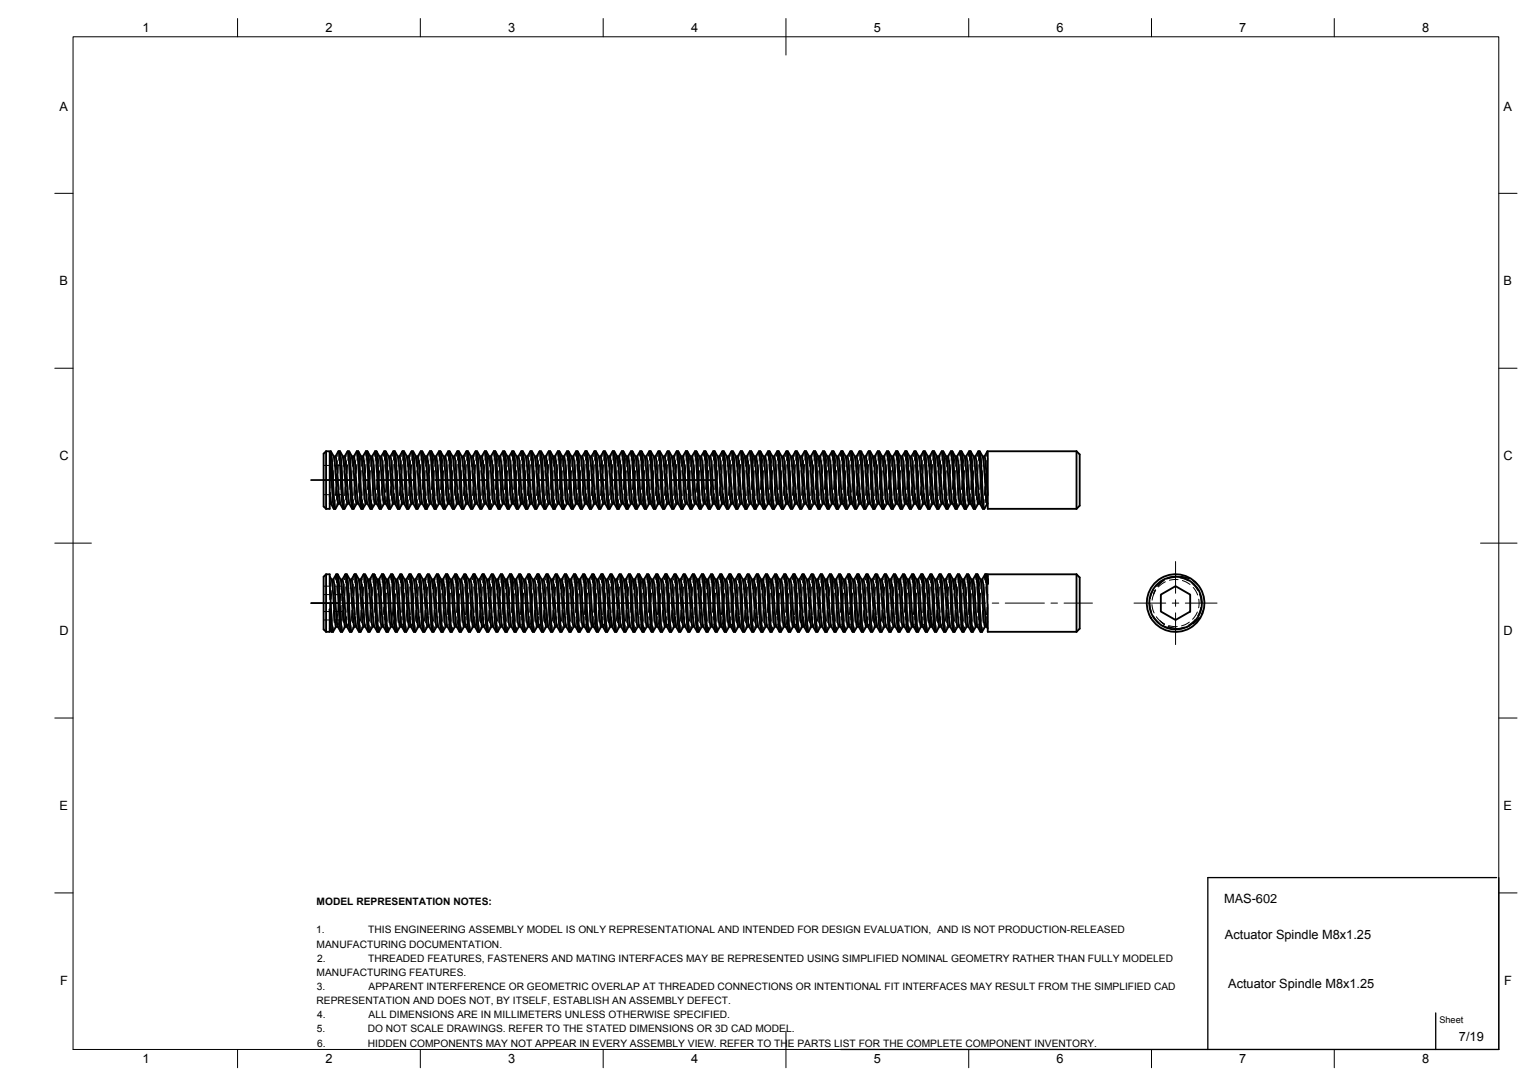
ISO-10303-21;
HEADER;
/* Generated by software containing ST-Developer
 * from STEP Tools, Inc. (www.steptools.com) 
 */

FILE_DESCRIPTION(
/* description */ (''),
/* implementation_level */ '2;1');

FILE_NAME(
/* name */ 'Actuator Spindle M8x1.25.step',
/* time_stamp */ '2026-10-15T14:42:47-07:00',
/* author */ (''),
/* organization */ (''),
/* preprocessor_version */ 'ST-DEVELOPER v20.2',
/* originating_system */ 'Autodesk Translation Framework v15.15.0.0',
/* authorisation */ '');

FILE_SCHEMA (('AUTOMOTIVE_DESIGN { 1 0 10303 214 3 1 1 }'));
ENDSEC;

DATA;
#10=MECHANICAL_DESIGN_GEOMETRIC_PRESENTATION_REPRESENTATION('',(#238),#85789);
#163=CONICAL_SURFACE('',#10500,0.375,0.785398163397451);
#164=CONICAL_SURFACE('',#10501,0.38,0.785398163397437);
#202=SHAPE_REPRESENTATION_RELATIONSHIP('SRR','None',#85867,#220);
#220=ADVANCED_BREP_SHAPE_REPRESENTATION('',(#256),#85775);
#238=STYLED_ITEM('',(#85966),#256);
#256=MANIFOLD_SOLID_BREP('Body1',#9885);
#381=B_SPLINE_SURFACE_WITH_KNOTS('',3,3,((#71919,#71920,#71921,#71922,#71923,
#71924,#71925,#71926,#71927,#71928,#71929,#71930,#71931,#71932,#71933,#71934,
#71935,#71936,#71937,#71938,#71939,#71940,#71941,#71942,#71943,#71944,#71945,
#71946,#71947,#71948,#71949,#71950,#71951,#71952,#71953,#71954,#71955,#71956,
#71957,#71958,#71959,#71960,#71961,#71962,#71963,#71964,#71965,#71966,#71967,
#71968,#71969,#71970,#71971,#71972,#71973,#71974,#71975,#71976,#71977,#71978,
#71979,#71980,#71981,#71982,#71983,#71984,#71985,#71986,#71987,#71988,#71989,
#71990,#71991,#71992,#71993,#71994,#71995,#71996,#71997,#71998,#71999,#72000,
#72001,#72002,#72003,#72004,#72005,#72006,#72007,#72008,#72009,#72010,#72011,
#72012,#72013,#72014,#72015,#72016,#72017,#72018,#72019,#72020,#72021,#72022,
#72023,#72024,#72025,#72026,#72027,#72028,#72029,#72030,#72031,#72032,#72033,
#72034,#72035,#72036,#72037,#72038,#72039,#72040,#72041,#72042,#72043,#72044,
#72045,#72046,#72047,#72048,#72049,#72050,#72051,#72052,#72053,#72054,#72055,
#72056,#72057,#72058,#72059,#72060,#72061,#72062,#72063,#72064,#72065,#72066,
#72067,#72068,#72069,#72070,#72071,#72072,#72073,#72074,#72075,#72076,#72077,
#72078,#72079,#72080,#72081,#72082,#72083,#72084,#72085,#72086,#72087,#72088,
#72089,#72090,#72091,#72092,#72093,#72094,#72095,#72096,#72097,#72098,#72099,
#72100,#72101,#72102,#72103,#72104,#72105,#72106,#72107,#72108,#72109,#72110,
#72111,#72112,#72113,#72114,#72115,#72116,#72117,#72118,#72119,#72120,#72121,
#72122,#72123,#72124,#72125,#72126,#72127,#72128,#72129,#72130,#72131,#72132,
#72133,#72134,#72135,#72136,#72137,#72138,#72139,#72140,#72141,#72142,#72143,
#72144,#72145,#72146,#72147,#72148,#72149,#72150,#72151,#72152,#72153,#72154,
#72155,#72156,#72157,#72158,#72159,#72160,#72161,#72162,#72163,#72164,#72165,
#72166,#72167,#72168,#72169,#72170,#72171,#72172,#72173,#72174,#72175,#72176,
#72177,#72178,#72179,#72180,#72181,#72182,#72183,#72184,#72185,#72186,#72187,
#72188,#72189,#72190,#72191,#72192,#72193,#72194,#72195,#72196,#72197,#72198,
#72199,#72200,#72201,#72202,#72203,#72204,#72205,#72206,#72207,#72208,#72209,
#72210,#72211,#72212,#72213,#72214,#72215,#72216,#72217,#72218,#72219,#72220,
#72221,#72222,#72223,#72224,#72225,#72226,#72227,#72228,#72229,#72230,#72231,
#72232,#72233,#72234,#72235,#72236,#72237,#72238,#72239,#72240,#72241,#72242,
#72243,#72244,#72245,#72246,#72247,#72248,#72249,#72250,#72251,#72252,#72253,
#72254,#72255,#72256,#72257,#72258,#72259,#72260,#72261,#72262,#72263,#72264,
#72265,#72266,#72267,#72268,#72269,#72270,#72271,#72272,#72273,#72274,#72275,
#72276,#72277,#72278,#72279,#72280,#72281,#72282,#72283,#72284,#72285,#72286,
#72287,#72288,#72289,#72290,#72291,#72292,#72293,#72294,#72295,#72296,#72297,
#72298,#72299,#72300,#72301,#72302,#72303,#72304,#72305,#72306,#72307,#72308,
#72309,#72310,#72311,#72312,#72313,#72314,#72315,#72316,#72317,#72318,#72319,
#72320,#72321,#72322,#72323,#72324,#72325,#72326,#72327,#72328,#72329,#72330,
#72331,#72332,#72333,#72334,#72335,#72336,#72337,#72338,#72339,#72340,#72341,
#72342,#72343,#72344,#72345,#72346,#72347,#72348,#72349,#72350,#72351,#72352,
#72353,#72354,#72355,#72356,#72357,#72358,#72359,#72360,#72361,#72362,#72363,
#72364,#72365,#72366,#72367,#72368,#72369,#72370,#72371,#72372,#72373,#72374,
#72375,#72376),(#72377,#72378,#72379,#72380,#72381,#72382,#72383,#72384,
#72385,#72386,#72387,#72388,#72389,#72390,#72391,#72392,#72393,#72394,#72395,
#72396,#72397,#72398,#72399,#72400,#72401,#72402,#72403,#72404,#72405,#72406,
#72407,#72408,#72409,#72410,#72411,#72412,#72413,#72414,#72415,#72416,#72417,
#72418,#72419,#72420,#72421,#72422,#72423,#72424,#72425,#72426,#72427,#72428,
#72429,#72430,#72431,#72432,#72433,#72434,#72435,#72436,#72437,#72438,#72439,
#72440,#72441,#72442,#72443,#72444,#72445,#72446,#72447,#72448,#72449,#72450,
#72451,#72452,#72453,#72454,#72455,#72456,#72457,#72458,#72459,#72460,#72461,
#72462,#72463,#72464,#72465,#72466,#72467,#72468,#72469,#72470,#72471,#72472,
#72473,#72474,#72475,#72476,#72477,#72478,#72479,#72480,#72481,#72482,#72483,
#72484,#72485,#72486,#72487,#72488,#72489,#72490,#72491,#72492,#72493,#72494,
#72495,#72496,#72497,#72498,#72499,#72500,#72501,#72502,#72503,#72504,#72505,
#72506,#72507,#72508,#72509,#72510,#72511,#72512,#72513,#72514,#72515,#72516,
#72517,#72518,#72519,#72520,#72521,#72522,#72523,#72524,#72525,#72526,#72527,
#72528,#72529,#72530,#72531,#72532,#72533,#72534,#72535,#72536,#72537,#72538,
#72539,#72540,#72541,#72542,#72543,#72544,#72545,#72546,#72547,#72548,#72549,
#72550,#72551,#72552,#72553,#72554,#72555,#72556,#72557,#72558,#72559,#72560,
#72561,#72562,#72563,#72564,#72565,#72566,#72567,#72568,#72569,#72570,#72571,
#72572,#72573,#72574,#72575,#72576,#72577,#72578,#72579,#72580,#72581,#72582,
#72583,#72584,#72585,#72586,#72587,#72588,#72589,#72590,#72591,#72592,#72593,
#72594,#72595,#72596,#72597,#72598,#72599,#72600,#72601,#72602,#72603,#72604,
#72605,#72606,#72607,#72608,#72609,#72610,#72611,#72612,#72613,#72614,#72615,
#72616,#72617,#72618,#72619,#72620,#72621,#72622,#72623,#72624,#72625,#72626,
#72627,#72628,#72629,#72630,#72631,#72632,#72633,#72634,#72635,#72636,#72637,
#72638,#72639,#72640,#72641,#72642,#72643,#72644,#72645,#72646,#72647,#72648,
#72649,#72650,#72651,#72652,#72653,#72654,#72655,#72656,#72657,#72658,#72659,
#72660,#72661,#72662,#72663,#72664,#72665,#72666,#72667,#72668,#72669,#72670,
#72671,#72672,#72673,#72674,#72675,#72676,#72677,#72678,#72679,#72680,#72681,
#72682,#72683,#72684,#72685,#72686,#72687,#72688,#72689,#72690,#72691,#72692,
#72693,#72694,#72695,#72696,#72697,#72698,#72699,#72700,#72701,#72702,#72703,
#72704,#72705,#72706,#72707,#72708,#72709,#72710,#72711,#72712,#72713,#72714,
#72715,#72716,#72717,#72718,#72719,#72720,#72721,#72722,#72723,#72724,#72725,
#72726,#72727,#72728,#72729,#72730,#72731,#72732,#72733,#72734,#72735,#72736,
#72737,#72738,#72739,#72740,#72741,#72742,#72743,#72744,#72745,#72746,#72747,
#72748,#72749,#72750,#72751,#72752,#72753,#72754,#72755,#72756,#72757,#72758,
#72759,#72760,#72761,#72762,#72763,#72764,#72765,#72766,#72767,#72768,#72769,
#72770,#72771,#72772,#72773,#72774,#72775,#72776,#72777,#72778,#72779,#72780,
#72781,#72782,#72783,#72784,#72785,#72786,#72787,#72788,#72789,#72790,#72791,
#72792,#72793,#72794,#72795,#72796,#72797,#72798,#72799,#72800,#72801,#72802,
#72803,#72804,#72805,#72806,#72807,#72808,#72809,#72810,#72811,#72812,#72813,
#72814,#72815,#72816,#72817,#72818,#72819,#72820,#72821,#72822,#72823,#72824,
#72825,#72826,#72827,#72828,#72829,#72830,#72831,#72832,#72833,#72834),
(#72835,#72836,#72837,#72838,#72839,#72840,#72841,#72842,#72843,#72844,
#72845,#72846,#72847,#72848,#72849,#72850,#72851,#72852,#72853,#72854,#72855,
#72856,#72857,#72858,#72859,#72860,#72861,#72862,#72863,#72864,#72865,#72866,
#72867,#72868,#72869,#72870,#72871,#72872,#72873,#72874,#72875,#72876,#72877,
#72878,#72879,#72880,#72881,#72882,#72883,#72884,#72885,#72886,#72887,#72888,
#72889,#72890,#72891,#72892,#72893,#72894,#72895,#72896,#72897,#72898,#72899,
#72900,#72901,#72902,#72903,#72904,#72905,#72906,#72907,#72908,#72909,#72910,
#72911,#72912,#72913,#72914,#72915,#72916,#72917,#72918,#72919,#72920,#72921,
#72922,#72923,#72924,#72925,#72926,#72927,#72928,#72929,#72930,#72931,#72932,
#72933,#72934,#72935,#72936,#72937,#72938,#72939,#72940,#72941,#72942,#72943,
#72944,#72945,#72946,#72947,#72948,#72949,#72950,#72951,#72952,#72953,#72954,
#72955,#72956,#72957,#72958,#72959,#72960,#72961,#72962,#72963,#72964,#72965,
#72966,#72967,#72968,#72969,#72970,#72971,#72972,#72973,#72974,#72975,#72976,
#72977,#72978,#72979,#72980,#72981,#72982,#72983,#72984,#72985,#72986,#72987,
#72988,#72989,#72990,#72991,#72992,#72993,#72994,#72995,#72996,#72997,#72998,
#72999,#73000,#73001,#73002,#73003,#73004,#73005,#73006,#73007,#73008,#73009,
#73010,#73011,#73012,#73013,#73014,#73015,#73016,#73017,#73018,#73019,#73020,
#73021,#73022,#73023,#73024,#73025,#73026,#73027,#73028,#73029,#73030,#73031,
#73032,#73033,#73034,#73035,#73036,#73037,#73038,#73039,#73040,#73041,#73042,
#73043,#73044,#73045,#73046,#73047,#73048,#73049,#73050,#73051,#73052,#73053,
#73054,#73055,#73056,#73057,#73058,#73059,#73060,#73061,#73062,#73063,#73064,
#73065,#73066,#73067,#73068,#73069,#73070,#73071,#73072,#73073,#73074,#73075,
#73076,#73077,#73078,#73079,#73080,#73081,#73082,#73083,#73084,#73085,#73086,
#73087,#73088,#73089,#73090,#73091,#73092,#73093,#73094,#73095,#73096,#73097,
#73098,#73099,#73100,#73101,#73102,#73103,#73104,#73105,#73106,#73107,#73108,
#73109,#73110,#73111,#73112,#73113,#73114,#73115,#73116,#73117,#73118,#73119,
#73120,#73121,#73122,#73123,#73124,#73125,#73126,#73127,#73128,#73129,#73130,
#73131,#73132,#73133,#73134,#73135,#73136,#73137,#73138,#73139,#73140,#73141,
#73142,#73143,#73144,#73145,#73146,#73147,#73148,#73149,#73150,#73151,#73152,
#73153,#73154,#73155,#73156,#73157,#73158,#73159,#73160,#73161,#73162,#73163,
#73164,#73165,#73166,#73167,#73168,#73169,#73170,#73171,#73172,#73173,#73174,
#73175,#73176,#73177,#73178,#73179,#73180,#73181,#73182,#73183,#73184,#73185,
#73186,#73187,#73188,#73189,#73190,#73191,#73192,#73193,#73194,#73195,#73196,
#73197,#73198,#73199,#73200,#73201,#73202,#73203,#73204,#73205,#73206,#73207,
#73208,#73209,#73210,#73211,#73212,#73213,#73214,#73215,#73216,#73217,#73218,
#73219,#73220,#73221,#73222,#73223,#73224,#73225,#73226,#73227,#73228,#73229,
#73230,#73231,#73232,#73233,#73234,#73235,#73236,#73237,#73238,#73239,#73240,
#73241,#73242,#73243,#73244,#73245,#73246,#73247,#73248,#73249,#73250,#73251,
#73252,#73253,#73254,#73255,#73256,#73257,#73258,#73259,#73260,#73261,#73262,
#73263,#73264,#73265,#73266,#73267,#73268,#73269,#73270,#73271,#73272,#73273,
#73274,#73275,#73276,#73277,#73278,#73279,#73280,#73281,#73282,#73283,#73284,
#73285,#73286,#73287,#73288,#73289,#73290,#73291,#73292),(#73293,#73294,
#73295,#73296,#73297,#73298,#73299,#73300,#73301,#73302,#73303,#73304,#73305,
#73306,#73307,#73308,#73309,#73310,#73311,#73312,#73313,#73314,#73315,#73316,
#73317,#73318,#73319,#73320,#73321,#73322,#73323,#73324,#73325,#73326,#73327,
#73328,#73329,#73330,#73331,#73332,#73333,#73334,#73335,#73336,#73337,#73338,
#73339,#73340,#73341,#73342,#73343,#73344,#73345,#73346,#73347,#73348,#73349,
#73350,#73351,#73352,#73353,#73354,#73355,#73356,#73357,#73358,#73359,#73360,
#73361,#73362,#73363,#73364,#73365,#73366,#73367,#73368,#73369,#73370,#73371,
#73372,#73373,#73374,#73375,#73376,#73377,#73378,#73379,#73380,#73381,#73382,
#73383,#73384,#73385,#73386,#73387,#73388,#73389,#73390,#73391,#73392,#73393,
#73394,#73395,#73396,#73397,#73398,#73399,#73400,#73401,#73402,#73403,#73404,
#73405,#73406,#73407,#73408,#73409,#73410,#73411,#73412,#73413,#73414,#73415,
#73416,#73417,#73418,#73419,#73420,#73421,#73422,#73423,#73424,#73425,#73426,
#73427,#73428,#73429,#73430,#73431,#73432,#73433,#73434,#73435,#73436,#73437,
#73438,#73439,#73440,#73441,#73442,#73443,#73444,#73445,#73446,#73447,#73448,
#73449,#73450,#73451,#73452,#73453,#73454,#73455,#73456,#73457,#73458,#73459,
#73460,#73461,#73462,#73463,#73464,#73465,#73466,#73467,#73468,#73469,#73470,
#73471,#73472,#73473,#73474,#73475,#73476,#73477,#73478,#73479,#73480,#73481,
#73482,#73483,#73484,#73485,#73486,#73487,#73488,#73489,#73490,#73491,#73492,
#73493,#73494,#73495,#73496,#73497,#73498,#73499,#73500,#73501,#73502,#73503,
#73504,#73505,#73506,#73507,#73508,#73509,#73510,#73511,#73512,#73513,#73514,
#73515,#73516,#73517,#73518,#73519,#73520,#73521,#73522,#73523,#73524,#73525,
#73526,#73527,#73528,#73529,#73530,#73531,#73532,#73533,#73534,#73535,#73536,
#73537,#73538,#73539,#73540,#73541,#73542,#73543,#73544,#73545,#73546,#73547,
#73548,#73549,#73550,#73551,#73552,#73553,#73554,#73555,#73556,#73557,#73558,
#73559,#73560,#73561,#73562,#73563,#73564,#73565,#73566,#73567,#73568,#73569,
#73570,#73571,#73572,#73573,#73574,#73575,#73576,#73577,#73578,#73579,#73580,
#73581,#73582,#73583,#73584,#73585,#73586,#73587,#73588,#73589,#73590,#73591,
#73592,#73593,#73594,#73595,#73596,#73597,#73598,#73599,#73600,#73601,#73602,
#73603,#73604,#73605,#73606,#73607,#73608,#73609,#73610,#73611,#73612,#73613,
#73614,#73615,#73616,#73617,#73618,#73619,#73620,#73621,#73622,#73623,#73624,
#73625,#73626,#73627,#73628,#73629,#73630,#73631,#73632,#73633,#73634,#73635,
#73636,#73637,#73638,#73639,#73640,#73641,#73642,#73643,#73644,#73645,#73646,
#73647,#73648,#73649,#73650,#73651,#73652,#73653,#73654,#73655,#73656,#73657,
#73658,#73659,#73660,#73661,#73662,#73663,#73664,#73665,#73666,#73667,#73668,
#73669,#73670,#73671,#73672,#73673,#73674,#73675,#73676,#73677,#73678,#73679,
#73680,#73681,#73682,#73683,#73684,#73685,#73686,#73687,#73688,#73689,#73690,
#73691,#73692,#73693,#73694,#73695,#73696,#73697,#73698,#73699,#73700,#73701,
#73702,#73703,#73704,#73705,#73706,#73707,#73708,#73709,#73710,#73711,#73712,
#73713,#73714,#73715,#73716,#73717,#73718,#73719,#73720,#73721,#73722,#73723,
#73724,#73725,#73726,#73727,#73728,#73729,#73730,#73731,#73732,#73733,#73734,
#73735,#73736,#73737,#73738,#73739,#73740,#73741,#73742,#73743,#73744,#73745,
#73746,#73747,#73748,#73749,#73750)),.UNSPECIFIED.,.F.,.F.,.F.,(4,4),(4,
1,1,1,1,1,1,1,1,1,1,1,1,1,1,1,1,1,1,1,1,1,1,1,1,1,1,1,1,1,1,1,1,1,1,1,1,
1,1,1,1,1,1,1,1,1,1,1,1,1,1,1,1,1,1,1,1,1,1,1,1,1,1,1,1,1,1,1,1,1,1,1,1,
1,1,1,1,1,1,1,1,1,1,1,1,1,1,1,1,1,1,1,1,1,1,1,1,1,1,1,1,1,1,1,1,1,1,1,1,
1,1,1,1,1,1,1,1,1,1,1,1,1,1,1,1,1,1,1,1,1,1,1,1,1,1,1,1,1,1,1,1,1,1,1,1,
1,1,1,1,1,1,1,1,1,1,1,1,1,1,1,1,1,1,1,1,1,1,1,1,1,1,1,1,1,1,1,1,1,1,1,1,
1,1,1,1,1,1,1,1,1,1,1,1,1,1,1,1,1,1,1,1,1,1,1,1,1,1,1,1,1,1,1,1,1,1,1,1,
1,1,1,1,1,1,1,1,1,1,1,1,1,1,1,1,1,1,1,1,1,1,1,1,1,1,1,1,1,1,1,1,1,1,1,1,
1,1,1,1,1,1,1,1,1,1,1,1,1,1,1,1,1,1,1,1,1,1,1,1,1,1,1,1,1,1,1,1,1,1,1,1,
1,1,1,1,1,1,1,1,1,1,1,1,1,1,1,1,1,1,1,1,1,1,1,1,1,1,1,1,1,1,1,1,1,1,1,1,
1,1,1,1,1,1,1,1,1,1,1,1,1,1,1,1,1,1,1,1,1,1,1,1,1,1,1,1,1,1,1,1,1,1,1,1,
1,1,1,1,1,1,1,1,1,1,1,1,1,1,1,1,1,1,1,1,1,1,1,1,1,1,1,1,1,1,1,1,1,1,1,1,
1,1,1,1,1,1,1,1,1,1,1,1,1,1,1,1,1,1,1,1,1,1,1,1,1,1,1,1,1,1,1,1,1,1,1,1,
1,1,1,1,1,1,1,1,1,1,1,1,1,1,1,1,1,1,1,1,1,1,4),(-0.000668976878624835,0.0823370872655779),
(12.7582013990964,13.7569938028644,14.7557862066324,15.7545786104004,16.7533710141684,
17.7521634179365,18.7509558217045,19.7497482254725,20.7485406292405,21.7473330330085,
22.7461254367765,23.7449178405445,24.7437102443125,25.7425026480806,26.7412950518486,
27.7400874556166,28.7388798593846,29.7376722631526,30.7364646669206,31.7352570706886,
32.7340494744567,33.7328418782247,34.7316342819927,35.7304266857607,36.7292190895287,
37.7280114932967,38.7268038970647,39.7255963008328,40.7243887046008,41.7231811083688,
42.7219735121368,43.7207659159048,44.7195583196728,45.7183507234408,46.7171431272089,
47.7159355309769,48.7147279347449,49.7135203385129,50.7123127422809,51.7111051460489,
52.7098975498169,53.708689953585,54.707482357353,55.706274761121,56.705067164889,
57.703859568657,58.702651972425,59.701444376193,60.700236779961,61.6990291837291,
62.6978215874971,63.6966139912651,64.6954063950331,65.6941987988011,66.6929912025691,
67.6917836063371,68.6905760101052,69.6893684138732,70.6881608176412,71.6869532214092,
72.6857456251772,73.6845380289452,74.6833304327132,75.6821228364813,76.6809152402493,
77.6797076440173,78.6785000477853,79.6772924515533,80.6760848553213,81.6748772590893,
82.6736696628573,83.6724620666254,84.6712544703934,85.6700468741614,86.6688392779294,
87.6676316816974,88.6664240854654,89.6652164892334,90.6640088930015,91.6628012967695,
92.6615937005375,93.6603861043055,94.6591785080735,95.6579709118415,96.6567633156095,
97.6555557193776,98.6543481231456,99.6531405269136,100.651932930682,101.65072533445,
102.649517738218,103.648310141986,104.647102545754,105.645894949522,106.64468735329,
107.643479757058,108.642272160826,109.641064564594,110.639856968362,111.63864937213,
112.637441775898,113.636234179666,114.635026583434,115.633818987202,116.63261139097,
117.631403794738,118.630196198506,119.628988602274,120.627781006042,121.62657340981,
122.625365813578,123.624158217346,124.622950621114,125.621743024882,126.62053542865,
127.619327832418,128.618120236186,129.616912639954,130.615705043722,131.61449744749,
132.613289851258,133.612082255026,134.610874658794,135.609667062562,136.60845946633,
137.607251870098,138.606044273866,139.604836677634,140.603629081402,141.60242148517,
142.601213888938,143.600006292706,144.598798696474,145.597591100242,146.59638350401,
147.595175907778,148.593968311546,149.592760715314,150.591553119082,151.59034552285,
152.589137926618,153.587930330386,154.586722734154,155.585515137922,156.58430754169,
157.583099945458,158.581892349226,159.580684752994,160.579477156762,161.57826956053,
162.577061964298,163.575854368066,164.574646771834,165.573439175602,166.572231579371,
167.571023983139,168.569816386907,169.568608790675,170.567401194443,171.566193598211,
172.564986001979,173.563778405747,174.562570809515,175.561363213283,176.560155617051,
177.558948020819,178.557740424587,179.556532828355,180.555325232123,181.554117635891,
182.552910039659,183.551702443427,184.550494847195,185.549287250963,186.548079654731,
187.546872058499,188.545664462267,189.544456866035,190.543249269803,191.542041673571,
192.540834077339,193.539626481107,194.538418884875,195.537211288643,196.536003692411,
197.534796096179,198.533588499947,199.532380903715,200.531173307483,201.529965711251,
202.528758115019,203.527550518787,204.526342922555,205.525135326323,206.523927730091,
207.522720133859,208.521512537627,209.520304941395,210.519097345163,211.517889748931,
212.516682152699,213.515474556467,214.514266960235,215.513059364003,216.511851767771,
217.510644171539,218.509436575307,219.508228979075,220.507021382843,221.505813786611,
222.504606190379,223.503398594147,224.502190997915,225.500983401683,226.499775805451,
227.498568209219,228.497360612987,229.496153016755,230.494945420523,231.493737824291,
232.492530228059,233.491322631827,234.490115035595,235.488907439363,236.487699843131,
237.486492246899,238.485284650667,239.484077054436,240.482869458204,241.481661861972,
242.48045426574,243.479246669508,244.478039073276,245.476831477044,246.475623880812,
247.47441628458,248.473208688348,249.472001092116,250.470793495884,251.469585899652,
252.46837830342,253.467170707188,254.465963110956,255.464755514724,256.463547918492,
257.46234032226,258.461132726028,259.459925129796,260.458717533564,261.457509937332,
262.4563023411,263.455094744868,264.453887148636,265.452679552404,266.451471956172,
267.45026435994,268.449056763708,269.447849167476,270.446641571244,271.445433975012,
272.44422637878,273.443018782548,274.441811186316,275.440603590084,276.439395993852,
277.43818839762,278.436980801388,279.435773205156,280.434565608924,281.433358012692,
282.43215041646,283.430942820228,284.429735223996,285.428527627764,286.427320031532,
287.4261124353,288.424904839068,289.423697242836,290.422489646604,291.421282050372,
292.42007445414,293.418866857908,294.417659261676,295.416451665444,296.415244069212,
297.41403647298,298.412828876748,299.411621280516,300.410413684284,301.409206088052,
302.40799849182,303.406790895588,304.405583299356,305.404375703124,306.403168106892,
307.40196051066,308.400752914428,309.399545318196,310.398337721964,311.397130125733,
312.395922529501,313.394714933269,314.393507337037,315.392299740805,316.391092144573,
317.389884548341,318.388676952109,319.387469355877,320.386261759645,321.385054163413,
322.383846567181,323.382638970949,324.381431374717,325.380223778485,326.379016182253,
327.377808586021,328.376600989789,329.375393393557,330.374185797325,331.372978201093,
332.371770604861,333.370563008629,334.369355412397,335.368147816165,336.366940219933,
337.365732623701,338.364525027469,339.363317431237,340.362109835005,341.360902238773,
342.359694642541,343.358487046309,344.357279450077,345.356071853845,346.354864257613,
347.353656661381,348.352449065149,349.351241468917,350.350033872685,351.348826276453,
352.347618680221,353.346411083989,354.345203487757,355.343995891525,356.342788295293,
357.341580699061,358.340373102829,359.339165506597,360.337957910365,361.336750314133,
362.335542717901,363.334335121669,364.333127525437,365.331919929205,366.330712332973,
367.329504736741,368.328297140509,369.327089544277,370.325881948045,371.324674351813,
372.323466755581,373.322259159349,374.321051563117,375.319843966885,376.318636370653,
377.317428774421,378.316221178189,379.315013581957,380.313805985725,381.312598389493,
382.311390793261,383.31018319703,384.308975600798,385.307768004566,386.306560408334,
387.305352812102,388.30414521587,389.302937619638,390.301730023406,391.300522427174,
392.299314830942,393.29810723471,394.296899638478,395.295692042246,396.294484446014,
397.293276849782,398.29206925355,399.290861657318,400.289654061086,401.288446464854,
402.287238868622,403.28603127239,404.284823676158,405.283616079926,406.282408483694,
407.281200887462,408.27999329123,409.278785694998,410.277578098766,411.276370502534,
412.275162906302,413.27395531007,414.272747713838,415.271540117606,416.270332521374,
417.269124925142,418.26791732891,419.266709732678,420.265502136446,421.264294540214,
422.263086943982,423.26187934775,424.260671751518,425.259464155286,426.258256559054,
427.257048962822,428.25584136659,429.254633770358,430.253426174126,431.252218577894,
432.251010981662,433.24980338543,434.248595789198,435.247388192966,436.246180596734,
437.244973000502,438.24376540427,439.242557808038,440.241350211806,441.240142615574,
442.238935019342,443.23772742311,444.236519826878,445.235312230646,446.234104634414,
447.232897038182,448.23168944195,449.230481845718,450.229274249486,451.228066653254,
452.226859057022,453.22565146079,454.224443864559,455.223236268327,456.222028672094,
457.220821075863,458.219613479631,459.218405883399,460.217198287167,461.215990690935,
462.214783094703,463.213575498471,464.212367902239,465.211160306007,466.209952709775,
467.209414090422),.UNSPECIFIED.);
#382=B_SPLINE_SURFACE_WITH_KNOTS('',3,3,((#73883,#73884,#73885,#73886,#73887,
#73888,#73889,#73890,#73891,#73892,#73893,#73894,#73895,#73896,#73897,#73898,
#73899,#73900,#73901,#73902,#73903,#73904,#73905,#73906,#73907,#73908,#73909,
#73910,#73911,#73912,#73913,#73914,#73915,#73916,#73917,#73918,#73919,#73920,
#73921,#73922,#73923,#73924,#73925,#73926,#73927,#73928,#73929,#73930,#73931,
#73932,#73933,#73934,#73935,#73936,#73937,#73938,#73939,#73940,#73941,#73942,
#73943,#73944,#73945,#73946,#73947,#73948,#73949,#73950,#73951,#73952,#73953,
#73954,#73955,#73956,#73957,#73958,#73959,#73960,#73961,#73962,#73963,#73964,
#73965,#73966,#73967,#73968,#73969,#73970,#73971,#73972,#73973,#73974,#73975,
#73976,#73977,#73978,#73979,#73980,#73981,#73982,#73983,#73984,#73985,#73986,
#73987,#73988,#73989,#73990,#73991,#73992,#73993,#73994,#73995,#73996,#73997,
#73998,#73999,#74000,#74001,#74002,#74003,#74004,#74005,#74006,#74007,#74008,
#74009,#74010,#74011,#74012,#74013,#74014,#74015,#74016,#74017,#74018,#74019,
#74020,#74021,#74022,#74023,#74024,#74025,#74026,#74027,#74028,#74029,#74030,
#74031,#74032,#74033,#74034,#74035,#74036,#74037,#74038,#74039,#74040,#74041,
#74042,#74043,#74044,#74045,#74046,#74047,#74048,#74049,#74050,#74051,#74052,
#74053,#74054,#74055,#74056,#74057,#74058,#74059,#74060,#74061,#74062,#74063,
#74064,#74065,#74066,#74067,#74068,#74069,#74070,#74071,#74072,#74073,#74074,
#74075,#74076,#74077,#74078,#74079,#74080,#74081,#74082,#74083,#74084,#74085,
#74086,#74087,#74088,#74089,#74090,#74091,#74092,#74093,#74094,#74095,#74096,
#74097,#74098,#74099,#74100,#74101,#74102,#74103,#74104,#74105,#74106,#74107,
#74108,#74109,#74110,#74111,#74112,#74113,#74114,#74115,#74116,#74117,#74118,
#74119,#74120,#74121,#74122,#74123,#74124,#74125,#74126,#74127,#74128,#74129,
#74130,#74131,#74132,#74133,#74134,#74135,#74136,#74137,#74138,#74139,#74140,
#74141,#74142,#74143,#74144,#74145,#74146,#74147,#74148,#74149,#74150,#74151,
#74152,#74153,#74154,#74155,#74156,#74157,#74158,#74159,#74160,#74161,#74162,
#74163,#74164,#74165,#74166,#74167,#74168,#74169,#74170,#74171,#74172,#74173,
#74174,#74175,#74176,#74177,#74178,#74179,#74180,#74181,#74182,#74183,#74184,
#74185,#74186,#74187,#74188,#74189,#74190,#74191,#74192,#74193,#74194,#74195,
#74196,#74197,#74198,#74199,#74200,#74201,#74202,#74203,#74204,#74205,#74206,
#74207,#74208,#74209,#74210,#74211,#74212,#74213,#74214,#74215,#74216,#74217,
#74218,#74219,#74220,#74221,#74222,#74223,#74224,#74225,#74226,#74227,#74228,
#74229,#74230,#74231,#74232,#74233,#74234,#74235,#74236,#74237,#74238,#74239,
#74240,#74241,#74242,#74243,#74244,#74245,#74246,#74247,#74248,#74249,#74250,
#74251,#74252,#74253,#74254,#74255,#74256,#74257,#74258,#74259,#74260,#74261,
#74262,#74263,#74264,#74265,#74266,#74267,#74268,#74269,#74270,#74271,#74272,
#74273,#74274,#74275,#74276,#74277,#74278,#74279,#74280,#74281,#74282,#74283,
#74284,#74285,#74286,#74287,#74288,#74289,#74290,#74291,#74292,#74293,#74294,
#74295,#74296,#74297,#74298,#74299,#74300,#74301,#74302,#74303,#74304,#74305,
#74306,#74307,#74308,#74309,#74310,#74311,#74312,#74313,#74314,#74315,#74316,
#74317,#74318,#74319,#74320,#74321,#74322,#74323,#74324,#74325,#74326,#74327,
#74328,#74329,#74330,#74331,#74332,#74333,#74334,#74335,#74336,#74337,#74338,
#74339,#74340),(#74341,#74342,#74343,#74344,#74345,#74346,#74347,#74348,
#74349,#74350,#74351,#74352,#74353,#74354,#74355,#74356,#74357,#74358,#74359,
#74360,#74361,#74362,#74363,#74364,#74365,#74366,#74367,#74368,#74369,#74370,
#74371,#74372,#74373,#74374,#74375,#74376,#74377,#74378,#74379,#74380,#74381,
#74382,#74383,#74384,#74385,#74386,#74387,#74388,#74389,#74390,#74391,#74392,
#74393,#74394,#74395,#74396,#74397,#74398,#74399,#74400,#74401,#74402,#74403,
#74404,#74405,#74406,#74407,#74408,#74409,#74410,#74411,#74412,#74413,#74414,
#74415,#74416,#74417,#74418,#74419,#74420,#74421,#74422,#74423,#74424,#74425,
#74426,#74427,#74428,#74429,#74430,#74431,#74432,#74433,#74434,#74435,#74436,
#74437,#74438,#74439,#74440,#74441,#74442,#74443,#74444,#74445,#74446,#74447,
#74448,#74449,#74450,#74451,#74452,#74453,#74454,#74455,#74456,#74457,#74458,
#74459,#74460,#74461,#74462,#74463,#74464,#74465,#74466,#74467,#74468,#74469,
#74470,#74471,#74472,#74473,#74474,#74475,#74476,#74477,#74478,#74479,#74480,
#74481,#74482,#74483,#74484,#74485,#74486,#74487,#74488,#74489,#74490,#74491,
#74492,#74493,#74494,#74495,#74496,#74497,#74498,#74499,#74500,#74501,#74502,
#74503,#74504,#74505,#74506,#74507,#74508,#74509,#74510,#74511,#74512,#74513,
#74514,#74515,#74516,#74517,#74518,#74519,#74520,#74521,#74522,#74523,#74524,
#74525,#74526,#74527,#74528,#74529,#74530,#74531,#74532,#74533,#74534,#74535,
#74536,#74537,#74538,#74539,#74540,#74541,#74542,#74543,#74544,#74545,#74546,
#74547,#74548,#74549,#74550,#74551,#74552,#74553,#74554,#74555,#74556,#74557,
#74558,#74559,#74560,#74561,#74562,#74563,#74564,#74565,#74566,#74567,#74568,
#74569,#74570,#74571,#74572,#74573,#74574,#74575,#74576,#74577,#74578,#74579,
#74580,#74581,#74582,#74583,#74584,#74585,#74586,#74587,#74588,#74589,#74590,
#74591,#74592,#74593,#74594,#74595,#74596,#74597,#74598,#74599,#74600,#74601,
#74602,#74603,#74604,#74605,#74606,#74607,#74608,#74609,#74610,#74611,#74612,
#74613,#74614,#74615,#74616,#74617,#74618,#74619,#74620,#74621,#74622,#74623,
#74624,#74625,#74626,#74627,#74628,#74629,#74630,#74631,#74632,#74633,#74634,
#74635,#74636,#74637,#74638,#74639,#74640,#74641,#74642,#74643,#74644,#74645,
#74646,#74647,#74648,#74649,#74650,#74651,#74652,#74653,#74654,#74655,#74656,
#74657,#74658,#74659,#74660,#74661,#74662,#74663,#74664,#74665,#74666,#74667,
#74668,#74669,#74670,#74671,#74672,#74673,#74674,#74675,#74676,#74677,#74678,
#74679,#74680,#74681,#74682,#74683,#74684,#74685,#74686,#74687,#74688,#74689,
#74690,#74691,#74692,#74693,#74694,#74695,#74696,#74697,#74698,#74699,#74700,
#74701,#74702,#74703,#74704,#74705,#74706,#74707,#74708,#74709,#74710,#74711,
#74712,#74713,#74714,#74715,#74716,#74717,#74718,#74719,#74720,#74721,#74722,
#74723,#74724,#74725,#74726,#74727,#74728,#74729,#74730,#74731,#74732,#74733,
#74734,#74735,#74736,#74737,#74738,#74739,#74740,#74741,#74742,#74743,#74744,
#74745,#74746,#74747,#74748,#74749,#74750,#74751,#74752,#74753,#74754,#74755,
#74756,#74757,#74758,#74759,#74760,#74761,#74762,#74763,#74764,#74765,#74766,
#74767,#74768,#74769,#74770,#74771,#74772,#74773,#74774,#74775,#74776,#74777,
#74778,#74779,#74780,#74781,#74782,#74783,#74784,#74785,#74786,#74787,#74788,
#74789,#74790,#74791,#74792,#74793,#74794,#74795,#74796,#74797,#74798),
(#74799,#74800,#74801,#74802,#74803,#74804,#74805,#74806,#74807,#74808,
#74809,#74810,#74811,#74812,#74813,#74814,#74815,#74816,#74817,#74818,#74819,
#74820,#74821,#74822,#74823,#74824,#74825,#74826,#74827,#74828,#74829,#74830,
#74831,#74832,#74833,#74834,#74835,#74836,#74837,#74838,#74839,#74840,#74841,
#74842,#74843,#74844,#74845,#74846,#74847,#74848,#74849,#74850,#74851,#74852,
#74853,#74854,#74855,#74856,#74857,#74858,#74859,#74860,#74861,#74862,#74863,
#74864,#74865,#74866,#74867,#74868,#74869,#74870,#74871,#74872,#74873,#74874,
#74875,#74876,#74877,#74878,#74879,#74880,#74881,#74882,#74883,#74884,#74885,
#74886,#74887,#74888,#74889,#74890,#74891,#74892,#74893,#74894,#74895,#74896,
#74897,#74898,#74899,#74900,#74901,#74902,#74903,#74904,#74905,#74906,#74907,
#74908,#74909,#74910,#74911,#74912,#74913,#74914,#74915,#74916,#74917,#74918,
#74919,#74920,#74921,#74922,#74923,#74924,#74925,#74926,#74927,#74928,#74929,
#74930,#74931,#74932,#74933,#74934,#74935,#74936,#74937,#74938,#74939,#74940,
#74941,#74942,#74943,#74944,#74945,#74946,#74947,#74948,#74949,#74950,#74951,
#74952,#74953,#74954,#74955,#74956,#74957,#74958,#74959,#74960,#74961,#74962,
#74963,#74964,#74965,#74966,#74967,#74968,#74969,#74970,#74971,#74972,#74973,
#74974,#74975,#74976,#74977,#74978,#74979,#74980,#74981,#74982,#74983,#74984,
#74985,#74986,#74987,#74988,#74989,#74990,#74991,#74992,#74993,#74994,#74995,
#74996,#74997,#74998,#74999,#75000,#75001,#75002,#75003,#75004,#75005,#75006,
#75007,#75008,#75009,#75010,#75011,#75012,#75013,#75014,#75015,#75016,#75017,
#75018,#75019,#75020,#75021,#75022,#75023,#75024,#75025,#75026,#75027,#75028,
#75029,#75030,#75031,#75032,#75033,#75034,#75035,#75036,#75037,#75038,#75039,
#75040,#75041,#75042,#75043,#75044,#75045,#75046,#75047,#75048,#75049,#75050,
#75051,#75052,#75053,#75054,#75055,#75056,#75057,#75058,#75059,#75060,#75061,
#75062,#75063,#75064,#75065,#75066,#75067,#75068,#75069,#75070,#75071,#75072,
#75073,#75074,#75075,#75076,#75077,#75078,#75079,#75080,#75081,#75082,#75083,
#75084,#75085,#75086,#75087,#75088,#75089,#75090,#75091,#75092,#75093,#75094,
#75095,#75096,#75097,#75098,#75099,#75100,#75101,#75102,#75103,#75104,#75105,
#75106,#75107,#75108,#75109,#75110,#75111,#75112,#75113,#75114,#75115,#75116,
#75117,#75118,#75119,#75120,#75121,#75122,#75123,#75124,#75125,#75126,#75127,
#75128,#75129,#75130,#75131,#75132,#75133,#75134,#75135,#75136,#75137,#75138,
#75139,#75140,#75141,#75142,#75143,#75144,#75145,#75146,#75147,#75148,#75149,
#75150,#75151,#75152,#75153,#75154,#75155,#75156,#75157,#75158,#75159,#75160,
#75161,#75162,#75163,#75164,#75165,#75166,#75167,#75168,#75169,#75170,#75171,
#75172,#75173,#75174,#75175,#75176,#75177,#75178,#75179,#75180,#75181,#75182,
#75183,#75184,#75185,#75186,#75187,#75188,#75189,#75190,#75191,#75192,#75193,
#75194,#75195,#75196,#75197,#75198,#75199,#75200,#75201,#75202,#75203,#75204,
#75205,#75206,#75207,#75208,#75209,#75210,#75211,#75212,#75213,#75214,#75215,
#75216,#75217,#75218,#75219,#75220,#75221,#75222,#75223,#75224,#75225,#75226,
#75227,#75228,#75229,#75230,#75231,#75232,#75233,#75234,#75235,#75236,#75237,
#75238,#75239,#75240,#75241,#75242,#75243,#75244,#75245,#75246,#75247,#75248,
#75249,#75250,#75251,#75252,#75253,#75254,#75255,#75256),(#75257,#75258,
#75259,#75260,#75261,#75262,#75263,#75264,#75265,#75266,#75267,#75268,#75269,
#75270,#75271,#75272,#75273,#75274,#75275,#75276,#75277,#75278,#75279,#75280,
#75281,#75282,#75283,#75284,#75285,#75286,#75287,#75288,#75289,#75290,#75291,
#75292,#75293,#75294,#75295,#75296,#75297,#75298,#75299,#75300,#75301,#75302,
#75303,#75304,#75305,#75306,#75307,#75308,#75309,#75310,#75311,#75312,#75313,
#75314,#75315,#75316,#75317,#75318,#75319,#75320,#75321,#75322,#75323,#75324,
#75325,#75326,#75327,#75328,#75329,#75330,#75331,#75332,#75333,#75334,#75335,
#75336,#75337,#75338,#75339,#75340,#75341,#75342,#75343,#75344,#75345,#75346,
#75347,#75348,#75349,#75350,#75351,#75352,#75353,#75354,#75355,#75356,#75357,
#75358,#75359,#75360,#75361,#75362,#75363,#75364,#75365,#75366,#75367,#75368,
#75369,#75370,#75371,#75372,#75373,#75374,#75375,#75376,#75377,#75378,#75379,
#75380,#75381,#75382,#75383,#75384,#75385,#75386,#75387,#75388,#75389,#75390,
#75391,#75392,#75393,#75394,#75395,#75396,#75397,#75398,#75399,#75400,#75401,
#75402,#75403,#75404,#75405,#75406,#75407,#75408,#75409,#75410,#75411,#75412,
#75413,#75414,#75415,#75416,#75417,#75418,#75419,#75420,#75421,#75422,#75423,
#75424,#75425,#75426,#75427,#75428,#75429,#75430,#75431,#75432,#75433,#75434,
#75435,#75436,#75437,#75438,#75439,#75440,#75441,#75442,#75443,#75444,#75445,
#75446,#75447,#75448,#75449,#75450,#75451,#75452,#75453,#75454,#75455,#75456,
#75457,#75458,#75459,#75460,#75461,#75462,#75463,#75464,#75465,#75466,#75467,
#75468,#75469,#75470,#75471,#75472,#75473,#75474,#75475,#75476,#75477,#75478,
#75479,#75480,#75481,#75482,#75483,#75484,#75485,#75486,#75487,#75488,#75489,
#75490,#75491,#75492,#75493,#75494,#75495,#75496,#75497,#75498,#75499,#75500,
#75501,#75502,#75503,#75504,#75505,#75506,#75507,#75508,#75509,#75510,#75511,
#75512,#75513,#75514,#75515,#75516,#75517,#75518,#75519,#75520,#75521,#75522,
#75523,#75524,#75525,#75526,#75527,#75528,#75529,#75530,#75531,#75532,#75533,
#75534,#75535,#75536,#75537,#75538,#75539,#75540,#75541,#75542,#75543,#75544,
#75545,#75546,#75547,#75548,#75549,#75550,#75551,#75552,#75553,#75554,#75555,
#75556,#75557,#75558,#75559,#75560,#75561,#75562,#75563,#75564,#75565,#75566,
#75567,#75568,#75569,#75570,#75571,#75572,#75573,#75574,#75575,#75576,#75577,
#75578,#75579,#75580,#75581,#75582,#75583,#75584,#75585,#75586,#75587,#75588,
#75589,#75590,#75591,#75592,#75593,#75594,#75595,#75596,#75597,#75598,#75599,
#75600,#75601,#75602,#75603,#75604,#75605,#75606,#75607,#75608,#75609,#75610,
#75611,#75612,#75613,#75614,#75615,#75616,#75617,#75618,#75619,#75620,#75621,
#75622,#75623,#75624,#75625,#75626,#75627,#75628,#75629,#75630,#75631,#75632,
#75633,#75634,#75635,#75636,#75637,#75638,#75639,#75640,#75641,#75642,#75643,
#75644,#75645,#75646,#75647,#75648,#75649,#75650,#75651,#75652,#75653,#75654,
#75655,#75656,#75657,#75658,#75659,#75660,#75661,#75662,#75663,#75664,#75665,
#75666,#75667,#75668,#75669,#75670,#75671,#75672,#75673,#75674,#75675,#75676,
#75677,#75678,#75679,#75680,#75681,#75682,#75683,#75684,#75685,#75686,#75687,
#75688,#75689,#75690,#75691,#75692,#75693,#75694,#75695,#75696,#75697,#75698,
#75699,#75700,#75701,#75702,#75703,#75704,#75705,#75706,#75707,#75708,#75709,
#75710,#75711,#75712,#75713,#75714)),.UNSPECIFIED.,.F.,.F.,.F.,(4,4),(4,
1,1,1,1,1,1,1,1,1,1,1,1,1,1,1,1,1,1,1,1,1,1,1,1,1,1,1,1,1,1,1,1,1,1,1,1,
1,1,1,1,1,1,1,1,1,1,1,1,1,1,1,1,1,1,1,1,1,1,1,1,1,1,1,1,1,1,1,1,1,1,1,1,
1,1,1,1,1,1,1,1,1,1,1,1,1,1,1,1,1,1,1,1,1,1,1,1,1,1,1,1,1,1,1,1,1,1,1,1,
1,1,1,1,1,1,1,1,1,1,1,1,1,1,1,1,1,1,1,1,1,1,1,1,1,1,1,1,1,1,1,1,1,1,1,1,
1,1,1,1,1,1,1,1,1,1,1,1,1,1,1,1,1,1,1,1,1,1,1,1,1,1,1,1,1,1,1,1,1,1,1,1,
1,1,1,1,1,1,1,1,1,1,1,1,1,1,1,1,1,1,1,1,1,1,1,1,1,1,1,1,1,1,1,1,1,1,1,1,
1,1,1,1,1,1,1,1,1,1,1,1,1,1,1,1,1,1,1,1,1,1,1,1,1,1,1,1,1,1,1,1,1,1,1,1,
1,1,1,1,1,1,1,1,1,1,1,1,1,1,1,1,1,1,1,1,1,1,1,1,1,1,1,1,1,1,1,1,1,1,1,1,
1,1,1,1,1,1,1,1,1,1,1,1,1,1,1,1,1,1,1,1,1,1,1,1,1,1,1,1,1,1,1,1,1,1,1,1,
1,1,1,1,1,1,1,1,1,1,1,1,1,1,1,1,1,1,1,1,1,1,1,1,1,1,1,1,1,1,1,1,1,1,1,1,
1,1,1,1,1,1,1,1,1,1,1,1,1,1,1,1,1,1,1,1,1,1,1,1,1,1,1,1,1,1,1,1,1,1,1,1,
1,1,1,1,1,1,1,1,1,1,1,1,1,1,1,1,1,1,1,1,1,1,1,1,1,1,1,1,1,1,1,1,1,1,1,1,
1,1,1,1,1,1,1,1,1,1,1,1,1,1,1,1,1,1,1,1,1,1,4),(-0.000353810282139617,0.0826815503419868),
(16.0580139323897,17.0574752807613,18.0562676845293,19.0550600882973,20.0538524920653,
21.0526448958333,22.0514372996014,23.0502297033694,24.0490221071374,25.0478145109054,
26.0466069146734,27.0453993184414,28.0441917222094,29.0429841259775,30.0417765297455,
31.0405689335135,32.0393613372815,33.0381537410495,34.0369461448175,35.0357385485855,
36.0345309523535,37.0333233561216,38.0321157598896,39.0309081636576,40.0297005674256,
41.0284929711936,42.0272853749616,43.0260777787296,44.0248701824977,45.0236625862657,
46.0224549900337,47.0212473938017,48.0200397975697,49.0188322013377,50.0176246051057,
51.0164170088737,52.0152094126418,53.0140018164098,54.0127942201778,55.0115866239458,
56.0103790277138,57.0091714314818,58.0079638352498,59.0067562390179,60.0055486427859,
61.0043410465539,62.0031334503219,63.0019258540899,64.0007182578579,64.9995106616259,
65.9983030653939,66.997095469162,67.99588787293,68.994680276698,69.993472680466,
70.992265084234,71.991057488002,72.98984989177,73.9886422955381,74.9874346993061,
75.9862271030741,76.9850195068421,77.9838119106101,78.9826043143781,79.9813967181461,
80.9801891219142,81.9789815256821,82.9777739294502,83.9765663332182,84.9753587369862,
85.9741511407542,86.9729435445222,87.9717359482902,88.9705283520582,89.9693207558263,
90.9681131595943,91.9669055633623,92.9656979671303,93.9644903708983,94.9632827746663,
95.9620751784343,96.9608675822024,97.9596599859704,98.9584523897384,99.9572447935064,
100.956037197274,101.954829601042,102.95362200481,103.952414408578,104.951206812346,
105.949999216114,106.948791619882,107.947584023651,108.946376427419,109.945168831187,
110.943961234955,111.942753638723,112.941546042491,113.940338446259,114.939130850027,
115.937923253795,116.936715657563,117.935508061331,118.934300465099,119.933092868867,
120.931885272635,121.930677676403,122.929470080171,123.928262483939,124.927054887707,
125.925847291475,126.924639695243,127.923432099011,128.922224502779,129.921016906547,
130.919809310315,131.918601714083,132.917394117851,133.916186521619,134.914978925387,
135.913771329155,136.912563732923,137.911356136691,138.910148540459,139.908940944227,
140.907733347995,141.906525751763,142.905318155531,143.904110559299,144.902902963067,
145.901695366835,146.900487770603,147.899280174371,148.898072578139,149.896864981907,
150.895657385675,151.894449789443,152.893242193211,153.892034596979,154.890827000747,
155.889619404515,156.888411808283,157.887204212051,158.885996615819,159.884789019587,
160.883581423355,161.882373827123,162.881166230891,163.879958634659,164.878751038427,
165.877543442195,166.876335845963,167.875128249731,168.873920653499,169.872713057267,
170.871505461035,171.870297864803,172.869090268571,173.867882672339,174.866675076107,
175.865467479875,176.864259883643,177.863052287411,178.861844691179,179.860637094947,
180.859429498715,181.858221902483,182.857014306252,183.85580671002,184.854599113788,
185.853391517556,186.852183921324,187.850976325092,188.84976872886,189.848561132628,
190.847353536396,191.846145940164,192.844938343932,193.8437307477,194.842523151468,
195.841315555236,196.840107959004,197.838900362772,198.83769276654,199.836485170308,
200.835277574076,201.834069977844,202.832862381612,203.83165478538,204.830447189148,
205.829239592916,206.828031996684,207.826824400452,208.82561680422,209.824409207988,
210.823201611756,211.821994015524,212.820786419292,213.81957882306,214.818371226828,
215.817163630596,216.815956034364,217.814748438132,218.8135408419,219.812333245668,
220.811125649436,221.809918053204,222.808710456972,223.80750286074,224.806295264508,
225.805087668276,226.803880072044,227.802672475812,228.80146487958,229.800257283348,
230.799049687116,231.797842090884,232.796634494652,233.79542689842,234.794219302188,
235.793011705956,236.791804109724,237.790596513492,238.78938891726,239.788181321028,
240.786973724796,241.785766128564,242.784558532332,243.7833509361,244.782143339868,
245.780935743636,246.779728147404,247.778520551172,248.77731295494,249.776105358708,
250.774897762476,251.773690166244,252.772482570012,253.77127497378,254.770067377548,
255.768859781316,256.767652185084,257.766444588852,258.76523699262,259.764029396389,
260.762821800157,261.761614203925,262.760406607693,263.759199011461,264.757991415229,
265.756783818997,266.755576222765,267.754368626533,268.753161030301,269.751953434069,
270.750745837837,271.749538241605,272.748330645373,273.747123049141,274.745915452909,
275.744707856677,276.743500260445,277.742292664213,278.741085067981,279.739877471749,
280.738669875517,281.737462279285,282.736254683053,283.735047086821,284.733839490589,
285.732631894357,286.731424298125,287.730216701893,288.729009105661,289.727801509429,
290.726593913197,291.725386316965,292.724178720733,293.722971124501,294.721763528269,
295.720555932037,296.719348335805,297.718140739573,298.716933143341,299.715725547109,
300.714517950877,301.713310354645,302.712102758413,303.710895162181,304.709687565949,
305.708479969717,306.707272373485,307.706064777253,308.704857181021,309.703649584789,
310.702441988557,311.701234392325,312.700026796093,313.698819199861,314.697611603629,
315.696404007397,316.695196411165,317.693988814933,318.692781218701,319.691573622469,
320.690366026237,321.689158430005,322.687950833773,323.686743237541,324.685535641309,
325.684328045077,326.683120448845,327.681912852613,328.680705256381,329.679497660149,
330.678290063917,331.677082467685,332.675874871453,333.674667275221,334.67345967899,
335.672252082757,336.671044486525,337.669836890294,338.668629294062,339.66742169783,
340.666214101598,341.665006505366,342.663798909134,343.662591312902,344.66138371667,
345.660176120438,346.658968524206,347.657760927974,348.656553331742,349.65534573551,
350.654138139278,351.652930543046,352.651722946814,353.650515350582,354.64930775435,
355.648100158118,356.646892561886,357.645684965654,358.644477369422,359.64326977319,
360.642062176958,361.640854580726,362.639646984494,363.638439388262,364.63723179203,
365.636024195798,366.634816599566,367.633609003334,368.632401407102,369.63119381087,
370.629986214638,371.628778618406,372.627571022174,373.626363425942,374.62515582971,
375.623948233478,376.622740637246,377.621533041014,378.620325444782,379.61911784855,
380.617910252318,381.616702656086,382.615495059854,383.614287463622,384.61307986739,
385.611872271158,386.610664674926,387.609457078694,388.608249482462,389.60704188623,
390.605834289998,391.604626693766,392.603419097534,393.602211501302,394.60100390507,
395.599796308838,396.598588712606,397.597381116374,398.596173520142,399.59496592391,
400.593758327678,401.592550731446,402.591343135214,403.590135538982,404.58892794275,
405.587720346518,406.586512750286,407.585305154054,408.584097557822,409.58288996159,
410.581682365359,411.580474769127,412.579267172895,413.578059576663,414.576851980431,
415.575644384199,416.574436787967,417.573229191735,418.572021595503,419.570813999271,
420.569606403039,421.568398806807,422.567191210575,423.565983614343,424.564776018111,
425.563568421879,426.562360825647,427.561153229415,428.559945633183,429.558738036951,
430.557530440719,431.556322844487,432.555115248255,433.553907652023,434.552700055791,
435.551492459559,436.550284863327,437.549077267095,438.547869670863,439.546662074631,
440.545454478399,441.544246882167,442.543039285935,443.541831689703,444.540624093471,
445.539416497239,446.538208901007,447.537001304775,448.535793708543,449.534586112311,
450.533378516079,451.532170919847,452.530963323615,453.529755727383,454.528548131151,
455.527340534919,456.526132938687,457.524925342455,458.523717746223,459.522510149991,
460.521302553759,461.520094957527,462.518887361295,463.517679765063,464.516472168831,
465.515264572599,466.514056976367,467.512849380135,468.511641783903,469.510434187671,
470.509226591439),.UNSPECIFIED.);
#437=FACE_BOUND('',#3219,.T.);
#438=FACE_BOUND('',#3220,.T.);
#439=FACE_BOUND('',#3237,.T.);
#661=B_SPLINE_CURVE_WITH_KNOTS('',3,(#23900,#23901,#23902,#23903,#23904,
#23905),.UNSPECIFIED.,.F.,.F.,(4,1,1,4),(-454.450543714446,-453.451751310678,
-452.45295890691,-452.038622507886),.UNSPECIFIED.);
#662=B_SPLINE_CURVE_WITH_KNOTS('',3,(#23907,#23908,#23909,#23910,#23911,
#23912,#23913,#23914,#23915,#23916),.UNSPECIFIED.,.F.,.F.,(4,1,1,1,1,1,
1,4),(-452.038622507886,-451.454166503142,-450.455374099374,-449.456581695606,
-448.457789291838,-447.45899688807,-446.460204484302,-445.755437200706),
 .UNSPECIFIED.);
#663=B_SPLINE_CURVE_WITH_KNOTS('',3,(#23918,#23919,#23920,#23921,#23922,
#23923,#23924,#23925,#23926,#23927,#23928,#23929,#23930,#23931,#23932,#23933,
#23934,#23935,#23936,#23937,#23938,#23939,#23940,#23941,#23942,#23943,#23944,
#23945,#23946,#23947,#23948,#23949,#23950,#23951,#23952,#23953,#23954,#23955,
#23956,#23957,#23958,#23959,#23960,#23961,#23962,#23963,#23964,#23965,#23966,
#23967,#23968,#23969,#23970,#23971,#23972,#23973,#23974,#23975,#23976,#23977,
#23978,#23979,#23980,#23981,#23982,#23983,#23984,#23985,#23986,#23987,#23988,
#23989,#23990,#23991,#23992,#23993,#23994,#23995,#23996,#23997,#23998,#23999,
#24000,#24001,#24002,#24003,#24004,#24005,#24006,#24007,#24008,#24009,#24010,
#24011,#24012,#24013,#24014,#24015,#24016,#24017,#24018,#24019,#24020,#24021,
#24022,#24023,#24024,#24025,#24026,#24027,#24028,#24029,#24030,#24031,#24032,
#24033,#24034,#24035,#24036,#24037,#24038,#24039,#24040,#24041,#24042,#24043,
#24044,#24045,#24046,#24047,#24048,#24049,#24050),.UNSPECIFIED.,.F.,.F.,
(4,3,3,3,3,3,3,3,3,3,3,3,3,3,3,3,3,3,3,3,3,3,3,3,3,3,3,3,3,3,3,3,3,3,3,
3,3,3,3,3,3,3,3,3,4),(-445.755437031918,-445.563647569504,-445.461412080534,
-445.303982702834,-445.146842808848,-444.989871571425,-444.832819606925,
-444.675719587285,-444.51827995468,-444.462619676766,-444.305197863777,
-444.148065737253,-443.991102442813,-443.834058588833,-443.676966786957,
-443.519535409268,-443.463827272998,-443.306400089056,-443.149262491187,
-442.992293644092,-442.835244182094,-442.678146733064,-442.520709734799,
-442.46503486923,-442.307608665139,-442.150472048908,-441.993504181851,
-441.836455685854,-441.679359195915,-441.521923131783,-441.466242465462,
-441.308817158692,-441.151681465853,-440.994714545015,-440.837667018058,
-440.680571511596,-440.523136437804,-440.467450061694,-440.31012564541,
-440.153090641361,-439.996223862719,-439.839276201223,-439.682279418494,
-439.524944479556,-439.472251893657),.UNSPECIFIED.);
#664=B_SPLINE_CURVE_WITH_KNOTS('',3,(#24052,#24053,#24054,#24055,#24056,
#24057,#24058,#24059,#24060,#24061,#24062,#24063,#24064,#24065,#24066,#24067,
#24068,#24069,#24070,#24071,#24072,#24073,#24074,#24075,#24076,#24077,#24078,
#24079,#24080,#24081,#24082,#24083,#24084,#24085,#24086,#24087,#24088,#24089,
#24090,#24091,#24092,#24093,#24094,#24095,#24096,#24097,#24098,#24099,#24100,
#24101,#24102,#24103,#24104,#24105,#24106,#24107,#24108,#24109,#24110,#24111,
#24112,#24113,#24114,#24115,#24116,#24117,#24118,#24119,#24120,#24121,#24122,
#24123,#24124,#24125,#24126,#24127,#24128,#24129,#24130,#24131,#24132,#24133,
#24134,#24135,#24136,#24137,#24138,#24139,#24140,#24141,#24142,#24143,#24144,
#24145,#24146,#24147,#24148,#24149,#24150,#24151,#24152,#24153,#24154,#24155,
#24156,#24157,#24158,#24159,#24160,#24161,#24162,#24163,#24164,#24165,#24166,
#24167,#24168,#24169,#24170,#24171,#24172,#24173,#24174,#24175,#24176,#24177,
#24178,#24179,#24180,#24181,#24182,#24183,#24184,#24185,#24186,#24187),
 .UNSPECIFIED.,.F.,.F.,(4,3,3,3,3,3,3,3,3,3,3,3,3,3,3,3,3,3,3,3,3,3,3,3,
3,3,3,3,3,3,3,3,3,3,3,3,3,3,3,3,3,3,3,3,3,4),(-439.472251893527,-439.468657657926,
-439.311231772696,-439.15409548774,-438.997127963201,-438.840079822431,
-438.682983695525,-438.525548000696,-438.469865254158,-438.312439469266,
-438.155303287897,-437.998335869829,-437.841287838569,-437.684191823072,
-437.526756240826,-437.47107285039,-437.313646957827,-437.156510666562,
-436.999543136757,-436.842494992339,-436.685398862719,-436.527963166623,
-436.472280446622,-436.314854587534,-436.157718330119,-436.000750834421,
-435.84370272409,-435.686606628587,-435.529170966138,-435.473488042854,
-435.316062193978,-435.158925947163,-435.001958462417,-434.844910363434,
-434.687814279521,-434.530378628852,-434.474695639086,-434.317269775444,
-434.160133513544,-434.003166013446,-433.846117898893,-433.689021799266,
-433.531586132904,-433.475903235318,-433.282382207345,-433.189066586492),
 .UNSPECIFIED.);
#665=B_SPLINE_CURVE_WITH_KNOTS('',3,(#24189,#24190,#24191,#24192,#24193,
#24194,#24195,#24196,#24197,#24198,#24199,#24200,#24201,#24202,#24203,#24204,
#24205,#24206,#24207,#24208,#24209,#24210,#24211,#24212,#24213,#24214,#24215,
#24216,#24217,#24218,#24219,#24220,#24221,#24222,#24223,#24224,#24225,#24226,
#24227,#24228,#24229,#24230,#24231,#24232,#24233,#24234,#24235,#24236,#24237,
#24238,#24239,#24240,#24241,#24242,#24243,#24244,#24245,#24246,#24247,#24248,
#24249,#24250,#24251,#24252,#24253,#24254,#24255,#24256,#24257,#24258,#24259,
#24260,#24261,#24262,#24263,#24264,#24265,#24266,#24267,#24268,#24269,#24270,
#24271,#24272,#24273,#24274,#24275,#24276,#24277,#24278,#24279,#24280,#24281,
#24282,#24283,#24284,#24285,#24286,#24287,#24288,#24289,#24290,#24291,#24292,
#24293,#24294,#24295,#24296,#24297,#24298,#24299,#24300,#24301,#24302,#24303,
#24304,#24305,#24306,#24307,#24308,#24309,#24310,#24311,#24312,#24313,#24314,
#24315,#24316,#24317,#24318,#24319,#24320,#24321),.UNSPECIFIED.,.F.,.F.,
(4,3,3,3,3,3,3,3,3,3,3,3,3,3,3,3,3,3,3,3,3,3,3,3,3,3,3,3,3,3,3,3,3,3,3,
3,3,3,3,3,3,3,3,3,4),(-433.189066586347,-433.033254193185,-432.877394202068,
-432.721515030693,-432.565286838749,-432.47711083155,-432.319684974318,
-432.162548718947,-432.005581225473,-431.848533117611,-431.69143702472,
-431.534001365061,-431.478318427782,-431.320892568569,-431.163756311173,
-431.006788815636,-430.849740705678,-430.69264461067,-430.535208948895,
-430.479526024014,-430.322100165682,-430.16496390918,-430.007996414548,
-429.850948305499,-429.693852211404,-429.536416550533,-429.480733620246,
-429.323307761953,-429.166171505494,-429.00920401091,-428.852155901915,
-428.695059807878,-428.537624147069,-428.481941216478,-428.324515357926,
-428.167379101201,-428.010411606347,-427.853363497076,-427.696267402761,
-427.538831741673,-427.48314881271,-427.322417720406,-427.162039311243,
-427.001921757567,-426.905881279168),.UNSPECIFIED.);
#666=B_SPLINE_CURVE_WITH_KNOTS('',3,(#24323,#24324,#24325,#24326,#24327,
#24328,#24329,#24330,#24331,#24332,#24333,#24334,#24335,#24336,#24337,#24338,
#24339,#24340,#24341,#24342,#24343,#24344,#24345,#24346,#24347,#24348,#24349,
#24350,#24351,#24352,#24353,#24354,#24355,#24356,#24357,#24358,#24359,#24360,
#24361,#24362,#24363,#24364,#24365,#24366,#24367,#24368,#24369,#24370,#24371,
#24372,#24373,#24374,#24375,#24376,#24377,#24378,#24379,#24380,#24381,#24382,
#24383,#24384,#24385,#24386,#24387,#24388,#24389,#24390,#24391,#24392,#24393,
#24394,#24395,#24396,#24397,#24398,#24399,#24400,#24401,#24402,#24403,#24404,
#24405,#24406,#24407,#24408,#24409,#24410,#24411,#24412,#24413,#24414,#24415,
#24416,#24417,#24418,#24419,#24420,#24421,#24422,#24423,#24424,#24425,#24426,
#24427,#24428,#24429,#24430,#24431,#24432,#24433,#24434,#24435,#24436,#24437,
#24438,#24439,#24440,#24441,#24442,#24443,#24444,#24445,#24446,#24447,#24448,
#24449,#24450,#24451,#24452,#24453,#24454,#24455),.UNSPECIFIED.,.F.,.F.,
(4,3,3,3,3,3,3,3,3,3,3,3,3,3,3,3,3,3,3,3,3,3,3,3,3,3,3,3,3,3,3,3,3,3,3,
3,3,3,3,3,3,3,3,3,4),(-426.905881278986,-426.734684431719,-426.562354361466,
-426.484356408942,-426.326930550519,-426.169794293926,-426.012826799205,
-425.85577869007,-425.698682595891,-425.54124693494,-425.485564005174,-425.328138146718,
-425.171001890091,-425.014034395336,-424.856986286166,-424.699890191952,
-424.542454530965,-424.486771601406,-424.32934574297,-424.172209486364,
-424.015241991629,-423.85819388248,-423.701097788287,-423.543662127321,
-423.487979197638,-423.330553339199,-423.173417082591,-423.016449587854,
-422.859401478702,-422.702305384507,-422.544869723539,-422.48918679387,
-422.331760935427,-422.174624678815,-422.017657184074,-421.860609074918,
-421.703512980719,-421.546077319746,-421.490394390102,-421.335204760125,
-421.180302064992,-421.025459880721,-420.870661563784,-420.715596582732,
-420.622695971988),.UNSPECIFIED.);
#667=B_SPLINE_CURVE_WITH_KNOTS('',3,(#24457,#24458,#24459,#24460,#24461,
#24462,#24463,#24464,#24465,#24466,#24467),.UNSPECIFIED.,.F.,.F.,(4,1,1,
1,1,1,1,1,4),(-420.622695971988,-420.491601986334,-419.492809582566,-418.494017178798,
-417.49522477503,-416.496432371262,-415.497639967494,-414.498847563725,
-414.339510664809),.UNSPECIFIED.);
#668=B_SPLINE_CURVE_WITH_KNOTS('',3,(#24469,#24470,#24471,#24472,#24473,
#24474,#24475,#24476,#24477,#24478,#24479,#24480,#24481,#24482,#24483,#24484,
#24485,#24486,#24487,#24488,#24489,#24490,#24491,#24492,#24493,#24494,#24495,
#24496,#24497,#24498,#24499,#24500,#24501,#24502,#24503,#24504,#24505,#24506,
#24507,#24508,#24509,#24510,#24511,#24512,#24513,#24514,#24515,#24516,#24517,
#24518,#24519,#24520,#24521,#24522,#24523,#24524,#24525,#24526,#24527,#24528,
#24529,#24530,#24531,#24532,#24533,#24534,#24535,#24536,#24537,#24538,#24539,
#24540,#24541,#24542,#24543,#24544,#24545,#24546,#24547,#24548,#24549,#24550,
#24551,#24552,#24553,#24554,#24555,#24556,#24557,#24558,#24559,#24560,#24561,
#24562,#24563,#24564,#24565,#24566,#24567,#24568,#24569,#24570,#24571,#24572,
#24573,#24574,#24575,#24576,#24577,#24578,#24579,#24580,#24581,#24582,#24583,
#24584,#24585,#24586,#24587,#24588,#24589,#24590,#24591,#24592,#24593,#24594,
#24595,#24596,#24597,#24598,#24599,#24600,#24601),.UNSPECIFIED.,.F.,.F.,
(4,3,3,3,3,3,3,3,3,3,3,3,3,3,3,3,3,3,3,3,3,3,3,3,3,3,3,3,3,3,3,3,3,3,3,
3,3,3,3,3,3,3,3,3,4),(-414.339510664809,-414.18459996589,-414.02990276154,
-413.875168508411,-413.720414365598,-413.565333554294,-413.500055159957,
-413.342629301517,-413.185493044907,-413.028525550168,-412.871477441014,
-412.714381346817,-412.556945685847,-412.501262756189,-412.343836897749,
-412.186700641139,-412.0297331464,-411.872685037246,-411.715588943049,-411.558153282079,
-411.502470352421,-411.34504449398,-411.18790823737,-411.030940742631,-410.873892633478,
-410.71679653928,-410.55936087831,-410.503677948653,-410.346252090213,-410.189115833602,
-410.032148338863,-409.87510022971,-409.718004135513,-409.560568474542,
-409.504885544885,-409.347459686444,-409.190323429834,-409.033355935095,
-408.876307825941,-408.719211731744,-408.561776070773,-408.506093141117,
-408.336537608055,-408.167873380534,-408.056325619396),.UNSPECIFIED.);
#669=B_SPLINE_CURVE_WITH_KNOTS('',3,(#24603,#24604,#24605,#24606,#24607,
#24608,#24609,#24610,#24611,#24612),.UNSPECIFIED.,.F.,.F.,(4,1,1,1,1,1,
1,4),(-408.056325357629,-407.507300737349,-406.508508333581,-405.509715929813,
-404.510923526045,-403.512131122277,-402.513338718509,-401.773140050449),
 .UNSPECIFIED.);
#670=B_SPLINE_CURVE_WITH_KNOTS('',3,(#24614,#24615,#24616,#24617,#24618,
#24619,#24620,#24621,#24622,#24623,#24624,#24625,#24626,#24627,#24628,#24629,
#24630,#24631,#24632,#24633,#24634,#24635,#24636,#24637,#24638,#24639,#24640,
#24641,#24642,#24643,#24644,#24645,#24646,#24647,#24648,#24649,#24650,#24651,
#24652,#24653,#24654,#24655,#24656,#24657,#24658,#24659,#24660,#24661,#24662,
#24663,#24664,#24665,#24666,#24667,#24668,#24669,#24670,#24671,#24672,#24673,
#24674,#24675,#24676,#24677,#24678,#24679,#24680,#24681,#24682,#24683,#24684,
#24685,#24686,#24687,#24688,#24689,#24690,#24691,#24692,#24693,#24694,#24695,
#24696,#24697,#24698,#24699,#24700,#24701,#24702,#24703,#24704,#24705,#24706,
#24707,#24708,#24709,#24710,#24711,#24712,#24713,#24714,#24715,#24716,#24717,
#24718,#24719,#24720,#24721,#24722,#24723,#24724,#24725,#24726,#24727,#24728,
#24729,#24730,#24731,#24732,#24733,#24734,#24735,#24736,#24737,#24738,#24739,
#24740,#24741,#24742,#24743,#24744,#24745,#24746,#24747,#24748,#24749),
 .UNSPECIFIED.,.F.,.F.,(4,3,3,3,3,3,3,3,3,3,3,3,3,3,3,3,3,3,3,3,3,3,3,3,
3,3,3,3,3,3,3,3,3,3,3,3,3,3,3,3,3,3,3,3,3,4),(-401.773139972096,-401.571895517567,
-401.514546314741,-401.3571204563,-401.19998419969,-401.04301670495,-400.885968595796,
-400.728872501598,-400.571436840628,-400.515753910973,-400.358328052533,
-400.201191795923,-400.044224301183,-399.88717619203,-399.730080097833,
-399.572644436863,-399.516961507205,-399.359535648765,-399.202399392154,
-399.045431897415,-398.888383788262,-398.731287694065,-398.573852033095,
-398.518169103437,-398.360743244997,-398.203606988386,-398.046639493647,
-397.889591384493,-397.732495290296,-397.575059629326,-397.519376699669,
-397.361950841229,-397.204814584618,-397.047847089879,-396.890798980726,
-396.733702886529,-396.576267225559,-396.520584295901,-396.36315843746,
-396.20602218085,-396.049054686111,-395.892006576957,-395.73491048276,-395.577474821789,
-395.521791892133,-395.48995474327),.UNSPECIFIED.);
#671=B_SPLINE_CURVE_WITH_KNOTS('',3,(#24751,#24752,#24753,#24754,#24755,
#24756,#24757,#24758,#24759,#24760,#24761,#24762,#24763,#24764,#24765,#24766,
#24767,#24768,#24769,#24770,#24771,#24772,#24773,#24774,#24775,#24776,#24777,
#24778,#24779,#24780,#24781,#24782,#24783,#24784,#24785,#24786,#24787,#24788,
#24789,#24790,#24791,#24792,#24793,#24794,#24795,#24796,#24797,#24798,#24799,
#24800,#24801,#24802,#24803,#24804,#24805,#24806,#24807,#24808,#24809,#24810,
#24811,#24812,#24813,#24814,#24815,#24816,#24817,#24818,#24819,#24820,#24821,
#24822,#24823,#24824,#24825,#24826,#24827,#24828,#24829,#24830,#24831,#24832,
#24833,#24834,#24835,#24836,#24837,#24838,#24839,#24840,#24841,#24842,#24843,
#24844,#24845,#24846,#24847,#24848,#24849,#24850,#24851,#24852,#24853,#24854,
#24855,#24856,#24857,#24858,#24859,#24860,#24861,#24862,#24863,#24864,#24865,
#24866,#24867,#24868,#24869,#24870,#24871,#24872,#24873,#24874,#24875,#24876,
#24877,#24878,#24879,#24880,#24881,#24882,#24883),.UNSPECIFIED.,.F.,.F.,
(4,3,3,3,3,3,3,3,3,3,3,3,3,3,3,3,3,3,3,3,3,3,3,3,3,3,3,3,3,3,3,3,3,3,3,
3,3,3,3,3,3,3,3,3,4),(-395.489954743044,-395.333356255252,-395.177042096409,
-395.013531444398,-394.857291860972,-394.700987210959,-394.544356112011,
-394.522999488365,-394.365573629925,-394.208437373314,-394.051469878575,
-393.894421769422,-393.737325675225,-393.579890014255,-393.524207084597,
-393.366781226157,-393.209644969546,-393.052677474807,-392.895629365654,
-392.738533271457,-392.581097610486,-392.525414680829,-392.367988822388,
-392.210852565778,-392.053885071039,-391.896836961886,-391.739740867688,
-391.582305206718,-391.526622277061,-391.369196418621,-391.21206016201,
-391.055092667271,-390.898044558118,-390.740948463921,-390.583512802951,
-390.527829873293,-390.370404014853,-390.213267758243,-390.056300263504,
-389.89925215435,-389.742156060153,-389.584720399183,-389.529037469525,
-389.343111524021,-389.206769436297),.UNSPECIFIED.);
#672=B_SPLINE_CURVE_WITH_KNOTS('',3,(#24885,#24886,#24887,#24888,#24889,
#24890,#24891,#24892,#24893,#24894,#24895,#24896,#24897,#24898,#24899,#24900,
#24901,#24902,#24903,#24904,#24905,#24906,#24907,#24908,#24909,#24910,#24911,
#24912,#24913,#24914,#24915,#24916,#24917,#24918,#24919,#24920,#24921,#24922,
#24923,#24924,#24925,#24926,#24927,#24928,#24929,#24930,#24931,#24932,#24933,
#24934,#24935,#24936,#24937,#24938,#24939,#24940,#24941,#24942,#24943,#24944,
#24945,#24946,#24947,#24948,#24949,#24950,#24951,#24952,#24953,#24954,#24955,
#24956,#24957,#24958,#24959,#24960,#24961,#24962,#24963,#24964,#24965,#24966,
#24967,#24968,#24969,#24970,#24971,#24972,#24973,#24974,#24975,#24976,#24977,
#24978,#24979,#24980,#24981,#24982,#24983,#24984,#24985,#24986,#24987,#24988,
#24989,#24990,#24991,#24992,#24993,#24994,#24995,#24996,#24997,#24998,#24999,
#25000,#25001,#25002,#25003,#25004,#25005,#25006,#25007,#25008,#25009,#25010,
#25011,#25012,#25013,#25014,#25015,#25016,#25017),.UNSPECIFIED.,.F.,.F.,
(4,3,3,3,3,3,3,3,3,3,3,3,3,3,3,3,3,3,3,3,3,3,3,3,3,3,3,3,3,3,3,3,3,3,3,
3,3,3,3,3,3,3,3,3,4),(-389.20676943609,-389.050212150193,-388.893556938872,
-388.736841628448,-388.57977489144,-388.530245065757,-388.372819207317,
-388.215682950706,-388.058715455967,-387.901667346814,-387.744571252616,
-387.587135591646,-387.531452661989,-387.374026803549,-387.216890546938,
-387.059923052199,-386.902874943046,-386.745778848848,-386.588343187878,
-386.532660258221,-386.375234399781,-386.21809814317,-386.061130648431,
-385.904082539278,-385.746986445081,-385.589550784111,-385.533867854453,
-385.376441996013,-385.219305739402,-385.062338244663,-384.90529013551,
-384.748194041312,-384.590758380342,-384.535075450685,-384.377649592244,
-384.220513335634,-384.063545840895,-383.906497731741,-383.749401637544,
-383.591965976573,-383.536283046917,-383.377122321744,-383.218286232242,
-383.059621574311,-382.923584128911),.UNSPECIFIED.);
#673=B_SPLINE_CURVE_WITH_KNOTS('',3,(#25019,#25020,#25021,#25022,#25023,
#25024,#25025,#25026,#25027,#25028),.UNSPECIFIED.,.F.,.F.,(4,1,1,1,1,1,
1,4),(-382.923576795181,-382.537490643149,-381.538698239381,-380.539905835613,
-379.541113431845,-378.542321028077,-377.543528624309,-376.64040770302),
 .UNSPECIFIED.);
#674=B_SPLINE_CURVE_WITH_KNOTS('',3,(#25030,#25031,#25032,#25033,#25034,
#25035,#25036,#25037,#25038,#25039,#25040,#25041,#25042,#25043,#25044,#25045,
#25046,#25047,#25048,#25049,#25050,#25051,#25052,#25053,#25054,#25055,#25056,
#25057,#25058,#25059,#25060,#25061,#25062,#25063,#25064,#25065,#25066,#25067,
#25068,#25069,#25070,#25071,#25072,#25073,#25074,#25075,#25076,#25077,#25078,
#25079,#25080,#25081,#25082,#25083,#25084,#25085,#25086,#25087,#25088,#25089,
#25090,#25091,#25092,#25093,#25094,#25095,#25096,#25097,#25098,#25099,#25100,
#25101,#25102,#25103,#25104,#25105,#25106,#25107,#25108,#25109,#25110,#25111,
#25112,#25113,#25114,#25115,#25116,#25117,#25118,#25119,#25120,#25121,#25122,
#25123,#25124,#25125,#25126,#25127,#25128,#25129,#25130,#25131,#25132,#25133,
#25134,#25135,#25136,#25137,#25138,#25139,#25140,#25141,#25142,#25143,#25144,
#25145,#25146,#25147,#25148,#25149,#25150,#25151,#25152,#25153,#25154,#25155,
#25156,#25157,#25158,#25159,#25160,#25161,#25162),.UNSPECIFIED.,.F.,.F.,
(4,3,3,3,3,3,3,3,3,3,3,3,3,3,3,3,3,3,3,3,3,3,3,3,3,3,3,3,3,3,3,3,3,3,3,
3,3,3,3,3,3,3,3,3,4),(-376.640398821731,-376.544736220541,-376.3873103621,
-376.23017410549,-376.073206610751,-375.916158501597,-375.7590624074,-375.60162674643,
-375.545943816773,-375.388517958333,-375.231381701722,-375.074414206983,
-374.91736609783,-374.760270003632,-374.602834342662,-374.547151413005,
-374.389725554565,-374.232589297955,-374.075621803215,-373.918573694062,
-373.761477599865,-373.604041938895,-373.548359009237,-373.390933150797,
-373.233796894186,-373.076829399447,-372.919781290294,-372.762685196096,
-372.605249535126,-372.549566605469,-372.392140747029,-372.235004490418,
-372.078036995679,-371.920988886525,-371.763892792328,-371.606457131358,
-371.550774201701,-371.393348343261,-371.23621208665,-371.079244591911,
-370.922196482758,-370.76510038856,-370.60766472759,-370.551981797933,-370.357213514552),
 .UNSPECIFIED.);
#675=B_SPLINE_CURVE_WITH_KNOTS('',3,(#25164,#25165,#25166,#25167,#25168,
#25169,#25170,#25171,#25172,#25173),.UNSPECIFIED.,.F.,.F.,(4,1,1,1,1,1,
1,4),(-370.357209727041,-369.553189394165,-368.554396990397,-367.555604586629,
-366.556812182861,-365.558019779093,-364.559227375325,-364.074029310628),
 .UNSPECIFIED.);
#676=B_SPLINE_CURVE_WITH_KNOTS('',3,(#25175,#25176,#25177,#25178,#25179,
#25180,#25181,#25182,#25183,#25184,#25185,#25186,#25187,#25188,#25189,#25190,
#25191,#25192,#25193,#25194,#25195,#25196,#25197,#25198,#25199,#25200,#25201,
#25202,#25203,#25204,#25205,#25206,#25207,#25208,#25209,#25210,#25211,#25212,
#25213,#25214,#25215,#25216,#25217,#25218,#25219,#25220,#25221,#25222,#25223,
#25224,#25225,#25226,#25227,#25228,#25229,#25230,#25231,#25232,#25233,#25234,
#25235,#25236,#25237,#25238,#25239,#25240,#25241,#25242,#25243,#25244,#25245,
#25246,#25247,#25248,#25249,#25250,#25251,#25252,#25253,#25254,#25255,#25256,
#25257,#25258,#25259,#25260,#25261,#25262,#25263,#25264,#25265,#25266,#25267,
#25268,#25269,#25270,#25271,#25272,#25273,#25274,#25275,#25276,#25277,#25278,
#25279,#25280,#25281,#25282,#25283,#25284,#25285,#25286,#25287,#25288,#25289,
#25290,#25291,#25292,#25293,#25294,#25295,#25296,#25297,#25298,#25299,#25300,
#25301,#25302,#25303,#25304,#25305,#25306,#25307),.UNSPECIFIED.,.F.,.F.,
(4,3,3,3,3,3,3,3,3,3,3,3,3,3,3,3,3,3,3,3,3,3,3,3,3,3,3,3,3,3,3,3,3,3,3,
3,3,3,3,3,3,3,3,3,4),(-364.074028207372,-363.910363618122,-363.746409744268,
-363.581908190044,-363.560434971557,-363.403009113117,-363.245872856506,
-363.088905361767,-362.931857252614,-362.774761158417,-362.617325497447,
-362.561642567789,-362.404216709349,-362.247080452738,-362.090112957999,
-361.933064848846,-361.775968754648,-361.618533093678,-361.562850164021,
-361.40542430558,-361.24828804897,-361.091320554231,-360.934272445078,-360.77717635088,
-360.61974068991,-360.564057760253,-360.406631901813,-360.249495645202,
-360.092528150463,-359.93548004131,-359.778383947113,-359.620948286143,
-359.565265356485,-359.407839498044,-359.250703241434,-359.093735746695,
-358.936687637542,-358.779591543344,-358.622155882374,-358.566472952717,
-358.411148615583,-358.256067606148,-358.101147748962,-357.945995324577,
-357.790842900193),.UNSPECIFIED.);
#677=B_SPLINE_CURVE_WITH_KNOTS('',3,(#25309,#25310,#25311,#25312,#25313,
#25314,#25315,#25316,#25317,#25318,#25319),.UNSPECIFIED.,.F.,.F.,(4,1,1,
1,1,1,1,1,4),(-357.790842900193,-357.567680548949,-356.568888145181,-355.570095741413,
-354.571303337645,-353.572510933877,-352.573718530109,-351.574926126341,
-351.507657593013),.UNSPECIFIED.);
#678=B_SPLINE_CURVE_WITH_KNOTS('',3,(#25321,#25322,#25323,#25324,#25325,
#25326,#25327,#25328,#25329,#25330,#25331,#25332,#25333,#25334,#25335,#25336,
#25337,#25338,#25339,#25340,#25341,#25342,#25343,#25344,#25345,#25346,#25347,
#25348,#25349,#25350,#25351,#25352,#25353,#25354,#25355,#25356,#25357,#25358,
#25359,#25360,#25361,#25362,#25363,#25364,#25365,#25366,#25367,#25368,#25369,
#25370,#25371,#25372,#25373,#25374,#25375,#25376,#25377,#25378,#25379,#25380,
#25381,#25382,#25383,#25384,#25385,#25386,#25387,#25388,#25389,#25390,#25391,
#25392,#25393,#25394,#25395,#25396,#25397,#25398,#25399,#25400,#25401,#25402,
#25403,#25404,#25405,#25406,#25407,#25408,#25409,#25410,#25411,#25412,#25413,
#25414,#25415,#25416,#25417,#25418,#25419,#25420,#25421,#25422,#25423,#25424,
#25425,#25426,#25427,#25428,#25429,#25430,#25431,#25432,#25433,#25434,#25435,
#25436,#25437,#25438,#25439,#25440,#25441,#25442,#25443,#25444,#25445,#25446,
#25447,#25448,#25449,#25450),.UNSPECIFIED.,.F.,.F.,(4,3,3,3,3,3,3,3,3,3,
3,3,3,3,3,3,3,3,3,3,3,3,3,3,3,3,3,3,3,3,3,3,3,3,3,3,3,3,3,3,3,3,3,4),(-351.507657593013,
-351.351786036364,-351.19618592939,-351.040599679445,-350.885048669655,
-350.72913646519,-350.576133722573,-350.418707864133,-350.261571607522,
-350.104604112783,-349.94755600363,-349.790459909432,-349.633024248462,
-349.577341318805,-349.419915460365,-349.262779203754,-349.105811709015,
-348.948763599862,-348.791667505664,-348.634231844694,-348.578548915037,
-348.421123056597,-348.263986799986,-348.107019305247,-347.949971196094,
-347.792875101896,-347.635439440926,-347.579756511269,-347.422330652829,
-347.265194396218,-347.108226901479,-346.951178792326,-346.794082698128,
-346.636647037158,-346.580964107501,-346.423538249061,-346.266401992451,
-346.109434497712,-345.952386388559,-345.795290294362,-345.637854633392,
-345.582171703733,-345.402219924872,-345.224472530763),.UNSPECIFIED.);
#679=B_SPLINE_CURVE_WITH_KNOTS('',3,(#25452,#25453,#25454,#25455,#25456,
#25457,#25458,#25459,#25460,#25461),.UNSPECIFIED.,.F.,.F.,(4,1,1,1,1,1,
1,4),(-345.224472285833,-344.583379299965,-343.584586896197,-342.585794492429,
-341.587002088661,-340.588209684893,-339.589417281125,-338.941286978654),
 .UNSPECIFIED.);
#680=B_SPLINE_CURVE_WITH_KNOTS('',3,(#25463,#25464,#25465,#25466,#25467,
#25468,#25469,#25470,#25471,#25472,#25473,#25474,#25475,#25476,#25477,#25478,
#25479,#25480,#25481,#25482,#25483,#25484,#25485,#25486,#25487,#25488,#25489,
#25490,#25491,#25492,#25493,#25494,#25495,#25496,#25497,#25498,#25499,#25500,
#25501,#25502,#25503,#25504,#25505,#25506,#25507,#25508,#25509,#25510,#25511,
#25512,#25513,#25514,#25515,#25516,#25517,#25518,#25519,#25520,#25521,#25522,
#25523,#25524,#25525,#25526,#25527,#25528,#25529,#25530,#25531,#25532,#25533,
#25534,#25535,#25536,#25537,#25538,#25539,#25540,#25541,#25542,#25543,#25544,
#25545,#25546,#25547,#25548,#25549,#25550,#25551,#25552,#25553,#25554,#25555,
#25556,#25557,#25558,#25559,#25560,#25561,#25562,#25563,#25564,#25565,#25566,
#25567,#25568,#25569,#25570,#25571,#25572,#25573,#25574,#25575,#25576,#25577,
#25578,#25579,#25580,#25581,#25582,#25583,#25584,#25585,#25586,#25587,#25588,
#25589,#25590,#25591,#25592),.UNSPECIFIED.,.F.,.F.,(4,3,3,3,3,3,3,3,3,3,
3,3,3,3,3,3,3,3,3,3,3,3,3,3,3,3,3,3,3,3,3,3,3,3,3,3,3,3,3,3,3,3,3,4),(-338.941286736142,
-338.760252301847,-338.590624877357,-338.433199018916,-338.276062762304,
-338.119095267564,-337.962047158409,-337.804951064211,-337.64751540324,
-337.591832473588,-337.434406615148,-337.277270358537,-337.120302863798,
-336.963254754645,-336.806158660448,-336.648722999478,-336.59304006982,
-336.43561421138,-336.27847795477,-336.121510460031,-335.964462350878,-335.807366256681,
-335.649930595711,-335.594247666052,-335.436821807611,-335.279685551001,
-335.122718056262,-334.965669947108,-334.808573852911,-334.651138191941,
-334.595455262284,-334.438029403844,-334.280893147233,-334.123925652494,
-333.966877543341,-333.809781449143,-333.652345788173,-333.596662858516,
-333.440630649672,-333.284885507811,-333.128189548727,-332.972529747918,
-332.815315709696,-332.658101671474),.UNSPECIFIED.);
#681=B_SPLINE_CURVE_WITH_KNOTS('',3,(#25594,#25595,#25596,#25597,#25598,
#25599,#25600,#25601,#25602,#25603,#25604,#25605),.UNSPECIFIED.,.F.,.F.,
(4,2,1,1,1,1,1,1,4),(-332.658101671474,-332.597870454748,-331.59907805098,
-330.600285647212,-329.601493243444,-328.602700839676,-327.603908435908,
-326.60511603214,-326.374916364295),.UNSPECIFIED.);
#682=B_SPLINE_CURVE_WITH_KNOTS('',3,(#25607,#25608,#25609,#25610,#25611,
#25612,#25613,#25614,#25615,#25616,#25617,#25618,#25619,#25620,#25621,#25622,
#25623,#25624,#25625,#25626,#25627,#25628,#25629,#25630,#25631,#25632,#25633,
#25634,#25635,#25636,#25637,#25638,#25639,#25640,#25641,#25642,#25643,#25644,
#25645,#25646,#25647,#25648,#25649,#25650,#25651,#25652,#25653,#25654,#25655,
#25656,#25657,#25658,#25659,#25660,#25661,#25662,#25663,#25664,#25665,#25666,
#25667,#25668,#25669,#25670,#25671,#25672,#25673,#25674,#25675,#25676,#25677,
#25678,#25679,#25680,#25681,#25682,#25683,#25684,#25685,#25686,#25687,#25688,
#25689,#25690,#25691,#25692,#25693,#25694,#25695,#25696,#25697,#25698,#25699,
#25700,#25701,#25702,#25703,#25704,#25705,#25706,#25707,#25708,#25709,#25710,
#25711,#25712,#25713,#25714,#25715,#25716,#25717,#25718,#25719,#25720,#25721,
#25722,#25723,#25724,#25725,#25726,#25727,#25728,#25729,#25730,#25731,#25732,
#25733,#25734,#25735,#25736,#25737,#25738,#25739),.UNSPECIFIED.,.F.,.F.,
(4,3,3,3,3,3,3,3,3,3,3,3,3,3,3,3,3,3,3,3,3,3,3,3,3,3,3,3,3,3,3,3,3,3,3,
3,3,3,3,3,3,3,3,3,4),(-326.374916364295,-326.21983494529,-326.064772095614,
-325.909746049644,-325.754364066725,-325.606323628372,-325.448897769932,
-325.291761513322,-325.134794018582,-324.977745909429,-324.820649815232,
-324.663214154262,-324.607531224604,-324.450105366164,-324.292969109553,
-324.136001614814,-323.978953505661,-323.821857411464,-323.664421750494,
-323.608738820836,-323.451312962395,-323.294176705785,-323.137209211046,
-322.980161101892,-322.823065007695,-322.665629346725,-322.609946417068,
-322.452520558628,-322.295384302017,-322.138416807278,-321.981368698125,
-321.824272603927,-321.666836942957,-321.6111540133,-321.45372815486,-321.296591898249,
-321.13962440351,-320.982576294357,-320.825480200159,-320.668044539189,
-320.612361609532,-320.448407729625,-320.284879993641,-320.121782250729,
-320.091731057115),.UNSPECIFIED.);
#683=B_SPLINE_CURVE_WITH_KNOTS('',3,(#25741,#25742,#25743,#25744,#25745,
#25746,#25747,#25748,#25749,#25750),.UNSPECIFIED.,.F.,.F.,(4,1,1,1,1,1,
1,4),(-320.091729415284,-319.613569205764,-318.614776801996,-317.615984398228,
-316.61719199446,-315.618399590692,-314.619607186924,-313.808550197804),
 .UNSPECIFIED.);
#684=B_SPLINE_CURVE_WITH_KNOTS('',3,(#25752,#25753,#25754,#25755,#25756,
#25757,#25758,#25759,#25760,#25761,#25762,#25763,#25764,#25765,#25766,#25767,
#25768,#25769,#25770,#25771,#25772,#25773,#25774,#25775,#25776,#25777,#25778,
#25779,#25780,#25781,#25782,#25783,#25784,#25785,#25786,#25787,#25788,#25789,
#25790,#25791,#25792,#25793,#25794,#25795,#25796,#25797,#25798,#25799,#25800,
#25801,#25802,#25803,#25804,#25805,#25806,#25807,#25808,#25809,#25810,#25811,
#25812,#25813,#25814,#25815,#25816,#25817,#25818,#25819,#25820,#25821,#25822,
#25823,#25824,#25825,#25826,#25827,#25828,#25829,#25830,#25831,#25832,#25833,
#25834,#25835,#25836,#25837,#25838,#25839,#25840,#25841,#25842,#25843,#25844,
#25845,#25846,#25847,#25848,#25849,#25850,#25851,#25852,#25853,#25854,#25855,
#25856,#25857,#25858,#25859,#25860,#25861,#25862,#25863,#25864,#25865,#25866,
#25867,#25868,#25869,#25870,#25871,#25872,#25873,#25874,#25875,#25876,#25877,
#25878,#25879,#25880,#25881,#25882,#25883,#25884),.UNSPECIFIED.,.F.,.F.,
(4,3,3,3,3,3,3,3,3,3,3,3,3,3,3,3,3,3,3,3,3,3,3,3,3,3,3,3,3,3,3,3,3,3,3,
3,3,3,3,3,3,3,3,3,4),(-313.808545749936,-313.620814783156,-313.463388924717,
-313.306252668109,-313.149285173372,-312.992237064221,-312.835140970025,
-312.677705309057,-312.622022379388,-312.464596520947,-312.307460264337,
-312.150492769598,-311.993444660444,-311.836348566246,-311.678912905276,
-311.62322997562,-311.465804117179,-311.308667860569,-311.151700365829,
-310.994652256676,-310.837556162478,-310.680120501508,-310.624437571852,
-310.467011713412,-310.309875456802,-310.152907962063,-309.995859852909,
-309.838763758712,-309.681328097742,-309.625645168084,-309.468219309644,
-309.311083053033,-309.154115558294,-308.997067449141,-308.839971354943,
-308.682535693973,-308.626852764316,-308.469426905875,-308.312290649265,
-308.155323154526,-307.998275045372,-307.841178951175,-307.683743290205,
-307.628060360548,-307.525360442756),.UNSPECIFIED.);
#685=B_SPLINE_CURVE_WITH_KNOTS('',3,(#25886,#25887,#25888,#25889,#25890,
#25891,#25892,#25893,#25894,#25895,#25896,#25897,#25898,#25899,#25900,#25901,
#25902,#25903,#25904,#25905,#25906,#25907,#25908,#25909,#25910,#25911,#25912,
#25913,#25914,#25915,#25916,#25917,#25918,#25919,#25920,#25921,#25922,#25923,
#25924,#25925,#25926,#25927,#25928,#25929,#25930,#25931,#25932,#25933,#25934,
#25935,#25936,#25937,#25938,#25939,#25940,#25941,#25942,#25943,#25944,#25945,
#25946,#25947,#25948,#25949,#25950,#25951,#25952,#25953,#25954,#25955,#25956,
#25957,#25958,#25959,#25960,#25961,#25962,#25963,#25964,#25965,#25966,#25967,
#25968,#25969,#25970,#25971,#25972,#25973,#25974,#25975,#25976,#25977,#25978,
#25979,#25980,#25981,#25982,#25983,#25984,#25985,#25986,#25987,#25988,#25989,
#25990,#25991,#25992,#25993,#25994,#25995,#25996,#25997,#25998,#25999,#26000,
#26001,#26002,#26003,#26004,#26005,#26006,#26007,#26008,#26009,#26010,#26011,
#26012,#26013,#26014,#26015,#26016,#26017,#26018),.UNSPECIFIED.,.F.,.F.,
(4,3,3,3,3,3,3,3,3,3,3,3,3,3,3,3,3,3,3,3,3,3,3,3,3,3,3,3,3,3,3,3,3,3,3,
3,3,3,3,3,3,3,3,3,4),(-307.52536044253,-307.37001604778,-307.214924493805,
-307.05983056049,-306.904753186811,-306.749329999325,-306.62926795678,-306.47184209834,
-306.314705841729,-306.15773834699,-306.000690237837,-305.84359414364,-305.686158482669,
-305.630475553012,-305.473049694572,-305.315913437961,-305.158945943222,
-305.001897834069,-304.844801739871,-304.687366078901,-304.631683149244,
-304.474257290804,-304.317121034193,-304.160153539454,-304.003105430301,
-303.846009336103,-303.688573675134,-303.632890745476,-303.475464887036,
-303.318328630425,-303.161361135686,-303.004313026533,-302.847216932335,
-302.689781271365,-302.634098341708,-302.476672483268,-302.319536226657,
-302.162568731918,-302.005520622765,-301.848424528568,-301.690988867598,
-301.63530593794,-301.459521411222,-301.285103403596,-301.242175365152),
 .UNSPECIFIED.);
#686=B_SPLINE_CURVE_WITH_KNOTS('',3,(#26020,#26021,#26022,#26023,#26024,
#26025,#26026,#26027,#26028,#26029),.UNSPECIFIED.,.F.,.F.,(4,1,1,1,1,1,
1,4),(-301.242175135576,-300.636513534172,-299.637721130404,-298.638928726636,
-297.640136322868,-296.6413439191,-295.642551515332,-294.958989828397),
 .UNSPECIFIED.);
#687=B_SPLINE_CURVE_WITH_KNOTS('',3,(#26031,#26032,#26033,#26034,#26035,
#26036,#26037,#26038,#26039,#26040,#26041,#26042,#26043,#26044,#26045,#26046,
#26047,#26048,#26049,#26050,#26051,#26052,#26053,#26054,#26055,#26056,#26057,
#26058,#26059,#26060,#26061,#26062,#26063,#26064,#26065,#26066,#26067,#26068,
#26069,#26070,#26071,#26072,#26073,#26074,#26075,#26076,#26077,#26078,#26079,
#26080,#26081,#26082,#26083,#26084,#26085,#26086,#26087,#26088,#26089,#26090,
#26091,#26092,#26093,#26094,#26095,#26096,#26097,#26098,#26099,#26100,#26101,
#26102,#26103,#26104,#26105,#26106,#26107,#26108,#26109,#26110,#26111,#26112,
#26113,#26114,#26115,#26116,#26117,#26118,#26119,#26120,#26121,#26122,#26123,
#26124,#26125,#26126,#26127,#26128,#26129,#26130,#26131,#26132,#26133,#26134,
#26135,#26136,#26137,#26138,#26139,#26140,#26141,#26142,#26143,#26144,#26145,
#26146,#26147,#26148,#26149,#26150,#26151,#26152,#26153,#26154,#26155,#26156,
#26157,#26158,#26159,#26160,#26161,#26162,#26163),.UNSPECIFIED.,.F.,.F.,
(4,3,3,3,3,3,3,3,3,3,3,3,3,3,3,3,3,3,3,3,3,3,3,3,3,3,3,3,3,3,3,3,3,3,3,
3,3,3,3,3,3,3,3,3,4),(-294.958989620074,-294.771703088725,-294.643759111564,
-294.486333253124,-294.329196996514,-294.172229501775,-294.015181392622,
-293.858085298424,-293.700649637455,-293.644966707796,-293.487540849356,
-293.330404592745,-293.173437098006,-293.016388988853,-292.859292894655,
-292.701857233685,-292.646174304028,-292.488748445588,-292.331612188977,
-292.174644694238,-292.017596585085,-291.860500490887,-291.703064829917,
-291.64738190026,-291.48995604182,-291.332819785209,-291.17585229047,-291.018804181317,
-290.861708087119,-290.704272426149,-290.648589496492,-290.491163638052,
-290.334027381441,-290.177059886702,-290.020011777549,-289.862915683352,
-289.705480022382,-289.649797092724,-289.493023928706,-289.336539147324,
-289.180219794627,-289.023819424796,-288.867364041646,-288.710580833308,
-288.675804521405),.UNSPECIFIED.);
#688=B_SPLINE_CURVE_WITH_KNOTS('',3,(#26165,#26166,#26167,#26168,#26169,
#26170,#26171,#26172,#26173,#26174,#26175,#26176,#26177,#26178,#26179,#26180,
#26181,#26182,#26183,#26184,#26185,#26186,#26187,#26188,#26189,#26190,#26191,
#26192,#26193,#26194,#26195,#26196,#26197,#26198,#26199,#26200,#26201,#26202,
#26203,#26204,#26205,#26206,#26207,#26208,#26209,#26210,#26211,#26212,#26213,
#26214,#26215,#26216,#26217,#26218,#26219,#26220,#26221,#26222,#26223,#26224,
#26225,#26226,#26227,#26228,#26229,#26230,#26231,#26232,#26233,#26234,#26235,
#26236,#26237,#26238,#26239,#26240,#26241,#26242,#26243,#26244,#26245,#26246,
#26247,#26248,#26249,#26250,#26251,#26252,#26253,#26254,#26255,#26256,#26257,
#26258,#26259,#26260,#26261,#26262,#26263,#26264,#26265,#26266,#26267,#26268,
#26269,#26270,#26271,#26272,#26273,#26274,#26275,#26276,#26277,#26278,#26279,
#26280,#26281,#26282,#26283,#26284,#26285,#26286,#26287,#26288,#26289,#26290,
#26291,#26292,#26293,#26294,#26295,#26296,#26297,#26298,#26299,#26300),
 .UNSPECIFIED.,.F.,.F.,(4,3,3,3,3,3,3,3,3,3,3,3,3,3,3,3,3,3,3,3,3,3,3,3,
3,3,3,3,3,3,3,3,3,3,3,3,3,3,3,3,3,3,3,3,3,4),(-288.675804521217,-288.651004688956,
-288.493578830515,-288.336442573905,-288.179475079166,-288.022426970012,
-287.865330875815,-287.707895214845,-287.652212285188,-287.494786426748,
-287.337650170137,-287.180682675398,-287.023634566245,-286.866538472047,
-286.709102811077,-286.65341988142,-286.49599402298,-286.338857766369,-286.18189027163,
-286.024842162477,-285.867746068279,-285.710310407309,-285.654627477652,
-285.497201619212,-285.340065362601,-285.183097867862,-285.026049758709,
-284.868953664511,-284.711518003541,-284.655835073884,-284.498409215444,
-284.341272958833,-284.184305464094,-284.027257354941,-283.870161260743,
-283.712725599773,-283.657042670116,-283.499616811676,-283.342480555065,
-283.185513060326,-283.028464951173,-282.871368856975,-282.713933196005,
-282.658250266348,-282.459103445106,-282.392619214225),.UNSPECIFIED.);
#689=B_SPLINE_CURVE_WITH_KNOTS('',3,(#26302,#26303,#26304,#26305,#26306,
#26307,#26308,#26309,#26310,#26311,#26312,#26313,#26314,#26315,#26316,#26317,
#26318,#26319,#26320,#26321,#26322,#26323,#26324,#26325,#26326,#26327,#26328,
#26329,#26330,#26331,#26332,#26333,#26334,#26335,#26336,#26337,#26338,#26339,
#26340,#26341,#26342,#26343,#26344,#26345,#26346,#26347,#26348,#26349,#26350,
#26351,#26352,#26353,#26354,#26355,#26356,#26357,#26358,#26359,#26360,#26361,
#26362,#26363,#26364,#26365,#26366,#26367,#26368,#26369,#26370,#26371,#26372,
#26373,#26374,#26375,#26376,#26377,#26378,#26379,#26380,#26381,#26382,#26383,
#26384,#26385,#26386,#26387,#26388,#26389,#26390,#26391,#26392,#26393,#26394,
#26395,#26396,#26397,#26398,#26399,#26400,#26401,#26402,#26403,#26404,#26405,
#26406,#26407,#26408,#26409,#26410,#26411,#26412,#26413,#26414,#26415,#26416,
#26417,#26418,#26419,#26420,#26421,#26422,#26423,#26424,#26425,#26426,#26427,
#26428,#26429,#26430,#26431,#26432,#26433,#26434),.UNSPECIFIED.,.F.,.F.,
(4,3,3,3,3,3,3,3,3,3,3,3,3,3,3,3,3,3,3,3,3,3,3,3,3,3,3,3,3,3,3,3,3,3,3,
3,3,3,3,3,3,3,3,3,4),(-282.392619214038,-282.237144823419,-282.08164941839,
-281.926157026577,-281.770314486552,-281.65945786258,-281.50203200414,-281.344895747529,
-281.18792825279,-281.030880143637,-280.873784049439,-280.716348388469,
-280.660665458812,-280.503239600372,-280.346103343761,-280.189135849022,
-280.032087739869,-279.874991645671,-279.717555984701,-279.661873055044,
-279.504447196604,-279.347310939993,-279.190343445254,-279.033295336101,
-278.876199241903,-278.718763580933,-278.663080651276,-278.505654792836,
-278.348518536225,-278.191551041486,-278.034502932333,-277.877406838136,
-277.719971177166,-277.664288247508,-277.506862389068,-277.349726132458,
-277.192758637719,-277.035710528565,-276.878614434368,-276.721178773398,
-276.66549584374,-276.50366837988,-276.342216082717,-276.181083091226,-276.109433906858),
 .UNSPECIFIED.);
#690=B_SPLINE_CURVE_WITH_KNOTS('',3,(#26436,#26437,#26438,#26439,#26440,
#26441,#26442,#26443,#26444,#26445),.UNSPECIFIED.,.F.,.F.,(4,1,1,1,1,1,
1,4),(-276.109429479534,-275.666703439972,-274.667911036204,-273.669118632436,
-272.670326228668,-271.6715338249,-270.672741421132,-269.8262558826),
 .UNSPECIFIED.);
#691=B_SPLINE_CURVE_WITH_KNOTS('',3,(#26447,#26448,#26449,#26450,#26451,
#26452,#26453,#26454,#26455,#26456,#26457,#26458,#26459,#26460,#26461,#26462,
#26463,#26464,#26465,#26466,#26467,#26468,#26469,#26470,#26471,#26472,#26473,
#26474,#26475,#26476,#26477,#26478,#26479,#26480,#26481,#26482,#26483,#26484,
#26485,#26486,#26487,#26488,#26489,#26490,#26491,#26492,#26493,#26494,#26495,
#26496,#26497,#26498,#26499,#26500,#26501,#26502,#26503,#26504,#26505,#26506,
#26507,#26508,#26509,#26510,#26511,#26512,#26513,#26514,#26515,#26516,#26517,
#26518,#26519,#26520,#26521,#26522,#26523,#26524,#26525,#26526,#26527,#26528,
#26529,#26530,#26531,#26532,#26533,#26534,#26535,#26536,#26537,#26538,#26539,
#26540,#26541,#26542,#26543,#26544,#26545,#26546,#26547,#26548,#26549,#26550,
#26551,#26552,#26553,#26554,#26555,#26556,#26557,#26558,#26559,#26560,#26561,
#26562,#26563,#26564,#26565,#26566,#26567,#26568,#26569,#26570,#26571,#26572,
#26573,#26574,#26575,#26576,#26577,#26578,#26579),.UNSPECIFIED.,.F.,.F.,
(4,3,3,3,3,3,3,3,3,3,3,3,3,3,3,3,3,3,3,3,3,3,3,3,3,3,3,3,3,3,3,3,3,3,3,
3,3,3,3,3,3,3,3,3,4),(-269.826248599679,-269.673949017364,-269.516523158924,
-269.359386902313,-269.202419407574,-269.04537129842,-268.888275204223,
-268.730839543253,-268.675156613596,-268.517730755156,-268.360594498545,
-268.203627003806,-268.046578894653,-267.889482800455,-267.732047139485,
-267.676364209828,-267.518938351388,-267.361802094777,-267.204834600038,
-267.047786490885,-266.890690396687,-266.733254735717,-266.67757180606,
-266.52014594762,-266.363009691009,-266.20604219627,-266.048994087117,-265.891897992919,
-265.734462331949,-265.678779402292,-265.521353543852,-265.364217287242,
-265.207249792503,-265.050201683349,-264.893105589152,-264.735669928182,
-264.679986998524,-264.522561140083,-264.365424883473,-264.208457388733,
-264.051409279579,-263.894313185381,-263.736877524411,-263.681194594755,
-263.543063292499),.UNSPECIFIED.);
#692=B_SPLINE_CURVE_WITH_KNOTS('',3,(#26581,#26582,#26583,#26584,#26585,
#26586,#26587,#26588,#26589,#26590),.UNSPECIFIED.,.F.,.F.,(4,1,1,1,1,1,
1,4),(-263.543055204836,-262.682402190987,-261.683609787219,-260.684817383451,
-259.686024979683,-258.687232575916,-257.688440172147,-257.259883482651),
 .UNSPECIFIED.);
#693=B_SPLINE_CURVE_WITH_KNOTS('',3,(#26592,#26593,#26594,#26595,#26596,
#26597,#26598,#26599,#26600,#26601,#26602,#26603,#26604,#26605,#26606,#26607,
#26608,#26609,#26610,#26611,#26612,#26613,#26614,#26615,#26616,#26617,#26618,
#26619,#26620,#26621,#26622,#26623,#26624,#26625,#26626,#26627,#26628,#26629,
#26630,#26631,#26632,#26633,#26634,#26635,#26636,#26637,#26638,#26639,#26640,
#26641,#26642,#26643,#26644,#26645,#26646,#26647,#26648,#26649,#26650,#26651,
#26652,#26653,#26654,#26655,#26656,#26657,#26658,#26659,#26660,#26661,#26662,
#26663,#26664,#26665,#26666,#26667,#26668,#26669,#26670,#26671,#26672,#26673,
#26674,#26675,#26676,#26677,#26678,#26679,#26680,#26681,#26682,#26683,#26684,
#26685,#26686,#26687,#26688,#26689,#26690,#26691,#26692,#26693,#26694,#26695,
#26696,#26697,#26698,#26699,#26700,#26701,#26702,#26703,#26704,#26705,#26706,
#26707,#26708,#26709,#26710,#26711,#26712,#26713,#26714,#26715,#26716,#26717,
#26718,#26719,#26720,#26721,#26722,#26723,#26724),.UNSPECIFIED.,.F.,.F.,
(4,3,3,3,3,3,3,3,3,3,3,3,3,3,3,3,3,3,3,3,3,3,3,3,3,3,3,3,3,3,3,3,3,3,3,
3,3,3,3,3,3,3,3,3,4),(-257.259877985319,-257.09937952014,-256.93874742661,
-256.777648047078,-256.689647768379,-256.532221909939,-256.375085653328,
-256.218118158589,-256.061070049436,-255.903973955238,-255.746538294268,
-255.690855364611,-255.533429506171,-255.37629324956,-255.219325754821,
-255.062277645668,-254.905181551471,-254.7477458905,-254.692062960843,-254.534637102403,
-254.377500845792,-254.220533351053,-254.0634852419,-253.906389147702,-253.748953486732,
-253.693270557075,-253.535844698635,-253.378708442024,-253.221740947285,
-253.064692838132,-252.907596743934,-252.750161082964,-252.694478153307,
-252.537052294866,-252.379916038256,-252.222948543517,-252.065900434364,
-251.908804340166,-251.751368679196,-251.695685749539,-251.539571791047,
-251.383743775657,-251.228086863493,-251.072362179131,-250.97669267814),
 .UNSPECIFIED.);
#694=B_SPLINE_CURVE_WITH_KNOTS('',3,(#26726,#26727,#26728,#26729,#26730,
#26731,#26732,#26733,#26734,#26735,#26736,#26737,#26738,#26739,#26740,#26741,
#26742,#26743,#26744,#26745,#26746,#26747,#26748,#26749,#26750,#26751,#26752,
#26753,#26754,#26755,#26756,#26757,#26758,#26759,#26760,#26761,#26762,#26763,
#26764,#26765,#26766,#26767,#26768,#26769,#26770,#26771,#26772,#26773,#26774,
#26775,#26776,#26777,#26778,#26779,#26780,#26781,#26782,#26783,#26784,#26785,
#26786,#26787,#26788,#26789,#26790,#26791,#26792,#26793,#26794,#26795,#26796,
#26797,#26798,#26799,#26800,#26801,#26802,#26803,#26804,#26805,#26806,#26807,
#26808,#26809,#26810,#26811,#26812,#26813,#26814,#26815,#26816,#26817,#26818,
#26819,#26820,#26821,#26822,#26823,#26824,#26825,#26826,#26827,#26828,#26829,
#26830,#26831,#26832,#26833,#26834,#26835,#26836,#26837,#26838,#26839,#26840,
#26841,#26842,#26843,#26844,#26845,#26846,#26847,#26848,#26849,#26850,#26851,
#26852,#26853,#26854,#26855,#26856,#26857,#26858,#26859,#26860,#26861),
 .UNSPECIFIED.,.F.,.F.,(4,3,3,3,3,3,3,3,3,3,3,3,3,3,3,3,3,3,3,3,3,3,3,3,
3,3,3,3,3,3,3,3,3,3,3,3,3,3,3,3,3,3,3,3,3,4),(-250.976692678011,-250.781410048543,
-250.696893345771,-250.539467487331,-250.382331230722,-250.225363735984,
-250.068315626831,-249.911219532634,-249.753783871665,-249.698100942003,
-249.540675083563,-249.383538826952,-249.226571332213,-249.06952322306,
-248.912427128862,-248.754991467892,-248.699308538235,-248.541882679794,
-248.384746423184,-248.227778928445,-248.070730819291,-247.913634725094,
-247.756199064124,-247.700516134467,-247.543090276027,-247.385954019416,
-247.228986524677,-247.071938415524,-246.914842321327,-246.757406660357,
-246.701723730699,-246.544297872259,-246.387161615648,-246.230194120909,
-246.073146011756,-245.916049917558,-245.758614256588,-245.702931326931,
-245.545505468491,-245.388369211881,-245.231401717141,-245.074353607988,
-244.917257513791,-244.759821852821,-244.704138923163,-244.69350737096),
 .UNSPECIFIED.);
#695=B_SPLINE_CURVE_WITH_KNOTS('',3,(#26863,#26864,#26865,#26866,#26867,
#26868,#26869,#26870,#26871,#26872,#26873,#26874,#26875,#26876,#26877,#26878,
#26879,#26880,#26881,#26882,#26883,#26884,#26885,#26886,#26887,#26888,#26889,
#26890,#26891,#26892,#26893,#26894,#26895,#26896,#26897,#26898,#26899,#26900,
#26901,#26902,#26903,#26904,#26905,#26906,#26907,#26908,#26909,#26910,#26911,
#26912,#26913,#26914,#26915,#26916,#26917,#26918,#26919,#26920,#26921,#26922,
#26923,#26924,#26925,#26926,#26927,#26928,#26929,#26930,#26931,#26932,#26933,
#26934,#26935,#26936,#26937,#26938,#26939,#26940,#26941,#26942,#26943,#26944,
#26945,#26946,#26947,#26948,#26949,#26950,#26951,#26952,#26953,#26954,#26955,
#26956,#26957,#26958,#26959,#26960,#26961,#26962,#26963,#26964,#26965,#26966,
#26967,#26968,#26969,#26970,#26971,#26972,#26973,#26974,#26975,#26976,#26977,
#26978,#26979,#26980,#26981,#26982,#26983,#26984,#26985,#26986,#26987,#26988,
#26989,#26990,#26991,#26992,#26993,#26994,#26995),.UNSPECIFIED.,.F.,.F.,
(4,3,3,3,3,3,3,3,3,3,3,3,3,3,3,3,3,3,3,3,3,3,3,3,3,3,3,3,3,3,3,3,3,3,3,
3,3,3,3,3,3,3,3,3,4),(-244.693507370801,-244.536376405573,-244.379534057459,
-244.222858503389,-244.066101113119,-243.909292124089,-243.752147502817,
-243.705346519395,-243.547920660955,-243.390784404344,-243.233816909605,
-243.076768800452,-242.919672706254,-242.762237045284,-242.706554115627,
-242.549128257187,-242.391992000576,-242.235024505837,-242.077976396684,
-241.920880302486,-241.763444641516,-241.707761711859,-241.550335853419,
-241.393199596808,-241.236232102069,-241.079183992916,-240.922087898719,
-240.764652237749,-240.708969308091,-240.551543449651,-240.39440719304,
-240.237439698301,-240.080391589148,-239.92329549495,-239.76585983398,-239.710176904323,
-239.552751045882,-239.395614789272,-239.238647294533,-239.081599185379,
-238.924503091182,-238.767067430211,-238.711384500555,-238.521147976858,
-238.410322247389),.UNSPECIFIED.);
#696=B_SPLINE_CURVE_WITH_KNOTS('',3,(#26997,#26998,#26999,#27000,#27001,
#27002,#27003,#27004,#27005,#27006),.UNSPECIFIED.,.F.,.F.,(4,1,1,1,1,1,
1,4),(-238.410322063781,-237.712592096787,-236.713799693019,-235.715007289251,
-234.716214885483,-233.717422481715,-232.718630077947,-232.127136756601),
 .UNSPECIFIED.);
#697=B_SPLINE_CURVE_WITH_KNOTS('',3,(#27008,#27009,#27010,#27011,#27012,
#27013,#27014,#27015,#27016,#27017,#27018,#27019,#27020,#27021,#27022,#27023,
#27024,#27025,#27026,#27027,#27028,#27029,#27030,#27031,#27032,#27033,#27034,
#27035,#27036,#27037,#27038,#27039,#27040,#27041,#27042,#27043,#27044,#27045,
#27046,#27047,#27048,#27049,#27050,#27051,#27052,#27053,#27054,#27055,#27056,
#27057,#27058,#27059,#27060,#27061,#27062,#27063,#27064,#27065,#27066,#27067,
#27068,#27069,#27070,#27071,#27072,#27073,#27074,#27075,#27076,#27077,#27078,
#27079,#27080,#27081,#27082,#27083,#27084,#27085,#27086,#27087,#27088,#27089,
#27090,#27091,#27092,#27093,#27094,#27095,#27096,#27097,#27098,#27099,#27100,
#27101,#27102,#27103,#27104,#27105,#27106,#27107,#27108,#27109,#27110,#27111,
#27112,#27113,#27114,#27115,#27116,#27117,#27118,#27119,#27120,#27121,#27122,
#27123,#27124,#27125,#27126,#27127,#27128,#27129,#27130,#27131,#27132,#27133,
#27134,#27135,#27136,#27137,#27138,#27139,#27140),.UNSPECIFIED.,.F.,.F.,
(4,3,3,3,3,3,3,3,3,3,3,3,3,3,3,3,3,3,3,3,3,3,3,3,3,3,3,3,3,3,3,3,3,3,3,
3,3,3,3,3,3,3,3,3,4),(-232.127136544053,-231.954428880424,-231.780471113885,
-231.719837674179,-231.562411815739,-231.405275559128,-231.248308064389,
-231.091259955236,-230.934163861038,-230.776728200068,-230.721045270411,
-230.563619411971,-230.40648315536,-230.249515660621,-230.092467551468,
-229.93537145727,-229.7779357963,-229.722252866643,-229.564827008203,-229.407690751592,
-229.250723256853,-229.0936751477,-228.936579053502,-228.779143392532,-228.723460462875,
-228.566034604435,-228.408898347824,-228.251930853085,-228.094882743932,
-227.937786649734,-227.780350988764,-227.724668059107,-227.567242200666,
-227.410105944056,-227.253138449317,-227.096090340163,-226.938994245966,
-226.781558584996,-226.725875655339,-226.570583424025,-226.415577817779,
-226.260626803486,-226.105720181143,-225.950529992756,-225.843951449422),
 .UNSPECIFIED.);
#698=B_SPLINE_CURVE_WITH_KNOTS('',3,(#27142,#27143,#27144,#27145,#27146,
#27147,#27148,#27149,#27150,#27151,#27152),.UNSPECIFIED.,.F.,.F.,(4,1,1,
1,1,1,1,1,4),(-225.843951449422,-225.727083251571,-224.728290847803,-223.729498444035,
-222.730706040267,-221.731913636499,-220.733121232731,-219.734328828963,
-219.560766142242),.UNSPECIFIED.);
#699=B_SPLINE_CURVE_WITH_KNOTS('',3,(#27154,#27155,#27156,#27157,#27158,
#27159,#27160,#27161,#27162,#27163,#27164,#27165,#27166,#27167,#27168,#27169,
#27170,#27171,#27172,#27173,#27174,#27175,#27176,#27177,#27178,#27179,#27180,
#27181,#27182,#27183,#27184,#27185,#27186,#27187,#27188,#27189,#27190,#27191,
#27192,#27193,#27194,#27195,#27196,#27197,#27198,#27199,#27200,#27201,#27202,
#27203,#27204,#27205,#27206,#27207,#27208,#27209,#27210,#27211,#27212,#27213,
#27214,#27215,#27216,#27217,#27218,#27219,#27220,#27221,#27222,#27223,#27224,
#27225,#27226,#27227,#27228,#27229,#27230,#27231,#27232,#27233,#27234,#27235,
#27236,#27237,#27238,#27239,#27240,#27241,#27242,#27243,#27244,#27245,#27246,
#27247,#27248,#27249,#27250,#27251,#27252,#27253,#27254,#27255,#27256,#27257,
#27258,#27259,#27260,#27261,#27262,#27263,#27264,#27265,#27266,#27267,#27268,
#27269,#27270,#27271,#27272,#27273,#27274,#27275,#27276,#27277,#27278,#27279,
#27280,#27281,#27282,#27283,#27284,#27285,#27286),.UNSPECIFIED.,.F.,.F.,
(4,3,3,3,3,3,3,3,3,3,3,3,3,3,3,3,3,3,3,3,3,3,3,3,3,3,3,3,3,3,3,3,3,3,3,
3,3,3,3,3,3,3,3,3,4),(-219.560766142242,-219.405885364159,-219.251206515928,
-219.096480412599,-218.941724077899,-218.786644708032,-218.735536425195,
-218.578110566755,-218.420974310144,-218.264006815405,-218.106958706252,
-217.949862612054,-217.792426951084,-217.736744021427,-217.579318162987,
-217.422181906376,-217.265214411637,-217.108166302484,-216.951070208286,
-216.793634547316,-216.737951617659,-216.580525759219,-216.423389502608,
-216.266422007869,-216.109373898716,-215.952277804518,-215.794842143548,
-215.739159213891,-215.581733355451,-215.42459709884,-215.267629604101,
-215.110581494948,-214.95348540075,-214.79604973978,-214.740366810123,-214.582940951683,
-214.425804695073,-214.268837200334,-214.111789091181,-213.954692996983,
-213.797257336014,-213.741574406355,-213.573311654301,-213.405853618667,
-213.277581026691),.UNSPECIFIED.);
#700=B_SPLINE_CURVE_WITH_KNOTS('',3,(#27288,#27289,#27290,#27291,#27292,
#27293,#27294,#27295,#27296,#27297),.UNSPECIFIED.,.F.,.F.,(4,1,1,1,1,1,
1,4),(-213.277580835062,-212.742782002587,-211.743989598819,-210.745197195051,
-209.746404791283,-208.747612387515,-207.748819983747,-206.994395527883),
 .UNSPECIFIED.);
#701=B_SPLINE_CURVE_WITH_KNOTS('',3,(#27299,#27300,#27301,#27302,#27303,
#27304,#27305,#27306,#27307,#27308,#27309,#27310,#27311,#27312,#27313,#27314,
#27315,#27316,#27317,#27318,#27319,#27320,#27321,#27322,#27323,#27324,#27325,
#27326,#27327,#27328,#27329,#27330,#27331,#27332,#27333,#27334,#27335,#27336,
#27337,#27338,#27339,#27340,#27341,#27342,#27343,#27344,#27345,#27346,#27347,
#27348,#27349,#27350,#27351,#27352,#27353,#27354,#27355,#27356,#27357,#27358,
#27359,#27360,#27361,#27362,#27363,#27364,#27365,#27366,#27367,#27368,#27369,
#27370,#27371,#27372,#27373,#27374,#27375,#27376,#27377,#27378,#27379,#27380,
#27381,#27382,#27383,#27384,#27385,#27386,#27387,#27388,#27389,#27390,#27391,
#27392,#27393,#27394,#27395,#27396,#27397,#27398,#27399,#27400,#27401,#27402,
#27403,#27404,#27405,#27406,#27407,#27408,#27409,#27410,#27411,#27412,#27413,
#27414,#27415,#27416,#27417,#27418,#27419,#27420,#27421,#27422,#27423,#27424,
#27425,#27426,#27427,#27428,#27429,#27430,#27431,#27432,#27433,#27434),
 .UNSPECIFIED.,.F.,.F.,(4,3,3,3,3,3,3,3,3,3,3,3,3,3,3,3,3,3,3,3,3,3,3,3,
3,3,3,3,3,3,3,3,3,3,3,3,3,3,3,3,3,3,3,3,3,4),(-206.994395456771,-206.788485113507,
-206.750027579979,-206.592601721539,-206.435465464928,-206.278497970189,
-206.121449861036,-205.964353766838,-205.806918105868,-205.751235176211,
-205.593809317771,-205.43667306116,-205.279705566421,-205.122657457268,
-204.96556136307,-204.8081257021,-204.752442772443,-204.595016914003,-204.437880657392,
-204.280913162653,-204.1238650535,-203.966768959303,-203.809333298333,-203.753650368675,
-203.596224510235,-203.439088253624,-203.282120758885,-203.125072649732,
-202.967976555534,-202.810540894564,-202.754857964907,-202.597432106467,
-202.440295849856,-202.283328355117,-202.126280245964,-201.969184151766,
-201.811748490796,-201.756065561139,-201.598639702699,-201.441503446089,
-201.28453595135,-201.127487842197,-200.970391748,-200.81295608703,-200.757273157371,
-200.711210220703),.UNSPECIFIED.);
#702=B_SPLINE_CURVE_WITH_KNOTS('',3,(#27436,#27437,#27438,#27439,#27440,
#27441,#27442,#27443,#27444,#27445,#27446,#27447,#27448,#27449,#27450,#27451,
#27452,#27453,#27454,#27455,#27456,#27457,#27458,#27459,#27460,#27461,#27462,
#27463,#27464,#27465,#27466,#27467,#27468,#27469,#27470,#27471,#27472,#27473,
#27474,#27475,#27476,#27477,#27478,#27479,#27480,#27481,#27482,#27483,#27484,
#27485,#27486,#27487,#27488,#27489,#27490,#27491,#27492,#27493,#27494,#27495,
#27496,#27497,#27498,#27499,#27500,#27501,#27502,#27503,#27504,#27505,#27506,
#27507,#27508,#27509,#27510,#27511,#27512,#27513,#27514,#27515,#27516,#27517,
#27518,#27519,#27520,#27521,#27522,#27523,#27524,#27525,#27526,#27527,#27528,
#27529,#27530,#27531,#27532,#27533,#27534,#27535,#27536,#27537,#27538,#27539,
#27540,#27541,#27542,#27543,#27544,#27545,#27546,#27547,#27548,#27549,#27550,
#27551,#27552,#27553,#27554,#27555,#27556,#27557,#27558,#27559,#27560,#27561,
#27562,#27563,#27564,#27565),.UNSPECIFIED.,.F.,.F.,(4,3,3,3,3,3,3,3,3,3,
3,3,3,3,3,3,3,3,3,3,3,3,3,3,3,3,3,3,3,3,3,3,3,3,3,3,3,3,3,3,3,3,3,4),(-200.71121022055,
-200.554927857576,-200.39892543186,-200.238814262296,-200.08287729828,-199.920679025941,
-199.758480753603,-199.601054895162,-199.443918638552,-199.286951143813,
-199.129903034659,-198.972806940462,-198.815371279492,-198.759688349835,
-198.602262491394,-198.445126234784,-198.288158740045,-198.131110630891,
-197.974014536694,-197.816578875724,-197.760895946067,-197.603470087627,
-197.446333831017,-197.289366336277,-197.132318227124,-196.975222132927,
-196.817786471957,-196.762103542299,-196.604677683859,-196.447541427248,
-196.290573932509,-196.133525823356,-195.976429729158,-195.818994068188,
-195.763311138531,-195.605885280091,-195.44874902348,-195.291781528741,
-195.134733419588,-194.97763732539,-194.82020166442,-194.764518734763,-194.581155261081,
-194.428024913746),.UNSPECIFIED.);
#703=B_SPLINE_CURVE_WITH_KNOTS('',3,(#27567,#27568,#27569,#27570,#27571,
#27572,#27573,#27574,#27575,#27576,#27577,#27578,#27579,#27580,#27581,#27582,
#27583,#27584,#27585,#27586,#27587,#27588,#27589,#27590,#27591,#27592,#27593,
#27594,#27595,#27596,#27597,#27598,#27599,#27600,#27601,#27602,#27603,#27604,
#27605,#27606,#27607,#27608,#27609,#27610,#27611,#27612,#27613,#27614,#27615,
#27616,#27617,#27618,#27619,#27620,#27621,#27622,#27623,#27624,#27625,#27626,
#27627,#27628,#27629,#27630,#27631,#27632,#27633,#27634,#27635,#27636,#27637,
#27638,#27639,#27640,#27641,#27642,#27643,#27644,#27645,#27646,#27647,#27648,
#27649,#27650,#27651,#27652,#27653,#27654,#27655,#27656,#27657,#27658,#27659,
#27660,#27661,#27662,#27663,#27664,#27665,#27666,#27667,#27668,#27669,#27670,
#27671,#27672,#27673,#27674,#27675,#27676,#27677,#27678,#27679,#27680,#27681,
#27682,#27683,#27684,#27685,#27686,#27687,#27688,#27689,#27690,#27691,#27692,
#27693,#27694,#27695,#27696,#27697,#27698,#27699),.UNSPECIFIED.,.F.,.F.,
(4,3,3,3,3,3,3,3,3,3,3,3,3,3,3,3,3,3,3,3,3,3,3,3,3,3,3,3,3,3,3,3,3,3,3,
3,3,3,3,3,3,3,3,3,4),(-194.428024913524,-194.271102313192,-194.114059104038,
-193.956937816817,-193.799462526794,-193.765726330995,-193.608300472555,
-193.451164215944,-193.294196721205,-193.137148612052,-192.980052517854,
-192.822616856884,-192.766933927227,-192.609508068787,-192.452371812176,
-192.295404317437,-192.138356208284,-191.981260114086,-191.823824453116,
-191.768141523459,-191.610715665019,-191.453579408408,-191.296611913669,
-191.139563804516,-190.982467710318,-190.825032049348,-190.769349119691,
-190.611923261251,-190.45478700464,-190.297819509901,-190.140771400748,
-189.98367530655,-189.82623964558,-189.770556715923,-189.613130857483,-189.455994600873,
-189.299027106134,-189.14197899698,-188.984882902783,-188.827447241813,
-188.771764312155,-188.613149272119,-188.454850209973,-188.296688673262,
-188.144839606344),.UNSPECIFIED.);
#704=B_SPLINE_CURVE_WITH_KNOTS('',3,(#27701,#27702,#27703,#27704,#27705,
#27706,#27707,#27708,#27709,#27710),.UNSPECIFIED.,.F.,.F.,(4,1,1,1,1,1,
1,4),(-188.144832027655,-187.772971908386,-186.774179504619,-185.775387100851,
-184.776594697082,-183.777802293314,-182.779009889546,-181.861662808607),
 .UNSPECIFIED.);
#705=B_SPLINE_CURVE_WITH_KNOTS('',3,(#27712,#27713,#27714,#27715,#27716,
#27717,#27718,#27719,#27720,#27721,#27722,#27723,#27724,#27725,#27726,#27727,
#27728,#27729,#27730,#27731,#27732,#27733,#27734,#27735,#27736,#27737,#27738,
#27739,#27740,#27741,#27742,#27743,#27744,#27745,#27746,#27747,#27748,#27749,
#27750,#27751,#27752,#27753,#27754,#27755,#27756,#27757,#27758,#27759,#27760,
#27761,#27762,#27763,#27764,#27765,#27766,#27767,#27768,#27769,#27770,#27771,
#27772,#27773,#27774,#27775,#27776,#27777,#27778,#27779,#27780,#27781,#27782,
#27783,#27784,#27785,#27786,#27787,#27788,#27789,#27790,#27791,#27792,#27793,
#27794,#27795,#27796,#27797,#27798,#27799,#27800,#27801,#27802,#27803,#27804,
#27805,#27806,#27807,#27808,#27809,#27810,#27811,#27812,#27813,#27814,#27815,
#27816,#27817,#27818,#27819,#27820,#27821,#27822,#27823,#27824,#27825,#27826,
#27827,#27828,#27829,#27830,#27831,#27832,#27833,#27834,#27835,#27836,#27837,
#27838,#27839,#27840,#27841,#27842,#27843,#27844),.UNSPECIFIED.,.F.,.F.,
(4,3,3,3,3,3,3,3,3,3,3,3,3,3,3,3,3,3,3,3,3,3,3,3,3,3,3,3,3,3,3,3,3,3,3,
3,3,3,3,3,3,3,3,3,4),(-181.861654299165,-181.780217485778,-181.622791627338,
-181.465655370728,-181.308687875988,-181.151639766835,-180.994543672638,
-180.837108011668,-180.78142508201,-180.62399922357,-180.466862966959,-180.30989547222,
-180.152847363067,-179.995751268869,-179.838315607899,-179.782632678242,
-179.625206819802,-179.468070563191,-179.311103068452,-179.154054959299,
-178.996958865101,-178.839523204131,-178.783840274474,-178.626414416034,
-178.469278159423,-178.312310664684,-178.155262555531,-177.998166461333,
-177.840730800363,-177.785047870706,-177.627622012266,-177.470485755655,
-177.313518260916,-177.156470151763,-176.999374057565,-176.841938396595,
-176.786255466938,-176.628829608497,-176.471693351887,-176.314725857148,
-176.157677747994,-176.000581653797,-175.843145992827,-175.78746306317,
-175.578468991985),.UNSPECIFIED.);
#706=B_SPLINE_CURVE_WITH_KNOTS('',3,(#27846,#27847,#27848,#27849,#27850,
#27851,#27852,#27853,#27854,#27855),.UNSPECIFIED.,.F.,.F.,(4,1,1,1,1,1,
1,4),(-175.578466593548,-174.788670659402,-173.789878255634,-172.791085851866,
-171.792293448098,-170.79350104433,-169.794708640562,-169.295283684806),
 .UNSPECIFIED.);
#707=B_SPLINE_CURVE_WITH_KNOTS('',3,(#27857,#27858,#27859,#27860,#27861,
#27862,#27863,#27864,#27865,#27866),.UNSPECIFIED.,.F.,.F.,(4,1,1,1,1,1,
1,4),(-169.295283684806,-168.795916236794,-167.797123833026,-166.798331429258,
-165.79953902549,-164.800746621722,-163.801954217954,-163.012100781783),
 .UNSPECIFIED.);
#708=B_SPLINE_CURVE_WITH_KNOTS('',3,(#27868,#27869,#27870,#27871,#27872,
#27873,#27874,#27875,#27876,#27877,#27878,#27879,#27880,#27881,#27882,#27883,
#27884,#27885,#27886,#27887,#27888,#27889,#27890,#27891,#27892,#27893,#27894,
#27895,#27896,#27897,#27898,#27899,#27900,#27901,#27902,#27903,#27904,#27905,
#27906,#27907,#27908,#27909,#27910,#27911,#27912,#27913,#27914,#27915,#27916,
#27917,#27918,#27919,#27920,#27921,#27922,#27923,#27924,#27925,#27926,#27927,
#27928,#27929,#27930,#27931,#27932,#27933,#27934,#27935,#27936,#27937,#27938,
#27939,#27940,#27941,#27942,#27943,#27944,#27945,#27946,#27947,#27948,#27949,
#27950,#27951,#27952,#27953,#27954,#27955,#27956,#27957,#27958,#27959,#27960,
#27961,#27962,#27963,#27964,#27965,#27966,#27967,#27968,#27969,#27970,#27971,
#27972,#27973,#27974,#27975,#27976,#27977,#27978,#27979,#27980,#27981,#27982,
#27983,#27984,#27985,#27986,#27987,#27988,#27989,#27990,#27991,#27992,#27993,
#27994,#27995,#27996,#27997,#27998,#27999,#28000),.UNSPECIFIED.,.F.,.F.,
(4,3,3,3,3,3,3,3,3,3,3,3,3,3,3,3,3,3,3,3,3,3,3,3,3,3,3,3,3,3,3,3,3,3,3,
3,3,3,3,3,3,3,3,3,4),(-163.012098377626,-162.803161814186,-162.645735955746,
-162.488599699136,-162.331632204397,-162.174584095244,-162.017488001047,
-161.860052340077,-161.804369410418,-161.646943551978,-161.489807295367,
-161.332839800628,-161.175791691475,-161.018695597277,-160.861259936307,
-160.80557700665,-160.64815114821,-160.491014891599,-160.33404739686,-160.176999287707,
-160.019903193509,-159.862467532539,-159.806784602882,-159.649358744442,
-159.492222487831,-159.335254993092,-159.178206883939,-159.021110789741,
-158.863675128771,-158.807992199114,-158.650566340674,-158.493430084063,
-158.336462589324,-158.179414480171,-158.022318385973,-157.864882725003,
-157.809199795346,-157.651773936906,-157.494637680296,-157.337670185556,
-157.180622076403,-157.023525982206,-156.866090321236,-156.810407391578,
-156.728913070446),.UNSPECIFIED.);
#709=B_SPLINE_CURVE_WITH_KNOTS('',3,(#28002,#28003,#28004,#28005,#28006,
#28007,#28008,#28009,#28010,#28011),.UNSPECIFIED.,.F.,.F.,(4,1,1,1,1,1,
1,4),(-156.728904558766,-155.81161498781,-154.812822584042,-153.814030180274,
-152.815237776506,-151.816445372738,-150.81765296897,-150.445735341375),
 .UNSPECIFIED.);
#710=B_SPLINE_CURVE_WITH_KNOTS('',3,(#28013,#28014,#28015,#28016,#28017,
#28018,#28019,#28020,#28021,#28022,#28023,#28024,#28025,#28026,#28027,#28028,
#28029,#28030,#28031,#28032,#28033,#28034,#28035,#28036,#28037,#28038,#28039,
#28040,#28041,#28042,#28043,#28044,#28045,#28046,#28047,#28048,#28049,#28050,
#28051,#28052,#28053,#28054,#28055,#28056,#28057,#28058,#28059,#28060,#28061,
#28062,#28063,#28064,#28065,#28066,#28067,#28068,#28069,#28070,#28071,#28072,
#28073,#28074,#28075,#28076,#28077,#28078,#28079,#28080,#28081,#28082,#28083,
#28084,#28085,#28086,#28087,#28088,#28089,#28090,#28091,#28092,#28093,#28094,
#28095,#28096,#28097,#28098,#28099,#28100,#28101,#28102,#28103,#28104,#28105,
#28106,#28107,#28108,#28109,#28110,#28111,#28112,#28113,#28114,#28115,#28116,
#28117,#28118,#28119,#28120,#28121,#28122,#28123,#28124,#28125,#28126,#28127,
#28128,#28129,#28130,#28131,#28132,#28133,#28134,#28135,#28136,#28137,#28138,
#28139,#28140,#28141,#28142,#28143,#28144,#28145),.UNSPECIFIED.,.F.,.F.,
(4,3,3,3,3,3,3,3,3,3,3,3,3,3,3,3,3,3,3,3,3,3,3,3,3,3,3,3,3,3,3,3,3,3,3,
3,3,3,3,3,3,3,3,3,4),(-150.445727763267,-150.287559345543,-150.12936657424,
-149.970749373709,-149.818860565202,-149.661434706762,-149.504298450152,
-149.347330955412,-149.190282846259,-149.033186752062,-148.875751091092,
-148.820068161434,-148.662642302994,-148.505506046383,-148.348538551644,
-148.191490442491,-148.034394348293,-147.876958687323,-147.821275757666,
-147.663849899226,-147.506713642615,-147.349746147876,-147.192698038723,
-147.035601944525,-146.878166283555,-146.822483353898,-146.665057495458,
-146.507921238847,-146.350953744108,-146.193905634955,-146.036809540757,
-145.879373879787,-145.82369095013,-145.66626509169,-145.50912883508,-145.35216134034,
-145.195113231187,-145.03801713699,-144.88058147602,-144.824898546362,-144.659309523793,
-144.502171753509,-144.345219652649,-144.188289944736,-144.162542456087),
 .UNSPECIFIED.);
#711=B_SPLINE_CURVE_WITH_KNOTS('',3,(#28147,#28148,#28149,#28150,#28151,
#28152,#28153,#28154,#28155,#28156,#28157,#28158,#28159,#28160,#28161,#28162,
#28163,#28164,#28165,#28166,#28167,#28168,#28169,#28170,#28171,#28172,#28173,
#28174,#28175,#28176,#28177,#28178,#28179,#28180,#28181,#28182,#28183,#28184,
#28185,#28186,#28187,#28188,#28189,#28190,#28191,#28192,#28193,#28194,#28195,
#28196,#28197,#28198,#28199,#28200,#28201,#28202,#28203,#28204,#28205,#28206,
#28207,#28208,#28209,#28210,#28211,#28212,#28213,#28214,#28215,#28216,#28217,
#28218,#28219,#28220,#28221,#28222,#28223,#28224,#28225,#28226,#28227,#28228,
#28229,#28230,#28231,#28232,#28233,#28234,#28235,#28236,#28237,#28238,#28239,
#28240,#28241,#28242,#28243,#28244,#28245,#28246,#28247,#28248,#28249,#28250,
#28251,#28252,#28253,#28254,#28255,#28256,#28257,#28258,#28259,#28260,#28261,
#28262,#28263,#28264,#28265,#28266,#28267,#28268,#28269,#28270,#28271,#28272,
#28273,#28274,#28275,#28276),.UNSPECIFIED.,.F.,.F.,(4,3,3,3,3,3,3,3,3,3,
3,3,3,3,3,3,3,3,3,3,3,3,3,3,3,3,3,3,3,3,3,3,3,3,3,3,3,3,3,3,3,3,3,4),(-144.162542455865,
-143.979169095402,-143.826106142594,-143.668680284153,-143.511544027543,
-143.354576532803,-143.197528423649,-143.040432329451,-142.882996668481,
-142.827313738826,-142.669887880386,-142.512751623775,-142.355784129036,
-142.198736019883,-142.041639925685,-141.884204264715,-141.828521335058,
-141.671095476618,-141.513959220008,-141.356991725268,-141.199943616115,
-141.042847521918,-140.885411860948,-140.82972893129,-140.67230307285,-140.515166816239,
-140.3581993215,-140.201151212347,-140.044055118149,-139.886619457179,-139.830936527522,
-139.673510669082,-139.516374412471,-139.359406917732,-139.202358808579,
-139.045262714381,-138.887827053411,-138.832144123754,-138.675840847802,
-138.519825091293,-138.359708105736,-138.203776393364,-138.041566771214,
-137.879357149064),.UNSPECIFIED.);
#712=B_SPLINE_CURVE_WITH_KNOTS('',3,(#28278,#28279,#28280,#28281,#28282,
#28283,#28284,#28285,#28286,#28287,#28288,#28289,#28290,#28291,#28292,#28293,
#28294,#28295,#28296,#28297,#28298,#28299,#28300,#28301,#28302,#28303,#28304,
#28305,#28306,#28307,#28308,#28309,#28310,#28311,#28312,#28313,#28314,#28315,
#28316,#28317,#28318,#28319,#28320,#28321,#28322,#28323,#28324,#28325,#28326,
#28327,#28328,#28329,#28330,#28331,#28332,#28333,#28334,#28335,#28336,#28337,
#28338,#28339,#28340,#28341,#28342,#28343,#28344,#28345,#28346,#28347,#28348,
#28349,#28350,#28351,#28352,#28353,#28354,#28355,#28356,#28357,#28358,#28359,
#28360,#28361,#28362,#28363,#28364,#28365,#28366,#28367,#28368,#28369,#28370,
#28371,#28372,#28373,#28374,#28375,#28376,#28377,#28378,#28379,#28380,#28381,
#28382,#28383,#28384,#28385,#28386,#28387,#28388,#28389,#28390,#28391,#28392,
#28393,#28394,#28395,#28396,#28397,#28398,#28399,#28400,#28401,#28402,#28403,
#28404,#28405,#28406,#28407,#28408,#28409,#28410,#28411,#28412,#28413),
 .UNSPECIFIED.,.F.,.F.,(4,3,3,3,3,3,3,3,3,3,3,3,3,3,3,3,3,3,3,3,3,3,3,3,
3,3,3,3,3,3,3,3,3,3,3,3,3,3,3,3,3,3,3,3,3,4),(-137.879357148908,-137.833351719986,
-137.675925861546,-137.518789604935,-137.361822110196,-137.204774001043,
-137.047677906846,-136.890242245876,-136.834559316218,-136.677133457778,
-136.519997201167,-136.363029706428,-136.205981597275,-136.048885503077,
-135.891449842107,-135.83576691245,-135.67834105401,-135.521204797399,-135.36423730266,
-135.207189193507,-135.050093099309,-134.892657438339,-134.836974508682,
-134.679548650242,-134.522412393631,-134.365444898892,-134.208396789739,
-134.051300695541,-133.893865034571,-133.838182104914,-133.680756246474,
-133.523619989863,-133.366652495124,-133.209604385971,-133.052508291773,
-132.895072630803,-132.839389701146,-132.681963842706,-132.524827586096,
-132.367860091357,-132.210811982203,-132.053715888006,-131.896280227036,
-131.840597297378,-131.634707085204,-131.596171913192),.UNSPECIFIED.);
#713=B_SPLINE_CURVE_WITH_KNOTS('',3,(#28415,#28416,#28417,#28418,#28419,
#28420,#28421,#28422,#28423,#28424),.UNSPECIFIED.,.F.,.F.,(4,1,1,1,1,1,
1,4),(-131.596171841728,-130.84180489361,-129.843012489842,-128.844220086074,
-127.845427682306,-126.846635278538,-125.84784287477,-125.312986534549),
 .UNSPECIFIED.);
#714=B_SPLINE_CURVE_WITH_KNOTS('',3,(#28426,#28427,#28428,#28429,#28430,
#28431,#28432,#28433,#28434,#28435,#28436,#28437,#28438,#28439,#28440,#28441,
#28442,#28443,#28444,#28445,#28446,#28447,#28448,#28449,#28450,#28451,#28452,
#28453,#28454,#28455,#28456,#28457,#28458,#28459,#28460,#28461,#28462,#28463,
#28464,#28465,#28466,#28467,#28468,#28469,#28470,#28471,#28472,#28473,#28474,
#28475,#28476,#28477,#28478,#28479,#28480,#28481,#28482,#28483,#28484,#28485,
#28486,#28487,#28488,#28489,#28490,#28491,#28492,#28493,#28494,#28495,#28496,
#28497,#28498,#28499,#28500,#28501,#28502,#28503,#28504,#28505,#28506,#28507,
#28508,#28509,#28510,#28511,#28512,#28513,#28514,#28515,#28516,#28517,#28518,
#28519,#28520,#28521,#28522,#28523,#28524,#28525,#28526,#28527,#28528,#28529,
#28530,#28531,#28532,#28533,#28534,#28535,#28536,#28537,#28538,#28539,#28540,
#28541,#28542,#28543,#28544,#28545,#28546,#28547,#28548,#28549,#28550,#28551,
#28552,#28553,#28554,#28555,#28556,#28557,#28558),.UNSPECIFIED.,.F.,.F.,
(4,3,3,3,3,3,3,3,3,3,3,3,3,3,3,3,3,3,3,3,3,3,3,3,3,3,3,3,3,3,3,3,3,3,3,
3,3,3,3,3,3,3,3,3,4),(-125.312986342626,-125.145692167388,-124.977524770016,
-124.849050471002,-124.691624612562,-124.534488355952,-124.377520861213,
-124.220472752059,-124.063376657862,-123.905940996892,-123.850258067234,
-123.692832208794,-123.535695952183,-123.378728457444,-123.221680348291,
-123.064584254093,-122.907148593123,-122.851465663466,-122.694039805026,
-122.536903548415,-122.379936053676,-122.222887944523,-122.065791850325,
-121.908356189355,-121.852673259698,-121.695247401258,-121.538111144647,
-121.381143649908,-121.224095540755,-121.066999446557,-120.909563785587,
-120.85388085593,-120.69645499749,-120.539318740879,-120.38235124614,-120.225303136987,
-120.06820704279,-119.91077138182,-119.855088452162,-119.70000916941,-119.545219027811,
-119.390509726915,-119.235844442665,-119.080963609224,-119.029801227369),
 .UNSPECIFIED.);
#715=B_SPLINE_CURVE_WITH_KNOTS('',3,(#28560,#28561,#28562,#28563,#28564,
#28565,#28566,#28567,#28568,#28569,#28570),.UNSPECIFIED.,.F.,.F.,(4,1,1,
1,1,1,1,1,4),(-119.029801227369,-118.856296048394,-117.857503644626,-116.858711240858,
-115.85991883709,-114.861126433322,-113.862334029554,-112.863541625786,
-112.746615920189),.UNSPECIFIED.);
#716=B_SPLINE_CURVE_WITH_KNOTS('',3,(#28572,#28573,#28574,#28575,#28576,
#28577,#28578,#28579,#28580,#28581,#28582,#28583,#28584,#28585,#28586,#28587,
#28588,#28589,#28590,#28591,#28592,#28593,#28594,#28595,#28596,#28597,#28598,
#28599,#28600,#28601,#28602,#28603,#28604,#28605,#28606,#28607,#28608,#28609,
#28610,#28611,#28612,#28613,#28614,#28615,#28616,#28617,#28618,#28619,#28620,
#28621,#28622,#28623,#28624,#28625,#28626,#28627,#28628,#28629,#28630,#28631,
#28632,#28633,#28634,#28635,#28636,#28637,#28638,#28639,#28640,#28641,#28642,
#28643,#28644,#28645,#28646,#28647,#28648,#28649,#28650,#28651,#28652,#28653,
#28654,#28655,#28656,#28657,#28658,#28659,#28660,#28661,#28662,#28663,#28664,
#28665,#28666,#28667,#28668,#28669,#28670,#28671,#28672,#28673,#28674,#28675,
#28676,#28677,#28678,#28679,#28680,#28681,#28682,#28683,#28684,#28685,#28686,
#28687,#28688,#28689,#28690,#28691,#28692,#28693,#28694,#28695,#28696,#28697,
#28698,#28699,#28700,#28701,#28702,#28703,#28704),.UNSPECIFIED.,.F.,.F.,
(4,3,3,3,3,3,3,3,3,3,3,3,3,3,3,3,3,3,3,3,3,3,3,3,3,3,3,3,3,3,3,3,3,3,3,
3,3,3,3,3,3,3,3,3,4),(-112.746615920189,-112.591427658643,-112.436483398331,
-112.281528987221,-112.126582709523,-111.971296091352,-111.864749222017,
-111.707323363577,-111.550187106966,-111.393219612227,-111.236171503074,
-111.079075408876,-110.921639747906,-110.865956818249,-110.708530959809,
-110.551394703198,-110.394427208459,-110.237379099306,-110.080283005108,
-109.922847344138,-109.867164414481,-109.709738556041,-109.55260229943,
-109.395634804691,-109.238586695538,-109.08149060134,-108.92405494037,-108.868372010713,
-108.710946152273,-108.553809895662,-108.396842400923,-108.23979429177,
-108.082698197572,-107.925262536602,-107.869579606945,-107.712153748504,
-107.555017491894,-107.398049997155,-107.241001888001,-107.083905793803,
-106.926470132833,-106.870787203177,-106.696751389778,-106.523937038518,
-106.463430825477),.UNSPECIFIED.);
#717=B_SPLINE_CURVE_WITH_KNOTS('',3,(#28706,#28707,#28708,#28709,#28710,
#28711,#28712,#28713,#28714,#28715),.UNSPECIFIED.,.F.,.F.,(4,1,1,1,1,1,
1,4),(-106.46343061301,-105.871994799409,-104.873202395641,-103.874409991873,
-102.875617588105,-101.876825184337,-100.878032780569,-100.18024530583),
 .UNSPECIFIED.);
#718=B_SPLINE_CURVE_WITH_KNOTS('',3,(#28717,#28718,#28719,#28720,#28721,
#28722,#28723,#28724,#28725,#28726,#28727,#28728,#28729,#28730,#28731,#28732,
#28733,#28734,#28735,#28736,#28737,#28738,#28739,#28740,#28741,#28742,#28743,
#28744,#28745,#28746,#28747,#28748,#28749,#28750,#28751,#28752,#28753,#28754,
#28755,#28756,#28757,#28758,#28759,#28760,#28761,#28762,#28763,#28764,#28765,
#28766,#28767,#28768,#28769,#28770,#28771,#28772,#28773,#28774,#28775,#28776,
#28777,#28778,#28779,#28780,#28781,#28782,#28783,#28784,#28785,#28786,#28787,
#28788,#28789,#28790,#28791,#28792,#28793,#28794,#28795,#28796,#28797,#28798,
#28799,#28800,#28801,#28802,#28803,#28804,#28805,#28806,#28807,#28808,#28809,
#28810,#28811,#28812,#28813,#28814,#28815,#28816,#28817,#28818,#28819,#28820,
#28821,#28822,#28823,#28824,#28825,#28826,#28827,#28828,#28829,#28830,#28831,
#28832,#28833,#28834,#28835,#28836,#28837,#28838,#28839,#28840,#28841,#28842,
#28843,#28844,#28845,#28846,#28847,#28848,#28849),.UNSPECIFIED.,.F.,.F.,
(4,3,3,3,3,3,3,3,3,3,3,3,3,3,3,3,3,3,3,3,3,3,3,3,3,3,3,3,3,3,3,3,3,3,3,
3,3,3,3,3,3,3,3,3,4),(-100.180245122334,-99.9899960061537,-99.8792403768013,
-99.7218145183607,-99.5646782617502,-99.4077107670109,-99.2506626578573,
-99.0935665636596,-98.9361309026894,-98.8804479730333,-98.7230221145929,
-98.5658858579827,-98.4089183632435,-98.2518702540902,-98.0947741598927,
-97.9373384989227,-97.8816555692653,-97.7242297108249,-97.5670934542147,
-97.4101259594756,-97.2530778503222,-97.0959817561248,-96.9385460951547,
-96.8828631654973,-96.7254373070569,-96.5683010504466,-96.4113335557074,
-96.254285446554,-96.0971893523565,-95.9397536913864,-95.8840707617293,
-95.7266449032889,-95.5695086466786,-95.4125411519395,-95.2554930427861,
-95.0983969485886,-94.9409612876185,-94.8852783579613,-94.728144675395,
-94.571300053841,-94.4146226728758,-94.2578641017484,-94.1010543235121,
-93.9439094261303,-93.8970599988234),.UNSPECIFIED.);
#719=B_SPLINE_CURVE_WITH_KNOTS('',3,(#28851,#28852,#28853,#28854,#28855,
#28856,#28857,#28858,#28859,#28860,#28861,#28862,#28863,#28864,#28865,#28866,
#28867,#28868,#28869,#28870,#28871,#28872,#28873,#28874,#28875,#28876,#28877,
#28878,#28879,#28880,#28881,#28882,#28883,#28884,#28885,#28886,#28887,#28888,
#28889,#28890,#28891,#28892,#28893,#28894,#28895,#28896,#28897,#28898,#28899,
#28900,#28901,#28902,#28903,#28904,#28905,#28906,#28907,#28908,#28909,#28910,
#28911,#28912,#28913,#28914,#28915,#28916,#28917,#28918,#28919,#28920,#28921,
#28922,#28923,#28924,#28925,#28926,#28927,#28928,#28929,#28930,#28931,#28932,
#28933,#28934,#28935,#28936,#28937,#28938,#28939,#28940,#28941,#28942,#28943,
#28944,#28945,#28946,#28947,#28948,#28949,#28950,#28951,#28952,#28953,#28954,
#28955,#28956,#28957,#28958,#28959,#28960,#28961,#28962,#28963,#28964,#28965,
#28966,#28967,#28968,#28969,#28970,#28971,#28972,#28973,#28974,#28975,#28976,
#28977,#28978,#28979,#28980,#28981,#28982,#28983,#28984,#28985,#28986),
 .UNSPECIFIED.,.F.,.F.,(4,3,3,3,3,3,3,3,3,3,3,3,3,3,3,3,3,3,3,3,3,3,3,3,
3,3,3,3,3,3,3,3,3,3,3,3,3,3,3,3,3,3,3,3,3,4),(-93.8970599986506,-93.8864859541932,
-93.7290600957528,-93.5719238391426,-93.4149563444034,-93.25790823525,-93.1008121410525,
-92.9433764800825,-92.8876935504252,-92.7302676919848,-92.5731314353745,
-92.4161639406354,-92.259115831482,-92.1020197372846,-91.9445840763145,
-91.8889011466572,-91.7314752882168,-91.5743390316065,-91.4173715368674,
-91.260323427714,-91.1032273335165,-90.9457916725464,-90.8901087428892,
-90.7326828844488,-90.5755466278386,-90.4185791330994,-90.261531023946,
-90.1044349297486,-89.9469992687786,-89.8913163391212,-89.7338904806808,
-89.5767542240706,-89.4197867293314,-89.262738620178,-89.1056425259805,
-88.9482068650105,-88.8925239353532,-88.7350980769127,-88.5779618203025,
-88.4209943255633,-88.2639462164099,-88.1068501222124,-87.9494144612423,
-87.8937315315851,-87.6984636965869,-87.6138746916003),.UNSPECIFIED.);
#720=B_SPLINE_CURVE_WITH_KNOTS('',3,(#28988,#28989,#28990,#28991,#28992,
#28993,#28994,#28995,#28996,#28997,#28998,#28999,#29000,#29001,#29002,#29003,
#29004,#29005,#29006,#29007,#29008,#29009,#29010,#29011,#29012,#29013,#29014,
#29015,#29016,#29017,#29018,#29019,#29020,#29021,#29022,#29023,#29024,#29025,
#29026,#29027,#29028,#29029,#29030,#29031,#29032,#29033,#29034,#29035,#29036,
#29037,#29038,#29039,#29040,#29041,#29042,#29043,#29044,#29045,#29046,#29047,
#29048,#29049,#29050,#29051,#29052,#29053,#29054,#29055,#29056,#29057,#29058,
#29059,#29060,#29061,#29062,#29063,#29064,#29065,#29066,#29067,#29068,#29069,
#29070,#29071,#29072,#29073,#29074,#29075,#29076,#29077,#29078,#29079,#29080,
#29081,#29082,#29083,#29084,#29085,#29086,#29087,#29088,#29089,#29090,#29091,
#29092,#29093,#29094,#29095,#29096,#29097,#29098,#29099,#29100,#29101,#29102,
#29103,#29104,#29105,#29106,#29107,#29108,#29109,#29110,#29111,#29112,#29113,
#29114,#29115,#29116,#29117,#29118,#29119,#29120),.UNSPECIFIED.,.F.,.F.,
(4,3,3,3,3,3,3,3,3,3,3,3,3,3,3,3,3,3,3,3,3,3,3,3,3,3,3,3,3,3,3,3,3,3,3,
3,3,3,3,3,3,3,3,3,4),(-87.613874691471,-87.4581822547,-87.3024512341524,
-87.1467085139083,-86.9906166055535,-86.8949391278171,-86.7375132693767,
-86.5803770127665,-86.4234095180274,-86.2663614088741,-86.1092653146766,
-85.9518296537067,-85.8961467240491,-85.7387208656087,-85.5815846089985,
-85.4246171142593,-85.2675690051059,-85.1104729109085,-84.9530372499385,
-84.8973543202811,-84.7399284618406,-84.5827922052304,-84.4258247104913,
-84.2687766013378,-84.1116805071403,-83.9542448461704,-83.8985619165131,
-83.7411360580727,-83.5839998014625,-83.4270323067233,-83.2699841975699,
-83.1128881033725,-82.9554524424025,-82.8997695127451,-82.7423436543047,
-82.5852073976945,-82.4282399029553,-82.2711917938019,-82.1140956996044,
-81.9566600386343,-81.9009771089771,-81.7398987646841,-81.5791799583681,
-81.4187407475093,-81.3306893842914),.UNSPECIFIED.);
#721=B_SPLINE_CURVE_WITH_KNOTS('',3,(#29122,#29123,#29124,#29125,#29126,
#29127,#29128,#29129,#29130,#29131),.UNSPECIFIED.,.F.,.F.,(4,1,1,1,1,1,
1,4),(-81.3306838834889,-80.9021847052091,-79.9033923014411,-78.9045998976731,
-77.905807493905,-76.907015090137,-75.908222686369,-75.0475121675532),
 .UNSPECIFIED.);
#722=B_SPLINE_CURVE_WITH_KNOTS('',3,(#29133,#29134,#29135,#29136,#29137,
#29138,#29139,#29140,#29141,#29142,#29143,#29144,#29145,#29146,#29147,#29148,
#29149,#29150,#29151,#29152,#29153,#29154,#29155,#29156,#29157,#29158,#29159,
#29160,#29161,#29162,#29163,#29164,#29165,#29166,#29167,#29168,#29169,#29170,
#29171,#29172,#29173,#29174,#29175,#29176,#29177,#29178,#29179,#29180,#29181,
#29182,#29183,#29184,#29185,#29186,#29187,#29188,#29189,#29190,#29191,#29192,
#29193,#29194,#29195,#29196,#29197,#29198,#29199,#29200,#29201,#29202,#29203,
#29204,#29205,#29206,#29207,#29208,#29209,#29210,#29211,#29212,#29213,#29214,
#29215,#29216,#29217,#29218,#29219,#29220,#29221,#29222,#29223,#29224,#29225,
#29226,#29227,#29228,#29229,#29230,#29231,#29232,#29233,#29234,#29235,#29236,
#29237,#29238,#29239,#29240,#29241,#29242,#29243,#29244,#29245,#29246,#29247,
#29248,#29249,#29250,#29251,#29252,#29253,#29254,#29255,#29256,#29257,#29258,
#29259,#29260,#29261,#29262,#29263,#29264,#29265),.UNSPECIFIED.,.F.,.F.,
(4,3,3,3,3,3,3,3,3,3,3,3,3,3,3,3,3,3,3,3,3,3,3,3,3,3,3,3,3,3,3,3,3,3,3,
3,3,3,3,3,3,3,3,3,4),(-75.0475040771118,-74.909430282601,-74.7520044241609,
-74.5948681675511,-74.4379006728122,-74.2808525636592,-74.1237564694621,
-73.9663208084924,-73.910637878833,-73.7532120203925,-73.5960757637822,
-73.439108269043,-73.2820601598895,-73.124964065692,-72.9675284047219,-72.911845475065,
-72.7544196166245,-72.5972833600143,-72.4403158652751,-72.2832677561216,
-72.1261716619241,-71.968736000954,-71.913053071297,-71.7556272128566,-71.5984909562464,
-71.4415234615072,-71.2844753523538,-71.1273792581563,-70.9699435971863,
-70.9142606675289,-70.7568348090885,-70.5996985524782,-70.4427310577391,
-70.2856829485857,-70.1285868543882,-69.9711511934181,-69.9154682637609,
-69.7580424053205,-69.6009061487103,-69.4439386539711,-69.2868905448178,
-69.1297944506203,-68.9723587896503,-68.9166758599929,-68.7643187699322),
 .UNSPECIFIED.);
#723=B_SPLINE_CURVE_WITH_KNOTS('',3,(#29267,#29268,#29269,#29270,#29271,
#29272,#29273,#29274,#29275,#29276),.UNSPECIFIED.,.F.,.F.,(4,1,1,1,1,1,
1,4),(-68.7643114907279,-67.9178834562249,-66.9190910524569,-65.9202986486889,
-64.9215062449209,-63.9227138411528,-62.9239214373848,-62.4811378862089),
 .UNSPECIFIED.);
#724=B_SPLINE_CURVE_WITH_KNOTS('',3,(#29278,#29279,#29280,#29281,#29282,
#29283,#29284,#29285,#29286,#29287,#29288,#29289,#29290,#29291,#29292,#29293,
#29294,#29295,#29296,#29297,#29298,#29299,#29300,#29301,#29302,#29303,#29304,
#29305,#29306,#29307,#29308,#29309,#29310,#29311,#29312,#29313,#29314,#29315,
#29316,#29317,#29318,#29319,#29320,#29321,#29322,#29323,#29324,#29325,#29326,
#29327,#29328,#29329,#29330,#29331,#29332,#29333,#29334,#29335,#29336,#29337,
#29338,#29339,#29340,#29341,#29342,#29343,#29344,#29345,#29346,#29347,#29348,
#29349,#29350,#29351,#29352,#29353,#29354,#29355,#29356,#29357,#29358,#29359,
#29360,#29361,#29362,#29363,#29364,#29365,#29366,#29367,#29368,#29369,#29370,
#29371,#29372,#29373,#29374,#29375,#29376,#29377,#29378,#29379,#29380,#29381,
#29382,#29383,#29384,#29385,#29386,#29387,#29388,#29389,#29390,#29391,#29392,
#29393,#29394,#29395,#29396,#29397,#29398,#29399,#29400,#29401,#29402,#29403,
#29404,#29405,#29406,#29407,#29408,#29409,#29410),.UNSPECIFIED.,.F.,.F.,
(4,3,3,3,3,3,3,3,3,3,3,3,3,3,3,3,3,3,3,3,3,3,3,3,3,3,3,3,3,3,3,3,3,3,3,
3,3,3,3,3,3,3,3,3,4),(-62.4811334627526,-62.3199251441198,-62.1585495109481,
-61.9966903768796,-61.9251290336168,-61.7677031751763,-61.6105669185661,
-61.4535994238269,-61.2965513146734,-61.1394552204759,-60.9820195595058,
-60.9263366298488,-60.7689107714084,-60.6117745147981,-60.454807020059,
-60.2977589109056,-60.1406628167082,-59.9832271557382,-59.9275442260808,
-59.7701183676404,-59.6129821110303,-59.456014616291,-59.2989665071376,
-59.1418704129402,-58.9844347519701,-58.9287518223128,-58.7713259638724,
-58.6141897072622,-58.457222212523,-58.3001741033696,-58.1430780091721,
-57.9856423482021,-57.9299594185448,-57.7725335601044,-57.6153973034943,
-57.4584298087551,-57.3013816996017,-57.1442856054042,-56.9868499444341,
-56.9311670147768,-56.7753043145904,-56.6197160121704,-56.4642955554139,
-56.3087841197039,-56.1979481555731),.UNSPECIFIED.);
#725=B_SPLINE_CURVE_WITH_KNOTS('',3,(#29412,#29413,#29414,#29415,#29416,
#29417,#29418,#29419,#29420,#29421,#29422,#29423,#29424,#29425,#29426,#29427,
#29428,#29429,#29430,#29431,#29432,#29433,#29434,#29435,#29436,#29437,#29438,
#29439,#29440,#29441,#29442,#29443,#29444,#29445,#29446,#29447,#29448,#29449,
#29450,#29451,#29452,#29453,#29454,#29455,#29456,#29457,#29458,#29459,#29460,
#29461,#29462,#29463,#29464,#29465,#29466,#29467,#29468,#29469,#29470,#29471,
#29472,#29473,#29474,#29475,#29476,#29477,#29478,#29479,#29480,#29481,#29482,
#29483,#29484,#29485,#29486,#29487,#29488,#29489,#29490,#29491,#29492,#29493,
#29494,#29495,#29496,#29497,#29498,#29499,#29500,#29501,#29502,#29503,#29504,
#29505,#29506,#29507,#29508,#29509,#29510,#29511,#29512,#29513,#29514,#29515,
#29516,#29517,#29518,#29519,#29520,#29521,#29522,#29523,#29524,#29525,#29526,
#29527,#29528,#29529,#29530,#29531,#29532,#29533,#29534,#29535,#29536,#29537,
#29538,#29539,#29540,#29541,#29542,#29543,#29544,#29545,#29546,#29547),
 .UNSPECIFIED.,.F.,.F.,(4,3,3,3,3,3,3,3,3,3,3,3,3,3,3,3,3,3,3,3,3,3,3,3,
3,3,3,3,3,3,3,3,3,3,3,3,3,3,3,3,3,3,3,3,3,4),(-56.1979481553862,-55.9987847029591,
-55.9323746110087,-55.7749487525684,-55.6178124959584,-55.4608450012194,
-55.3037968920661,-55.1467007978688,-54.9892651368989,-54.9335822072407,
-54.7761563488003,-54.61902009219,-54.4620525974508,-54.3050044882974,-54.1479083941,
-53.9904727331299,-53.9347898034727,-53.7773639450323,-53.620227688422,
-53.4632601936828,-53.3062120845294,-53.1491159903319,-52.9916803293619,
-52.9359973997047,-52.7785715412643,-52.6214352846541,-52.4644677899149,
-52.3074196807615,-52.1503235865641,-51.9928879255941,-51.9372049959367,
-51.7797791374963,-51.622642880886,-51.4656753861469,-51.3086272769935,
-51.151531182796,-50.9940955218259,-50.9384125921687,-50.7809867337283,
-50.6238504771181,-50.466882982379,-50.3098348732256,-50.1527387790282,
-49.9953031180581,-49.9396201884007,-49.9147628483934),.UNSPECIFIED.);
#726=B_SPLINE_CURVE_WITH_KNOTS('',3,(#29549,#29550,#29551,#29552,#29553,
#29554,#29555,#29556,#29557,#29558,#29559,#29560,#29561,#29562,#29563,#29564,
#29565,#29566,#29567,#29568,#29569,#29570,#29571,#29572,#29573,#29574,#29575,
#29576,#29577,#29578,#29579,#29580,#29581,#29582,#29583,#29584,#29585,#29586,
#29587,#29588,#29589,#29590,#29591,#29592,#29593,#29594,#29595,#29596,#29597,
#29598,#29599,#29600,#29601,#29602,#29603,#29604,#29605,#29606,#29607,#29608,
#29609,#29610,#29611,#29612,#29613,#29614,#29615,#29616,#29617,#29618,#29619,
#29620,#29621,#29622,#29623,#29624,#29625,#29626,#29627,#29628,#29629,#29630,
#29631,#29632,#29633,#29634,#29635,#29636,#29637,#29638,#29639,#29640,#29641,
#29642,#29643,#29644,#29645,#29646,#29647,#29648,#29649,#29650,#29651,#29652,
#29653,#29654,#29655,#29656,#29657,#29658,#29659,#29660,#29661,#29662,#29663,
#29664,#29665,#29666,#29667,#29668,#29669,#29670,#29671,#29672,#29673,#29674,
#29675,#29676,#29677,#29678,#29679,#29680,#29681),.UNSPECIFIED.,.F.,.F.,
(4,3,3,3,3,3,3,3,3,3,3,3,3,3,3,3,3,3,3,3,3,3,3,3,3,3,3,3,3,3,3,3,3,3,3,
3,3,3,3,3,3,3,3,3,4),(-49.9147628482126,-49.7579972342683,-49.601517677362,
-49.4452012318009,-49.2888004018216,-49.1323425683609,-48.9755541490261,
-48.9408277846327,-48.7834019261923,-48.6262656695821,-48.4692981748429,
-48.3122500656895,-48.1551539714921,-47.9977183105221,-47.9420353808647,
-47.7846095224242,-47.627473265814,-47.4705057710747,-47.3134576619212,
-47.1563615677237,-46.9989259067536,-46.9432429770966,-46.7858171186562,
-46.6286808620461,-46.4717133673068,-46.3146652581534,-46.157569163956,
-46.000133502986,-45.9444505733286,-45.7870247148882,-45.629888458278,-45.4729209635388,
-45.3158728543854,-45.1587767601879,-45.0013410992178,-44.9456581695606,
-44.7882323111202,-44.6310960545101,-44.474128559771,-44.3170804506176,
-44.1599843564201,-44.0025486954501,-43.9468657657926,-43.7595906204688,
-43.6315777496244),.UNSPECIFIED.);
#727=B_SPLINE_CURVE_WITH_KNOTS('',3,(#29683,#29684,#29685,#29686,#29687,
#29688,#29689,#29690,#29691,#29692),.UNSPECIFIED.,.F.,.F.,(4,1,1,1,1,1,
1,4),(-43.6315775412138,-42.9480733620246,-41.9492809582566,-40.9504885544885,
-39.9516961507205,-38.9529037469525,-37.9541113431845,-37.3483922340342),
 .UNSPECIFIED.);
#728=B_SPLINE_CURVE_WITH_KNOTS('',3,(#29694,#29695,#29696,#29697,#29698,
#29699,#29700,#29701,#29702,#29703,#29704,#29705,#29706,#29707,#29708,#29709,
#29710,#29711,#29712,#29713,#29714,#29715,#29716,#29717,#29718,#29719,#29720,
#29721,#29722,#29723,#29724,#29725,#29726,#29727,#29728,#29729,#29730,#29731,
#29732,#29733,#29734,#29735,#29736,#29737,#29738,#29739,#29740,#29741,#29742,
#29743,#29744,#29745,#29746,#29747,#29748,#29749,#29750,#29751,#29752,#29753,
#29754,#29755,#29756,#29757,#29758,#29759,#29760,#29761,#29762,#29763,#29764,
#29765,#29766,#29767,#29768,#29769,#29770,#29771,#29772,#29773,#29774,#29775,
#29776,#29777,#29778,#29779,#29780,#29781,#29782,#29783,#29784,#29785,#29786,
#29787,#29788,#29789,#29790,#29791,#29792,#29793,#29794,#29795,#29796,#29797,
#29798,#29799,#29800,#29801,#29802,#29803,#29804,#29805,#29806,#29807,#29808,
#29809,#29810,#29811,#29812,#29813,#29814,#29815,#29816,#29817,#29818,#29819,
#29820,#29821,#29822,#29823,#29824,#29825,#29826),.UNSPECIFIED.,.F.,.F.,
(4,3,3,3,3,3,3,3,3,3,3,3,3,3,3,3,3,3,3,3,3,3,3,3,3,3,3,3,3,3,3,3,3,3,3,
3,3,3,3,3,3,3,3,3,4),(-37.3483920044007,-37.1740560776412,-36.9983336164258,
-36.9553189394165,-36.7978930809762,-36.6407568243661,-36.483789329627,
-36.3267412204737,-36.1696451262764,-36.0122094653064,-35.9565265356485,
-35.7991006772078,-35.6419644205973,-35.4849969258578,-35.3279488167041,
-35.1708527225064,-35.013417061536,-34.9577341318805,-34.8003082734402,
-34.6431720168302,-34.4862045220911,-34.3291564129379,-34.1720603187406,
-34.0146246577706,-33.9589417281124,-33.8015158696727,-33.6443796130633,
-33.4874121183249,-33.3303640091722,-33.1732679149755,-33.0158322540062,
-32.9601493243444,-32.8027234659016,-32.6455872092891,-32.4886197145476,
-32.3315716053919,-32.1744755111921,-32.0170398502199,-31.9613569205764,
-31.8059289511626,-31.6507874821997,-31.495695171176,-31.3406480503224,
-31.1853007557434,-31.0652069270835),.UNSPECIFIED.);
#729=B_SPLINE_CURVE_WITH_KNOTS('',3,(#29828,#29829,#29830,#29831,#29832,
#29833,#29834,#29835,#29836,#29837,#29838,#29839,#29840,#29841,#29842,#29843,
#29844,#29845,#29846,#29847,#29848,#29849,#29850,#29851,#29852,#29853,#29854,
#29855,#29856,#29857,#29858,#29859,#29860,#29861,#29862,#29863,#29864,#29865,
#29866,#29867,#29868,#29869,#29870,#29871,#29872,#29873,#29874,#29875,#29876,
#29877,#29878,#29879,#29880,#29881,#29882,#29883,#29884,#29885,#29886,#29887,
#29888,#29889,#29890,#29891,#29892,#29893,#29894,#29895,#29896,#29897,#29898,
#29899,#29900,#29901,#29902,#29903,#29904,#29905,#29906,#29907,#29908,#29909,
#29910,#29911,#29912,#29913,#29914,#29915,#29916,#29917,#29918,#29919,#29920,
#29921,#29922,#29923,#29924,#29925,#29926,#29927,#29928,#29929,#29930,#29931,
#29932,#29933,#29934,#29935,#29936,#29937,#29938,#29939,#29940,#29941,#29942,
#29943,#29944,#29945,#29946,#29947,#29948,#29949,#29950,#29951,#29952,#29953,
#29954,#29955,#29956,#29957,#29958,#29959,#29960),.UNSPECIFIED.,.F.,.F.,
(4,3,3,3,3,3,3,3,3,3,3,3,3,3,3,3,3,3,3,3,3,3,3,3,3,3,3,3,3,3,3,3,3,3,3,
3,3,3,3,3,3,3,3,3,4),(-31.0652069268547,-30.9625645168084,-30.8051386583722,
-30.6480024017662,-30.4910349070314,-30.3339867978823,-30.1768907036891,
-30.0194550427234,-29.9637721130404,-29.8063462545833,-29.6492099979563,
-29.4922425032005,-29.3351943940307,-29.1780982998169,-29.020662638831,
-28.9649797092724,-28.8075538508509,-28.6504175942594,-28.4934500995388,
-28.3364019904035,-28.1793058962238,-28.0218702352708,-27.9661873055044,
-27.8087614470865,-27.6516251904992,-27.4946576957833,-27.3376095866533,
-27.1805134924793,-27.0230778315326,-26.9673949017364,-26.8099690431787,
-26.652832786451,-26.4958652915946,-26.3388171823254,-26.181721088013,-26.0242854269309,
-25.9686024979683,-25.8111766396887,-25.6540403832383,-25.4970728886576,
-25.3400247796587,-25.1829286856137,-25.0254930247908,-24.9698100942003,
-24.7820216196751),.UNSPECIFIED.);
#730=B_SPLINE_CURVE_WITH_KNOTS('',3,(#29962,#29963,#29964,#29965,#29966,
#29967,#29968,#29969,#29970,#29971),.UNSPECIFIED.,.F.,.F.,(4,1,1,1,1,1,
1,4),(-24.7820171771123,-23.9710176904323,-22.9722252866643,-21.9734328828963,
-20.9746404791283,-19.9758480753603,-18.9770556715922,-18.4988379499898),
 .UNSPECIFIED.);
#731=B_SPLINE_CURVE_WITH_KNOTS('',3,(#29973,#29974,#29975,#29976,#29977,
#29978,#29979,#29980,#29981,#29982,#29983,#29984,#29985,#29986,#29987,#29988,
#29989,#29990,#29991,#29992,#29993,#29994,#29995,#29996,#29997,#29998,#29999,
#30000,#30001,#30002,#30003,#30004,#30005,#30006,#30007,#30008,#30009,#30010,
#30011,#30012,#30013,#30014,#30015,#30016,#30017,#30018,#30019,#30020,#30021,
#30022,#30023,#30024,#30025,#30026,#30027,#30028,#30029,#30030,#30031,#30032,
#30033,#30034,#30035,#30036,#30037,#30038,#30039,#30040,#30041,#30042,#30043,
#30044,#30045,#30046,#30047,#30048,#30049,#30050,#30051,#30052,#30053,#30054,
#30055,#30056,#30057,#30058,#30059,#30060,#30061,#30062,#30063,#30064,#30065,
#30066,#30067,#30068,#30069,#30070,#30071,#30072,#30073,#30074,#30075,#30076,
#30077,#30078,#30079,#30080,#30081,#30082,#30083,#30084,#30085,#30086,#30087,
#30088,#30089,#30090,#30091,#30092,#30093,#30094,#30095,#30096,#30097,#30098,
#30099,#30100,#30101,#30102,#30103,#30104,#30105),.UNSPECIFIED.,.F.,.F.,
(4,3,3,3,3,3,3,3,3,3,3,3,3,3,3,3,3,3,3,3,3,3,3,3,3,3,3,3,3,3,3,3,3,3,3,
3,3,3,3,3,3,3,3,3,4),(-18.4988363124955,-18.3356133666513,-18.1721238367137,
-18.0080989678902,-17.9782632678242,-17.8208373743237,-17.6637010824669,
-17.5067335524134,-17.3496854082564,-17.1925892791905,-17.035153584078,
-16.9794708640562,-16.8220450841236,-16.6649089058851,-16.5079414891278,
-16.3508934564909,-16.1937974380605,-16.0363618506131,-15.9806784602882,
-15.8232525681947,-15.6661162789071,-15.5091487525538,-15.3521006136902,
-15.1950044908435,-15.0375688032116,-14.9818860565202,-14.8244599770603,
-14.6673234979013,-14.5103557798413,-14.3533074488336,-14.196211133349,
-14.0387752552734,-13.9830936527522,-13.8256683799556,-13.668532708559,
-13.5115657966989,-13.3545182603062,-13.1974227337522,-13.0399876243365,
-12.9843012489842,-12.8289087549843,-12.6737644033177,-12.5187820442914,
-12.3636506841468,-12.2156510053159),.UNSPECIFIED.);
#732=B_SPLINE_CURVE_WITH_KNOTS('',3,(#30107,#30108,#30109,#30110,#30111,
#30112,#30113,#30114,#30115,#30116,#30117),.UNSPECIFIED.,.F.,.F.,(4,1,1,
1,1,1,1,1,4),(-12.2156510053159,-11.9855088452162,-10.9867164414481,-9.98792403768013,
-8.98913163391212,-7.99033923014411,-6.99154682637609,-5.99275442260808,
-5.93246569813632),.UNSPECIFIED.);
#733=B_SPLINE_CURVE_WITH_KNOTS('',3,(#30119,#30120,#30121,#30122,#30123,
#30124,#30125,#30126,#30127,#30128,#30129,#30130,#30131,#30132,#30133,#30134,
#30135,#30136,#30137,#30138,#30139,#30140,#30141,#30142,#30143,#30144,#30145,
#30146,#30147,#30148,#30149,#30150,#30151,#30152,#30153,#30154,#30155,#30156,
#30157,#30158,#30159,#30160,#30161,#30162,#30163,#30164,#30165,#30166,#30167,
#30168,#30169,#30170,#30171,#30172,#30173,#30174,#30175,#30176,#30177,#30178,
#30179,#30180,#30181,#30182,#30183,#30184,#30185,#30186,#30187,#30188,#30189,
#30190,#30191,#30192,#30193,#30194,#30195,#30196,#30197),.UNSPECIFIED.,
 .F.,.F.,(4,3,3,3,3,3,3,3,3,3,3,3,3,3,3,3,3,3,3,3,3,3,3,3,3,3,4),(-5.93246569813632,
-5.77641800085584,-5.62064407302824,-5.4639735594812,-5.30825355217736,
-5.15110778550871,-4.99396201884007,-4.8367491311759,-4.67982626504034,
-4.52307188923757,-4.36623406611058,-4.20934690291075,-4.05211503034409,
-3.99516961507205,-3.83744358884951,-3.68000888850026,-3.52274564504591,
-3.36540915336445,-3.20802859481956,-3.05031852022946,-2.99637721130404,
-2.8403043537898,-2.68451357335128,-2.52868632450517,-2.3729713138078,-2.21690906463917,
-2.06120457796682),.UNSPECIFIED.);
#734=B_SPLINE_CURVE_WITH_KNOTS('',3,(#30199,#30200,#30201,#30202),
 .UNSPECIFIED.,.F.,.F.,(4,4),(-0.00791600890681302,0.),.UNSPECIFIED.);
#735=B_SPLINE_CURVE_WITH_KNOTS('',3,(#30206,#30207,#30208,#30209,#30210,
#30211),.UNSPECIFIED.,.F.,.F.,(4,1,1,4),(0.,0.998792403768015,1.99758480753603,
2.94976186885485),.UNSPECIFIED.);
#736=B_SPLINE_CURVE_WITH_KNOTS('',3,(#30213,#30214,#30215,#30216,#30217,
#30218,#30219,#30220,#30221,#30222,#30223),.UNSPECIFIED.,.F.,.F.,(4,1,1,
1,1,1,1,1,4),(2.94976186885485,2.99637721130404,3.99516961507206,4.99396201884008,
5.9927544226081,6.99154682637612,7.99033923014414,8.98913163391216,9.23294717603444),
 .UNSPECIFIED.);
#737=B_SPLINE_CURVE_WITH_KNOTS('',3,(#30225,#30226,#30227,#30228,#30229,
#30230,#30231,#30232,#30233,#30234),.UNSPECIFIED.,.F.,.F.,(4,1,1,1,1,1,
1,4),(9.23294717603444,9.98792403768017,10.9867164414482,11.9855088452162,
12.9843012489842,13.9830936527522,14.9818860565202,15.516132483214),
 .UNSPECIFIED.);
#738=B_SPLINE_CURVE_WITH_KNOTS('',3,(#30236,#30237,#30238,#30239,#30240,
#30241,#30242,#30243,#30244,#30245,#30246,#30247,#30248,#30249,#30250,#30251,
#30252,#30253,#30254,#30255,#30256,#30257,#30258,#30259,#30260,#30261,#30262,
#30263,#30264,#30265,#30266,#30267,#30268,#30269,#30270,#30271,#30272,#30273,
#30274,#30275,#30276,#30277,#30278,#30279,#30280,#30281,#30282,#30283,#30284,
#30285,#30286,#30287,#30288,#30289,#30290,#30291,#30292,#30293,#30294,#30295,
#30296,#30297,#30298,#30299,#30300,#30301,#30302,#30303,#30304,#30305,#30306,
#30307,#30308,#30309,#30310,#30311,#30312,#30313,#30314,#30315,#30316,#30317,
#30318,#30319,#30320,#30321,#30322,#30323,#30324,#30325,#30326,#30327,#30328,
#30329,#30330,#30331,#30332,#30333,#30334,#30335,#30336,#30337,#30338,#30339,
#30340,#30341,#30342,#30343,#30344,#30345,#30346,#30347,#30348,#30349,#30350,
#30351,#30352,#30353,#30354,#30355,#30356,#30357,#30358,#30359,#30360,#30361,
#30362,#30363,#30364,#30365,#30366,#30367,#30368),.UNSPECIFIED.,.F.,.F.,
(4,3,3,3,3,3,3,3,3,3,3,3,3,3,3,3,3,3,3,3,3,3,3,3,3,3,3,3,3,3,3,3,3,3,3,
3,3,3,3,3,3,3,3,3,4),(15.5161326720168,15.6833768003707,15.8514912044741,
15.9806784602882,16.1381042453226,16.295240426837,16.4522078450532,16.6092558764632,
16.7663518921126,16.9237874745117,16.9794708640563,17.1368967565385,17.2940330477215,
17.4510005774442,17.6080487217782,17.7651448513149,17.9225805473274,17.9782632678243,
18.1356891269169,18.2928253843364,18.4497928800386,18.6068409903732,18.7639370858797,
18.9213727483317,18.9770556715923,19.1344815204902,19.2916177673265,19.4485852520946,
19.6056333511011,19.7627294350371,19.9201650857285,19.9758480753603,20.1332739389886,
20.2904102008745,20.4473777009587,20.6044258154971,20.7615219151095,20.9189575814576,
20.9746404791283,21.1297203095798,21.2845109513251,21.4392204316573,21.5938858731285,
21.7487661283071,21.7993177903936),.UNSPECIFIED.);
#739=B_SPLINE_CURVE_WITH_KNOTS('',3,(#30370,#30371,#30372,#30373,#30374,
#30375,#30376,#30377,#30378,#30379,#30380),.UNSPECIFIED.,.F.,.F.,(4,1,1,
1,1,1,1,1,4),(21.7993177903936,21.9734328828963,22.9722252866643,23.9710176904323,
24.9698100942003,25.9686024979684,26.9673949017364,27.9661873055044,28.0825030975732),
 .UNSPECIFIED.);
#740=B_SPLINE_CURVE_WITH_KNOTS('',3,(#30382,#30383,#30384,#30385,#30386,
#30387,#30388,#30389,#30390,#30391,#30392,#30393,#30394,#30395,#30396,#30397,
#30398,#30399,#30400,#30401,#30402,#30403,#30404,#30405,#30406,#30407,#30408,
#30409,#30410,#30411,#30412,#30413,#30414,#30415,#30416,#30417,#30418,#30419,
#30420,#30421,#30422,#30423,#30424,#30425,#30426,#30427,#30428,#30429,#30430,
#30431,#30432,#30433,#30434,#30435,#30436,#30437,#30438,#30439,#30440,#30441,
#30442,#30443,#30444,#30445,#30446,#30447,#30448,#30449,#30450,#30451,#30452,
#30453,#30454,#30455,#30456,#30457,#30458,#30459,#30460,#30461,#30462,#30463,
#30464,#30465,#30466,#30467,#30468,#30469,#30470,#30471,#30472,#30473,#30474,
#30475,#30476,#30477,#30478,#30479,#30480,#30481,#30482,#30483,#30484,#30485,
#30486,#30487,#30488,#30489,#30490,#30491,#30492,#30493,#30494,#30495,#30496,
#30497,#30498,#30499,#30500,#30501,#30502,#30503,#30504,#30505,#30506,#30507,
#30508,#30509,#30510,#30511,#30512,#30513,#30514),.UNSPECIFIED.,.F.,.F.,
(4,3,3,3,3,3,3,3,3,3,3,3,3,3,3,3,3,3,3,3,3,3,3,3,3,3,3,3,3,3,3,3,3,3,3,
3,3,3,3,3,3,3,3,3,4),(28.0825030975732,28.2376974030802,28.3926473134147,
28.5476070278282,28.7025582372351,28.8578500130469,28.9649797092724,29.1224055677287,
29.2795418243551,29.4365093191107,29.5935574282807,29.7506535224949,29.9080891834816,
29.9637721130404,30.1211979714765,30.2783342280825,30.4353017228172,30.5923498319662,
30.7494459261594,30.9068815871251,30.9625645168084,31.119990375247,31.2771266318553,
31.4340941265926,31.5911422357439,31.7482383299393,31.9056739909073,31.9613569205764,
32.118782779019,32.2759190356316,32.4328865303731,32.5899346395289,32.7470307337286,
32.904466394701,32.9601493243444,33.1175751827841,33.2747114393934,33.4316789341318,
33.5887270432845,33.7458231374812,33.9032587984505,33.9589417281124,34.1330497198208,
34.3059304641482,34.3656881914393),.UNSPECIFIED.);
#741=B_SPLINE_CURVE_WITH_KNOTS('',3,(#30516,#30517,#30518,#30519,#30520,
#30521,#30522,#30523,#30524,#30525),.UNSPECIFIED.,.F.,.F.,(4,1,1,1,1,1,
1,4),(34.3656884047528,34.9577341318804,35.9565265356485,36.9553189394165,
37.9541113431845,38.9529037469526,39.9516961507206,40.6488737119324),
 .UNSPECIFIED.);
#742=B_SPLINE_CURVE_WITH_KNOTS('',3,(#30527,#30528,#30529,#30530,#30531,
#30532,#30533,#30534,#30535,#30536,#30537,#30538,#30539,#30540,#30541,#30542,
#30543,#30544,#30545,#30546,#30547,#30548,#30549,#30550,#30551,#30552,#30553,
#30554,#30555,#30556,#30557,#30558,#30559,#30560,#30561,#30562,#30563,#30564,
#30565,#30566,#30567,#30568,#30569,#30570,#30571,#30572,#30573,#30574,#30575,
#30576,#30577,#30578,#30579,#30580,#30581,#30582,#30583,#30584,#30585,#30586,
#30587,#30588,#30589,#30590,#30591,#30592,#30593,#30594,#30595,#30596,#30597,
#30598,#30599,#30600,#30601,#30602,#30603,#30604,#30605,#30606,#30607,#30608,
#30609,#30610,#30611,#30612,#30613,#30614,#30615,#30616,#30617,#30618,#30619,
#30620,#30621,#30622,#30623,#30624,#30625,#30626,#30627,#30628,#30629,#30630,
#30631,#30632,#30633,#30634,#30635,#30636,#30637,#30638,#30639,#30640,#30641,
#30642,#30643,#30644,#30645,#30646,#30647,#30648,#30649,#30650,#30651,#30652,
#30653,#30654,#30655,#30656,#30657,#30658,#30659),.UNSPECIFIED.,.F.,.F.,
(4,3,3,3,3,3,3,3,3,3,3,3,3,3,3,3,3,3,3,3,3,3,3,3,3,3,3,3,3,3,3,3,3,3,3,
3,3,3,3,3,3,3,3,3,4),(40.6488738966027,40.8389897275225,40.9504885544886,
41.107914412929,41.2650506695392,41.4220181642784,41.5790662734318,41.7361623676293,
41.8935980285994,41.9492809582566,42.106706816697,42.2638430733072,42.4208105680465,
42.5778586771999,42.7349547713973,42.8923904323674,42.9480733620246,43.105499220465,
43.2626354770752,43.4196029718143,43.5766510809677,43.7337471751652,43.8911828361352,
43.9468657657926,44.1042916242331,44.2614278808433,44.4183953755826,44.575443484736,
44.7325395789335,44.8899752399036,44.9456581695607,45.1030840280011,45.2602202846113,
45.4171877793505,45.5742358885039,45.7313319827014,45.8887676436714,45.9444505733287,
46.1015680379833,46.2583964719956,46.4150577485581,46.5718002293858,46.7285940925013,
46.8857227911254,46.93205901893),.UNSPECIFIED.);
#743=B_SPLINE_CURVE_WITH_KNOTS('',3,(#30661,#30662,#30663,#30664,#30665,
#30666,#30667,#30668,#30669,#30670,#30671,#30672,#30673,#30674,#30675,#30676,
#30677,#30678,#30679,#30680,#30681,#30682,#30683,#30684,#30685,#30686,#30687,
#30688,#30689,#30690,#30691,#30692,#30693,#30694,#30695,#30696,#30697,#30698,
#30699,#30700,#30701,#30702,#30703,#30704,#30705,#30706,#30707,#30708,#30709,
#30710,#30711,#30712,#30713,#30714,#30715,#30716,#30717,#30718,#30719,#30720,
#30721,#30722,#30723,#30724,#30725,#30726,#30727,#30728,#30729,#30730,#30731,
#30732,#30733,#30734,#30735,#30736,#30737,#30738,#30739,#30740,#30741,#30742,
#30743,#30744,#30745,#30746,#30747,#30748,#30749,#30750,#30751,#30752,#30753,
#30754,#30755,#30756,#30757,#30758,#30759,#30760,#30761,#30762,#30763,#30764,
#30765,#30766,#30767,#30768,#30769,#30770,#30771,#30772,#30773,#30774,#30775,
#30776,#30777,#30778,#30779,#30780,#30781,#30782,#30783,#30784,#30785,#30786,
#30787,#30788,#30789,#30790,#30791,#30792,#30793,#30794,#30795,#30796),
 .UNSPECIFIED.,.F.,.F.,(4,3,3,3,3,3,3,3,3,3,3,3,3,3,3,3,3,3,3,3,3,3,3,3,
3,3,3,3,3,3,3,3,3,3,3,3,3,3,3,3,3,3,3,3,3,4),(46.932059019112,46.9432429770967,
47.1006688355372,47.2578050921474,47.4147725868865,47.57182069604,47.7289167902374,
47.8863524512075,47.9420353808647,48.0994612393051,48.2565974959154,48.4135649906546,
48.570613099808,48.7277091940054,48.8851448549755,48.9408277846327,49.0982536430731,
49.2553898996833,49.4123573944225,49.5694055035759,49.7265015977733,49.8839372587433,
49.9396201884007,50.0970460468411,50.2541823034514,50.4111497981906,50.568197907344,
50.7252940015415,50.8827296625115,50.9384125921687,51.0958384506091,51.2529747072194,
51.4099422019585,51.5669903111119,51.7240864053094,51.8815220662794,51.9372049959367,
52.0946308543771,52.2517671109873,52.4087346057264,52.5657827148798,52.7228788090773,
52.8803144700473,52.9359973997047,53.1314224868731,53.2152443261636),
 .UNSPECIFIED.);
#744=B_SPLINE_CURVE_WITH_KNOTS('',3,(#30798,#30799,#30800,#30801,#30802,
#30803,#30804,#30805,#30806,#30807,#30808,#30809,#30810,#30811,#30812,#30813,
#30814,#30815,#30816,#30817,#30818,#30819,#30820,#30821,#30822,#30823,#30824,
#30825,#30826,#30827,#30828,#30829,#30830,#30831,#30832,#30833,#30834,#30835,
#30836,#30837,#30838,#30839,#30840,#30841,#30842,#30843,#30844,#30845,#30846,
#30847,#30848,#30849,#30850,#30851,#30852,#30853,#30854,#30855,#30856,#30857,
#30858,#30859,#30860,#30861,#30862,#30863,#30864,#30865,#30866,#30867,#30868,
#30869,#30870,#30871,#30872,#30873,#30874,#30875,#30876,#30877,#30878,#30879,
#30880,#30881,#30882,#30883,#30884,#30885,#30886,#30887,#30888,#30889,#30890,
#30891,#30892,#30893,#30894,#30895,#30896,#30897,#30898,#30899,#30900,#30901,
#30902,#30903,#30904,#30905,#30906,#30907,#30908,#30909,#30910,#30911,#30912,
#30913,#30914,#30915,#30916,#30917,#30918,#30919,#30920,#30921,#30922,#30923,
#30924,#30925,#30926,#30927,#30928,#30929,#30930),.UNSPECIFIED.,.F.,.F.,
(4,3,3,3,3,3,3,3,3,3,3,3,3,3,3,3,3,3,3,3,3,3,3,3,3,3,3,3,3,3,3,3,3,3,3,
3,3,3,3,3,3,3,3,3,4),(53.2152443262915,53.370926689653,53.5266468618019,
53.6823780883531,53.8384585272822,53.9347898034727,54.0922156619131,54.2493519185232,
54.4063194132625,54.5633675224159,54.7204636166133,54.8778992775833,54.9335822072407,
55.0910080656812,55.2481443222914,55.4051118170306,55.562159926184,55.7192560203815,
55.8766916813516,55.9323746110088,56.0898004694492,56.2469367260595,56.4039042207987,
56.5609523299522,56.7180484241497,56.8754840851197,56.9311670147768,57.0885928732172,
57.2457291298273,57.4026966245663,57.5597447337196,57.7168408279169,57.8742764888869,
57.9299594185448,58.0873852769852,58.2445215335953,58.4014890283344,58.5585371374879,
58.7156332316853,58.8730688926553,58.9287518223128,59.0898611342064,59.250610284966,
59.4110781810322,59.4984296334711),.UNSPECIFIED.);
#745=B_SPLINE_CURVE_WITH_KNOTS('',3,(#30932,#30933,#30934,#30935,#30936,
#30937,#30938,#30939,#30940,#30941),.UNSPECIFIED.,.F.,.F.,(4,1,1,1,1,1,
1,4),(59.4984349204034,59.9275442260809,60.9263366298489,61.9251290336169,
62.9239214373849,63.9227138411529,64.9215062449209,65.7816068796228),
 .UNSPECIFIED.);
#746=B_SPLINE_CURVE_WITH_KNOTS('',3,(#30943,#30944,#30945,#30946,#30947,
#30948,#30949,#30950,#30951,#30952,#30953,#30954,#30955,#30956,#30957,#30958,
#30959,#30960,#30961,#30962,#30963,#30964,#30965,#30966,#30967,#30968,#30969,
#30970,#30971,#30972,#30973,#30974,#30975,#30976,#30977,#30978,#30979,#30980,
#30981,#30982,#30983,#30984,#30985,#30986,#30987,#30988,#30989,#30990,#30991,
#30992,#30993,#30994,#30995,#30996,#30997,#30998,#30999,#31000,#31001,#31002,
#31003,#31004,#31005,#31006,#31007,#31008,#31009,#31010,#31011,#31012,#31013,
#31014,#31015,#31016,#31017,#31018,#31019,#31020,#31021,#31022,#31023,#31024,
#31025,#31026,#31027,#31028,#31029,#31030,#31031,#31032,#31033,#31034,#31035,
#31036,#31037,#31038,#31039,#31040,#31041,#31042,#31043,#31044,#31045,#31046,
#31047,#31048,#31049,#31050,#31051,#31052,#31053,#31054,#31055,#31056,#31057,
#31058,#31059,#31060,#31061,#31062,#31063,#31064,#31065,#31066,#31067,#31068,
#31069,#31070,#31071,#31072,#31073,#31074,#31075),.UNSPECIFIED.,.F.,.F.,
(4,3,3,3,3,3,3,3,3,3,3,3,3,3,3,3,3,3,3,3,3,3,3,3,3,3,3,3,3,3,3,3,3,3,3,
3,3,3,3,3,3,3,3,3,4),(65.7816149406508,65.9202986486889,66.0777245071298,
66.2348607637404,66.39182825848,66.5488763676339,66.7059724618319,66.8634081228024,
66.9190910524569,67.0765169108973,67.2336531675074,67.3906206622465,67.5476687713999,
67.7047648655973,67.8622005265673,67.9178834562249,68.0753093146652,68.2324455712754,
68.3894130660145,68.5464611751678,68.7035572693652,68.8609929303351,68.9166758599929,
69.0741017184334,69.2312379750437,69.3882054697829,69.5452535789364,69.702349673134,
69.8597853341041,69.915468263761,70.0728941222014,70.2300303788117,70.3869978735509,
70.5440459827043,70.7011420769017,70.8585777378718,70.914260667529,71.0716865259694,
71.2288227825796,71.3857902773188,71.5428383864722,71.6999344806696,71.8573701416396,
71.913053071297,72.0648002478303),.UNSPECIFIED.);
#747=B_SPLINE_CURVE_WITH_KNOTS('',3,(#31077,#31078,#31079,#31080,#31081,
#31082,#31083,#31084,#31085,#31086),.UNSPECIFIED.,.F.,.F.,(4,1,1,1,1,1,
1,4),(72.0648075666675,72.911845475065,73.910637878833,74.909430282601,
75.908222686369,76.9070150901371,77.9058074939051,78.3479810907392),
 .UNSPECIFIED.);
#748=B_SPLINE_CURVE_WITH_KNOTS('',3,(#31088,#31089,#31090,#31091,#31092,
#31093,#31094,#31095,#31096,#31097,#31098,#31099,#31100,#31101,#31102,#31103,
#31104,#31105,#31106,#31107,#31108,#31109,#31110,#31111,#31112,#31113,#31114,
#31115,#31116,#31117,#31118,#31119,#31120,#31121,#31122,#31123,#31124,#31125,
#31126,#31127,#31128,#31129,#31130,#31131,#31132,#31133,#31134,#31135,#31136,
#31137,#31138,#31139,#31140,#31141,#31142,#31143,#31144,#31145,#31146,#31147,
#31148,#31149,#31150,#31151,#31152,#31153,#31154,#31155,#31156,#31157,#31158,
#31159,#31160,#31161,#31162,#31163,#31164,#31165,#31166,#31167,#31168,#31169,
#31170,#31171,#31172,#31173,#31174,#31175,#31176,#31177,#31178,#31179,#31180,
#31181,#31182,#31183,#31184,#31185,#31186,#31187,#31188,#31189,#31190,#31191,
#31192,#31193,#31194,#31195,#31196,#31197,#31198,#31199,#31200,#31201,#31202,
#31203,#31204,#31205,#31206,#31207,#31208,#31209,#31210,#31211,#31212,#31213,
#31214,#31215,#31216,#31217,#31218,#31219,#31220),.UNSPECIFIED.,.F.,.F.,
(4,3,3,3,3,3,3,3,3,3,3,3,3,3,3,3,3,3,3,3,3,3,3,3,3,3,3,3,3,3,3,3,3,3,3,
3,3,3,3,3,3,3,3,3,4),(78.3479855550099,78.5091623284623,78.6705049083517,
78.8323302432885,78.9045998976731,79.0620257561135,79.2191620127237,79.3761295074628,
79.5331776166161,79.6902737108135,79.8477093717835,79.9033923014411,80.0608181598815,
80.2179544164917,80.3749219112309,80.5319700203843,80.6890661145817,80.8465017755518,
80.9021847052091,81.0596105636496,81.2167468202599,81.3737143149991,81.5307624241525,
81.6878585183501,81.8452941793201,81.9009771089771,82.0584029674175,82.2155392240278,
82.3725067187669,82.5295548279203,82.6866509221178,82.8440865830878,82.8997695127452,
83.0571953711857,83.214331627796,83.371299122535,83.5283472316885,83.685443325886,
83.8428789868561,83.8985619165132,84.0544346455478,84.2100324943769,84.3654623696513,
84.5209822278603,84.6311708621895),.UNSPECIFIED.);
#749=B_SPLINE_CURVE_WITH_KNOTS('',3,(#31222,#31223,#31224,#31225,#31226,
#31227,#31228,#31229,#31230,#31231,#31232,#31233,#31234,#31235,#31236,#31237,
#31238,#31239,#31240,#31241,#31242,#31243,#31244,#31245,#31246,#31247,#31248,
#31249,#31250,#31251,#31252,#31253,#31254,#31255,#31256,#31257,#31258,#31259,
#31260,#31261,#31262,#31263,#31264,#31265,#31266,#31267,#31268,#31269,#31270,
#31271,#31272,#31273,#31274,#31275,#31276,#31277,#31278,#31279,#31280,#31281,
#31282,#31283,#31284,#31285,#31286,#31287,#31288,#31289,#31290,#31291,#31292,
#31293,#31294,#31295,#31296,#31297,#31298,#31299,#31300,#31301,#31302,#31303,
#31304,#31305,#31306,#31307,#31308,#31309,#31310,#31311,#31312,#31313,#31314,
#31315,#31316,#31317,#31318,#31319,#31320,#31321,#31322,#31323,#31324,#31325,
#31326,#31327,#31328,#31329,#31330,#31331,#31332,#31333,#31334,#31335,#31336,
#31337,#31338,#31339,#31340,#31341,#31342,#31343,#31344,#31345,#31346,#31347,
#31348,#31349,#31350,#31351,#31352,#31353,#31354,#31355,#31356,#31357),
 .UNSPECIFIED.,.F.,.F.,(4,3,3,3,3,3,3,3,3,3,3,3,3,3,3,3,3,3,3,3,3,3,3,3,
3,3,3,3,3,3,3,3,3,3,3,3,3,3,3,3,3,3,3,3,3,4),(84.6311708623796,84.8301583421363,
84.8973543202812,85.0547801787217,85.211916435332,85.3688839300712,85.5259320392247,
85.6830281334222,85.8404637943923,85.8961467240492,86.0535725824896,86.2107088390998,
86.367676333839,86.5247244429924,86.6818205371899,86.8392561981599,86.8949391278172,
87.0523649862576,87.2095012428678,87.366468737607,87.5235168467604,87.6806129409579,
87.8380486019279,87.8937315315852,88.0511573900256,88.2082936466359,88.365261141375,
88.5223092505284,88.6794053447259,88.8368410056959,88.8925239353532,89.0499497937936,
89.2070860504038,89.364053545143,89.5211016542964,89.6781977484939,89.8356334094639,
89.8913163391212,90.0487421975616,90.2058784541718,90.362845948911,90.5198940580644,
90.6769901522618,90.8344258132319,90.8901087428892,90.9143561693691),
 .UNSPECIFIED.);
#750=B_SPLINE_CURVE_WITH_KNOTS('',3,(#31359,#31360,#31361,#31362,#31363,
#31364,#31365,#31366,#31367,#31368,#31369,#31370,#31371,#31372,#31373,#31374,
#31375,#31376,#31377,#31378,#31379,#31380,#31381,#31382,#31383,#31384,#31385,
#31386,#31387,#31388,#31389,#31390,#31391,#31392,#31393,#31394,#31395,#31396,
#31397,#31398,#31399,#31400,#31401,#31402,#31403,#31404,#31405,#31406,#31407,
#31408,#31409,#31410,#31411,#31412,#31413,#31414,#31415,#31416,#31417,#31418,
#31419,#31420,#31421,#31422,#31423,#31424,#31425,#31426,#31427,#31428,#31429,
#31430,#31431,#31432,#31433,#31434,#31435,#31436,#31437,#31438,#31439,#31440,
#31441,#31442,#31443,#31444,#31445,#31446,#31447,#31448,#31449,#31450,#31451,
#31452,#31453,#31454,#31455,#31456,#31457,#31458,#31459,#31460,#31461,#31462,
#31463,#31464,#31465,#31466,#31467,#31468,#31469,#31470,#31471,#31472,#31473,
#31474,#31475,#31476,#31477,#31478,#31479,#31480,#31481,#31482,#31483,#31484,
#31485,#31486,#31487,#31488,#31489,#31490,#31491),.UNSPECIFIED.,.F.,.F.,
(4,3,3,3,3,3,3,3,3,3,3,3,3,3,3,3,3,3,3,3,3,3,3,3,3,3,3,3,3,3,3,3,3,3,3,
3,3,3,3,3,3,3,3,3,4),(90.9143561695458,91.071136765442,91.2276311674691,
91.3839622773045,91.540377642471,91.696849766663,91.8536526876333,91.8889011466572,
92.0463270050976,92.2034632617077,92.3604307564468,92.5174788656002,92.6745749597977,
92.8320106207677,92.8876935504252,93.0451194088657,93.202255665476,93.3592231602152,
93.5162712693686,93.6733673635661,93.8308030245362,93.8864859541933,94.0439118126337,
94.2010480692439,94.358015563983,94.5150636731364,94.6721597673337,94.8295954283037,
94.8852783579613,95.0427042164017,95.1998404730119,95.3568079677511,95.5138560769045,
95.6709521711019,95.8283878320719,95.8840707617293,96.0414966201698,96.19863287678,
96.3556003715192,96.5126484806726,96.6697445748702,96.8271802358402,96.8828631654974,
97.0702592987996,97.1975412690878),.UNSPECIFIED.);
#751=B_SPLINE_CURVE_WITH_KNOTS('',3,(#31493,#31494,#31495,#31496,#31497,
#31498,#31499,#31500,#31501,#31502),.UNSPECIFIED.,.F.,.F.,(4,1,1,1,1,1,
1,4),(97.1975414765487,97.8816555692654,98.8804479730334,99.8792403768014,
100.878032780569,101.876825184337,102.875617588105,103.480726783728),
 .UNSPECIFIED.);
#752=B_SPLINE_CURVE_WITH_KNOTS('',3,(#31504,#31505,#31506,#31507,#31508,
#31509,#31510,#31511,#31512,#31513,#31514,#31515,#31516,#31517,#31518,#31519,
#31520,#31521,#31522,#31523,#31524,#31525,#31526,#31527,#31528,#31529,#31530,
#31531,#31532,#31533,#31534,#31535,#31536,#31537,#31538,#31539,#31540,#31541,
#31542,#31543,#31544,#31545,#31546,#31547,#31548,#31549,#31550,#31551,#31552,
#31553,#31554,#31555,#31556,#31557,#31558,#31559,#31560,#31561,#31562,#31563,
#31564,#31565,#31566,#31567,#31568,#31569,#31570,#31571,#31572,#31573,#31574,
#31575,#31576,#31577,#31578,#31579,#31580,#31581,#31582,#31583,#31584,#31585,
#31586,#31587,#31588,#31589,#31590,#31591,#31592,#31593,#31594,#31595,#31596,
#31597,#31598,#31599,#31600,#31601,#31602,#31603,#31604,#31605,#31606,#31607,
#31608,#31609,#31610,#31611,#31612,#31613,#31614,#31615,#31616,#31617,#31618,
#31619,#31620,#31621,#31622,#31623,#31624,#31625,#31626,#31627,#31628,#31629,
#31630,#31631,#31632,#31633,#31634,#31635,#31636),.UNSPECIFIED.,.F.,.F.,
(4,3,3,3,3,3,3,3,3,3,3,3,3,3,3,3,3,3,3,3,3,3,3,3,3,3,3,3,3,3,3,3,3,3,3,
3,3,3,3,3,3,3,3,3,4),(103.480727012744,103.654990565238,103.830634353272,
103.874409991873,104.031835850313,104.188972106924,104.345939601663,104.502987710817,
104.660083805014,104.817519465984,104.873202395641,105.030628254081,105.187764510692,
105.344732005431,105.501780114584,105.658876208782,105.816311869752,105.871994799409,
106.029420657849,106.186556914459,106.343524409198,106.500572518352,106.657668612549,
106.815104273519,106.870787203177,107.028213061618,107.185349318228,107.342316812968,
107.499364922122,107.65646101632,107.81389667729,107.869579606946,108.027005465387,
108.184141721997,108.341109216736,108.49815732589,108.655253420087,108.812689081058,
108.868372010714,109.023793477623,109.178928442311,109.334014026415,109.48905446015,
109.644394363258,109.763912090679),.UNSPECIFIED.);
#753=B_SPLINE_CURVE_WITH_KNOTS('',3,(#31638,#31639,#31640,#31641,#31642,
#31643,#31644,#31645,#31646,#31647,#31648,#31649,#31650,#31651,#31652,#31653,
#31654,#31655,#31656,#31657,#31658,#31659,#31660,#31661,#31662,#31663,#31664,
#31665,#31666,#31667,#31668,#31669,#31670,#31671,#31672,#31673,#31674,#31675,
#31676,#31677,#31678,#31679,#31680,#31681,#31682,#31683,#31684,#31685,#31686,
#31687,#31688,#31689,#31690,#31691,#31692,#31693,#31694,#31695,#31696,#31697,
#31698,#31699,#31700,#31701,#31702,#31703,#31704,#31705,#31706,#31707,#31708,
#31709,#31710,#31711,#31712,#31713,#31714,#31715,#31716,#31717,#31718,#31719,
#31720,#31721,#31722,#31723,#31724,#31725,#31726,#31727,#31728,#31729,#31730,
#31731,#31732,#31733,#31734,#31735,#31736,#31737,#31738,#31739,#31740,#31741,
#31742,#31743,#31744,#31745,#31746,#31747,#31748,#31749,#31750,#31751,#31752,
#31753,#31754,#31755,#31756,#31757,#31758,#31759,#31760,#31761,#31762,#31763,
#31764,#31765,#31766,#31767,#31768,#31769,#31770),.UNSPECIFIED.,.F.,.F.,
(4,3,3,3,3,3,3,3,3,3,3,3,3,3,3,3,3,3,3,3,3,3,3,3,3,3,3,3,3,3,3,3,3,3,3,
3,3,3,3,3,3,3,3,3,4),(109.763912090908,109.867164414482,110.02459027292,
110.181726529529,110.338694024266,110.495742133417,110.652838227612,110.81027388858,
110.86595681825,111.023382676691,111.180518933301,111.337486428041,111.494534537194,
111.651630631392,111.809066292363,111.864749222018,112.022175080459,112.179311337069,
112.336278831809,112.493326940962,112.65042303516,112.80785869613,112.863541625786,
113.020967484226,113.178103740836,113.335071235575,113.492119344728,113.649215438926,
113.806651099895,113.862334029554,114.019759887994,114.176896144605,114.333863639344,
114.490911748497,114.648007842695,114.805443503665,114.861126433322,115.018552291763,
115.175688548373,115.332656043113,115.489704152267,115.646800246464,115.804235907435,
115.85991883709,116.047097398087),.UNSPECIFIED.);
#754=B_SPLINE_CURVE_WITH_KNOTS('',3,(#31772,#31773,#31774,#31775,#31776,
#31777,#31778,#31779,#31780,#31781),.UNSPECIFIED.,.F.,.F.,(4,1,1,1,1,1,
1,4),(116.047101897182,116.858711240858,117.857503644626,118.856296048394,
119.855088452162,120.85388085593,121.852673259698,122.330281021608),
 .UNSPECIFIED.);
#755=B_SPLINE_CURVE_WITH_KNOTS('',3,(#31783,#31784,#31785,#31786,#31787,
#31788,#31789,#31790,#31791,#31792,#31793,#31794,#31795,#31796,#31797,#31798,
#31799,#31800,#31801,#31802,#31803,#31804,#31805,#31806,#31807,#31808,#31809,
#31810,#31811,#31812,#31813,#31814,#31815,#31816,#31817,#31818,#31819,#31820,
#31821,#31822,#31823,#31824,#31825,#31826,#31827,#31828,#31829,#31830,#31831,
#31832,#31833,#31834,#31835,#31836,#31837,#31838,#31839,#31840,#31841,#31842,
#31843,#31844,#31845,#31846,#31847,#31848,#31849,#31850,#31851,#31852,#31853,
#31854,#31855,#31856,#31857,#31858,#31859,#31860,#31861,#31862,#31863,#31864,
#31865,#31866,#31867,#31868,#31869,#31870,#31871,#31872,#31873,#31874,#31875,
#31876,#31877,#31878,#31879,#31880,#31881,#31882,#31883,#31884,#31885,#31886,
#31887,#31888,#31889,#31890,#31891,#31892,#31893,#31894,#31895,#31896,#31897,
#31898,#31899,#31900,#31901,#31902,#31903,#31904,#31905,#31906,#31907,#31908,
#31909,#31910,#31911,#31912,#31913,#31914,#31915),.UNSPECIFIED.,.F.,.F.,
(4,3,3,3,3,3,3,3,3,3,3,3,3,3,3,3,3,3,3,3,3,3,3,3,3,3,3,3,3,3,3,3,3,3,3,
3,3,3,3,3,3,3,3,3,4),(122.330282705267,122.493467815871,122.656917583374,
122.820901647644,122.851465663466,123.008891521906,123.166027778516,123.322995273255,
123.480043382409,123.637139476606,123.794575137576,123.850258067234,124.007683925674,
124.164820182285,124.321787677024,124.478835786177,124.635931880375,124.793367541345,
124.849050471002,125.006476329442,125.163612586053,125.320580080792,125.477628189945,
125.634724284143,125.792159945113,125.84784287477,126.00526873321,126.162404989821,
126.31937248456,126.476420593713,126.633516687911,126.790952348881,126.846635278538,
127.004061136978,127.161197393589,127.318164888328,127.475212997481,127.632309091679,
127.789744752649,127.845427682306,128.000825675512,128.155975118574,128.310962499579,
128.466097903113,128.613468012447),.UNSPECIFIED.);
#756=B_SPLINE_CURVE_WITH_KNOTS('',3,(#31917,#31918,#31919,#31920,#31921,
#31922,#31923,#31924,#31925,#31926,#31927),.UNSPECIFIED.,.F.,.F.,(4,1,1,
1,1,1,1,1,4),(128.613468012447,128.844220086074,129.843012489842,130.84180489361,
131.840597297378,132.839389701146,133.838182104914,134.836974508682,134.896653319626),
 .UNSPECIFIED.);
#757=B_SPLINE_CURVE_WITH_KNOTS('',3,(#31929,#31930,#31931,#31932,#31933,
#31934,#31935,#31936,#31937,#31938,#31939,#31940,#31941,#31942,#31943,#31944,
#31945,#31946,#31947,#31948,#31949,#31950,#31951,#31952,#31953,#31954,#31955,
#31956,#31957,#31958,#31959,#31960,#31961,#31962,#31963,#31964,#31965,#31966,
#31967,#31968,#31969,#31970,#31971,#31972,#31973,#31974,#31975,#31976,#31977,
#31978,#31979,#31980,#31981,#31982,#31983,#31984,#31985,#31986,#31987,#31988,
#31989,#31990,#31991,#31992,#31993,#31994,#31995,#31996,#31997,#31998,#31999,
#32000,#32001,#32002,#32003,#32004,#32005,#32006,#32007,#32008,#32009,#32010,
#32011,#32012,#32013,#32014,#32015,#32016,#32017,#32018,#32019,#32020,#32021,
#32022,#32023,#32024,#32025,#32026,#32027,#32028,#32029,#32030,#32031,#32032,
#32033,#32034,#32035,#32036,#32037,#32038,#32039,#32040,#32041,#32042,#32043,
#32044,#32045,#32046,#32047,#32048,#32049,#32050,#32051,#32052,#32053,#32054,
#32055,#32056,#32057,#32058),.UNSPECIFIED.,.F.,.F.,(4,3,3,3,3,3,3,3,3,3,
3,3,3,3,3,3,3,3,3,3,3,3,3,3,3,3,3,3,3,3,3,3,3,3,3,3,3,3,3,3,3,3,3,4),(134.896653319626,
135.05266364742,135.208399238582,135.365241157049,135.520921408202,135.678344160326,
135.83576691245,135.99319277089,136.150329027501,136.30729652224,136.464344631393,
136.621440725591,136.778876386561,136.834559316218,136.991985174658,137.149121431269,
137.306088926008,137.463137035161,137.620233129359,137.777668790329,137.833351719986,
137.990777578426,138.147913835037,138.304881329776,138.461929438929,138.619025533127,
138.776461194097,138.832144123754,138.989569982194,139.146706238805,139.303673733544,
139.460721842697,139.617817936895,139.775253597865,139.830936527522,139.988362385962,
140.145498642573,140.302466137312,140.459514246465,140.616610340663,140.774046001633,
140.82972893129,141.010850350131,141.179838384518),.UNSPECIFIED.);
#758=B_SPLINE_CURVE_WITH_KNOTS('',3,(#32060,#32061,#32062,#32063,#32064,
#32065,#32066,#32067,#32068,#32069),.UNSPECIFIED.,.F.,.F.,(4,1,1,1,1,1,
1,4),(141.179838626806,141.828521335058,142.827313738826,143.826106142594,
144.824898546362,145.82369095013,146.822483353898,147.463023933985),
 .UNSPECIFIED.);
#759=B_SPLINE_CURVE_WITH_KNOTS('',3,(#32071,#32072,#32073,#32074,#32075,
#32076,#32077,#32078,#32079,#32080,#32081,#32082,#32083,#32084,#32085,#32086,
#32087,#32088,#32089,#32090,#32091,#32092,#32093,#32094,#32095,#32096,#32097,
#32098,#32099,#32100,#32101,#32102,#32103,#32104,#32105,#32106,#32107,#32108,
#32109,#32110,#32111,#32112,#32113,#32114,#32115,#32116,#32117,#32118,#32119,
#32120,#32121,#32122,#32123,#32124,#32125,#32126,#32127,#32128,#32129,#32130,
#32131,#32132,#32133,#32134,#32135,#32136,#32137,#32138,#32139,#32140,#32141,
#32142,#32143,#32144,#32145,#32146,#32147,#32148,#32149,#32150,#32151,#32152,
#32153,#32154,#32155,#32156,#32157,#32158,#32159,#32160,#32161,#32162,#32163,
#32164,#32165,#32166,#32167,#32168,#32169,#32170,#32171,#32172,#32173,#32174,
#32175,#32176,#32177,#32178,#32179,#32180,#32181,#32182,#32183,#32184,#32185,
#32186,#32187,#32188,#32189,#32190,#32191,#32192,#32193,#32194,#32195,#32196,
#32197,#32198,#32199,#32200),.UNSPECIFIED.,.F.,.F.,(4,3,3,3,3,3,3,3,3,3,
3,3,3,3,3,3,3,3,3,3,3,3,3,3,3,3,3,3,3,3,3,3,3,3,3,3,3,3,3,3,3,3,3,4),(147.463024178982,
147.642892926041,147.821275757666,147.978701616106,148.135837872716,148.292805367455,
148.449853476608,148.606949570805,148.764385231775,148.820068161434,148.977494019874,
149.134630276485,149.291597771224,149.448645880377,149.605741974574,149.763177635544,
149.818860565202,149.976286423642,150.133422680253,150.290390174992,150.447438284145,
150.604534378343,150.761970039313,150.81765296897,150.97507882741,151.132215084021,
151.28918257876,151.446230687913,151.603326782111,151.760762443081,151.816445372738,
151.973871231178,152.131007487789,152.287974982528,152.445023091681,152.602119185878,
152.759554846848,152.815237776506,152.971139595369,153.126754540017,153.282331372718,
153.437859901489,153.593727172196,153.746209241165),.UNSPECIFIED.);
#760=B_SPLINE_CURVE_WITH_KNOTS('',3,(#32202,#32203,#32204,#32205,#32206,
#32207,#32208,#32209,#32210,#32211,#32212),.UNSPECIFIED.,.F.,.F.,(4,1,1,
1,1,1,1,1,4),(153.746209241165,153.814030180274,154.812822584042,155.81161498781,
156.810407391578,157.809199795346,158.807992199114,159.806784602882,160.029394548344),
 .UNSPECIFIED.);
#761=B_SPLINE_CURVE_WITH_KNOTS('',3,(#32214,#32215,#32216,#32217,#32218,
#32219,#32220,#32221,#32222,#32223,#32224,#32225,#32226,#32227,#32228,#32229,
#32230,#32231,#32232,#32233,#32234,#32235,#32236,#32237,#32238,#32239,#32240,
#32241,#32242,#32243,#32244,#32245,#32246,#32247,#32248,#32249,#32250,#32251,
#32252,#32253,#32254,#32255,#32256,#32257,#32258,#32259,#32260,#32261,#32262,
#32263,#32264,#32265,#32266,#32267,#32268,#32269,#32270,#32271,#32272,#32273,
#32274,#32275,#32276,#32277,#32278,#32279,#32280,#32281,#32282,#32283,#32284,
#32285,#32286,#32287,#32288,#32289,#32290,#32291,#32292,#32293,#32294,#32295,
#32296,#32297,#32298,#32299,#32300,#32301,#32302,#32303,#32304,#32305,#32306,
#32307,#32308,#32309,#32310,#32311,#32312,#32313,#32314,#32315,#32316,#32317,
#32318,#32319,#32320,#32321,#32322,#32323,#32324,#32325,#32326,#32327,#32328,
#32329,#32330,#32331,#32332,#32333,#32334,#32335,#32336,#32337,#32338,#32339,
#32340,#32341,#32342,#32343,#32344,#32345,#32346),.UNSPECIFIED.,.F.,.F.,
(4,3,3,3,3,3,3,3,3,3,3,3,3,3,3,3,3,3,3,3,3,3,3,3,3,3,3,3,3,3,3,3,3,3,3,
3,3,3,3,3,3,3,3,3,4),(160.029394548344,160.184418985519,160.339708490802,
160.494663051404,160.650120029027,160.80557700665,160.96300286509,161.1201391217,
161.27710661644,161.434154725593,161.59125081979,161.74868648076,161.804369410418,
161.961795268858,162.118931525469,162.275899020208,162.432947129361,162.590043223559,
162.747478884529,162.803161814186,162.960587672626,163.117723929237,163.274691423976,
163.431739533129,163.588835627327,163.746271288297,163.801954217954,163.959380076394,
164.116516333005,164.273483827744,164.430531936897,164.587628031094,164.745063692064,
164.800746621722,164.958172480162,165.115308736773,165.272276231512,165.429324340665,
165.586420434863,165.743856095833,165.79953902549,165.96400090799,166.12802293368,
166.291588382925,166.312579855524),.UNSPECIFIED.);
#762=B_SPLINE_CURVE_WITH_KNOTS('',3,(#32348,#32349,#32350,#32351,#32352,
#32353,#32354,#32355,#32356,#32357),.UNSPECIFIED.,.F.,.F.,(4,1,1,1,1,1,
1,4),(166.31258091617,166.798331429258,167.797123833026,168.795916236794,
169.794708640562,170.79350104433,171.792293448098,172.595761427539),
 .UNSPECIFIED.);
#763=B_SPLINE_CURVE_WITH_KNOTS('',3,(#32359,#32360,#32361,#32362,#32363,
#32364,#32365,#32366,#32367,#32368,#32369,#32370,#32371,#32372,#32373,#32374,
#32375,#32376,#32377,#32378,#32379,#32380,#32381,#32382,#32383,#32384,#32385,
#32386,#32387,#32388,#32389,#32390,#32391,#32392,#32393,#32394,#32395,#32396,
#32397,#32398,#32399,#32400,#32401,#32402,#32403,#32404,#32405,#32406,#32407,
#32408,#32409,#32410,#32411,#32412,#32413,#32414,#32415,#32416,#32417,#32418,
#32419,#32420,#32421,#32422,#32423,#32424,#32425,#32426,#32427,#32428,#32429,
#32430,#32431,#32432,#32433,#32434,#32435,#32436,#32437,#32438,#32439,#32440,
#32441,#32442,#32443,#32444,#32445,#32446,#32447,#32448,#32449,#32450,#32451,
#32452,#32453,#32454,#32455,#32456,#32457,#32458,#32459,#32460,#32461,#32462,
#32463,#32464,#32465,#32466,#32467,#32468,#32469,#32470,#32471,#32472,#32473,
#32474,#32475,#32476,#32477,#32478,#32479,#32480,#32481,#32482,#32483,#32484,
#32485,#32486,#32487,#32488,#32489,#32490,#32491),.UNSPECIFIED.,.F.,.F.,
(4,3,3,3,3,3,3,3,3,3,3,3,3,3,3,3,3,3,3,3,3,3,3,3,3,3,3,3,3,3,3,3,3,3,3,
3,3,3,3,3,3,3,3,3,4),(172.595765162704,172.791085851866,172.948511710308,
173.105647966921,173.262615461662,173.419663570818,173.576759665017,173.734195325989,
173.789878255634,173.947304114074,174.104440370684,174.261407865423,174.418455974576,
174.575552068773,174.732987729743,174.788670659402,174.946096517842,175.103232774452,
175.260200269191,175.417248378344,175.574344472541,175.731780133511,175.78746306317,
175.944888921611,176.102025178221,176.25899267296,176.416040782114,176.573136876312,
176.730572537282,176.786255466938,176.943681325378,177.100817581989,177.257785076728,
177.414833185881,177.571929280079,177.729364941049,177.785047870706,177.942473729146,
178.099609985756,178.256577480495,178.413625589649,178.570721683846,178.728157344816,
178.783840274474,178.878950469883),.UNSPECIFIED.);
#764=B_SPLINE_CURVE_WITH_KNOTS('',3,(#32493,#32494,#32495,#32496,#32497,
#32498,#32499,#32500,#32501,#32502),.UNSPECIFIED.,.F.,.F.,(4,1,1,1,1,1,
1,4),(178.878959343412,179.782632678242,180.781425082011,181.780217485779,
182.779009889547,183.777802293315,184.776594697083,185.162128430314),
 .UNSPECIFIED.);
#765=B_SPLINE_CURVE_WITH_KNOTS('',3,(#32504,#32505,#32506,#32507,#32508,
#32509,#32510,#32511,#32512,#32513,#32514,#32515,#32516,#32517,#32518,#32519,
#32520,#32521,#32522,#32523,#32524,#32525,#32526,#32527,#32528,#32529,#32530,
#32531,#32532,#32533,#32534,#32535,#32536,#32537,#32538,#32539,#32540,#32541,
#32542,#32543,#32544,#32545,#32546,#32547,#32548,#32549,#32550,#32551,#32552,
#32553,#32554,#32555,#32556,#32557,#32558,#32559,#32560,#32561,#32562,#32563,
#32564,#32565,#32566,#32567,#32568,#32569,#32570,#32571,#32572,#32573,#32574,
#32575,#32576,#32577,#32578,#32579,#32580,#32581,#32582,#32583,#32584,#32585,
#32586,#32587,#32588,#32589,#32590,#32591,#32592,#32593,#32594,#32595,#32596,
#32597,#32598,#32599,#32600,#32601,#32602,#32603,#32604,#32605,#32606,#32607,
#32608,#32609,#32610,#32611,#32612,#32613,#32614,#32615,#32616,#32617,#32618,
#32619,#32620,#32621,#32622,#32623,#32624,#32625,#32626,#32627,#32628,#32629,
#32630,#32631,#32632,#32633,#32634,#32635,#32636),.UNSPECIFIED.,.F.,.F.,
(4,3,3,3,3,3,3,3,3,3,3,3,3,3,3,3,3,3,3,3,3,3,3,3,3,3,3,3,3,3,3,3,3,3,3,
3,3,3,3,3,3,3,3,3,4),(185.162135777063,185.320796314776,185.479504458316,
185.638644472916,185.775387100851,185.932812959291,186.089949215902,186.246916710641,
186.403964819794,186.561060913992,186.718496574962,186.774179504619,186.931605363059,
187.08874161967,187.245709114409,187.402757223562,187.559853317759,187.717288978729,
187.772971908387,187.930397766827,188.087534023438,188.244501518177,188.401549627331,
188.558645721528,188.716081382498,188.771764312155,188.929190170595,189.086326427206,
189.243293921945,189.400342031098,189.557438125296,189.714873786266,189.770556715923,
189.927982574364,190.085118830974,190.242086325713,190.399134434867,190.556230529064,
190.713666190034,190.769349119691,190.926450963375,191.083227689836,191.239819279954,
191.396408525495,191.445321084242),.UNSPECIFIED.);
#766=B_SPLINE_CURVE_WITH_KNOTS('',3,(#32638,#32639,#32640,#32641,#32642,
#32643,#32644,#32645,#32646,#32647,#32648,#32649,#32650,#32651,#32652,#32653,
#32654,#32655,#32656,#32657,#32658,#32659,#32660,#32661,#32662,#32663,#32664,
#32665,#32666,#32667,#32668,#32669,#32670,#32671,#32672,#32673,#32674,#32675,
#32676,#32677,#32678,#32679,#32680,#32681,#32682,#32683,#32684,#32685,#32686,
#32687,#32688,#32689,#32690,#32691,#32692,#32693,#32694,#32695,#32696,#32697,
#32698,#32699,#32700,#32701,#32702,#32703,#32704,#32705,#32706,#32707,#32708,
#32709,#32710,#32711,#32712,#32713,#32714,#32715,#32716,#32717,#32718,#32719,
#32720,#32721,#32722,#32723,#32724,#32725,#32726,#32727,#32728,#32729,#32730,
#32731,#32732,#32733,#32734,#32735,#32736,#32737,#32738,#32739,#32740,#32741,
#32742,#32743,#32744,#32745,#32746,#32747,#32748,#32749,#32750,#32751,#32752,
#32753,#32754,#32755,#32756,#32757,#32758,#32759,#32760,#32761,#32762,#32763,
#32764,#32765,#32766,#32767,#32768,#32769,#32770),.UNSPECIFIED.,.F.,.F.,
(4,3,3,3,3,3,3,3,3,3,3,3,3,3,3,3,3,3,3,3,3,3,3,3,3,3,3,3,3,3,3,3,3,3,3,
3,3,3,3,3,3,3,3,3,4),(191.44532108445,191.631142952482,191.768141523459,
191.925567381899,192.082703638508,192.239671133246,192.396719242399,192.553815336595,
192.711250997564,192.766933927227,192.924359785667,193.081496042278,193.238463537017,
193.39551164617,193.552607740368,193.710043401338,193.765726330995,193.923152189436,
194.080288446046,194.237255940785,194.394304049939,194.551400144136,194.708835805107,
194.764518734763,194.921944593203,195.079080849813,195.236048344553,195.393096453706,
195.550192547903,195.707628208873,195.763311138531,195.920736996971,196.077873253582,
196.234840748321,196.391888857474,196.548984951672,196.706420612642,196.762103542299,
196.918699351543,197.075007110055,197.238381930338,197.39460584084,197.550891671694,
197.70749924213,197.728506391186),.UNSPECIFIED.);
#767=B_SPLINE_CURVE_WITH_KNOTS('',3,(#32772,#32773,#32774,#32775,#32776,
#32777,#32778,#32779,#32780,#32781,#32782,#32783,#32784,#32785,#32786,#32787,
#32788,#32789,#32790,#32791,#32792,#32793,#32794,#32795,#32796,#32797,#32798,
#32799,#32800,#32801,#32802,#32803,#32804,#32805,#32806,#32807,#32808,#32809,
#32810,#32811,#32812,#32813,#32814,#32815,#32816,#32817,#32818,#32819,#32820,
#32821,#32822,#32823,#32824,#32825,#32826,#32827,#32828,#32829,#32830,#32831,
#32832,#32833,#32834,#32835,#32836,#32837,#32838,#32839,#32840,#32841,#32842,
#32843,#32844,#32845,#32846,#32847,#32848,#32849,#32850,#32851,#32852,#32853,
#32854,#32855,#32856,#32857,#32858,#32859,#32860,#32861,#32862,#32863,#32864,
#32865,#32866,#32867,#32868,#32869,#32870,#32871,#32872,#32873,#32874,#32875,
#32876,#32877,#32878,#32879,#32880,#32881,#32882,#32883,#32884,#32885,#32886,
#32887,#32888,#32889,#32890,#32891,#32892,#32893,#32894,#32895,#32896,#32897,
#32898,#32899,#32900,#32901,#32902,#32903,#32904,#32905,#32906,#32907),
 .UNSPECIFIED.,.F.,.F.,(4,3,3,3,3,3,3,3,3,3,3,3,3,3,3,3,3,3,3,3,3,3,3,3,
3,3,3,3,3,3,3,3,3,3,3,3,3,3,3,3,3,3,3,3,3,4),(197.728506391422,197.760895946067,
197.918321804507,198.075458061117,198.232425555857,198.38947366501,198.546569759207,
198.704005420177,198.759688349835,198.917114208275,199.074250464886,199.231217959625,
199.388266068778,199.545362162976,199.702797823946,199.758480753603,199.915906612043,
200.073042868654,200.230010363393,200.387058472546,200.544154566744,200.701590227714,
200.757273157371,200.914699015811,201.071835272422,201.228802767161,201.385850876314,
201.542946970511,201.700382631481,201.756065561139,201.913491419579,202.07062767619,
202.227595170929,202.384643280082,202.54173937428,202.69917503525,202.754857964907,
202.912283823348,203.069420079958,203.226387574697,203.383435683851,203.540531778049,
203.697967439019,203.753650368675,203.955064998701,204.011691621862),
 .UNSPECIFIED.);
#768=B_SPLINE_CURVE_WITH_KNOTS('',3,(#32909,#32910,#32911,#32912,#32913,
#32914,#32915,#32916,#32917,#32918),.UNSPECIFIED.,.F.,.F.,(4,1,1,1,1,1,
1,4),(204.011691698601,204.752442772443,205.751235176211,206.750027579979,
207.748819983747,208.747612387515,209.746404791283,210.294877005781),
 .UNSPECIFIED.);
#769=B_SPLINE_CURVE_WITH_KNOTS('',3,(#32920,#32921,#32922,#32923,#32924,
#32925,#32926,#32927,#32928,#32929,#32930,#32931,#32932,#32933,#32934,#32935,
#32936,#32937,#32938,#32939,#32940,#32941,#32942,#32943,#32944,#32945,#32946,
#32947,#32948,#32949,#32950,#32951,#32952,#32953,#32954,#32955,#32956,#32957,
#32958,#32959,#32960,#32961,#32962,#32963,#32964,#32965,#32966,#32967,#32968,
#32969,#32970,#32971,#32972,#32973,#32974,#32975,#32976,#32977,#32978,#32979,
#32980,#32981,#32982,#32983,#32984,#32985,#32986,#32987,#32988,#32989,#32990,
#32991,#32992,#32993,#32994,#32995,#32996,#32997,#32998,#32999,#33000,#33001,
#33002,#33003,#33004,#33005,#33006,#33007,#33008,#33009,#33010,#33011,#33012,
#33013,#33014,#33015,#33016,#33017,#33018,#33019,#33020,#33021,#33022,#33023,
#33024,#33025,#33026,#33027,#33028,#33029,#33030,#33031,#33032,#33033,#33034,
#33035,#33036,#33037,#33038,#33039,#33040,#33041,#33042,#33043,#33044,#33045,
#33046,#33047,#33048,#33049,#33050,#33051,#33052),.UNSPECIFIED.,.F.,.F.,
(4,3,3,3,3,3,3,3,3,3,3,3,3,3,3,3,3,3,3,3,3,3,3,3,3,3,3,3,3,3,3,3,3,3,3,
3,3,3,3,3,3,3,3,3,4),(210.294877264932,210.46333437215,210.632735937725,
210.745197195051,210.902623053491,211.059759310102,211.216726804841,211.373774913994,
211.530871008192,211.688306669162,211.743989598819,211.901415457259,212.05855171387,
212.215519208609,212.372567317762,212.52966341196,212.68709907293,212.742782002587,
212.900207861027,213.057344117638,213.214311612377,213.37135972153,213.528455815728,
213.685891476698,213.741574406355,213.899000264795,214.056136521406,214.213104016145,
214.370152125298,214.527248219496,214.684683880466,214.740366810123,214.897792668563,
215.054928925173,215.211896419913,215.368944529066,215.526040623263,215.683476284233,
215.739159213891,215.894242030097,216.04903664284,216.203757367494,216.358434417139,
216.513343457364,216.578062312961),.UNSPECIFIED.);
#770=B_SPLINE_CURVE_WITH_KNOTS('',3,(#33054,#33055,#33056,#33057,#33058,
#33059,#33060,#33061,#33062,#33063,#33064),.UNSPECIFIED.,.F.,.F.,(4,1,1,
1,1,1,1,1,4),(216.578062312961,216.737951617659,217.736744021427,218.735536425195,
219.734328828963,220.733121232731,221.731913636499,222.730706040267,222.86124762014),
 .UNSPECIFIED.);
#771=B_SPLINE_CURVE_WITH_KNOTS('',3,(#33066,#33067,#33068,#33069,#33070,
#33071,#33072,#33073,#33074,#33075,#33076,#33077,#33078,#33079,#33080,#33081,
#33082,#33083,#33084,#33085,#33086,#33087,#33088,#33089,#33090,#33091,#33092,
#33093,#33094,#33095,#33096,#33097,#33098,#33099,#33100,#33101,#33102,#33103,
#33104,#33105,#33106,#33107,#33108,#33109,#33110,#33111,#33112,#33113,#33114,
#33115,#33116,#33117,#33118,#33119,#33120,#33121,#33122,#33123,#33124,#33125,
#33126,#33127,#33128,#33129,#33130,#33131,#33132,#33133,#33134,#33135,#33136,
#33137,#33138,#33139,#33140,#33141,#33142,#33143,#33144,#33145,#33146,#33147,
#33148,#33149,#33150,#33151,#33152,#33153,#33154,#33155,#33156,#33157,#33158,
#33159,#33160,#33161,#33162,#33163,#33164,#33165,#33166,#33167,#33168,#33169,
#33170,#33171,#33172,#33173,#33174,#33175,#33176,#33177,#33178,#33179,#33180,
#33181,#33182,#33183,#33184,#33185,#33186,#33187,#33188,#33189,#33190,#33191,
#33192,#33193,#33194,#33195,#33196,#33197,#33198),.UNSPECIFIED.,.F.,.F.,
(4,3,3,3,3,3,3,3,3,3,3,3,3,3,3,3,3,3,3,3,3,3,3,3,3,3,3,3,3,3,3,3,3,3,3,
3,3,3,3,3,3,3,3,3,4),(222.86124762014,223.016316100705,223.171149712576,
223.326001519616,223.480853724508,223.636041436024,223.729498444035,223.886924302475,
224.044060559086,224.201028053825,224.358076162978,224.515172257176,224.672607918146,
224.728290847803,224.885716706243,225.042852962854,225.199820457593,225.356868566746,
225.513964660944,225.671400321914,225.727083251571,225.884509110011,226.041645366622,
226.198612861361,226.355660970514,226.512757064712,226.670192725682,226.725875655339,
226.883301513779,227.04043777039,227.197405265129,227.354453374282,227.51154946848,
227.66898512945,227.724668059107,227.882093917547,228.039230174158,228.196197668897,
228.35324577805,228.510341872248,228.667777533218,228.723460462875,228.895945905797,
229.067330276234,229.144432927137),.UNSPECIFIED.);
#772=B_SPLINE_CURVE_WITH_KNOTS('',3,(#33200,#33201,#33202,#33203,#33204,
#33205,#33206,#33207,#33208,#33209,#33210,#33211,#33212,#33213,#33214,#33215,
#33216,#33217,#33218,#33219,#33220,#33221,#33222,#33223,#33224,#33225,#33226,
#33227,#33228,#33229,#33230,#33231,#33232,#33233,#33234,#33235,#33236,#33237,
#33238,#33239,#33240,#33241,#33242,#33243,#33244,#33245,#33246,#33247,#33248,
#33249,#33250,#33251,#33252,#33253,#33254,#33255,#33256,#33257,#33258,#33259,
#33260,#33261,#33262,#33263,#33264,#33265,#33266,#33267,#33268,#33269,#33270,
#33271,#33272,#33273,#33274,#33275,#33276,#33277,#33278,#33279,#33280,#33281,
#33282,#33283,#33284,#33285,#33286,#33287,#33288,#33289,#33290,#33291,#33292,
#33293,#33294,#33295,#33296,#33297,#33298,#33299,#33300,#33301,#33302,#33303,
#33304,#33305,#33306,#33307,#33308,#33309,#33310,#33311,#33312,#33313,#33314,
#33315,#33316,#33317,#33318,#33319,#33320,#33321,#33322,#33323,#33324,#33325,
#33326,#33327,#33328,#33329,#33330,#33331,#33332),.UNSPECIFIED.,.F.,.F.,
(4,3,3,3,3,3,3,3,3,3,3,3,3,3,3,3,3,3,3,3,3,3,3,3,3,3,3,3,3,3,3,3,3,3,3,
3,3,3,3,3,3,3,3,3,4),(229.14443292732,229.304574268111,229.464832452386,
229.625550244693,229.722252866643,229.879678725084,230.036814981694,230.193782476433,
230.350830585587,230.507926679784,230.665362340755,230.721045270411,230.878471128851,
231.035607385462,231.192574880201,231.349622989354,231.506719083552,231.664154744522,
231.719837674179,231.877263532619,232.03439978923,232.191367283969,232.348415393122,
232.50551148732,232.66294714829,232.718630077947,232.876055936387,233.033192192998,
233.190159687737,233.34720779689,233.504303891088,233.661739552058,233.717422481715,
233.874848340155,234.031984596766,234.188952091505,234.346000200658,234.503096294856,
234.660531955826,234.716214885483,234.872477893564,235.028448536676,235.184246088232,
235.34009904764,235.427618234499),.UNSPECIFIED.);
#773=B_SPLINE_CURVE_WITH_KNOTS('',3,(#33334,#33335,#33336,#33337,#33338,
#33339,#33340,#33341,#33342,#33343,#33344,#33345,#33346,#33347,#33348,#33349,
#33350,#33351,#33352,#33353,#33354,#33355,#33356,#33357,#33358,#33359,#33360,
#33361,#33362,#33363,#33364,#33365,#33366,#33367,#33368,#33369,#33370,#33371,
#33372,#33373,#33374,#33375,#33376,#33377,#33378,#33379,#33380,#33381,#33382,
#33383,#33384,#33385,#33386,#33387,#33388,#33389,#33390,#33391,#33392,#33393,
#33394,#33395,#33396,#33397,#33398,#33399,#33400,#33401,#33402,#33403,#33404,
#33405,#33406,#33407,#33408,#33409,#33410,#33411,#33412,#33413,#33414,#33415,
#33416,#33417,#33418,#33419,#33420,#33421,#33422,#33423,#33424,#33425,#33426,
#33427,#33428,#33429,#33430,#33431,#33432,#33433,#33434,#33435,#33436,#33437,
#33438,#33439,#33440,#33441,#33442,#33443,#33444,#33445,#33446,#33447,#33448,
#33449,#33450,#33451,#33452,#33453,#33454,#33455,#33456,#33457,#33458,#33459,
#33460,#33461,#33462,#33463,#33464,#33465,#33466,#33467,#33468,#33469),
 .UNSPECIFIED.,.F.,.F.,(4,3,3,3,3,3,3,3,3,3,3,3,3,3,3,3,3,3,3,3,3,3,3,3,
3,3,3,3,3,3,3,3,3,3,3,3,3,3,3,3,3,3,3,3,3,4),(235.427618234645,235.621005037013,
235.715007289251,235.872433147691,236.029569404302,236.186536899041,236.343585008195,
236.500681102392,236.658116763362,236.713799693019,236.871225551459,237.02836180807,
237.185329302809,237.342377411962,237.49947350616,237.65690916713,237.712592096787,
237.870017955227,238.027154211838,238.184121706577,238.34116981573,238.498265909927,
238.655701570897,238.711384500555,238.868810358995,239.025946615606,239.182914110345,
239.339962219498,239.497058313696,239.654493974666,239.710176904323,239.867602762763,
240.024739019374,240.181706514113,240.338754623266,240.495850717464,240.653286378434,
240.708969308091,240.866395166531,241.023531423141,241.18049891788,241.337547027033,
241.49464312123,241.6520787822,241.707761711859,241.710803541679),
 .UNSPECIFIED.);
#774=B_SPLINE_CURVE_WITH_KNOTS('',3,(#33471,#33472,#33473,#33474,#33475,
#33476,#33477,#33478,#33479,#33480,#33481,#33482,#33483,#33484,#33485,#33486,
#33487,#33488,#33489,#33490,#33491,#33492,#33493,#33494,#33495,#33496,#33497,
#33498,#33499,#33500,#33501,#33502,#33503,#33504,#33505,#33506,#33507,#33508,
#33509,#33510,#33511,#33512,#33513,#33514,#33515,#33516,#33517,#33518,#33519,
#33520,#33521,#33522,#33523,#33524,#33525,#33526,#33527,#33528,#33529,#33530,
#33531,#33532,#33533,#33534,#33535,#33536,#33537,#33538,#33539,#33540,#33541,
#33542,#33543,#33544,#33545,#33546,#33547,#33548,#33549,#33550,#33551,#33552,
#33553,#33554,#33555,#33556,#33557,#33558,#33559,#33560,#33561,#33562,#33563,
#33564,#33565,#33566,#33567,#33568,#33569,#33570,#33571,#33572,#33573,#33574,
#33575,#33576,#33577,#33578,#33579,#33580,#33581,#33582,#33583,#33584,#33585,
#33586,#33587,#33588,#33589,#33590,#33591,#33592,#33593,#33594,#33595,#33596,
#33597,#33598,#33599,#33600,#33601,#33602,#33603),.UNSPECIFIED.,.F.,.F.,
(4,3,3,3,3,3,3,3,3,3,3,3,3,3,3,3,3,3,3,3,3,3,3,3,3,3,3,3,3,3,3,3,3,3,3,
3,3,3,3,3,3,3,3,3,4),(241.710803541844,241.868143106838,242.02519326494,
242.1820751511,242.339037937249,242.496049703508,242.653399897405,242.706554115627,
242.863979974067,243.021116230678,243.178083725417,243.33513183457,243.492227928768,
243.649663589738,243.705346519395,243.862772377836,244.019908634446,244.176876129185,
244.333924238339,244.491020332536,244.648455993506,244.704138923163,244.861564781603,
245.018701038214,245.175668532953,245.332716642106,245.489812736304,245.647248397274,
245.702931326931,245.860357185371,246.017493441982,246.174460936721,246.331509045874,
246.488605140071,246.646040801041,246.701723730699,246.859149589139,247.01628584575,
247.173253340489,247.330301449642,247.48739754384,247.64483320481,247.700516134467,
247.89246141975,247.993988848699),.UNSPECIFIED.);
#775=B_SPLINE_CURVE_WITH_KNOTS('',3,(#33605,#33606,#33607,#33608,#33609,
#33610,#33611,#33612,#33613,#33614,#33615,#33616,#33617,#33618,#33619,#33620,
#33621,#33622,#33623,#33624,#33625,#33626,#33627,#33628,#33629,#33630,#33631,
#33632,#33633,#33634,#33635,#33636,#33637,#33638,#33639,#33640,#33641,#33642,
#33643,#33644,#33645,#33646,#33647,#33648,#33649,#33650,#33651,#33652,#33653,
#33654,#33655,#33656,#33657,#33658,#33659,#33660,#33661,#33662,#33663,#33664,
#33665,#33666,#33667,#33668,#33669,#33670,#33671,#33672,#33673,#33674,#33675,
#33676,#33677,#33678,#33679,#33680,#33681,#33682,#33683,#33684,#33685,#33686,
#33687,#33688,#33689,#33690,#33691,#33692,#33693,#33694,#33695,#33696,#33697,
#33698,#33699,#33700,#33701,#33702,#33703,#33704,#33705,#33706,#33707,#33708,
#33709,#33710,#33711,#33712,#33713,#33714,#33715,#33716,#33717,#33718,#33719,
#33720,#33721,#33722,#33723,#33724,#33725,#33726,#33727,#33728,#33729,#33730,
#33731,#33732,#33733,#33734,#33735,#33736,#33737),.UNSPECIFIED.,.F.,.F.,
(4,3,3,3,3,3,3,3,3,3,3,3,3,3,3,3,3,3,3,3,3,3,3,3,3,3,3,3,3,3,3,3,3,3,3,
3,3,3,3,3,3,3,3,3,4),(247.993988848858,248.149923326116,248.305914227325,
248.461931588476,248.618298001352,248.699308538235,248.856734396675,249.013870653285,
249.170838148025,249.327886257178,249.484982351375,249.642418012345,249.698100942003,
249.855526800444,250.012663057055,250.169630551794,250.326678660948,250.483774755146,
250.641210416116,250.696893345772,250.854319204212,251.011455460823,251.168422955562,
251.325471064715,251.482567158913,251.640002819883,251.69568574954,251.85311160798,
252.01024786459,252.167215359329,252.324263468482,252.48135956268,252.63879522365,
252.694478153308,252.851904011749,253.009040268359,253.166007763098,253.323055872252,
253.480151966449,253.637587627419,253.693270557076,253.853683463077,254.013749755245,
254.173572614727,254.277174156038),.UNSPECIFIED.);
#776=B_SPLINE_CURVE_WITH_KNOTS('',3,(#33739,#33740,#33741,#33742,#33743,
#33744,#33745,#33746,#33747,#33748,#33749,#33750,#33751,#33752,#33753,#33754,
#33755,#33756,#33757,#33758,#33759,#33760,#33761,#33762,#33763,#33764,#33765,
#33766,#33767,#33768,#33769,#33770,#33771,#33772,#33773,#33774,#33775,#33776,
#33777,#33778,#33779,#33780,#33781,#33782,#33783,#33784,#33785,#33786,#33787,
#33788,#33789,#33790,#33791,#33792,#33793,#33794,#33795,#33796,#33797,#33798,
#33799,#33800,#33801,#33802,#33803,#33804,#33805,#33806,#33807,#33808,#33809,
#33810,#33811,#33812,#33813,#33814,#33815,#33816,#33817,#33818,#33819,#33820,
#33821,#33822,#33823,#33824,#33825,#33826,#33827,#33828,#33829,#33830,#33831,
#33832,#33833,#33834,#33835,#33836,#33837,#33838,#33839,#33840,#33841,#33842,
#33843,#33844,#33845,#33846,#33847,#33848,#33849,#33850,#33851,#33852,#33853,
#33854,#33855,#33856,#33857,#33858,#33859,#33860,#33861,#33862,#33863,#33864,
#33865,#33866,#33867,#33868,#33869,#33870,#33871),.UNSPECIFIED.,.F.,.F.,
(4,3,3,3,3,3,3,3,3,3,3,3,3,3,3,3,3,3,3,3,3,3,3,3,3,3,3,3,3,3,3,3,3,3,3,
3,3,3,3,3,3,3,3,3,4),(254.27717415623,254.449061850417,254.622135068757,
254.692062960844,254.849488819284,255.006625075894,255.163592570633,255.320640679786,
255.477736773983,255.635172434953,255.690855364612,255.848281223052,256.005417479663,
256.162384974402,256.319433083555,256.476529177753,256.633964838723,256.68964776838,
256.84707362682,257.004209883431,257.16117737817,257.318225487324,257.475321581521,
257.632757242491,257.688440172148,257.845866030588,258.003002287199,258.159969781938,
258.317017891091,258.474113985288,258.631549646258,258.687232575916,258.844658434356,
259.001794690967,259.158762185706,259.315810294859,259.472906389057,259.630342050027,
259.686024979684,259.841258359922,259.996204973962,260.151093896897,260.305938742112,
260.461058165079,260.560359463218),.UNSPECIFIED.);
#777=B_SPLINE_CURVE_WITH_KNOTS('',3,(#33873,#33874,#33875,#33876,#33877,
#33878,#33879,#33880,#33881,#33882,#33883),.UNSPECIFIED.,.F.,.F.,(4,1,1,
1,1,1,1,1,4),(260.560359463218,260.684817383452,261.68360978722,262.682402190988,
263.681194594756,264.679986998524,265.678779402292,266.67757180606,266.843544770397),
 .UNSPECIFIED.);
#778=B_SPLINE_CURVE_WITH_KNOTS('',3,(#33885,#33886,#33887,#33888,#33889,
#33890,#33891,#33892,#33893,#33894,#33895,#33896,#33897,#33898,#33899,#33900,
#33901,#33902,#33903,#33904,#33905,#33906,#33907,#33908,#33909,#33910,#33911,
#33912,#33913,#33914,#33915,#33916,#33917,#33918,#33919,#33920,#33921,#33922,
#33923,#33924,#33925,#33926,#33927,#33928,#33929,#33930,#33931,#33932,#33933,
#33934,#33935,#33936,#33937,#33938,#33939,#33940,#33941,#33942,#33943,#33944,
#33945,#33946,#33947,#33948,#33949,#33950,#33951,#33952,#33953,#33954,#33955,
#33956,#33957,#33958,#33959,#33960,#33961,#33962,#33963,#33964,#33965,#33966,
#33967,#33968,#33969,#33970,#33971,#33972,#33973,#33974,#33975,#33976,#33977,
#33978,#33979,#33980,#33981,#33982,#33983,#33984,#33985,#33986,#33987,#33988,
#33989,#33990,#33991,#33992,#33993,#33994,#33995,#33996,#33997,#33998,#33999,
#34000,#34001,#34002,#34003,#34004,#34005,#34006,#34007,#34008,#34009,#34010,
#34011,#34012,#34013,#34014,#34015,#34016,#34017),.UNSPECIFIED.,.F.,.F.,
(4,3,3,3,3,3,3,3,3,3,3,3,3,3,3,3,3,3,3,3,3,3,3,3,3,3,3,3,3,3,3,3,3,3,3,
3,3,3,3,3,3,3,3,3,4),(266.843544770397,266.998437545715,267.153122139019,
267.3078484695,267.4625994556,267.617675353046,267.676364209828,267.833790068268,
267.990926324879,268.147893819617,268.304941928771,268.462038022968,268.619473683938,
268.675156613596,268.832582472036,268.989718728646,269.146686223386,269.303734332539,
269.460830426736,269.618266087706,269.673949017364,269.831374875804,269.988511132415,
270.145478627154,270.302526736308,270.459622830505,270.617058491475,270.672741421132,
270.830167279572,270.987303536183,271.144271030922,271.301319140075,271.458415234273,
271.615850895243,271.6715338249,271.82895968334,271.986095939951,272.14306343469,
272.300111543843,272.457207638041,272.614643299011,272.670326228668,272.839266884683,
273.007357802531,273.126729847806),.UNSPECIFIED.);
#779=B_SPLINE_CURVE_WITH_KNOTS('',3,(#34019,#34020,#34021,#34022,#34023,
#34024,#34025,#34026,#34027,#34028),.UNSPECIFIED.,.F.,.F.,(4,1,1,1,1,1,
1,4),(273.126730077577,273.669118632436,274.667911036204,275.666703439972,
276.66549584374,277.664288247508,278.663080651276,279.409915384756),
 .UNSPECIFIED.);
#780=B_SPLINE_CURVE_WITH_KNOTS('',3,(#34030,#34031,#34032,#34033,#34034,
#34035,#34036,#34037,#34038,#34039,#34040,#34041,#34042,#34043,#34044,#34045,
#34046,#34047,#34048,#34049,#34050,#34051,#34052,#34053,#34054,#34055,#34056,
#34057,#34058,#34059,#34060,#34061,#34062,#34063,#34064,#34065,#34066,#34067,
#34068,#34069,#34070,#34071,#34072,#34073,#34074,#34075,#34076,#34077,#34078,
#34079,#34080,#34081,#34082,#34083,#34084,#34085,#34086,#34087,#34088,#34089,
#34090,#34091,#34092,#34093,#34094,#34095,#34096,#34097,#34098,#34099,#34100,
#34101,#34102,#34103,#34104,#34105,#34106,#34107,#34108,#34109,#34110,#34111,
#34112,#34113,#34114,#34115,#34116,#34117,#34118,#34119,#34120,#34121,#34122,
#34123,#34124,#34125,#34126,#34127,#34128,#34129,#34130,#34131,#34132,#34133,
#34134,#34135,#34136,#34137,#34138,#34139,#34140,#34141,#34142,#34143,#34144,
#34145,#34146,#34147,#34148,#34149,#34150,#34151,#34152,#34153,#34154,#34155,
#34156,#34157,#34158,#34159,#34160,#34161,#34162,#34163,#34164,#34165),
 .UNSPECIFIED.,.F.,.F.,(4,3,3,3,3,3,3,3,3,3,3,3,3,3,3,3,3,3,3,3,3,3,3,3,
3,3,3,3,3,3,3,3,3,3,3,3,3,3,3,3,3,3,3,3,3,4),(279.409915502333,279.613260937759,
279.661873055044,279.819298913484,279.976435170093,280.133402664831,280.290450773984,
280.447546868181,280.60498252915,280.660665458812,280.818091317252,280.975227573863,
281.132195068602,281.289243177756,281.446339271953,281.603774932923,281.65945786258,
281.816883721021,281.974019977631,282.13098747237,282.288035581524,282.445131675721,
282.602567336692,282.658250266348,282.815676124788,282.972812381398,283.129779876137,
283.286827985291,283.443924079488,283.601359740458,283.657042670116,283.814468528556,
283.971604785167,284.128572279906,284.285620389059,284.442716483257,284.600152144227,
284.655835073884,284.813260932324,284.970397188935,285.127364683674,285.284412792827,
285.441508887025,285.598944547995,285.654627477652,285.693100691936),
 .UNSPECIFIED.);
#781=B_SPLINE_CURVE_WITH_KNOTS('',3,(#34167,#34168,#34169,#34170,#34171,
#34172,#34173,#34174,#34175,#34176),.UNSPECIFIED.,.F.,.F.,(4,1,1,1,1,1,
1,4),(285.69310580607,286.65341988142,287.652212285188,288.651004688956,
289.649797092724,290.648589496492,291.64738190026,291.976278941454),
 .UNSPECIFIED.);
#782=B_SPLINE_CURVE_WITH_KNOTS('',3,(#34178,#34179,#34180,#34181,#34182,
#34183,#34184,#34185,#34186,#34187,#34188,#34189,#34190,#34191,#34192,#34193,
#34194,#34195,#34196,#34197,#34198,#34199,#34200,#34201,#34202,#34203,#34204,
#34205,#34206,#34207,#34208,#34209,#34210,#34211,#34212,#34213,#34214,#34215,
#34216,#34217,#34218,#34219,#34220,#34221,#34222,#34223,#34224,#34225,#34226,
#34227,#34228,#34229,#34230,#34231,#34232,#34233,#34234,#34235,#34236,#34237,
#34238,#34239,#34240,#34241,#34242,#34243,#34244,#34245,#34246,#34247,#34248,
#34249,#34250,#34251,#34252,#34253,#34254,#34255,#34256,#34257,#34258,#34259,
#34260,#34261,#34262,#34263,#34264,#34265,#34266,#34267,#34268,#34269,#34270,
#34271,#34272,#34273,#34274,#34275,#34276,#34277,#34278,#34279,#34280,#34281,
#34282,#34283,#34284,#34285,#34286,#34287,#34288,#34289,#34290,#34291,#34292,
#34293,#34294,#34295,#34296,#34297,#34298,#34299,#34300,#34301,#34302,#34303,
#34304,#34305,#34306,#34307,#34308,#34309,#34310),.UNSPECIFIED.,.F.,.F.,
(4,3,3,3,3,3,3,3,3,3,3,3,3,3,3,3,3,3,3,3,3,3,3,3,3,3,3,3,3,3,3,3,3,3,3,
3,3,3,3,3,3,3,3,3,4),(291.976285999115,292.133008839732,292.289839990702,
292.446739507181,292.603991533183,292.646174304028,292.803600162468,292.960736419079,
293.117703913818,293.274752022971,293.431848117168,293.589283778138,293.644966707796,
293.802392566236,293.959528822847,294.116496317586,294.273544426739,294.430640520936,
294.588076181906,294.643759111564,294.801184970004,294.958321226615,295.115288721354,
295.272336830507,295.429432924705,295.586868585675,295.642551515332,295.799977373772,
295.957113630383,296.114081125122,296.271129234275,296.428225328473,296.585660989443,
296.6413439191,296.79876977754,296.95590603415,297.112873528889,297.269921638043,
297.42701773224,297.58445339321,297.640136322868,297.799036718426,297.957616676704,
298.116041131907,298.259471306295),.UNSPECIFIED.);
#783=B_SPLINE_CURVE_WITH_KNOTS('',3,(#34312,#34313,#34314,#34315,#34316,
#34317,#34318,#34319,#34320,#34321),.UNSPECIFIED.,.F.,.F.,(4,1,1,1,1,1,
1,4),(298.259478779105,298.638928726636,299.637721130404,300.636513534172,
301.63530593794,302.634098341708,303.632890745476,304.542647862618),
 .UNSPECIFIED.);
#784=B_SPLINE_CURVE_WITH_KNOTS('',3,(#34323,#34324,#34325,#34326,#34327,
#34328,#34329,#34330,#34331,#34332,#34333,#34334,#34335,#34336,#34337,#34338,
#34339,#34340,#34341,#34342,#34343,#34344,#34345,#34346,#34347,#34348,#34349,
#34350,#34351,#34352,#34353,#34354,#34355,#34356,#34357,#34358,#34359,#34360,
#34361,#34362,#34363,#34364,#34365,#34366,#34367,#34368,#34369,#34370,#34371,
#34372,#34373,#34374,#34375,#34376,#34377,#34378,#34379,#34380,#34381,#34382,
#34383,#34384,#34385,#34386,#34387,#34388,#34389,#34390,#34391,#34392,#34393,
#34394,#34395,#34396,#34397,#34398,#34399,#34400,#34401,#34402,#34403,#34404,
#34405,#34406,#34407,#34408,#34409,#34410,#34411,#34412,#34413,#34414,#34415,
#34416,#34417,#34418,#34419,#34420,#34421,#34422,#34423,#34424,#34425,#34426,
#34427,#34428,#34429,#34430,#34431,#34432,#34433,#34434,#34435,#34436,#34437,
#34438,#34439,#34440,#34441,#34442,#34443,#34444,#34445,#34446,#34447,#34448,
#34449,#34450,#34451,#34452,#34453,#34454,#34455),.UNSPECIFIED.,.F.,.F.,
(4,3,3,3,3,3,3,3,3,3,3,3,3,3,3,3,3,3,3,3,3,3,3,3,3,3,3,3,3,3,3,3,3,3,3,
3,3,3,3,3,3,3,3,3,4),(304.542656613474,304.631683149244,304.789109007684,
304.946245264295,305.103212759034,305.260260868187,305.417356962385,305.574792623355,
305.630475553012,305.787901411452,305.945037668063,306.102005162802,306.259053271955,
306.416149366152,306.573585027122,306.62926795678,306.78669381522,306.943830071831,
307.10079756657,307.257845675723,307.414941769921,307.572377430891,307.628060360548,
307.785486218988,307.942622475599,308.099589970338,308.256638079491,308.413734173689,
308.571169834659,308.626852764316,308.784278622756,308.941414879367,309.098382374106,
309.255430483259,309.412526577457,309.569962238427,309.625645168084,309.783071026524,
309.940207283134,310.097174777873,310.254222887027,310.411318981224,310.568754642194,
310.624437571852,310.825841920654),.UNSPECIFIED.);
#785=B_SPLINE_CURVE_WITH_KNOTS('',3,(#34457,#34458,#34459,#34460,#34461,
#34462,#34463,#34464,#34465,#34466,#34467,#34468,#34469,#34470,#34471,#34472,
#34473,#34474,#34475,#34476,#34477,#34478,#34479,#34480,#34481,#34482,#34483,
#34484,#34485,#34486,#34487,#34488,#34489,#34490,#34491,#34492,#34493,#34494,
#34495,#34496,#34497,#34498,#34499,#34500,#34501,#34502,#34503,#34504,#34505,
#34506,#34507,#34508,#34509,#34510,#34511,#34512,#34513,#34514,#34515,#34516,
#34517,#34518,#34519,#34520,#34521,#34522,#34523,#34524,#34525,#34526,#34527,
#34528,#34529,#34530,#34531,#34532,#34533,#34534,#34535,#34536,#34537,#34538,
#34539,#34540,#34541,#34542,#34543,#34544,#34545,#34546,#34547,#34548,#34549,
#34550,#34551,#34552,#34553,#34554,#34555,#34556,#34557,#34558,#34559,#34560,
#34561,#34562,#34563,#34564,#34565,#34566,#34567,#34568,#34569,#34570,#34571,
#34572,#34573,#34574,#34575,#34576,#34577,#34578,#34579,#34580,#34581,#34582,
#34583,#34584,#34585,#34586,#34587,#34588,#34589),.UNSPECIFIED.,.F.,.F.,
(4,3,3,3,3,3,3,3,3,3,3,3,3,3,3,3,3,3,3,3,3,3,3,3,3,3,3,3,3,3,3,3,3,3,3,
3,3,3,3,3,3,3,3,3,4),(310.825841920814,310.98075688353,311.141375156553,
311.296181572029,311.451044128878,311.606222849238,311.62322997562,311.78065583406,
311.937792090671,312.09475958541,312.251807694563,312.408903788761,312.566339449731,
312.622022379388,312.779448237828,312.936584494439,313.093551989178,313.250600098331,
313.407696192529,313.565131853499,313.620814783156,313.778240641596,313.935376898207,
314.092344392946,314.249392502099,314.406488596297,314.563924257267,314.619607186924,
314.777033045364,314.934169301975,315.091136796714,315.248184905867,315.405281000065,
315.562716661035,315.618399590692,315.775825449132,315.932961705742,316.089929200481,
316.246977309634,316.404073403831,316.561509064801,316.61719199446,316.78318166121,
316.948512755425,317.109027227671),.UNSPECIFIED.);
#786=B_SPLINE_CURVE_WITH_KNOTS('',3,(#34591,#34592,#34593,#34594,#34595,
#34596,#34597,#34598,#34599,#34600,#34601,#34602,#34603,#34604,#34605,#34606,
#34607,#34608,#34609,#34610,#34611,#34612,#34613,#34614,#34615,#34616,#34617,
#34618,#34619,#34620,#34621,#34622,#34623,#34624,#34625,#34626,#34627,#34628,
#34629,#34630,#34631,#34632,#34633,#34634,#34635,#34636,#34637,#34638,#34639,
#34640,#34641,#34642,#34643,#34644,#34645,#34646,#34647,#34648,#34649,#34650,
#34651,#34652,#34653,#34654,#34655,#34656,#34657,#34658,#34659,#34660,#34661,
#34662,#34663,#34664,#34665,#34666,#34667,#34668,#34669,#34670,#34671,#34672,
#34673,#34674,#34675,#34676,#34677,#34678,#34679,#34680,#34681,#34682,#34683,
#34684,#34685,#34686,#34687,#34688,#34689,#34690,#34691,#34692,#34693,#34694,
#34695,#34696,#34697,#34698,#34699,#34700,#34701,#34702,#34703,#34704,#34705,
#34706,#34707,#34708,#34709,#34710,#34711,#34712,#34713,#34714,#34715,#34716,
#34717,#34718,#34719,#34720),.UNSPECIFIED.,.F.,.F.,(4,3,3,3,3,3,3,3,3,3,
3,3,3,3,3,3,3,3,3,3,3,3,3,3,3,3,3,3,3,3,3,3,3,3,3,3,3,3,3,3,3,3,3,4),(317.109027227834,
317.273126322695,317.444555360461,317.615984398228,317.773410256669,317.93054651328,
318.087514008019,318.244562117173,318.401658211371,318.559093872342,318.614776801996,
318.772202660437,318.929338917047,319.086306411786,319.243354520939,319.400450615137,
319.557886276107,319.613569205764,319.770995064204,319.928131320814,320.085098815553,
320.242146924706,320.399243018903,320.556678679873,320.612361609532,320.769787467973,
320.926923724584,321.083891219324,321.240939328478,321.398035422676,321.555471083646,
321.611154013301,321.768579871741,321.925716128351,322.08268362309,322.239731732243,
322.39682782644,322.554263487409,322.609946417068,322.76521431044,322.921963866583,
323.076831294499,323.234521914756,323.392212535013),.UNSPECIFIED.);
#787=B_SPLINE_CURVE_WITH_KNOTS('',3,(#34722,#34723,#34724,#34725,#34726,
#34727,#34728,#34729,#34730,#34731,#34732),.UNSPECIFIED.,.F.,.F.,(4,1,1,
1,1,1,1,1,4),(323.392212535013,323.608738820837,324.607531224605,325.606323628372,
326.605116032141,327.603908435909,328.602700839677,329.601493243445,329.675397842193),
 .UNSPECIFIED.);
#788=B_SPLINE_CURVE_WITH_KNOTS('',3,(#34734,#34735,#34736,#34737,#34738,
#34739,#34740,#34741,#34742,#34743,#34744,#34745,#34746,#34747,#34748,#34749,
#34750,#34751,#34752,#34753,#34754,#34755,#34756,#34757,#34758,#34759,#34760,
#34761,#34762,#34763,#34764,#34765,#34766,#34767,#34768,#34769,#34770,#34771,
#34772,#34773,#34774,#34775,#34776,#34777,#34778,#34779,#34780,#34781,#34782,
#34783,#34784,#34785,#34786,#34787,#34788,#34789,#34790,#34791,#34792,#34793,
#34794,#34795,#34796,#34797,#34798,#34799,#34800,#34801,#34802,#34803,#34804,
#34805,#34806,#34807,#34808,#34809,#34810,#34811,#34812,#34813,#34814,#34815,
#34816,#34817,#34818,#34819,#34820,#34821,#34822,#34823,#34824,#34825,#34826,
#34827,#34828,#34829,#34830,#34831,#34832,#34833,#34834,#34835,#34836,#34837,
#34838,#34839,#34840,#34841,#34842,#34843,#34844,#34845,#34846,#34847,#34848,
#34849,#34850,#34851,#34852,#34853,#34854,#34855,#34856,#34857,#34858,#34859,
#34860,#34861,#34862,#34863),.UNSPECIFIED.,.F.,.F.,(4,3,3,3,3,3,3,3,3,3,
3,3,3,3,3,3,3,3,3,3,3,3,3,3,3,3,3,3,3,3,3,3,3,3,3,3,3,3,3,3,3,3,3,4),(329.675397842193,
329.831155571038,329.986644937876,330.142123120359,330.297569297493,330.453373608074,
330.600285647213,330.757711505653,330.914847762264,331.071815257003,331.228863366156,
331.385959460353,331.543395121324,331.599078050981,331.756503909421,331.913640166032,
332.070607660771,332.227655769924,332.384751864121,332.542187525091,332.597870454749,
332.755296313189,332.9124325698,333.069400064539,333.226448173692,333.38354426789,
333.54097992886,333.596662858517,333.754088716957,333.911224973568,334.068192468307,
334.22524057746,334.382336671657,334.539772332627,334.595455262285,334.752881120726,
334.910017377336,335.066984872075,335.224032981229,335.381129075426,335.538564736397,
335.594247666053,335.776415407595,335.958583149137),.UNSPECIFIED.);
#789=B_SPLINE_CURVE_WITH_KNOTS('',3,(#34865,#34866,#34867,#34868,#34869,
#34870,#34871,#34872,#34873,#34874,#34875,#34876,#34877,#34878,#34879,#34880,
#34881,#34882,#34883,#34884,#34885,#34886,#34887,#34888,#34889,#34890,#34891,
#34892,#34893,#34894,#34895,#34896,#34897,#34898,#34899,#34900,#34901,#34902,
#34903,#34904,#34905,#34906,#34907,#34908,#34909,#34910,#34911,#34912,#34913,
#34914,#34915,#34916,#34917,#34918,#34919,#34920,#34921,#34922,#34923,#34924,
#34925,#34926,#34927,#34928,#34929,#34930,#34931,#34932,#34933,#34934,#34935,
#34936,#34937,#34938,#34939,#34940,#34941,#34942,#34943,#34944,#34945,#34946,
#34947,#34948,#34949,#34950,#34951,#34952,#34953,#34954,#34955,#34956,#34957,
#34958,#34959,#34960,#34961,#34962,#34963,#34964,#34965,#34966,#34967,#34968,
#34969,#34970,#34971,#34972,#34973,#34974,#34975,#34976,#34977,#34978,#34979,
#34980,#34981,#34982,#34983,#34984,#34985,#34986,#34987,#34988,#34989,#34990,
#34991,#34992,#34993,#34994,#34995,#34996,#34997),.UNSPECIFIED.,.F.,.F.,
(4,3,3,3,3,3,3,3,3,3,3,3,3,3,3,3,3,3,3,3,3,3,3,3,3,3,3,3,3,3,3,3,3,3,3,
3,3,3,3,3,3,3,3,3,4),(335.958583149372,336.117197379484,336.275121374349,
336.434080722085,336.593040069821,336.750465928261,336.907602184871,337.06456967961,
337.221617788763,337.37871388296,337.53614954393,337.591832473589,337.749258332029,
337.90639458864,338.063362083379,338.220410192532,338.377506286729,338.534941947699,
338.590624877357,338.748050735798,338.905186992408,339.062154487147,339.219202596301,
339.376298690498,339.533734351468,339.589417281125,339.746843139565,339.903979396176,
340.060946890915,340.217995000068,340.375091094266,340.532526755236,340.588209684893,
340.745635543333,340.902771799944,341.059739294683,341.216787403836,341.373883498034,
341.531319159004,341.587002088661,341.750693680634,341.908058796137,342.065232937769,
342.222371717184,342.241768456552),.UNSPECIFIED.);
#790=B_SPLINE_CURVE_WITH_KNOTS('',3,(#34999,#35000,#35001,#35002,#35003,
#35004,#35005,#35006,#35007,#35008,#35009,#35010,#35011,#35012,#35013,#35014,
#35015,#35016,#35017,#35018,#35019,#35020,#35021,#35022,#35023,#35024,#35025,
#35026,#35027,#35028,#35029,#35030,#35031,#35032,#35033,#35034,#35035,#35036,
#35037,#35038,#35039,#35040,#35041,#35042,#35043,#35044,#35045,#35046,#35047,
#35048,#35049,#35050,#35051,#35052,#35053,#35054,#35055,#35056,#35057,#35058,
#35059,#35060,#35061,#35062,#35063,#35064,#35065,#35066,#35067,#35068,#35069,
#35070,#35071,#35072,#35073,#35074,#35075,#35076,#35077,#35078,#35079,#35080,
#35081,#35082,#35083,#35084,#35085,#35086,#35087,#35088,#35089,#35090,#35091,
#35092,#35093,#35094,#35095,#35096,#35097,#35098,#35099,#35100,#35101,#35102,
#35103,#35104,#35105,#35106,#35107,#35108,#35109,#35110,#35111,#35112,#35113,
#35114,#35115,#35116,#35117,#35118,#35119,#35120,#35121,#35122,#35123,#35124,
#35125,#35126,#35127,#35128),.UNSPECIFIED.,.F.,.F.,(4,3,3,3,3,3,3,3,3,3,
3,3,3,3,3,3,3,3,3,3,3,3,3,3,3,3,3,3,3,3,3,3,3,3,3,3,3,3,3,3,3,3,3,4),(342.241768456779,
342.423867884614,342.585794492429,342.743220350869,342.900356607479,343.057324102218,
343.214372211372,343.371468305569,343.528903966539,343.584586896197,343.742012754637,
343.899149011248,344.056116505987,344.21316461514,344.370260709338,344.527696370308,
344.583379299965,344.740805158405,344.897941415016,345.054908909755,345.211957018908,
345.369053113106,345.526488774076,345.582171703733,345.739597562173,345.896733818784,
346.053701313523,346.210749422676,346.367845516874,346.525281177844,346.580964107501,
346.738389965942,346.895526222552,347.052493717291,347.209541826445,347.366637920642,
347.524073581612,347.579756511269,347.735910813974,347.891777852744,348.050071830491,
348.205854264497,348.365404014114,348.524953763731),.UNSPECIFIED.);
#791=B_SPLINE_CURVE_WITH_KNOTS('',3,(#35130,#35131,#35132,#35133,#35134,
#35135,#35136,#35137,#35138,#35139,#35140,#35141),.UNSPECIFIED.,.F.,.F.,
(4,2,1,1,1,1,1,1,4),(348.524953763731,348.578548915037,349.577341318805,
350.576133722573,351.574926126341,352.573718530109,353.572510933877,354.571303337645,
354.808138699911),.UNSPECIFIED.);
#792=B_SPLINE_CURVE_WITH_KNOTS('',3,(#35143,#35144,#35145,#35146,#35147,
#35148,#35149,#35150,#35151,#35152,#35153,#35154,#35155,#35156,#35157,#35158,
#35159,#35160,#35161,#35162,#35163,#35164,#35165,#35166,#35167,#35168,#35169,
#35170,#35171,#35172,#35173,#35174,#35175,#35176,#35177,#35178,#35179,#35180,
#35181,#35182,#35183,#35184,#35185,#35186,#35187,#35188,#35189,#35190,#35191,
#35192,#35193,#35194,#35195,#35196,#35197,#35198,#35199,#35200,#35201,#35202,
#35203,#35204,#35205,#35206,#35207,#35208,#35209,#35210,#35211,#35212,#35213,
#35214,#35215,#35216,#35217,#35218,#35219,#35220,#35221,#35222,#35223,#35224,
#35225,#35226,#35227,#35228,#35229,#35230,#35231,#35232,#35233,#35234,#35235,
#35236,#35237,#35238,#35239,#35240,#35241,#35242,#35243,#35244,#35245,#35246,
#35247,#35248,#35249,#35250,#35251,#35252,#35253,#35254,#35255,#35256,#35257,
#35258,#35259,#35260,#35261,#35262,#35263,#35264,#35265,#35266,#35267,#35268,
#35269,#35270,#35271,#35272,#35273,#35274,#35275),.UNSPECIFIED.,.F.,.F.,
(4,3,3,3,3,3,3,3,3,3,3,3,3,3,3,3,3,3,3,3,3,3,3,3,3,3,3,3,3,3,3,3,3,3,3,
3,3,3,3,3,3,3,3,3,4),(354.808139070911,354.963278088943,355.118405533254,
355.273502210574,355.428953389041,355.570095741413,355.727521599853,355.884657856464,
356.041625351203,356.198673460356,356.355769554553,356.513205215523,356.568888145181,
356.726314003621,356.883450260232,357.040417754971,357.197465864124,357.354561958322,
357.511997619292,357.567680548949,357.725106407389,357.882242664,358.039210158739,
358.196258267892,358.35335436209,358.51079002306,358.566472952717,358.723898811157,
358.881035067768,359.038002562507,359.19505067166,359.352146765858,359.509582426828,
359.565265356485,359.722691214925,359.879827471535,360.036794966274,360.193843075428,
360.350939169625,360.508374830595,360.564057760253,360.727583305717,360.890693796198,
361.053396591264,361.091324378091),.UNSPECIFIED.);
#793=B_SPLINE_CURVE_WITH_KNOTS('',3,(#35277,#35278,#35279,#35280,#35281,
#35282,#35283,#35284,#35285,#35286),.UNSPECIFIED.,.F.,.F.,(4,1,1,1,1,1,
1,4),(361.091326518203,361.562850164021,362.561642567789,363.560434971557,
364.559227375325,365.558019779093,366.556812182861,367.37450968527),
 .UNSPECIFIED.);
#794=B_SPLINE_CURVE_WITH_KNOTS('',3,(#35288,#35289,#35290,#35291,#35292,
#35293,#35294,#35295,#35296,#35297,#35298),.UNSPECIFIED.,.F.,.F.,(4,1,1,
1,1,1,1,1,4),(367.37450968527,367.555604586629,368.554396990397,369.553189394165,
370.551981797933,371.550774201701,372.549566605469,373.548359009237,373.65769499245),
 .UNSPECIFIED.);
#795=B_SPLINE_CURVE_WITH_KNOTS('',3,(#35300,#35301,#35302,#35303,#35304,
#35305,#35306,#35307,#35308,#35309,#35310,#35311,#35312,#35313,#35314,#35315,
#35316,#35317,#35318,#35319,#35320,#35321,#35322,#35323,#35324,#35325,#35326,
#35327,#35328,#35329,#35330,#35331,#35332,#35333,#35334,#35335,#35336,#35337,
#35338,#35339,#35340,#35341,#35342,#35343,#35344,#35345,#35346,#35347,#35348,
#35349,#35350,#35351,#35352,#35353,#35354,#35355,#35356,#35357,#35358,#35359,
#35360,#35361,#35362,#35363,#35364,#35365,#35366,#35367,#35368,#35369,#35370,
#35371,#35372,#35373,#35374,#35375,#35376,#35377,#35378,#35379,#35380,#35381,
#35382,#35383,#35384,#35385,#35386,#35387,#35388,#35389,#35390,#35391,#35392,
#35393,#35394,#35395,#35396,#35397,#35398,#35399,#35400,#35401,#35402,#35403,
#35404,#35405,#35406,#35407,#35408,#35409,#35410,#35411,#35412,#35413,#35414,
#35415,#35416,#35417,#35418,#35419,#35420,#35421,#35422,#35423,#35424,#35425,
#35426,#35427,#35428,#35429,#35430,#35431,#35432),.UNSPECIFIED.,.F.,.F.,
(4,3,3,3,3,3,3,3,3,3,3,3,3,3,3,3,3,3,3,3,3,3,3,3,3,3,3,3,3,3,3,3,3,3,3,
3,3,3,3,3,3,3,3,3,4),(373.65769499245,373.812962610095,373.967981418969,
374.123006149566,374.278018188158,374.43337343482,374.547151413005,374.704577271445,
374.861713528056,375.018681022795,375.175729131948,375.332825226146,375.490260887116,
375.545943816773,375.703369675213,375.860505931824,376.017473426563,376.174521535716,
376.331617629914,376.489053290884,376.544736220541,376.702162078981,376.859298335592,
377.016265830331,377.173313939484,377.330410033682,377.487845694652,377.543528624309,
377.700954482749,377.85809073936,378.015058234099,378.172106343252,378.32920243745,
378.48663809842,378.542321028077,378.699746886517,378.856883143128,379.013850637867,
379.17089874702,379.327994841218,379.485430502188,379.541113431845,379.716064966872,
379.889720377981,379.94088007731),.UNSPECIFIED.);
#796=B_SPLINE_CURVE_WITH_KNOTS('',3,(#35434,#35435,#35436,#35437,#35438,
#35439,#35440,#35441,#35442,#35443),.UNSPECIFIED.,.F.,.F.,(4,1,1,1,1,1,
1,4),(379.940880299629,380.539905835613,381.538698239381,382.537490643149,
383.536283046917,384.535075450685,385.533867854453,386.224065606809),
 .UNSPECIFIED.);
#797=B_SPLINE_CURVE_WITH_KNOTS('',3,(#35445,#35446,#35447,#35448,#35449,
#35450,#35451,#35452,#35453,#35454,#35455,#35456,#35457,#35458,#35459,#35460,
#35461,#35462,#35463,#35464,#35465,#35466,#35467,#35468,#35469,#35470,#35471,
#35472,#35473,#35474,#35475,#35476,#35477,#35478,#35479,#35480,#35481,#35482,
#35483,#35484,#35485,#35486,#35487,#35488,#35489,#35490,#35491,#35492,#35493,
#35494,#35495,#35496,#35497,#35498,#35499,#35500,#35501,#35502,#35503,#35504,
#35505,#35506,#35507,#35508,#35509,#35510,#35511,#35512,#35513,#35514,#35515,
#35516,#35517,#35518,#35519,#35520,#35521,#35522,#35523,#35524,#35525,#35526,
#35527,#35528,#35529,#35530,#35531,#35532,#35533,#35534,#35535,#35536,#35537,
#35538,#35539,#35540,#35541,#35542,#35543,#35544,#35545,#35546,#35547,#35548,
#35549,#35550,#35551,#35552,#35553,#35554,#35555,#35556,#35557,#35558,#35559,
#35560,#35561,#35562,#35563,#35564,#35565,#35566,#35567,#35568,#35569,#35570,
#35571,#35572,#35573,#35574,#35575,#35576,#35577),.UNSPECIFIED.,.F.,.F.,
(4,3,3,3,3,3,3,3,3,3,3,3,3,3,3,3,3,3,3,3,3,3,3,3,3,3,3,3,3,3,3,3,3,3,3,
3,3,3,3,3,3,3,3,3,4),(386.224065804283,386.412697267132,386.532660258221,
386.690086116662,386.847222373273,387.004189868013,387.161237977167,387.318334071365,
387.475769732336,387.531452661989,387.688878520429,387.84601477704,388.002982271779,
388.160030380932,388.317126475129,388.4745621361,388.530245065757,388.687670924197,
388.844807180807,389.001774675546,389.1588227847,389.315918878897,389.473354539867,
389.529037469525,389.686463327965,389.843599584576,390.000567079315,390.157615188469,
390.314711282666,390.472146943636,390.527829873293,390.685255731733,390.842391988344,
390.999359483083,391.156407592236,391.313503686434,391.470939347404,391.526622277061,
391.683559019512,391.840207071128,391.996688881692,392.15325191782,392.30986826289,
392.466816005711,392.507250913988),.UNSPECIFIED.);
#798=B_SPLINE_CURVE_WITH_KNOTS('',3,(#35579,#35580,#35581,#35582,#35583,
#35584,#35585,#35586,#35587,#35588,#35589,#35590),.UNSPECIFIED.,.F.,.F.,
(4,2,1,1,1,1,1,1,4),(392.507250913988,392.525414680829,393.524207084597,
394.522999488365,395.521791892133,396.520584295901,397.51937669967,398.518169103438,
398.790432579651),.UNSPECIFIED.);
#799=B_SPLINE_CURVE_WITH_KNOTS('',3,(#35592,#35593,#35594,#35595,#35596,
#35597,#35598,#35599,#35600,#35601,#35602,#35603,#35604,#35605,#35606,#35607,
#35608,#35609,#35610,#35611,#35612,#35613,#35614,#35615,#35616,#35617,#35618,
#35619,#35620,#35621,#35622,#35623,#35624,#35625,#35626,#35627,#35628,#35629,
#35630,#35631,#35632,#35633,#35634,#35635,#35636,#35637,#35638,#35639,#35640,
#35641,#35642,#35643,#35644,#35645,#35646,#35647,#35648,#35649,#35650,#35651,
#35652,#35653,#35654,#35655,#35656,#35657,#35658,#35659,#35660,#35661,#35662,
#35663,#35664,#35665,#35666,#35667,#35668,#35669,#35670,#35671,#35672,#35673,
#35674,#35675,#35676,#35677,#35678,#35679,#35680,#35681,#35682,#35683,#35684,
#35685,#35686,#35687,#35688,#35689,#35690,#35691,#35692,#35693,#35694,#35695,
#35696,#35697,#35698,#35699,#35700,#35701,#35702,#35703,#35704,#35705,#35706,
#35707,#35708,#35709,#35710,#35711,#35712,#35713,#35714,#35715,#35716,#35717,
#35718,#35719,#35720,#35721,#35722,#35723,#35724),.UNSPECIFIED.,.F.,.F.,
(4,3,3,3,3,3,3,3,3,3,3,3,3,3,3,3,3,3,3,3,3,3,3,3,3,3,3,3,3,3,3,3,3,3,3,
3,3,3,3,3,3,3,3,3,4),(398.790436221168,398.946007945138,399.101608749528,
399.257213317091,399.413167483264,399.516961507206,399.674387365646,399.831523622256,
399.988491116995,400.145539226149,400.302635320346,400.460070981316,400.515753910974,
400.673179769414,400.830316026025,400.987283520764,401.144331629917,401.301427724115,
401.458863385085,401.514546314742,401.671972173182,401.829108429793,401.986075924532,
402.143124033685,402.300220127883,402.457655788853,402.51333871851,402.67076457695,
402.827900833561,402.9848683283,403.141916437453,403.299012531651,403.456448192621,
403.512131122278,403.669556980718,403.826693237329,403.983660732068,404.140708841221,
404.297804935419,404.455240596389,404.510923526046,404.672394501581,404.833497892842,
404.994300774243,405.073621528348),.UNSPECIFIED.);
#800=B_SPLINE_CURVE_WITH_KNOTS('',3,(#35726,#35727,#35728,#35729,#35730,
#35731,#35732,#35733,#35734,#35735),.UNSPECIFIED.,.F.,.F.,(4,1,1,1,1,1,
1,4),(405.073626388949,405.509715929814,406.508508333582,407.50730073735,
408.506093141118,409.504885544886,410.503677948654,411.356799146851),
 .UNSPECIFIED.);
#801=B_SPLINE_CURVE_WITH_KNOTS('',3,(#35737,#35738,#35739,#35740,#35741,
#35742,#35743,#35744,#35745,#35746,#35747,#35748,#35749,#35750,#35751,#35752,
#35753,#35754,#35755,#35756,#35757,#35758,#35759,#35760,#35761,#35762,#35763,
#35764,#35765,#35766,#35767,#35768,#35769,#35770,#35771,#35772,#35773,#35774,
#35775,#35776,#35777,#35778,#35779,#35780,#35781,#35782,#35783,#35784,#35785,
#35786,#35787,#35788,#35789,#35790,#35791,#35792,#35793,#35794,#35795,#35796,
#35797,#35798,#35799,#35800,#35801,#35802,#35803,#35804,#35805,#35806,#35807,
#35808,#35809,#35810,#35811,#35812,#35813,#35814,#35815,#35816,#35817,#35818,
#35819,#35820,#35821,#35822,#35823,#35824,#35825,#35826,#35827,#35828,#35829,
#35830,#35831,#35832,#35833,#35834,#35835,#35836,#35837,#35838,#35839,#35840,
#35841,#35842,#35843,#35844,#35845,#35846,#35847,#35848,#35849,#35850,#35851,
#35852,#35853,#35854,#35855,#35856,#35857,#35858,#35859,#35860,#35861,#35862,
#35863,#35864,#35865,#35866,#35867,#35868,#35869),.UNSPECIFIED.,.F.,.F.,
(4,3,3,3,3,3,3,3,3,3,3,3,3,3,3,3,3,3,3,3,3,3,3,3,3,3,3,3,3,3,3,3,3,3,3,
3,3,3,3,3,3,3,3,3,4),(411.356806835527,411.502470352422,411.659896210861,
411.81703246747,411.973999962208,412.13104807136,412.288144165556,412.445579826525,
412.50126275619,412.658688614631,412.815824871241,412.97279236598,413.129840475134,
413.286936569332,413.444372230302,413.500055159958,413.657481018399,413.814617275009,
413.971584769748,414.128632878902,414.285728973099,414.443164634069,414.498847563726,
414.656273422166,414.813409678776,414.970377173515,415.127425282669,415.284521376866,
415.441957037836,415.497639967494,415.655065825935,415.812202082545,415.969169577284,
416.126217686438,416.283313780635,416.440749441605,416.496432371262,416.653858229702,
416.810994486313,416.967961981052,417.125010090205,417.282106184402,417.439541845373,
417.49522477503,417.639992142707),.UNSPECIFIED.);
#802=B_SPLINE_CURVE_WITH_KNOTS('',3,(#35871,#35872,#35873,#35874,#35875,
#35876,#35877,#35878,#35879,#35880),.UNSPECIFIED.,.F.,.F.,(4,1,1,1,1,1,
1,4),(417.63999988239,418.494017178798,419.492809582566,420.491601986334,
421.490394390102,422.48918679387,423.487979197638,423.923172532797),
 .UNSPECIFIED.);
#803=B_SPLINE_CURVE_WITH_KNOTS('',3,(#35882,#35883,#35884,#35885,#35886,
#35887,#35888,#35889,#35890,#35891,#35892,#35893,#35894,#35895,#35896,#35897,
#35898,#35899,#35900,#35901,#35902,#35903,#35904,#35905,#35906,#35907,#35908,
#35909,#35910,#35911,#35912,#35913,#35914,#35915,#35916,#35917,#35918,#35919,
#35920,#35921,#35922,#35923,#35924,#35925,#35926,#35927,#35928,#35929,#35930,
#35931,#35932,#35933,#35934,#35935,#35936,#35937,#35938,#35939,#35940,#35941,
#35942,#35943,#35944,#35945,#35946,#35947,#35948,#35949,#35950,#35951,#35952,
#35953,#35954,#35955,#35956,#35957,#35958,#35959,#35960,#35961,#35962,#35963,
#35964,#35965,#35966,#35967,#35968,#35969,#35970,#35971,#35972,#35973,#35974,
#35975,#35976,#35977,#35978,#35979,#35980,#35981,#35982,#35983,#35984,#35985,
#35986,#35987,#35988,#35989,#35990,#35991,#35992,#35993,#35994,#35995,#35996,
#35997,#35998,#35999,#36000,#36001,#36002,#36003,#36004,#36005,#36006,#36007,
#36008,#36009,#36010,#36011,#36012,#36013,#36014),.UNSPECIFIED.,.F.,.F.,
(4,3,3,3,3,3,3,3,3,3,3,3,3,3,3,3,3,3,3,3,3,3,3,3,3,3,3,3,3,3,3,3,3,3,3,
3,3,3,3,3,3,3,3,3,4),(423.923177449886,424.08400036725,424.244972248657,
424.406418676567,424.486771601406,424.644197459863,424.80133371649,424.958301211245,
425.115349320415,425.272445414628,425.429881075614,425.485564005174,425.642989863596,
425.800126120187,425.957093614907,426.114141724043,426.271237818222,426.428673479175,
426.484356408942,426.64178226736,426.798918523948,426.955886018664,427.112934127794,
427.270030221968,427.427465882915,427.48314881271,427.640574671267,427.797710927994,
427.95467842285,428.111726532119,428.268822626431,428.426258287513,428.481941216478,
428.639367074758,428.796503331209,428.95347082579,429.110518934789,429.267615028834,
429.425050689657,429.480733620246,429.636725845168,429.792437589937,429.947979823974,
430.103600649651,430.206362757066),.UNSPECIFIED.);
#804=B_SPLINE_CURVE_WITH_KNOTS('',3,(#36016,#36017,#36018,#36019,#36020,
#36021,#36022,#36023,#36024,#36025,#36026),.UNSPECIFIED.,.F.,.F.,(4,1,1,
1,1,1,1,1,4),(430.206366472598,430.479526024014,431.478318427782,432.47711083155,
433.475903235318,434.474695639086,435.473488042854,436.472280446622,436.489548064245),
 .UNSPECIFIED.);
#805=B_SPLINE_CURVE_WITH_KNOTS('',3,(#36028,#36029,#36030,#36031,#36032,
#36033,#36034,#36035,#36036,#36037,#36038,#36039,#36040,#36041,#36042,#36043,
#36044,#36045,#36046,#36047,#36048,#36049,#36050,#36051,#36052,#36053,#36054,
#36055,#36056,#36057,#36058,#36059,#36060,#36061,#36062,#36063,#36064,#36065,
#36066,#36067,#36068,#36069,#36070,#36071,#36072,#36073,#36074,#36075,#36076,
#36077,#36078,#36079,#36080,#36081,#36082,#36083,#36084,#36085,#36086,#36087,
#36088,#36089,#36090,#36091,#36092,#36093,#36094,#36095,#36096,#36097,#36098,
#36099,#36100,#36101,#36102,#36103,#36104,#36105,#36106,#36107,#36108,#36109,
#36110,#36111,#36112,#36113,#36114,#36115,#36116,#36117,#36118,#36119,#36120,
#36121,#36122,#36123,#36124,#36125,#36126,#36127,#36128,#36129,#36130,#36131,
#36132,#36133,#36134,#36135,#36136,#36137,#36138,#36139,#36140,#36141,#36142,
#36143,#36144,#36145,#36146,#36147,#36148,#36149,#36150,#36151,#36152,#36153,
#36154,#36155,#36156,#36157,#36158,#36159,#36160),.UNSPECIFIED.,.F.,.F.,
(4,3,3,3,3,3,3,3,3,3,3,3,3,3,3,3,3,3,3,3,3,3,3,3,3,3,3,3,3,3,3,3,3,3,3,
3,3,3,3,3,3,3,3,3,4),(436.489548064245,436.646504491129,436.803173327651,
436.959676946089,437.11626346617,437.272904027796,437.429877834427,437.47107285039,
437.628498630474,437.785634808864,437.942602225772,438.099650258557,438.256746277134,
438.414181864723,438.469865254158,438.627291146232,438.784427435501,438.941394961838,
439.098443100689,439.255539223524,439.412974911147,439.468657657926,439.626083736926,
439.783220215622,439.940187933218,440.097236263765,440.254332578791,440.411768456417,
440.467450061694,440.624875335439,440.782011007782,440.938977920586,441.096025457905,
441.253120985378,441.410556095686,441.466242465462,441.623668724918,441.780805375985,
441.93777325746,442.094821737711,442.251918194449,442.409354199941,442.46503486923,
442.653850055278,442.772733175584),.UNSPECIFIED.);
#806=B_SPLINE_CURVE_WITH_KNOTS('',3,(#36162,#36163,#36164,#36165,#36166,
#36167,#36168,#36169,#36170,#36171),.UNSPECIFIED.,.F.,.F.,(4,1,1,1,1,1,
1,4),(442.772733371425,443.463827272998,444.462619676766,445.461412080534,
446.460204484302,447.45899688807,448.457789291838,449.055918678604),
 .UNSPECIFIED.);
#807=B_SPLINE_CURVE_WITH_KNOTS('',3,(#36173,#36174,#36175,#36176,#36177,
#36178,#36179,#36180,#36181,#36182,#36183,#36184,#36185,#36186,#36187,#36188,
#36189,#36190,#36191,#36192,#36193,#36194,#36195,#36196,#36197,#36198,#36199,
#36200,#36201,#36202,#36203,#36204,#36205,#36206,#36207,#36208,#36209,#36210,
#36211,#36212,#36213,#36214,#36215,#36216,#36217,#36218,#36219,#36220,#36221,
#36222,#36223,#36224,#36225,#36226,#36227,#36228,#36229,#36230,#36231,#36232,
#36233,#36234,#36235,#36236,#36237,#36238,#36239,#36240,#36241,#36242),
 .UNSPECIFIED.,.F.,.F.,(4,3,3,3,3,3,3,3,3,3,3,3,3,3,3,3,3,3,3,3,3,3,3,4),
(449.055918897709,449.229610385918,449.404629850206,449.456581695606,449.613794725139,
449.770717733325,449.92747225092,450.084310213884,450.241197515991,450.398429524026,
450.455374099374,450.613100063877,450.770534703474,450.927797887324,451.085134321733,
451.242514824289,451.400224845591,451.454166503142,451.6102390889,451.766029595577,
451.921856980043,452.07757171625,452.233633694466,452.389339133442),
 .UNSPECIFIED.);
#808=B_SPLINE_CURVE_WITH_KNOTS('',3,(#36243,#36244,#36245,#36246),
 .UNSPECIFIED.,.F.,.F.,(4,4),(-0.00791586410721434,0.),.UNSPECIFIED.);
#809=B_SPLINE_CURVE_WITH_KNOTS('',3,(#36252,#36253,#36254,#36255,#36256,
#36257,#36258,#36259,#36260,#36261,#36262,#36263,#36264,#36265,#36266,#36267,
#36268,#36269,#36270,#36271,#36272,#36273,#36274,#36275,#36276,#36277,#36278,
#36279,#36280,#36281,#36282,#36283,#36284,#36285,#36286,#36287,#36288,#36289,
#36290,#36291,#36292,#36293,#36294,#36295,#36296,#36297,#36298,#36299,#36300,
#36301,#36302,#36303,#36304,#36305,#36306,#36307,#36308,#36309,#36310,#36311,
#36312,#36313,#36314,#36315,#36316,#36317,#36318,#36319,#36320,#36321,#36322,
#36323,#36324,#36325,#36326,#36327,#36328,#36329,#36330,#36331,#36332,#36333,
#36334,#36335,#36336,#36337,#36338,#36339,#36340,#36341,#36342,#36343,#36344,
#36345,#36346,#36347,#36348,#36349,#36350,#36351,#36352,#36353,#36354,#36355,
#36356,#36357,#36358,#36359,#36360,#36361,#36362,#36363,#36364,#36365,#36366,
#36367,#36368,#36369,#36370,#36371,#36372,#36373,#36374,#36375,#36376,#36377,
#36378,#36379,#36380,#36381,#36382,#36383,#36384,#36385,#36386,#36387,#36388,
#36389,#36390,#36391,#36392,#36393,#36394,#36395,#36396,#36397,#36398,#36399,
#36400,#36401,#36402,#36403,#36404,#36405,#36406,#36407,#36408,#36409,#36410,
#36411,#36412,#36413,#36414,#36415,#36416,#36417,#36418,#36419,#36420,#36421,
#36422,#36423,#36424,#36425,#36426,#36427,#36428,#36429,#36430,#36431,#36432,
#36433,#36434,#36435,#36436,#36437,#36438,#36439,#36440,#36441,#36442,#36443,
#36444,#36445,#36446,#36447,#36448,#36449,#36450,#36451,#36452,#36453,#36454,
#36455,#36456,#36457,#36458,#36459,#36460,#36461,#36462,#36463,#36464,#36465,
#36466,#36467,#36468,#36469,#36470,#36471,#36472,#36473,#36474,#36475,#36476,
#36477,#36478,#36479,#36480,#36481,#36482,#36483,#36484,#36485,#36486,#36487,
#36488,#36489,#36490,#36491,#36492,#36493,#36494,#36495,#36496,#36497,#36498,
#36499,#36500,#36501,#36502,#36503,#36504,#36505,#36506,#36507,#36508,#36509,
#36510,#36511,#36512,#36513,#36514,#36515,#36516,#36517,#36518,#36519,#36520,
#36521,#36522,#36523,#36524,#36525,#36526,#36527,#36528,#36529,#36530,#36531,
#36532,#36533,#36534,#36535,#36536,#36537,#36538,#36539,#36540,#36541,#36542,
#36543,#36544,#36545,#36546,#36547,#36548,#36549,#36550,#36551,#36552,#36553,
#36554,#36555,#36556,#36557,#36558,#36559,#36560,#36561,#36562,#36563,#36564,
#36565,#36566,#36567,#36568,#36569,#36570,#36571,#36572,#36573,#36574,#36575,
#36576,#36577,#36578,#36579,#36580,#36581,#36582,#36583,#36584,#36585,#36586,
#36587,#36588,#36589,#36590,#36591,#36592,#36593,#36594,#36595,#36596,#36597,
#36598,#36599,#36600,#36601,#36602,#36603,#36604,#36605,#36606,#36607,#36608,
#36609,#36610,#36611,#36612,#36613,#36614,#36615,#36616,#36617,#36618,#36619,
#36620,#36621,#36622,#36623,#36624,#36625,#36626,#36627,#36628,#36629,#36630,
#36631,#36632,#36633,#36634,#36635,#36636,#36637,#36638,#36639,#36640,#36641,
#36642,#36643,#36644,#36645,#36646,#36647,#36648,#36649,#36650,#36651,#36652,
#36653,#36654,#36655,#36656,#36657,#36658,#36659,#36660,#36661,#36662,#36663,
#36664,#36665,#36666,#36667,#36668,#36669,#36670,#36671,#36672,#36673,#36674,
#36675,#36676,#36677,#36678,#36679,#36680,#36681,#36682,#36683,#36684,#36685,
#36686,#36687,#36688,#36689,#36690,#36691,#36692,#36693,#36694,#36695,#36696,
#36697,#36698,#36699,#36700,#36701,#36702,#36703,#36704,#36705,#36706,#36707,
#36708,#36709,#36710,#36711,#36712,#36713,#36714,#36715,#36716,#36717,#36718,
#36719,#36720,#36721,#36722,#36723,#36724,#36725,#36726,#36727,#36728,#36729,
#36730,#36731,#36732,#36733,#36734,#36735,#36736,#36737,#36738,#36739,#36740,
#36741,#36742,#36743,#36744,#36745,#36746,#36747,#36748,#36749,#36750,#36751,
#36752,#36753,#36754,#36755,#36756,#36757),.UNSPECIFIED.,.F.,.F.,(4,2,2,
2,2,2,2,2,2,2,2,2,2,2,2,2,2,2,2,2,2,2,2,2,2,2,2,2,2,2,2,2,2,2,2,2,2,2,2,
2,2,2,2,2,2,2,2,2,2,2,2,2,2,2,2,2,2,2,2,2,2,2,2,2,2,2,2,2,2,2,2,2,2,2,2,
2,2,2,2,2,2,2,2,2,2,2,2,2,2,2,2,2,2,2,2,2,2,2,2,2,2,2,2,2,2,2,2,2,2,2,2,
2,2,2,2,2,2,2,2,2,2,2,2,2,2,2,2,2,2,2,2,2,2,2,2,2,2,2,2,2,2,2,2,2,2,2,2,
2,2,2,2,2,2,2,2,2,2,2,2,2,2,2,2,2,2,2,2,2,2,2,2,2,2,2,2,2,2,2,2,2,2,2,2,
2,2,2,2,2,2,2,2,2,2,2,2,2,2,2,2,2,2,2,2,2,2,2,2,2,2,2,2,2,2,2,2,2,2,2,2,
2,2,2,2,2,2,2,2,2,2,2,2,2,2,2,2,2,2,2,2,2,2,2,2,2,2,2,2,2,2,2,2,2,4),(-4.17452195813823,
-4.17439487871219,-4.17304371703842,-4.16751898071022,-4.07124317834127,
-4.02097805912889,-4.01701665778691,-4.01534436649435,-4.01413689822972,
-4.01303804791001,-4.01157109034297,-4.00799980412009,-3.97328510288968,
-3.96118187303754,-3.9582040937554,-3.89038190714491,-3.87738595554472,
-3.85814999858147,-3.85480064281765,-3.85370197759768,-3.85308691584411,
-3.85245796441397,-3.85164581171374,-3.85007115774084,-3.84152283536915,
-3.77306526540815,-3.69755844438976,-3.69408939869832,-3.69250543612561,
-3.69131332219653,-3.69019345986971,-3.68864403344617,-3.68552149338136,
-3.65627889517135,-3.56912341648603,-3.55046426996838,-3.5348819440858,
-3.53192697001401,-3.5308802384808,-3.5302665262556,-3.5296160239285,-3.52876217519765,
-3.52699267942285,-3.51447063710142,-3.4256357067731,-3.37485758225468,
-3.37133073336013,-3.36973597872587,-3.3685421000649,-3.3674252013535,-3.36588714975239,
-3.36198324460933,-3.29990085229795,-3.21557943783811,-3.20968778140487,
-3.20834675534203,-3.20771412400482,-3.2070622900077,-3.20632719290959,
-3.20508990975243,-3.20076038784155,-3.11858442813876,-3.05192537786328,
-3.04847706608442,-3.04689684025256,-3.04570516431406,-3.04458397065106,
-3.04302993385378,-3.03903110229173,-2.9736797987165,-2.92623538023344,
-2.89150516915689,-2.88837953755055,-2.88611908469317,-2.8851899209631,
-2.88457346685516,-2.88390536838238,-2.88295809372591,-2.88070618432958,
-2.846599585726,-2.82902895629226,-2.77999802358922,-2.72939691692005,-2.72587105570796,
-2.72427652294097,-2.72308271924257,-2.72196582464215,-2.72042767521092,
-2.71652297644831,-2.6541488213404,-2.64041511211457,-2.59287158752175,
-2.57370876219136,-2.56462291761118,-2.56310018676764,-2.5622999809912,
-2.56170844946875,-2.56096241590814,-2.55968830753537,-2.55525276888979,
-2.45753641714127,-2.41157754200579,-2.40425448525077,-2.40213215900515,
-2.40082880405687,-2.39964586996712,-2.39812641827048,-2.39499263315095,
-2.37482154214041,-2.36901236391043,-2.29320657331557,-2.26810504573274,
-2.24489949690437,-2.24115118541617,-2.24000487821059,-2.23928736561258,
-2.2386225564605,-2.23775013322241,-2.23627684319443,-2.22724976920248,
-2.12312025780303,-2.08757228391103,-2.08143573950935,-2.07937077994688,
-2.07820909670758,-2.07714875883562,-2.0757300491835,-2.07308560424089,
-2.05858157330693,-2.02958123014083,-1.97997480343435,-1.92993335560801,
-1.9194627325079,-1.91774992846371,-1.91691055448302,-1.91625274508118,
-1.91551208466408,-1.91425954678137,-1.90944716770033,-1.87364533974832,
-1.77763326522993,-1.76032089329098,-1.75736695874268,-1.75586440948753,
-1.75468473501134,-1.75337481351886,-1.75121865243197,-1.74354918289198,
-1.71778119473499,-1.67436127825297,-1.59993326204173,-1.59587681081144,
-1.59464687167504,-1.59398463612504,-1.5933295392782,-1.59252085711016,
-1.59095721723457,-1.58088363471824,-1.55707818709128,-1.46645659202487,
-1.43821329232126,-1.43477389122103,-1.43321229954982,-1.43201914392537,
-1.43074664416405,-1.42876366757775,-1.42266901134504,-1.38863668929722,
-1.29214239504961,-1.28788675215526,-1.28676987080638,-1.27406106364352,
-1.27228294938027,-1.27142652550335,-1.27077572626754,-1.27007213124424,
-1.26894548662688,-1.26539033076042,-1.21319444198684,-1.14094231228655,
-1.13310940677126,-1.11547537849553,-1.11249762009222,-1.11098684629006,
-1.10980260227608,-1.10848954203071,-1.10633262823352,-1.09870476246025,
-1.07304168430524,-1.02985381806037,-0.962252279246089,-0.9516570962742,
-0.949972117162118,-0.949136321961259,-0.948489038628986,-0.947784741284802,
-0.946630355721876,-0.942753838349444,-0.918104484049999,-0.871376559550471,
-0.822886524110304,-0.814246672214374,-0.812483583562317,-0.806669877582027,
-0.791872501432713,-0.789320986427135,-0.787787048264001,-0.786605308780887,
-0.785335469360111,-0.783336799056528,-0.777037574735127,-0.740984582715386,
-0.687841760955233,-0.669496699765245,-0.629806478653441,-0.627297823410744,
-0.62630856066437,-0.625633113403179,-0.624970056093921,-0.624298559150293,
-0.622583053997668,-0.607486838643412,-0.579308217741458,-0.56048587428884,
-0.490617654251995,-0.469131099911989,-0.465927403096475,-0.464405844367376,
-0.463213996302834,-0.461913463564495,-0.459823609433707,-0.452868693162849,
-0.410757858894963,-0.363208647058619,-0.337648196126533,-0.306577047628254,
-0.304350317573486,-0.303399891016416,-0.302721331596898,-0.302028285969172,
-0.301001549021682,-0.298306739488092,-0.240705848798112,-0.177330690865758,
-0.151226259779667,-0.147821601327506,-0.146251722472837,-0.145042059850584,
-0.143741943667973,-0.141694963979227,-0.135236843584198,-0.0982832532670226,
-0.00581586883394552),.UNSPECIFIED.);
#810=B_SPLINE_CURVE_WITH_KNOTS('',3,(#36761,#36762,#36763,#36764,#36765,
#36766,#36767,#36768,#36769,#36770,#36771,#36772,#36773,#36774,#36775,#36776,
#36777,#36778,#36779,#36780,#36781,#36782,#36783,#36784,#36785,#36786,#36787,
#36788,#36789,#36790,#36791,#36792,#36793,#36794,#36795,#36796,#36797,#36798,
#36799,#36800,#36801,#36802,#36803,#36804,#36805,#36806,#36807,#36808,#36809,
#36810,#36811,#36812,#36813,#36814,#36815,#36816,#36817,#36818,#36819,#36820,
#36821,#36822,#36823,#36824,#36825,#36826,#36827,#36828,#36829,#36830,#36831,
#36832,#36833,#36834,#36835,#36836,#36837,#36838,#36839,#36840,#36841,#36842,
#36843,#36844,#36845,#36846,#36847,#36848,#36849,#36850,#36851,#36852,#36853,
#36854,#36855,#36856,#36857,#36858,#36859,#36860),.UNSPECIFIED.,.F.,.F.,
(4,3,3,3,3,3,3,3,3,3,3,3,3,3,3,3,3,3,3,3,3,3,3,3,3,3,3,3,3,3,3,3,3,4),(461.814120077872,
461.996678916982,462.180661142849,462.214783094703,462.380022213048,462.544944361337,
462.712102145621,462.876947800157,463.045261649314,463.213575498471,463.379353738302,
463.544813520999,463.711702116309,463.877070819623,464.044719360931,464.212367902239,
464.378036200707,464.543393437582,464.710335154688,464.8756207972,465.043390551604,
465.211160306007,465.37487731671,465.538278868406,465.706197328749,465.869554386492,
466.039753548133,466.209952709775,466.379993374218,466.54965327262,466.719100095224,
466.888395573125,467.05782179669,467.208745113543),.UNSPECIFIED.);
#811=B_SPLINE_CURVE_WITH_KNOTS('',3,(#36862,#36863,#36864,#36865,#36866,
#36867,#36868,#36869,#36870,#36871,#36872,#36873,#36874,#36875,#36876,#36877,
#36878,#36879,#36880,#36881,#36882,#36883,#36884,#36885,#36886,#36887,#36888,
#36889,#36890,#36891,#36892,#36893,#36894,#36895,#36896,#36897,#36898,#36899,
#36900,#36901,#36902,#36903,#36904,#36905,#36906,#36907,#36908,#36909,#36910,
#36911,#36912,#36913,#36914,#36915,#36916,#36917,#36918,#36919,#36920,#36921,
#36922,#36923,#36924,#36925,#36926,#36927,#36928,#36929,#36930,#36931,#36932,
#36933,#36934,#36935,#36936,#36937,#36938,#36939,#36940,#36941,#36942,#36943,
#36944,#36945,#36946,#36947,#36948,#36949,#36950,#36951,#36952,#36953,#36954,
#36955,#36956,#36957,#36958,#36959,#36960,#36961,#36962,#36963,#36964,#36965,
#36966,#36967,#36968,#36969,#36970,#36971,#36972,#36973,#36974,#36975,#36976,
#36977,#36978,#36979,#36980,#36981,#36982,#36983,#36984,#36985,#36986,#36987,
#36988,#36989,#36990,#36991,#36992,#36993,#36994,#36995,#36996,#36997,#36998,
#36999,#37000,#37001,#37002,#37003,#37004,#37005,#37006,#37007,#37008,#37009,
#37010,#37011,#37012,#37013,#37014,#37015,#37016,#37017,#37018,#37019,#37020,
#37021,#37022,#37023,#37024,#37025,#37026,#37027,#37028,#37029,#37030,#37031,
#37032,#37033,#37034,#37035,#37036,#37037,#37038,#37039,#37040,#37041,#37042,
#37043,#37044,#37045,#37046,#37047,#37048,#37049,#37050,#37051,#37052,#37053,
#37054,#37055,#37056,#37057,#37058,#37059,#37060,#37061,#37062,#37063,#37064,
#37065,#37066,#37067,#37068,#37069,#37070,#37071,#37072,#37073,#37074,#37075,
#37076,#37077,#37078,#37079,#37080,#37081,#37082,#37083,#37084,#37085,#37086,
#37087,#37088,#37089,#37090,#37091,#37092,#37093,#37094,#37095,#37096,#37097,
#37098,#37099,#37100,#37101,#37102,#37103,#37104,#37105,#37106,#37107,#37108,
#37109,#37110,#37111,#37112,#37113,#37114,#37115,#37116,#37117,#37118,#37119,
#37120,#37121,#37122,#37123,#37124,#37125,#37126,#37127,#37128,#37129,#37130,
#37131,#37132,#37133,#37134,#37135,#37136,#37137,#37138,#37139,#37140,#37141,
#37142,#37143,#37144,#37145,#37146,#37147,#37148,#37149,#37150,#37151,#37152,
#37153,#37154,#37155,#37156,#37157,#37158,#37159,#37160,#37161,#37162,#37163,
#37164,#37165,#37166,#37167,#37168,#37169,#37170,#37171,#37172,#37173,#37174,
#37175,#37176,#37177,#37178,#37179,#37180,#37181,#37182,#37183,#37184,#37185,
#37186,#37187,#37188,#37189,#37190,#37191,#37192,#37193,#37194,#37195,#37196,
#37197,#37198,#37199,#37200,#37201,#37202,#37203,#37204,#37205,#37206,#37207,
#37208,#37209,#37210,#37211,#37212,#37213,#37214,#37215,#37216,#37217,#37218,
#37219,#37220,#37221,#37222,#37223,#37224,#37225,#37226,#37227,#37228,#37229,
#37230,#37231,#37232,#37233,#37234,#37235,#37236,#37237,#37238,#37239,#37240,
#37241,#37242,#37243,#37244,#37245,#37246,#37247,#37248,#37249,#37250,#37251,
#37252,#37253,#37254,#37255,#37256,#37257,#37258,#37259,#37260,#37261,#37262,
#37263,#37264,#37265,#37266,#37267,#37268,#37269,#37270,#37271,#37272,#37273,
#37274,#37275,#37276,#37277,#37278,#37279,#37280,#37281,#37282,#37283,#37284,
#37285,#37286,#37287,#37288,#37289,#37290,#37291,#37292,#37293,#37294,#37295,
#37296,#37297,#37298,#37299,#37300,#37301,#37302,#37303,#37304,#37305,#37306,
#37307,#37308,#37309,#37310,#37311,#37312,#37313,#37314,#37315,#37316,#37317,
#37318,#37319,#37320,#37321,#37322,#37323,#37324,#37325,#37326,#37327,#37328,
#37329,#37330,#37331,#37332,#37333,#37334,#37335,#37336,#37337,#37338,#37339,
#37340,#37341,#37342,#37343,#37344,#37345,#37346,#37347,#37348,#37349,#37350,
#37351,#37352,#37353,#37354,#37355,#37356,#37357,#37358,#37359,#37360,#37361,
#37362,#37363,#37364,#37365,#37366,#37367,#37368,#37369,#37370,#37371,#37372,
#37373,#37374,#37375,#37376,#37377,#37378,#37379,#37380,#37381,#37382,#37383,
#37384,#37385,#37386,#37387,#37388,#37389,#37390,#37391,#37392,#37393,#37394,
#37395,#37396,#37397,#37398,#37399,#37400,#37401,#37402,#37403,#37404,#37405,
#37406,#37407),.UNSPECIFIED.,.F.,.F.,(4,2,2,2,2,2,2,2,2,2,2,2,2,2,2,2,2,
2,2,2,2,2,2,2,2,2,2,2,2,2,2,2,2,2,2,2,2,2,2,2,2,2,2,2,2,2,2,2,2,2,2,2,2,
2,2,2,2,2,2,2,2,2,2,2,2,2,2,2,2,2,2,2,2,2,2,2,2,2,2,2,2,2,2,2,2,2,2,2,2,
2,2,2,2,2,2,2,2,2,2,2,2,2,2,2,2,2,2,2,2,2,2,2,2,2,2,2,2,2,2,2,2,2,2,2,2,
2,2,2,2,2,2,2,2,2,2,2,2,2,2,2,2,2,2,2,2,2,2,2,2,2,2,2,2,2,2,2,2,2,2,2,2,
2,2,2,2,2,2,2,2,2,2,2,2,2,2,2,2,2,2,2,2,2,2,2,2,2,2,2,2,2,2,2,2,2,2,2,2,
2,2,2,2,2,2,2,2,2,2,2,2,2,2,2,2,2,2,2,2,2,2,2,2,2,2,2,2,2,2,2,2,2,2,2,2,
2,2,2,2,2,2,2,2,2,2,2,2,2,2,2,2,2,2,2,2,2,2,2,2,2,2,2,2,2,2,2,2,2,2,2,2,
2,2,2,4),(-4.0609209577756,-4.03439321587138,-4.03202807571868,-4.03052003469874,
-4.02935948148285,-4.02822854629725,-4.02710794456281,-4.02556121498386,
-4.0216162442498,-4.01215908496159,-4.00388370548196,-4.00093305540347,
-3.99428904551967,-3.91873599607122,-3.87220276864995,-3.86938848356587,
-3.86835932384938,-3.86766582874838,-3.86699358753679,-3.86618053102651,
-3.8642152986347,-3.84635442487326,-3.83486398267195,-3.74760157037942,
-3.7234393793014,-3.71524001563234,-3.70974579616973,-3.70784583793269,
-3.70674393341832,-3.70556180449928,-3.70404874302576,-3.70094705356752,
-3.68147362314665,-3.61903469940853,-3.61262187825567,-3.60527147043571,
-3.58079108255082,-3.56407050344909,-3.54798380771523,-3.54624993420277,
-3.54540667860522,-3.54481003896041,-3.54417970546147,-3.54310804563247,
-3.54022069661968,-3.53952156374914,-3.48257860387633,-3.43265590626405,
-3.40325216161727,-3.39353828947865,-3.38936163390965,-3.38711944361243,
-3.38519418901268,-3.38394694089309,-3.38275686070036,-3.38120416118785,
-3.37780404584238,-3.3506621669407,-3.34773906234186,-3.26554351356637,
-3.25161369395554,-3.23434213896093,-3.22499747588465,-3.2234650725166,
-3.22266352656457,-3.22207235386216,-3.22142335000057,-3.22026045340737,
-3.21674254182672,-3.15757669428901,-3.10841311809563,-3.07103655670531,
-3.06675776042096,-3.06447505468622,-3.06300280933877,-3.06162833065377,
-3.06047769156413,-3.05910398508388,-3.0567299255297,-3.04765934519056,
-3.04405390035487,-3.04140484031206,-3.03667589549175,-2.94284246935056,
-2.90670832928653,-2.90187060822497,-2.90061455799448,-2.89987241325827,
-2.89921440724647,-2.89837570211009,-2.89672209553241,-2.8869985567319,
-2.78348914037489,-2.74800551641451,-2.74385673988027,-2.74162474667482,
-2.73970543804909,-2.73845927642587,-2.73726706900813,-2.73570746443624,
-2.73227548412224,-2.70421493127265,-2.68405882127573,-2.61733468972596,
-2.58372331487403,-2.58065226290383,-2.5784234476627,-2.57748879271198,
-2.57681643961353,-2.57619983968093,-2.57536179578987,-2.57371799905378,
-2.56069484014506,-2.47137188838082,-2.42649443838459,-2.42173191388313,
-2.41814775891608,-2.41654305129541,-2.4153481323626,-2.41423488022111,
-2.41270905730336,-2.40887383573535,-2.35682755459862,-2.32103693855499,
-2.2852853276149,-2.26020966070372,-2.25628431377604,-2.25511895574868,
-2.25439757655385,-2.25373506052437,-2.25287353623011,-2.25106556977928,
-2.23790071218223,-2.2373472829386,-2.23493750603952,-2.23404679642131,
-2.14624863249812,-2.09906537571398,-2.09550871743851,-2.09390897257151,
-2.09271478742372,-2.09160008133662,-2.09006892886611,-2.0862028946839,
-2.03072694426372,-1.95510369053103,-1.9537167130423,-1.9350259399944,-1.93301371475446,
-1.93220672578147,-1.93153694824017,-1.93084478355361,-1.9298122889228,
-1.92695601908714,-1.90795003050569,-1.87171203057028,-1.79704687752457,
-1.79559057131351,-1.77578747397896,-1.77267171358367,-1.77115635367021,
-1.76997450057847,-1.76867019849177,-1.76654151457586,-1.75915004078413,
-1.71243495772883,-1.61562634520975,-1.6111292899295,-1.60984875534357,
-1.60910147516649,-1.60851036405338,-1.60771254222833,-1.6062002744661,
-1.59733729142129,-1.57840112291465,-1.53177633150656,-1.48324703370828,
-1.45365517357835,-1.45052395126507,-1.44897260408948,-1.44785247230227,
-1.44666111040255,-1.44507991820199,-1.44162400375511,-1.37189982512988,
-1.29991349191457,-1.2892206701147,-1.28749709406024,-1.28665570221722,
-1.28601254744694,-1.28529232581667,-1.28453511863891,-1.28341150400969,
-1.2813973641174,-1.2653768742639,-1.24558351684465,-1.16119822249368,-1.15358879321061,
-1.13056623712461,-1.12763702464534,-1.12613690667462,-1.12503003572176,
-1.12383008227053,-1.12219758857568,-1.11846145279996,-1.11344638931789,
-1.08779003937515,-1.0445925519493,-0.977297545623666,-0.966541711980067,
-0.964815020125381,-0.963973006930939,-0.963330382181621,-0.962610803367827,
-0.961854416453928,-0.960732749519643,-0.958723488056508,-0.942771741214701,
-0.923152353188501,-0.83686818747535,-0.808177203438175,-0.804770117859193,
-0.803332640447792,-0.802131979067573,-0.800898253959374,-0.79909223911427,
-0.794294574676434,-0.734845483977622,-0.647556156406522,-0.643014023176239,
-0.641743547849181,-0.640991097522692,-0.640348640109639,-0.63954966544356,
-0.638681977310649,-0.637294631095284,-0.634595557617483,-0.607894259800219,
-0.558522785536575,-0.524607542742761,-0.522661135807599,-0.507119234441697,
-0.504636140169383,-0.484956702527465,-0.481845869628993,-0.480331171432535,
-0.479149046927936,-0.477843643597691,-0.475711351835398,-0.468289728454649,
-0.421261761948019,-0.3788988760285,-0.334917217031607,-0.321347113347151,
-0.319499460976579,-0.318643031633751,-0.317996770370094,-0.317291566010471,
-0.316556003234873,-0.315484609900675,-0.31360124079712,-0.30950414220205,
-0.223780335750519,-0.163513190743061,-0.159616851340557,-0.158080336353971,
-0.156964049035915,-0.155770351035245,-0.154175025343039,-0.150643605247865,
-0.0987622606105739,-0.057506443010482,-0.000958348145723925),
 .UNSPECIFIED.);
#812=B_SPLINE_CURVE_WITH_KNOTS('',3,(#37409,#37410,#37411,#37412,#37413,
#37414,#37415,#37416,#37417,#37418,#37419,#37420,#37421,#37422,#37423,#37424,
#37425,#37426,#37427,#37428,#37429,#37430,#37431,#37432,#37433,#37434,#37435,
#37436,#37437,#37438,#37439,#37440,#37441,#37442,#37443,#37444,#37445,#37446,
#37447,#37448,#37449,#37450,#37451,#37452,#37453,#37454,#37455,#37456,#37457,
#37458,#37459,#37460,#37461,#37462,#37463,#37464,#37465,#37466,#37467,#37468,
#37469,#37470,#37471,#37472,#37473,#37474,#37475,#37476,#37477,#37478,#37479,
#37480,#37481,#37482,#37483,#37484,#37485,#37486,#37487,#37488,#37489,#37490,
#37491,#37492,#37493,#37494,#37495,#37496,#37497,#37498,#37499,#37500,#37501,
#37502,#37503,#37504,#37505,#37506,#37507,#37508,#37509,#37510,#37511,#37512,
#37513,#37514,#37515,#37516,#37517,#37518,#37519,#37520,#37521,#37522,#37523,
#37524,#37525,#37526),.UNSPECIFIED.,.F.,.F.,(4,3,3,3,3,3,3,3,3,3,3,3,3,
3,3,3,3,3,3,3,3,3,3,3,3,3,3,3,3,3,3,3,3,3,3,3,3,3,3,4),(442.964564156351,
443.171659902652,443.23772742311,443.403190236612,443.568336524023,443.735382349737,
443.900448657001,444.068484241939,444.236519826878,444.401982638167,444.56712892337,
444.734174750189,444.899241055297,445.067276642971,445.235312230646,445.400775043039,
445.565921329316,445.73296715559,445.898033461685,446.06606904805,446.234104634414,
446.399567452715,446.564713744946,446.731759568255,446.896825880289,447.064861459235,
447.232897038182,447.398359840069,447.563506115897,447.73055194741,447.895618243399,
448.063653842675,448.23168944195,448.397152256145,448.562298544091,448.729344369498,
448.894410676911,449.062446261315,449.230481845718,449.24774946334),
 .UNSPECIFIED.);
#813=B_SPLINE_CURVE_WITH_KNOTS('',3,(#37528,#37529,#37530,#37531,#37532,
#37533,#37534,#37535,#37536,#37537,#37538,#37539,#37540,#37541,#37542,#37543,
#37544,#37545,#37546,#37547,#37548,#37549,#37550,#37551,#37552,#37553,#37554,
#37555,#37556,#37557,#37558,#37559,#37560,#37561,#37562,#37563,#37564,#37565,
#37566,#37567,#37568,#37569,#37570,#37571,#37572,#37573,#37574,#37575,#37576,
#37577,#37578,#37579,#37580,#37581,#37582,#37583,#37584,#37585,#37586,#37587,
#37588,#37589,#37590,#37591,#37592,#37593,#37594,#37595,#37596,#37597,#37598,
#37599,#37600,#37601,#37602,#37603,#37604,#37605,#37606,#37607,#37608,#37609,
#37610,#37611,#37612,#37613,#37614,#37615,#37616,#37617,#37618,#37619,#37620,
#37621,#37622,#37623,#37624,#37625,#37626,#37627,#37628,#37629,#37630,#37631,
#37632,#37633,#37634,#37635,#37636,#37637,#37638,#37639,#37640,#37641,#37642,
#37643,#37644,#37645,#37646,#37647,#37648,#37649,#37650,#37651,#37652,#37653,
#37654,#37655,#37656,#37657,#37658,#37659,#37660,#37661,#37662,#37663,#37664,
#37665,#37666,#37667,#37668,#37669,#37670,#37671,#37672,#37673,#37674,#37675,
#37676,#37677,#37678,#37679,#37680,#37681,#37682,#37683,#37684,#37685,#37686,
#37687,#37688,#37689,#37690,#37691,#37692,#37693,#37694,#37695,#37696,#37697,
#37698,#37699,#37700,#37701,#37702,#37703,#37704,#37705,#37706,#37707,#37708,
#37709,#37710,#37711,#37712,#37713,#37714,#37715,#37716,#37717,#37718,#37719,
#37720,#37721,#37722,#37723,#37724,#37725,#37726,#37727,#37728,#37729,#37730,
#37731,#37732,#37733,#37734,#37735,#37736,#37737,#37738,#37739,#37740,#37741,
#37742,#37743,#37744,#37745,#37746,#37747,#37748,#37749,#37750,#37751,#37752,
#37753,#37754,#37755,#37756,#37757,#37758,#37759,#37760,#37761,#37762,#37763,
#37764,#37765,#37766,#37767,#37768,#37769,#37770,#37771,#37772,#37773,#37774,
#37775,#37776,#37777,#37778,#37779,#37780,#37781,#37782,#37783,#37784,#37785,
#37786,#37787,#37788,#37789,#37790,#37791,#37792,#37793,#37794,#37795,#37796,
#37797,#37798,#37799,#37800,#37801,#37802,#37803,#37804,#37805,#37806,#37807,
#37808,#37809,#37810,#37811,#37812,#37813,#37814,#37815,#37816,#37817,#37818,
#37819,#37820,#37821,#37822,#37823,#37824,#37825,#37826,#37827,#37828,#37829,
#37830,#37831,#37832,#37833,#37834,#37835,#37836,#37837,#37838,#37839,#37840,
#37841,#37842,#37843,#37844,#37845,#37846,#37847,#37848,#37849,#37850,#37851,
#37852,#37853,#37854,#37855,#37856,#37857,#37858,#37859,#37860,#37861,#37862,
#37863,#37864,#37865,#37866,#37867,#37868,#37869,#37870,#37871,#37872,#37873,
#37874,#37875,#37876,#37877,#37878,#37879,#37880,#37881,#37882,#37883,#37884,
#37885,#37886,#37887,#37888,#37889,#37890,#37891,#37892,#37893,#37894,#37895,
#37896,#37897,#37898,#37899,#37900,#37901,#37902,#37903,#37904,#37905,#37906,
#37907,#37908,#37909,#37910,#37911,#37912,#37913,#37914,#37915,#37916,#37917,
#37918,#37919,#37920,#37921,#37922,#37923,#37924,#37925,#37926,#37927,#37928,
#37929,#37930,#37931,#37932,#37933,#37934,#37935,#37936,#37937,#37938,#37939,
#37940,#37941,#37942,#37943,#37944,#37945,#37946,#37947,#37948,#37949,#37950,
#37951,#37952,#37953,#37954,#37955,#37956,#37957,#37958,#37959,#37960,#37961,
#37962,#37963,#37964,#37965,#37966,#37967,#37968,#37969,#37970,#37971,#37972,
#37973,#37974,#37975,#37976,#37977,#37978,#37979,#37980,#37981,#37982,#37983,
#37984,#37985,#37986,#37987,#37988,#37989,#37990,#37991,#37992,#37993,#37994,
#37995,#37996,#37997,#37998,#37999,#38000,#38001,#38002,#38003,#38004,#38005,
#38006,#38007,#38008,#38009,#38010,#38011,#38012,#38013,#38014,#38015,#38016,
#38017,#38018,#38019,#38020,#38021,#38022,#38023,#38024,#38025,#38026,#38027,
#38028,#38029,#38030,#38031,#38032,#38033,#38034,#38035,#38036,#38037,#38038,
#38039,#38040,#38041,#38042,#38043,#38044,#38045,#38046,#38047,#38048,#38049,
#38050,#38051,#38052,#38053,#38054,#38055,#38056,#38057),.UNSPECIFIED.,
 .F.,.F.,(4,2,2,2,2,2,2,2,2,2,2,2,2,2,2,2,2,2,2,2,2,2,2,2,2,2,2,2,2,2,2,
2,2,2,2,2,2,2,2,2,2,2,2,2,2,2,2,2,2,2,2,2,2,2,2,2,2,2,2,2,2,2,2,2,2,2,2,
2,2,2,2,2,2,2,2,2,2,2,2,2,2,2,2,2,2,2,2,2,2,2,2,2,2,2,2,2,2,2,2,2,2,2,2,
2,2,2,2,2,2,2,2,2,2,2,2,2,2,2,2,2,2,2,2,2,2,2,2,2,2,2,2,2,2,2,2,2,2,2,2,
2,2,2,2,2,2,2,2,2,2,2,2,2,2,2,2,2,2,2,2,2,2,2,2,2,2,2,2,2,2,2,2,2,2,2,2,
2,2,2,2,2,2,2,2,2,2,2,2,2,2,2,2,2,2,2,2,2,2,2,2,2,2,2,2,2,2,2,2,2,2,2,2,
2,2,2,2,2,2,2,2,2,2,2,2,2,2,2,2,2,2,2,2,2,2,2,2,2,2,2,2,2,2,2,2,2,2,2,2,
2,2,2,2,2,2,2,2,2,2,2,2,2,2,2,2,2,4),(-4.06054070524022,-3.99326051522267,
-3.99084428973821,-3.98931615075845,-3.98815039828341,-3.9869598316091,
-3.98583955478882,-3.98428658768096,-3.98028941894997,-3.91492271730446,
-3.89784305425163,-3.88168222377462,-3.8380713848695,-3.82863919750129,
-3.82709453356329,-3.8262900523961,-3.82563527152188,-3.82497056070661,
-3.82372888627286,-3.81957427593269,-3.74572513344288,-3.71937329977857,
-3.6862450786394,-3.67528013525912,-3.66839009918962,-3.66684849532081,
-3.66567798593909,-3.66448493392157,-3.66336908462542,-3.66183291190795,
-3.65793606789556,-3.59717372685146,-3.54276346777064,-3.51528145248087,
-3.50611532054715,-3.50458209341171,-3.50378001734271,-3.50318868262822,
-3.50253991045274,-3.50137728144466,-3.49785946278574,-3.43882426589436,
-3.40366292571612,-3.36436568411959,-3.34715033410808,-3.34439294550577,
-3.34321876996622,-3.34202373463892,-3.34091099648772,-3.33938684556923,
-3.33556085018345,-3.28432065404834,-3.21647747064557,-3.19358693672542,
-3.18369494262758,-3.18211699045145,-3.18130551124483,-3.18071312094093,
-3.18006904065185,-3.17912903492342,-3.17641828224889,-3.12853473407145,
-3.07577633330864,-3.03068256462879,-3.02590696022578,-3.02234437803812,
-3.02074693341714,-3.01954774819364,-3.01844087030313,-3.01693965210507,
-3.01400506094663,-2.99081508337822,-2.9763909121661,-2.89394559692313,
-2.86478218931693,-2.86051073143986,-2.85929602441597,-2.8585635696021,
-2.85790416305989,-2.85705019405579,-2.85526214381779,-2.84314230454785,
-2.84059228620198,-2.83282051251006,-2.817411616467,-2.74375975325612,-2.70705827826076,
-2.70282637917681,-2.69959266466719,-2.69806013403569,-2.69687168889515,
-2.69574679483467,-2.69417681033429,-2.69007707858343,-2.62117099375599,
-2.57691919067398,-2.55016405954213,-2.53865515159709,-2.5370404052921,
-2.53622126402496,-2.53556546133188,-2.53481137501156,-2.53353312678784,
-2.52891455966321,-2.44162726308138,-2.38043945137047,-2.37701431828801,
-2.37543923089102,-2.37424914701846,-2.37312777059087,-2.37157080257494,
-2.36754980656784,-2.31785008679071,-2.2927495632976,-2.24442945571271,
-2.21920637061212,-2.21526738715837,-2.2141005949072,-2.2133789238333,-2.21271663834819,
-2.21185601493605,-2.21005196114373,-2.19698443919665,-2.19383724275246,
-2.09593000097063,-2.06151341737643,-2.05537760401702,-2.05339089919288,
-2.05211847979351,-2.05092715038737,-2.04937046576136,-2.04675857594624,
-2.03104681987095,-2.00018903714906,-1.89649175050529,-1.89259974624666,
-1.89138933387924,-1.89073085713579,-1.89007530094762,-1.88925972897669,
-1.88766232294627,-1.87666583152726,-1.84848841454193,-1.80430877568617,
-1.76243080427412,-1.73519416476745,-1.73178888311709,-1.7302343950116,
-1.72904317930188,-1.72776935545361,-1.72577729684793,-1.71960036080034,
-1.68480867900998,-1.58511244918773,-1.58466726188599,-1.58400038227583,
-1.57099684002269,-1.56935353426866,-1.56851554481753,-1.56789888880882,
-1.56722640704725,-1.56629139935074,-1.56406090175465,-1.56098713675671,
-1.52732831510471,-1.44443562120157,-1.41263262841465,-1.40909090643026,
-1.40765350960922,-1.40645291839276,-1.40521926831581,-1.40341336871755,
-1.39861604174526,-1.33917040317465,-1.25186972236286,-1.24734225255723,
-1.24607338656308,-1.24532133852643,-1.24467130491806,-1.24386825644434,
-1.2423103831265,-1.24032727550266,-1.22474461305183,-1.20607691229983,
-1.14438025761629,-1.09048239542283,-1.08662903660657,-1.08509983565135,
-1.08398546816295,-1.08279062542378,-1.08118823267201,-1.07761840113263,
-1.02466724597505,-0.941159406369667,-0.938807059458008,-0.936068876591834,
-0.925373720310044,-0.923649920493063,-0.92280843870987,-0.922150272100306,
-0.921425238248575,-0.920293060536237,-0.918900933774189,-0.916189100617598,
-0.889269126479808,-0.842096112473254,-0.768651788895451,-0.764147673727876,
-0.762513352248259,-0.761370684610278,-0.760306743782586,-0.758851318376796,
-0.756031252266613,-0.737463917338268,-0.721333257226002,-0.676176616696737,
-0.627001089408738,-0.622974664504605,-0.603192450440141,-0.601354113354206,
-0.6004672624776,-0.599837660986247,-0.599240023440999,-0.598598800769223,
-0.597195423405945,-0.590329047383933,-0.576735512846013,-0.537794237235253,
-0.466422934081607,-0.444043731308734,-0.441138033208306,-0.439643913526779,
-0.438538502051963,-0.437337258003372,-0.435697867853547,-0.431923422307785,
-0.372418154913922,-0.345927432654378,-0.316207596183532,-0.303440638885575,
-0.301491700462127,-0.29572331895682,-0.292460426386885,-0.280178858544415,
-0.27856171791013,-0.277730409380508,-0.277115405793912,-0.276493627558292,
-0.275834062359139,-0.274954698785619,-0.270835113653864,-0.244989287461306,
-0.225911490542072,-0.159529503985296,-0.146375748866441,-0.140912668496702,
-0.121244625231708,-0.118134463827853,-0.116619957686544,-0.11543792180178,
-0.114132553933041,-0.112000179080363,-0.104576891054096,-0.0575288054657179,
-0.000958222783552507),.UNSPECIFIED.);
#814=B_SPLINE_CURVE_WITH_KNOTS('',3,(#38059,#38060,#38061,#38062,#38063,
#38064,#38065,#38066,#38067,#38068,#38069),.UNSPECIFIED.,.F.,.F.,(4,1,1,
1,1,1,1,1,4),(424.115008234622,424.260671751518,425.259464155286,426.258256559054,
427.257048962822,428.25584136659,429.254633770358,430.253426174126,430.398193541802),
 .UNSPECIFIED.);
#815=B_SPLINE_CURVE_WITH_KNOTS('',3,(#38071,#38072,#38073,#38074,#38075,
#38076,#38077,#38078,#38079,#38080,#38081,#38082,#38083,#38084,#38085,#38086,
#38087,#38088,#38089,#38090,#38091,#38092,#38093,#38094,#38095,#38096,#38097,
#38098,#38099,#38100,#38101,#38102,#38103,#38104,#38105,#38106,#38107,#38108,
#38109,#38110,#38111,#38112,#38113,#38114,#38115,#38116,#38117,#38118,#38119,
#38120,#38121,#38122,#38123,#38124,#38125,#38126,#38127,#38128,#38129,#38130,
#38131,#38132,#38133,#38134,#38135,#38136,#38137,#38138,#38139,#38140,#38141,
#38142,#38143,#38144,#38145,#38146,#38147,#38148,#38149,#38150,#38151,#38152,
#38153,#38154,#38155,#38156,#38157,#38158,#38159,#38160,#38161,#38162,#38163,
#38164,#38165,#38166,#38167,#38168,#38169,#38170,#38171,#38172,#38173,#38174,
#38175,#38176,#38177,#38178,#38179,#38180,#38181,#38182,#38183,#38184,#38185,
#38186,#38187,#38188,#38189,#38190,#38191,#38192,#38193,#38194,#38195,#38196,
#38197,#38198,#38199,#38200,#38201,#38202,#38203,#38204,#38205,#38206,#38207,
#38208,#38209,#38210,#38211,#38212,#38213,#38214,#38215,#38216,#38217,#38218,
#38219,#38220,#38221,#38222,#38223,#38224,#38225,#38226,#38227,#38228,#38229,
#38230,#38231,#38232,#38233,#38234,#38235,#38236,#38237,#38238,#38239,#38240,
#38241,#38242,#38243,#38244,#38245,#38246,#38247,#38248,#38249,#38250,#38251,
#38252,#38253,#38254,#38255,#38256,#38257,#38258,#38259,#38260,#38261,#38262,
#38263,#38264,#38265,#38266,#38267,#38268,#38269,#38270,#38271,#38272,#38273,
#38274,#38275,#38276,#38277,#38278,#38279,#38280,#38281,#38282,#38283,#38284,
#38285,#38286,#38287,#38288,#38289,#38290,#38291,#38292,#38293,#38294,#38295,
#38296,#38297,#38298,#38299,#38300,#38301,#38302,#38303,#38304,#38305,#38306,
#38307,#38308,#38309,#38310,#38311,#38312,#38313,#38314,#38315,#38316,#38317,
#38318,#38319,#38320,#38321,#38322,#38323,#38324,#38325,#38326,#38327,#38328,
#38329,#38330,#38331,#38332,#38333,#38334,#38335,#38336,#38337,#38338,#38339,
#38340,#38341,#38342,#38343,#38344,#38345,#38346,#38347,#38348,#38349,#38350,
#38351,#38352,#38353,#38354,#38355,#38356,#38357,#38358,#38359,#38360,#38361,
#38362,#38363,#38364,#38365,#38366,#38367,#38368,#38369,#38370,#38371,#38372,
#38373,#38374,#38375,#38376,#38377,#38378,#38379,#38380,#38381,#38382,#38383,
#38384,#38385,#38386,#38387,#38388,#38389,#38390,#38391,#38392,#38393,#38394,
#38395,#38396,#38397,#38398,#38399,#38400,#38401,#38402,#38403,#38404,#38405,
#38406,#38407,#38408,#38409,#38410,#38411,#38412,#38413,#38414,#38415,#38416,
#38417,#38418,#38419,#38420,#38421,#38422,#38423,#38424,#38425,#38426,#38427,
#38428,#38429,#38430,#38431,#38432,#38433,#38434,#38435,#38436,#38437,#38438,
#38439,#38440,#38441,#38442,#38443,#38444,#38445,#38446,#38447,#38448,#38449,
#38450,#38451,#38452,#38453,#38454,#38455,#38456,#38457,#38458,#38459,#38460,
#38461,#38462,#38463,#38464,#38465,#38466,#38467,#38468,#38469,#38470,#38471,
#38472,#38473,#38474,#38475,#38476,#38477,#38478,#38479,#38480,#38481,#38482,
#38483,#38484,#38485,#38486,#38487,#38488,#38489,#38490,#38491,#38492,#38493,
#38494,#38495,#38496,#38497,#38498,#38499,#38500,#38501,#38502,#38503,#38504,
#38505,#38506,#38507,#38508,#38509,#38510,#38511,#38512,#38513,#38514,#38515,
#38516,#38517,#38518,#38519,#38520,#38521,#38522,#38523,#38524,#38525,#38526,
#38527,#38528,#38529,#38530,#38531,#38532,#38533,#38534,#38535,#38536,#38537,
#38538,#38539,#38540,#38541,#38542,#38543,#38544,#38545,#38546,#38547,#38548,
#38549,#38550,#38551,#38552,#38553,#38554,#38555,#38556,#38557,#38558,#38559,
#38560,#38561,#38562,#38563,#38564,#38565,#38566,#38567,#38568,#38569,#38570,
#38571,#38572,#38573,#38574,#38575,#38576,#38577,#38578,#38579,#38580,#38581,
#38582,#38583,#38584,#38585,#38586,#38587,#38588,#38589,#38590,#38591,#38592,
#38593,#38594,#38595,#38596,#38597,#38598,#38599,#38600,#38601,#38602,#38603,
#38604),.UNSPECIFIED.,.F.,.F.,(4,2,2,2,2,2,2,2,2,2,2,2,2,2,2,2,2,2,2,2,
2,2,2,2,2,2,2,2,2,2,2,2,2,2,2,2,2,2,2,2,2,2,2,2,2,2,2,2,2,2,2,2,2,2,2,2,
2,2,2,2,2,2,2,2,2,2,2,2,2,2,2,2,2,2,2,2,2,2,2,2,2,2,2,2,2,2,2,2,2,2,2,2,
2,2,2,2,2,2,2,2,2,2,2,2,2,2,2,2,2,2,2,2,2,2,2,2,2,2,2,2,2,2,2,2,2,2,2,2,
2,2,2,2,2,2,2,2,2,2,2,2,2,2,2,2,2,2,2,2,2,2,2,2,2,2,2,2,2,2,2,2,2,2,2,2,
2,2,2,2,2,2,2,2,2,2,2,2,2,2,2,2,2,2,2,2,2,2,2,2,2,2,2,2,2,2,2,2,2,2,2,2,
2,2,2,2,2,2,2,2,2,2,2,2,2,2,2,2,2,2,2,2,2,2,2,2,2,2,2,2,2,2,2,2,2,2,2,2,
2,2,2,2,2,2,2,2,2,2,2,2,2,2,2,2,2,2,2,2,2,2,2,2,2,2,2,2,2,2,4),(-4.06128115076983,
-4.00337659414285,-3.95352302031363,-3.94957161734353,-3.94790154736699,
-3.94669494696125,-3.9455963828194,-3.94412906224133,-3.94055326902321,
-3.90559299010059,-3.8368217081903,-3.81768545738403,-3.79159930410022,
-3.78755815697234,-3.78668393196703,-3.78602630358188,-3.78540356010347,
-3.78478696598889,-3.78394907758219,-3.78230602442402,-3.76930673038337,
-3.76863966891963,-3.76819168911594,-3.75999889310883,-3.74441486304274,
-3.70533616580739,-3.66160033400585,-3.63578804248566,-3.6307197329802,
-3.62695177247449,-3.62531371958506,-3.62411288752704,-3.6230074560461,
-3.62151270429965,-3.6186039949592,-3.59613200008761,-3.52500687123347,
-3.48608234689981,-3.47507879755007,-3.46882499231493,-3.4662541052831,
-3.4643704359761,-3.46348018927821,-3.46281245739004,-3.46218948636098,
-3.46132714418981,-3.45912151703814,-3.42855538280345,-3.35907064735365,
-3.30773731462055,-3.30420911024686,-3.30261452431006,-3.30142109014958,
-3.30030483839994,-3.2987680409429,-3.29486923924047,-3.23392552169708,
-3.14880966393129,-3.14473376851407,-3.14196324095807,-3.14094514444701,
-3.14033173564655,-3.13966607051309,-3.13878578942747,-3.13680953610409,
-3.11941123736714,-3.03329993736812,-2.98501206607016,-2.98144836068129,
-2.97984716754302,-2.97865259497721,-2.97753802799056,-2.97600784860362,
-2.9721483542671,-2.91753651599664,-2.86807179042429,-2.8220572752161,-2.82017292792062,
-2.81867839614772,-2.81788893339083,-2.81729702038061,-2.81664971294239,
-2.81549516423628,-2.81204450935921,-2.75356883955704,-2.70437714124751,
-2.66271084634879,-2.65893443580827,-2.65729481503383,-2.65609364060156,
-2.65498845929144,-2.65349490229749,-2.6505910268777,-2.62825383294246,
-2.61606463596482,-2.53348155342824,-2.49863139135094,-2.49639056203132,
-2.49545374118098,-2.49478087569752,-2.49416453650912,-2.49332793739305,
-2.4916902107832,-2.47884728178292,-2.47806462670788,-2.47769236150409,
-2.47504493173271,-2.39790274120544,-2.36139330307826,-2.33875490108667,
-2.33580258184672,-2.33431993345178,-2.33325240956193,-2.33212112374322,
-2.33052823529818,-2.32628713884829,-2.25466613807874,-2.2093451006254,
-2.18508298235749,-2.17492628945015,-2.17335939963952,-2.1725500318806,
-2.17189469691472,-2.17123236148917,-2.17000344137782,-2.16596020381263,
-2.09676533278558,-2.05116792033457,-2.03140263621282,-2.01598204196407,
-2.01338474614578,-2.01183193430983,-2.0106407342294,-2.00936568881703,
-2.00736914768313,-2.00115816462975,-1.96606095971846,-1.86481930244715,
-1.85250218388215,-1.85088350930598,-1.85005173062519,-1.84943653542393,
-1.84876241531573,-1.84781942465291,-1.84554278641683,-1.80695006036606,
-1.71343611487381,-1.6934499114707,-1.69032494587288,-1.68880742949498,
-1.687624944379,-1.68632101109549,-1.68419533076884,-1.67683751282148,-1.63049373803252,
-1.57868466808116,-1.53109496508983,-1.52838549505615,-1.52744538764341,
-1.52680107799704,-1.52620834710958,-1.52539620912519,-1.52381631789719,
-1.51332027859801,-1.48741257196877,-1.37919231130839,-1.37721715169979,
-1.36919970601454,-1.36693359164968,-1.36558531054388,-1.36441002992956,
-1.36299285283188,-1.36032092503336,-1.35697180176389,-1.33244220570106,
-1.30905353004349,-1.23891413147441,-1.20758216523041,-1.20536578365824,
-1.20450157852215,-1.20387808014675,-1.20321059344723,-1.20230376136192,
-1.20032258346949,-1.17594256282558,-1.15235604387838,-1.07786204735764,
-1.04849551262255,-1.04537029860268,-1.04382044329179,-1.04270069403241,
-1.04150909383619,-1.03995816966256,-1.0366441828275,-1.03227559272862,
-0.993545917142618,-0.936759736440181,-0.900595964710359,-0.897359591211616,
-0.884318026493944,-0.882514669170517,-0.88165400466934,-0.880991517306588,
-0.880269449090748,-0.879101641326377,-0.875479742595385,-0.855345527380135,
-0.833722679499318,-0.77513345553407,-0.759604049652812,-0.749048769023668,
-0.743696504220069,-0.742457047935872,-0.741444596131449,-0.725098798543921,
-0.722452903789449,-0.720885835671027,-0.719692308580539,-0.718423090326915,
-0.716492130495393,-0.710770547526889,-0.702131962488849,-0.676242052192464,
-0.629271359365302,-0.573991840740875,-0.561699969203501,-0.5600825111822,
-0.559251144753252,-0.55863614999014,-0.557962140697752,-0.557019112314918,
-0.555965932379833,-0.547989704585828,-0.519751055138522,-0.465130511749062,
-0.404051412908648,-0.400151822098393,-0.398614797756203,-0.39749841033699,
-0.396304858474342,-0.395133871924719,-0.393591707124422,-0.386700638707445,
-0.375734121714229,-0.342562064166752,-0.315967694274086,-0.242234264453372,
-0.238109900227528,-0.236871385224489,-0.236207106160641,-0.235551937691001,
-0.234745804418132,-0.233194404707153,-0.223614723738133,-0.18027538427235,
-0.164193136826247,-0.147201617351755,-0.134960680961682,-0.0813583254433141,
-0.0775075171895236,-0.0759787046126711,-0.0748644000197485,-0.0736694170058863,
-0.0724958425958789,-0.0709465811315708,-0.0684807738006665,-0.000956977264331218),
 .UNSPECIFIED.);
#816=B_SPLINE_CURVE_WITH_KNOTS('',3,(#38606,#38607,#38608,#38609,#38610,
#38611,#38612,#38613,#38614,#38615,#38616,#38617,#38618,#38619,#38620,#38621,
#38622,#38623,#38624,#38625,#38626,#38627,#38628,#38629,#38630,#38631,#38632,
#38633,#38634,#38635,#38636,#38637,#38638,#38639,#38640,#38641,#38642,#38643,
#38644,#38645,#38646,#38647,#38648,#38649,#38650,#38651,#38652,#38653,#38654,
#38655,#38656,#38657,#38658,#38659,#38660,#38661,#38662,#38663,#38664,#38665,
#38666,#38667,#38668,#38669,#38670,#38671,#38672,#38673,#38674,#38675,#38676,
#38677,#38678,#38679,#38680,#38681,#38682,#38683,#38684,#38685,#38686,#38687,
#38688,#38689,#38690,#38691,#38692,#38693,#38694,#38695,#38696,#38697,#38698,
#38699,#38700,#38701,#38702,#38703,#38704,#38705,#38706,#38707,#38708,#38709,
#38710,#38711,#38712,#38713,#38714,#38715,#38716,#38717,#38718,#38719,#38720,
#38721,#38722,#38723,#38724,#38725,#38726,#38727,#38728,#38729,#38730,#38731,
#38732,#38733,#38734,#38735,#38736,#38737,#38738,#38739,#38740,#38741,#38742,
#38743,#38744,#38745,#38746,#38747,#38748,#38749,#38750,#38751,#38752,#38753,
#38754,#38755,#38756,#38757,#38758,#38759,#38760,#38761,#38762,#38763,#38764,
#38765,#38766,#38767,#38768,#38769,#38770,#38771,#38772,#38773,#38774,#38775,
#38776,#38777,#38778,#38779,#38780,#38781,#38782,#38783,#38784,#38785,#38786,
#38787,#38788,#38789,#38790,#38791,#38792,#38793,#38794,#38795,#38796,#38797,
#38798,#38799,#38800,#38801,#38802,#38803,#38804,#38805,#38806,#38807,#38808,
#38809,#38810,#38811,#38812,#38813,#38814,#38815,#38816,#38817,#38818,#38819,
#38820,#38821,#38822,#38823,#38824,#38825,#38826,#38827,#38828,#38829,#38830,
#38831,#38832,#38833,#38834,#38835,#38836,#38837,#38838,#38839,#38840,#38841,
#38842,#38843,#38844,#38845,#38846,#38847,#38848,#38849,#38850,#38851,#38852,
#38853,#38854,#38855,#38856,#38857,#38858,#38859,#38860,#38861,#38862,#38863,
#38864,#38865,#38866,#38867,#38868,#38869,#38870,#38871,#38872,#38873,#38874,
#38875,#38876,#38877,#38878,#38879,#38880,#38881,#38882,#38883,#38884,#38885,
#38886,#38887,#38888,#38889,#38890,#38891,#38892,#38893,#38894,#38895,#38896,
#38897,#38898,#38899,#38900,#38901,#38902,#38903,#38904,#38905,#38906,#38907,
#38908,#38909,#38910,#38911,#38912,#38913,#38914,#38915,#38916,#38917,#38918,
#38919,#38920,#38921,#38922,#38923,#38924,#38925,#38926,#38927,#38928,#38929,
#38930,#38931,#38932,#38933,#38934,#38935,#38936,#38937,#38938,#38939,#38940,
#38941,#38942,#38943,#38944,#38945,#38946,#38947,#38948,#38949,#38950,#38951,
#38952,#38953,#38954,#38955,#38956,#38957,#38958,#38959,#38960,#38961,#38962,
#38963,#38964,#38965,#38966,#38967,#38968,#38969,#38970,#38971,#38972,#38973,
#38974,#38975,#38976,#38977,#38978,#38979,#38980,#38981,#38982,#38983,#38984,
#38985,#38986,#38987,#38988,#38989,#38990,#38991,#38992,#38993,#38994,#38995,
#38996,#38997,#38998,#38999,#39000,#39001,#39002,#39003,#39004,#39005,#39006,
#39007,#39008,#39009,#39010,#39011,#39012,#39013,#39014,#39015,#39016,#39017,
#39018,#39019,#39020,#39021,#39022,#39023,#39024,#39025,#39026,#39027,#39028,
#39029,#39030,#39031,#39032,#39033,#39034,#39035,#39036,#39037,#39038,#39039,
#39040,#39041,#39042,#39043,#39044,#39045,#39046,#39047,#39048,#39049,#39050,
#39051,#39052,#39053,#39054,#39055,#39056,#39057,#39058,#39059,#39060,#39061,
#39062,#39063,#39064,#39065,#39066,#39067,#39068,#39069,#39070,#39071,#39072,
#39073,#39074,#39075,#39076,#39077,#39078,#39079,#39080,#39081,#39082,#39083,
#39084,#39085,#39086,#39087,#39088,#39089,#39090,#39091,#39092,#39093,#39094,
#39095,#39096,#39097,#39098,#39099,#39100,#39101,#39102,#39103,#39104,#39105,
#39106,#39107,#39108,#39109,#39110,#39111,#39112,#39113,#39114,#39115,#39116,
#39117,#39118,#39119,#39120,#39121,#39122,#39123,#39124,#39125,#39126,#39127,
#39128,#39129,#39130,#39131,#39132,#39133,#39134,#39135,#39136,#39137,#39138,
#39139,#39140,#39141,#39142,#39143,#39144,#39145,#39146,#39147,#39148,#39149,
#39150,#39151,#39152,#39153,#39154,#39155,#39156,#39157,#39158,#39159),
 .UNSPECIFIED.,.F.,.F.,(4,2,2,2,2,2,2,2,2,2,2,2,2,2,2,2,2,2,2,2,2,2,2,2,
2,2,2,2,2,2,2,2,2,2,2,2,2,2,2,2,2,2,2,2,2,2,2,2,2,2,2,2,2,2,2,2,2,2,2,2,
2,2,2,2,2,2,2,2,2,2,2,2,2,2,2,2,2,2,2,2,2,2,2,2,2,2,2,2,2,2,2,2,2,2,2,2,
2,2,2,2,2,2,2,2,2,2,2,2,2,2,2,2,2,2,2,2,2,2,2,2,2,2,2,2,2,2,2,2,2,2,2,2,
2,2,2,2,2,2,2,2,2,2,2,2,2,2,2,2,2,2,2,2,2,2,2,2,2,2,2,2,2,2,2,2,2,2,2,2,
2,2,2,2,2,2,2,2,2,2,2,2,2,2,2,2,2,2,2,2,2,2,2,2,2,2,2,2,2,2,2,2,2,2,2,2,
2,2,2,2,2,2,2,2,2,2,2,2,2,2,2,2,2,2,2,2,2,2,2,2,2,2,2,2,2,2,2,2,2,2,2,2,
2,2,2,2,2,2,2,2,2,2,2,2,2,2,2,2,2,2,2,2,2,2,2,2,2,2,2,2,2,2,2,2,2,2,2,2,
4),(-4.05985743828913,-3.98106395518661,-3.97680103017906,-3.97486204276291,
-3.97332002043937,-3.97251595153039,-3.9718610068192,-3.97119569804348,
-3.96995167127704,-3.9657787694658,-3.88585078515522,-3.86156563159282,
-3.82145877603785,-3.81454745049971,-3.81300456299151,-3.81183342341244,
-3.81063987760159,-3.80952398859958,-3.80798842330925,-3.80409660868656,
-3.74463547220707,-3.71789674876764,-3.69343816938377,-3.6637093792152,
-3.65616423834442,-3.65171328125454,-3.65048402520685,-3.64974826673558,
-3.64908951364081,-3.64824133078364,-3.64648296426891,-3.63504026937692,
-3.63169376695359,-3.57314380418947,-3.53617855770479,-3.50740527140734,
-3.49303723778487,-3.49049128560377,-3.48931798295473,-3.48812328122201,
-3.48700928408048,-3.48548096369386,-3.48163176439891,-3.42811659408292,
-3.37055317819946,-3.34110133333759,-3.32983839807071,-3.32822471360337,
-3.32740572167076,-3.32681231171474,-3.32617151466645,-3.32504913309249,
-3.3218238451119,-3.2668501478598,-3.22121042548354,-3.19142570765562,-3.17175828935828,
-3.16840941546383,-3.16681013853851,-3.16561041803425,-3.16450363120402,
-3.16300342809437,-3.16007345325645,-3.13702141581217,-3.12169001243361,
-3.12059699685356,-3.05160505551728,-3.01851110288221,-3.00906417778853,
-3.00622573654037,-3.00518367675347,-3.00448942659501,-3.00382110778999,
-3.00301977642636,-3.00104176527535,-2.9835754275094,-2.98258362100267,
-2.96169349755182,-2.90110354445804,-2.8543562195395,-2.84698763269912,
-2.84486545126362,-2.84355282047403,-2.84237259512579,-2.84087192920865,
-2.83792982668611,-2.82086845005743,-2.72774275613119,-2.69977444870512,
-2.68481544954595,-2.68306703983701,-2.68222073105265,-2.68162336705582,
-2.68099335091522,-2.68010482418368,-2.67825944683945,-2.65817256352403,
-2.57653368260059,-2.53141716864186,-2.52663953363931,-2.52304606603765,
-2.52143941812909,-2.52024394585335,-2.51913081867179,-2.51760616259377,
-2.51377904289108,-2.46261765454206,-2.41120234152801,-2.38668470816203,
-2.36471386623158,-2.36108729843683,-2.35995542605194,-2.35924140515383,
-2.35857605299654,-2.35769737667367,-2.35572968591057,-2.3386122673445,
-2.30475007271722,-2.27176024030886,-2.20383193979933,-2.20038124661493,
-2.19880105498407,-2.19760987191412,-2.19648948516118,-2.19493711269822,
-2.1918017124163,-2.16204976718353,-2.15533292734962,-2.15275649463431,
-2.07765511115172,-2.05105530133829,-2.03933454567053,-2.03771254873463,
-2.03689177143429,-2.03624166189933,-2.0355873184034,-2.03439792951514,
-2.0306758647374,-2.00696098453929,-1.98169586986702,-1.90736841965064,
-1.90030844786412,-1.88066125606198,-1.87755227542641,-1.87603809151406,
-1.87485619231357,-1.8735508584449,-1.87141827480954,-1.86399168064906,
-1.81690468959429,-1.73053643092043,-1.7296787087585,-1.7169314927229,-1.71529718085327,
-1.71446144291625,-1.71384530708451,-1.71317221686676,-1.71223429750922,
-1.70998713566387,-1.70688451499964,-1.67263436164602,-1.59667365656093,
-1.58012220228514,-1.57730250298544,-1.5579116062293,-1.55481437597069,
-1.55330244804808,-1.55212073037944,-1.55081398492712,-1.54867544280821,
-1.54119225270003,-1.49349391160159,-1.41226623373603,-1.41137044057747,
-1.40810797810299,-1.40771070033884,-1.40654210682658,-1.39418190137152,
-1.39256172677024,-1.39172959774865,-1.39111434957101,-1.39044038598459,
-1.38949799400813,-1.38722461899358,-1.3508423790782,-1.25468698857249,
-1.23510004256043,-1.23199369686486,-1.23047997103966,-1.22929805428327,
-1.22801882442329,-1.22601249914877,-1.22361457160696,-1.21903537545228,
-1.17708311059049,-1.11623759507788,-1.07280239378291,-1.07007881361724,
-1.06913670367478,-1.06849186704026,-1.06789932858539,-1.06708846882598,
-1.06551450329995,-1.05517373512465,-1.02999223416893,-0.942734046483729,
-0.912974669409553,-0.909838954291059,-0.908286468547347,-0.907166022319952,
-0.905974796722467,-0.904426378215918,-0.901116681102006,-0.896759600139733,
-0.886479685882287,-0.877946982304953,-0.8477495815758,-0.805027311266354,
-0.764761127191685,-0.764375447447097,-0.761909822788837,-0.748807362816994,
-0.747001668251853,-0.746140539198567,-0.745477990564899,-0.744756162913993,
-0.743589392958526,-0.739652996946715,-0.714468018027886,-0.634921719703111,
-0.617202650393045,-0.590239216616583,-0.587181911668168,-0.585649195014072,
-0.584533991959473,-0.583339878398973,-0.582167749984219,-0.579618215288261,
-0.565297903938635,-0.53661582355207,-0.504538023011802,-0.429480439559194,
-0.425194615601626,-0.423937544995388,-0.423269560418945,-0.422620992515017,
-0.421823837010682,-0.420314780187632,-0.411522214186124,-0.392719808588656,
-0.355169878331043,-0.317400746147991,-0.306945402869458,-0.306369479989895,
-0.299572074835488,-0.290155004601213,-0.267426832381596,-0.264508421846414,
-0.263011075402667,-0.261904898166456,-0.26070439083222,-0.259520738794475,
-0.257943610873731,-0.250507995535723,-0.218273638583761,-0.196668849510435,
-0.116468794268212,-0.103532088314514,-0.101890955606238,-0.101053461440696,
-0.100436872281089,-0.0997641562184845,-0.0988282840761091,-0.0965932001016937,
-0.0935115890801095,-0.0596963921842725,-0.000958062901417849),
 .UNSPECIFIED.);
#817=B_SPLINE_CURVE_WITH_KNOTS('',3,(#39161,#39162,#39163,#39164,#39165,
#39166,#39167,#39168,#39169,#39170,#39171,#39172,#39173,#39174,#39175,#39176,
#39177,#39178,#39179,#39180,#39181,#39182,#39183,#39184,#39185,#39186,#39187,
#39188,#39189,#39190,#39191,#39192,#39193,#39194,#39195,#39196,#39197,#39198,
#39199,#39200,#39201,#39202,#39203,#39204,#39205,#39206,#39207,#39208,#39209,
#39210,#39211,#39212,#39213,#39214,#39215,#39216,#39217,#39218,#39219,#39220,
#39221,#39222,#39223,#39224,#39225,#39226,#39227,#39228,#39229,#39230,#39231,
#39232,#39233,#39234,#39235,#39236,#39237,#39238,#39239,#39240,#39241,#39242,
#39243,#39244,#39245,#39246,#39247,#39248,#39249,#39250,#39251,#39252,#39253,
#39254,#39255,#39256,#39257,#39258,#39259,#39260,#39261,#39262,#39263,#39264,
#39265,#39266,#39267,#39268,#39269,#39270,#39271,#39272,#39273,#39274,#39275,
#39276,#39277,#39278,#39279,#39280,#39281,#39282,#39283,#39284,#39285,#39286,
#39287,#39288,#39289,#39290,#39291,#39292,#39293,#39294,#39295,#39296,#39297,
#39298,#39299,#39300,#39301,#39302,#39303,#39304,#39305,#39306,#39307,#39308,
#39309,#39310,#39311,#39312,#39313,#39314,#39315,#39316,#39317,#39318,#39319,
#39320,#39321,#39322,#39323,#39324,#39325,#39326,#39327,#39328,#39329,#39330,
#39331,#39332,#39333,#39334,#39335,#39336,#39337,#39338,#39339,#39340,#39341,
#39342,#39343,#39344,#39345,#39346,#39347,#39348,#39349,#39350,#39351,#39352,
#39353,#39354,#39355,#39356,#39357,#39358,#39359,#39360,#39361,#39362,#39363,
#39364,#39365,#39366,#39367,#39368,#39369,#39370,#39371,#39372,#39373,#39374,
#39375,#39376,#39377,#39378,#39379,#39380,#39381,#39382,#39383,#39384,#39385,
#39386,#39387,#39388,#39389,#39390,#39391,#39392,#39393,#39394,#39395,#39396,
#39397,#39398,#39399,#39400,#39401,#39402,#39403,#39404,#39405,#39406,#39407,
#39408,#39409,#39410,#39411,#39412,#39413,#39414,#39415,#39416,#39417,#39418,
#39419,#39420,#39421,#39422,#39423,#39424,#39425,#39426,#39427,#39428,#39429,
#39430,#39431,#39432,#39433,#39434,#39435,#39436,#39437,#39438,#39439,#39440,
#39441,#39442,#39443,#39444,#39445,#39446,#39447,#39448,#39449,#39450,#39451,
#39452,#39453,#39454,#39455,#39456,#39457,#39458,#39459,#39460,#39461,#39462,
#39463,#39464,#39465,#39466,#39467,#39468,#39469,#39470,#39471,#39472,#39473,
#39474,#39475,#39476,#39477,#39478,#39479,#39480,#39481,#39482,#39483,#39484,
#39485,#39486,#39487,#39488,#39489,#39490,#39491,#39492,#39493,#39494,#39495,
#39496,#39497,#39498,#39499,#39500,#39501,#39502,#39503,#39504,#39505,#39506,
#39507,#39508,#39509,#39510,#39511,#39512,#39513,#39514,#39515,#39516,#39517,
#39518,#39519,#39520,#39521,#39522,#39523,#39524,#39525,#39526,#39527,#39528,
#39529,#39530,#39531,#39532,#39533,#39534,#39535,#39536,#39537,#39538,#39539,
#39540,#39541,#39542,#39543,#39544,#39545,#39546,#39547,#39548,#39549,#39550,
#39551,#39552,#39553,#39554,#39555,#39556,#39557,#39558,#39559,#39560,#39561,
#39562,#39563,#39564,#39565,#39566,#39567,#39568,#39569,#39570,#39571,#39572,
#39573,#39574,#39575,#39576,#39577,#39578,#39579,#39580,#39581,#39582,#39583,
#39584,#39585,#39586,#39587,#39588,#39589,#39590,#39591,#39592,#39593,#39594,
#39595,#39596,#39597,#39598,#39599,#39600,#39601,#39602,#39603,#39604,#39605,
#39606,#39607,#39608,#39609,#39610,#39611,#39612,#39613,#39614,#39615,#39616,
#39617,#39618,#39619,#39620,#39621,#39622,#39623,#39624,#39625,#39626,#39627,
#39628,#39629,#39630,#39631,#39632,#39633,#39634,#39635,#39636,#39637,#39638,
#39639,#39640,#39641,#39642,#39643,#39644,#39645,#39646,#39647,#39648,#39649,
#39650,#39651,#39652,#39653,#39654,#39655,#39656,#39657,#39658,#39659,#39660,
#39661,#39662,#39663,#39664,#39665,#39666,#39667,#39668,#39669,#39670,#39671,
#39672,#39673,#39674,#39675,#39676,#39677,#39678,#39679,#39680,#39681,#39682,
#39683,#39684,#39685,#39686,#39687,#39688,#39689,#39690),.UNSPECIFIED.,
 .F.,.F.,(4,2,2,2,2,2,2,2,2,2,2,2,2,2,2,2,2,2,2,2,2,2,2,2,2,2,2,2,2,2,2,
2,2,2,2,2,2,2,2,2,2,2,2,2,2,2,2,2,2,2,2,2,2,2,2,2,2,2,2,2,2,2,2,2,2,2,2,
2,2,2,2,2,2,2,2,2,2,2,2,2,2,2,2,2,2,2,2,2,2,2,2,2,2,2,2,2,2,2,2,2,2,2,2,
2,2,2,2,2,2,2,2,2,2,2,2,2,2,2,2,2,2,2,2,2,2,2,2,2,2,2,2,2,2,2,2,2,2,2,2,
2,2,2,2,2,2,2,2,2,2,2,2,2,2,2,2,2,2,2,2,2,2,2,2,2,2,2,2,2,2,2,2,2,2,2,2,
2,2,2,2,2,2,2,2,2,2,2,2,2,2,2,2,2,2,2,2,2,2,2,2,2,2,2,2,2,2,2,2,2,2,2,2,
2,2,2,2,2,2,2,2,2,2,2,2,2,2,2,2,2,2,2,2,2,2,2,2,2,2,2,2,2,2,2,2,2,2,2,2,
2,2,2,2,2,2,2,2,2,2,2,2,2,2,2,2,2,4),(-4.06149043156728,-4.00581837979675,
-4.00334052717035,-4.00178628162882,-4.00061102447297,-3.99941522130083,
-3.99830270846965,-3.99678032563153,-3.9929663227205,-3.94283496208982,
-3.93559399747636,-3.87968837448941,-3.84519178415838,-3.84047227863743,
-3.83922752365697,-3.83848824736919,-3.83783011075537,-3.83698779698057,
-3.83531667968692,-3.82524707161149,-3.74956953807414,-3.72705312271508,
-3.70183475903954,-3.68877618215616,-3.68357298393008,-3.67975352803847,
-3.67846556257491,-3.67736342681777,-3.67618331263081,-3.6746837860935,
-3.67174704957063,-3.65478633014764,-3.6497991264112,-3.64080269878064,
-3.62963927160084,-3.62119804548356,-3.56915981071388,-3.56226667259324,
-3.55375611423414,-3.52996644183405,-3.51854339461683,-3.51693125579535,
-3.51611256109848,-3.51545668146772,-3.51479972799191,-3.5135971869704,
-3.50976983199108,-3.4438120568791,-3.40895540672335,-3.37551292595806,
-3.36485612104462,-3.36038094796908,-3.35701000241388,-3.35544335312315,
-3.35424924112962,-3.35313409756134,-3.3516015533835,-3.34854486019619,
-3.3216003522927,-3.30781712735768,-3.23425926036023,-3.20760663529798,
-3.19595596739138,-3.1943362950531,-3.19351602136316,-3.1928599871863,-3.19210638615152,
-3.19083068630761,-3.18623814228809,-3.09927251374508,-3.06419745889802,
-3.0398873146221,-3.03495246253299,-3.03313056723441,-3.03203058020372,
-3.03084154274146,-3.02930145570258,-3.02674681264277,-3.01209429340659,
-2.92550237231264,-2.87597029708654,-2.87234064557186,-2.87120838025185,
-2.87049425032792,-2.86982889785374,-2.86895036320901,-2.86698358020463,
-2.84988436079185,-2.84610545088336,-2.8339040425937,-2.76707668920941,
-2.74317764024306,-2.71744032039752,-2.7139981239142,-2.71126457943566,
-2.70983467542399,-2.70877036626216,-2.70762957077994,-2.70600174033468,
-2.70153932156986,-2.62636815547472,-2.57848969904921,-2.55497182236745,
-2.54996177484238,-2.54869112691636,-2.54794601922052,-2.54728880331071,
-2.54645577824458,-2.54514290787178,-2.53874260340388,-2.53753068473454,
-2.43187177127406,-2.39608482198018,-2.38979856009269,-2.38779313408404,
-2.38651625470472,-2.38532603246938,-2.3837783271904,-2.38119788586569,
-2.36608168458047,-2.32868683484901,-2.30734968855432,-2.26884607016408,
-2.23915095658938,-2.2278257226389,-2.22621691611165,-2.22539893422557,
-2.22474313903802,-2.22398803317378,-2.22270568490794,-2.21804897784234,
-2.1224969681484,-2.07489168827986,-2.06741711229514,-2.06527989616845,
-2.06397371394796,-2.06279234437239,-2.06128063840442,-2.05818307814034,
-2.03876978304821,-2.03128645458859,-2.00806069687948,-1.91679494318129,
-1.90531267034533,-1.90355244270604,-1.90270386033932,-1.90204502495239,
-1.90130941352252,-1.9000809464414,-1.89553587648808,-1.86332732056405,
-1.77640356362562,-1.74694669602831,-1.74381948038043,-1.74226926418756,
-1.74114954963591,-1.73995826071737,-1.7383765341345,-1.73491693651275,
-1.66348636388095,-1.59378958334992,-1.5825878482876,-1.58084044382942,
-1.57999439925936,-1.57933586474762,-1.57859881715422,-1.57736392762368,
-1.57275065278929,-1.5396694464484,-1.45177421040225,-1.42415310459325,
-1.42073536778248,-1.41917852633211,-1.41798689147565,-1.41671396585027,
-1.41472609853827,-1.40858381501322,-1.37410887584643,-1.2758921062224,
-1.27551632601284,-1.27306129249557,-1.25994681084638,-1.25814062957277,
-1.25727939546349,-1.25661682381564,-1.25590959008994,-1.25478076286552,
-1.25344606864184,-1.2508869384759,-1.22653272970793,-1.16286503555609,
-1.10223416078169,-1.09833655796127,-1.09679991229468,-1.09568365846267,
-1.0944901167414,-1.09289520753166,-1.08936555611704,-1.03779243771172,
-0.954186998239568,-0.952818853464944,-0.950404095374525,-0.937242366165131,
-0.935434237443029,-0.934572568802144,-0.93390988750529,-0.933202848443735,
-0.93207816308745,-0.930746999402649,-0.928197281272552,-0.843264101451716,
-0.779452437028871,-0.775546063270499,-0.774007904665031,-0.772891230327678,
-0.771697874907397,-0.770104309525041,-0.766582089573682,-0.71652326986269,
-0.632559474657294,-0.614681095467125,-0.612889293889667,-0.612013881822162,
-0.611387364557665,-0.610758022268843,-0.60990144278341,-0.608095843627627,
-0.605707421512541,-0.600049862069215,-0.581766784428509,-0.54946158457254,
-0.477931658881291,-0.455610072691515,-0.452706520684026,-0.451212959758374,
-0.450107693983158,-0.44890634864501,-0.447266354709601,-0.443488469021795,
-0.400776041374453,-0.360042451484228,-0.317073704317198,-0.310223492392585,
-0.308061028469674,-0.304857846820642,-0.291805659796358,-0.290001525663102,
-0.289140664167135,-0.288478104317273,-0.287864276067738,-0.286820424401417,
-0.283894010626118,-0.279512944889678,-0.266531095712988,-0.245716058379996,
-0.149910075152829,-0.132532027916332,-0.129573024619506,-0.128068681687065,
-0.126887980762742,-0.125577311835715,-0.123420817605302,-0.115759217333069,
-0.0900082820838625,-0.000958367751892826),.UNSPECIFIED.);
#818=B_SPLINE_CURVE_WITH_KNOTS('',3,(#39692,#39693,#39694,#39695,#39696,
#39697,#39698,#39699,#39700,#39701,#39702,#39703,#39704,#39705,#39706,#39707,
#39708,#39709,#39710,#39711,#39712,#39713,#39714,#39715,#39716,#39717,#39718,
#39719,#39720,#39721,#39722,#39723,#39724,#39725,#39726,#39727,#39728,#39729,
#39730,#39731,#39732,#39733,#39734,#39735,#39736,#39737,#39738,#39739,#39740,
#39741,#39742,#39743,#39744,#39745,#39746,#39747,#39748,#39749,#39750,#39751,
#39752,#39753,#39754,#39755,#39756,#39757,#39758,#39759,#39760,#39761,#39762,
#39763,#39764,#39765,#39766,#39767,#39768,#39769,#39770,#39771,#39772,#39773,
#39774,#39775,#39776,#39777,#39778,#39779,#39780,#39781,#39782,#39783,#39784,
#39785,#39786,#39787,#39788,#39789,#39790,#39791,#39792,#39793,#39794,#39795,
#39796,#39797,#39798,#39799,#39800,#39801,#39802,#39803,#39804,#39805,#39806,
#39807,#39808,#39809,#39810,#39811,#39812,#39813,#39814,#39815,#39816,#39817,
#39818,#39819,#39820,#39821,#39822,#39823,#39824,#39825,#39826,#39827,#39828,
#39829,#39830,#39831,#39832,#39833,#39834,#39835,#39836,#39837,#39838,#39839,
#39840,#39841,#39842,#39843,#39844,#39845,#39846,#39847,#39848,#39849,#39850,
#39851,#39852,#39853,#39854,#39855,#39856,#39857,#39858,#39859,#39860,#39861,
#39862,#39863,#39864,#39865,#39866,#39867,#39868,#39869,#39870,#39871,#39872,
#39873,#39874,#39875,#39876,#39877,#39878,#39879,#39880,#39881,#39882,#39883,
#39884,#39885,#39886,#39887,#39888,#39889,#39890,#39891,#39892,#39893,#39894,
#39895,#39896,#39897,#39898,#39899,#39900,#39901,#39902,#39903,#39904,#39905,
#39906,#39907,#39908,#39909,#39910,#39911,#39912,#39913,#39914,#39915,#39916,
#39917,#39918,#39919,#39920,#39921,#39922,#39923,#39924,#39925,#39926,#39927,
#39928,#39929,#39930,#39931,#39932,#39933,#39934,#39935,#39936,#39937,#39938,
#39939,#39940,#39941,#39942,#39943,#39944,#39945,#39946,#39947,#39948,#39949,
#39950,#39951,#39952,#39953,#39954,#39955,#39956,#39957,#39958,#39959,#39960,
#39961,#39962,#39963,#39964,#39965,#39966,#39967,#39968,#39969,#39970,#39971,
#39972,#39973,#39974,#39975,#39976,#39977,#39978,#39979,#39980,#39981,#39982,
#39983,#39984,#39985,#39986,#39987,#39988,#39989,#39990,#39991,#39992,#39993,
#39994,#39995,#39996,#39997,#39998,#39999,#40000,#40001,#40002,#40003,#40004,
#40005,#40006,#40007,#40008,#40009,#40010,#40011,#40012,#40013,#40014,#40015,
#40016,#40017,#40018,#40019,#40020,#40021,#40022,#40023,#40024,#40025,#40026,
#40027,#40028,#40029,#40030,#40031,#40032,#40033,#40034,#40035,#40036,#40037,
#40038,#40039,#40040,#40041,#40042,#40043,#40044,#40045,#40046,#40047,#40048,
#40049,#40050,#40051,#40052,#40053,#40054,#40055,#40056,#40057,#40058,#40059,
#40060,#40061,#40062,#40063,#40064,#40065,#40066,#40067,#40068,#40069,#40070,
#40071,#40072,#40073,#40074,#40075,#40076,#40077,#40078,#40079,#40080,#40081,
#40082,#40083,#40084,#40085,#40086,#40087,#40088,#40089,#40090,#40091,#40092,
#40093,#40094,#40095,#40096,#40097,#40098,#40099,#40100,#40101,#40102,#40103,
#40104,#40105,#40106,#40107,#40108,#40109,#40110,#40111,#40112,#40113,#40114,
#40115,#40116,#40117,#40118,#40119,#40120,#40121,#40122,#40123,#40124,#40125,
#40126,#40127,#40128,#40129,#40130,#40131,#40132,#40133,#40134,#40135,#40136,
#40137,#40138,#40139,#40140,#40141,#40142,#40143,#40144,#40145,#40146,#40147,
#40148,#40149,#40150,#40151,#40152,#40153,#40154,#40155,#40156,#40157,#40158,
#40159,#40160,#40161,#40162,#40163,#40164,#40165,#40166,#40167,#40168,#40169,
#40170,#40171,#40172,#40173,#40174,#40175,#40176,#40177,#40178,#40179,#40180,
#40181,#40182,#40183,#40184,#40185,#40186,#40187,#40188,#40189,#40190,#40191,
#40192,#40193,#40194,#40195,#40196,#40197,#40198,#40199,#40200,#40201,#40202,
#40203,#40204,#40205,#40206,#40207,#40208,#40209,#40210,#40211,#40212,#40213,
#40214,#40215,#40216,#40217,#40218,#40219,#40220,#40221,#40222,#40223,#40224,
#40225,#40226,#40227,#40228,#40229),.UNSPECIFIED.,.F.,.F.,(4,2,2,2,2,2,
2,2,2,2,2,2,2,2,2,2,2,2,2,2,2,2,2,2,2,2,2,2,2,2,2,2,2,2,2,2,2,2,2,2,2,2,
2,2,2,2,2,2,2,2,2,2,2,2,2,2,2,2,2,2,2,2,2,2,2,2,2,2,2,2,2,2,2,2,2,2,2,2,
2,2,2,2,2,2,2,2,2,2,2,2,2,2,2,2,2,2,2,2,2,2,2,2,2,2,2,2,2,2,2,2,2,2,2,2,
2,2,2,2,2,2,2,2,2,2,2,2,2,2,2,2,2,2,2,2,2,2,2,2,2,2,2,2,2,2,2,2,2,2,2,2,
2,2,2,2,2,2,2,2,2,2,2,2,2,2,2,2,2,2,2,2,2,2,2,2,2,2,2,2,2,2,2,2,2,2,2,2,
2,2,2,2,2,2,2,2,2,2,2,2,2,2,2,2,2,2,2,2,2,2,2,2,2,2,2,2,2,2,2,2,2,2,2,2,
2,2,2,2,2,2,2,2,2,2,2,2,2,2,2,2,2,2,2,2,2,2,2,2,2,2,2,2,2,2,2,2,2,2,2,2,
2,2,2,2,2,2,2,2,2,2,4),(-4.05959170843589,-4.02798711726565,-4.02657574666584,
-4.02569821081773,-4.02503952340485,-4.02441785342737,-4.02380279807382,
-4.02297028217099,-4.02134745348974,-4.0088930553482,-4.00781230425048,
-4.00480247029707,-4.00114129986191,-3.99233246825957,-3.98763530297311,
-3.9434148687593,-3.86927957203281,-3.86581573957689,-3.86423358099403,
-3.86304258753128,-3.86192360430866,-3.86037511972845,-3.85725362582928,
-3.82797508100751,-3.74835191021271,-3.72072764495734,-3.71415512390831,
-3.70470467091717,-3.70317176642285,-3.70251732366205,-3.70189290390233,
-3.70127357243822,-3.70042444524356,-3.69829465712175,-3.67238030116506,
-3.62040322323536,-3.61386687090801,-3.60607360222308,-3.57809194091337,
-3.55232520402001,-3.54464998508198,-3.54249273969563,-3.54118226876108,
-3.54000216914384,-3.53849917290203,-3.53554465022416,-3.5182343440434,
-3.51716278962261,-3.44842864192744,-3.41466763944054,-3.39216925670531,
-3.38562606821739,-3.38296857253047,-3.38099666855917,-3.38011091194923,
-3.37948878097006,-3.37887302211558,-3.37803784867234,-3.37640480201369,
-3.36367387713198,-3.36281187431033,-3.36071597296969,-3.35921473934554,
-3.27710713547334,-3.2295566911765,-3.22208803118854,-3.21995181281495,
-3.21864608964093,-3.21746503683688,-3.21595359983778,-3.21285611134719,
-3.1934310514034,-3.19164298126378,-3.11651102403723,-3.06491849121795,
-3.06124173862927,-3.05950275761514,-3.05848997089653,-3.0575870177305,
-3.05692949007532,-3.05631226864745,-3.05547136787374,-3.05338928383838,
-3.02995432911439,-2.93804353213902,-2.90513156133943,-2.89916269867738,
-2.89719680546365,-2.89592905286439,-2.8947359090102,-2.89316789906629,
-2.89051719910072,-2.87405772839289,-2.86864187383323,-2.79501023455936,
-2.73883219948443,-2.73701457363469,-2.73556391599424,-2.73478390243403,
-2.73413569056969,-2.73346759948526,-2.73220895436189,-2.7279057944492,
-2.64578563096422,-2.57912436625523,-2.57567932553791,-2.57410069523568,
-2.57291026331147,-2.571790270368,-2.5702379465274,-2.56710109160943,-2.53724638501829,
-2.45240391603141,-2.41867513926482,-2.41559887887888,-2.41336722508491,
-2.41243227407602,-2.41176003166997,-2.41114373973155,-2.41030645342166,
-2.40866515011107,-2.39570330269601,-2.39501330388163,-2.39461986295685,
-2.35709791092524,-2.32507368568797,-2.28800103281986,-2.26219999296711,
-2.25450712227595,-2.25234806647501,-2.25103716404954,-2.24985710736786,
-2.2483547576235,-2.24540337338364,-2.22815376632442,-2.22710952100059,
-2.13180547075541,-2.09629386730067,-2.09150163144771,-2.09025047514336,
-2.08950988168835,-2.08885218442694,-2.08801259258559,-2.08629709132287,
-2.07575758475101,-2.03111979608886,-1.96202548950655,-1.93401694556256,
-1.93058726062162,-1.92902832378566,-1.92783647108931,-1.9265646579175,
-1.92458130412699,-1.91847439723487,-1.84860619257299,-1.773215877696,-1.76890874629722,
-1.76764943626648,-1.76698109419472,-1.76633270332482,-1.76553651031646,
-1.76403148021447,-1.75532006576985,-1.736692212934,-1.69376311188224,-1.61347885469631,
-1.60864071011227,-1.60676991358382,-1.6056473715245,-1.60445772764382,
-1.60288605630931,-1.59947947694814,-1.54223161526436,-1.45742577332668,
-1.44700629233833,-1.44529663457791,-1.44445813270749,-1.44380046163443,
-1.4430590051924,-1.44180432220659,-1.43697426621603,-1.40093573483828,
-1.30514423660583,-1.28793023346886,-1.28498034768431,-1.28347816113017,
-1.28232213462967,-1.28104467696072,-1.27971133456328,-1.2777586111607,
-1.27431441707586,-1.24854296775392,-1.22462062232874,-1.12803431070674,
-1.12351111501504,-1.12222777887664,-1.12147989787315,-1.12088889653328,
-1.12009196880907,-1.11858380023822,-1.10980843781875,-1.09104153112899,
-1.04549286747864,-0.967707292849795,-0.9630985500505,-0.961448635164033,
-0.960301833748963,-0.95914578438976,-0.957684738309002,-0.956095222590293,
-0.953533309485896,-0.948519761545539,-0.922869431236602,-0.879683448242287,
-0.805052043420515,-0.800803387252043,-0.799550588532969,-0.798883484985961,
-0.798234893918666,-0.797436457537563,-0.795921249659214,-0.786993428910357,
-0.767954563458636,-0.714399064015869,-0.64441466213088,-0.640272145304883,
-0.638694996162758,-0.637568032008948,-0.636403942213641,-0.634889982478615,
-0.633227355967408,-0.630490671408316,-0.625005403129887,-0.610980677314018,
-0.579014859223885,-0.482701703188247,-0.478134850864779,-0.476861754824126,
-0.476108695900897,-0.475452491655252,-0.474631177215927,-0.473006793268334,
-0.46121491224806,-0.434680390385411,-0.389734046836864,-0.363625549918173,
-0.321079887567511,-0.3173748532572,-0.315871108856177,-0.314763235660489,
-0.313587787999309,-0.312006293674183,-0.310250194492015,-0.307288458700993,
-0.301182403455599,-0.284969422389137,-0.267066104057562,-0.217777237427747,
-0.158675528990929,-0.155256064423844,-0.154106105485343,-0.153459647922484,
-0.15286742197733,-0.152059677053076,-0.150500785779767,-0.140551006233259,
-0.117516965148734,-0.0706498920877946,-0.000957648626825045),
 .UNSPECIFIED.);
#819=B_SPLINE_CURVE_WITH_KNOTS('',3,(#40231,#40232,#40233,#40234,#40235,
#40236,#40237,#40238,#40239,#40240,#40241,#40242,#40243,#40244,#40245,#40246,
#40247,#40248,#40249,#40250,#40251,#40252,#40253,#40254,#40255,#40256,#40257,
#40258,#40259,#40260,#40261,#40262,#40263,#40264,#40265,#40266,#40267,#40268,
#40269,#40270,#40271,#40272,#40273,#40274,#40275,#40276,#40277,#40278,#40279,
#40280,#40281,#40282,#40283,#40284,#40285,#40286,#40287,#40288,#40289,#40290,
#40291,#40292,#40293,#40294,#40295,#40296,#40297,#40298,#40299,#40300,#40301,
#40302,#40303,#40304,#40305,#40306,#40307,#40308,#40309,#40310,#40311,#40312,
#40313,#40314,#40315,#40316,#40317,#40318,#40319,#40320,#40321,#40322,#40323,
#40324,#40325,#40326,#40327,#40328,#40329,#40330,#40331,#40332,#40333,#40334,
#40335,#40336,#40337,#40338,#40339,#40340,#40341,#40342,#40343,#40344,#40345,
#40346,#40347,#40348,#40349,#40350,#40351,#40352,#40353,#40354,#40355,#40356,
#40357,#40358,#40359,#40360,#40361,#40362,#40363,#40364,#40365,#40366,#40367,
#40368,#40369,#40370,#40371,#40372,#40373,#40374,#40375,#40376,#40377,#40378,
#40379,#40380,#40381,#40382,#40383,#40384,#40385,#40386,#40387,#40388,#40389,
#40390,#40391,#40392,#40393,#40394,#40395,#40396,#40397,#40398,#40399,#40400,
#40401,#40402,#40403,#40404,#40405,#40406,#40407,#40408,#40409,#40410,#40411,
#40412,#40413,#40414,#40415,#40416,#40417,#40418,#40419,#40420,#40421,#40422,
#40423,#40424,#40425,#40426,#40427,#40428,#40429,#40430,#40431,#40432,#40433,
#40434,#40435,#40436,#40437,#40438,#40439,#40440,#40441,#40442,#40443,#40444,
#40445,#40446,#40447,#40448,#40449,#40450,#40451,#40452,#40453,#40454,#40455,
#40456,#40457,#40458,#40459,#40460,#40461,#40462,#40463,#40464,#40465,#40466,
#40467,#40468,#40469,#40470,#40471,#40472,#40473,#40474,#40475,#40476,#40477,
#40478,#40479,#40480,#40481,#40482,#40483,#40484,#40485,#40486,#40487,#40488,
#40489,#40490,#40491,#40492,#40493,#40494,#40495,#40496,#40497,#40498,#40499,
#40500,#40501,#40502,#40503,#40504,#40505,#40506,#40507,#40508,#40509,#40510,
#40511,#40512,#40513,#40514,#40515,#40516,#40517,#40518,#40519,#40520,#40521,
#40522,#40523,#40524,#40525,#40526,#40527,#40528,#40529,#40530,#40531,#40532,
#40533,#40534,#40535,#40536,#40537,#40538,#40539,#40540,#40541,#40542,#40543,
#40544,#40545,#40546,#40547,#40548,#40549,#40550,#40551,#40552,#40553,#40554,
#40555,#40556,#40557,#40558,#40559,#40560,#40561,#40562,#40563,#40564,#40565,
#40566,#40567,#40568,#40569,#40570,#40571,#40572,#40573,#40574,#40575,#40576,
#40577,#40578,#40579,#40580,#40581,#40582,#40583,#40584,#40585,#40586,#40587,
#40588,#40589,#40590,#40591,#40592,#40593,#40594,#40595,#40596,#40597,#40598,
#40599,#40600,#40601,#40602,#40603,#40604,#40605,#40606,#40607,#40608,#40609,
#40610,#40611,#40612,#40613,#40614,#40615,#40616,#40617,#40618,#40619,#40620,
#40621,#40622,#40623,#40624,#40625,#40626,#40627,#40628,#40629,#40630,#40631,
#40632,#40633,#40634,#40635,#40636,#40637,#40638,#40639,#40640,#40641,#40642,
#40643,#40644,#40645,#40646,#40647,#40648,#40649,#40650,#40651,#40652,#40653,
#40654,#40655,#40656,#40657,#40658,#40659,#40660,#40661,#40662,#40663,#40664,
#40665,#40666,#40667,#40668,#40669,#40670,#40671,#40672,#40673,#40674,#40675,
#40676,#40677,#40678,#40679,#40680,#40681,#40682,#40683,#40684,#40685,#40686,
#40687,#40688,#40689,#40690,#40691,#40692,#40693,#40694,#40695,#40696,#40697,
#40698,#40699,#40700,#40701,#40702,#40703,#40704,#40705,#40706,#40707,#40708,
#40709,#40710,#40711,#40712,#40713,#40714,#40715,#40716,#40717,#40718,#40719,
#40720,#40721,#40722,#40723,#40724,#40725,#40726,#40727,#40728,#40729,#40730,
#40731,#40732,#40733,#40734,#40735,#40736,#40737,#40738,#40739,#40740,#40741,
#40742,#40743,#40744,#40745,#40746,#40747,#40748,#40749,#40750,#40751,#40752,
#40753,#40754,#40755,#40756,#40757,#40758,#40759,#40760,#40761,#40762,#40763,
#40764,#40765,#40766,#40767,#40768),.UNSPECIFIED.,.F.,.F.,(4,2,2,2,2,2,
2,2,2,2,2,2,2,2,2,2,2,2,2,2,2,2,2,2,2,2,2,2,2,2,2,2,2,2,2,2,2,2,2,2,2,2,
2,2,2,2,2,2,2,2,2,2,2,2,2,2,2,2,2,2,2,2,2,2,2,2,2,2,2,2,2,2,2,2,2,2,2,2,
2,2,2,2,2,2,2,2,2,2,2,2,2,2,2,2,2,2,2,2,2,2,2,2,2,2,2,2,2,2,2,2,2,2,2,2,
2,2,2,2,2,2,2,2,2,2,2,2,2,2,2,2,2,2,2,2,2,2,2,2,2,2,2,2,2,2,2,2,2,2,2,2,
2,2,2,2,2,2,2,2,2,2,2,2,2,2,2,2,2,2,2,2,2,2,2,2,2,2,2,2,2,2,2,2,2,2,2,2,
2,2,2,2,2,2,2,2,2,2,2,2,2,2,2,2,2,2,2,2,2,2,2,2,2,2,2,2,2,2,2,2,2,2,2,2,
2,2,2,2,2,2,2,2,2,2,2,2,2,2,2,2,2,2,2,2,2,2,2,2,2,2,2,2,2,2,2,2,2,2,2,2,
2,2,2,2,2,2,2,2,2,2,4),(-4.06107074159402,-4.05792311628498,-4.05505650757302,
-4.05370667619582,-4.05259411403693,-4.05153489084243,-4.05017190820217,
-4.04784210490371,-4.0400948612384,-3.93199530309746,-3.89746054387593,
-3.89273812527517,-3.89149306368082,-3.89075369604527,-3.89009553725701,
-3.88925327460879,-3.88758250956353,-3.87752097976065,-3.8329010998466,
-3.74206956993004,-3.73625782372181,-3.73340214139118,-3.73169003707714,
-3.7301406158905,-3.72897086964434,-3.72785500279065,-3.72631964798947,
-3.72242931441017,-3.66334154064967,-3.63357801875161,-3.6095968340008,
-3.57480694936298,-3.57167926388291,-3.56941789073379,-3.5684776896975,
-3.56780428551313,-3.56718881993942,-3.56635535935952,-3.56472954220267,
-3.55220740780105,-3.45124318580869,-3.42216011295069,-3.41476286397144,
-3.41134991418941,-3.40940977234448,-3.40769653027833,-3.40649592577635,
-3.40530301910232,-3.40384782014859,-3.40034032993913,-3.36812601629823,
-3.30885430922902,-3.29670936875526,-3.28408722341385,-3.25190585175597,
-3.24736375079728,-3.24613568924646,-3.2454002408586,-3.24474149748169,
-3.24389296294816,-3.2421325801564,-3.23064271199369,-3.22889460598271,
-3.13766056856445,-3.11518768505876,-3.0978575536199,-3.09144417073204,
-3.08837338372757,-3.08657262658688,-3.08496109143267,-3.08422957136854,
-3.08307422431332,-3.08157287593419,-3.07862660602756,-3.06147774582934,
-2.96760109378171,-2.9263314851616,-2.92405188672545,-2.92310866049859,
-2.92243472855039,-2.92181996208877,-2.92098912924519,-2.91937337264755,
-2.90711995962076,-2.90383673018631,-2.90348884890933,-2.90216993680237,
-2.82659539722198,-2.77308276103603,-2.76783062472699,-2.76517994034335,
-2.76355330198508,-2.76206548727548,-2.76090529718656,-2.75976937624903,
-2.75815870001489,-2.75380551969949,-2.68523113948357,-2.63071785528902,
-2.61158196328927,-2.6025657961901,-2.60104678115628,-2.60024761945674,
-2.59959910054777,-2.59893265756538,-2.59768278639568,-2.59345855794327,
-2.51561258175736,-2.44455929077339,-2.44110104609599,-2.43951967186602,
-2.43832853823853,-2.4372088878825,-2.43535300003718,-2.430606158018,-2.35644157996629,
-2.32154146527208,-2.29147218849282,-2.28006957227897,-2.27845833559954,
-2.27763991479335,-2.27698416316504,-2.27622954893315,-2.27494905409372,
-2.27030910629864,-2.17460824598838,-2.12176670714617,-2.11838631518486,
-2.11681970664643,-2.11563093859031,-2.11450702992522,-2.11262875425422,
-2.10774354659412,-2.03074199268243,-1.96056778899028,-1.95664786367709,
-1.95543405589394,-1.95477490662266,-1.95411945766315,-1.95330516073203,
-1.95171383258012,-1.94088853168741,-1.91348114940625,-1.83555327327358,
-1.81902461912921,-1.81385186794283,-1.79837384614871,-1.79577411452154,
-1.794220875633,-1.79302995314925,-1.79175579531467,-1.78976187043001,-1.78356863919322,
-1.74862592498321,-1.6481671615945,-1.63500535769052,-1.63319747792301,
-1.6323359560139,-1.63167340033351,-1.63095187098498,-1.62978622831091,
-1.62585952717989,-1.60077650712587,-1.55311615216838,-1.47805206329176,
-1.47362265767696,-1.47200005079682,-1.47086079708855,-1.46979624400581,
-1.46833410814099,-1.46548062513414,-1.44596870537084,-1.42667819134169,
-1.3293843991285,-1.32837123575537,-1.32705135095524,-1.31236557973351,
-1.31066505810144,-1.30981248943284,-1.30919204807235,-1.30853602327453,
-1.30764469821822,-1.30664796874454,-1.30494874151072,-1.25941885562339,
-1.17012498809876,-1.15299958690595,-1.15005397843829,-1.14855252708944,
-1.14737217627416,-1.14605991459967,-1.14389624544586,-1.13616262978701,
-1.11110702888269,-1.06866311766076,-1.00288118907866,-1.00077557592566,
-0.989457363641942,-0.98770449530953,-0.986857327793933,-0.986213632432669,
-0.985540233875388,-0.984414129577513,-0.983082568101587,-0.980531701875951,
-0.895536280521014,-0.831804152416426,-0.827898274939483,-0.826360288186352,
-0.825243730393034,-0.824050491819685,-0.822457069219483,-0.81893511095283,
-0.768863694892824,-0.757168978242177,-0.670295445749342,-0.665869313808614,
-0.664596510676812,-0.663850925036437,-0.663206762745967,-0.662398481959153,
-0.661517129204842,-0.660097023996654,-0.657309889348625,-0.650329849046117,
-0.635813018063733,-0.61119151185388,-0.536618651195705,-0.508303071883821,
-0.504862921997067,-0.503301738897064,-0.502109205807514,-0.50083767116124,
-0.498856820316133,-0.492773497165741,-0.3994197498584,-0.385142560644,
-0.360855134446266,-0.34424935647815,-0.342491366236673,-0.341624353986918,
-0.34100008658254,-0.340346422548127,-0.33945549313304,-0.338471074793271,
-0.336801977663959,-0.333325827066347,-0.323885484307112,-0.300378522497625,
-0.214977475826035,-0.185568068886635,-0.182441649627592,-0.180891475629612,
-0.179771626636407,-0.178580041525473,-0.17699766082912,-0.173535592333841,
-0.101309985512579,-0.0368048490202745,-0.0326796191665078,-0.0212083070452828,
-0.0194483451149031,-0.0185997227515182,-0.0179648019798001,-0.0173504645605992,
-0.0166340895606322,-0.0156094238509372,-0.0138416644030553,-0.0009566108525659),
 .UNSPECIFIED.);
#820=B_SPLINE_CURVE_WITH_KNOTS('',3,(#40770,#40771,#40772,#40773,#40774,
#40775,#40776,#40777,#40778,#40779,#40780,#40781,#40782,#40783,#40784,#40785,
#40786,#40787,#40788,#40789,#40790,#40791,#40792,#40793,#40794,#40795,#40796,
#40797,#40798,#40799,#40800,#40801,#40802,#40803,#40804,#40805,#40806,#40807,
#40808,#40809,#40810,#40811,#40812,#40813,#40814,#40815,#40816,#40817,#40818,
#40819,#40820,#40821,#40822,#40823,#40824,#40825,#40826,#40827,#40828,#40829,
#40830,#40831,#40832,#40833,#40834,#40835,#40836,#40837,#40838,#40839,#40840,
#40841,#40842,#40843,#40844,#40845,#40846,#40847,#40848,#40849,#40850,#40851,
#40852,#40853,#40854,#40855,#40856,#40857,#40858,#40859,#40860,#40861,#40862,
#40863,#40864,#40865,#40866,#40867,#40868,#40869,#40870,#40871,#40872,#40873,
#40874,#40875,#40876,#40877,#40878,#40879,#40880,#40881,#40882,#40883,#40884,
#40885,#40886,#40887,#40888,#40889,#40890,#40891,#40892,#40893,#40894,#40895,
#40896,#40897,#40898,#40899,#40900,#40901,#40902,#40903,#40904,#40905,#40906,
#40907,#40908,#40909,#40910,#40911,#40912,#40913,#40914,#40915,#40916,#40917,
#40918,#40919,#40920,#40921,#40922,#40923,#40924,#40925,#40926,#40927,#40928,
#40929,#40930,#40931,#40932,#40933,#40934,#40935,#40936,#40937,#40938,#40939,
#40940,#40941,#40942,#40943,#40944,#40945,#40946,#40947,#40948,#40949,#40950,
#40951,#40952,#40953,#40954,#40955,#40956,#40957,#40958,#40959,#40960,#40961,
#40962,#40963,#40964,#40965,#40966,#40967,#40968,#40969,#40970,#40971,#40972,
#40973,#40974,#40975,#40976,#40977,#40978,#40979,#40980,#40981,#40982,#40983,
#40984,#40985,#40986,#40987,#40988,#40989,#40990,#40991,#40992,#40993,#40994,
#40995,#40996,#40997,#40998,#40999,#41000,#41001,#41002,#41003,#41004,#41005,
#41006,#41007,#41008,#41009,#41010,#41011,#41012,#41013,#41014,#41015,#41016,
#41017,#41018,#41019,#41020,#41021,#41022,#41023,#41024,#41025,#41026,#41027,
#41028,#41029,#41030,#41031,#41032,#41033,#41034,#41035,#41036,#41037,#41038,
#41039,#41040,#41041,#41042,#41043,#41044,#41045,#41046,#41047,#41048,#41049,
#41050,#41051,#41052,#41053,#41054,#41055,#41056,#41057,#41058,#41059,#41060,
#41061,#41062,#41063,#41064,#41065,#41066,#41067,#41068,#41069,#41070,#41071,
#41072,#41073,#41074,#41075,#41076,#41077,#41078,#41079,#41080,#41081,#41082,
#41083,#41084,#41085,#41086,#41087,#41088,#41089,#41090,#41091,#41092,#41093,
#41094,#41095,#41096,#41097,#41098,#41099,#41100,#41101,#41102,#41103,#41104,
#41105,#41106,#41107,#41108,#41109,#41110,#41111,#41112,#41113,#41114,#41115,
#41116,#41117,#41118,#41119,#41120,#41121,#41122,#41123,#41124,#41125,#41126,
#41127,#41128,#41129,#41130,#41131,#41132,#41133,#41134,#41135,#41136,#41137,
#41138,#41139,#41140,#41141,#41142,#41143,#41144,#41145,#41146,#41147,#41148,
#41149,#41150,#41151,#41152,#41153,#41154,#41155,#41156,#41157,#41158,#41159,
#41160,#41161,#41162,#41163,#41164,#41165,#41166,#41167,#41168,#41169,#41170,
#41171,#41172,#41173,#41174,#41175,#41176,#41177,#41178,#41179,#41180,#41181,
#41182,#41183,#41184,#41185,#41186,#41187,#41188,#41189,#41190,#41191,#41192,
#41193,#41194,#41195,#41196,#41197,#41198,#41199,#41200,#41201,#41202,#41203,
#41204,#41205,#41206,#41207,#41208,#41209,#41210,#41211,#41212,#41213,#41214,
#41215,#41216,#41217,#41218,#41219,#41220,#41221,#41222,#41223,#41224,#41225,
#41226,#41227,#41228,#41229,#41230,#41231,#41232,#41233,#41234,#41235,#41236,
#41237,#41238,#41239,#41240,#41241,#41242,#41243,#41244,#41245,#41246,#41247,
#41248,#41249,#41250,#41251,#41252,#41253,#41254,#41255,#41256,#41257,#41258,
#41259,#41260,#41261,#41262,#41263,#41264,#41265,#41266,#41267,#41268,#41269,
#41270,#41271,#41272,#41273,#41274,#41275,#41276,#41277,#41278,#41279,#41280,
#41281,#41282,#41283,#41284,#41285,#41286,#41287,#41288,#41289,#41290,#41291,
#41292,#41293,#41294,#41295,#41296,#41297,#41298,#41299,#41300,#41301,#41302,
#41303,#41304,#41305,#41306,#41307,#41308,#41309,#41310,#41311,#41312,#41313),
 .UNSPECIFIED.,.F.,.F.,(4,2,2,2,2,2,2,2,2,2,2,2,2,2,2,2,2,2,2,2,2,2,2,2,
2,2,2,2,2,2,2,2,2,2,2,2,2,2,2,2,2,2,2,2,2,2,2,2,2,2,2,2,2,2,2,2,2,2,2,2,
2,2,2,2,2,2,2,2,2,2,2,2,2,2,2,2,2,2,2,2,2,2,2,2,2,2,2,2,2,2,2,2,2,2,2,2,
2,2,2,2,2,2,2,2,2,2,2,2,2,2,2,2,2,2,2,2,2,2,2,2,2,2,2,2,2,2,2,2,2,2,2,2,
2,2,2,2,2,2,2,2,2,2,2,2,2,2,2,2,2,2,2,2,2,2,2,2,2,2,2,2,2,2,2,2,2,2,2,2,
2,2,2,2,2,2,2,2,2,2,2,2,2,2,2,2,2,2,2,2,2,2,2,2,2,2,2,2,2,2,2,2,2,2,2,2,
2,2,2,2,2,2,2,2,2,2,2,2,2,2,2,2,2,2,2,2,2,2,2,2,2,2,2,2,2,2,2,2,2,2,2,2,
2,2,2,2,2,2,2,2,2,2,2,2,2,2,2,2,2,2,2,2,2,2,2,2,2,2,2,2,2,2,2,4),(-4.05989992915858,
-3.97542443936791,-3.93765455717652,-3.92075434847969,-3.91800229329291,
-3.91656200837748,-3.91550079003599,-3.9143529952597,-3.91269759599141,
-3.90804737278844,-3.90631984662432,-3.80199691578861,-3.77276469656581,
-3.7624611628741,-3.75875738490944,-3.75700914207113,-3.75599266351523,
-3.75508712065577,-3.75442878185482,-3.75381229442994,-3.75297385899741,
-3.7509052150137,-3.72808158417878,-3.70106738734646,-3.67010396306551,
-3.59933306399446,-3.59587696631157,-3.59429641058669,-3.59310582598412,
-3.59198664222436,-3.59043695264855,-3.58731013996494,-3.55781949030078,
-3.50926534502195,-3.46260451063372,-3.44410441135709,-3.43797090977061,
-3.43543693431227,-3.43411204714131,-3.4329901408467,-3.43228475338396,
-3.43163940778628,-3.43078546161704,-3.42894856062762,-3.4156186331254,
-3.41336492226598,-3.37186293663109,-3.32767837629357,-3.27709402895805,
-3.27357159087048,-3.27197866744232,-3.27078609390776,-3.26967036873029,
-3.26813385911199,-3.26423347986733,-3.20212173215203,-3.1178012262114,
-3.11400200536771,-3.11222071053332,-3.11119076549668,-3.11027612591858,
-3.10961580166741,-3.10900141840892,-3.10817148144552,-3.10655857385836,
-3.09435390097841,-3.02852226239184,-2.98547801671621,-2.9598898293343,
-2.95489291930771,-2.95116798346484,-2.94953809268848,-2.94833916501601,
-2.94723261366667,-2.94573197376895,-2.94279891321758,-2.91963642512135,
-2.90924047069381,-2.82808197429416,-2.80811523523283,-2.79203145273174,
-2.79001350443487,-2.78888858665651,-2.78813101468013,-2.7874106617429,
-2.78676854826433,-2.78592895750131,-2.78421292656896,-2.77365769947996,
-2.70263332844547,-2.66325605466512,-2.63750362485612,-2.62983551501849,
-2.62767905344853,-2.6263688005181,-2.62518873038106,-2.62368554267905,
-2.6207299201731,-2.60339672062262,-2.59988350424946,-2.50659162148337,
-2.47160765921039,-2.46847128889202,-2.46620507044399,-2.46526420928015,
-2.46459082196739,-2.46397572556954,-2.46314326925843,-2.46152089551297,
-2.44908318904217,-2.44798724320224,-2.44719932912115,-2.35930037503475,
-2.31433114387829,-2.30956342873598,-2.30597627554167,-2.30437120860514,
-2.30317641546634,-2.30206356321773,-2.30053872793626,-2.29670827133356,
-2.24497720441269,-2.18356750964765,-2.15778809962833,-2.14500176960697,
-2.14334811708189,-2.14252109110296,-2.14192678431162,-2.14128980403439,
-2.14018583739283,-2.13709092590166,-2.08189503917666,-2.03127542672754,
-2.01340219610737,-2.00541130457527,-1.98633703691398,-1.98325594197837,
-1.98174770766263,-1.98056696349491,-1.97925933553833,-1.97711489369088,
-1.96956686947523,-1.94404662555513,-1.90115540616016,-1.82611898482838,
-1.82183424126883,-1.82057758765004,-1.81990984550191,-1.81926152612959,
-1.81846469480406,-1.81695630714273,-1.80816910186986,-1.78937795610727,
-1.74357943140737,-1.66624566491097,-1.6615519351191,-1.65988960276889,
-1.65873956150045,-1.65767825263551,-1.65624084775174,-1.65350433614937,
-1.63699137157467,-1.60130056304688,-1.50365757092414,-1.49921723976541,
-1.49794307209154,-1.49719730067033,-1.4966061252213,-1.49580660541988,
-1.49428589520743,-1.48523174864873,-1.46608681513765,-1.41865485452393,
-1.34325277039749,-1.33879352171768,-1.33716642457734,-1.33602601164056,
-1.3348673659768,-1.33339313369555,-1.33178343321872,-1.32917319361608,
-1.32402987412637,-1.27256836805075,-1.18764356064116,-1.17730115115038,
-1.17559538295946,-1.17475765623421,-1.17410006170739,-1.17335811896915,
-1.17210128045753,-1.16724715466541,-1.14410806064156,-1.09852152421232,
-1.06305474521822,-1.01959415314777,-1.01587383840937,-1.01436765133685,
-1.01325933700123,-1.01208498608285,-1.01050489176729,-1.0087524102339,
-1.00579911276715,-0.999716081230722,-0.909180692343531,-0.86463435908407,
-0.854630615426017,-0.852962805667472,-0.852121178630782,-0.851463096720103,
-0.850723363950881,-0.849476650676588,-0.844736036962455,-0.809959015231754,
-0.716801035759007,-0.713222103223423,-0.695616152401385,-0.692645460919935,
-0.691138689759898,-0.689957793804983,-0.688674980095775,-0.686599911262268,
-0.684141212044954,-0.679401829828679,-0.667887674497593,-0.645236433402913,
-0.542631233300566,-0.531856118149043,-0.530128443210877,-0.529286221068031,
-0.528628009626192,-0.527888490519846,-0.526642964388592,-0.521916366951134,
-0.487334555192299,-0.477630447403251,-0.469693261699333,-0.462940795973436,
-0.404264453894064,-0.398833268763276,-0.393157078777552,-0.373071154468099,
-0.369941760184237,-0.368423412135481,-0.367240874792499,-0.366139496366874,
-0.364248863128718,-0.358827964164018,-0.350763826460689,-0.327132169738837,
-0.305848227375618,-0.222471394104182,-0.209343778077339,-0.20753681575816,
-0.206675320794779,-0.206012599221801,-0.205290695751057,-0.204124040741387,
-0.200190203975901,-0.175036332214692,-0.0902231898238672,-0.0835047851764577,
-0.0757971263120287,-0.0702444836189663,-0.0502993545465698,-0.047176311950564,
-0.0456591956395599,-0.0444767807691945,-0.0433753113320354,-0.042096307549911,
-0.0402758606323557,-0.0371576634159707,-0.000956516702297368),
 .UNSPECIFIED.);
#821=B_SPLINE_CURVE_WITH_KNOTS('',3,(#41315,#41316,#41317,#41318,#41319,
#41320,#41321,#41322,#41323,#41324,#41325,#41326,#41327,#41328,#41329,#41330,
#41331,#41332,#41333,#41334,#41335,#41336,#41337,#41338,#41339,#41340,#41341,
#41342,#41343,#41344,#41345,#41346,#41347,#41348,#41349,#41350,#41351,#41352,
#41353,#41354,#41355,#41356,#41357,#41358,#41359,#41360,#41361,#41362,#41363,
#41364,#41365,#41366,#41367,#41368,#41369,#41370,#41371,#41372,#41373,#41374,
#41375,#41376,#41377,#41378,#41379,#41380,#41381,#41382,#41383,#41384,#41385,
#41386,#41387,#41388,#41389,#41390,#41391,#41392,#41393,#41394,#41395,#41396,
#41397,#41398,#41399,#41400,#41401,#41402,#41403,#41404,#41405,#41406,#41407,
#41408,#41409,#41410,#41411,#41412,#41413,#41414,#41415,#41416,#41417,#41418,
#41419,#41420,#41421,#41422,#41423,#41424,#41425,#41426,#41427,#41428,#41429,
#41430,#41431,#41432,#41433,#41434,#41435,#41436,#41437,#41438,#41439,#41440,
#41441,#41442,#41443,#41444,#41445,#41446,#41447,#41448,#41449,#41450,#41451,
#41452,#41453,#41454,#41455,#41456,#41457,#41458,#41459,#41460,#41461,#41462,
#41463,#41464,#41465,#41466,#41467,#41468,#41469,#41470,#41471,#41472,#41473,
#41474,#41475,#41476,#41477,#41478,#41479,#41480,#41481,#41482,#41483,#41484,
#41485,#41486,#41487,#41488,#41489,#41490,#41491,#41492,#41493,#41494,#41495,
#41496,#41497,#41498,#41499,#41500,#41501,#41502,#41503,#41504,#41505,#41506,
#41507,#41508,#41509,#41510,#41511,#41512,#41513,#41514,#41515,#41516,#41517,
#41518,#41519,#41520,#41521,#41522,#41523,#41524,#41525,#41526,#41527,#41528,
#41529,#41530,#41531,#41532,#41533,#41534,#41535,#41536,#41537,#41538,#41539,
#41540,#41541,#41542,#41543,#41544,#41545,#41546,#41547,#41548,#41549,#41550,
#41551,#41552,#41553,#41554,#41555,#41556,#41557,#41558,#41559,#41560,#41561,
#41562,#41563,#41564,#41565,#41566,#41567,#41568,#41569,#41570,#41571,#41572,
#41573,#41574,#41575,#41576,#41577,#41578,#41579,#41580,#41581,#41582,#41583,
#41584,#41585,#41586,#41587,#41588,#41589,#41590,#41591,#41592,#41593,#41594,
#41595,#41596,#41597,#41598,#41599,#41600,#41601,#41602,#41603,#41604,#41605,
#41606,#41607,#41608,#41609,#41610,#41611,#41612,#41613,#41614,#41615,#41616,
#41617,#41618,#41619,#41620,#41621,#41622,#41623,#41624,#41625,#41626,#41627,
#41628,#41629,#41630,#41631,#41632,#41633,#41634,#41635,#41636,#41637,#41638,
#41639,#41640,#41641,#41642,#41643,#41644,#41645,#41646,#41647,#41648,#41649,
#41650,#41651,#41652,#41653,#41654,#41655,#41656,#41657,#41658,#41659,#41660,
#41661,#41662,#41663,#41664,#41665,#41666,#41667,#41668,#41669,#41670,#41671,
#41672,#41673,#41674,#41675,#41676,#41677,#41678,#41679,#41680,#41681,#41682,
#41683,#41684,#41685,#41686,#41687,#41688,#41689,#41690,#41691,#41692,#41693,
#41694,#41695,#41696,#41697,#41698,#41699,#41700,#41701,#41702,#41703,#41704,
#41705,#41706,#41707,#41708,#41709,#41710,#41711,#41712,#41713,#41714,#41715,
#41716,#41717,#41718,#41719,#41720,#41721,#41722,#41723,#41724,#41725,#41726,
#41727,#41728,#41729,#41730,#41731,#41732,#41733,#41734,#41735,#41736,#41737,
#41738,#41739,#41740,#41741,#41742,#41743,#41744,#41745,#41746,#41747,#41748,
#41749,#41750,#41751,#41752,#41753,#41754,#41755,#41756,#41757,#41758,#41759,
#41760,#41761,#41762,#41763,#41764,#41765,#41766,#41767,#41768,#41769,#41770,
#41771,#41772,#41773,#41774,#41775,#41776,#41777,#41778,#41779,#41780,#41781,
#41782,#41783,#41784,#41785,#41786,#41787,#41788,#41789,#41790,#41791,#41792,
#41793,#41794,#41795,#41796,#41797,#41798,#41799,#41800,#41801,#41802,#41803,
#41804,#41805,#41806,#41807,#41808,#41809,#41810,#41811,#41812,#41813,#41814,
#41815,#41816,#41817,#41818,#41819,#41820,#41821,#41822,#41823,#41824,#41825,
#41826,#41827,#41828,#41829,#41830,#41831,#41832,#41833,#41834,#41835,#41836,
#41837,#41838,#41839,#41840,#41841,#41842,#41843,#41844,#41845,#41846,#41847,
#41848,#41849,#41850,#41851,#41852,#41853,#41854,#41855,#41856,#41857,#41858,
#41859,#41860,#41861,#41862),.UNSPECIFIED.,.F.,.F.,(4,2,2,2,2,2,2,2,2,2,
2,2,2,2,2,2,2,2,2,2,2,2,2,2,2,2,2,2,2,2,2,2,2,2,2,2,2,2,2,2,2,2,2,2,2,2,
2,2,2,2,2,2,2,2,2,2,2,2,2,2,2,2,2,2,2,2,2,2,2,2,2,2,2,2,2,2,2,2,2,2,2,2,
2,2,2,2,2,2,2,2,2,2,2,2,2,2,2,2,2,2,2,2,2,2,2,2,2,2,2,2,2,2,2,2,2,2,2,2,
2,2,2,2,2,2,2,2,2,2,2,2,2,2,2,2,2,2,2,2,2,2,2,2,2,2,2,2,2,2,2,2,2,2,2,2,
2,2,2,2,2,2,2,2,2,2,2,2,2,2,2,2,2,2,2,2,2,2,2,2,2,2,2,2,2,2,2,2,2,2,2,2,
2,2,2,2,2,2,2,2,2,2,2,2,2,2,2,2,2,2,2,2,2,2,2,2,2,2,2,2,2,2,2,2,2,2,2,2,
2,2,2,2,2,2,2,2,2,2,2,2,2,2,2,2,2,2,2,2,2,2,2,2,2,2,2,2,2,2,2,2,2,2,2,2,
2,2,2,2,2,2,2,2,2,2,2,4),(-4.06041562041457,-3.97343373173595,-3.95442637936347,
-3.94552365114943,-3.9440094887776,-3.943211233984,-3.94262004933636,-3.9418730039183,
-3.94059365560091,-3.93610794809912,-3.83922561225848,-3.82378937695582,
-3.79883945183429,-3.7904400024817,-3.78484711605959,-3.78293070092868,
-3.78182868750865,-3.78064830464436,-3.77914651357275,-3.77619929512866,
-3.75904312305322,-3.75541945648697,-3.7453832706041,-3.69732964688064,
-3.65701679974696,-3.62669353702674,-3.62230232341125,-3.6210886746521,
-3.62035636985202,-3.61969677087007,-3.61885619033214,-3.61709054005959,
-3.60548840513624,-3.51441887903404,-3.48000390925606,-3.46927265032198,
-3.46477437144957,-3.46240747593738,-3.46046666904196,-3.45918231783831,
-3.45800178343789,-3.45649788911251,-3.45354051305316,-3.43618873919216,
-3.43267368496004,-3.34938925944133,-3.30125482638702,-3.29899089305309,
-3.29805022928541,-3.29737671144118,-3.29676129938635,-3.29592813578425,
-3.29430355912873,-3.28181680640983,-3.28075703227766,-3.28037076031094,
-3.18055889701578,-3.1513675222654,-3.144181290362,-3.14084068950504,-3.13817341164928,
-3.13675796465361,-3.13559024372659,-3.13424376827514,-3.13198473102816,
-3.12403044560653,-3.12208368966232,-3.11903957250021,-3.11780884970613,
-3.11727654513758,-3.01779313833982,-2.9816575315634,-2.97682098244964,
-2.97556562844794,-2.97482397204346,-2.97416624943387,-2.97332785229426,
-2.97161898594325,-2.96121786679749,-2.87640807894311,-2.82493709196789,
-2.81979239873427,-2.81718149568649,-2.81557142903982,-2.81409538474537,
-2.81293664330545,-2.8117957851141,-2.81016745872443,-2.80570115155815,
-2.73039280987081,-2.68284351026427,-2.66372927624845,-2.65459362421853,
-2.65306911543051,-2.65226871850029,-2.65167737901053,-2.65093204250992,
-2.64966014263574,-2.64524146220511,-2.54740940156743,-2.49724161640787,
-2.49328380176823,-2.49161267734301,-2.49040592455061,-2.48930763870141,
-2.48784130693746,-2.48427092634136,-2.44953359574334,-2.38894156324582,
-2.33479000225473,-2.33116065888664,-2.3300285409666,-2.32931451650866,
-2.32864927141295,-2.32777089134027,-2.32580450750855,-2.30871097218493,
-2.30795433433687,-2.21148500795778,-2.17740349962264,-2.17130406700221,
-2.16932155794159,-2.16804987991084,-2.16685786560042,-2.16529830206433,
-2.16186555155248,-2.13376380973773,-2.04300015957484,-2.03018259416502,
-2.02902064859929,-2.02623546315635,-2.02351236954705,-2.02312326527646,
-2.0220348670207,-2.00958164150667,-2.00795839386974,-2.00712560524734,
-2.00651031913182,-2.00583678158825,-2.00489581178174,-2.00262981289646,
-1.94255157521496,-1.8753141094043,-1.86999915480501,-1.85061091931076,
-1.84751433983441,-1.84600275672387,-1.84482132092562,-1.84351489979493,
-1.84137691708646,-1.83389596665621,-1.78621390301534,-1.69046509587776,
-1.68598186903667,-1.6847028005894,-1.68395582202063,-1.68336463433024,
-1.68256630618228,-1.68105177716823,-1.67214069206191,-1.65312563544515,
-1.60618808240319,-1.55857587910291,-1.54870089229428,-1.54513009798313,
-1.5277634439923,-1.5248048741991,-1.52330055441126,-1.52211977532819,-1.52080892043176,
-1.51865189280043,-1.51098608940735,-1.4852261079304,-1.44182071639483,
-1.37969492070576,-1.36443061245622,-1.36252200274486,-1.36165416321048,
-1.36099052740503,-1.36027170789321,-1.3591416760238,-1.35551061089498,
-1.33334748547279,-1.29921277754502,-1.21616519692179,-1.20973743340778,
-1.20347601002975,-1.20139492324095,-1.20023046698983,-1.19917136678551,
-1.19775983746112,-1.19519860151676,-1.18207388930441,-1.15628747752221,
-1.0798590212369,-1.06037940120976,-1.05897140949891,-1.04182132728312,
-1.03985296054016,-1.03897411040627,-1.0383086791725,-1.03759462594159,
-1.03648553617086,-1.0330470238798,-1.01276700576541,-0.978282491595887,
-0.926031259196154,-0.907175992822879,-0.901971993996287,-0.882629988255019,
-0.879535055799057,-0.878023586020754,-0.876841923804009,-0.875534930454254,
-0.873395281027855,-0.866062899257342,-0.845347959064553,-0.822499607975562,
-0.767714687448652,-0.720346744892809,-0.717637366356654,-0.716697317367491,
-0.716053055579729,-0.7154603749953,-0.714648315348204,-0.713100295116653,
-0.703295363356361,-0.681328181737579,-0.631702109315803,-0.562038965925123,
-0.557622006226427,-0.556001113337803,-0.554862175966818,-0.553797212589503,
-0.552333416039696,-0.550767739263672,-0.543513221464304,-0.510480090555925,
-0.457090986234711,-0.413789226998515,-0.396595588845203,-0.394625226119335,
-0.393746006282068,-0.393080507627494,-0.392366596534047,-0.391634700669151,
-0.390572149836311,-0.38230141922074,-0.36477321204531,-0.339801867883332,
-0.316013676478843,-0.267491300050972,-0.237991136785178,-0.2348621134535,
-0.233311232442798,-0.232191145826705,-0.230999561446941,-0.229417613474607,
-0.227688461671877,-0.224791860166281,-0.206410607915776,-0.167801940267825,
-0.153709455984689,-0.139205909096901,-0.0764075034383618,-0.0727010087366635,
-0.0715135301317433,-0.0708595309664283,-0.0702092879277642,-0.0693876372283512,
-0.0685038164500342,-0.0670778526692987,-0.0642749993481048,-0.00095719944665948),
 .UNSPECIFIED.);
#822=B_SPLINE_CURVE_WITH_KNOTS('',3,(#41864,#41865,#41866,#41867,#41868,
#41869,#41870,#41871,#41872,#41873,#41874,#41875,#41876,#41877,#41878,#41879,
#41880,#41881,#41882,#41883,#41884,#41885,#41886,#41887,#41888,#41889,#41890,
#41891,#41892,#41893,#41894,#41895,#41896,#41897,#41898,#41899,#41900,#41901,
#41902,#41903,#41904,#41905,#41906,#41907,#41908,#41909,#41910,#41911,#41912,
#41913,#41914,#41915,#41916,#41917,#41918,#41919,#41920,#41921,#41922,#41923,
#41924,#41925,#41926,#41927,#41928,#41929,#41930,#41931,#41932,#41933,#41934,
#41935,#41936,#41937,#41938,#41939,#41940,#41941,#41942,#41943,#41944,#41945,
#41946,#41947,#41948,#41949,#41950,#41951,#41952,#41953,#41954,#41955,#41956,
#41957,#41958,#41959,#41960,#41961,#41962,#41963,#41964,#41965,#41966,#41967,
#41968,#41969,#41970,#41971,#41972,#41973,#41974,#41975,#41976,#41977,#41978,
#41979,#41980,#41981,#41982,#41983,#41984,#41985,#41986,#41987,#41988,#41989,
#41990,#41991,#41992,#41993,#41994,#41995,#41996,#41997,#41998,#41999,#42000,
#42001,#42002,#42003,#42004,#42005,#42006,#42007,#42008,#42009,#42010,#42011,
#42012,#42013,#42014,#42015,#42016,#42017,#42018,#42019,#42020,#42021,#42022,
#42023,#42024,#42025,#42026,#42027,#42028,#42029,#42030,#42031,#42032,#42033,
#42034,#42035,#42036,#42037,#42038,#42039,#42040,#42041,#42042,#42043,#42044,
#42045,#42046,#42047,#42048,#42049,#42050,#42051,#42052,#42053,#42054,#42055,
#42056,#42057,#42058,#42059,#42060,#42061,#42062,#42063,#42064,#42065,#42066,
#42067,#42068,#42069,#42070,#42071,#42072,#42073,#42074,#42075,#42076,#42077,
#42078,#42079,#42080,#42081,#42082,#42083,#42084,#42085,#42086,#42087,#42088,
#42089,#42090,#42091,#42092,#42093,#42094,#42095,#42096,#42097,#42098,#42099,
#42100,#42101,#42102,#42103,#42104,#42105,#42106,#42107,#42108,#42109,#42110,
#42111,#42112,#42113,#42114,#42115,#42116,#42117,#42118,#42119,#42120,#42121,
#42122,#42123,#42124,#42125,#42126,#42127,#42128,#42129,#42130,#42131,#42132,
#42133,#42134,#42135,#42136,#42137,#42138,#42139,#42140,#42141,#42142,#42143,
#42144,#42145,#42146,#42147,#42148,#42149,#42150,#42151,#42152,#42153,#42154,
#42155,#42156,#42157,#42158,#42159,#42160,#42161,#42162,#42163,#42164,#42165,
#42166,#42167,#42168,#42169,#42170,#42171,#42172,#42173,#42174,#42175,#42176,
#42177,#42178,#42179,#42180,#42181,#42182,#42183,#42184,#42185,#42186,#42187,
#42188,#42189,#42190,#42191,#42192,#42193,#42194,#42195,#42196,#42197,#42198,
#42199,#42200,#42201,#42202,#42203,#42204,#42205,#42206,#42207,#42208,#42209,
#42210,#42211,#42212,#42213,#42214,#42215,#42216,#42217,#42218,#42219,#42220,
#42221,#42222,#42223,#42224,#42225,#42226,#42227,#42228,#42229,#42230,#42231,
#42232,#42233,#42234,#42235,#42236,#42237,#42238,#42239,#42240,#42241,#42242,
#42243,#42244,#42245,#42246,#42247,#42248,#42249,#42250,#42251,#42252,#42253,
#42254,#42255,#42256,#42257,#42258,#42259,#42260,#42261,#42262,#42263,#42264,
#42265,#42266,#42267,#42268,#42269,#42270,#42271,#42272,#42273,#42274,#42275,
#42276,#42277,#42278,#42279,#42280,#42281,#42282,#42283,#42284,#42285,#42286,
#42287,#42288,#42289,#42290,#42291,#42292,#42293,#42294,#42295,#42296,#42297,
#42298,#42299,#42300,#42301,#42302,#42303,#42304,#42305,#42306,#42307,#42308,
#42309,#42310,#42311,#42312,#42313,#42314,#42315,#42316,#42317,#42318,#42319,
#42320,#42321,#42322,#42323,#42324,#42325,#42326,#42327,#42328,#42329,#42330,
#42331,#42332,#42333,#42334,#42335,#42336,#42337,#42338,#42339,#42340,#42341,
#42342,#42343,#42344,#42345,#42346,#42347,#42348,#42349,#42350,#42351,#42352,
#42353,#42354,#42355,#42356,#42357,#42358,#42359,#42360,#42361,#42362,#42363,
#42364,#42365,#42366,#42367,#42368,#42369,#42370,#42371,#42372,#42373,#42374,
#42375,#42376,#42377,#42378,#42379,#42380,#42381,#42382,#42383,#42384,#42385,
#42386,#42387,#42388,#42389,#42390,#42391,#42392,#42393,#42394,#42395,#42396,
#42397,#42398,#42399,#42400,#42401,#42402,#42403,#42404,#42405,#42406,#42407,
#42408,#42409,#42410,#42411,#42412,#42413),.UNSPECIFIED.,.F.,.F.,(4,2,2,
2,2,2,2,2,2,2,2,2,2,2,2,2,2,2,2,2,2,2,2,2,2,2,2,2,2,2,2,2,2,2,2,2,2,2,2,
2,2,2,2,2,2,2,2,2,2,2,2,2,2,2,2,2,2,2,2,2,2,2,2,2,2,2,2,2,2,2,2,2,2,2,2,
2,2,2,2,2,2,2,2,2,2,2,2,2,2,2,2,2,2,2,2,2,2,2,2,2,2,2,2,2,2,2,2,2,2,2,2,
2,2,2,2,2,2,2,2,2,2,2,2,2,2,2,2,2,2,2,2,2,2,2,2,2,2,2,2,2,2,2,2,2,2,2,2,
2,2,2,2,2,2,2,2,2,2,2,2,2,2,2,2,2,2,2,2,2,2,2,2,2,2,2,2,2,2,2,2,2,2,2,2,
2,2,2,2,2,2,2,2,2,2,2,2,2,2,2,2,2,2,2,2,2,2,2,2,2,2,2,2,2,2,2,2,2,2,2,2,
2,2,2,2,2,2,2,2,2,2,2,2,2,2,2,2,2,2,2,2,2,2,2,2,2,2,2,2,2,2,2,2,2,2,2,2,
2,2,2,2,2,2,2,2,2,2,2,2,2,2,2,2,2,2,2,4),(-4.06118295712417,-3.98211311604588,
-3.97644294279158,-3.97363861190561,-3.97194779832783,-3.97039356686888,
-3.96920630782604,-3.96807792437117,-3.96617799409728,-3.96115936628375,
-3.88063000612101,-3.86738208081769,-3.85530621393031,-3.82455397146885,
-3.81447091198009,-3.81022650951905,-3.80933937825198,-3.80867698975359,
-3.80800771516406,-3.80738693666036,-3.80653300532399,-3.8048270122616,
-3.78996955365318,-3.74420383960097,-3.71058124848428,-3.66945208894434,
-3.65783372939953,-3.65062812128208,-3.6485023565452,-3.64719852771346,
-3.646016239894,-3.64449911967408,-3.64137547730347,-3.62141062734092,-3.61584327457818,
-3.60996843848164,-3.56324438329713,-3.51729269495054,-3.48952380635042,
-3.48716796591025,-3.4864248372299,-3.48570321263414,-3.48504058017505,
-3.48417897362813,-3.48237097094483,-3.46921022854859,-3.46865148064511,
-3.42969023402925,-3.37730868182414,-3.35520199811677,-3.33028716769455,
-3.32687968901845,-3.32528588792883,-3.32409247509484,-3.32297583243125,
-3.32143785155262,-3.31753263986351,-3.25456046812247,-3.2030118460561,
-3.16975020542093,-3.16513981973647,-3.16390663852299,-3.16316425798306,
-3.1625065981479,-3.16166922071452,-3.15996563090189,-3.14967028922102,
-3.11975194399027,-3.05528580736834,-3.01238489575362,-3.00774493928961,
-3.00426724670723,-3.00266367227569,-3.00146864842984,-3.00035461527145,
-2.99882665741777,-2.99498052075771,-2.94185030915788,-2.86921429642131,
-2.84602740326167,-2.84230128704041,-2.84115732267686,-2.84043530822821,
-2.8397727183528,-2.83891171403643,-2.83710691366071,-2.82404061289285,
-2.82341841818583,-2.81554325220902,-2.73458895160555,-2.68987839994468,
-2.68270085362783,-2.68057876481697,-2.67927572959313,-2.67809320051751,
-2.67657442987716,-2.67344262427273,-2.65330016605262,-2.6474347849823,
-2.55816159860061,-2.52436800867107,-2.52128767476886,-2.5190533820556,
-2.51811762759138,-2.51744491812701,-2.51682827845283,-2.51599063521607,
-2.51434897543042,-2.50139846809973,-2.50069396172303,-2.50030745961547,
-2.49611419600537,-2.39974424935917,-2.36568378350806,-2.35958598376295,
-2.35760331310739,-2.35633135360042,-2.3551389493318,-2.35357869400014,
-2.35014368186173,-2.32199384286331,-2.29888025520422,-2.23652893784328,
-2.20171556484457,-2.19697265285033,-2.19572567293247,-2.19498584889564,
-2.19432772821767,-2.19348611110426,-2.19176136089304,-2.18104455412962,
-2.12971248022178,-2.08066028111303,-2.04350005525189,-2.03706571655508,
-2.03504246157936,-2.03376147465491,-2.03257245622639,-2.03103342476346,
-2.02771181533641,-1.98265141333053,-1.93173207378056,-1.89325120690849,
-1.89075578823583,-1.87546977624396,-1.8735604454921,-1.87269247641007,
-1.87202882472033,-1.87131007337671,-1.87015720271819,-1.86634745038487,
-1.80231610756,-1.73520862996575,-1.73050394039338,-1.71588025371117,-1.71332703843383,
-1.71178728240709,-1.71059818782047,-1.70931759750449,-1.70729598052919,
-1.7008751298571,-1.66383362274122,-1.61480484408027,-1.55509371647749,
-1.55154713338003,-1.55038059160043,-1.5497308394822,-1.54913936049699,
-1.54833819448639,-1.54681032248342,-1.53760121559862,-1.51867611163583,
-1.43242489056261,-1.41531919246473,-1.39376633022646,-1.39057272416088,
-1.38904182794259,-1.38785779492124,-1.3865610690264,-1.38446694909769,
-1.37754816629822,-1.33545229980823,-1.2486627014256,-1.24747675315554,
-1.23014820467172,-1.22817389191375,-1.227293935712,-1.22662829719309,-1.22591465705775,
-1.22480752906661,-1.22139152473007,-1.20131909365852,-1.18020668891759,
-1.11699025287132,-1.07200283660609,-1.06825850763392,-1.0667479787668,
-1.06563840473277,-1.06444029415,-1.06281875574569,-1.0592447868625,-1.05444598372259,
-1.00897857547919,-0.942659332969499,-0.930458760582793,-0.92756937748556,
-0.925593923114355,-0.924126266116316,-0.923102869098739,-0.922744752673963,
-0.918996009614837,-0.907196344752186,-0.905421716912551,-0.904570190128336,
-0.903910878779164,-0.903176643667838,-0.901979284361568,-0.897736699952111,
-0.890656098386216,-0.864007414556588,-0.814926569374454,-0.749708244432522,
-0.745711008230603,-0.744157569267698,-0.74303679961236,-0.741845567971649,
-0.740265923008089,-0.736931913235841,-0.710715145917066,-0.687631517090654,
-0.632997939871476,-0.585963303592128,-0.583250732446281,-0.582310204413956,
-0.581665798425558,-0.581073132881324,-0.580441933148174,-0.579647286269328,
-0.576769176761861,-0.551118626112138,-0.507552637445211,-0.42819069875983,
-0.423358545685806,-0.421488347259271,-0.420365659671687,-0.419175484552386,
-0.417602475056706,-0.415885694530514,-0.405890347343375,-0.388003491259941,
-0.349198859767511,-0.317635880389431,-0.274134685423581,-0.261926768880253,
-0.260312994489756,-0.259482565055744,-0.258867793410923,-0.258193538498627,
-0.257522546673939,-0.256612516479973,-0.251983468614956,-0.216101133322779,
-0.192485391147722,-0.163640355683076,-0.104291462426126,-0.100399528533765,
-0.0988637483901995,-0.0977476442925963,-0.0965538130989758,-0.0949577418306583,
-0.0932090108039047,-0.0902650433328994,-0.0842084620057397,-0.0681728321545726,
-0.000957725592193056),.UNSPECIFIED.);
#823=B_SPLINE_CURVE_WITH_KNOTS('',3,(#42415,#42416,#42417,#42418,#42419,
#42420,#42421,#42422,#42423,#42424,#42425),.UNSPECIFIED.,.F.,.F.,(4,1,1,
1,1,1,1,1,4),(317.30085801257,317.389884548341,318.388676952109,319.387469355877,
320.386261759645,321.385054163413,322.383846567181,323.382638970949,323.584043319749),
 .UNSPECIFIED.);
#824=B_SPLINE_CURVE_WITH_KNOTS('',3,(#42427,#42428,#42429,#42430,#42431,
#42432,#42433,#42434,#42435,#42436,#42437,#42438,#42439,#42440,#42441,#42442,
#42443,#42444,#42445,#42446,#42447,#42448,#42449,#42450,#42451,#42452,#42453,
#42454,#42455,#42456,#42457,#42458,#42459,#42460,#42461,#42462,#42463,#42464,
#42465,#42466,#42467,#42468,#42469,#42470,#42471,#42472,#42473,#42474,#42475,
#42476,#42477,#42478,#42479,#42480,#42481,#42482,#42483,#42484,#42485,#42486,
#42487,#42488,#42489,#42490,#42491,#42492,#42493,#42494,#42495,#42496,#42497,
#42498,#42499,#42500,#42501,#42502,#42503,#42504,#42505,#42506,#42507,#42508,
#42509,#42510,#42511,#42512,#42513,#42514,#42515,#42516,#42517,#42518,#42519,
#42520,#42521,#42522,#42523,#42524,#42525,#42526,#42527,#42528,#42529,#42530,
#42531,#42532,#42533,#42534,#42535,#42536,#42537,#42538,#42539,#42540,#42541,
#42542,#42543,#42544,#42545,#42546,#42547,#42548,#42549,#42550,#42551,#42552,
#42553,#42554,#42555,#42556,#42557,#42558,#42559,#42560,#42561,#42562,#42563,
#42564,#42565,#42566,#42567,#42568,#42569,#42570,#42571,#42572,#42573,#42574,
#42575,#42576,#42577,#42578,#42579,#42580,#42581,#42582,#42583,#42584,#42585,
#42586,#42587,#42588,#42589,#42590,#42591,#42592,#42593,#42594,#42595,#42596,
#42597,#42598,#42599,#42600,#42601,#42602,#42603,#42604,#42605,#42606,#42607,
#42608,#42609,#42610,#42611,#42612,#42613,#42614,#42615,#42616,#42617,#42618,
#42619,#42620,#42621,#42622,#42623,#42624,#42625,#42626,#42627,#42628,#42629,
#42630,#42631,#42632,#42633,#42634,#42635,#42636,#42637,#42638,#42639,#42640,
#42641,#42642,#42643,#42644,#42645,#42646,#42647,#42648,#42649,#42650,#42651,
#42652,#42653,#42654,#42655,#42656,#42657,#42658,#42659,#42660,#42661,#42662,
#42663,#42664,#42665,#42666,#42667,#42668,#42669,#42670,#42671,#42672,#42673,
#42674,#42675,#42676,#42677,#42678,#42679,#42680,#42681,#42682,#42683,#42684,
#42685,#42686,#42687,#42688,#42689,#42690,#42691,#42692,#42693,#42694,#42695,
#42696,#42697,#42698,#42699,#42700,#42701,#42702,#42703,#42704,#42705,#42706,
#42707,#42708,#42709,#42710,#42711,#42712,#42713,#42714,#42715,#42716,#42717,
#42718,#42719,#42720,#42721,#42722,#42723,#42724,#42725,#42726,#42727,#42728,
#42729,#42730,#42731,#42732,#42733,#42734,#42735,#42736,#42737,#42738,#42739,
#42740,#42741,#42742,#42743,#42744,#42745,#42746,#42747,#42748,#42749,#42750,
#42751,#42752,#42753,#42754,#42755,#42756,#42757,#42758,#42759,#42760,#42761,
#42762,#42763,#42764,#42765,#42766,#42767,#42768,#42769,#42770,#42771,#42772,
#42773,#42774,#42775,#42776,#42777,#42778,#42779,#42780,#42781,#42782,#42783,
#42784,#42785,#42786,#42787,#42788,#42789,#42790,#42791,#42792,#42793,#42794,
#42795,#42796,#42797,#42798,#42799,#42800,#42801,#42802,#42803,#42804,#42805,
#42806,#42807,#42808,#42809,#42810,#42811,#42812,#42813,#42814,#42815,#42816,
#42817,#42818,#42819,#42820,#42821,#42822,#42823,#42824,#42825,#42826,#42827,
#42828,#42829,#42830,#42831,#42832,#42833,#42834,#42835,#42836,#42837,#42838,
#42839,#42840,#42841,#42842,#42843,#42844,#42845,#42846,#42847,#42848,#42849,
#42850,#42851,#42852,#42853,#42854,#42855,#42856,#42857,#42858,#42859,#42860,
#42861,#42862,#42863,#42864,#42865,#42866,#42867,#42868,#42869,#42870,#42871,
#42872,#42873,#42874,#42875,#42876,#42877,#42878,#42879,#42880,#42881,#42882,
#42883,#42884,#42885,#42886,#42887,#42888,#42889,#42890,#42891,#42892,#42893,
#42894,#42895,#42896,#42897,#42898,#42899,#42900,#42901,#42902,#42903,#42904,
#42905,#42906,#42907,#42908,#42909,#42910,#42911,#42912,#42913,#42914,#42915,
#42916,#42917,#42918,#42919,#42920,#42921,#42922,#42923,#42924,#42925,#42926,
#42927,#42928,#42929,#42930,#42931,#42932,#42933,#42934,#42935,#42936,#42937,
#42938,#42939,#42940,#42941,#42942,#42943,#42944,#42945,#42946,#42947,#42948,
#42949,#42950,#42951,#42952,#42953,#42954,#42955,#42956),.UNSPECIFIED.,
 .F.,.F.,(4,2,2,2,2,2,2,2,2,2,2,2,2,2,2,2,2,2,2,2,2,2,2,2,2,2,2,2,2,2,2,
2,2,2,2,2,2,2,2,2,2,2,2,2,2,2,2,2,2,2,2,2,2,2,2,2,2,2,2,2,2,2,2,2,2,2,2,
2,2,2,2,2,2,2,2,2,2,2,2,2,2,2,2,2,2,2,2,2,2,2,2,2,2,2,2,2,2,2,2,2,2,2,2,
2,2,2,2,2,2,2,2,2,2,2,2,2,2,2,2,2,2,2,2,2,2,2,2,2,2,2,2,2,2,2,2,2,2,2,2,
2,2,2,2,2,2,2,2,2,2,2,2,2,2,2,2,2,2,2,2,2,2,2,2,2,2,2,2,2,2,2,2,2,2,2,2,
2,2,2,2,2,2,2,2,2,2,2,2,2,2,2,2,2,2,2,2,2,2,2,2,2,2,2,2,2,2,2,2,2,2,2,2,
2,2,2,2,2,2,2,2,2,2,2,2,2,2,2,2,2,2,2,2,2,2,2,2,2,2,2,2,2,2,2,2,2,2,2,2,
2,2,2,2,2,2,2,2,2,2,2,2,2,2,2,2,2,4),(-4.06040964561679,-3.98577442246086,
-3.93893319569508,-3.9315307619444,-3.92940168895388,-3.92809775376205,
-3.92691662965147,-3.92540275583632,-3.92229200046219,-3.90257088644096,
-3.80854396101611,-3.79058345342708,-3.77614413483332,-3.77141276241636,
-3.76830242735159,-3.76723576547339,-3.76662166886513,-3.765961860903,-3.76511742955535,
-3.76333047339507,-3.75122530414168,-3.71729793051633,-3.69565671967811,
-3.64961571939171,-3.61495714264574,-3.6087950177933,-3.60680522868895,
-3.60553221785033,-3.60434131197846,-3.60278658230598,-3.59937816776643,
-3.57201472591715,-3.49678407291162,-3.47205391189842,-3.45613517563977,
-3.44992047336824,-3.44736175308571,-3.4460274341408,-3.4448989989047,-3.44419210142687,
-3.44352991255855,-3.4426692674781,-3.44123370278448,-3.43287802978631,
-3.3399185899079,-3.29383985603283,-3.28650847633488,-3.28438664762852,
-3.28308424158774,-3.28190259224227,-3.28038538232006,-3.27725832681917,
-3.25718681962563,-3.25101149101381,-3.17609338625293,-3.15086311026694,
-3.12728564476051,-3.12477492318587,-3.12345880661998,-3.12234405295131,
-3.12163986945302,-3.12097682627877,-3.12011051114461,-3.1182082502366,
-3.10311080545929,-3.00442537761231,-2.96983933106461,-2.96368547108904,
-2.9616968538812,-2.96042421146976,-2.95923338098841,-2.95767836361995,
-2.95426775893715,-2.92682594871354,-2.83503539249743,-2.80534153389682,
-2.80247450732444,-2.80102512600825,-2.79981812317432,-2.7990932050262,
-2.79843559929225,-2.79759534769825,-2.79587583017119,-2.78524894509229,
-2.6931370875211,-2.65877949560347,-2.64246378499209,-2.63973639527301,
-2.63830114346262,-2.63724030887634,-2.63608969596705,-2.63442466387267,
-2.6297110584361,-2.62811991407275,-2.52474010105074,-2.49030118424195,
-2.47904559697547,-2.47743960454078,-2.47662238778397,-2.47596687480535,
-2.47521172356809,-2.47392844215611,-2.46925988115289,-2.37393859904464,
-2.32619141322845,-2.31870501775659,-2.31656710587581,-2.31526108047867,
-2.31408023243763,-2.31256971968188,-2.30947645091701,-2.29013697739414,
-2.28493573117174,-2.27611629161686,-2.1887148059889,-2.17291957383105,
-2.15664482164633,-2.15490741837159,-2.15406356422295,-2.15346683357274,
-2.15283644531442,-2.1519457702465,-2.14956516720639,-2.108146195482,-2.07607399590741,
-2.03133671541162,-2.02191906619643,-1.99818686477163,-1.99494780603417,
-1.99340194042678,-1.99221236630473,-1.99093542972142,-1.98892833855414,
-1.98262427865746,-1.94665812573461,-1.83923226976501,-1.83348353798078,
-1.8322204848993,-1.83140297849735,-1.83074726726674,-1.82999192575177,
-1.8286747316449,-1.82309156854107,-1.77159308623169,-1.70783689142447,
-1.70126442191182,-1.69538244522534,-1.67525894959784,-1.67212860612456,
-1.67061037662563,-1.66942819303013,-1.6681254615819,-1.66600369477159,
-1.65867822121284,-1.61266552303177,-1.51501325243428,-1.51057129171881,
-1.50929679781292,-1.50855086734493,-1.50795958401203,-1.50715994162477,
-1.50563907405082,-1.4965860742773,-1.47743806532743,-1.43000244982692,
-1.35459493606651,-1.35012229719897,-1.3484929716044,-1.34735181663008,
-1.34628771785427,-1.34485892334156,-1.34212911942674,-1.33869325129303,
-1.3130346889574,-1.2891507358596,-1.19233242586767,-1.18783485338364,-1.18655414538241,
-1.18580675807785,-1.18521555834548,-1.18441761175837,-1.18290509183925,
-1.17404021032996,-1.1551001465338,-1.10846474531658,-1.10004340279443,
-1.03131955522699,-1.02721989757726,-1.02564956978989,-1.02452430505125,
-1.0233353541832,-1.02180216717406,-1.01856922825714,-1.01433718830831,
-0.977638117205385,-0.925356260986364,-0.868347523858927,-0.867570238411694,
-0.864739352032805,-0.863675755516375,-0.863046517893452,-0.86244871110684,
-0.86159990118064,-0.859839112739079,-0.842394362771705,-0.822215862735034,
-0.741598431603388,-0.730184971472503,-0.707266364136139,-0.70434085591106,
-0.702841646923932,-0.701734963681853,-0.700534747465418,-0.698933818264108,
-0.695343560068391,-0.690528215521247,-0.678765413623159,-0.65567590209208,
-0.618355621546792,-0.586314657975289,-0.544537318760841,-0.541994009187242,
-0.541078719614582,-0.54044135733045,-0.53984674837383,-0.539019388178445,
-0.537365370906282,-0.524589923543127,-0.49879741296503,-0.490229440657184,
-0.483193161660451,-0.42812524813827,-0.409355732401675,-0.403959957494881,
-0.384471094233728,-0.381369253702139,-0.379856397854258,-0.378674557149575,
-0.377572948198401,-0.376291827866456,-0.372541553437571,-0.367454793507337,
-0.354788965616532,-0.316603940198361,-0.238251005602333,-0.221015515594709,
-0.219043797322051,-0.218164280125862,-0.217498681633816,-0.216784789800207,
-0.215653918492291,-0.212037136454894,-0.190171432233036,-0.113280126528247,
-0.106297187583923,-0.0907254957169124,-0.0622845918280095,-0.0588402204557976,
-0.0572781379280803,-0.0560853370877337,-0.0549850786347227,-0.05373861614479,
-0.0519987323967031,-0.0490762387654415,-0.000956587084948417),
 .UNSPECIFIED.);
#825=B_SPLINE_CURVE_WITH_KNOTS('',3,(#42958,#42959,#42960,#42961,#42962,
#42963,#42964,#42965,#42966,#42967,#42968,#42969,#42970,#42971,#42972,#42973,
#42974,#42975,#42976,#42977,#42978,#42979,#42980,#42981,#42982,#42983,#42984,
#42985,#42986,#42987,#42988,#42989,#42990,#42991,#42992,#42993,#42994,#42995,
#42996,#42997,#42998,#42999,#43000,#43001,#43002,#43003,#43004,#43005,#43006,
#43007,#43008,#43009,#43010,#43011,#43012,#43013,#43014,#43015,#43016,#43017,
#43018,#43019,#43020,#43021,#43022,#43023,#43024,#43025,#43026,#43027,#43028,
#43029,#43030,#43031,#43032,#43033,#43034,#43035,#43036,#43037,#43038,#43039,
#43040,#43041,#43042,#43043,#43044,#43045,#43046,#43047,#43048,#43049,#43050,
#43051,#43052,#43053,#43054,#43055,#43056,#43057,#43058,#43059,#43060,#43061,
#43062,#43063,#43064,#43065,#43066,#43067,#43068,#43069,#43070,#43071,#43072,
#43073,#43074,#43075,#43076,#43077,#43078,#43079,#43080,#43081,#43082,#43083,
#43084,#43085,#43086,#43087,#43088,#43089,#43090,#43091,#43092,#43093,#43094,
#43095,#43096,#43097,#43098,#43099,#43100,#43101,#43102,#43103,#43104,#43105,
#43106,#43107,#43108,#43109,#43110,#43111,#43112,#43113,#43114,#43115,#43116,
#43117,#43118,#43119,#43120,#43121,#43122,#43123,#43124,#43125,#43126,#43127,
#43128,#43129,#43130,#43131,#43132,#43133,#43134,#43135,#43136,#43137,#43138,
#43139,#43140,#43141,#43142,#43143,#43144,#43145,#43146,#43147,#43148,#43149,
#43150,#43151,#43152,#43153,#43154,#43155,#43156,#43157,#43158,#43159,#43160,
#43161,#43162,#43163,#43164,#43165,#43166,#43167,#43168,#43169,#43170,#43171,
#43172,#43173,#43174,#43175,#43176,#43177,#43178,#43179,#43180,#43181,#43182,
#43183,#43184,#43185,#43186,#43187,#43188,#43189,#43190,#43191,#43192,#43193,
#43194,#43195,#43196,#43197,#43198,#43199,#43200,#43201,#43202,#43203,#43204,
#43205,#43206,#43207,#43208,#43209,#43210,#43211,#43212,#43213,#43214,#43215,
#43216,#43217,#43218,#43219,#43220,#43221,#43222,#43223,#43224,#43225,#43226,
#43227,#43228,#43229,#43230,#43231,#43232,#43233,#43234,#43235,#43236,#43237,
#43238,#43239,#43240,#43241,#43242,#43243,#43244,#43245,#43246,#43247,#43248,
#43249,#43250,#43251,#43252,#43253,#43254,#43255,#43256,#43257,#43258,#43259,
#43260,#43261,#43262,#43263,#43264,#43265,#43266,#43267,#43268,#43269,#43270,
#43271,#43272,#43273,#43274,#43275,#43276,#43277,#43278,#43279,#43280,#43281,
#43282,#43283,#43284,#43285,#43286,#43287,#43288,#43289,#43290,#43291,#43292,
#43293,#43294,#43295,#43296,#43297,#43298,#43299,#43300,#43301,#43302,#43303,
#43304,#43305,#43306,#43307,#43308,#43309,#43310,#43311,#43312,#43313,#43314,
#43315,#43316,#43317,#43318,#43319,#43320,#43321,#43322,#43323,#43324,#43325,
#43326,#43327,#43328,#43329,#43330,#43331,#43332,#43333,#43334,#43335,#43336,
#43337,#43338,#43339,#43340,#43341,#43342,#43343,#43344,#43345,#43346,#43347,
#43348,#43349,#43350,#43351,#43352,#43353,#43354,#43355,#43356,#43357,#43358,
#43359,#43360,#43361,#43362,#43363,#43364,#43365,#43366,#43367,#43368,#43369,
#43370,#43371,#43372,#43373,#43374,#43375,#43376,#43377,#43378,#43379,#43380,
#43381,#43382,#43383,#43384,#43385,#43386,#43387,#43388,#43389,#43390,#43391,
#43392,#43393,#43394,#43395,#43396,#43397,#43398,#43399,#43400,#43401,#43402,
#43403,#43404,#43405,#43406,#43407,#43408,#43409,#43410,#43411,#43412,#43413,
#43414,#43415,#43416,#43417,#43418,#43419,#43420,#43421,#43422,#43423,#43424,
#43425,#43426,#43427,#43428,#43429,#43430,#43431,#43432,#43433,#43434,#43435,
#43436,#43437,#43438,#43439,#43440,#43441,#43442,#43443,#43444,#43445,#43446,
#43447,#43448,#43449,#43450,#43451,#43452,#43453,#43454,#43455,#43456,#43457,
#43458,#43459,#43460,#43461,#43462,#43463,#43464,#43465,#43466,#43467,#43468,
#43469,#43470,#43471,#43472,#43473,#43474,#43475,#43476,#43477,#43478,#43479,
#43480,#43481),.UNSPECIFIED.,.F.,.F.,(4,2,2,2,2,2,2,2,2,2,2,2,2,2,2,2,2,
2,2,2,2,2,2,2,2,2,2,2,2,2,2,2,2,2,2,2,2,2,2,2,2,2,2,2,2,2,2,2,2,2,2,2,2,
2,2,2,2,2,2,2,2,2,2,2,2,2,2,2,2,2,2,2,2,2,2,2,2,2,2,2,2,2,2,2,2,2,2,2,2,
2,2,2,2,2,2,2,2,2,2,2,2,2,2,2,2,2,2,2,2,2,2,2,2,2,2,2,2,2,2,2,2,2,2,2,2,
2,2,2,2,2,2,2,2,2,2,2,2,2,2,2,2,2,2,2,2,2,2,2,2,2,2,2,2,2,2,2,2,2,2,2,2,
2,2,2,2,2,2,2,2,2,2,2,2,2,2,2,2,2,2,2,2,2,2,2,2,2,2,2,2,2,2,2,2,2,2,2,2,
2,2,2,2,2,2,2,2,2,2,2,2,2,2,2,2,2,2,2,2,2,2,2,2,2,2,2,2,2,2,2,2,2,2,2,2,
2,2,2,2,2,2,2,2,2,2,2,2,2,2,2,2,2,2,2,2,2,2,2,2,2,2,2,2,4),(-4.0602155392693,
-3.99823060173568,-3.96839489076751,-3.9570393989674,-3.95542940171613,
-3.95461110461063,-3.95395520086939,-3.95320013103987,-3.95191821573228,
-3.94726674682146,-3.85267067305009,-3.83142314384518,-3.79931803791138,
-3.79556874229651,-3.79428634359585,-3.79318479384265,-3.79200350565062,
-3.79049378420746,-3.78740688070022,-3.76822690106404,-3.76312316617948,
-3.74464537484264,-3.70635129238098,-3.67255223568283,-3.63843561254961,
-3.63374434705983,-3.63250222505594,-3.63176356148629,-3.63110534927944,
-3.63026210267512,-3.6285287751609,-3.61763370621091,-3.54354528604912,
-3.50514756935874,-3.48538627545259,-3.47462063049694,-3.4722087301611,
-3.47106977239965,-3.4700019387804,-3.46887210927611,-3.4672841875383,-3.46400501857127,
-3.42823187279132,-3.34993742083824,-3.31580192115324,-3.31110912856822,
-3.30986682046659,-3.30912808934533,-3.30846984511238,-3.30762659541212,
-3.30589339318106,-3.29500227145687,-3.20295867582908,-3.16872443801467,
-3.15800831240741,-3.1535147257588,-3.15114961814424,-3.14920452771105,
-3.14792185507935,-3.14674096702465,-3.14523417638961,-3.14226335011876,
-3.12465409572201,-3.12107470177142,-3.02537247551533,-2.99942481964225,
-2.98892164373728,-2.98734168212667,-2.98652961066877,-2.98593697225873,
-2.98529280508737,-2.98435297842529,-2.98164480407284,-2.93402020877064,
-2.87153303115491,-2.83479784545156,-2.83056315754493,-2.82733018007156,
-2.82579604960904,-2.82467120212098,-2.82355841583567,-2.82203515693363,
-2.81821636357285,-2.76779774313479,-2.70486907523802,-2.66706070469614,
-2.66497908350776,-2.66407005491187,-2.66340219690131,-2.66277928574838,
-2.66191729167346,-2.65971394732196,-2.6293191856938,-2.54885957167821,
-2.52560834887318,-2.50718662003834,-2.50437234604507,-2.5029182682703,
-2.50185463610962,-2.50071165429682,-2.49907579122292,-2.49456056198429,
-2.41870805169403,-2.37152835481226,-2.35244886586808,-2.34349443308676,
-2.34197795363165,-2.34117922214147,-2.34053058543046,-2.3398636071348,
-2.33861153909123,-2.33436964322727,-2.25983583946856,-2.18546836497904,
-2.18200242797144,-2.18041940391096,-2.17922779848189,-2.17810826924329,
-2.17625390127099,-2.17151779012193,-2.09757404088505,-2.04947672295402,
-2.03045394643723,-2.02099913170587,-2.01936050304138,-2.01852513816433,
-2.01786773140263,-2.01712419855575,-2.01586044975354,-2.01092901556941,
-1.98760098772583,-1.94092169293096,-1.86477752126815,-1.86000075050033,
-1.8581397283213,-1.85701892521598,-1.85582802666224,-1.85424944927688,
-1.8508071877283,-1.78549054557636,-1.70202201451824,-1.69760055350719,
-1.69632824704829,-1.69558276073249,-1.69499135181605,-1.6941909267222,
-1.69266657501858,-1.68353762834365,-1.66441984611714,-1.61690988530063,
-1.54158321115397,-1.53713227783861,-1.53550619126619,-1.53436586014014,
-1.53330138411472,-1.53184103407294,-1.52899688879344,-1.50976124773764,
-1.49997146723766,-1.47605987209602,-1.39206049736505,-1.38887298287399,
-1.38725079395284,-1.3757140981856,-1.37395113771415,-1.37310190208313,
-1.37244286177031,-1.37170734109236,-1.37047974725895,-1.36604254428399,
-1.33499202393868,-1.24773502753606,-1.24132309248633,-1.23608079615596,
-1.21672852472928,-1.21363317555186,-1.21212164977253,-1.21094001105244,
-1.20963311243577,-1.20753652026161,-1.20041761092466,-1.15627423956649,
-1.09265468754004,-1.06323654697815,-1.05291665787788,-1.05121179448688,
-1.0503741486475,-1.04971644688079,-1.04897419907327,-1.0477164148588,-1.04297989480434,
-1.00801005710205,-0.941688168879405,-0.929280981215799,-0.894878741849937,
-0.891268479386463,-0.889819639711263,-0.888615961189213,-0.887385749087742,
-0.886153129845173,-0.882874298809824,-0.861188705103079,-0.82590504431776,
-0.78176496033359,-0.744246958058379,-0.743702717531739,-0.73051609918907,
-0.728707054836243,-0.727845220868044,-0.727182535586847,-0.726460979473548,
-0.725295534527965,-0.721462390562413,-0.715266492935087,-0.698177037992769,
-0.634445914960613,-0.572797638557261,-0.568896077388422,-0.567358727415494,
-0.566242260934364,-0.565048772174144,-0.563877895180517,-0.561331822488007,
-0.547162298058298,-0.518801594335806,-0.477093344383485,-0.410757078412684,
-0.406824343885069,-0.405608733818244,-0.404949085388673,-0.404293456647265,
-0.403479401099224,-0.402606132987589,-0.398586629346373,-0.391992691841185,
-0.368965929448184,-0.342948439432188,-0.316568198202258,-0.282648837701999,
-0.272301123937339,-0.2491590419796,-0.246225282132891,-0.244723946205397,
-0.243616718716812,-0.242416901452655,-0.24123452570869,-0.239660963587682,
-0.237137319333108,-0.219061549673271,-0.186160493229908,-0.174139202419186,
-0.160956235357465,-0.0881422054516073,-0.0842268030630355,-0.0830132382568326,
-0.0823539636508675,-0.0816982199509651,-0.0808833068662808,-0.0800088694986765,
-0.0786053941585817,-0.0758631083913248,-0.000957591977515441),
 .UNSPECIFIED.);
#826=B_SPLINE_CURVE_WITH_KNOTS('',3,(#43483,#43484,#43485,#43486,#43487,
#43488,#43489,#43490,#43491,#43492,#43493,#43494,#43495,#43496,#43497,#43498,
#43499,#43500,#43501,#43502,#43503,#43504,#43505,#43506,#43507,#43508,#43509,
#43510,#43511,#43512,#43513,#43514,#43515,#43516,#43517,#43518,#43519,#43520,
#43521,#43522,#43523,#43524,#43525,#43526,#43527,#43528,#43529,#43530,#43531,
#43532,#43533,#43534,#43535,#43536,#43537,#43538,#43539,#43540,#43541,#43542,
#43543,#43544,#43545,#43546,#43547,#43548,#43549,#43550,#43551,#43552,#43553,
#43554,#43555,#43556,#43557,#43558,#43559,#43560,#43561,#43562,#43563,#43564,
#43565,#43566,#43567,#43568,#43569,#43570,#43571,#43572,#43573,#43574,#43575,
#43576,#43577,#43578,#43579,#43580,#43581,#43582,#43583,#43584,#43585,#43586,
#43587,#43588,#43589,#43590,#43591,#43592,#43593,#43594,#43595,#43596,#43597,
#43598,#43599,#43600,#43601,#43602,#43603,#43604,#43605,#43606,#43607,#43608,
#43609,#43610,#43611,#43612,#43613,#43614,#43615,#43616,#43617,#43618,#43619,
#43620,#43621,#43622,#43623,#43624,#43625,#43626,#43627,#43628,#43629,#43630,
#43631,#43632,#43633,#43634,#43635,#43636,#43637,#43638,#43639,#43640,#43641,
#43642,#43643,#43644,#43645,#43646,#43647,#43648,#43649,#43650,#43651,#43652,
#43653,#43654,#43655,#43656,#43657,#43658,#43659,#43660,#43661,#43662,#43663,
#43664,#43665,#43666,#43667,#43668,#43669,#43670,#43671,#43672,#43673,#43674,
#43675,#43676,#43677,#43678,#43679,#43680,#43681,#43682,#43683,#43684,#43685,
#43686,#43687,#43688,#43689,#43690,#43691,#43692,#43693,#43694,#43695,#43696,
#43697,#43698,#43699,#43700,#43701,#43702,#43703,#43704,#43705,#43706,#43707,
#43708,#43709,#43710,#43711,#43712,#43713,#43714,#43715,#43716,#43717,#43718,
#43719,#43720,#43721,#43722,#43723,#43724,#43725,#43726,#43727,#43728,#43729,
#43730,#43731,#43732,#43733,#43734,#43735,#43736,#43737,#43738,#43739,#43740,
#43741,#43742,#43743,#43744,#43745,#43746,#43747,#43748,#43749,#43750,#43751,
#43752,#43753,#43754,#43755,#43756,#43757,#43758,#43759,#43760,#43761,#43762,
#43763,#43764,#43765,#43766,#43767,#43768,#43769,#43770,#43771,#43772,#43773,
#43774,#43775,#43776,#43777,#43778,#43779,#43780,#43781,#43782,#43783,#43784,
#43785,#43786,#43787,#43788,#43789,#43790,#43791,#43792,#43793,#43794,#43795,
#43796,#43797,#43798,#43799,#43800,#43801,#43802,#43803,#43804,#43805,#43806,
#43807,#43808,#43809,#43810,#43811,#43812,#43813,#43814,#43815,#43816,#43817,
#43818,#43819,#43820,#43821,#43822,#43823,#43824,#43825,#43826,#43827,#43828,
#43829,#43830,#43831,#43832,#43833,#43834,#43835,#43836,#43837,#43838,#43839,
#43840,#43841,#43842,#43843,#43844,#43845,#43846,#43847,#43848,#43849,#43850,
#43851,#43852,#43853,#43854,#43855,#43856,#43857,#43858,#43859,#43860,#43861,
#43862,#43863,#43864,#43865,#43866,#43867,#43868,#43869,#43870,#43871,#43872,
#43873,#43874,#43875,#43876,#43877,#43878,#43879,#43880,#43881,#43882,#43883,
#43884,#43885,#43886,#43887,#43888,#43889,#43890,#43891,#43892,#43893,#43894,
#43895,#43896,#43897,#43898,#43899,#43900,#43901,#43902,#43903,#43904,#43905,
#43906,#43907,#43908,#43909,#43910,#43911,#43912,#43913,#43914,#43915,#43916,
#43917,#43918,#43919,#43920,#43921,#43922,#43923,#43924,#43925,#43926,#43927,
#43928,#43929,#43930,#43931,#43932,#43933,#43934,#43935,#43936,#43937,#43938,
#43939,#43940,#43941,#43942,#43943,#43944,#43945,#43946,#43947,#43948,#43949,
#43950,#43951,#43952,#43953,#43954,#43955,#43956,#43957,#43958,#43959,#43960,
#43961,#43962,#43963,#43964,#43965,#43966,#43967,#43968,#43969,#43970,#43971,
#43972,#43973,#43974,#43975,#43976,#43977,#43978,#43979,#43980,#43981,#43982,
#43983,#43984,#43985,#43986,#43987,#43988,#43989,#43990,#43991,#43992,#43993,
#43994,#43995,#43996,#43997,#43998,#43999,#44000,#44001,#44002,#44003,#44004,
#44005,#44006,#44007,#44008,#44009,#44010,#44011,#44012,#44013,#44014,#44015,
#44016,#44017,#44018,#44019,#44020,#44021,#44022),.UNSPECIFIED.,.F.,.F.,
(4,2,2,2,2,2,2,2,2,2,2,2,2,2,2,2,2,2,2,2,2,2,2,2,2,2,2,2,2,2,2,2,2,2,2,
2,2,2,2,2,2,2,2,2,2,2,2,2,2,2,2,2,2,2,2,2,2,2,2,2,2,2,2,2,2,2,2,2,2,2,2,
2,2,2,2,2,2,2,2,2,2,2,2,2,2,2,2,2,2,2,2,2,2,2,2,2,2,2,2,2,2,2,2,2,2,2,2,
2,2,2,2,2,2,2,2,2,2,2,2,2,2,2,2,2,2,2,2,2,2,2,2,2,2,2,2,2,2,2,2,2,2,2,2,
2,2,2,2,2,2,2,2,2,2,2,2,2,2,2,2,2,2,2,2,2,2,2,2,2,2,2,2,2,2,2,2,2,2,2,2,
2,2,2,2,2,2,2,2,2,2,2,2,2,2,2,2,2,2,2,2,2,2,2,2,2,2,2,2,2,2,2,2,2,2,2,2,
2,2,2,2,2,2,2,2,2,2,2,2,2,2,2,2,2,2,2,2,2,2,2,2,2,2,2,2,2,2,2,2,2,2,2,2,
2,2,2,2,2,2,2,2,2,2,2,2,2,2,2,2,2,2,4),(-4.06122042211378,-3.98730337121336,
-3.98478298796875,-3.98321096509116,-3.9817426771538,-3.98067739930817,
-3.97954090655895,-3.97792812220703,-3.97356141876023,-3.90239136750869,
-3.88744857196921,-3.87338246909838,-3.83815753939089,-3.82315510258274,
-3.8217559239748,-3.82088339969083,-3.820069942818,-3.81941453579877,-3.81875488824774,
-3.81753866236554,-3.81359905183284,-3.74561337849167,-3.71806506483374,
-3.68218021724648,-3.66982917492818,-3.66227714388483,-3.66069270293434,
-3.65921543834216,-3.65814892068119,-3.65701602956684,-3.65541648733755,
-3.65113256754568,-3.58453589773527,-3.53280112881335,-3.50307982617067,
-3.49917624551057,-3.49831109495267,-3.49750292936578,-3.49691085238028,
-3.49626501258054,-3.49511732416295,-3.49171187607518,-3.43500939814268,
-3.39559396279255,-3.35772012967898,-3.34081249585685,-3.33806787342071,
-3.33689489079826,-3.33570039657015,-3.33458625774305,-3.33305722018905,
-3.32920349293516,-3.27517438759,-3.22009809872474,-3.19939260063911,-3.18134519051984,
-3.17682314732775,-3.17556114273915,-3.17481807792218,-3.17416072589412,
-3.17332495577946,-3.17162875370144,-3.16147761245603,-3.15818554928967,
-3.13276854286616,-3.08213645610593,-3.04171154835074,-3.01938446255512,
-3.01596083833761,-3.01436766540178,-3.01317455093995,-3.01205806258737,
-3.01052009807253,-3.00661389087386,-2.9425802188186,-2.85783054741572,
-2.85401482038519,-2.85284841101573,-2.85212667964196,-2.85146412986671,
-2.85060287768581,-2.84879649434053,-2.8356755135456,-2.83261639571709,
-2.8294418849335,-2.82821064920523,-2.81567553258686,-2.73974766712154,
-2.70089663279329,-2.69651971096086,-2.6931967079389,-2.69162638755515,
-2.69043677664342,-2.68931353249669,-2.68743983348207,-2.68258497771407,
-2.67587768014566,-2.67356927017684,-2.67110782495242,-2.57183333383073,
-2.53622755813954,-2.5314277913914,-2.5301756442988,-2.52943465357279,-2.52877672603962,
-2.52793700419617,-2.5266023638827,-2.51988537181546,-2.51947214958272,
-2.41772564013066,-2.37403572369145,-2.37041209038707,-2.36879996069456,
-2.3676035913794,-2.36649190689406,-2.36497275570634,-2.36117765877328,
-2.31255583175956,-2.28650709652996,-2.23637804959072,-2.21781326933854,
-2.20913098770327,-2.20762715014145,-2.20683113650648,-2.20624021316018,
-2.20558776706399,-2.20440761635382,-2.20075624521831,-2.14050161171187,
-2.09175191631063,-2.06844345436592,-2.05019943743177,-2.04739195426642,
-2.04593932268583,-2.04477443514057,-2.04343476415978,-2.04114844799486,
-2.03319218162742,-2.03124545084192,-2.01389769449877,-1.9913965784436,
-1.89996390509604,-1.8869704300372,-1.88532734585329,-1.88448936729588,
-1.88387266975754,-1.88320009159846,-1.88226486030631,-1.88003341010227,
-1.87695807918521,-1.84327045884236,-1.75800399175919,-1.72848354193204,
-1.72535415684697,-1.72380324491251,-1.72268320532421,-1.72149173535969,
-1.71991004888465,-1.71645165664784,-1.6457963850695,-1.57544824360086,
-1.56410033746409,-1.56234596674019,-1.56149844354663,-1.56083962454671,
-1.56010317742488,-1.55887138016999,-1.55429274431194,-1.52166277449236,
-1.43836967100109,-1.43087542000263,-1.42524780827744,-1.40519956296268,
-1.40207204850946,-1.40055414024952,-1.39937173203908,-1.398068271477,-1.39594423441197,
-1.38860051188451,-1.34240265391867,-1.26300660503229,-1.25535542778925,
-1.25495320468321,-1.25373684375561,-1.24143474105209,-1.23981679469797,
-1.23898526413092,-1.23837019057029,-1.23769613931494,-1.23677211008846,
-1.23460662059235,-1.23161136531513,-1.19952162699187,-1.13704526953143,
-1.08369366942478,-1.07984521221592,-1.07831679637746,-1.07720259212926,
-1.07600753849208,-1.07440419299453,-1.07082946946612,-1.02317867966916,
-0.94435449843721,-0.936115112965031,-0.918981701666313,-0.917013651069756,
-0.91613479335376,-0.915469295708838,-0.914855791275076,-0.913835631132868,
-0.911054556891232,-0.906957898634397,-0.821252614542162,-0.760959494831596,
-0.757062876779412,-0.75552627607693,-0.754409934935059,-0.753216187307075,
-0.751620808957072,-0.748089328074736,-0.696225977430358,-0.633654586601938,
-0.618594202933411,-0.612365763547671,-0.609432652356723,-0.608021727178315,
-0.595946880155507,-0.594160278029042,-0.593315538340491,-0.592655278393957,
-0.592040705716364,-0.590972788021841,-0.587873645667218,-0.583157999019995,
-0.568790227843729,-0.527324513288269,-0.45733008687709,-0.452320031875047,
-0.43666565197809,-0.434055745011115,-0.432499174284159,-0.431307309032712,
-0.430033711634002,-0.428043914507691,-0.421888832961478,-0.387303638297796,
-0.3511214309649,-0.317569991591704,-0.274702820330594,-0.2719968592842,
-0.271057308472001,-0.270413186513801,-0.269820472695677,-0.269189143689019,
-0.268394019388826,-0.265462270474878,-0.234321212494021,-0.213785909967768,
-0.152702400364498,-0.139501408467639,-0.134046470652641,-0.114406872628747,
-0.111297993682692,-0.109783727919976,-0.108601705146172,-0.107296173994659,
-0.105163130596233,-0.0977335934131149,-0.0506185946559123,-0.000958062894794184),
 .UNSPECIFIED.);
#827=B_SPLINE_CURVE_WITH_KNOTS('',3,(#44024,#44025,#44026,#44027,#44028,
#44029,#44030,#44031,#44032,#44033,#44034,#44035,#44036,#44037,#44038,#44039,
#44040,#44041,#44042,#44043,#44044,#44045,#44046,#44047,#44048,#44049,#44050,
#44051,#44052,#44053,#44054,#44055,#44056,#44057,#44058,#44059,#44060,#44061,
#44062,#44063,#44064,#44065,#44066,#44067,#44068,#44069,#44070,#44071,#44072,
#44073,#44074,#44075,#44076,#44077,#44078,#44079,#44080,#44081,#44082,#44083,
#44084,#44085,#44086,#44087,#44088,#44089,#44090,#44091,#44092,#44093,#44094,
#44095,#44096,#44097,#44098,#44099,#44100,#44101,#44102,#44103,#44104,#44105,
#44106,#44107,#44108,#44109,#44110,#44111,#44112,#44113,#44114,#44115,#44116,
#44117,#44118,#44119,#44120,#44121,#44122,#44123,#44124,#44125,#44126,#44127,
#44128,#44129,#44130,#44131,#44132,#44133,#44134,#44135,#44136,#44137,#44138,
#44139,#44140,#44141,#44142,#44143,#44144,#44145,#44146,#44147,#44148,#44149,
#44150,#44151,#44152,#44153,#44154,#44155,#44156,#44157,#44158,#44159,#44160,
#44161,#44162,#44163,#44164,#44165,#44166,#44167,#44168,#44169,#44170,#44171,
#44172,#44173,#44174,#44175,#44176,#44177,#44178,#44179,#44180,#44181,#44182,
#44183,#44184,#44185,#44186,#44187,#44188,#44189,#44190,#44191,#44192,#44193,
#44194,#44195,#44196,#44197,#44198,#44199,#44200,#44201,#44202,#44203,#44204,
#44205,#44206,#44207,#44208,#44209,#44210,#44211,#44212,#44213,#44214,#44215,
#44216,#44217,#44218,#44219,#44220,#44221,#44222,#44223,#44224,#44225,#44226,
#44227,#44228,#44229,#44230,#44231,#44232,#44233,#44234,#44235,#44236,#44237,
#44238,#44239,#44240,#44241,#44242,#44243,#44244,#44245,#44246,#44247,#44248,
#44249,#44250,#44251,#44252,#44253,#44254,#44255,#44256,#44257,#44258,#44259,
#44260,#44261,#44262,#44263,#44264,#44265,#44266,#44267,#44268,#44269,#44270,
#44271,#44272,#44273,#44274,#44275,#44276,#44277,#44278,#44279,#44280,#44281,
#44282,#44283,#44284,#44285,#44286,#44287,#44288,#44289,#44290,#44291,#44292,
#44293,#44294,#44295,#44296,#44297,#44298,#44299,#44300,#44301,#44302,#44303,
#44304,#44305,#44306,#44307,#44308,#44309,#44310,#44311,#44312,#44313,#44314,
#44315,#44316,#44317,#44318,#44319,#44320,#44321,#44322,#44323,#44324,#44325,
#44326,#44327,#44328,#44329,#44330,#44331,#44332,#44333,#44334,#44335,#44336,
#44337,#44338,#44339,#44340,#44341,#44342,#44343,#44344,#44345,#44346,#44347,
#44348,#44349,#44350,#44351,#44352,#44353,#44354,#44355,#44356,#44357,#44358,
#44359,#44360,#44361,#44362,#44363,#44364,#44365,#44366,#44367,#44368,#44369,
#44370,#44371,#44372,#44373,#44374,#44375,#44376,#44377,#44378,#44379,#44380,
#44381,#44382,#44383,#44384,#44385,#44386,#44387,#44388,#44389,#44390,#44391,
#44392,#44393,#44394,#44395,#44396,#44397,#44398,#44399,#44400,#44401,#44402,
#44403,#44404,#44405,#44406,#44407,#44408,#44409,#44410,#44411,#44412,#44413,
#44414,#44415,#44416,#44417,#44418,#44419,#44420,#44421,#44422,#44423,#44424,
#44425,#44426,#44427,#44428,#44429,#44430,#44431,#44432,#44433,#44434,#44435,
#44436,#44437,#44438,#44439,#44440,#44441,#44442,#44443,#44444,#44445,#44446,
#44447,#44448,#44449,#44450,#44451,#44452,#44453,#44454,#44455,#44456,#44457,
#44458,#44459,#44460,#44461,#44462,#44463,#44464,#44465,#44466,#44467,#44468,
#44469,#44470,#44471,#44472,#44473,#44474,#44475,#44476,#44477,#44478,#44479,
#44480,#44481,#44482,#44483,#44484,#44485,#44486,#44487,#44488,#44489,#44490,
#44491,#44492,#44493,#44494,#44495,#44496,#44497,#44498,#44499,#44500,#44501,
#44502,#44503,#44504,#44505,#44506,#44507,#44508,#44509,#44510,#44511,#44512,
#44513,#44514,#44515,#44516,#44517,#44518,#44519,#44520,#44521,#44522,#44523,
#44524,#44525,#44526,#44527,#44528,#44529,#44530,#44531,#44532,#44533,#44534,
#44535,#44536,#44537,#44538,#44539,#44540,#44541,#44542,#44543,#44544,#44545,
#44546,#44547,#44548,#44549,#44550,#44551,#44552,#44553,#44554,#44555,#44556,
#44557),.UNSPECIFIED.,.F.,.F.,(4,2,2,2,2,2,2,2,2,2,2,2,2,2,2,2,2,2,2,2,
2,2,2,2,2,2,2,2,2,2,2,2,2,2,2,2,2,2,2,2,2,2,2,2,2,2,2,2,2,2,2,2,2,2,2,2,
2,2,2,2,2,2,2,2,2,2,2,2,2,2,2,2,2,2,2,2,2,2,2,2,2,2,2,2,2,2,2,2,2,2,2,2,
2,2,2,2,2,2,2,2,2,2,2,2,2,2,2,2,2,2,2,2,2,2,2,2,2,2,2,2,2,2,2,2,2,2,2,2,
2,2,2,2,2,2,2,2,2,2,2,2,2,2,2,2,2,2,2,2,2,2,2,2,2,2,2,2,2,2,2,2,2,2,2,2,
2,2,2,2,2,2,2,2,2,2,2,2,2,2,2,2,2,2,2,2,2,2,2,2,2,2,2,2,2,2,2,2,2,2,2,2,
2,2,2,2,2,2,2,2,2,2,2,2,2,2,2,2,2,2,2,2,2,2,2,2,2,2,2,2,2,2,2,2,2,2,2,2,
2,2,2,2,2,2,2,2,2,2,2,2,2,2,2,2,2,2,2,2,2,2,2,2,2,2,2,2,2,2,4),(-4.05973415353602,
-4.01165008765246,-4.00941701345505,-4.00820757326979,-4.00741466348188,
-4.00678423325295,-4.00619211720911,-4.00554748056146,-4.00460522964405,
-4.00187830154151,-3.953499761186,-3.9407436132943,-3.92894404673932,-3.90389673324836,
-3.85647816948271,-3.84902159477275,-3.84688660388739,-3.84558114606902,
-3.84440001653371,-3.84288804216987,-3.83978790765343,-3.82030680562777,
-3.81856999517357,-3.74357053098659,-3.70602312480943,-3.69306381939591,
-3.68868923990147,-3.68576254376805,-3.68497012177565,-3.68433980616281,
-3.68374771774191,-3.68310274248955,-3.6821593771321,-3.67942501539386,
-3.6354928188547,-3.58335735510639,-3.57536856879101,-3.54428219867686,
-3.52765264463386,-3.52491120482614,-3.52347279545918,-3.52241141106925,
-3.52126193496572,-3.51960153076107,-3.51492048885988,-3.43608850068325,
-3.39839813611484,-3.37730850941143,-3.36439194251438,-3.36273991838272,
-3.36207266482662,-3.36140074222927,-3.36078400597841,-3.35994505488879,
-3.35787425309426,-3.33500100197902,-3.3225115932881,-3.25775013710391,
-3.21138978858522,-3.20403133177031,-3.20190640750415,-3.20060314457192,
-3.19942140299544,-3.19790502983747,-3.19478308919397,-3.17483339903091,
-3.16833847387493,-3.12544874744067,-3.06951526246094,-3.0449270624279,
-3.04235441627532,-3.04043585084003,-3.03955861285647,-3.03889330104224,
-3.03826699813792,-3.03739156536359,-3.03559870241415,-3.01766680112572,
-3.01043924554607,-2.92127555932061,-2.88730218082688,-2.88121531380936,
-2.87923468500324,-2.87796364647946,-2.87677182961388,-2.87521194533933,
-2.87177613125532,-2.84355473352583,-2.82514131656146,-2.75616139052032,
-2.73702073731538,-2.7212607474561,-2.71926564682063,-2.71770178154918,
-2.71689695755096,-2.71630342083122,-2.71566405735846,-2.71454807610885,
-2.71136852971746,-2.65750448828532,-2.56470146473298,-2.55864349571014,
-2.55666653453603,-2.55539636993102,-2.55420432076727,-2.55264261500176,
-2.54919659398856,-2.52064032476493,-2.428239838504,-2.40013784496887,-2.39735922975404,
-2.39530113304027,-2.39439658872299,-2.39372974887369,-2.39310607413245,
-2.39224045303626,-2.39001417403211,-2.35786194069184,-2.32326723923747,
-2.29119389622761,-2.25429315592853,-2.2375637856402,-2.23481804435973,
-2.2333787099457,-2.23231720291208,-2.23116813713329,-2.22950925883561,
-2.22483858503327,-2.1504415040563,-2.10257062196525,-2.07735925641474,
-2.07342143193023,-2.07225479566735,-2.07153317836553,-2.07087091220759,
-2.07001027293374,-2.06820604071313,-2.05512824558456,-2.052648969683,-2.0522565185369,
-2.04549023016851,-2.0314480931122,-1.9437020134791,-1.91604838355523,-1.91263035985199,
-1.91107373796341,-1.9098824165392,-1.90860996703368,-1.906623135393,-1.900486315262,
-1.86605474786771,-1.76801477730732,-1.76588993846838,-1.76551364586657,
-1.76477055613347,-1.751876636334,-1.75023752101634,-1.74940071972699,-1.74878447710516,
-1.74811197016471,-1.74717609249539,-1.74493960392291,-1.74185521492002,
-1.70797044623799,-1.62503875622738,-1.61721685831853,-1.61220492892579,
-1.59288245182046,-1.58978938287022,-1.5882786712886,-1.5870975325393,-1.58579104736821,
-1.58365206915085,-1.57615884923341,-1.52833608089518,-1.43300273999321,
-1.42832939480946,-1.42704533676396,-1.42628984447174,-1.42563410833287,
-1.42481670858595,-1.42321065587256,-1.4119657976086,-1.37873792632746,
-1.27420013715539,-1.26822401220228,-1.26618259088209,-1.26502635141361,
-1.26387200040643,-1.2624318529962,-1.26087135638339,-1.25837829902198,
-1.253547656717,-1.20754014024346,-1.10989601028361,-1.10545456186501,-1.1041801983673,
-1.10343434048311,-1.10284311255049,-1.10204354235009,-1.10052280318078,
-1.09147032340054,-1.07232405365638,-1.02489228675618,-0.949483034791866,
-0.94501793268378,-0.94338985059188,-0.942249102753054,-0.9410914226805,
-0.939617726288424,-0.938009184552817,-0.935401826011992,-0.930266421810447,
-0.878954944912198,-0.794033865938783,-0.783522167594479,-0.781807752648127,
-0.780968247286719,-0.780310410687896,-0.779569435747449,-0.77831711744584,
-0.773514363053926,-0.737869422258917,-0.693744178714172,-0.626115874048793,
-0.622141206881874,-0.620591626859499,-0.619471990823366,-0.618304254010764,
-0.616767022916174,-0.615072223276405,-0.612258255970519,-0.606561416940706,
-0.591800522012533,-0.556561498511098,-0.473857630813761,-0.461020699778079,
-0.459383220290059,-0.458546695490058,-0.457930384791895,-0.457257522698231,
-0.456320657620648,-0.454079490688016,-0.450987246239434,-0.416950593013296,
-0.37456923187825,-0.350874429196386,-0.303200284114423,-0.299416426494504,
-0.297899091423329,-0.296787779646623,-0.295663857057532,-0.294125059982821,
-0.290864735347415,-0.286588215198992,-0.276563774393582,-0.250721402949624,
-0.142605721723476,-0.137449755167389,-0.136117170556043,-0.1353501552857,
-0.134694950961937,-0.133891441341708,-0.132353129778761,-0.122909554726513,
-0.110769040180773,-0.000958105903751487),.UNSPECIFIED.);
#828=B_SPLINE_CURVE_WITH_KNOTS('',3,(#44559,#44560,#44561,#44562,#44563,
#44564,#44565,#44566,#44567,#44568,#44569,#44570,#44571,#44572,#44573,#44574,
#44575,#44576,#44577,#44578,#44579,#44580,#44581,#44582,#44583,#44584,#44585,
#44586,#44587,#44588,#44589,#44590,#44591,#44592,#44593,#44594,#44595,#44596,
#44597,#44598,#44599,#44600,#44601,#44602,#44603,#44604,#44605,#44606,#44607,
#44608,#44609,#44610,#44611,#44612,#44613,#44614,#44615,#44616,#44617,#44618,
#44619,#44620,#44621,#44622,#44623,#44624,#44625,#44626,#44627,#44628,#44629,
#44630,#44631,#44632,#44633,#44634,#44635,#44636,#44637,#44638,#44639,#44640,
#44641,#44642,#44643,#44644,#44645,#44646,#44647,#44648,#44649,#44650,#44651,
#44652,#44653,#44654,#44655,#44656,#44657,#44658,#44659,#44660,#44661,#44662,
#44663,#44664,#44665,#44666,#44667,#44668,#44669,#44670,#44671,#44672,#44673,
#44674,#44675,#44676,#44677,#44678,#44679,#44680,#44681,#44682,#44683,#44684,
#44685,#44686,#44687,#44688,#44689,#44690,#44691,#44692,#44693,#44694,#44695,
#44696,#44697,#44698,#44699,#44700,#44701,#44702,#44703,#44704,#44705,#44706,
#44707,#44708,#44709,#44710,#44711,#44712,#44713,#44714,#44715,#44716,#44717,
#44718,#44719,#44720,#44721,#44722,#44723,#44724,#44725,#44726,#44727,#44728,
#44729,#44730,#44731,#44732,#44733,#44734,#44735,#44736,#44737,#44738,#44739,
#44740,#44741,#44742,#44743,#44744,#44745,#44746,#44747,#44748,#44749,#44750,
#44751,#44752,#44753,#44754,#44755,#44756,#44757,#44758,#44759,#44760,#44761,
#44762,#44763,#44764,#44765,#44766,#44767,#44768,#44769,#44770,#44771,#44772,
#44773,#44774,#44775,#44776,#44777,#44778,#44779,#44780,#44781,#44782,#44783,
#44784,#44785,#44786,#44787,#44788,#44789,#44790,#44791,#44792,#44793,#44794,
#44795,#44796,#44797,#44798,#44799,#44800,#44801,#44802,#44803,#44804,#44805,
#44806,#44807,#44808,#44809,#44810,#44811,#44812,#44813,#44814,#44815,#44816,
#44817,#44818,#44819,#44820,#44821,#44822,#44823,#44824,#44825,#44826,#44827,
#44828,#44829,#44830,#44831,#44832,#44833,#44834,#44835,#44836,#44837,#44838,
#44839,#44840,#44841,#44842,#44843,#44844,#44845,#44846,#44847,#44848,#44849,
#44850,#44851,#44852,#44853,#44854,#44855,#44856,#44857,#44858,#44859,#44860,
#44861,#44862,#44863,#44864,#44865,#44866,#44867,#44868,#44869,#44870,#44871,
#44872,#44873,#44874,#44875,#44876,#44877,#44878,#44879,#44880,#44881,#44882,
#44883,#44884,#44885,#44886,#44887,#44888,#44889,#44890,#44891,#44892,#44893,
#44894,#44895,#44896,#44897,#44898,#44899,#44900,#44901,#44902,#44903,#44904,
#44905,#44906,#44907,#44908,#44909,#44910,#44911,#44912,#44913,#44914,#44915,
#44916,#44917,#44918,#44919,#44920,#44921,#44922,#44923,#44924,#44925,#44926,
#44927,#44928,#44929,#44930,#44931,#44932,#44933,#44934,#44935,#44936,#44937,
#44938,#44939,#44940,#44941,#44942,#44943,#44944,#44945,#44946,#44947,#44948,
#44949,#44950,#44951,#44952,#44953,#44954,#44955,#44956,#44957,#44958,#44959,
#44960,#44961,#44962,#44963,#44964,#44965,#44966,#44967,#44968,#44969,#44970,
#44971,#44972,#44973,#44974,#44975,#44976,#44977,#44978,#44979,#44980,#44981,
#44982,#44983,#44984,#44985,#44986,#44987,#44988,#44989,#44990,#44991,#44992,
#44993,#44994,#44995,#44996,#44997,#44998,#44999,#45000,#45001,#45002,#45003,
#45004,#45005,#45006,#45007,#45008,#45009,#45010,#45011,#45012,#45013,#45014,
#45015,#45016,#45017,#45018,#45019,#45020,#45021,#45022,#45023,#45024,#45025,
#45026,#45027,#45028,#45029,#45030,#45031,#45032,#45033,#45034,#45035,#45036,
#45037,#45038,#45039,#45040,#45041,#45042,#45043,#45044,#45045,#45046,#45047,
#45048,#45049,#45050,#45051,#45052,#45053,#45054,#45055,#45056,#45057,#45058,
#45059,#45060,#45061,#45062,#45063,#45064,#45065,#45066,#45067,#45068,#45069,
#45070,#45071,#45072,#45073,#45074),.UNSPECIFIED.,.F.,.F.,(4,2,2,2,2,2,
2,2,2,2,2,2,2,2,2,2,2,2,2,2,2,2,2,2,2,2,2,2,2,2,2,2,2,2,2,2,2,2,2,2,2,2,
2,2,2,2,2,2,2,2,2,2,2,2,2,2,2,2,2,2,2,2,2,2,2,2,2,2,2,2,2,2,2,2,2,2,2,2,
2,2,2,2,2,2,2,2,2,2,2,2,2,2,2,2,2,2,2,2,2,2,2,2,2,2,2,2,2,2,2,2,2,2,2,2,
2,2,2,2,2,2,2,2,2,2,2,2,2,2,2,2,2,2,2,2,2,2,2,2,2,2,2,2,2,2,2,2,2,2,2,2,
2,2,2,2,2,2,2,2,2,2,2,2,2,2,2,2,2,2,2,2,2,2,2,2,2,2,2,2,2,2,2,2,2,2,2,2,
2,2,2,2,2,2,2,2,2,2,2,2,2,2,2,2,2,2,2,2,2,2,2,2,2,2,2,2,2,2,2,2,2,2,2,2,
2,2,2,2,2,2,2,2,2,2,2,2,2,2,2,2,2,2,2,2,2,2,2,2,2,2,2,2,2,2,2,2,2,2,2,4),
(-4.06138658790065,-4.04525241163887,-4.03846191229691,-4.03666092753074,
-4.03538999670297,-4.03428943243753,-4.0331563620915,-4.03165174002101,
-4.02869099557283,-4.01127521650964,-4.00463316959338,-3.91388733812666,
-3.88766769835203,-3.87545379763928,-3.8738164497094,-3.87299254319138,
-3.872342181756,-3.87159326005671,-3.87030535664154,-3.86574026801696,-3.77929695118869,
-3.7468547043871,-3.72658633695271,-3.71938768854679,-3.71604271295157,
-3.71337219610962,-3.71195598426428,-3.71078834129195,-3.70961535245074,
-3.70749155857786,-3.70090479208845,-3.64437843326429,-3.62082143422239,
-3.61351181260872,-3.5887119174071,-3.55374002091052,-3.55149054298406,
-3.5505523496365,-3.54987931514528,-3.54926341341319,-3.54842825567468,
-3.5467958593838,-3.53409453311114,-3.53222923279084,-3.44955845594532,
-3.41069222553109,-3.39941376081397,-3.39474637538757,-3.39231497368581,
-3.39025708166305,-3.38897900269922,-3.38785652538869,-3.38637188283222,
-3.38405385564009,-3.37306413002367,-3.27195599684365,-3.25804829741409,
-3.23889995046674,-3.22986700835319,-3.22834700082605,-3.22754752621136,
-3.22689886127196,-3.2262323638511,-3.22498266551041,-3.22076137410961,
-3.14641217631126,-3.10308740060867,-3.07744641362685,-3.07236114234358,
-3.06977232276382,-3.06817146731439,-3.06670352426636,-3.06554545092442,
-3.06440205700285,-3.06276471772964,-3.05823982532329,-2.98177355295227,
-2.93502155321649,-2.91605566486271,-2.90717834065533,-2.90566536383059,
-2.90486737099974,-2.90427622252356,-2.90352901202327,-2.90224887775492,
-2.89775581107323,-2.80095027050559,-2.77708855281743,-2.75144959754393,
-2.74801504644824,-2.74606609070927,-2.74473421884656,-2.74345823526503,
-2.74230323499458,-2.74079960205125,-2.73784371726531,-2.72052292009604,
-2.71943493637124,-2.71399311393548,-2.70338460738783,-2.68299215731286,
-2.61150387683504,-2.58762057446811,-2.58380774021796,-2.58265459193284,
-2.58193582147778,-2.5812722616217,-2.58040456433567,-2.57849643800812,
-2.56324257006605,-2.56284113790527,-2.49424016638539,-2.42646157202313,
-2.4230114609258,-2.42143141735595,-2.42024029680739,-2.41911993282674,
-2.41756753466397,-2.41443190369425,-2.38466755091193,-2.35828764980881,
-2.32971131761324,-2.30384082362538,-2.27349143018919,-2.26203079994999,
-2.26041744615178,-2.2595985131647,-2.25894863630183,-2.25819638136289,
-2.25692628545334,-2.25238598992755,-2.15596388265476,-2.10392345594794,
-2.10039235584378,-2.09879736395309,-2.09760399249313,-2.09648806514285,
-2.09495213124828,-2.0910577185451,-2.03100349848463,-1.94326144648473,
-1.93867924312219,-1.93740466986524,-1.93665135137414,-1.93599531592502,
-1.93517472307456,-1.93355340164878,-1.92184983294585,-1.89525337202058,
-1.82010363391883,-1.81634216012349,-1.78136733622026,-1.77779111100459,
-1.77632369740808,-1.7752250949,-1.77401848331915,-1.77234845688319,-1.76839743106462,
-1.7185592353649,-1.65194598019134,-1.61764235640656,-1.61538917797913,
-1.61451888789625,-1.61389381410069,-1.61322740868621,-1.61232669109436,
-1.61029096919824,-1.57144352511198,-1.47664352940298,-1.47287352042536,
-1.45751080195113,-1.45491704310786,-1.45336545826207,-1.45217467670617,
-1.45089956858808,-1.44890186683498,-1.44267891762859,-1.40746688306336,
-1.30556611214595,-1.29401768875948,-1.29229015591586,-1.29144527636687,
-1.29079797096109,-1.29018433764201,-1.28912711292849,-1.28609385627485,
-1.26980592579601,-1.24821124225988,-1.15252031810644,-1.13487340368952,
-1.13190051483468,-1.13039323847186,-1.12921224291411,-1.1279033092496,
-1.12575438319312,-1.11816714771936,-1.09256378057833,-1.0494813961342,
-0.981977876192697,-0.971243972851883,-0.969553511358955,-0.968716515004169,
-0.968073670182242,-0.96745990049205,-0.966393903719686,-0.963295090148569,
-0.946408748241712,-0.92437473002101,-0.829596135355245,-0.812158646992164,
-0.809196786859625,-0.807691939666551,-0.806511305547638,-0.805201186870975,
-0.803046688473379,-0.795403224139457,-0.769689062514448,-0.74252759107259,
-0.652294086378226,-0.647742400429921,-0.646481593411662,-0.645741227288095,
-0.645086413421815,-0.644455761117519,-0.643133303953209,-0.637483987186614,
-0.553944449314733,-0.49088067354032,-0.486975890216483,-0.485438081575016,
-0.484321564930764,-0.483128287719782,-0.481534671322991,-0.478011706145282,
-0.427749858845276,-0.343769422459311,-0.339033058243669,-0.325887387833028,
-0.324093831314113,-0.323235193404797,-0.3225841284291,-0.321970737394989,
-0.320931437945029,-0.318027856959303,-0.259287722059132,-0.189731327803648,
-0.167066713047837,-0.164150739366711,-0.162654056856414,-0.16154808284931,
-0.160347518212909,-0.15871136463824,-0.154954499626856,-0.0722293716752518,
-0.00817606052254369,-0.00244148803838146,-0.00108799394096062,-0.000957397290290128),
 .UNSPECIFIED.);
#829=B_SPLINE_CURVE_WITH_KNOTS('',3,(#45076,#45077,#45078,#45079,#45080,
#45081,#45082,#45083,#45084,#45085,#45086,#45087,#45088,#45089,#45090,#45091,
#45092,#45093,#45094,#45095,#45096,#45097,#45098,#45099,#45100,#45101,#45102,
#45103,#45104,#45105,#45106,#45107,#45108,#45109,#45110,#45111,#45112,#45113,
#45114,#45115,#45116,#45117,#45118,#45119,#45120,#45121,#45122,#45123,#45124,
#45125,#45126,#45127,#45128,#45129,#45130,#45131,#45132,#45133,#45134,#45135,
#45136,#45137,#45138,#45139,#45140,#45141,#45142,#45143,#45144,#45145,#45146,
#45147,#45148,#45149,#45150,#45151,#45152,#45153,#45154,#45155,#45156,#45157,
#45158,#45159,#45160,#45161,#45162,#45163,#45164,#45165,#45166,#45167,#45168,
#45169,#45170,#45171,#45172,#45173,#45174,#45175,#45176,#45177,#45178,#45179,
#45180,#45181,#45182,#45183,#45184,#45185,#45186,#45187,#45188,#45189,#45190,
#45191,#45192,#45193,#45194,#45195,#45196,#45197,#45198,#45199,#45200,#45201,
#45202,#45203,#45204,#45205,#45206,#45207,#45208,#45209,#45210,#45211,#45212,
#45213,#45214,#45215,#45216,#45217,#45218,#45219,#45220,#45221,#45222,#45223,
#45224,#45225,#45226,#45227,#45228,#45229,#45230,#45231,#45232,#45233,#45234,
#45235,#45236,#45237,#45238,#45239,#45240,#45241,#45242,#45243,#45244,#45245,
#45246,#45247,#45248,#45249,#45250,#45251,#45252,#45253,#45254,#45255,#45256,
#45257,#45258,#45259,#45260,#45261,#45262,#45263,#45264,#45265,#45266,#45267,
#45268,#45269,#45270,#45271,#45272,#45273,#45274,#45275,#45276,#45277,#45278,
#45279,#45280,#45281,#45282,#45283,#45284,#45285,#45286,#45287,#45288,#45289,
#45290,#45291,#45292,#45293,#45294,#45295,#45296,#45297,#45298,#45299,#45300,
#45301,#45302,#45303,#45304,#45305,#45306,#45307,#45308,#45309,#45310,#45311,
#45312,#45313,#45314,#45315,#45316,#45317,#45318,#45319,#45320,#45321,#45322,
#45323,#45324,#45325,#45326,#45327,#45328,#45329,#45330,#45331,#45332,#45333,
#45334,#45335,#45336,#45337,#45338,#45339,#45340,#45341,#45342,#45343,#45344,
#45345,#45346,#45347,#45348,#45349,#45350,#45351,#45352,#45353,#45354,#45355,
#45356,#45357,#45358,#45359,#45360,#45361,#45362,#45363,#45364,#45365,#45366,
#45367,#45368,#45369,#45370,#45371,#45372,#45373,#45374,#45375,#45376,#45377,
#45378,#45379,#45380,#45381,#45382,#45383,#45384,#45385,#45386,#45387,#45388,
#45389,#45390,#45391,#45392,#45393,#45394,#45395,#45396,#45397,#45398,#45399,
#45400,#45401,#45402,#45403,#45404,#45405,#45406,#45407,#45408,#45409,#45410,
#45411,#45412,#45413,#45414,#45415,#45416,#45417,#45418,#45419,#45420,#45421,
#45422,#45423,#45424,#45425,#45426,#45427,#45428,#45429,#45430,#45431,#45432,
#45433,#45434,#45435,#45436,#45437,#45438,#45439,#45440,#45441,#45442,#45443,
#45444,#45445,#45446,#45447,#45448,#45449,#45450,#45451,#45452,#45453,#45454,
#45455,#45456,#45457,#45458,#45459,#45460,#45461,#45462,#45463,#45464,#45465,
#45466,#45467,#45468,#45469,#45470,#45471,#45472,#45473,#45474,#45475,#45476,
#45477,#45478,#45479,#45480,#45481,#45482,#45483,#45484,#45485,#45486,#45487,
#45488,#45489,#45490,#45491,#45492,#45493,#45494,#45495,#45496,#45497,#45498,
#45499,#45500,#45501,#45502,#45503,#45504,#45505,#45506,#45507,#45508,#45509,
#45510,#45511,#45512,#45513,#45514,#45515,#45516,#45517,#45518,#45519,#45520,
#45521,#45522,#45523,#45524,#45525,#45526,#45527,#45528,#45529,#45530,#45531,
#45532,#45533,#45534,#45535,#45536,#45537,#45538,#45539,#45540,#45541,#45542,
#45543,#45544,#45545,#45546,#45547,#45548,#45549,#45550,#45551,#45552,#45553,
#45554,#45555,#45556,#45557,#45558,#45559,#45560,#45561,#45562,#45563,#45564,
#45565,#45566,#45567,#45568,#45569,#45570,#45571,#45572,#45573,#45574,#45575,
#45576,#45577,#45578,#45579,#45580,#45581,#45582,#45583,#45584,#45585,#45586,
#45587,#45588,#45589,#45590,#45591,#45592,#45593,#45594,#45595,#45596,#45597,
#45598,#45599,#45600,#45601,#45602,#45603,#45604,#45605,#45606,#45607,#45608,
#45609),.UNSPECIFIED.,.F.,.F.,(4,2,2,2,2,2,2,2,2,2,2,2,2,2,2,2,2,2,2,2,
2,2,2,2,2,2,2,2,2,2,2,2,2,2,2,2,2,2,2,2,2,2,2,2,2,2,2,2,2,2,2,2,2,2,2,2,
2,2,2,2,2,2,2,2,2,2,2,2,2,2,2,2,2,2,2,2,2,2,2,2,2,2,2,2,2,2,2,2,2,2,2,2,
2,2,2,2,2,2,2,2,2,2,2,2,2,2,2,2,2,2,2,2,2,2,2,2,2,2,2,2,2,2,2,2,2,2,2,2,
2,2,2,2,2,2,2,2,2,2,2,2,2,2,2,2,2,2,2,2,2,2,2,2,2,2,2,2,2,2,2,2,2,2,2,2,
2,2,2,2,2,2,2,2,2,2,2,2,2,2,2,2,2,2,2,2,2,2,2,2,2,2,2,2,2,2,2,2,2,2,2,2,
2,2,2,2,2,2,2,2,2,2,2,2,2,2,2,2,2,2,2,2,2,2,2,2,2,2,2,2,2,2,2,2,2,2,2,2,
2,2,2,2,2,2,2,2,2,2,2,2,2,2,2,2,2,2,2,2,2,2,2,2,2,2,2,2,2,2,4),(-4.06110231792537,
-4.06059741070819,-4.05996580577075,-4.05933590414146,-4.05826813906809,
-4.0554087310575,-4.04937630105949,-3.94277587088132,-3.90832838972063,
-3.90218897453181,-3.90020172041202,-3.89892910673986,-3.89773770683121,
-3.89618109001173,-3.89276351515535,-3.86512999257404,-3.77706897567989,
-3.75790191539855,-3.74601483661137,-3.7397702817228,-3.73878654213019,
-3.73790440067179,-3.73725014548363,-3.7366274668612,-3.73576587196678,
-3.733563234126,-3.70318058322381,-3.69255561533879,-3.67083191200692,-3.66437087297449,
-3.65695814206526,-3.64825416453209,-3.62011616390153,-3.58579194243182,
-3.5796657402366,-3.57767992654376,-3.57640750985249,-3.57521578101949,
-3.57365799694234,-3.57023487072491,-3.54243864676609,-3.47022326564263,
-3.41827233294287,-3.41689595392164,-3.41603294795876,-3.41523744421432,
-3.41459457234492,-3.41383969120689,-3.4125808892788,-3.40804684495158,
-3.32081205913109,-3.26140035644468,-3.25660247897048,-3.25479670490801,
-3.25356324461595,-3.2523629182605,-3.25092593253144,-3.24738571736261,
-3.21561771217929,-3.13063232111741,-3.10529573203479,-3.09492438590364,
-3.09381035386053,-3.09283561624489,-3.09216323351753,-3.09150098794294,
-3.09068364441675,-3.08873501335054,-3.07086385413203,-2.98790742626346,
-2.94192899190128,-2.93460586754559,-2.9324843537103,-2.93118168282318,
-2.9299994918125,-2.92848116572453,-2.92535031368259,-2.90521496225671,
-2.89938169300854,-2.82364872032709,-2.79853250517755,-2.78059361839539,
-2.7721601370065,-2.77109783418148,-2.77036611949277,-2.76966375921583,
-2.76901700678208,-2.76815550911277,-2.76638627477777,-2.75385130888327,
-2.6871097790703,-2.61422968186529,-2.61076723108315,-2.60918503011165,
-2.6079937266623,-2.60687424849963,-2.60532475605336,-2.60220022496166,
-2.57283694244002,-2.48736718002324,-2.45369478931186,-2.45062080994688,
-2.44839031707323,-2.44745538021443,-2.4467829748781,-2.44616640763326,
-2.44532856638664,-2.4436856373655,-2.43068863961419,-2.43002032068448,
-2.42959984484413,-2.42545707184824,-2.42417351647987,-2.4186935107769,
-2.36246464586216,-2.29157434075268,-2.2881161545123,-2.28653469650209,
-2.28534345408835,-2.28422366798839,-2.28267316979721,-2.27954480480314,
-2.25004398139601,-2.20147191609034,-2.1547746321519,-2.13582306906476,
-2.12695367730483,-2.12544128862174,-2.12464351748277,-2.12405249474332,
-2.12330539175791,-2.1220253188847,-2.11753134328931,-2.03168865576719,
-1.96971099301032,-1.96580945938898,-1.96427235728451,-1.96315615354021,
-1.9619630231965,-1.96036928001642,-1.9568447199659,-1.9061529388742,-1.80814635274863,
-1.80374482359099,-1.80247482054093,-1.80172990465991,-1.80113850227119,
-1.8003375129953,-1.79881021647817,-1.78961128900764,-1.77065428408413,
-1.72326988821991,-1.64818516290193,-1.64341894849573,-1.64155967795843,
-1.64043923043578,-1.63924818351396,-1.63766851560675,-1.63422032918383,
-1.56708663846734,-1.492223457132,-1.48179818789063,-1.48008807289792,-1.47924941019955,
-1.47859164268512,-1.47785010948254,-1.47659537088837,-1.47176597658992,
-1.4357416479433,-1.33991695954287,-1.32269957882989,-1.31974922991974,
-1.31824682277088,-1.31709199203695,-1.31581531081975,-1.31448254766303,
-1.3125313911441,-1.30909127835176,-1.28337600732234,-1.25947202550202,
-1.16276358981913,-1.15825399096052,-1.15697202037141,-1.15622437892236,
-1.15563325175887,-1.15483575231578,-1.15332520635122,-1.14450181567692,
-1.1256382856919,-1.07938310532923,-1.00235919364528,-0.997803538136437,
-0.996161493317348,-0.995016770317971,-0.993859025196569,-0.992393788122643,
-0.990796945037483,-0.988217733036795,-0.983158169121833,-0.957365478500339,
-0.913898705315078,-0.839693607501277,-0.835495494522066,-0.834248393551776,
-0.833582378921313,-0.832927341465691,-0.83212402627691,-0.830586056253903,
-0.821143681474916,-0.809178803263304,-0.792924440093603,-0.781210538963257,
-0.696000642247555,-0.693934704437293,-0.677191860501416,-0.674266279491795,
-0.672769072921257,-0.671639867787227,-0.670366718425579,-0.668330683683048,
-0.665931106127077,-0.661347528796306,-0.650341225383484,-0.613416194063387,
-0.517394322672244,-0.512782188437959,-0.511504230423305,-0.51074998977896,
-0.51009384310111,-0.509274003451231,-0.50765702101082,-0.496098177550979,
-0.469378204704691,-0.443954440514808,-0.436901610220834,-0.4128835759767,
-0.355950659448746,-0.352071564871792,-0.350537824893103,-0.349422142178519,
-0.348251680833586,-0.346699304797494,-0.343362176706676,-0.338965634788529,
-0.328560923706869,-0.29976664066489,-0.249535658250077,-0.193171981183607,
-0.189834820803438,-0.188695515824215,-0.188051160826892,-0.187458379460019,
-0.186646159145829,-0.185066063001477,-0.174567135399675,-0.148647967678681,
-0.053616501139824,-0.0469471354448575,-0.0315419778726503,-0.0289453529413174,
-0.0273926669385131,-0.0262014013607221,-0.0251011774085411,-0.0238508068138008,
-0.0221011664640548,-0.019155079023621,-0.00095669269283294),
 .UNSPECIFIED.);
#830=B_SPLINE_CURVE_WITH_KNOTS('',3,(#45611,#45612,#45613,#45614,#45615,
#45616,#45617,#45618,#45619,#45620,#45621,#45622,#45623,#45624,#45625,#45626,
#45627,#45628,#45629,#45630,#45631,#45632,#45633,#45634,#45635,#45636,#45637,
#45638,#45639,#45640,#45641,#45642,#45643,#45644,#45645,#45646,#45647,#45648,
#45649,#45650,#45651,#45652,#45653,#45654,#45655,#45656,#45657,#45658,#45659,
#45660,#45661,#45662,#45663,#45664,#45665,#45666,#45667,#45668,#45669,#45670,
#45671,#45672,#45673,#45674,#45675,#45676,#45677,#45678,#45679,#45680,#45681,
#45682,#45683,#45684,#45685,#45686,#45687,#45688,#45689,#45690,#45691,#45692,
#45693,#45694,#45695,#45696,#45697,#45698,#45699,#45700,#45701,#45702,#45703,
#45704,#45705,#45706,#45707,#45708,#45709,#45710,#45711,#45712,#45713,#45714,
#45715,#45716,#45717,#45718,#45719,#45720,#45721,#45722,#45723,#45724,#45725,
#45726,#45727,#45728,#45729,#45730,#45731,#45732,#45733,#45734,#45735,#45736,
#45737,#45738,#45739,#45740,#45741,#45742,#45743,#45744,#45745,#45746,#45747,
#45748,#45749,#45750,#45751,#45752,#45753,#45754,#45755,#45756,#45757,#45758,
#45759,#45760,#45761,#45762,#45763,#45764,#45765,#45766,#45767,#45768,#45769,
#45770,#45771,#45772,#45773,#45774,#45775,#45776,#45777,#45778,#45779,#45780,
#45781,#45782,#45783,#45784,#45785,#45786,#45787,#45788,#45789,#45790,#45791,
#45792,#45793,#45794,#45795,#45796,#45797,#45798,#45799,#45800,#45801,#45802,
#45803,#45804,#45805,#45806,#45807,#45808,#45809,#45810,#45811,#45812,#45813,
#45814,#45815,#45816,#45817,#45818,#45819,#45820,#45821,#45822,#45823,#45824,
#45825,#45826,#45827,#45828,#45829,#45830,#45831,#45832,#45833,#45834,#45835,
#45836,#45837,#45838,#45839,#45840,#45841,#45842,#45843,#45844,#45845,#45846,
#45847,#45848,#45849,#45850,#45851,#45852,#45853,#45854,#45855,#45856,#45857,
#45858,#45859,#45860,#45861,#45862,#45863,#45864,#45865,#45866,#45867,#45868,
#45869,#45870,#45871,#45872,#45873,#45874,#45875,#45876,#45877,#45878,#45879,
#45880,#45881,#45882,#45883,#45884,#45885,#45886,#45887,#45888,#45889,#45890,
#45891,#45892,#45893,#45894,#45895,#45896,#45897,#45898,#45899,#45900,#45901,
#45902,#45903,#45904,#45905,#45906,#45907,#45908,#45909,#45910,#45911,#45912,
#45913,#45914,#45915,#45916,#45917,#45918,#45919,#45920,#45921,#45922,#45923,
#45924,#45925,#45926,#45927,#45928,#45929,#45930,#45931,#45932,#45933,#45934,
#45935,#45936,#45937,#45938,#45939,#45940,#45941,#45942,#45943,#45944,#45945,
#45946,#45947,#45948,#45949,#45950,#45951,#45952,#45953,#45954,#45955,#45956,
#45957,#45958,#45959,#45960,#45961,#45962,#45963,#45964,#45965,#45966,#45967,
#45968,#45969,#45970,#45971,#45972,#45973,#45974,#45975,#45976,#45977,#45978,
#45979,#45980,#45981,#45982,#45983,#45984,#45985,#45986,#45987,#45988,#45989,
#45990,#45991,#45992,#45993,#45994,#45995,#45996,#45997,#45998,#45999,#46000,
#46001,#46002,#46003,#46004,#46005,#46006,#46007,#46008,#46009,#46010,#46011,
#46012,#46013,#46014,#46015,#46016,#46017,#46018,#46019,#46020,#46021,#46022,
#46023,#46024,#46025,#46026,#46027,#46028,#46029,#46030,#46031,#46032,#46033,
#46034,#46035,#46036,#46037,#46038,#46039,#46040,#46041,#46042,#46043,#46044,
#46045,#46046,#46047,#46048,#46049,#46050,#46051,#46052,#46053,#46054,#46055,
#46056,#46057,#46058,#46059,#46060,#46061,#46062,#46063,#46064,#46065,#46066,
#46067,#46068,#46069,#46070,#46071,#46072,#46073,#46074,#46075,#46076,#46077,
#46078,#46079,#46080,#46081,#46082,#46083,#46084,#46085,#46086,#46087,#46088,
#46089,#46090,#46091,#46092,#46093,#46094,#46095,#46096,#46097,#46098,#46099,
#46100,#46101,#46102,#46103,#46104,#46105,#46106,#46107,#46108,#46109,#46110,
#46111,#46112,#46113,#46114,#46115,#46116,#46117,#46118,#46119,#46120,#46121,
#46122,#46123,#46124,#46125,#46126,#46127,#46128,#46129,#46130,#46131,#46132,
#46133,#46134,#46135,#46136,#46137,#46138,#46139,#46140,#46141,#46142,#46143,
#46144,#46145,#46146,#46147,#46148,#46149,#46150,#46151,#46152,#46153,#46154,
#46155,#46156,#46157,#46158,#46159,#46160,#46161,#46162,#46163,#46164,#46165,
#46166),.UNSPECIFIED.,.F.,.F.,(4,2,2,2,2,2,2,2,2,2,2,2,2,2,2,2,2,2,2,2,
2,2,2,2,2,2,2,2,2,2,2,2,2,2,2,2,2,2,2,2,2,2,2,2,2,2,2,2,2,2,2,2,2,2,2,2,
2,2,2,2,2,2,2,2,2,2,2,2,2,2,2,2,2,2,2,2,2,2,2,2,2,2,2,2,2,2,2,2,2,2,2,2,
2,2,2,2,2,2,2,2,2,2,2,2,2,2,2,2,2,2,2,2,2,2,2,2,2,2,2,2,2,2,2,2,2,2,2,2,
2,2,2,2,2,2,2,2,2,2,2,2,2,2,2,2,2,2,2,2,2,2,2,2,2,2,2,2,2,2,2,2,2,2,2,2,
2,2,2,2,2,2,2,2,2,2,2,2,2,2,2,2,2,2,2,2,2,2,2,2,2,2,2,2,2,2,2,2,2,2,2,2,
2,2,2,2,2,2,2,2,2,2,2,2,2,2,2,2,2,2,2,2,2,2,2,2,2,2,2,2,2,2,2,2,2,2,2,2,
2,2,2,2,2,2,2,2,2,2,2,2,2,2,2,2,2,2,2,2,2,2,2,2,2,2,2,2,2,2,2,2,2,2,2,2,
2,2,2,2,2,4),(-4.0605457412234,-3.95495941481507,-3.93605529689604,-3.92721261541421,
-3.92570135227873,-3.92490377647833,-3.92431272510179,-3.92366118587011,
-3.92248546477351,-3.91886818171779,-3.85821424937071,-3.80958345116075,
-3.78440016141353,-3.77371376972052,-3.76922939015871,-3.76584033044454,
-3.76427722502882,-3.76310532795215,-3.76199310489736,-3.76047177328619,
-3.75666378541168,-3.70702156991851,-3.68142349363787,-3.63212488138626,
-3.61340035922391,-3.60464695455006,-3.60313982719317,-3.60234313118875,
-3.6017521635418,-3.6010041380274,-3.599720108492,-3.59519036891763,-3.50103821214206,
-3.4674935331529,-3.45311739894622,-3.44753063720286,-3.4447568329863,-3.44307879429006,
-3.44156915823026,-3.44040208399134,-3.43928163976136,-3.43772864791244,
-3.43373254322522,-3.36580403816991,-3.32035709763325,-3.28619006579357,
-3.28149517993135,-3.28025277480128,-3.27951407625275,-3.27885592000855,
-3.2780128624221,-3.27628033052043,-3.26540002771946,-3.18084688690849,
-3.12963207179594,-3.12450159442338,-3.12189607550668,-3.12028833303438,
-3.11881504912169,-3.1176575248148,-3.11651662893626,-3.11488782789022,
-3.11041759778343,-3.03501358337079,-2.98753685354794,-2.96838463685861,
-2.95933030812582,-2.95780956317301,-2.95701002650281,-2.95641884002651,
-2.95567305433016,-2.95439886470307,-2.94995849008219,-2.85235244396182,
-2.80636117448341,-2.80153098738271,-2.79903805153858,-2.79747759034302,
-2.79603744803748,-2.79488308071807,-2.79372680612787,-2.79168527657539,
-2.78570850087434,-2.68101841539463,-2.65204860258694,-2.63682145768169,
-2.63510579681138,-2.63426609524447,-2.63366982354743,-2.6330375626047,
-2.63214053437816,-2.62971705181821,-2.62838360526375,-2.57111421107401,
-2.52129948201764,-2.50144384006515,-2.47784068896493,-2.47486215488716,
-2.47337432032641,-2.47230619697623,-2.47117717034562,-2.46959218536517,
-2.46632492806459,-2.43107980335647,-2.36283488955639,-2.34216953783651,
-2.32301471011016,-2.3139443231393,-2.31242276755273,-2.31162301916312,
-2.31097441051002,-2.31030821754058,-2.30905979838784,-2.30484887839261,
-2.23058927259819,-2.18721893608051,-2.16146923462119,-2.1538047600535,
-2.15164811237091,-2.15033748927902,-2.14915691955492,-2.14765286726362,
-2.14469482349819,-2.12733099566277,-2.12380863786516,-2.03050706077327,
-2.00448716407665,-1.99171874193385,-1.99008379879637,-1.98924794756592,
-1.98863183023296,-1.98795886582634,-1.98702130744568,-1.98477588633959,
-1.98167619965725,-1.94748355837829,-1.87031765955104,-1.86623396982405,
-1.8564347390615,-1.8512016785329,-1.84955458623469,-1.83252383751663,-1.8295832664142,
-1.82808288913795,-1.82690264967444,-1.82558975378762,-1.82342329244579,
-1.81566172260695,-1.76482143772875,-1.68339801706031,-1.68240981448849,
-1.68074183692639,-1.66895912088893,-1.66718531308258,-1.66633397738605,
-1.66567472245422,-1.66494045377003,-1.66371830352068,-1.65924062390827,
-1.62787615169194,-1.53574800671381,-1.53007716391375,-1.50999702229069,
-1.50686822955255,-1.50535013796723,-1.50416778437731,-1.50286458428999,
-1.50074142192853,-1.49340505481238,-1.44728282375824,-1.35816464610307,
-1.34617961392421,-1.34439693098774,-1.34355296614099,-1.34289282968718,
-1.34217692863619,-1.34101378341309,-1.33962671722753,-1.33692836280511,
-1.31023881101801,-1.23992340099507,-1.18842429058249,-1.18459442000821,
-1.18306921381325,-1.18195587723007,-1.18076036198855,-1.17915397509614,
-1.17556241757058,-1.17078787472338,-1.12571707123542,-1.04241426828205,
-1.0400186392906,-1.03735999983631,-1.03693121703044,-1.03546018938973,
-1.02345391881338,-1.02167022790515,-1.02082603295498,-1.02016582700799,
-1.01955119947373,-1.01848230681004,-1.01534964374975,-0.998004841984789,
-0.979774025687205,-0.929382224820403,-0.865817219792452,-0.861910648978565,
-0.86037232695504,-0.859255504045153,-0.858061961801052,-0.856468098664971,
-0.852945024212992,-0.802814543466148,-0.735058523114656,-0.723450420410497,
-0.717572148309861,-0.716579692962732,-0.715091123950269,-0.714402455123496,
-0.713493952462066,-0.7008111751004,-0.699179115564311,-0.698343923447362,
-0.697727894595342,-0.697054615184667,-0.696134801679296,-0.693981909072773,
-0.691014472993845,-0.683411980673527,-0.668764816073677,-0.626851623497077,
-0.544816326077868,-0.539653895849157,-0.537731260439277,-0.536598291095981,
-0.535531231102925,-0.534052474615969,-0.531119627625107,-0.509160075740331,
-0.480584905678525,-0.472919564824374,-0.421344772650733,-0.379062284009604,
-0.376646090636205,-0.375749909188097,-0.375117766447727,-0.37452119778218,
-0.37388198845198,-0.373061440047274,-0.369788544786334,-0.364740988205064,
-0.348971260915309,-0.316617121280693,-0.241013005218912,-0.239368640393978,
-0.23375366102006,-0.218721242931479,-0.216145015309578,-0.214598376534375,
-0.21340811279378,-0.212130342967928,-0.210121747339512,-0.203811403693268,
-0.167800535756291,-0.13390336521264,-0.119119785035649,-0.111456026177537,
-0.102609890371343,-0.0568649904542864,-0.0541277106612172,-0.0531836123562101,
-0.0525382162060769,-0.0519458039985288,-0.0513151666505216,-0.0505224083733557,
-0.0493137674931764,-0.0470833369860782,-0.000956627395017071),
 .UNSPECIFIED.);
#831=B_SPLINE_CURVE_WITH_KNOTS('',3,(#46168,#46169,#46170,#46171,#46172,
#46173,#46174,#46175,#46176,#46177,#46178,#46179,#46180,#46181,#46182,#46183,
#46184,#46185,#46186,#46187,#46188,#46189,#46190,#46191,#46192,#46193,#46194,
#46195,#46196,#46197,#46198,#46199,#46200,#46201,#46202,#46203,#46204,#46205,
#46206,#46207,#46208,#46209,#46210,#46211,#46212,#46213,#46214,#46215,#46216,
#46217,#46218,#46219,#46220,#46221,#46222,#46223,#46224,#46225,#46226,#46227,
#46228,#46229,#46230,#46231,#46232,#46233,#46234,#46235,#46236,#46237,#46238,
#46239,#46240,#46241,#46242,#46243,#46244,#46245,#46246,#46247,#46248,#46249,
#46250,#46251,#46252,#46253,#46254,#46255,#46256,#46257,#46258,#46259,#46260,
#46261,#46262,#46263,#46264,#46265,#46266,#46267,#46268,#46269,#46270,#46271,
#46272,#46273,#46274,#46275,#46276,#46277,#46278,#46279,#46280,#46281,#46282,
#46283,#46284,#46285,#46286,#46287,#46288,#46289,#46290,#46291,#46292,#46293,
#46294,#46295,#46296,#46297,#46298,#46299,#46300,#46301,#46302,#46303,#46304,
#46305,#46306,#46307,#46308,#46309,#46310,#46311,#46312,#46313,#46314,#46315,
#46316,#46317,#46318,#46319,#46320,#46321,#46322,#46323,#46324,#46325,#46326,
#46327,#46328,#46329,#46330,#46331,#46332,#46333,#46334,#46335,#46336,#46337,
#46338,#46339,#46340,#46341,#46342,#46343,#46344,#46345,#46346,#46347,#46348,
#46349,#46350,#46351,#46352,#46353,#46354,#46355,#46356,#46357,#46358,#46359,
#46360,#46361,#46362,#46363,#46364,#46365,#46366,#46367,#46368,#46369,#46370,
#46371,#46372,#46373,#46374,#46375,#46376,#46377,#46378,#46379,#46380,#46381,
#46382,#46383,#46384,#46385,#46386,#46387,#46388,#46389,#46390,#46391,#46392,
#46393,#46394,#46395,#46396,#46397,#46398,#46399,#46400,#46401,#46402,#46403,
#46404,#46405,#46406,#46407,#46408,#46409,#46410,#46411,#46412,#46413,#46414,
#46415,#46416,#46417,#46418,#46419,#46420,#46421,#46422,#46423,#46424,#46425,
#46426,#46427,#46428,#46429,#46430,#46431,#46432,#46433,#46434,#46435,#46436,
#46437,#46438,#46439,#46440,#46441,#46442,#46443,#46444,#46445,#46446,#46447,
#46448,#46449,#46450,#46451,#46452,#46453,#46454,#46455,#46456,#46457,#46458,
#46459,#46460,#46461,#46462,#46463,#46464,#46465,#46466,#46467,#46468,#46469,
#46470,#46471,#46472,#46473,#46474,#46475,#46476,#46477,#46478,#46479,#46480,
#46481,#46482,#46483,#46484,#46485,#46486,#46487,#46488,#46489,#46490,#46491,
#46492,#46493,#46494,#46495,#46496,#46497,#46498,#46499,#46500,#46501,#46502,
#46503,#46504,#46505,#46506,#46507,#46508,#46509,#46510,#46511,#46512,#46513,
#46514,#46515,#46516,#46517,#46518,#46519,#46520,#46521,#46522,#46523,#46524,
#46525,#46526,#46527,#46528,#46529,#46530,#46531,#46532,#46533,#46534,#46535,
#46536,#46537,#46538,#46539,#46540,#46541,#46542,#46543,#46544,#46545,#46546,
#46547,#46548,#46549,#46550,#46551,#46552,#46553,#46554,#46555,#46556,#46557,
#46558,#46559,#46560,#46561,#46562,#46563,#46564,#46565,#46566,#46567,#46568,
#46569,#46570,#46571,#46572,#46573,#46574,#46575,#46576,#46577,#46578,#46579,
#46580,#46581,#46582,#46583,#46584,#46585,#46586,#46587,#46588,#46589,#46590,
#46591,#46592,#46593,#46594,#46595,#46596,#46597,#46598,#46599,#46600,#46601,
#46602,#46603,#46604,#46605,#46606,#46607,#46608,#46609,#46610,#46611,#46612,
#46613,#46614,#46615,#46616,#46617,#46618,#46619,#46620,#46621,#46622,#46623,
#46624,#46625,#46626,#46627,#46628,#46629,#46630,#46631,#46632,#46633,#46634,
#46635,#46636,#46637,#46638,#46639,#46640,#46641,#46642,#46643,#46644,#46645,
#46646,#46647,#46648,#46649,#46650,#46651,#46652,#46653,#46654,#46655,#46656,
#46657,#46658,#46659,#46660,#46661,#46662,#46663,#46664,#46665,#46666,#46667,
#46668,#46669,#46670,#46671,#46672,#46673,#46674,#46675,#46676,#46677,#46678,
#46679,#46680,#46681,#46682,#46683,#46684,#46685,#46686,#46687,#46688,#46689,
#46690,#46691,#46692,#46693,#46694,#46695,#46696,#46697,#46698,#46699,#46700,
#46701,#46702,#46703,#46704,#46705,#46706,#46707,#46708,#46709,#46710,#46711,
#46712,#46713,#46714,#46715,#46716,#46717,#46718,#46719,#46720,#46721),
 .UNSPECIFIED.,.F.,.F.,(4,2,2,2,2,2,2,2,2,2,2,2,2,2,2,2,2,2,2,2,2,2,2,2,
2,2,2,2,2,2,2,2,2,2,2,2,2,2,2,2,2,2,2,2,2,2,2,2,2,2,2,2,2,2,2,2,2,2,2,2,
2,2,2,2,2,2,2,2,2,2,2,2,2,2,2,2,2,2,2,2,2,2,2,2,2,2,2,2,2,2,2,2,2,2,2,2,
2,2,2,2,2,2,2,2,2,2,2,2,2,2,2,2,2,2,2,2,2,2,2,2,2,2,2,2,2,2,2,2,2,2,2,2,
2,2,2,2,2,2,2,2,2,2,2,2,2,2,2,2,2,2,2,2,2,2,2,2,2,2,2,2,2,2,2,2,2,2,2,2,
2,2,2,2,2,2,2,2,2,2,2,2,2,2,2,2,2,2,2,2,2,2,2,2,2,2,2,2,2,2,2,2,2,2,2,2,
2,2,2,2,2,2,2,2,2,2,2,2,2,2,2,2,2,2,2,2,2,2,2,2,2,2,2,2,2,2,2,2,2,2,2,2,
2,2,2,2,2,2,2,2,2,2,2,2,2,2,2,2,2,2,2,2,2,2,2,2,2,2,2,2,2,2,2,2,2,2,2,2,
4),(-4.0609788184019,-4.00866642356526,-3.9622189686826,-3.95485125516697,
-3.95272487499133,-3.95142098668034,-3.95023885368475,-3.94872222297658,
-3.94560061967941,-3.92567577860323,-3.91910962273465,-3.84451357365953,
-3.82463915663187,-3.79644211610828,-3.7919166627445,-3.79101266772559,
-3.79034399343397,-3.78967113518626,-3.78905495559564,-3.78821879227068,
-3.78658256831569,-3.77377743525769,-3.74567300673567,-3.7172947752388,
-3.69104820239805,-3.64012326544441,-3.63235344849039,-3.63018614150046,
-3.62887303918123,-3.62769281099133,-3.62619271709054,-3.62325354357833,
-3.60624935277244,-3.60508574413159,-3.53550558301462,-3.50395737138832,
-3.48297147628572,-3.47008198186087,-3.46843116320325,-3.46776383146117,
-3.46709174279417,-3.46647460408832,-3.46563474528434,-3.46355990069386,
-3.44052065177945,-3.42835541185941,-3.36348567029141,-3.31702672563774,
-3.30965775158974,-3.30753115721253,-3.30622717043367,-3.30504496974713,
-3.30352828225823,-3.3004066686601,-3.28048454713631,-3.27493716517512,
-3.2693006994607,-3.22139689263948,-3.16890801158127,-3.1543342565617,-3.1495700940871,
-3.14644015973378,-3.14537195735264,-3.14475745351601,-3.14409732184783,
-3.14325295577327,-3.14146791333144,-3.12942523191849,-3.1279904141707,
-3.12756547711261,-3.12493694457629,-3.11918479294339,-3.04050216464289,
-2.99436248242678,-2.98702362337251,-2.98490022564278,-2.98359698786865,
-2.98241467026504,-2.9808967227992,-2.97776857532028,-2.95770133269436,
-2.95147453944668,-2.87551111338551,-2.82649084827573,-2.82458055885322,
-2.82306933193775,-2.82227626629028,-2.82168394016734,-2.82103846324157,
-2.81989304668468,-2.81650428737606,-2.75605169087254,-2.70782513030004,
-2.69049533933717,-2.66836959595389,-2.66368090849853,-2.66189131865701,
-2.66066098283838,-2.65945751856181,-2.65800933952221,-2.65440284857104,
-2.62014814612835,-2.5554966661241,-2.5028793287234,-2.50075551801354,-2.49983898739581,
-2.49916981475595,-2.49854879982022,-2.49769405472408,-2.49598493500843,
-2.48103202026078,-2.47938604794757,-2.47724620682195,-2.46724122118361,
-2.3953263364527,-2.3490772991632,-2.34172791400156,-2.33960331099505,-2.33829973890291,
-2.33711738442581,-2.33559976116754,-2.33247360129391,-2.31245379295056,
-2.30685210527078,-2.29928541322426,-2.21216400881897,-2.18923797233965,
-2.17930383630521,-2.1777456102822,-2.17693802458532,-2.17628275195416,
-2.17561929287301,-2.17438493261303,-2.17029619948591,-2.09733814828702,
-2.05323732778228,-2.03115804564348,-2.01987506424795,-2.01753554792348,
-2.01604405972935,-2.01486464943839,-2.01354625058169,-2.0113557603419,
-2.00335045118365,-1.94957367917654,-1.90234606560747,-1.85842438290727,
-1.855688818845,-1.8547449541557,-1.85409961332037,-1.85350716850772,-1.85269726983292,
-1.85112798255955,-1.84091089063801,-1.81633934729496,-1.74554443504995,
-1.73456767888231,-1.69886672991483,-1.69558865124381,-1.69400082012411,
-1.69287085927456,-1.69180274295321,-1.69031633837819,-1.68734586074425,
-1.66406133114606,-1.64421743627329,-1.59451983909221,-1.53659719867375,
-1.53532427031233,-1.53291838693435,-1.53202365053207,-1.53139191046668,
-1.5307951968944,-1.52995341029328,-1.52822798223787,-1.51257067267507,
-1.497970204683,-1.39688420716353,-1.39533186032094,-1.37531188201319,-1.37218578383384,
-1.37066820848688,-1.36948589939231,-1.36818238550509,-1.3661003402545,
-1.35909700605417,-1.31616034360945,-1.2432399876416,-1.2122600926433,-1.2100485282218,
-1.20918513583259,-1.20856185162933,-1.20789422535592,-1.20698658023976,
-1.20500534478483,-1.18124167263197,-1.15817381780203,-1.08687740829314,
-1.07631694061834,-1.07095763301991,-1.0697347942762,-1.06881936404228,
-1.05237711931534,-1.04972624040801,-1.04815771076098,-1.046963934731,-1.04569528308365,
-1.0437668637843,-1.03807131887419,-1.00732914871179,-0.941998861679551,
-0.901176518104308,-0.888945650466202,-0.887331016101719,-0.886500371624823,
-0.885885552575492,-0.885211362260221,-0.884267418257439,-0.882048584492347,
-0.861312534551039,-0.840358333536931,-0.783870125826784,-0.73122869800768,
-0.727387367122493,-0.725860220365159,-0.724746391537273,-0.723551221274738,
-0.722377237264457,-0.71962537544249,-0.702558799711768,-0.663949053345918,
-0.626101853298485,-0.568650044098605,-0.565226594825065,-0.564076136958853,
-0.563429622347094,-0.562837485490563,-0.562030072562951,-0.561166054812463,
-0.557281884264004,-0.482338907568888,-0.456611693894247,-0.438171115204648,
-0.429792806267884,-0.423959576314824,-0.407158322533423,-0.40422941604127,
-0.402731467374079,-0.401551403795752,-0.400236905419175,-0.398879849102493,
-0.394344100034094,-0.387899407240713,-0.370455320918639,-0.340726568160529,
-0.315917526678635,-0.246441876297017,-0.242669182214931,-0.241473342321605,
-0.240817664224122,-0.24016770932153,-0.239349317046014,-0.238470025158611,
-0.237054895837823,-0.22200306052267,-0.185840048669332,-0.171380597991612,
-0.156037810867822,-0.0867025073468892,-0.082337101894122,-0.0807241987399237,
-0.0795874328015257,-0.0785217481162206,-0.0770526634393246,-0.075479676809945,
-0.0729574043667461,-0.000957116809526677),.UNSPECIFIED.);
#832=B_SPLINE_CURVE_WITH_KNOTS('',3,(#46723,#46724,#46725,#46726,#46727,
#46728,#46729,#46730,#46731,#46732,#46733),.UNSPECIFIED.,.F.,.F.,(4,1,1,
1,1,1,1,1,4),(210.486707790517,210.519097345163,211.517889748931,212.516682152699,
213.515474556467,214.514266960235,215.513059364003,216.511851767771,216.769890768902),
 .UNSPECIFIED.);
#833=B_SPLINE_CURVE_WITH_KNOTS('',3,(#46735,#46736,#46737,#46738,#46739,
#46740,#46741,#46742,#46743,#46744,#46745,#46746,#46747,#46748,#46749,#46750,
#46751,#46752,#46753,#46754,#46755,#46756,#46757,#46758,#46759,#46760,#46761,
#46762,#46763,#46764,#46765,#46766,#46767,#46768,#46769,#46770,#46771,#46772,
#46773,#46774,#46775,#46776,#46777,#46778,#46779,#46780,#46781,#46782,#46783,
#46784,#46785,#46786,#46787,#46788,#46789,#46790,#46791,#46792,#46793,#46794,
#46795,#46796,#46797,#46798,#46799,#46800,#46801,#46802,#46803,#46804,#46805,
#46806,#46807,#46808,#46809,#46810,#46811,#46812,#46813,#46814,#46815,#46816,
#46817,#46818,#46819,#46820,#46821,#46822,#46823,#46824,#46825,#46826,#46827,
#46828,#46829,#46830,#46831,#46832,#46833,#46834,#46835,#46836,#46837,#46838,
#46839,#46840,#46841,#46842,#46843,#46844,#46845,#46846,#46847,#46848,#46849,
#46850,#46851,#46852,#46853,#46854,#46855,#46856,#46857,#46858,#46859,#46860,
#46861,#46862,#46863,#46864,#46865,#46866,#46867,#46868,#46869,#46870,#46871,
#46872,#46873,#46874,#46875,#46876,#46877,#46878,#46879,#46880,#46881,#46882,
#46883,#46884,#46885,#46886,#46887,#46888,#46889,#46890,#46891,#46892,#46893,
#46894,#46895,#46896,#46897,#46898,#46899,#46900,#46901,#46902,#46903,#46904,
#46905,#46906,#46907,#46908,#46909,#46910,#46911,#46912,#46913,#46914,#46915,
#46916,#46917,#46918,#46919,#46920,#46921,#46922,#46923,#46924,#46925,#46926,
#46927,#46928,#46929,#46930,#46931,#46932,#46933,#46934,#46935,#46936,#46937,
#46938,#46939,#46940,#46941,#46942,#46943,#46944,#46945,#46946,#46947,#46948,
#46949,#46950,#46951,#46952,#46953,#46954,#46955,#46956,#46957,#46958,#46959,
#46960,#46961,#46962,#46963,#46964,#46965,#46966,#46967,#46968,#46969,#46970,
#46971,#46972,#46973,#46974,#46975,#46976,#46977,#46978,#46979,#46980,#46981,
#46982,#46983,#46984,#46985,#46986,#46987,#46988,#46989,#46990,#46991,#46992,
#46993,#46994,#46995,#46996,#46997,#46998,#46999,#47000,#47001,#47002,#47003,
#47004,#47005,#47006,#47007,#47008,#47009,#47010,#47011,#47012,#47013,#47014,
#47015,#47016,#47017,#47018,#47019,#47020,#47021,#47022,#47023,#47024,#47025,
#47026,#47027,#47028,#47029,#47030,#47031,#47032,#47033,#47034,#47035,#47036,
#47037,#47038,#47039,#47040,#47041,#47042,#47043,#47044,#47045,#47046,#47047,
#47048,#47049,#47050,#47051,#47052,#47053,#47054,#47055,#47056,#47057,#47058,
#47059,#47060,#47061,#47062,#47063,#47064,#47065,#47066,#47067,#47068,#47069,
#47070,#47071,#47072,#47073,#47074,#47075,#47076,#47077,#47078,#47079,#47080,
#47081,#47082,#47083,#47084,#47085,#47086,#47087,#47088,#47089,#47090,#47091,
#47092,#47093,#47094,#47095,#47096,#47097,#47098,#47099,#47100,#47101,#47102,
#47103,#47104,#47105,#47106,#47107,#47108,#47109,#47110,#47111,#47112,#47113,
#47114,#47115,#47116,#47117,#47118,#47119,#47120,#47121,#47122,#47123,#47124,
#47125,#47126,#47127,#47128,#47129,#47130,#47131,#47132,#47133,#47134,#47135,
#47136,#47137,#47138,#47139,#47140,#47141,#47142,#47143,#47144,#47145,#47146,
#47147,#47148,#47149,#47150,#47151,#47152,#47153,#47154,#47155,#47156,#47157,
#47158,#47159,#47160,#47161,#47162,#47163,#47164,#47165,#47166,#47167,#47168,
#47169,#47170,#47171,#47172,#47173,#47174,#47175,#47176,#47177,#47178,#47179,
#47180,#47181,#47182,#47183,#47184,#47185,#47186,#47187,#47188,#47189,#47190,
#47191,#47192,#47193,#47194,#47195,#47196,#47197,#47198,#47199,#47200,#47201,
#47202,#47203,#47204,#47205,#47206,#47207,#47208,#47209,#47210,#47211,#47212,
#47213,#47214,#47215,#47216,#47217,#47218,#47219,#47220,#47221,#47222,#47223,
#47224,#47225,#47226,#47227,#47228,#47229,#47230,#47231,#47232,#47233,#47234,
#47235,#47236,#47237,#47238,#47239,#47240,#47241,#47242,#47243,#47244,#47245,
#47246,#47247,#47248,#47249,#47250,#47251,#47252,#47253,#47254,#47255,#47256,
#47257,#47258,#47259,#47260,#47261,#47262,#47263,#47264,#47265,#47266),
 .UNSPECIFIED.,.F.,.F.,(4,2,2,2,2,2,2,2,2,2,2,2,2,2,2,2,2,2,2,2,2,2,2,2,
2,2,2,2,2,2,2,2,2,2,2,2,2,2,2,2,2,2,2,2,2,2,2,2,2,2,2,2,2,2,2,2,2,2,2,2,
2,2,2,2,2,2,2,2,2,2,2,2,2,2,2,2,2,2,2,2,2,2,2,2,2,2,2,2,2,2,2,2,2,2,2,2,
2,2,2,2,2,2,2,2,2,2,2,2,2,2,2,2,2,2,2,2,2,2,2,2,2,2,2,2,2,2,2,2,2,2,2,2,
2,2,2,2,2,2,2,2,2,2,2,2,2,2,2,2,2,2,2,2,2,2,2,2,2,2,2,2,2,2,2,2,2,2,2,2,
2,2,2,2,2,2,2,2,2,2,2,2,2,2,2,2,2,2,2,2,2,2,2,2,2,2,2,2,2,2,2,2,2,2,2,2,
2,2,2,2,2,2,2,2,2,2,2,2,2,2,2,2,2,2,2,2,2,2,2,2,2,2,2,2,2,2,2,2,2,2,2,2,
2,2,2,2,2,2,2,2,2,2,2,2,2,2,2,2,2,2,2,2,2,2,2,2,2,4),(-4.06174778365555,
-3.97407821427973,-3.93332815143193,-3.91576821953131,-3.91298827734529,
-3.91154176535403,-3.91047944312257,-3.90933381163376,-3.90768726084685,
-3.90309868088443,-3.90128705189473,-3.7968662166107,-3.77197426577817,
-3.75865740411268,-3.75419547490943,-3.75219036244142,-3.75107047055428,
-3.75031492793865,-3.74959590326309,-3.7489536188135,-3.74811123050883,
-3.74638173034892,-3.73554974641793,-3.73145347876651,-3.69061690225986,
-3.65180739794179,-3.61077431393014,-3.5931511537124,-3.59036829280424,
-3.58892100383195,-3.58785841927253,-3.58671280138022,-3.58506677492246,
-3.58048288141944,-3.57866526790208,-3.47171092280664,-3.44887812563339,
-3.43586500901309,-3.43147681479097,-3.42949603870758,-3.42838576007372,
-3.42763415577764,-3.42691790025777,-3.42627459984244,-3.42542666417021,
-3.42366972755144,-3.41226049279543,-3.3599373194685,-3.30233937946984,
-3.27682592065431,-3.2692802519617,-3.26713555588305,-3.26582757352176,
-3.26464637963791,-3.26313739178246,-3.26015648102918,-3.24235272231414,
-3.23641911176208,-3.22600132007023,-3.1387927937191,-3.11041445780607,
-3.10761965763419,-3.10619673734846,-3.10531421854298,-3.10450467607211,
-3.10386166914311,-3.10311693510834,-3.1018479120146,-3.09745577830531,
-3.01488994575547,-2.94869918100383,-2.94525399451907,-2.94367485250364,
-2.94248385015836,-2.94136318498728,-2.93980971388008,-2.93666986684746,
-2.90674795862577,-2.89987802721406,-2.81529709026957,-2.78758407885472,
-2.78482697181267,-2.78341803867974,-2.78254135301491,-2.78173594099039,
-2.78109296749668,-2.78034521141131,-2.77906269374259,-2.77454795816053,
-2.67811470950687,-2.63112048038978,-2.62370171375662,-2.62157000240831,
-2.62026490151303,-2.61908301622177,-2.61756857638303,-2.61445810436376,
-2.59477618260641,-2.58930250594203,-2.58298148302896,-2.57546014550829,
-2.49972193863163,-2.47305853847825,-2.46142033155656,-2.45980102699445,
-2.4589808149304,-2.45832476848596,-2.45757108486188,-2.45629508801446,
-2.45169994648714,-2.36452226515802,-2.30510009210387,-2.30030002260929,
-2.29849371525789,-2.29725998200503,-2.29605946051729,-2.29462232539572,
-2.29108217459988,-2.25933473238075,-2.2525732509643,-2.21408312266448,
-2.16672499017184,-2.14759593055792,-2.13859149669784,-2.13707287411684,
-2.13627373765975,-2.1356825371403,-2.13493632085368,-2.13366041418807,
-2.12920516591373,-2.03178623989194,-2.00896333428079,-1.98052293943271,
-1.97707942868522,-1.97551781026475,-1.97432539425451,-1.97305441959847,
-1.97107533607067,-1.96500428674648,-1.87191544085489,-1.82833588508653,
-1.81623548191366,-1.81444806746021,-1.81360328330832,-1.81294314013824,
-1.8122131644932,-1.81100985364388,-1.80672264779518,-1.77763136083035,
-1.69059261305607,-1.68196198475348,-1.67664345115794,-1.65725261470817,
-1.65415594585717,-1.65264435830329,-1.6514629368924,-1.65015654991202,
-1.64801866446179,-1.64053846185211,-1.59286405460848,-1.49732575892265,
-1.4926626513942,-1.49137951690636,-1.49062415903468,-1.48996827858595,
-1.48915036367255,-1.48754223627872,-1.47624249086549,-1.44667590651447,
-1.35094146560641,-1.33422005613513,-1.3312959435933,-1.32979916987074,
-1.32861940222463,-1.32733133220273,-1.32522867923072,-1.32273261500098,
-1.31789439215066,-1.27176851588104,-1.17423652309346,-1.16978371726422,
-1.16850793169171,-1.16776165523788,-1.16717033131905,-1.16637093337437,
-1.16485150288376,-1.15583369120007,-1.13669886303454,-1.08933971745287,
-1.01376294840054,-1.00930586145034,-1.00767880189868,-1.00653818296948,
-1.00537912452925,-1.00390561490426,-1.00229562642329,-0.999685083882543,
-0.994541534144163,-0.94308936070041,-0.858072665365449,-0.847761472937839,
-0.846056923665103,-0.845219286895199,-0.844561523990065,-0.843819133575337,
-0.842560936109431,-0.837694423263264,-0.814521171928508,-0.801118091233252,
-0.698692004858174,-0.690100189746012,-0.686200697117783,-0.684663684219583,
-0.683547295593433,-0.682420036920345,-0.680895677813379,-0.677701107060043,
-0.673534468134852,-0.663855264501745,-0.634474644762605,-0.584539288754084,
-0.527442131871906,-0.525459937638349,-0.523441448586807,-0.522633371478737,
-0.521963250054693,-0.52127129592785,-0.520240220579407,-0.517394766296325,
-0.467966172681365,-0.459924480473994,-0.453025925961595,-0.446982642310207,
-0.38855746526378,-0.383280281586546,-0.366006831476073,-0.36305315022849,
-0.361549871404574,-0.360369203037076,-0.359267130600406,-0.357352664030385,
-0.351748454604558,-0.343338465763197,-0.318344772119302,-0.226191147667687,
-0.202897911910209,-0.200817615268097,-0.199976705905959,-0.199359214191771,
-0.198687170903307,-0.197755130993993,-0.195542679678349,-0.192500375416105,
-0.159484016818544,-0.0764828869227818,-0.0698452084274265,-0.0633781307863137,
-0.04342066476137,-0.0402970536293278,-0.0387798227567039,-0.0375973917206149,
-0.0364959251413158,-0.0352169765653819,-0.0333966675439099,-0.0302788094196745,
-0.000956542473226251),.UNSPECIFIED.);
#834=B_SPLINE_CURVE_WITH_KNOTS('',3,(#47268,#47269,#47270,#47271,#47272,
#47273,#47274,#47275,#47276,#47277,#47278,#47279,#47280,#47281,#47282,#47283,
#47284,#47285,#47286,#47287,#47288,#47289,#47290,#47291,#47292,#47293,#47294,
#47295,#47296,#47297,#47298,#47299,#47300,#47301,#47302,#47303,#47304,#47305,
#47306,#47307,#47308,#47309,#47310,#47311,#47312,#47313,#47314,#47315,#47316,
#47317,#47318,#47319,#47320,#47321,#47322,#47323,#47324,#47325,#47326,#47327,
#47328,#47329,#47330,#47331,#47332,#47333,#47334,#47335,#47336,#47337,#47338,
#47339,#47340,#47341,#47342,#47343,#47344,#47345,#47346,#47347,#47348,#47349,
#47350,#47351,#47352,#47353,#47354,#47355,#47356,#47357,#47358,#47359,#47360,
#47361,#47362,#47363,#47364,#47365,#47366,#47367,#47368,#47369,#47370,#47371,
#47372,#47373,#47374,#47375,#47376,#47377,#47378,#47379,#47380,#47381,#47382,
#47383,#47384,#47385,#47386,#47387,#47388,#47389,#47390,#47391,#47392,#47393,
#47394,#47395,#47396,#47397,#47398,#47399,#47400,#47401,#47402,#47403,#47404,
#47405,#47406,#47407,#47408,#47409,#47410,#47411,#47412,#47413,#47414,#47415,
#47416,#47417,#47418,#47419,#47420,#47421,#47422,#47423,#47424,#47425,#47426,
#47427,#47428,#47429,#47430,#47431,#47432,#47433,#47434,#47435,#47436,#47437,
#47438,#47439,#47440,#47441,#47442,#47443,#47444,#47445,#47446,#47447,#47448,
#47449,#47450,#47451,#47452,#47453,#47454,#47455,#47456,#47457,#47458,#47459,
#47460,#47461,#47462,#47463,#47464,#47465,#47466,#47467,#47468,#47469,#47470,
#47471,#47472,#47473,#47474,#47475,#47476,#47477,#47478,#47479,#47480,#47481,
#47482,#47483,#47484,#47485,#47486,#47487,#47488,#47489,#47490,#47491,#47492,
#47493,#47494,#47495,#47496,#47497,#47498,#47499,#47500,#47501,#47502,#47503,
#47504,#47505,#47506,#47507,#47508,#47509,#47510,#47511,#47512,#47513,#47514,
#47515,#47516,#47517,#47518,#47519,#47520,#47521,#47522,#47523,#47524,#47525,
#47526,#47527,#47528,#47529,#47530,#47531,#47532,#47533,#47534,#47535,#47536,
#47537,#47538,#47539,#47540,#47541,#47542,#47543,#47544,#47545,#47546,#47547,
#47548,#47549,#47550,#47551,#47552,#47553,#47554,#47555,#47556,#47557,#47558,
#47559,#47560,#47561,#47562,#47563,#47564,#47565,#47566,#47567,#47568,#47569,
#47570,#47571,#47572,#47573,#47574,#47575,#47576,#47577,#47578,#47579,#47580,
#47581,#47582,#47583,#47584,#47585,#47586,#47587,#47588,#47589,#47590,#47591,
#47592,#47593,#47594,#47595,#47596,#47597,#47598,#47599,#47600,#47601,#47602,
#47603,#47604,#47605,#47606,#47607,#47608,#47609,#47610,#47611,#47612,#47613,
#47614,#47615,#47616,#47617,#47618,#47619,#47620,#47621,#47622,#47623,#47624,
#47625,#47626,#47627,#47628,#47629,#47630,#47631,#47632,#47633,#47634,#47635,
#47636,#47637,#47638,#47639,#47640,#47641,#47642,#47643,#47644,#47645,#47646,
#47647,#47648,#47649,#47650,#47651,#47652,#47653,#47654,#47655,#47656,#47657,
#47658,#47659,#47660,#47661,#47662,#47663,#47664,#47665,#47666,#47667,#47668,
#47669,#47670,#47671,#47672,#47673,#47674,#47675,#47676,#47677,#47678,#47679,
#47680,#47681,#47682,#47683,#47684,#47685,#47686,#47687,#47688,#47689,#47690,
#47691,#47692,#47693,#47694,#47695,#47696,#47697,#47698,#47699,#47700,#47701,
#47702,#47703,#47704,#47705,#47706,#47707,#47708,#47709,#47710,#47711,#47712,
#47713,#47714,#47715,#47716,#47717,#47718,#47719,#47720,#47721,#47722,#47723,
#47724,#47725,#47726,#47727,#47728,#47729,#47730,#47731,#47732,#47733,#47734,
#47735,#47736,#47737,#47738,#47739,#47740,#47741,#47742,#47743,#47744,#47745,
#47746,#47747,#47748,#47749,#47750,#47751,#47752,#47753,#47754,#47755,#47756,
#47757,#47758,#47759,#47760,#47761,#47762,#47763,#47764,#47765,#47766,#47767,
#47768,#47769,#47770,#47771,#47772,#47773,#47774,#47775,#47776,#47777,#47778,
#47779,#47780,#47781,#47782,#47783,#47784,#47785,#47786,#47787,#47788,#47789,
#47790,#47791,#47792,#47793,#47794,#47795,#47796,#47797,#47798,#47799),
 .UNSPECIFIED.,.F.,.F.,(4,2,2,2,2,2,2,2,2,2,2,2,2,2,2,2,2,2,2,2,2,2,2,2,
2,2,2,2,2,2,2,2,2,2,2,2,2,2,2,2,2,2,2,2,2,2,2,2,2,2,2,2,2,2,2,2,2,2,2,2,
2,2,2,2,2,2,2,2,2,2,2,2,2,2,2,2,2,2,2,2,2,2,2,2,2,2,2,2,2,2,2,2,2,2,2,2,
2,2,2,2,2,2,2,2,2,2,2,2,2,2,2,2,2,2,2,2,2,2,2,2,2,2,2,2,2,2,2,2,2,2,2,2,
2,2,2,2,2,2,2,2,2,2,2,2,2,2,2,2,2,2,2,2,2,2,2,2,2,2,2,2,2,2,2,2,2,2,2,2,
2,2,2,2,2,2,2,2,2,2,2,2,2,2,2,2,2,2,2,2,2,2,2,2,2,2,2,2,2,2,2,2,2,2,2,2,
2,2,2,2,2,2,2,2,2,2,2,2,2,2,2,2,2,2,2,2,2,2,2,2,2,2,2,2,2,2,2,2,2,2,2,2,
2,2,2,2,2,2,2,2,2,2,2,2,2,2,2,2,2,2,2,2,2,2,2,2,2,4),(-4.06096092462694,
-3.97919081284745,-3.94033500558184,-3.93805777042456,-3.93711465117569,
-3.93644048212338,-3.93582527337599,-3.93499352137346,-3.9333750346416,
-3.92106458908294,-3.91985519612799,-3.91901773292882,-3.91098115606398,
-3.81779744927564,-3.7925796260781,-3.78411144645442,-3.77847919840453,
-3.77655910402029,-3.77545667801708,-3.77427619058045,-3.77277588947607,
-3.76983669382993,-3.75284089231725,-3.74908203550039,-3.70284492101176,
-3.67125287897349,-3.62158546829895,-3.61606029256375,-3.61474721828114,
-3.61399259013788,-3.61333648551473,-3.61251718684841,-3.61124896035528,
-3.60543924597834,-3.49807606421452,-3.47068586556569,-3.46165372547933,
-3.4576955395516,-3.45463431840227,-3.45313499416033,-3.45200085814923,
-3.4508743372669,-3.4492991686473,-3.44516953008477,-3.3749519331859,-3.33250984507165,
-3.29782268325609,-3.29308893409011,-3.29184277570622,-3.29110312769775,
-3.29044496090269,-3.28960301255844,-3.2879338939263,-3.27790650441158,
-3.23332785876528,-3.14265283140812,-3.13670464526738,-3.13379964360183,
-3.1320670656346,-3.13050457567412,-3.12933354947813,-3.12822215533321,
-3.12670423181934,-3.12291646816968,-3.07486489963749,-3.00935084624,-2.98278616443645,
-2.97102064211608,-2.9693972220211,-2.96857615633364,-2.96792003390814,
-2.96716693740208,-2.96589347977399,-2.96132245636345,-2.87343455784002,
-2.81377925554977,-2.81096567830702,-2.80927104058542,-2.8077339113591,
-2.80656621012,-2.80544657157215,-2.80389692980886,-2.80077232391329,-2.77142101164101,
-2.70065042425994,-2.67527034076667,-2.65129433730004,-2.64747264838896,
-2.64631851734601,-2.64559953061925,-2.64493605350787,-2.64406885382279,
-2.64216338063635,-2.62698734961467,-2.6239264351805,-2.52767801945915,
-2.49364925344703,-2.48755539849178,-2.48557344872218,-2.48430180735438,
-2.48310959893817,-2.48154945241806,-2.4789266715549,-2.46301935409514,
-2.45825570391109,-2.45659282719115,-2.4478634850003,-2.36333676902471,
-2.32955878393936,-2.32647953231094,-2.32424596611931,-2.32331046004482,
-2.32263790868039,-2.32202139904669,-2.32118391109189,-2.31954249215766,
-2.30659127209733,-2.22404316406299,-2.16729451034805,-2.16389025215467,
-2.16231889678326,-2.16112917563126,-2.1600063256552,-2.15813446347704,
-2.15329062032496,-2.07740918849232,-2.0305643032039,-2.00372512134957,
-2.00157821529496,-2.00072596041949,-2.00010565285986,-1.99943613202562,
-1.99851721985672,-1.99637943581422,-1.96270500880362,-1.90382748872865,
-1.84548459933442,-1.84159870500729,-1.84006411146326,-1.83894845067498,
-1.83775470009993,-1.83615805739424,-1.83261862684281,-1.82792991562823,
-1.78424142083256,-1.69117083407885,-1.68033281081321,-1.67860208995183,
-1.67775928122458,-1.67710102742307,-1.67636190541698,-1.67511807014486,
-1.67040958034455,-1.6360724371505,-1.5353607953123,-1.53302452807617,-1.53086549361769,
-1.52306053400685,-1.51887907574776,-1.51729563335629,-1.5161669891372,
-1.5149799365889,-1.51342677422842,-1.51011814444593,-1.46638725455222,
-1.36703319645439,-1.35735260342995,-1.35570139520562,-1.35486325784665,
-1.35420548032741,-1.35346348126207,-1.35223209496953,-1.34762653656585,
-1.31446555010206,-1.24170156206602,-1.22297656488153,-1.21789899329235,
-1.19856427264209,-1.1954696696151,-1.1939582600312,-1.19277659894218,-1.19146955989951,
-1.18932972913495,-1.18201513977918,-1.13580444033686,-1.06350016492354,
-1.05107270995833,-1.04795365866589,-1.03491309958993,-1.03310961117931,
-1.03224885488227,-1.03158628353944,-1.03086410996496,-1.02971955350319,
-1.02597361674185,-1.00261460985047,-0.940962288820962,-0.877193553653152,
-0.873286853876515,-0.871748551065455,-0.870631766515194,-0.86943828813933,
-0.867844549661155,-0.864413867689255,-0.796413570174008,-0.749673593210714,
-0.734915281116713,-0.730123414619615,-0.727544333706052,-0.712341835463116,
-0.710435256216269,-0.709567770414391,-0.708904165946427,-0.708185134751287,
-0.70705427062878,-0.703426334404997,-0.697658431284722,-0.678985762418818,
-0.630851046052793,-0.592942186412587,-0.591456976229329,-0.578840357702262,
-0.573267665794149,-0.553286287470415,-0.55016159218077,-0.548644149694129,
-0.547461696208307,-0.546157771458345,-0.544032045744125,-0.536822288208567,
-0.501335979505161,-0.444284655203243,-0.399570296274313,-0.389411811306336,
-0.387714827289933,-0.38687872657509,-0.386221141160508,-0.385477839332605,
-0.384703735225948,-0.381994031174152,-0.378028633093763,-0.36671474966148,
-0.339395872545463,-0.315836239073396,-0.233629652658549,-0.228454237645428,
-0.226529667729118,-0.225396348703753,-0.224329473870766,-0.222851786464301,
-0.219923980427594,-0.201887954758125,-0.157677129325545,-0.141943403594944,
-0.134109145857688,-0.124858185245046,-0.0689282052345134,-0.0657149562395191,
-0.064594021162722,-0.0639534146177227,-0.063359765784039,-0.062726389614209,
-0.0619244189171355,-0.0606938192310203,-0.0584068393442843,-0.000956966008258823),
 .UNSPECIFIED.);
#835=B_SPLINE_CURVE_WITH_KNOTS('',3,(#47801,#47802,#47803,#47804,#47805,
#47806,#47807,#47808,#47809,#47810,#47811,#47812,#47813,#47814,#47815,#47816,
#47817,#47818,#47819,#47820,#47821,#47822,#47823,#47824,#47825,#47826,#47827,
#47828,#47829,#47830,#47831,#47832,#47833,#47834,#47835,#47836,#47837,#47838,
#47839,#47840,#47841,#47842,#47843,#47844,#47845,#47846,#47847,#47848,#47849,
#47850,#47851,#47852,#47853,#47854,#47855,#47856,#47857,#47858,#47859,#47860,
#47861,#47862,#47863,#47864,#47865,#47866,#47867,#47868,#47869,#47870,#47871,
#47872,#47873,#47874,#47875,#47876,#47877,#47878,#47879,#47880,#47881,#47882,
#47883,#47884,#47885,#47886,#47887,#47888,#47889,#47890,#47891,#47892,#47893,
#47894,#47895,#47896,#47897,#47898,#47899,#47900,#47901,#47902,#47903,#47904,
#47905,#47906,#47907,#47908,#47909,#47910,#47911,#47912,#47913,#47914,#47915,
#47916,#47917,#47918,#47919,#47920,#47921,#47922,#47923,#47924,#47925,#47926,
#47927,#47928,#47929,#47930,#47931,#47932,#47933,#47934,#47935,#47936,#47937,
#47938,#47939,#47940,#47941,#47942,#47943,#47944,#47945,#47946,#47947,#47948,
#47949,#47950,#47951,#47952,#47953,#47954,#47955,#47956,#47957,#47958,#47959,
#47960,#47961,#47962,#47963,#47964,#47965,#47966,#47967,#47968,#47969,#47970,
#47971,#47972,#47973,#47974,#47975,#47976,#47977,#47978,#47979,#47980,#47981,
#47982,#47983,#47984,#47985,#47986,#47987,#47988,#47989,#47990,#47991,#47992,
#47993,#47994,#47995,#47996,#47997,#47998,#47999,#48000,#48001,#48002,#48003,
#48004,#48005,#48006,#48007,#48008,#48009,#48010,#48011,#48012,#48013,#48014,
#48015,#48016,#48017,#48018,#48019,#48020,#48021,#48022,#48023,#48024,#48025,
#48026,#48027,#48028,#48029,#48030,#48031,#48032,#48033,#48034,#48035,#48036,
#48037,#48038,#48039,#48040,#48041,#48042,#48043,#48044,#48045,#48046,#48047,
#48048,#48049,#48050,#48051,#48052,#48053,#48054,#48055,#48056,#48057,#48058,
#48059,#48060,#48061,#48062,#48063,#48064,#48065,#48066,#48067,#48068,#48069,
#48070,#48071,#48072,#48073,#48074,#48075,#48076,#48077,#48078,#48079,#48080,
#48081,#48082,#48083,#48084,#48085,#48086,#48087,#48088,#48089,#48090,#48091,
#48092,#48093,#48094,#48095,#48096,#48097,#48098,#48099,#48100,#48101,#48102,
#48103,#48104,#48105,#48106,#48107,#48108,#48109,#48110,#48111,#48112,#48113,
#48114,#48115,#48116,#48117,#48118,#48119,#48120,#48121,#48122,#48123,#48124,
#48125,#48126,#48127,#48128,#48129,#48130,#48131,#48132,#48133,#48134,#48135,
#48136,#48137,#48138,#48139,#48140,#48141,#48142,#48143,#48144,#48145,#48146,
#48147,#48148,#48149,#48150,#48151,#48152,#48153,#48154,#48155,#48156,#48157,
#48158,#48159,#48160,#48161,#48162,#48163,#48164,#48165,#48166,#48167,#48168,
#48169,#48170,#48171,#48172,#48173,#48174,#48175,#48176,#48177,#48178,#48179,
#48180,#48181,#48182,#48183,#48184,#48185,#48186,#48187,#48188,#48189,#48190,
#48191,#48192,#48193,#48194,#48195,#48196,#48197,#48198,#48199,#48200,#48201,
#48202,#48203,#48204,#48205,#48206,#48207,#48208,#48209,#48210,#48211,#48212,
#48213,#48214,#48215,#48216,#48217,#48218,#48219,#48220,#48221,#48222,#48223,
#48224,#48225,#48226,#48227,#48228,#48229,#48230,#48231,#48232,#48233,#48234,
#48235,#48236,#48237,#48238,#48239,#48240,#48241,#48242,#48243,#48244,#48245,
#48246,#48247,#48248,#48249,#48250,#48251,#48252,#48253,#48254,#48255,#48256,
#48257,#48258,#48259,#48260,#48261,#48262,#48263,#48264,#48265,#48266,#48267,
#48268,#48269,#48270,#48271,#48272,#48273,#48274,#48275,#48276,#48277,#48278,
#48279,#48280,#48281,#48282,#48283,#48284,#48285,#48286,#48287,#48288,#48289,
#48290,#48291,#48292,#48293,#48294,#48295,#48296,#48297,#48298,#48299,#48300,
#48301,#48302,#48303,#48304,#48305,#48306,#48307,#48308,#48309,#48310,#48311,
#48312,#48313,#48314,#48315,#48316,#48317,#48318,#48319,#48320,#48321,#48322,
#48323,#48324,#48325,#48326,#48327,#48328,#48329,#48330,#48331,#48332,#48333,
#48334,#48335,#48336,#48337,#48338,#48339,#48340,#48341,#48342,#48343,#48344,
#48345,#48346,#48347,#48348),.UNSPECIFIED.,.F.,.F.,(4,2,2,2,2,2,2,2,2,2,
2,2,2,2,2,2,2,2,2,2,2,2,2,2,2,2,2,2,2,2,2,2,2,2,2,2,2,2,2,2,2,2,2,2,2,2,
2,2,2,2,2,2,2,2,2,2,2,2,2,2,2,2,2,2,2,2,2,2,2,2,2,2,2,2,2,2,2,2,2,2,2,2,
2,2,2,2,2,2,2,2,2,2,2,2,2,2,2,2,2,2,2,2,2,2,2,2,2,2,2,2,2,2,2,2,2,2,2,2,
2,2,2,2,2,2,2,2,2,2,2,2,2,2,2,2,2,2,2,2,2,2,2,2,2,2,2,2,2,2,2,2,2,2,2,2,
2,2,2,2,2,2,2,2,2,2,2,2,2,2,2,2,2,2,2,2,2,2,2,2,2,2,2,2,2,2,2,2,2,2,2,2,
2,2,2,2,2,2,2,2,2,2,2,2,2,2,2,2,2,2,2,2,2,2,2,2,2,2,2,2,2,2,2,2,2,2,2,2,
2,2,2,2,2,2,2,2,2,2,2,2,2,2,2,2,2,2,2,2,2,2,2,2,2,2,2,2,2,2,2,2,2,2,2,2,
2,2,2,2,2,2,2,2,2,2,2,4),(-4.06063664256222,-3.9728178653946,-3.96817330428761,
-3.9657507498166,-3.96367747480607,-3.96238573583193,-3.96120092584095,
-3.95968695719411,-3.95649406725477,-3.93493627213538,-3.86545558219806,
-3.84400846894577,-3.81634787817368,-3.8037176287448,-3.80255261287607,
-3.80177826638475,-3.80103490784806,-3.80037775516869,-3.79954284817197,
-3.79785045644931,-3.78776924566413,-3.74314913233184,-3.7028571063676,
-3.66212385612992,-3.64458691523146,-3.64179477780974,-3.64034562897998,
-3.63928290790934,-3.63813832268918,-3.6364957850218,-3.63193437846331,
-3.55354239276756,-3.52026447987411,-3.49539654248139,-3.48590024901914,
-3.48062133497725,-3.47932741146448,-3.47869710940945,-3.47810498614432,
-3.47745975370476,-3.47651564343172,-3.47377661279283,-3.42957611463609,
-3.37789844381286,-3.33913756950115,-3.32787573899105,-3.32321367863729,
-3.31969049779254,-3.31809707691609,-3.31690406525402,-3.31578788249488,
-3.31425066783107,-3.31034810324101,-3.2479466649981,-3.24466367312895,
-3.19705334943805,-3.17066212060436,-3.16805341048395,-3.16175651348737,
-3.15787657825751,-3.15671772812344,-3.15599250547556,-3.1553312746245,
-3.15447785933283,-3.15264481825705,-3.13942692546299,-3.13706519897787,
-3.13629580488889,-3.13273989195526,-3.13070018276657,-3.1187752230506,
-3.05039087455928,-3.00554675310395,-3.00078645005306,-2.9972036889808,
-2.99559930268966,-2.99440450141676,-2.99329127127823,-2.99176534197486,
-2.98792914036917,-2.93567331288154,-2.86966758136114,-2.83977626819666,
-2.83689812605837,-2.83480204324943,-2.83388997418697,-2.83321841567928,
-2.83260107284997,-2.83175993863321,-2.82967693439173,-2.80620846151174,
-2.79530017976929,-2.75282523622438,-2.70939755154346,-2.68361732756857,
-2.67855896665505,-2.67479709393872,-2.67316032287313,-2.67195990608139,
-2.67085448896474,-2.669359198528,-2.66644780319447,-2.64389122647826,-2.62797009405563,
-2.54168710712269,-2.5225670373368,-2.51343885502548,-2.51191480693229,
-2.51111456304351,-2.51052329827946,-2.50987330853131,-2.50870509694854,
-2.50514482550405,-2.4452942361457,-2.39638309240506,-2.35595728609159,
-2.35219227850474,-2.35055484572774,-2.3493542133943,-2.34824878701673,
-2.34675377107795,-2.34384375240974,-2.32133066419765,-2.3093759256781,
-2.30651133911038,-2.22614148173872,-2.21306479921595,-2.19807704877291,
-2.19069577436681,-2.18925930575926,-2.18847776658479,-2.18788798960529,
-2.18722683183057,-2.18600341058304,-2.18200512326269,-2.10839354612462,
-2.06456239763841,-2.04285411725367,-2.03128814812829,-2.02906211760091,
-2.02760605098205,-2.02643017420149,-2.02508932024748,-2.02279745460101,
-2.01366457292012,-1.92301641362903,-1.87843044210397,-1.86841663284503,
-1.86674832126655,-1.86590659186958,-1.86524850416418,-1.86450884435705,
-1.86326243714262,-1.85852509452477,-1.8237926680234,-1.75920738999232,
-1.74209262665134,-1.71032180766946,-1.70678084090183,-1.70534352766242,
-1.70414291693203,-1.70290915482323,-1.70110292152006,-1.69630372436184,
-1.63685608857803,-1.54954496195863,-1.54502339463764,-1.54374008332427,
-1.54299211938131,-1.54240099736511,-1.54160383661386,-1.54009500073034,
-1.53130980242522,-1.51252239106176,-1.46831150343087,-1.38934816350616,
-1.38462112602489,-1.38276810689587,-1.3816487374047,-1.38045680590794,
-1.37887250440868,-1.37547991775868,-1.37098840600033,-1.330394282525,-1.24904970785202,
-1.22368995246028,-1.22156928119658,-1.22072139781746,-1.22010212265929,
-1.21943153754818,-1.218526009025,-1.21644407536694,-1.21360312740583,-1.18440561095295,
-1.11378335987303,-1.09698358280725,-1.09103226273566,-1.08359681820421,
-1.06416544494335,-1.06106615847322,-1.05955375610123,-1.05837190877296,
-1.05706526618667,-1.05492745070177,-1.04762253296447,-1.00153532937066,
-0.940726580746427,-0.910788015951101,-0.900344788758057,-0.898633567308237,
-0.897794598631607,-0.897136701931812,-0.896395142303076,-0.89516580761412,
-0.890753706111515,-0.883241711181622,-0.853749490623139,-0.803324583181019,
-0.742812467511629,-0.73891469103731,-0.737377850468346,-0.736261410874336,
-0.735067629084746,-0.733472327651497,-0.730057724747939,-0.705652102521991,
-0.684040781967298,-0.632371602551695,-0.587717762908069,-0.57766970465921,
-0.57599943593632,-0.57515719891526,-0.574498950271726,-0.57375936200942,
-0.572990538453649,-0.570363704605121,-0.542260763949439,-0.495407151417223,
-0.421281763420022,-0.416570350297911,-0.41490486562672,-0.41375357292122,
-0.41269182850815,-0.411254918768642,-0.409726510486734,-0.40303963017123,
-0.392491121041141,-0.361153547439554,-0.338623823357926,-0.315775038181721,
-0.293356939098674,-0.27708334631547,-0.274302794911084,-0.270004373124783,
-0.25534124621658,-0.253641393744814,-0.252788972599971,-0.252168549433432,
-0.251498909276072,-0.250579842701529,-0.249560258049507,-0.242554944214925,
-0.205199585427156,-0.192062276384384,-0.178004956326378,-0.0987760072086423,
-0.0939756485195223,-0.0921106418679364,-0.0909889742155074,-0.0897983089261329,
-0.0882219927980785,-0.0865006229289555,-0.0836227576680198,-0.000957501929126401),
 .UNSPECIFIED.);
#836=B_SPLINE_CURVE_WITH_KNOTS('',3,(#48350,#48351,#48352,#48353,#48354,
#48355,#48356,#48357,#48358,#48359,#48360,#48361,#48362,#48363,#48364,#48365,
#48366,#48367,#48368,#48369,#48370,#48371,#48372,#48373,#48374,#48375,#48376,
#48377,#48378,#48379,#48380,#48381,#48382,#48383,#48384,#48385,#48386,#48387,
#48388,#48389,#48390,#48391,#48392,#48393,#48394,#48395,#48396,#48397,#48398,
#48399,#48400,#48401,#48402,#48403,#48404,#48405,#48406,#48407,#48408,#48409,
#48410,#48411,#48412,#48413,#48414,#48415,#48416,#48417,#48418,#48419,#48420,
#48421,#48422,#48423,#48424,#48425,#48426,#48427,#48428,#48429,#48430,#48431,
#48432,#48433,#48434,#48435,#48436,#48437,#48438,#48439,#48440,#48441,#48442,
#48443,#48444,#48445,#48446,#48447,#48448,#48449,#48450,#48451,#48452,#48453,
#48454,#48455,#48456,#48457,#48458,#48459,#48460,#48461,#48462,#48463,#48464,
#48465,#48466,#48467,#48468,#48469,#48470,#48471,#48472,#48473,#48474,#48475,
#48476,#48477,#48478,#48479,#48480,#48481,#48482,#48483,#48484,#48485,#48486,
#48487,#48488,#48489,#48490,#48491,#48492,#48493,#48494,#48495,#48496,#48497,
#48498,#48499,#48500,#48501,#48502,#48503,#48504,#48505,#48506,#48507,#48508,
#48509,#48510,#48511,#48512,#48513,#48514,#48515,#48516,#48517,#48518,#48519,
#48520,#48521,#48522,#48523,#48524,#48525,#48526,#48527,#48528,#48529,#48530,
#48531,#48532,#48533,#48534,#48535,#48536,#48537,#48538,#48539,#48540,#48541,
#48542,#48543,#48544,#48545,#48546,#48547,#48548,#48549,#48550,#48551,#48552,
#48553,#48554,#48555,#48556,#48557,#48558,#48559,#48560,#48561,#48562,#48563,
#48564,#48565,#48566,#48567,#48568,#48569,#48570,#48571,#48572,#48573,#48574,
#48575,#48576,#48577,#48578,#48579,#48580,#48581,#48582,#48583,#48584,#48585,
#48586,#48587,#48588,#48589,#48590,#48591,#48592,#48593,#48594,#48595,#48596,
#48597,#48598,#48599,#48600,#48601,#48602,#48603,#48604,#48605,#48606,#48607,
#48608,#48609,#48610,#48611,#48612,#48613,#48614,#48615,#48616,#48617,#48618,
#48619,#48620,#48621,#48622,#48623,#48624,#48625,#48626,#48627,#48628,#48629,
#48630,#48631,#48632,#48633,#48634,#48635,#48636,#48637,#48638,#48639,#48640,
#48641,#48642,#48643,#48644,#48645,#48646,#48647,#48648,#48649,#48650,#48651,
#48652,#48653,#48654,#48655,#48656,#48657,#48658,#48659,#48660,#48661,#48662,
#48663,#48664,#48665,#48666,#48667,#48668,#48669,#48670,#48671,#48672,#48673,
#48674,#48675,#48676,#48677,#48678,#48679,#48680,#48681,#48682,#48683,#48684,
#48685,#48686,#48687,#48688,#48689,#48690,#48691,#48692,#48693,#48694,#48695,
#48696,#48697,#48698,#48699,#48700,#48701,#48702,#48703,#48704,#48705,#48706,
#48707,#48708,#48709,#48710,#48711,#48712,#48713,#48714,#48715,#48716,#48717,
#48718,#48719,#48720,#48721,#48722,#48723,#48724,#48725,#48726,#48727,#48728,
#48729,#48730,#48731,#48732,#48733,#48734,#48735,#48736,#48737,#48738,#48739,
#48740,#48741,#48742,#48743,#48744,#48745,#48746,#48747,#48748,#48749,#48750,
#48751,#48752,#48753,#48754,#48755,#48756,#48757,#48758,#48759,#48760,#48761,
#48762,#48763,#48764,#48765,#48766,#48767,#48768,#48769,#48770,#48771,#48772,
#48773,#48774,#48775,#48776,#48777,#48778,#48779,#48780,#48781,#48782,#48783,
#48784,#48785,#48786,#48787,#48788,#48789,#48790,#48791,#48792,#48793,#48794,
#48795,#48796,#48797,#48798,#48799,#48800,#48801,#48802,#48803,#48804,#48805,
#48806,#48807,#48808,#48809,#48810,#48811,#48812,#48813,#48814,#48815,#48816,
#48817,#48818,#48819,#48820,#48821,#48822,#48823,#48824,#48825,#48826,#48827,
#48828,#48829,#48830,#48831,#48832,#48833,#48834,#48835,#48836,#48837,#48838,
#48839,#48840,#48841,#48842,#48843,#48844,#48845,#48846,#48847,#48848,#48849,
#48850,#48851,#48852,#48853,#48854,#48855,#48856,#48857,#48858,#48859,#48860,
#48861,#48862,#48863,#48864,#48865,#48866,#48867,#48868,#48869,#48870,#48871,
#48872,#48873,#48874,#48875,#48876,#48877,#48878,#48879,#48880,#48881,#48882,
#48883),.UNSPECIFIED.,.F.,.F.,(4,2,2,2,2,2,2,2,2,2,2,2,2,2,2,2,2,2,2,2,
2,2,2,2,2,2,2,2,2,2,2,2,2,2,2,2,2,2,2,2,2,2,2,2,2,2,2,2,2,2,2,2,2,2,2,2,
2,2,2,2,2,2,2,2,2,2,2,2,2,2,2,2,2,2,2,2,2,2,2,2,2,2,2,2,2,2,2,2,2,2,2,2,
2,2,2,2,2,2,2,2,2,2,2,2,2,2,2,2,2,2,2,2,2,2,2,2,2,2,2,2,2,2,2,2,2,2,2,2,
2,2,2,2,2,2,2,2,2,2,2,2,2,2,2,2,2,2,2,2,2,2,2,2,2,2,2,2,2,2,2,2,2,2,2,2,
2,2,2,2,2,2,2,2,2,2,2,2,2,2,2,2,2,2,2,2,2,2,2,2,2,2,2,2,2,2,2,2,2,2,2,2,
2,2,2,2,2,2,2,2,2,2,2,2,2,2,2,2,2,2,2,2,2,2,2,2,2,2,2,2,2,2,2,2,2,2,2,2,
2,2,2,2,2,2,2,2,2,2,2,2,2,2,2,2,2,2,2,2,2,2,2,2,2,2,2,2,2,2,4),(-4.05990386301481,
-3.99809978947004,-3.99329731683281,-3.99118058419593,-3.99001654462979,
-3.98924255633462,-3.98849941570817,-3.98784209154762,-3.98700648300469,
-3.98531103532073,-3.97517420561014,-3.91790465072373,-3.90349953819912,
-3.88952171232384,-3.85022696325981,-3.83220288589521,-3.83015917988238,
-3.8283518218361,-3.82711796754219,-3.82591778855667,-3.82448161296133,
-3.82094664451944,-3.78937563652594,-3.74241734817476,-3.70107118295529,
-3.67842030014143,-3.67186269223417,-3.66786055663566,-3.66698856612843,
-3.66617548566487,-3.6655828384482,-3.66493938266889,-3.66380357887516,
-3.66048214296812,-3.60021574213842,-3.54785805956159,-3.51554597851715,
-3.50831024070987,-3.50674610250057,-3.50528349867359,-3.50421894217199,
-3.50308000412431,-3.50145837970363,-3.49703494125092,-3.42735988875566,
-3.36958128648223,-3.35788674054822,-3.34999530397017,-3.34694611635174,
-3.34474696217604,-3.34380756220566,-3.34313433951493,-3.34251875596786,
-3.34168473033736,-3.34005661562455,-3.32746495053866,-3.32451647161291,
-3.32404258249264,-3.28871981961329,-3.23098335755258,-3.2119967744143,
-3.18802299072834,-3.18456695288459,-3.18296869510608,-3.18177473915713,
-3.18065961025899,-3.17912688121026,-3.17525165366302,-3.11857540687163,
-3.05358203563633,-3.0267980218711,-3.02409466204222,-3.02209086728244,
-3.02119040572553,-3.02052407569213,-3.01989898649335,-3.01902854539786,
-3.01677425456922,-2.98239576250505,-2.91469295678513,-2.89156866853065,
-2.86574662930738,-2.86208326201571,-2.86044439034833,-2.85924347024299,
-2.85813831662987,-2.8566444845232,-2.85373915870461,-2.83135527151072,
-2.81617070534995,-2.73789931218056,-2.71144423867707,-2.70084225317016,
-2.69926353447726,-2.6984450634278,-2.69779520564332,-2.6970425788064,-2.695770956751,
-2.69121656660287,-2.60047483629661,-2.56784767512706,-2.5446312311509,
-2.53980539856664,-2.53799531628337,-2.53676085042842,-2.5355610380772,
-2.53412644758612,-2.53060124549272,-2.49938595077448,-2.45210082174036,
-2.40578140197482,-2.38253098633032,-2.37763400335865,-2.37637338338913,
-2.37563060559363,-2.37497316820974,-2.37413683835302,-2.37281293792719,
-2.36624760419868,-2.33003236169214,-2.30944857313231,-2.26904627921545,
-2.22504435723991,-2.22033566737779,-2.21678402087101,-2.21518514185618,
-2.21399104248703,-2.21287601143916,-2.2113437794367,-2.20828819047212,
-2.18137788033073,-2.11010362850301,-2.05754398831667,-2.05462387519191,
-2.05358231327164,-2.05288816212063,-2.05221975457724,-2.05141810813354,
-2.04943824975472,-2.03190840475543,-2.03109405519523,-2.00923307740926,
-1.91416105030042,-1.89676801896583,-1.89380852661887,-1.8923042047372,
-1.89112365198092,-1.88981328307948,-1.88765759311611,-1.88000200014614,
-1.85426433717289,-1.8109004304892,-1.7365594184233,-1.73234282535337,-1.73109375147995,
-1.73042742447984,-1.72977882241033,-1.72897927818886,-1.72745869700733,
-1.71841014094023,-1.69926446724877,-1.65183970628718,-1.57656337189498,
-1.57199196957249,-1.57034770605514,-1.5692024871226,-1.56813962458352,
-1.56669096618924,-1.56390210499777,-1.54613431562565,-1.50440614888028,
-1.41424308808466,-1.40971241970672,-1.40844325838421,-1.40769116812338,
-1.40704118315682,-1.40622179330454,-1.40460650452707,-1.39309147515017,
-1.36634447841407,-1.29007771480206,-1.2758049359357,-1.27070870511949,
-1.25158021601765,-1.24849562692751,-1.24698632025105,-1.24580502849872,
-1.24452364449189,-1.24245962435419,-1.24001310677164,-1.23530602811917,
-1.19132536773386,-1.09816103091897,-1.08770160457215,-1.08598960818337,
-1.08515050121917,-1.08449260916141,-1.08375117640228,-1.08249716703844,
-1.07767716192421,-1.04179210820542,-0.932979853549016,-0.926861018594506,
-0.924799321776232,-0.923638811965763,-0.92248039566963,-0.921045977327254,
-0.91829137570206,-0.914816120234125,-0.907236322188173,-0.885497732320572,
-0.834913320862327,-0.827720600789962,-0.767417386168433,-0.766248960361632,
-0.763645653552049,-0.762721360619905,-0.762081541310863,-0.761487770125752,
-0.760666353912119,-0.759041138451033,-0.747217539699004,-0.720712657359132,
-0.631583153642152,-0.626015848650499,-0.606046136625364,-0.60292253799403,
-0.601405541820202,-0.600223397106319,-0.598945957379322,-0.596930387124626,
-0.590344869714719,-0.580002100953146,-0.57077636487165,-0.531147450016179,
-0.44580743247836,-0.441412174168298,-0.440142817797402,-0.439398016944631,
-0.438806554467441,-0.438005289159411,-0.436476830082254,-0.427252967703651,
-0.408395126312187,-0.36508996999871,-0.34365648788856,-0.311616565005529,
-0.283889620025191,-0.280467939168452,-0.278910157702366,-0.277718158730201,
-0.276618033213144,-0.275369989578078,-0.271954392446,-0.245419946775437,
-0.224207543775412,-0.133231880603835,-0.132268129062042,-0.119655658966594,
-0.118026183930549,-0.117191659800277,-0.11657580415066,-0.115902382723439,
-0.114962879382259,-0.112706609127926,-0.0783863747249849,-0.00095823755941713),
 .UNSPECIFIED.);
#837=B_SPLINE_CURVE_WITH_KNOTS('',3,(#48885,#48886,#48887,#48888,#48889,
#48890,#48891,#48892,#48893,#48894,#48895,#48896,#48897,#48898,#48899,#48900,
#48901,#48902,#48903,#48904,#48905,#48906,#48907,#48908,#48909,#48910,#48911,
#48912,#48913,#48914,#48915,#48916,#48917,#48918,#48919,#48920,#48921,#48922,
#48923,#48924,#48925,#48926,#48927,#48928,#48929,#48930,#48931,#48932,#48933,
#48934,#48935,#48936,#48937,#48938,#48939,#48940,#48941,#48942,#48943,#48944,
#48945,#48946,#48947,#48948,#48949,#48950,#48951,#48952,#48953,#48954,#48955,
#48956,#48957,#48958,#48959,#48960,#48961,#48962,#48963,#48964,#48965,#48966,
#48967,#48968,#48969,#48970,#48971,#48972,#48973,#48974,#48975,#48976,#48977,
#48978,#48979,#48980,#48981,#48982,#48983,#48984,#48985,#48986,#48987,#48988,
#48989,#48990,#48991,#48992,#48993,#48994,#48995,#48996,#48997,#48998,#48999,
#49000,#49001,#49002,#49003,#49004,#49005,#49006,#49007,#49008,#49009,#49010,
#49011,#49012,#49013,#49014,#49015,#49016,#49017,#49018,#49019,#49020,#49021,
#49022,#49023,#49024,#49025,#49026,#49027,#49028,#49029,#49030,#49031,#49032,
#49033,#49034,#49035,#49036,#49037,#49038,#49039,#49040,#49041,#49042,#49043,
#49044,#49045,#49046,#49047,#49048,#49049,#49050,#49051,#49052,#49053,#49054,
#49055,#49056,#49057,#49058,#49059,#49060,#49061,#49062,#49063,#49064,#49065,
#49066,#49067,#49068,#49069,#49070,#49071,#49072,#49073,#49074,#49075,#49076,
#49077,#49078,#49079,#49080,#49081,#49082,#49083,#49084,#49085,#49086,#49087,
#49088,#49089,#49090,#49091,#49092,#49093,#49094,#49095,#49096,#49097,#49098,
#49099,#49100,#49101,#49102,#49103,#49104,#49105,#49106,#49107,#49108,#49109,
#49110,#49111,#49112,#49113,#49114,#49115,#49116,#49117,#49118,#49119,#49120,
#49121,#49122,#49123,#49124,#49125,#49126,#49127,#49128,#49129,#49130,#49131,
#49132,#49133,#49134,#49135,#49136,#49137,#49138,#49139,#49140,#49141,#49142,
#49143,#49144,#49145,#49146,#49147,#49148,#49149,#49150,#49151,#49152,#49153,
#49154,#49155,#49156,#49157,#49158,#49159,#49160,#49161,#49162,#49163,#49164,
#49165,#49166,#49167,#49168,#49169,#49170,#49171,#49172,#49173,#49174,#49175,
#49176,#49177,#49178,#49179,#49180,#49181,#49182,#49183,#49184,#49185,#49186,
#49187,#49188,#49189,#49190,#49191,#49192,#49193,#49194,#49195,#49196,#49197,
#49198,#49199,#49200,#49201,#49202,#49203,#49204,#49205,#49206,#49207,#49208,
#49209,#49210,#49211,#49212,#49213,#49214,#49215,#49216,#49217,#49218,#49219,
#49220,#49221,#49222,#49223,#49224,#49225,#49226,#49227,#49228,#49229,#49230,
#49231,#49232,#49233,#49234,#49235,#49236,#49237,#49238,#49239,#49240,#49241,
#49242,#49243,#49244,#49245,#49246,#49247,#49248,#49249,#49250,#49251,#49252,
#49253,#49254,#49255,#49256,#49257,#49258,#49259,#49260,#49261,#49262,#49263,
#49264,#49265,#49266,#49267,#49268,#49269,#49270,#49271,#49272,#49273,#49274,
#49275,#49276,#49277,#49278,#49279,#49280,#49281,#49282,#49283,#49284,#49285,
#49286,#49287,#49288,#49289,#49290,#49291,#49292,#49293,#49294,#49295,#49296,
#49297,#49298,#49299,#49300,#49301,#49302,#49303,#49304,#49305,#49306,#49307,
#49308,#49309,#49310,#49311,#49312,#49313,#49314,#49315,#49316,#49317,#49318,
#49319,#49320,#49321,#49322,#49323,#49324,#49325,#49326,#49327,#49328,#49329,
#49330,#49331,#49332,#49333,#49334,#49335,#49336,#49337,#49338,#49339,#49340,
#49341,#49342,#49343,#49344,#49345,#49346,#49347,#49348,#49349,#49350,#49351,
#49352,#49353,#49354,#49355,#49356,#49357,#49358,#49359,#49360,#49361,#49362,
#49363,#49364,#49365,#49366,#49367,#49368,#49369,#49370,#49371,#49372,#49373,
#49374,#49375,#49376,#49377,#49378,#49379,#49380,#49381,#49382,#49383,#49384,
#49385,#49386,#49387,#49388,#49389,#49390,#49391,#49392,#49393,#49394,#49395,
#49396,#49397,#49398,#49399,#49400,#49401,#49402,#49403,#49404,#49405,#49406,
#49407,#49408,#49409,#49410,#49411,#49412,#49413,#49414,#49415,#49416,#49417,
#49418,#49419,#49420,#49421,#49422,#49423,#49424,#49425,#49426,#49427,#49428,
#49429,#49430,#49431,#49432),.UNSPECIFIED.,.F.,.F.,(4,2,2,2,2,2,2,2,2,2,
2,2,2,2,2,2,2,2,2,2,2,2,2,2,2,2,2,2,2,2,2,2,2,2,2,2,2,2,2,2,2,2,2,2,2,2,
2,2,2,2,2,2,2,2,2,2,2,2,2,2,2,2,2,2,2,2,2,2,2,2,2,2,2,2,2,2,2,2,2,2,2,2,
2,2,2,2,2,2,2,2,2,2,2,2,2,2,2,2,2,2,2,2,2,2,2,2,2,2,2,2,2,2,2,2,2,2,2,2,
2,2,2,2,2,2,2,2,2,2,2,2,2,2,2,2,2,2,2,2,2,2,2,2,2,2,2,2,2,2,2,2,2,2,2,2,
2,2,2,2,2,2,2,2,2,2,2,2,2,2,2,2,2,2,2,2,2,2,2,2,2,2,2,2,2,2,2,2,2,2,2,2,
2,2,2,2,2,2,2,2,2,2,2,2,2,2,2,2,2,2,2,2,2,2,2,2,2,2,2,2,2,2,2,2,2,2,2,2,
2,2,2,2,2,2,2,2,2,2,2,2,2,2,2,2,2,2,2,2,2,2,2,2,2,2,2,2,2,2,2,2,2,2,2,2,
2,2,2,2,2,2,2,2,2,2,2,4),(-4.0615853247519,-4.02242115167359,-4.01976680171588,
-4.01813846529024,-4.01693563272314,-4.0158299389595,-4.01462605130291,
-4.01317645156132,-4.0095616346049,-3.974972001932,-3.96821340270505,-3.89257618382849,
-3.86105884083779,-3.85656913179024,-3.85534576415173,-3.85461118817929,
-3.85395193827115,-3.85310099528578,-3.85132937746257,-3.83959863761468,
-3.83788523478661,-3.75570548965892,-3.73436892678005,-3.710146306358,-3.70193131382897,
-3.69643081722656,-3.69452920617676,-3.69342752729212,-3.69224586983523,
-3.69073455672694,-3.6876404737086,-3.66831681430305,-3.66067303746865,
-3.65468401750256,-3.60075211613687,-3.59467993113346,-3.58764087790891,
-3.56299376065091,-3.54412326640003,-3.53448774585898,-3.53294169785175,
-3.53213669128762,-3.5314815838859,-3.53081662888454,-3.52957474771371,
-3.52542154258814,-3.45155763404129,-3.41526421989712,-3.38857542624335,
-3.37972920512222,-3.37389724025494,-3.3719534373843,-3.37070161902936,
-3.36951133561992,-3.36796429092388,-3.36472183621126,-3.34093357471604,
-3.24942312001461,-3.21584913996433,-3.2111980544736,-3.20995940421589,
-3.20922137970232,-3.20856280298063,-3.20771782904293,-3.20597656207676,
-3.19491436744379,-3.10309116474825,-3.05853451189306,-3.05379100091248,
-3.05133054946257,-3.0492547074056,-3.04797137999622,-3.04679029313389,
-3.04528384000711,-3.04231555517221,-3.02476481368793,-3.02112813493968,
-2.92444249614953,-2.89279808066718,-2.88829787869645,-2.88707340695115,
-2.88633852702102,-2.88567924293765,-2.88482858126335,-2.88305870718342,
-2.8713708317866,-2.77888643774241,-2.73550962963286,-2.73083944201038,
-2.72840676438722,-2.72634819919006,-2.7250698082245,-2.72388755388883,
-2.72237193521343,-2.71925654731477,-2.69947892073897,-2.69397925913445,
-2.68668761940822,-2.61796497725257,-2.56719032595463,-2.56490486088029,
-2.56396041781971,-2.56328605110428,-2.56267120089874,-2.56184069926522,
-2.56022688773267,-2.557968215489,-2.50018554060422,-2.45049410969333,-2.41218437505629,
-2.4056278258838,-2.40359011374764,-2.40230578561648,-2.40111767053597,
-2.39958542040838,-2.39630024250671,-2.37250082557052,-2.35807007133607,
-2.32052232573239,-2.28966457476984,-2.25480222673668,-2.24353590746572,
-2.2419286884762,-2.24111087623875,-2.2404548998698,-2.23969923075482,-2.23841510616025,
-2.23374384282472,-2.13834438787572,-2.09057279507353,-2.08308196913468,
-2.08094263741557,-2.07963571112717,-2.0784540266717,-2.07694241371128,
-2.07384678561521,-2.0544898637708,-2.04948056942048,-2.030837653146,-1.98110066310485,
-1.95692879108548,-1.94458784122884,-1.9388605493758,-1.9213806224272,-1.9194020178155,
-1.91860051835575,-1.9179320895786,-1.91723775699851,-1.91619563234267,
-1.91327207302077,-1.86860989974576,-1.77656720039791,-1.76165632680691,
-1.7590871060386,-1.75754266172103,-1.75635289353232,-1.75507448174804,
-1.75306241357917,-1.74672137471996,-1.71042246519912,-1.65450394745586,
-1.61177042204784,-1.60981710574321,-1.59834592264835,-1.59658612180481,
-1.59573759390254,-1.59507873186691,-1.59434301774896,-1.59311421429564,
-1.58856609781781,-1.5563205587097,-1.46927492364261,-1.43996426443403,
-1.43684084698413,-1.43529153695447,-1.43417201988404,-1.43298051647101,
-1.43139778167085,-1.42793309213504,-1.35419563179135,-1.28692153919386,
-1.27560958728518,-1.27385703865407,-1.27300994774475,-1.27236701104544,
-1.27165034004064,-1.27089816105163,-1.26978653446161,-1.26780243528164,
-1.25220445802589,-1.23349399149988,-1.14616005544479,-1.1172270624114,
-1.11381296577539,-1.11237431608101,-1.11117344103699,-1.10994028382185,
-1.10813655135382,-1.10335334149979,-1.08047464184013,-1.05873879601757,
-0.955864770861231,-0.951898753551426,-0.950679066036687,-0.95001857327729,
-0.949375930009211,-0.948616738863242,-0.947774642249744,-0.946448394884249,
-0.943911683735059,-0.919926691522573,-0.919114712932559,-0.87209914397502,
-0.82512008103244,-0.819597922451927,-0.814001121436301,-0.793985308394998,
-0.790859078482923,-0.789341346565783,-0.788158873621436,-0.786855136591932,
-0.78473018760486,-0.777378867600789,-0.731103012288167,-0.687701559380429,
-0.643668720257757,-0.64185792032517,-0.630231835406725,-0.628464896421524,
-0.627614885106117,-0.626979223326688,-0.62626627194827,-0.625112765307508,
-0.623742147387329,-0.621087741911813,-0.614556601901783,-0.592231259110943,
-0.504760637523064,-0.495016552353321,-0.471522317778034,-0.468290225047729,
-0.466745308548937,-0.465555395112721,-0.464277042262853,-0.462265518216169,
-0.455929825738729,-0.419682223977332,-0.372108397671492,-0.348971229836516,
-0.327531577286781,-0.307976259323787,-0.306143325672652,-0.305257848179888,
-0.304628664821996,-0.303977708079013,-0.30311636710413,-0.302161872168732,
-0.300565515336198,-0.297294254060778,-0.288607719310095,-0.26662265207392,
-0.187935169392622,-0.181960621682548,-0.173524698132422,-0.168130440016484,
-0.148645466892783,-0.145544070868586,-0.144031410881682,-0.14284971365204,
-0.141543595625807,-0.139407450883285,-0.131946124360121,-0.084482302582598,
-0.000958182641776821),.UNSPECIFIED.);
#838=B_SPLINE_CURVE_WITH_KNOTS('',3,(#49434,#49435,#49436,#49437,#49438,
#49439,#49440,#49441,#49442,#49443,#49444,#49445,#49446,#49447,#49448,#49449,
#49450,#49451,#49452,#49453,#49454,#49455,#49456,#49457,#49458,#49459,#49460,
#49461,#49462,#49463,#49464,#49465,#49466,#49467,#49468,#49469,#49470,#49471,
#49472,#49473,#49474,#49475,#49476,#49477,#49478,#49479,#49480,#49481,#49482,
#49483,#49484,#49485,#49486,#49487,#49488,#49489,#49490,#49491,#49492,#49493,
#49494,#49495,#49496,#49497,#49498,#49499,#49500,#49501,#49502,#49503,#49504,
#49505,#49506,#49507,#49508,#49509,#49510,#49511,#49512,#49513,#49514,#49515,
#49516,#49517,#49518,#49519,#49520,#49521,#49522,#49523,#49524,#49525,#49526,
#49527,#49528,#49529,#49530,#49531,#49532,#49533,#49534,#49535,#49536,#49537,
#49538,#49539,#49540,#49541,#49542,#49543,#49544,#49545,#49546,#49547,#49548,
#49549,#49550,#49551,#49552,#49553,#49554,#49555,#49556,#49557,#49558,#49559,
#49560,#49561,#49562,#49563,#49564,#49565,#49566,#49567,#49568,#49569,#49570,
#49571,#49572,#49573,#49574,#49575,#49576,#49577,#49578,#49579,#49580,#49581,
#49582,#49583,#49584,#49585,#49586,#49587,#49588,#49589,#49590,#49591,#49592,
#49593,#49594,#49595,#49596,#49597,#49598,#49599,#49600,#49601,#49602,#49603,
#49604,#49605,#49606,#49607,#49608,#49609,#49610,#49611,#49612,#49613,#49614,
#49615,#49616,#49617,#49618,#49619,#49620,#49621,#49622,#49623,#49624,#49625,
#49626,#49627,#49628,#49629,#49630,#49631,#49632,#49633,#49634,#49635,#49636,
#49637,#49638,#49639,#49640,#49641,#49642,#49643,#49644,#49645,#49646,#49647,
#49648,#49649,#49650,#49651,#49652,#49653,#49654,#49655,#49656,#49657,#49658,
#49659,#49660,#49661,#49662,#49663,#49664,#49665,#49666,#49667,#49668,#49669,
#49670,#49671,#49672,#49673,#49674,#49675,#49676,#49677,#49678,#49679,#49680,
#49681,#49682,#49683,#49684,#49685,#49686,#49687,#49688,#49689,#49690,#49691,
#49692,#49693,#49694,#49695,#49696,#49697,#49698,#49699,#49700,#49701,#49702,
#49703,#49704,#49705,#49706,#49707,#49708,#49709,#49710,#49711,#49712,#49713,
#49714,#49715,#49716,#49717,#49718,#49719,#49720,#49721,#49722,#49723,#49724,
#49725,#49726,#49727,#49728,#49729,#49730,#49731,#49732,#49733,#49734,#49735,
#49736,#49737,#49738,#49739,#49740,#49741,#49742,#49743,#49744,#49745,#49746,
#49747,#49748,#49749,#49750,#49751,#49752,#49753,#49754,#49755,#49756,#49757,
#49758,#49759,#49760,#49761,#49762,#49763,#49764,#49765,#49766,#49767,#49768,
#49769,#49770,#49771,#49772,#49773,#49774,#49775,#49776,#49777,#49778,#49779,
#49780,#49781,#49782,#49783,#49784,#49785,#49786,#49787,#49788,#49789,#49790,
#49791,#49792,#49793,#49794,#49795,#49796,#49797,#49798,#49799,#49800,#49801,
#49802,#49803,#49804,#49805,#49806,#49807,#49808,#49809,#49810,#49811,#49812,
#49813,#49814,#49815,#49816,#49817,#49818,#49819,#49820,#49821,#49822,#49823,
#49824,#49825,#49826,#49827,#49828,#49829,#49830,#49831,#49832,#49833,#49834,
#49835,#49836,#49837,#49838,#49839,#49840,#49841,#49842,#49843,#49844,#49845,
#49846,#49847,#49848,#49849,#49850,#49851,#49852,#49853,#49854,#49855,#49856,
#49857,#49858,#49859,#49860,#49861,#49862,#49863,#49864,#49865,#49866,#49867,
#49868,#49869,#49870,#49871,#49872,#49873,#49874,#49875,#49876,#49877,#49878,
#49879,#49880,#49881,#49882,#49883,#49884,#49885,#49886,#49887,#49888,#49889,
#49890,#49891,#49892,#49893,#49894,#49895,#49896,#49897,#49898,#49899,#49900,
#49901,#49902,#49903,#49904,#49905,#49906,#49907,#49908,#49909,#49910,#49911,
#49912,#49913,#49914,#49915,#49916,#49917,#49918,#49919,#49920,#49921,#49922,
#49923,#49924,#49925,#49926,#49927,#49928,#49929,#49930,#49931,#49932,#49933,
#49934,#49935,#49936,#49937,#49938,#49939,#49940,#49941,#49942,#49943,#49944,
#49945,#49946,#49947,#49948,#49949,#49950,#49951,#49952,#49953,#49954,#49955,
#49956,#49957,#49958,#49959,#49960,#49961,#49962,#49963,#49964,#49965,#49966,
#49967,#49968,#49969,#49970,#49971,#49972,#49973,#49974,#49975,#49976,#49977,
#49978,#49979,#49980,#49981,#49982,#49983,#49984,#49985,#49986,#49987,#49988,
#49989,#49990,#49991,#49992,#49993,#49994,#49995,#49996,#49997,#49998,#49999),
 .UNSPECIFIED.,.F.,.F.,(4,2,2,2,2,2,2,2,2,2,2,2,2,2,2,2,2,2,2,2,2,2,2,2,
2,2,2,2,2,2,2,2,2,2,2,2,2,2,2,2,2,2,2,2,2,2,2,2,2,2,2,2,2,2,2,2,2,2,2,2,
2,2,2,2,2,2,2,2,2,2,2,2,2,2,2,2,2,2,2,2,2,2,2,2,2,2,2,2,2,2,2,2,2,2,2,2,
2,2,2,2,2,2,2,2,2,2,2,2,2,2,2,2,2,2,2,2,2,2,2,2,2,2,2,2,2,2,2,2,2,2,2,2,
2,2,2,2,2,2,2,2,2,2,2,2,2,2,2,2,2,2,2,2,2,2,2,2,2,2,2,2,2,2,2,2,2,2,2,2,
2,2,2,2,2,2,2,2,2,2,2,2,2,2,2,2,2,2,2,2,2,2,2,2,2,2,2,2,2,2,2,2,2,2,2,2,
2,2,2,2,2,2,2,2,2,2,2,2,2,2,2,2,2,2,2,2,2,2,2,2,2,2,2,2,2,2,2,2,2,2,2,2,
2,2,2,2,2,2,2,2,2,2,2,2,2,2,2,2,2,2,2,2,2,2,2,2,2,2,2,2,2,2,2,2,2,2,2,2,
2,2,2,2,2,2,4),(-4.06131821400407,-4.04564568548944,-4.04423736326734,-4.04336096921321,
-4.04270254315682,-4.04208025663957,-4.04146439300674,-4.04062941647786,
-4.03899775737188,-4.02631729079821,-4.02541205256894,-4.02124691612192,
-3.92430896333871,-3.8903369049557,-3.88424942352277,-3.8822683184449,-3.88099690321561,
-3.8798046826896,-3.87824419742475,-3.87480676355946,-3.84656015452383,
-3.75871054150758,-3.7329862113546,-3.72581388357961,-3.72297083700817,
-3.7215301087255,-3.72032995840551,-3.71960581947867,-3.71898397851182,
-3.71816005225614,-3.71687647612268,-3.71086537974348,-3.65137253589725,
-3.64546905306771,-3.6386940874131,-3.63076020183689,-3.60244471287889,
-3.56781024225568,-3.56164952089861,-3.55965925344438,-3.5583856993459,
-3.55719411775863,-3.55563826579553,-3.55222642121411,-3.52479766965239,
-3.43264887977656,-3.409457218603,-3.40284612211045,-3.40016802113991,-3.39878856214657,
-3.39762951250618,-3.39691509447215,-3.39628146277456,-3.39543527924312,
-3.39368758827325,-3.38248417711807,-3.37885294651681,-3.29339445746787,
-3.24656247878386,-3.23915862061927,-3.23702837819871,-3.23572356047329,
-3.23454152797887,-3.23302633834211,-3.22991234366088,-3.21015681989116,
-3.20466319199457,-3.19883819372107,-3.1259723095705,-3.08162213331746,
-3.07812412241491,-3.07644738687807,-3.07545986212116,-3.07457570657534,
-3.0739207598933,-3.07329867432616,-3.07243984129997,-3.07025506025273,
-3.04112751227071,-2.97132731880923,-2.92396025630536,-2.91650678132836,
-2.91437138282476,-2.91306539379091,-2.91188359936975,-2.91037051829683,
-2.90726721496302,-2.88774317427366,-2.88603520771294,-2.8106881892503,
-2.755636261938,-2.75386574303573,-2.752839964163,-2.75192794674054,-2.75126847074818,
-2.75065298898022,-2.74981978188696,-2.74819527025819,-2.73571486474279,
-2.73265287581106,-2.73225838126724,-2.63405043846526,-2.59956072069251,
-2.59341582964281,-2.59142746680557,-2.59015431253714,-2.58896252629415,
-2.58740557662876,-2.58398796673873,-2.55638147282693,-2.51475910784884,
-2.50711923059234,-2.45956758530017,-2.44044280636558,-2.43131547523018,
-2.42979132415948,-2.42899099848852,-2.42839966133318,-2.42774957990476,
-2.42658117168864,-2.42302008340547,-2.3590863807765,-2.33352106812079,
-2.30442029773425,-2.27879006787232,-2.2737814837377,-2.27004915666551,
-2.26841740945389,-2.26721764951944,-2.26611070583004,-2.26461010654667,
-2.26167881622215,-2.23858845479701,-2.22741245502535,-2.14053720211954,
-2.11228847391277,-2.10950092384306,-2.10743732759163,-2.10653150746877,
-2.10586417593835,-2.10524037910688,-2.10437509575746,-2.10215240373267,
-2.07035172374347,-2.03176400962034,-1.95295629825287,-1.94794654281236,
-1.94604794429724,-1.94491977411415,-1.94373231372073,-1.94217711415402,
-1.93885843641365,-1.8941040247194,-1.8433409018295,-1.81654973446563,-1.78709866599404,
-1.78490902523997,-1.78404937179746,-1.78342708060911,-1.78275881954532,
-1.78184742917021,-1.77975254094595,-1.77691192178312,-1.74771709598557,
-1.66061729017535,-1.65338674685689,-1.64760709120416,-1.62748664461858,
-1.62435604834044,-1.62283761033761,-1.62165522561563,-1.62035223322294,
-1.61822995308544,-1.61090185925383,-1.56486697364556,-1.46721507321892,
-1.4627707987802,-1.46149591163686,-1.46074981205669,-1.46015842948497,
-1.45935869750305,-1.45783780452602,-1.44878863695427,-1.42963852230472,
-1.38220501211115,-1.30678559778606,-1.30229847765498,-1.30066677079691,
-1.2995248386961,-1.29836612291056,-1.29689206018115,-1.29528460874432,
-1.29268018683795,-1.28755317628312,-1.23640758794081,-1.15280526635326,
-1.14086045406957,-1.1390793541436,-1.13823563176969,-1.1375754580195,-1.13684453127135,
-1.13563763042193,-1.13131697739016,-1.10184197864858,-1.0097799992895,
-1.00390478867719,-1.00213764007245,-0.99693115151631,-0.981478722311891,
-0.978879592153521,-0.977326186010432,-0.976159846183014,-0.975003880785112,
-0.973745564895992,-0.971976115754497,-0.968981989974722,-0.96278523948794,
-0.946245021233967,-0.926636323654967,-0.876268719643402,-0.820228425271349,
-0.816978932638856,-0.815852988955089,-0.815211364379053,-0.814617971319561,
-0.813800191930205,-0.812193023496927,-0.800926341443691,-0.765575119764493,
-0.754839614433181,-0.69177111415986,-0.689399716267035,-0.659769061711834,
-0.656635825249673,-0.655083857456858,-0.653963453773098,-0.652795820697045,
-0.651260370465129,-0.64956792169078,-0.646759854999155,-0.641079628516428,
-0.626377918485184,-0.591409248339216,-0.513683636509949,-0.4957582549922,
-0.493964678127234,-0.493088785420703,-0.492462101306534,-0.491796333240201,
-0.490900399770547,-0.488891803162583,-0.48619725163834,-0.459575420234084,
-0.432925952443986,-0.424314982348876,-0.394898026981938,-0.337786390603463,
-0.333906726971192,-0.332372884651655,-0.331257170519479,-0.330086821488342,
-0.328534911378537,-0.326819609350674,-0.323956621613555,-0.31812523584596,
-0.227248109447834,-0.182585044773427,-0.172534228610469,-0.170863609535287,
-0.17002120968391,-0.169362840582242,-0.168623124253374,-0.167377219729346,
-0.162648656051969,-0.128047325479992,-0.0182103218958969,-0.0117709783369783,
-0.00966671952489206,-0.00849750027836917,-0.00733258565330951,-0.00620266545220797,
-0.00478645794291243,-0.000957137645843165),.UNSPECIFIED.);
#839=B_SPLINE_CURVE_WITH_KNOTS('',3,(#50001,#50002,#50003,#50004,#50005,
#50006,#50007,#50008,#50009,#50010,#50011,#50012,#50013,#50014,#50015,#50016,
#50017,#50018,#50019,#50020,#50021,#50022,#50023,#50024,#50025,#50026,#50027,
#50028,#50029,#50030,#50031,#50032,#50033,#50034,#50035,#50036,#50037,#50038,
#50039,#50040,#50041,#50042,#50043,#50044,#50045,#50046,#50047,#50048,#50049,
#50050,#50051,#50052,#50053,#50054,#50055,#50056,#50057,#50058,#50059,#50060,
#50061,#50062,#50063,#50064,#50065,#50066,#50067,#50068,#50069,#50070,#50071,
#50072,#50073,#50074,#50075,#50076,#50077,#50078,#50079,#50080,#50081,#50082,
#50083,#50084,#50085,#50086,#50087,#50088,#50089,#50090,#50091,#50092,#50093,
#50094,#50095,#50096,#50097,#50098,#50099,#50100,#50101,#50102,#50103,#50104,
#50105,#50106,#50107,#50108,#50109,#50110,#50111,#50112,#50113,#50114,#50115,
#50116,#50117,#50118,#50119,#50120,#50121,#50122,#50123,#50124,#50125,#50126,
#50127,#50128,#50129,#50130,#50131,#50132,#50133,#50134,#50135,#50136,#50137,
#50138,#50139,#50140,#50141,#50142,#50143,#50144,#50145,#50146,#50147,#50148,
#50149,#50150,#50151,#50152,#50153,#50154,#50155,#50156,#50157,#50158,#50159,
#50160,#50161,#50162,#50163,#50164,#50165,#50166,#50167,#50168,#50169,#50170,
#50171,#50172,#50173,#50174,#50175,#50176,#50177,#50178,#50179,#50180,#50181,
#50182,#50183,#50184,#50185,#50186,#50187,#50188,#50189,#50190,#50191,#50192,
#50193,#50194,#50195,#50196,#50197,#50198,#50199,#50200,#50201,#50202,#50203,
#50204,#50205,#50206,#50207,#50208,#50209,#50210,#50211,#50212,#50213,#50214,
#50215,#50216,#50217,#50218,#50219,#50220,#50221,#50222,#50223,#50224,#50225,
#50226,#50227,#50228,#50229,#50230,#50231,#50232,#50233,#50234,#50235,#50236,
#50237,#50238,#50239,#50240,#50241,#50242,#50243,#50244,#50245,#50246,#50247,
#50248,#50249,#50250,#50251,#50252,#50253,#50254,#50255,#50256,#50257,#50258,
#50259,#50260,#50261,#50262,#50263,#50264,#50265,#50266,#50267,#50268,#50269,
#50270,#50271,#50272,#50273,#50274,#50275,#50276,#50277,#50278,#50279,#50280,
#50281,#50282,#50283,#50284,#50285,#50286,#50287,#50288,#50289,#50290,#50291,
#50292,#50293,#50294,#50295,#50296,#50297,#50298,#50299,#50300,#50301,#50302,
#50303,#50304,#50305,#50306,#50307,#50308,#50309,#50310,#50311,#50312,#50313,
#50314,#50315,#50316,#50317,#50318,#50319,#50320,#50321,#50322,#50323,#50324,
#50325,#50326,#50327,#50328,#50329,#50330,#50331,#50332,#50333,#50334,#50335,
#50336,#50337,#50338,#50339,#50340,#50341,#50342,#50343,#50344,#50345,#50346,
#50347,#50348,#50349,#50350,#50351,#50352,#50353,#50354,#50355,#50356,#50357,
#50358,#50359,#50360,#50361,#50362,#50363,#50364,#50365,#50366,#50367,#50368,
#50369,#50370,#50371,#50372,#50373,#50374,#50375,#50376,#50377,#50378,#50379,
#50380,#50381,#50382,#50383,#50384,#50385,#50386,#50387,#50388,#50389,#50390,
#50391,#50392,#50393,#50394,#50395,#50396,#50397,#50398,#50399,#50400,#50401,
#50402,#50403,#50404,#50405,#50406,#50407,#50408,#50409,#50410,#50411,#50412,
#50413,#50414,#50415,#50416,#50417,#50418,#50419,#50420,#50421,#50422,#50423,
#50424,#50425,#50426,#50427,#50428,#50429,#50430,#50431,#50432,#50433,#50434,
#50435,#50436,#50437,#50438,#50439,#50440,#50441,#50442,#50443,#50444,#50445,
#50446,#50447,#50448,#50449,#50450,#50451,#50452,#50453,#50454,#50455,#50456,
#50457,#50458,#50459,#50460,#50461,#50462,#50463,#50464,#50465,#50466,#50467,
#50468,#50469,#50470,#50471,#50472,#50473,#50474,#50475,#50476,#50477,#50478,
#50479,#50480,#50481,#50482,#50483,#50484,#50485,#50486,#50487,#50488,#50489,
#50490,#50491,#50492,#50493,#50494,#50495,#50496,#50497,#50498,#50499,#50500,
#50501,#50502,#50503,#50504,#50505,#50506,#50507,#50508,#50509,#50510,#50511,
#50512,#50513,#50514,#50515,#50516,#50517,#50518,#50519,#50520,#50521,#50522,
#50523,#50524,#50525,#50526,#50527,#50528,#50529,#50530,#50531,#50532,#50533,
#50534,#50535,#50536,#50537,#50538,#50539,#50540,#50541,#50542),
 .UNSPECIFIED.,.F.,.F.,(4,2,2,2,2,2,2,2,2,2,2,2,2,2,2,2,2,2,2,2,2,2,2,2,
2,2,2,2,2,2,2,2,2,2,2,2,2,2,2,2,2,2,2,2,2,2,2,2,2,2,2,2,2,2,2,2,2,2,2,2,
2,2,2,2,2,2,2,2,2,2,2,2,2,2,2,2,2,2,2,2,2,2,2,2,2,2,2,2,2,2,2,2,2,2,2,2,
2,2,2,2,2,2,2,2,2,2,2,2,2,2,2,2,2,2,2,2,2,2,2,2,2,2,2,2,2,2,2,2,2,2,2,2,
2,2,2,2,2,2,2,2,2,2,2,2,2,2,2,2,2,2,2,2,2,2,2,2,2,2,2,2,2,2,2,2,2,2,2,2,
2,2,2,2,2,2,2,2,2,2,2,2,2,2,2,2,2,2,2,2,2,2,2,2,2,2,2,2,2,2,2,2,2,2,2,2,
2,2,2,2,2,2,2,2,2,2,2,2,2,2,2,2,2,2,2,2,2,2,2,2,2,2,2,2,2,2,2,2,2,2,2,2,
2,2,2,2,2,2,2,2,2,2,2,2,2,2,2,2,2,2,2,2,2,2,2,2,2,2,2,2,2,2,4),(-4.06091416108814,
-4.0556667509442,-3.9436925009123,-3.91010830592124,-3.90797102344079,-3.90705212921347,
-3.90638254636448,-3.90576212589432,-3.90490963505416,-3.9032094234937,
-3.8885334434254,-3.88617042623338,-3.88390122518972,-3.8827905315805,-3.87843199784321,
-3.81552956527625,-3.75223282399225,-3.74938487599442,-3.74767592701344,
-3.74612844383602,-3.744958977978,-3.74384225751226,-3.74230391594249,-3.73839632725442,
-3.67353063739135,-3.66582520044604,-3.61454556991071,-3.5954565230365,
-3.58649414972096,-3.58497729887887,-3.58417848360081,-3.58358725564961,
-3.58284065139721,-3.581563240286,-3.57709509492826,-3.4799776413505,-3.42977925247706,
-3.42679373682979,-3.42502793931893,-3.42343955040443,-3.4222630654745,
-3.42115722499087,-3.41966082261222,-3.41599666233606,-3.3756269175606,
-3.31550394113404,-3.30229013156382,-3.26799199500219,-3.26488763570596,
-3.26263963984912,-3.2617016913217,-3.26102869654279,-3.260412732604,-3.25957734951944,
-3.25794409567889,-3.24521959032898,-3.24176591405113,-3.23798518151985,
-3.23593808786589,-3.23334438802609,-3.16536605761403,-3.10625205613832,
-3.1036763256634,-3.10208101039202,-3.10061575169611,-3.09945922894538,
-3.098314237039,-3.09667084970325,-3.09210683550982,-3.0152065257964,-2.96883198009591,
-2.94557025935954,-2.94066893252356,-2.93940787217447,-2.93866496412505,
-2.93800749445283,-2.93717123391376,-2.93547288269604,-2.92528228694502,
-2.89550521360718,-2.83378145309395,-2.78390625696618,-2.78120855655403,
-2.77956219286603,-2.77805996635305,-2.77689765044283,-2.77576668374344,
-2.77417463497587,-2.76993988947724,-2.70436133204095,-2.67280355717629,
-2.61968405261242,-2.61739681355262,-2.61645223209729,-2.61577797984619,
-2.61516338742918,-2.61433345179782,-2.61272137710549,-2.60055380308683,
-2.59922739949456,-2.59700610554675,-2.59461440062683,-2.58721427415502,
-2.49649018312904,-2.46386889162928,-2.45793164818458,-2.4559692501439,
-2.45470193620988,-2.45350790348953,-2.45193683120957,-2.44927674159865,
-2.43264900388173,-2.430436058951,-2.42530531166532,-2.35811727265227,-2.33168453464077,
-2.29985675129688,-2.29534262724214,-2.29411715051974,-2.29338223518648,
-2.29272329619763,-2.29187359325637,-2.29010753782797,-2.27849393606782,
-2.20343714200941,-2.14135564521112,-2.13533536153555,-2.13336258889569,
-2.13209301207089,-2.13090001554844,-2.12933490038084,-2.12669507330763,
-2.11045885270608,-2.10484327172566,-2.03072314084274,-1.9757882926889,
-1.97250065147887,-1.97136924064359,-1.97072663313535,-1.97013370922062,
-1.96931865681988,-1.96772402255746,-1.95681039801111,-1.92900910995094,
-1.87121573337088,-1.81598635147893,-1.81212211723945,-1.81059123154371,
-1.80947656257617,-1.80828226932987,-1.80668212572828,-1.80312353706856,
-1.75370694917921,-1.66228023394796,-1.65091083266486,-1.64915558540535,
-1.64830793108314,-1.64764914370586,-1.64691287346963,-1.64568169293121,
-1.64110888290018,-1.60855113487346,-1.5207548039168,-1.49247756617037,
-1.4890388110489,-1.48747795839738,-1.48628555279233,-1.48501403307291,
-1.4830329564316,-1.47694703141396,-1.38352956024237,-1.32989974993652,
-1.32692713878969,-1.32584180784821,-1.32520831786053,-1.32455927944164,
-1.32371185416105,-1.32277559304969,-1.32122341409803,-1.31807522979958,
-1.2828579225852,-1.18854229333696,-1.16911742243247,-1.16601890123848,
-1.16450683966619,-1.16332524377902,-1.16201886400042,-1.15988144407788,
-1.1524073366178,-1.10480340074239,-1.01774553687216,-1.00538332313789,
-1.0037631972345,-1.00293112475591,-1.00231593383974,-1.00165603226417,
-1.00074209091452,-0.99971405163293,-0.997937976138313,-0.994154913084048,
-0.910333229606811,-0.847648011780672,-0.843743669122313,-0.84220585481626,
-0.841089271534206,-0.839895864505766,-0.83830197385835,-0.834777991860088,
-0.784375553338656,-0.697424836094035,-0.682716460602723,-0.681015084363849,
-0.680162256653613,-0.679541707109479,-0.678916356535199,-0.678043725881779,
-0.676142772124824,-0.673604316395439,-0.667458298973885,-0.649066011455502,
-0.613828560200457,-0.54375115014343,-0.523646891457507,-0.520516633834204,
-0.518998102423274,-0.517815528623805,-0.51651220989175,-0.514389133104203,
-0.507055741874997,-0.46097035809489,-0.451408864897502,-0.443627658960177,
-0.437077711691942,-0.384066163695826,-0.379460679110359,-0.3784661848796,
-0.377226172996081,-0.374543689670793,-0.372594755724589,-0.35995792329208,
-0.358327629382752,-0.357492921968437,-0.356877046274825,-0.35625471220879,
-0.355367567839754,-0.353395220552537,-0.350734636646391,-0.344182815422075,
-0.321609991224706,-0.234226633730324,-0.225826474101105,-0.220421206119031,
-0.200914784647962,-0.197812232088737,-0.196299278479867,-0.19511747496863,
-0.193811365053867,-0.19167551799272,-0.184218022278526,-0.136798209850487,
-0.0687485708789001,-0.0641404148857407,-0.0377946982054035,-0.0356562163948424,
-0.034805315206907,-0.034185289084645,-0.0335602932984056,-0.0329057838157608,
-0.0320403943492102,-0.0306585186817549,-0.000956380862327205),
 .UNSPECIFIED.);
#840=B_SPLINE_CURVE_WITH_KNOTS('',3,(#50544,#50545,#50546,#50547,#50548,
#50549,#50550,#50551,#50552,#50553,#50554,#50555,#50556,#50557,#50558,#50559,
#50560,#50561,#50562,#50563,#50564,#50565,#50566,#50567,#50568,#50569,#50570,
#50571,#50572,#50573,#50574,#50575,#50576,#50577,#50578,#50579,#50580,#50581,
#50582,#50583,#50584,#50585,#50586,#50587,#50588,#50589,#50590,#50591,#50592,
#50593,#50594,#50595,#50596,#50597,#50598,#50599,#50600,#50601,#50602,#50603,
#50604,#50605,#50606,#50607,#50608,#50609,#50610,#50611,#50612,#50613,#50614,
#50615,#50616,#50617,#50618,#50619,#50620,#50621,#50622,#50623,#50624,#50625,
#50626,#50627,#50628,#50629,#50630,#50631,#50632,#50633,#50634,#50635,#50636,
#50637,#50638,#50639,#50640,#50641,#50642,#50643,#50644,#50645,#50646,#50647,
#50648,#50649,#50650,#50651,#50652,#50653,#50654,#50655,#50656,#50657,#50658,
#50659,#50660,#50661,#50662,#50663,#50664,#50665,#50666,#50667,#50668,#50669,
#50670,#50671,#50672,#50673,#50674,#50675,#50676,#50677,#50678,#50679,#50680,
#50681,#50682,#50683,#50684,#50685,#50686,#50687,#50688,#50689,#50690,#50691,
#50692,#50693,#50694,#50695,#50696,#50697,#50698,#50699,#50700,#50701,#50702,
#50703,#50704,#50705,#50706,#50707,#50708,#50709,#50710,#50711,#50712,#50713,
#50714,#50715,#50716,#50717,#50718,#50719,#50720,#50721,#50722,#50723,#50724,
#50725,#50726,#50727,#50728,#50729,#50730,#50731,#50732,#50733,#50734,#50735,
#50736,#50737,#50738,#50739,#50740,#50741,#50742,#50743,#50744,#50745,#50746,
#50747,#50748,#50749,#50750,#50751,#50752,#50753,#50754,#50755,#50756,#50757,
#50758,#50759,#50760,#50761,#50762,#50763,#50764,#50765,#50766,#50767,#50768,
#50769,#50770,#50771,#50772,#50773,#50774,#50775,#50776,#50777,#50778,#50779,
#50780,#50781,#50782,#50783,#50784,#50785,#50786,#50787,#50788,#50789,#50790,
#50791,#50792,#50793,#50794,#50795,#50796,#50797,#50798,#50799,#50800,#50801,
#50802,#50803,#50804,#50805,#50806,#50807,#50808,#50809,#50810,#50811,#50812,
#50813,#50814,#50815,#50816,#50817,#50818,#50819,#50820,#50821,#50822,#50823,
#50824,#50825,#50826,#50827,#50828,#50829,#50830,#50831,#50832,#50833,#50834,
#50835,#50836,#50837,#50838,#50839,#50840,#50841,#50842,#50843,#50844,#50845,
#50846,#50847,#50848,#50849,#50850,#50851,#50852,#50853,#50854,#50855,#50856,
#50857,#50858,#50859,#50860,#50861,#50862,#50863,#50864,#50865,#50866,#50867,
#50868,#50869,#50870,#50871,#50872,#50873,#50874,#50875,#50876,#50877,#50878,
#50879,#50880,#50881,#50882,#50883,#50884,#50885,#50886,#50887,#50888,#50889,
#50890,#50891,#50892,#50893,#50894,#50895,#50896,#50897,#50898,#50899,#50900,
#50901,#50902,#50903,#50904,#50905,#50906,#50907,#50908,#50909,#50910,#50911,
#50912,#50913,#50914,#50915,#50916,#50917,#50918,#50919,#50920,#50921,#50922,
#50923,#50924,#50925,#50926,#50927,#50928,#50929,#50930,#50931,#50932,#50933,
#50934,#50935,#50936,#50937,#50938,#50939,#50940,#50941,#50942,#50943,#50944,
#50945,#50946,#50947,#50948,#50949,#50950,#50951,#50952,#50953,#50954,#50955,
#50956,#50957,#50958,#50959,#50960,#50961,#50962,#50963,#50964,#50965,#50966,
#50967,#50968,#50969,#50970,#50971,#50972,#50973,#50974,#50975,#50976,#50977,
#50978,#50979,#50980,#50981,#50982,#50983,#50984,#50985,#50986,#50987,#50988,
#50989,#50990,#50991,#50992,#50993,#50994,#50995,#50996,#50997,#50998,#50999,
#51000,#51001,#51002,#51003,#51004,#51005,#51006,#51007,#51008,#51009,#51010,
#51011,#51012,#51013,#51014,#51015,#51016,#51017,#51018,#51019,#51020,#51021,
#51022,#51023,#51024,#51025,#51026,#51027,#51028,#51029,#51030,#51031,#51032,
#51033,#51034,#51035,#51036,#51037,#51038,#51039,#51040,#51041,#51042,#51043,
#51044,#51045,#51046,#51047,#51048,#51049,#51050,#51051,#51052,#51053,#51054,
#51055,#51056,#51057,#51058,#51059,#51060,#51061,#51062,#51063,#51064,#51065,
#51066,#51067,#51068,#51069,#51070,#51071,#51072,#51073,#51074,#51075,#51076,
#51077,#51078,#51079),.UNSPECIFIED.,.F.,.F.,(4,2,2,2,2,2,2,2,2,2,2,2,2,
2,2,2,2,2,2,2,2,2,2,2,2,2,2,2,2,2,2,2,2,2,2,2,2,2,2,2,2,2,2,2,2,2,2,2,2,
2,2,2,2,2,2,2,2,2,2,2,2,2,2,2,2,2,2,2,2,2,2,2,2,2,2,2,2,2,2,2,2,2,2,2,2,
2,2,2,2,2,2,2,2,2,2,2,2,2,2,2,2,2,2,2,2,2,2,2,2,2,2,2,2,2,2,2,2,2,2,2,2,
2,2,2,2,2,2,2,2,2,2,2,2,2,2,2,2,2,2,2,2,2,2,2,2,2,2,2,2,2,2,2,2,2,2,2,2,
2,2,2,2,2,2,2,2,2,2,2,2,2,2,2,2,2,2,2,2,2,2,2,2,2,2,2,2,2,2,2,2,2,2,2,2,
2,2,2,2,2,2,2,2,2,2,2,2,2,2,2,2,2,2,2,2,2,2,2,2,2,2,2,2,2,2,2,2,2,2,2,2,
2,2,2,2,2,2,2,2,2,2,2,2,2,2,2,2,2,2,2,2,2,2,2,2,2,2,2,2,2,2,2,2,2,2,2,2,
2,2,4),(-4.06173053606492,-3.99264303614414,-3.94484835785685,-3.93735559998355,
-3.93521614870415,-3.93390924307517,-3.93272763841237,-3.93121621213845,
-3.92812126335377,-3.90877612379454,-3.9036422234948,-3.89712050512331,
-3.8128236543981,-3.78845749278649,-3.77949768982423,-3.77615167430205,
-3.77378674945593,-3.77282831858377,-3.77221389430502,-3.7715453283576,
-3.770743397285,-3.76876235051928,-3.75120052475007,-3.75036001707103,-3.71927516592442,
-3.69746709833839,-3.64791831888225,-3.62231286077033,-3.61472294684731,
-3.61257343342437,-3.61126417835272,-3.61008291637658,-3.60857533248586,
-3.60560193780343,-3.5879540991384,-3.58310720217572,-3.51111422070594,
-3.47868490999338,-3.46064605434355,-3.4550531182303,-3.45268485188964,
-3.45089138372212,-3.45003730221702,-3.44940721684852,-3.44877963568405,
-3.44790032963799,-3.44559200185814,-3.40550548517388,-3.38214724556063,
-3.33866800639041,-3.29471002283131,-3.29094935811541,-3.28931233540183,
-3.28811143515288,-3.28700536304904,-3.28550886820951,-3.28259419288882,
-3.2599757286754,-3.25196197466975,-3.20451516546109,-3.15681553436925,
-3.13445693623121,-3.13099240456683,-3.12932739559036,-3.12797725110428,
-3.12721884766654,-3.12662545940449,-3.12585638729191,-3.12451460157863,
-3.11926016132402,-3.0113154327832,-2.97527745973739,-2.96896372002264,
-2.96695483347477,-2.96567707553461,-2.96448696048117,-2.96294070992385,
-2.95970198306808,-2.93600909727482,-2.92651184440248,-2.83901753091584,
-2.81037632474626,-2.80756663156588,-2.80613814904991,-2.80525327646317,
-2.80444191581472,-2.80379749096938,-2.80305330001174,-2.80178694138151,
-2.79741950095655,-2.71478282397944,-2.6486154801934,-2.64517000979253,
-2.64359071003381,-2.64239957726533,-2.64127878095986,-2.63972511469512,
-2.63658483139031,-2.60665635943988,-2.53331614478316,-2.50881070835075,
-2.48686198874991,-2.48323741860155,-2.48210568448133,-2.48139163237983,
-2.48072616472114,-2.47984721455847,-2.47787840611672,-2.46071583876957,
-2.45732241253205,-2.36294042199256,-2.32938153115206,-2.32333934188926,
-2.32136360610057,-2.32009321355554,-2.31890022777551,-2.31733625067446,
-2.31470082572,-2.29855623104818,-2.29667865817754,-2.2908076709268,-2.28006334183379,
-2.27403223640754,-2.19972198979496,-2.17319586770569,-2.16137911881433,
-2.15975402547841,-2.15893259981489,-2.15827642912776,-2.15752354308551,
-2.15625104959744,-2.15168935952669,-2.05539045819502,-2.03142774934723,
-2.00311358054126,-1.99967362779058,-1.99811253654006,-1.99692007459681,
-1.99564861676447,-1.99366788754656,-1.98758495296315,-1.89423735176611,
-1.85004337640933,-1.83875090562492,-1.83699913316001,-1.83615214829198,
-1.83549341972214,-1.83475672571841,-1.83352372569639,-1.82893189463437,
-1.79613151984194,-1.70811750861109,-1.68029497816602,-1.67687044583286,
-1.67531220196706,-1.67412019566093,-1.67284755511164,-1.67086154161174,
-1.66473588138089,-1.57029637613813,-1.5258475857883,-1.51584740628491,
-1.51417967546572,-1.51333802211168,-1.51267988705974,-1.51194005969009,
-1.51069310663446,-1.50595065573003,-1.47115109057596,-1.41273715946364,
-1.35830366104016,-1.35444511952713,-1.35291502561912,-1.35180041766073,
-1.35060570389171,-1.34903626622373,-1.34560972519387,-1.34106665314426,
-1.29967671956274,-1.23207162864324,-1.20706582530678,-1.20636022675044,
-1.19340938410148,-1.19176779043052,-1.1909301916008,-1.19031358879223,
-1.18964092329423,-1.18870523628331,-1.18647113261794,-1.18339119837556,
-1.14960945984518,-1.05588195739435,-1.03444739855447,-1.03125881967434,
-1.02974532527445,-1.02856019315321,-1.02745966805291,-1.02560020435027,
-1.02040272412348,-0.993933753576714,-0.934129392697989,-0.890644343056778,
-0.886883653438565,-0.883837406146768,-0.870704975186686,-0.868898099530721,
-0.868036727203534,-0.867374136961964,-0.866652414899742,-0.865486133933068,
-0.861554297337804,-0.836418227264234,-0.752953776746852,-0.739198709708271,
-0.712124426480502,-0.708724022951162,-0.707170302706462,-0.705979067048614,
-0.704879072209079,-0.703074810278662,-0.698257353894672,-0.691310069017453,
-0.671994125756401,-0.625410528122825,-0.551241930370032,-0.54704823483272,
-0.545801712935961,-0.545135852452928,-0.544480867136637,-0.543677472609889,
-0.542138920352289,-0.53268038504514,-0.523995392220786,-0.498244311534951,
-0.491131377823437,-0.437441734161144,-0.41923535604897,-0.389644431834765,
-0.386513155906929,-0.384961768628703,-0.383841601530186,-0.382650196159206,
-0.381483304089254,-0.378798378120559,-0.363251857950231,-0.34101501112171,
-0.314201777393347,-0.228847067213466,-0.224450586783784,-0.223180989816218,
-0.222436073329684,-0.221844533658508,-0.221043182586111,-0.219514621411093,
-0.210291879048887,-0.191420421920683,-0.122635644191065,-0.115494019344356,
-0.0967744990380212,-0.0669614794112179,-0.0638240600062391,-0.0622710547105643,
-0.0611503848441586,-0.0599590617582436,-0.0587924486679108,-0.0572628352817411,
-0.0548437482695064,-0.000956655812675297),.UNSPECIFIED.);
#841=B_SPLINE_CURVE_WITH_KNOTS('',3,(#51081,#51082,#51083,#51084,#51085,
#51086,#51087,#51088,#51089,#51090),.UNSPECIFIED.,.F.,.F.,(4,1,1,1,1,1,
1,4),(103.67256099167,104.647102545754,105.645894949522,106.64468735329,
107.643479757058,108.642272160826,109.641064564594,109.955736404437),
 .UNSPECIFIED.);
#842=B_SPLINE_CURVE_WITH_KNOTS('',3,(#51092,#51093,#51094,#51095,#51096,
#51097,#51098,#51099,#51100,#51101,#51102,#51103,#51104,#51105,#51106,#51107,
#51108,#51109,#51110,#51111,#51112,#51113,#51114,#51115,#51116,#51117,#51118,
#51119,#51120,#51121,#51122,#51123,#51124,#51125,#51126,#51127,#51128,#51129,
#51130,#51131,#51132,#51133,#51134,#51135,#51136,#51137,#51138,#51139,#51140,
#51141,#51142,#51143,#51144,#51145,#51146,#51147,#51148,#51149,#51150,#51151,
#51152,#51153,#51154,#51155,#51156,#51157,#51158,#51159,#51160,#51161,#51162,
#51163,#51164,#51165,#51166,#51167,#51168,#51169,#51170,#51171,#51172,#51173,
#51174,#51175,#51176,#51177,#51178,#51179,#51180,#51181,#51182,#51183,#51184,
#51185,#51186,#51187,#51188,#51189,#51190,#51191,#51192,#51193,#51194,#51195,
#51196,#51197,#51198,#51199,#51200,#51201,#51202,#51203,#51204,#51205,#51206,
#51207,#51208,#51209,#51210,#51211,#51212,#51213,#51214,#51215,#51216,#51217,
#51218,#51219,#51220,#51221,#51222,#51223,#51224,#51225,#51226,#51227,#51228,
#51229,#51230,#51231,#51232,#51233,#51234,#51235,#51236,#51237,#51238,#51239,
#51240,#51241,#51242,#51243,#51244,#51245,#51246,#51247,#51248,#51249,#51250,
#51251,#51252,#51253,#51254,#51255,#51256,#51257,#51258,#51259,#51260,#51261,
#51262,#51263,#51264,#51265,#51266,#51267,#51268,#51269,#51270,#51271,#51272,
#51273,#51274,#51275,#51276,#51277,#51278,#51279,#51280,#51281,#51282,#51283,
#51284,#51285,#51286,#51287,#51288,#51289,#51290,#51291,#51292,#51293,#51294,
#51295,#51296,#51297,#51298,#51299,#51300,#51301,#51302,#51303,#51304,#51305,
#51306,#51307,#51308,#51309,#51310,#51311,#51312,#51313,#51314,#51315,#51316,
#51317,#51318,#51319,#51320,#51321,#51322,#51323,#51324,#51325,#51326,#51327,
#51328,#51329,#51330,#51331,#51332,#51333,#51334,#51335,#51336,#51337,#51338,
#51339,#51340,#51341,#51342,#51343,#51344,#51345,#51346,#51347,#51348,#51349,
#51350,#51351,#51352,#51353,#51354,#51355,#51356,#51357,#51358,#51359,#51360,
#51361,#51362,#51363,#51364,#51365,#51366,#51367,#51368,#51369,#51370,#51371,
#51372,#51373,#51374,#51375,#51376,#51377,#51378,#51379,#51380,#51381,#51382,
#51383,#51384,#51385,#51386,#51387,#51388,#51389,#51390,#51391,#51392,#51393,
#51394,#51395,#51396,#51397,#51398,#51399,#51400,#51401,#51402,#51403,#51404,
#51405,#51406,#51407,#51408,#51409,#51410,#51411,#51412,#51413,#51414,#51415,
#51416,#51417,#51418,#51419,#51420,#51421,#51422,#51423,#51424,#51425,#51426,
#51427,#51428,#51429,#51430,#51431,#51432,#51433,#51434,#51435,#51436,#51437,
#51438,#51439,#51440,#51441,#51442,#51443,#51444,#51445,#51446,#51447,#51448,
#51449,#51450,#51451,#51452,#51453,#51454,#51455,#51456,#51457,#51458,#51459,
#51460,#51461,#51462,#51463,#51464,#51465,#51466,#51467,#51468,#51469,#51470,
#51471,#51472,#51473,#51474,#51475,#51476,#51477,#51478,#51479,#51480,#51481,
#51482,#51483,#51484,#51485,#51486,#51487,#51488,#51489,#51490,#51491,#51492,
#51493,#51494,#51495,#51496,#51497,#51498,#51499,#51500,#51501,#51502,#51503,
#51504,#51505,#51506,#51507,#51508,#51509,#51510,#51511,#51512,#51513,#51514,
#51515,#51516,#51517,#51518,#51519,#51520,#51521,#51522,#51523,#51524,#51525,
#51526,#51527,#51528,#51529,#51530,#51531,#51532,#51533,#51534,#51535,#51536,
#51537,#51538,#51539,#51540,#51541,#51542,#51543,#51544,#51545,#51546,#51547,
#51548,#51549,#51550,#51551,#51552,#51553,#51554,#51555,#51556,#51557,#51558,
#51559,#51560,#51561,#51562,#51563,#51564,#51565,#51566,#51567,#51568,#51569,
#51570,#51571,#51572,#51573,#51574,#51575,#51576,#51577,#51578,#51579,#51580,
#51581,#51582,#51583,#51584,#51585,#51586,#51587,#51588,#51589,#51590,#51591,
#51592,#51593,#51594,#51595,#51596,#51597,#51598,#51599,#51600,#51601,#51602,
#51603,#51604,#51605,#51606,#51607,#51608,#51609,#51610,#51611,#51612,#51613,
#51614,#51615,#51616,#51617,#51618,#51619,#51620,#51621,#51622,#51623,#51624,
#51625,#51626,#51627,#51628,#51629,#51630,#51631,#51632,#51633,#51634,#51635,
#51636,#51637,#51638,#51639,#51640,#51641,#51642,#51643,#51644,#51645,#51646,
#51647,#51648,#51649,#51650,#51651,#51652,#51653,#51654,#51655,#51656,#51657),
 .UNSPECIFIED.,.F.,.F.,(4,2,2,2,2,2,2,2,2,2,2,2,2,2,2,2,2,2,2,2,2,2,2,2,
2,2,2,2,2,2,2,2,2,2,2,2,2,2,2,2,2,2,2,2,2,2,2,2,2,2,2,2,2,2,2,2,2,2,2,2,
2,2,2,2,2,2,2,2,2,2,2,2,2,2,2,2,2,2,2,2,2,2,2,2,2,2,2,2,2,2,2,2,2,2,2,2,
2,2,2,2,2,2,2,2,2,2,2,2,2,2,2,2,2,2,2,2,2,2,2,2,2,2,2,2,2,2,2,2,2,2,2,2,
2,2,2,2,2,2,2,2,2,2,2,2,2,2,2,2,2,2,2,2,2,2,2,2,2,2,2,2,2,2,2,2,2,2,2,2,
2,2,2,2,2,2,2,2,2,2,2,2,2,2,2,2,2,2,2,2,2,2,2,2,2,2,2,2,2,2,2,2,2,2,2,2,
2,2,2,2,2,2,2,2,2,2,2,2,2,2,2,2,2,2,2,2,2,2,2,2,2,2,2,2,2,2,2,2,2,2,2,2,
2,2,2,2,2,2,2,2,2,2,2,2,2,2,2,2,2,2,2,2,2,2,2,2,2,2,2,2,2,2,2,2,2,2,2,2,
2,2,2,2,2,2,4),(-4.06063781096923,-4.05731981415401,-4.05493204612338,-4.05405547611466,
-4.05339709140699,-4.05277509561439,-4.05215957747037,-4.05132546753032,
-4.04969667783987,-4.04746614297703,-4.04326403066187,-3.94880956986452,
-3.90262327008353,-3.89528130962922,-3.89315817124286,-3.89185534755516,
-3.89067357316091,-3.88915655679123,-3.88603115813888,-3.86600337926848,
-3.8603899284599,-3.85467508185895,-3.84907160635317,-3.76365865655495,
-3.73940431971863,-3.73497260055438,-3.73297753766551,-3.73186166916856,
-3.73088572015443,-3.73021286442228,-3.72954682458925,-3.7287282515589,
-3.72672707238446,-3.70746908969222,-3.68432038179969,-3.66318293918734,
-3.65679254868836,-3.64945588456887,-3.64083689242829,-3.61260525155242,
-3.57860803202467,-3.57251809823496,-3.57053686265228,-3.56926553528361,
-3.56807351891859,-3.56651347630985,-3.56307773206154,-3.53487372840895,
-3.44427731738438,-3.42049611574097,-3.41382017520459,-3.41112300830772,
-3.40973652448865,-3.40886929940274,-3.40807086265942,-3.4074277753202,
-3.40667522572414,-3.40540365976966,-3.40084875387618,-3.31504627451749,
-3.3030766389839,-3.25246312756124,-3.24893910967758,-3.24734548121225,
-3.24615238365218,-3.24503617098564,-3.24349899437376,-3.23959694494856,
-3.17747264417216,-3.09314260630246,-3.08931743941957,-3.08752700375098,
-3.08649321755663,-3.08557553430906,-3.08514651218657,-3.08450219141766,
-3.08364870901516,-3.08186342670908,-3.06981126832831,-2.97798900654007,
-2.93442642431781,-2.92974537644303,-2.92621058904379,-2.92461492913071,
-2.92342146248629,-2.92230573934755,-2.92077054630504,-2.91688043320047,
-2.85768622918004,-2.85113583616591,-2.84358304026967,-2.79462941547942,
-2.76842342281109,-2.76575399182482,-2.76437789215205,-2.7635150158085,
-2.76271965410571,-2.76207688741806,-2.76141980250643,-2.76021630248024,
-2.75638035113015,-2.68838080293436,-2.63791704732392,-2.61241871416025,
-2.60487965747516,-2.60273585316696,-2.60142820171785,-2.60024716813251,
-2.59873819371189,-2.5956542923349,-2.57652993769076,-2.57143880879908,
-2.55715257302761,-2.48087638175396,-2.45415898466579,-2.44259823607874,
-2.4409816855277,-2.44016213160225,-2.43950624720595,-2.43884986580951,
-2.43764994699046,-2.43384303510625,-2.36765949138991,-2.3517713323542,
-2.28445680503371,-2.2810085667686,-2.2794290072221,-2.27823809670365,-2.27711781658982,
-2.27556535396729,-2.27242902849891,-2.24262579203528,-2.19463350944136,
-2.14775173422193,-2.12952698900693,-2.11991166596451,-2.11836679794293,
-2.11756218312176,-2.11690727930576,-2.1162424314581,-2.1150004660964,-2.11084458825208,
-2.03147581385238,-2.01273883292165,-1.9625415108435,-1.95872612421727,
-1.95720367157684,-1.95609127818727,-1.95489576499217,-1.9532876183956,
-1.94968477857289,-1.90768421633015,-1.85807797372953,-1.79985106899913,
-1.79656818735679,-1.79543769614386,-1.79479531335656,-1.79420240462004,
-1.79338708311564,-1.79179092470171,-1.78083064960815,-1.75281713394966,
-1.72536071318246,-1.66468690849567,-1.65897623391533,-1.6388787947221,
-1.6357496092877,-1.63423159923777,-1.63304943200903,-1.6317465619234,-1.62962421723337,
-1.62229336690498,-1.57622403306197,-1.47864046183971,-1.4741926747754,
-1.47291753111798,-1.47217145073474,-1.47158017990598,-1.47078072271387,
-1.46926075412567,-1.46022810565488,-1.44108668051645,-1.39369339702938,
-1.31821706740442,-1.31374164539671,-1.31211188378765,-1.31097060156912,
-1.30981193278721,-1.30833724215702,-1.30672860705067,-1.30412115494985,
-1.29898569538024,-1.24767773288631,-1.16277868956499,-1.15222826906672,
-1.15051179179217,-1.14967182182469,-1.14901387570077,-1.14827305076915,
-1.14702161918303,-1.14222966479954,-1.10674082459561,-1.01315844462675,
-0.993326489122193,-0.99020904934278,-0.988693212961755,-0.987536006302111,
-0.986805087038092,-0.985207420311045,-0.983427834613196,-0.980408883842235,
-0.974142071959428,-0.957346917346883,-0.93616504367092,-0.832378145149048,
-0.828486794726983,-0.827276141811284,-0.826617435097182,-0.825961584237627,
-0.825145548902246,-0.823546930831487,-0.812530941472452,-0.784274767680891,
-0.772585675630654,-0.721053344311418,-0.671698824144621,-0.667892739487543,
-0.66637147899449,-0.665259063070078,-0.664086743499903,-0.662523488591205,
-0.660792023553347,-0.657889968463439,-0.651950269948339,-0.636332925815105,
-0.61644592932972,-0.566621020365257,-0.509141635531219,-0.50571884665159,
-0.504568372423816,-0.503921785534318,-0.5033295425707,-0.502521925532216,
-0.500963786439337,-0.491034709971074,-0.468147849628446,-0.442831005654773,
-0.434738535995411,-0.407453215973505,-0.349167784872187,-0.345280978576924,
-0.343745921623834,-0.34262988776584,-0.341459615721182,-0.339910127097627,
-0.338196986888664,-0.3353392168193,-0.329522257885625,-0.314340344843652,
-0.276961113514679,-0.202877031195031,-0.200028666006729,-0.199673487941102,
-0.196055536991565,-0.184123393789331,-0.182342738898069,-0.181489934620054,
-0.180830362306391,-0.180096602163226,-0.178877228846258,-0.174430310859571,
-0.143448522374149,-0.0400412049537006,-0.0331754686402422,-0.0310183526667614,
-0.0235248573812635,-0.0212903812577373,-0.0199621151414786,-0.0188042245762228,
-0.0176704612255242,-0.0162411519802988,-0.0140600772172354,-0.000956836703198815),
 .UNSPECIFIED.);
#843=B_SPLINE_CURVE_WITH_KNOTS('',3,(#51659,#51660,#51661,#51662,#51663,
#51664,#51665,#51666,#51667,#51668,#51669,#51670,#51671,#51672,#51673,#51674,
#51675,#51676,#51677,#51678,#51679,#51680,#51681,#51682,#51683,#51684,#51685,
#51686,#51687,#51688,#51689,#51690,#51691,#51692,#51693,#51694,#51695,#51696,
#51697,#51698,#51699,#51700,#51701,#51702,#51703,#51704,#51705,#51706,#51707,
#51708,#51709,#51710,#51711,#51712,#51713,#51714,#51715,#51716,#51717,#51718,
#51719,#51720,#51721,#51722,#51723,#51724,#51725,#51726,#51727,#51728,#51729,
#51730,#51731,#51732,#51733,#51734,#51735,#51736,#51737,#51738,#51739,#51740,
#51741,#51742,#51743,#51744,#51745,#51746,#51747,#51748,#51749,#51750,#51751,
#51752,#51753,#51754,#51755,#51756,#51757,#51758,#51759,#51760,#51761,#51762,
#51763,#51764,#51765,#51766,#51767,#51768,#51769,#51770,#51771,#51772,#51773,
#51774,#51775,#51776,#51777,#51778,#51779,#51780,#51781,#51782,#51783,#51784,
#51785,#51786,#51787,#51788,#51789,#51790,#51791,#51792,#51793,#51794,#51795,
#51796,#51797,#51798,#51799,#51800,#51801,#51802,#51803,#51804,#51805,#51806,
#51807,#51808,#51809,#51810,#51811,#51812,#51813,#51814,#51815,#51816,#51817,
#51818,#51819,#51820,#51821,#51822,#51823,#51824,#51825,#51826,#51827,#51828,
#51829,#51830,#51831,#51832,#51833,#51834,#51835,#51836,#51837,#51838,#51839,
#51840,#51841,#51842,#51843,#51844,#51845,#51846,#51847,#51848,#51849,#51850,
#51851,#51852,#51853,#51854,#51855,#51856,#51857,#51858,#51859,#51860,#51861,
#51862,#51863,#51864,#51865,#51866,#51867,#51868,#51869,#51870,#51871,#51872,
#51873,#51874,#51875,#51876,#51877,#51878,#51879,#51880,#51881,#51882,#51883,
#51884,#51885,#51886,#51887,#51888,#51889,#51890,#51891,#51892,#51893,#51894,
#51895,#51896,#51897,#51898,#51899,#51900,#51901,#51902,#51903,#51904,#51905,
#51906,#51907,#51908,#51909,#51910,#51911,#51912,#51913,#51914,#51915,#51916,
#51917,#51918,#51919,#51920,#51921,#51922,#51923,#51924,#51925,#51926,#51927,
#51928,#51929,#51930,#51931,#51932,#51933,#51934,#51935,#51936,#51937,#51938,
#51939,#51940,#51941,#51942,#51943,#51944,#51945,#51946,#51947,#51948,#51949,
#51950,#51951,#51952,#51953,#51954,#51955,#51956,#51957,#51958,#51959,#51960,
#51961,#51962,#51963,#51964,#51965,#51966,#51967,#51968,#51969,#51970,#51971,
#51972,#51973,#51974,#51975,#51976,#51977,#51978,#51979,#51980,#51981,#51982,
#51983,#51984,#51985,#51986,#51987,#51988,#51989,#51990,#51991,#51992,#51993,
#51994,#51995,#51996,#51997,#51998,#51999,#52000,#52001,#52002,#52003,#52004,
#52005,#52006,#52007,#52008,#52009,#52010,#52011,#52012,#52013,#52014,#52015,
#52016,#52017,#52018,#52019,#52020,#52021,#52022,#52023,#52024,#52025,#52026,
#52027,#52028,#52029,#52030,#52031,#52032,#52033,#52034,#52035,#52036,#52037,
#52038,#52039,#52040,#52041,#52042,#52043,#52044,#52045,#52046,#52047,#52048,
#52049,#52050,#52051,#52052,#52053,#52054,#52055,#52056,#52057,#52058,#52059,
#52060,#52061,#52062,#52063,#52064,#52065,#52066,#52067,#52068,#52069,#52070,
#52071,#52072,#52073,#52074,#52075,#52076,#52077,#52078,#52079,#52080,#52081,
#52082,#52083,#52084,#52085,#52086,#52087,#52088,#52089,#52090,#52091,#52092,
#52093,#52094,#52095,#52096,#52097,#52098,#52099,#52100,#52101,#52102,#52103,
#52104,#52105,#52106,#52107,#52108,#52109,#52110,#52111,#52112,#52113,#52114,
#52115,#52116,#52117,#52118,#52119,#52120,#52121,#52122,#52123,#52124,#52125,
#52126,#52127,#52128,#52129,#52130,#52131,#52132,#52133,#52134,#52135,#52136,
#52137,#52138,#52139,#52140,#52141,#52142,#52143,#52144,#52145,#52146,#52147,
#52148,#52149,#52150,#52151,#52152,#52153,#52154,#52155,#52156,#52157,#52158,
#52159,#52160,#52161,#52162,#52163,#52164,#52165,#52166,#52167,#52168,#52169,
#52170,#52171,#52172,#52173,#52174,#52175,#52176,#52177,#52178,#52179,#52180,
#52181,#52182,#52183,#52184,#52185,#52186,#52187,#52188,#52189,#52190,#52191,
#52192,#52193,#52194),.UNSPECIFIED.,.F.,.F.,(4,2,2,2,2,2,2,2,2,2,2,2,2,
2,2,2,2,2,2,2,2,2,2,2,2,2,2,2,2,2,2,2,2,2,2,2,2,2,2,2,2,2,2,2,2,2,2,2,2,
2,2,2,2,2,2,2,2,2,2,2,2,2,2,2,2,2,2,2,2,2,2,2,2,2,2,2,2,2,2,2,2,2,2,2,2,
2,2,2,2,2,2,2,2,2,2,2,2,2,2,2,2,2,2,2,2,2,2,2,2,2,2,2,2,2,2,2,2,2,2,2,2,
2,2,2,2,2,2,2,2,2,2,2,2,2,2,2,2,2,2,2,2,2,2,2,2,2,2,2,2,2,2,2,2,2,2,2,2,
2,2,2,2,2,2,2,2,2,2,2,2,2,2,2,2,2,2,2,2,2,2,2,2,2,2,2,2,2,2,2,2,2,2,2,2,
2,2,2,2,2,2,2,2,2,2,2,2,2,2,2,2,2,2,2,2,2,2,2,2,2,2,2,2,2,2,2,2,2,2,2,2,
2,2,2,2,2,2,2,2,2,2,2,2,2,2,2,2,2,2,2,2,2,2,2,2,2,2,2,2,2,2,2,2,2,2,2,2,
2,2,4),(-4.05932261802918,-3.94718619145327,-3.92809093087277,-3.91911955207525,
-3.91760275599314,-3.91680415072275,-3.91621315676654,-3.9154669527404,
-3.91419047575874,-3.90972786546289,-3.81963845278496,-3.78303009534929,
-3.76798484889305,-3.76220738073496,-3.75936439301799,-3.7576577503187,
-3.75611523835994,-3.75494619777213,-3.7538302195544,-3.75229342938824,
-3.74839269670435,-3.68633818526492,-3.64994132301906,-3.59749009169381,
-3.59536753150999,-3.5944514929179,-3.59378266126145,-3.59316194920748,
-3.59230760096305,-3.59059921323149,-3.57564990070719,-3.49350528039842,
-3.45961154536527,-3.44515804416145,-3.43954952387634,-3.43676800928572,
-3.43508692889591,-3.43357991698403,-3.43241235435313,-3.43129387235999,
-3.42974745254961,-3.42578929679905,-3.35923772249199,-3.31285592803571,
-3.27827970434388,-3.27355529763417,-3.27231044614131,-3.27157134749633,
-3.27091352211781,-3.27007181242301,-3.26840254246408,-3.25835945977218,
-3.21377491260917,-3.12304217155674,-3.11718705469083,-3.11431604883399,
-3.11259784567634,-3.11104443473474,-3.10987611414841,-3.1087625394867,
-3.10723465212028,-3.10338578050594,-3.04975306427779,-2.99055093928644,
-2.95575563221633,-2.9510153783639,-2.94976913604699,-2.94902975720943,
-2.94837203750011,-2.94753093977968,-2.94580727683437,-2.93509776667768,
-2.85042628699211,-2.7992048379846,-2.79407490710356,-2.79146986087013,
-2.78986251625508,-2.78838865962902,-2.78723069243043,-2.78608989200054,
-2.78446046249791,-2.7799837361825,-2.70426021262851,-2.65702289994102,
-2.63793011095452,-2.62895936355373,-2.62744280433519,-2.62664433870224,
-2.62605345455559,-2.62530739780633,-2.6240311932988,-2.61956972223699,
-2.5224212750323,-2.47609700951169,-2.46874269201359,-2.46661853933616,
-2.46531565640758,-2.46413419817715,-2.46261810327591,-2.45949643285783,
-2.43954054311265,-2.43307202513359,-2.35890687780683,-2.33463762251458,
-2.31558609092321,-2.30642638894341,-2.30490148448641,-2.30410128749428,
-2.30351027160373,-2.30286077194628,-2.30169401085176,-2.29814207532942,
-2.23794795641187,-2.18917912263447,-2.16590504525583,-2.14755958793992,
-2.14474951693844,-2.14329685993158,-2.14223395771725,-2.14109146478605,
-2.1391176462441,-2.13361096972731,-2.12789383645975,-2.02995606576609,
-1.98574053698561,-1.98300114252315,-1.98205706583568,-1.98141190307608,
-1.98081987958671,-1.98001094213419,-1.97844481528347,-1.9682906528721,
-1.94402702210448,-1.89479969303414,-1.85196781063417,-1.84544048437153,
-1.82552509248755,-1.82240479476043,-1.82088878504062,-1.81970712997985,
-1.81840376263382,-1.81627821815792,-1.80891327157105,-1.76247270539797,
-1.66536748421636,-1.66090129785883,-1.65962434422935,-1.65887798358763,
-1.65828693393508,-1.65748834314583,-1.65597186177543,-1.64701003779624,
-1.62792989175814,-1.5807598081821,-1.53641146788433,-1.52662423648838,
-1.5214276050629,-1.51961808611955,-1.50270251044742,-1.49976790446488,
-1.4982690088048,-1.49708916705714,-1.49577591863669,-1.49360704095215,
-1.48581784599507,-1.43464507918231,-1.34296925524164,-1.33833599228516,
-1.33705606755409,-1.33630151172824,-1.33564563219065,-1.33484332967692,
-1.33329099785979,-1.33131500157843,-1.28021233633798,-1.21142834937144,
-1.20597253903291,-1.20032869042724,-1.18026882970569,-1.17714113711538,
-1.17562333563879,-1.17444109791264,-1.17313791385746,-1.17101452653429,
-1.16367496702171,-1.11751629708463,-1.02559224838059,-1.01624816366084,
-1.01461550586423,-1.01378139561017,-1.01312407850158,-1.01239478592759,
-1.01116959810087,-1.00969358508122,-1.00675484102546,-0.975746885084139,
-0.92590922596784,-0.883985483800203,-0.877563261099115,-0.85758806507461,
-0.854463848941587,-0.852946581351915,-0.851764238012896,-0.850460408183944,
-0.848334777470833,-0.840975982669745,-0.794618226968018,-0.72145079869608,
-0.694435476053143,-0.692285122685145,-0.691432178962731,-0.690811609428396,
-0.690142047054751,-0.689241995945121,-0.68719685873267,-0.684414828456267,
-0.677452391139539,-0.662978159807999,-0.623447930895032,-0.552965890060782,
-0.551914756275635,-0.534692463460466,-0.531741409121149,-0.530238660709844,
-0.529058014210598,-0.527746171099943,-0.525584910186803,-0.517877491787067,
-0.492036811824751,-0.461993250933704,-0.455553082600992,-0.407179502722541,
-0.394575463562312,-0.37170295819498,-0.369631365047125,-0.368792032874973,
-0.368174994851585,-0.36755193213565,-0.366894525696385,-0.365336455877824,
-0.355275959863369,-0.33148116118891,-0.311723113356212,-0.249933768699635,
-0.245226592200497,-0.239242005766237,-0.231549569889586,-0.212276439618882,
-0.209184742222764,-0.20767391298561,-0.206492322725152,-0.205184970528625,
-0.203043738003696,-0.19553436804252,-0.147549550928869,-0.0923282060039677,
-0.087045437847226,-0.0654385759082482,-0.0611863058379246,-0.0486395021768235,
-0.0470125458883691,-0.0461787094473289,-0.0455630670267084,-0.0449408873179125,
-0.0442820125657699,-0.0434045401258508,-0.041993761853196,-0.000956483055879518),
 .UNSPECIFIED.);
#844=B_SPLINE_CURVE_WITH_KNOTS('',3,(#52196,#52197,#52198,#52199,#52200,
#52201,#52202,#52203,#52204,#52205,#52206,#52207,#52208,#52209,#52210,#52211,
#52212,#52213,#52214,#52215,#52216,#52217,#52218,#52219,#52220,#52221,#52222,
#52223,#52224,#52225,#52226,#52227,#52228,#52229,#52230,#52231,#52232,#52233,
#52234,#52235,#52236,#52237,#52238,#52239,#52240,#52241,#52242,#52243,#52244,
#52245,#52246,#52247,#52248,#52249,#52250,#52251,#52252,#52253,#52254,#52255,
#52256,#52257,#52258,#52259,#52260,#52261,#52262,#52263,#52264,#52265,#52266,
#52267,#52268,#52269,#52270,#52271,#52272,#52273,#52274,#52275,#52276,#52277,
#52278,#52279,#52280,#52281,#52282,#52283,#52284,#52285,#52286,#52287,#52288,
#52289,#52290,#52291,#52292,#52293,#52294,#52295,#52296,#52297,#52298,#52299,
#52300,#52301,#52302,#52303,#52304,#52305,#52306,#52307,#52308,#52309,#52310,
#52311,#52312,#52313,#52314,#52315,#52316,#52317,#52318,#52319,#52320,#52321,
#52322,#52323,#52324,#52325,#52326,#52327,#52328,#52329,#52330,#52331,#52332,
#52333,#52334,#52335,#52336,#52337,#52338,#52339,#52340,#52341,#52342,#52343,
#52344,#52345,#52346,#52347,#52348,#52349,#52350,#52351,#52352,#52353,#52354,
#52355,#52356,#52357,#52358,#52359,#52360,#52361,#52362,#52363,#52364,#52365,
#52366,#52367,#52368,#52369,#52370,#52371,#52372,#52373,#52374,#52375,#52376,
#52377,#52378,#52379,#52380,#52381,#52382,#52383,#52384,#52385,#52386,#52387,
#52388,#52389,#52390,#52391,#52392,#52393,#52394,#52395,#52396,#52397,#52398,
#52399,#52400,#52401,#52402,#52403,#52404,#52405,#52406,#52407,#52408,#52409,
#52410,#52411,#52412,#52413,#52414,#52415,#52416,#52417,#52418,#52419,#52420,
#52421,#52422,#52423,#52424,#52425,#52426,#52427,#52428,#52429,#52430,#52431,
#52432,#52433,#52434,#52435,#52436,#52437,#52438,#52439,#52440,#52441,#52442,
#52443,#52444,#52445,#52446,#52447,#52448,#52449,#52450,#52451,#52452,#52453,
#52454,#52455,#52456,#52457,#52458,#52459,#52460,#52461,#52462,#52463,#52464,
#52465,#52466,#52467,#52468,#52469,#52470,#52471,#52472,#52473,#52474,#52475,
#52476,#52477,#52478,#52479,#52480,#52481,#52482,#52483,#52484,#52485,#52486,
#52487,#52488,#52489,#52490,#52491,#52492,#52493,#52494,#52495,#52496,#52497,
#52498,#52499,#52500,#52501,#52502,#52503,#52504,#52505,#52506,#52507,#52508,
#52509,#52510,#52511,#52512,#52513,#52514,#52515,#52516,#52517,#52518,#52519,
#52520,#52521,#52522,#52523,#52524,#52525,#52526,#52527,#52528,#52529,#52530,
#52531,#52532,#52533,#52534,#52535,#52536,#52537,#52538,#52539,#52540,#52541,
#52542,#52543,#52544,#52545,#52546,#52547,#52548,#52549,#52550,#52551,#52552,
#52553,#52554,#52555,#52556,#52557,#52558,#52559,#52560,#52561,#52562,#52563,
#52564,#52565,#52566,#52567,#52568,#52569,#52570,#52571,#52572,#52573,#52574,
#52575,#52576,#52577,#52578,#52579,#52580,#52581,#52582,#52583,#52584,#52585,
#52586,#52587,#52588,#52589,#52590,#52591,#52592,#52593,#52594,#52595,#52596,
#52597,#52598,#52599,#52600,#52601,#52602,#52603,#52604,#52605,#52606,#52607,
#52608,#52609,#52610,#52611,#52612,#52613,#52614,#52615,#52616,#52617,#52618,
#52619,#52620,#52621,#52622,#52623,#52624,#52625,#52626,#52627,#52628,#52629,
#52630,#52631,#52632,#52633,#52634,#52635,#52636,#52637,#52638,#52639,#52640,
#52641,#52642,#52643,#52644,#52645,#52646,#52647,#52648,#52649,#52650,#52651,
#52652,#52653,#52654,#52655,#52656,#52657,#52658,#52659,#52660,#52661,#52662,
#52663,#52664,#52665,#52666,#52667,#52668,#52669,#52670,#52671,#52672,#52673,
#52674,#52675,#52676,#52677,#52678,#52679,#52680,#52681,#52682,#52683,#52684,
#52685,#52686,#52687,#52688,#52689,#52690,#52691,#52692,#52693,#52694,#52695,
#52696,#52697,#52698,#52699,#52700,#52701,#52702,#52703,#52704,#52705,#52706,
#52707,#52708,#52709,#52710,#52711,#52712,#52713,#52714,#52715,#52716,#52717,
#52718,#52719,#52720,#52721,#52722,#52723,#52724,#52725,#52726,#52727,#52728,
#52729,#52730,#52731,#52732,#52733),.UNSPECIFIED.,.F.,.F.,(4,2,2,2,2,2,
2,2,2,2,2,2,2,2,2,2,2,2,2,2,2,2,2,2,2,2,2,2,2,2,2,2,2,2,2,2,2,2,2,2,2,2,
2,2,2,2,2,2,2,2,2,2,2,2,2,2,2,2,2,2,2,2,2,2,2,2,2,2,2,2,2,2,2,2,2,2,2,2,
2,2,2,2,2,2,2,2,2,2,2,2,2,2,2,2,2,2,2,2,2,2,2,2,2,2,2,2,2,2,2,2,2,2,2,2,
2,2,2,2,2,2,2,2,2,2,2,2,2,2,2,2,2,2,2,2,2,2,2,2,2,2,2,2,2,2,2,2,2,2,2,2,
2,2,2,2,2,2,2,2,2,2,2,2,2,2,2,2,2,2,2,2,2,2,2,2,2,2,2,2,2,2,2,2,2,2,2,2,
2,2,2,2,2,2,2,2,2,2,2,2,2,2,2,2,2,2,2,2,2,2,2,2,2,2,2,2,2,2,2,2,2,2,2,2,
2,2,2,2,2,2,2,2,2,2,2,2,2,2,2,2,2,2,2,2,2,2,2,2,2,2,2,2,2,2,2,2,2,2,2,2,
2,2,2,2,2,2,2,2,2,2,4),(-4.06075874161792,-3.98610762050859,-3.95340645274498,
-3.9474606547773,-3.94549738830649,-3.94423002723069,-3.94303631844564,
-3.94146620849038,-3.93880894078993,-3.92222994581067,-3.83224930180272,
-3.81338738761118,-3.78833954713899,-3.78466199201783,-3.78381231749805,
-3.78316346566348,-3.78253436033305,-3.78190809079028,-3.78103306267748,
-3.77924217307012,-3.76138047146936,-3.75549508160315,-3.74467557349034,
-3.70875708554463,-3.67353861318805,-3.63201582196343,-3.62512873620835,
-3.62305415550328,-3.62176196458069,-3.62057698380681,-3.61906313144738,
-3.61587173865262,-3.59435953321201,-3.52074269448731,-3.48166490862495,
-3.4690884380765,-3.46480754080062,-3.46193259088222,-3.46089707261786,
-3.4602835696196,-3.45962028693457,-3.45875385961736,-3.45685215405933,
-3.44178686432493,-3.44091362949828,-3.43996393494279,-3.43890085556761,
-3.42821658954846,-3.35551603382603,-3.32019785963148,-3.30374186790685,
-3.3010073976106,-3.29957024076967,-3.29850876661142,-3.29735820759772,
-3.29569454193968,-3.29099323181756,-3.21690141014196,-3.16951644080574,
-3.14359960058933,-3.14094714620724,-3.13957738556252,-3.13845756751828,
-3.13773712125085,-3.13707829057859,-3.13622941643561,-3.13446752527795,
-3.12294646837749,-3.03729236060468,-2.98233991551047,-2.97879692406513,
-2.97719975237968,-2.97600604238203,-2.97489073408241,-2.97335711798215,
-2.96947628774928,-2.91192121149933,-2.84918011621408,-2.82117667906771,
-2.81840334273092,-2.81698847611232,-2.81580484066623,-2.81508511272102,
-2.81442613587945,-2.81357587565009,-2.81180685465431,-2.80012509457277,
-2.73444980666313,-2.69097716257303,-2.66517191390396,-2.65747822020727,
-2.65531875128943,-2.65400755940859,-2.65282721722685,-2.65132446981306,
-2.64837219647718,-2.63111495355163,-2.62983958543947,-2.62591535226356,
-2.61343356176322,-2.61126508376648,-2.52897106090484,-2.49592048130302,
-2.49378806707527,-2.49287011322963,-2.49220077585795,-2.49158025672335,
-2.49072715012814,-2.489024239535,-2.47425858190168,-2.41081878901101,-2.33699496964111,
-2.33353041523372,-2.33194775507372,-2.33075631312879,-2.3296368566074,
-2.32808763474004,-2.32496439836249,-2.29565519526841,-2.20856706358912,
-2.17631048193914,-2.17176204625211,-2.1705332319086,-2.16979752728574,
-2.16913868314289,-2.16829019380492,-2.16653052333102,-2.1550616792619,
-2.15328717158991,-2.15271201634402,-2.07317271502636,-2.03108706288559,
-2.01359300382855,-2.01062807591605,-2.00912252161027,-2.00794174782285,
-2.00663190107838,-2.00447882682588,-1.99685028422291,-1.97116486856814,
-1.92790563909832,-1.85338733248369,-1.84915060408523,-1.84789916009374,
-1.84723232384135,-1.8465837049106,-1.84578482358669,-1.84426754609871,
-1.83529438921099,-1.81619944533137,-1.76898332023829,-1.69334280549139,
-1.68877911326154,-1.68713594169643,-1.68599097175559,-1.68492793907007,
-1.68347843485539,-1.68068585328748,-1.66282740169784,-1.62061964251767,
-1.53096068330205,-1.5264817316112,-1.52520309023005,-1.52445618328523,
-1.5238649512425,-1.52306643402025,-1.52155112836383,-1.51262423005136,
-1.49358583541313,-1.4465660167532,-1.37054170574068,-1.36602322587058,
-1.36438680213263,-1.36324361691271,-1.362179944736,-1.36075522499681,-1.35804794864587,
-1.35464493259904,-1.32941742698359,-1.30570090387805,-1.23661501946852,
-1.2053610088884,-1.20314559311054,-1.20228152571019,-1.201658043469,-1.20099049161116,
-1.20008343177585,-1.19801298489131,-1.17337970931843,-1.14954723994569,
-1.07324781701648,-1.04615544681051,-1.04275415699607,-1.0412001626498,
-1.04000877141227,-1.03873421980967,-1.0367797619644,-1.03087615570099,
-0.998308332499085,-0.938115476308948,-0.896417365984515,-0.895463838611336,
-0.893920111382816,-0.881997981016917,-0.880218070907458,-0.879374659349585,
-0.878714615556626,-0.877983711867653,-0.876776582342343,-0.872558965221797,
-0.852506048067094,-0.830635033430468,-0.770835500925901,-0.756434778586312,
-0.747830464485669,-0.7424976129598,-0.72309082939253,-0.719992877017493,
-0.718480814695982,-0.717299091384188,-0.715992441203287,-0.713897001627106,
-0.70677851346872,-0.695341957177579,-0.655430644261318,-0.621223779417774,
-0.595643798136869,-0.582563855194721,-0.559930677976956,-0.557864447900867,
-0.557026071541431,-0.556409293441287,-0.555736846206907,-0.554802180215169,
-0.552573871011485,-0.535911022564283,-0.512196359182349,-0.460384618762866,
-0.401806256750432,-0.397918534883089,-0.396383504313612,-0.395267625491593,
-0.394073735252269,-0.392902131807994,-0.391358267573132,-0.384442103852216,
-0.373423985716377,-0.340830663919388,-0.315466307354785,-0.240212044051322,
-0.23591280778266,-0.234654140707828,-0.233985793734345,-0.23333718013636,
-0.232540403798336,-0.231033354238017,-0.22245407097745,-0.177126902451215,
-0.160485085827147,-0.14284817708322,-0.079177482182616,-0.0752709206875294,
-0.0737326398628456,-0.072615859952655,-0.071422375926071,-0.0702516132194086,
-0.0687102326821668,-0.0662631654880025,-0.00095691374464929),
 .UNSPECIFIED.);
#845=B_SPLINE_CURVE_WITH_KNOTS('',3,(#52735,#52736,#52737,#52738,#52739,
#52740,#52741,#52742,#52743,#52744,#52745,#52746,#52747,#52748,#52749,#52750,
#52751,#52752,#52753,#52754,#52755,#52756,#52757,#52758,#52759,#52760,#52761,
#52762,#52763,#52764,#52765,#52766,#52767,#52768,#52769,#52770,#52771,#52772,
#52773,#52774,#52775,#52776,#52777,#52778,#52779,#52780,#52781,#52782,#52783,
#52784,#52785,#52786,#52787,#52788,#52789,#52790,#52791,#52792,#52793,#52794,
#52795,#52796,#52797,#52798,#52799,#52800,#52801,#52802,#52803,#52804,#52805,
#52806,#52807,#52808,#52809,#52810,#52811,#52812,#52813,#52814,#52815,#52816,
#52817,#52818,#52819,#52820,#52821,#52822,#52823,#52824,#52825,#52826,#52827,
#52828,#52829,#52830,#52831,#52832,#52833,#52834,#52835,#52836,#52837,#52838,
#52839,#52840,#52841,#52842,#52843,#52844,#52845,#52846,#52847,#52848,#52849,
#52850,#52851,#52852,#52853,#52854,#52855,#52856,#52857,#52858,#52859,#52860,
#52861,#52862,#52863,#52864,#52865,#52866,#52867,#52868,#52869,#52870,#52871,
#52872,#52873,#52874,#52875,#52876,#52877,#52878,#52879,#52880,#52881,#52882,
#52883,#52884,#52885,#52886,#52887,#52888,#52889,#52890,#52891,#52892,#52893,
#52894,#52895,#52896,#52897,#52898,#52899,#52900,#52901,#52902,#52903,#52904,
#52905,#52906,#52907,#52908,#52909,#52910,#52911,#52912,#52913,#52914,#52915,
#52916,#52917,#52918,#52919,#52920,#52921,#52922,#52923,#52924,#52925,#52926,
#52927,#52928,#52929,#52930,#52931,#52932,#52933,#52934,#52935,#52936,#52937,
#52938,#52939,#52940,#52941,#52942,#52943,#52944,#52945,#52946,#52947,#52948,
#52949,#52950,#52951,#52952,#52953,#52954,#52955,#52956,#52957,#52958,#52959,
#52960,#52961,#52962,#52963,#52964,#52965,#52966,#52967,#52968,#52969,#52970,
#52971,#52972,#52973,#52974,#52975,#52976,#52977,#52978,#52979,#52980,#52981,
#52982,#52983,#52984,#52985,#52986,#52987,#52988,#52989,#52990,#52991,#52992,
#52993,#52994,#52995,#52996,#52997,#52998,#52999,#53000,#53001,#53002,#53003,
#53004,#53005,#53006,#53007,#53008,#53009,#53010,#53011,#53012,#53013,#53014,
#53015,#53016,#53017,#53018,#53019,#53020,#53021,#53022,#53023,#53024,#53025,
#53026,#53027,#53028,#53029,#53030,#53031,#53032,#53033,#53034,#53035,#53036,
#53037,#53038,#53039,#53040,#53041,#53042,#53043,#53044,#53045,#53046,#53047,
#53048,#53049,#53050,#53051,#53052,#53053,#53054,#53055,#53056,#53057,#53058,
#53059,#53060,#53061,#53062,#53063,#53064,#53065,#53066,#53067,#53068,#53069,
#53070,#53071,#53072,#53073,#53074,#53075,#53076,#53077,#53078,#53079,#53080,
#53081,#53082,#53083,#53084,#53085,#53086,#53087,#53088,#53089,#53090,#53091,
#53092,#53093,#53094,#53095,#53096,#53097,#53098,#53099,#53100,#53101,#53102,
#53103,#53104,#53105,#53106,#53107,#53108,#53109,#53110,#53111,#53112,#53113,
#53114,#53115,#53116,#53117,#53118,#53119,#53120,#53121,#53122,#53123,#53124,
#53125,#53126,#53127,#53128,#53129,#53130,#53131,#53132,#53133,#53134,#53135,
#53136,#53137,#53138,#53139,#53140,#53141,#53142,#53143,#53144,#53145,#53146,
#53147,#53148,#53149,#53150,#53151,#53152,#53153,#53154,#53155,#53156,#53157,
#53158,#53159,#53160,#53161,#53162,#53163,#53164,#53165,#53166,#53167,#53168,
#53169,#53170,#53171,#53172,#53173,#53174,#53175,#53176,#53177,#53178,#53179,
#53180,#53181,#53182,#53183,#53184,#53185,#53186,#53187,#53188,#53189,#53190,
#53191,#53192,#53193,#53194,#53195,#53196,#53197,#53198,#53199,#53200,#53201,
#53202,#53203,#53204,#53205,#53206,#53207,#53208,#53209,#53210,#53211,#53212,
#53213,#53214,#53215,#53216,#53217,#53218,#53219,#53220,#53221,#53222,#53223,
#53224,#53225,#53226,#53227,#53228,#53229,#53230,#53231,#53232,#53233,#53234,
#53235,#53236,#53237,#53238,#53239,#53240,#53241,#53242,#53243,#53244,#53245,
#53246,#53247,#53248,#53249,#53250,#53251,#53252,#53253,#53254),
 .UNSPECIFIED.,.F.,.F.,(4,2,2,2,2,2,2,2,2,2,2,2,2,2,2,2,2,2,2,2,2,2,2,2,
2,2,2,2,2,2,2,2,2,2,2,2,2,2,2,2,2,2,2,2,2,2,2,2,2,2,2,2,2,2,2,2,2,2,2,2,
2,2,2,2,2,2,2,2,2,2,2,2,2,2,2,2,2,2,2,2,2,2,2,2,2,2,2,2,2,2,2,2,2,2,2,2,
2,2,2,2,2,2,2,2,2,2,2,2,2,2,2,2,2,2,2,2,2,2,2,2,2,2,2,2,2,2,2,2,2,2,2,2,
2,2,2,2,2,2,2,2,2,2,2,2,2,2,2,2,2,2,2,2,2,2,2,2,2,2,2,2,2,2,2,2,2,2,2,2,
2,2,2,2,2,2,2,2,2,2,2,2,2,2,2,2,2,2,2,2,2,2,2,2,2,2,2,2,2,2,2,2,2,2,2,2,
2,2,2,2,2,2,2,2,2,2,2,2,2,2,2,2,2,2,2,2,2,2,2,2,2,2,2,2,2,2,2,2,2,2,2,2,
2,2,2,2,2,2,2,2,2,2,2,2,2,2,2,2,2,2,2,4),(-4.06019698931433,-3.97695450267513,
-3.97393430511519,-3.97242861270744,-3.9711715913942,-3.97042959900369,
-3.96977199694071,-3.96893431166321,-3.96722879794313,-3.95689198784149,
-3.88192677400402,-3.8582425023994,-3.81955722427489,-3.81263606631032,
-3.81109250666641,-3.80992112016608,-3.80872743624955,-3.80761174065082,
-3.80607694701041,-3.80218974761543,-3.74361678277193,-3.70939383921679,
-3.6721353974461,-3.65743604732047,-3.65017091372532,-3.64873262127818,
-3.64795070345073,-3.64736092079791,-3.64670004868253,-3.64547797456863,
-3.64149068181466,-3.56757946105376,-3.52167896423041,-3.49287889367005,
-3.4890962464564,-3.48781037005358,-3.48654510797325,-3.48535013417216,
-3.48377362205424,-3.48024934141457,-3.44906595356631,-3.42878102578146,
-3.37143223682587,-3.34994720088628,-3.33727572783858,-3.32778759648618,
-3.32624039650016,-3.32543526253,-3.32484348615073,-3.32419604933717,-3.32304054723902,
-3.31957519008414,-3.26226178790138,-3.21498640899134,-3.18878903266453,
-3.16956631082883,-3.16638241131776,-3.16481605482077,-3.16362204206302,
-3.16250695753445,-3.16097444188294,-3.15791764472456,-3.13096404153667,
-3.11730469568757,-3.03933576752033,-3.00900464465246,-3.00610242521389,
-3.00397155059318,-3.00305384839157,-3.00238453751884,-3.00176392648197,
-3.00091052193429,-2.99920649048525,-2.98440730571568,-2.95737942641187,
-2.89625865408434,-2.85209637626979,-2.8449741804413,-2.84287802279331,
-2.84157134124282,-2.84038986344522,-2.83887849458754,-2.83578329528635,
-2.81642725008816,-2.81119577506522,-2.71219985435423,-2.68587963827327,
-2.68320313489041,-2.68120540100166,-2.68031152975641,-2.67964616826552,
-2.67901900803923,-2.67814113759271,-2.67633930714462,-2.65806568901537,
-2.57662859146933,-2.52963081727253,-2.52221147984607,-2.52007960156352,
-2.5187743978272,-2.51759241898612,-2.51607785869288,-2.51296713722453,
-2.4932835840774,-2.4878094536777,-2.47969271490891,-2.39666445416615,-2.37756620746901,
-2.36011538934497,-2.35835452905756,-2.35750572288416,-2.35690793373471,
-2.35627872838251,-2.3553932986818,-2.3535607259485,-2.33402700947926,-2.3178193934521,
-2.29581995466206,-2.25485338266581,-2.22564735180887,-2.20354607498151,
-2.19886026173639,-2.19707097617181,-2.19584059635912,-2.19463689124796,
-2.19318818370314,-2.18957912386824,-2.1552335095384,-2.15085432803292,
-2.07559028822923,-2.04131006289086,-2.03820615353857,-2.03595828626849,
-2.03502020391007,-2.03434704482447,-2.03373088098402,-2.03289515592525,
-2.03084445992978,-1.98907413668802,-1.88255440830362,-1.87653891062244,
-1.87449166139925,-1.87333399718429,-1.8722737224416,-1.87084975525582,
-1.86817825385619,-1.85310479057138,-1.82366100193944,-1.77352520511806,
-1.71697181757311,-1.71477968917716,-1.71294521429595,-1.71209134300707,
-1.71142985225814,-1.71070443984429,-1.70952175546062,-1.70543655679243,
-1.67863485773535,-1.62917572259533,-1.55777039446591,-1.55336706805946,
-1.55174834902818,-1.55061005438552,-1.54954498699203,-1.54807995007571,
-1.54521311589833,-1.5253228467184,-1.49913234576748,-1.41878552333166,
-1.39260282759426,-1.39046723933438,-1.38961683016286,-1.38899692907907,
-1.38832690018277,-1.38740566224938,-1.38525518770638,-1.35008188092155,
-1.23745863427864,-1.23110328786188,-1.22900983257798,-1.22784298537131,
-1.22667798402257,-1.22525261919757,-1.222551130484,-1.21915051180542,-1.19395106498149,
-1.15818353674507,-1.07268972362682,-1.06826463307934,-1.06699197582423,
-1.06624644089026,-1.06565508306576,-1.06485484217533,-1.06333121611249,
-1.05421702760808,-1.03508612247613,-0.948062505052561,-0.93404923849643,
-0.91041607797363,-0.907179835080305,-0.905634175246147,-0.904444247483404,
-0.903344263855925,-0.901529639300561,-0.896644063786488,-0.889572242278826,
-0.860448827482918,-0.811095125566238,-0.759527163979478,-0.746544608070626,
-0.744902095371414,-0.744064329640685,-0.743447750564691,-0.74277526222774,
-0.741840086822431,-0.739608446855437,-0.736532659260694,-0.702831044992888,
-0.633651012381926,-0.588633424816174,-0.584889148175464,-0.583378786367023,
-0.582269387496917,-0.581071516246165,-0.579892454359496,-0.577063472711181,
-0.558261868175069,-0.536261813073066,-0.502268776363443,-0.427250267455445,
-0.42296735270491,-0.421710635059904,-0.42104273377329,-0.4203941809635,
-0.41959695041246,-0.418087473885397,-0.409285138478339,-0.39046306605224,
-0.353885815073532,-0.317450310587326,-0.266166494941265,-0.262338855956694,
-0.260814088923615,-0.259700914135983,-0.258505422367755,-0.257330791189235,
-0.255778397529117,-0.248726494873167,-0.214666778752984,-0.192598282054413,
-0.104966044982071,-0.1003768607073,-0.0991013916488177,-0.098347772748269,
-0.0976916228600743,-0.0968710769117434,-0.0952504564359993,-0.083576346611283,
-0.0569497684135954,-0.000958016727391121),.UNSPECIFIED.);
#846=B_SPLINE_CURVE_WITH_KNOTS('',3,(#53256,#53257,#53258,#53259,#53260,
#53261,#53262,#53263,#53264,#53265,#53266,#53267,#53268,#53269,#53270,#53271,
#53272,#53273,#53274,#53275,#53276,#53277,#53278,#53279,#53280,#53281,#53282,
#53283,#53284,#53285,#53286,#53287,#53288,#53289,#53290,#53291,#53292,#53293,
#53294,#53295,#53296,#53297,#53298,#53299,#53300,#53301,#53302,#53303,#53304,
#53305,#53306,#53307,#53308,#53309,#53310,#53311,#53312,#53313,#53314,#53315,
#53316,#53317,#53318,#53319,#53320,#53321,#53322,#53323,#53324,#53325,#53326,
#53327,#53328,#53329,#53330,#53331,#53332,#53333,#53334,#53335,#53336,#53337,
#53338,#53339,#53340,#53341,#53342,#53343,#53344,#53345,#53346,#53347,#53348,
#53349,#53350,#53351,#53352,#53353,#53354,#53355,#53356,#53357,#53358,#53359,
#53360,#53361,#53362,#53363,#53364,#53365,#53366,#53367,#53368,#53369,#53370,
#53371,#53372,#53373,#53374,#53375,#53376,#53377,#53378,#53379,#53380,#53381,
#53382,#53383,#53384,#53385,#53386,#53387,#53388,#53389,#53390,#53391,#53392,
#53393,#53394,#53395,#53396,#53397,#53398,#53399,#53400,#53401,#53402,#53403,
#53404,#53405,#53406,#53407,#53408,#53409,#53410,#53411,#53412,#53413,#53414,
#53415,#53416,#53417,#53418,#53419,#53420,#53421,#53422,#53423,#53424,#53425,
#53426,#53427,#53428,#53429,#53430,#53431,#53432,#53433,#53434,#53435,#53436,
#53437,#53438,#53439,#53440,#53441,#53442,#53443,#53444,#53445,#53446,#53447,
#53448,#53449,#53450,#53451,#53452,#53453,#53454,#53455,#53456,#53457,#53458,
#53459,#53460,#53461,#53462,#53463,#53464,#53465,#53466,#53467,#53468,#53469,
#53470,#53471,#53472,#53473,#53474,#53475,#53476,#53477,#53478,#53479,#53480,
#53481,#53482,#53483,#53484,#53485,#53486,#53487,#53488,#53489,#53490,#53491,
#53492,#53493,#53494,#53495,#53496,#53497,#53498,#53499,#53500,#53501,#53502,
#53503,#53504,#53505,#53506,#53507,#53508,#53509,#53510,#53511,#53512,#53513,
#53514,#53515,#53516,#53517,#53518,#53519,#53520,#53521,#53522,#53523,#53524,
#53525,#53526,#53527,#53528,#53529,#53530,#53531,#53532,#53533,#53534,#53535,
#53536,#53537,#53538,#53539,#53540,#53541,#53542,#53543,#53544,#53545,#53546,
#53547,#53548,#53549,#53550,#53551,#53552,#53553,#53554,#53555,#53556,#53557,
#53558,#53559,#53560,#53561,#53562,#53563,#53564,#53565,#53566,#53567,#53568,
#53569,#53570,#53571,#53572,#53573,#53574,#53575,#53576,#53577,#53578,#53579,
#53580,#53581,#53582,#53583,#53584,#53585,#53586,#53587,#53588,#53589,#53590,
#53591,#53592,#53593,#53594,#53595,#53596,#53597,#53598,#53599,#53600,#53601,
#53602,#53603,#53604,#53605,#53606,#53607,#53608,#53609,#53610,#53611,#53612,
#53613,#53614,#53615,#53616,#53617,#53618,#53619,#53620,#53621,#53622,#53623,
#53624,#53625,#53626,#53627,#53628,#53629,#53630,#53631,#53632,#53633,#53634,
#53635,#53636,#53637,#53638,#53639,#53640,#53641,#53642,#53643,#53644,#53645,
#53646,#53647,#53648,#53649,#53650,#53651,#53652,#53653,#53654,#53655,#53656,
#53657,#53658,#53659,#53660,#53661,#53662,#53663,#53664,#53665,#53666,#53667,
#53668,#53669,#53670,#53671,#53672,#53673,#53674,#53675,#53676,#53677,#53678,
#53679,#53680,#53681,#53682,#53683,#53684,#53685,#53686,#53687,#53688,#53689,
#53690,#53691,#53692,#53693,#53694,#53695,#53696,#53697,#53698,#53699,#53700,
#53701,#53702,#53703,#53704,#53705,#53706,#53707,#53708,#53709,#53710,#53711,
#53712,#53713,#53714,#53715,#53716,#53717,#53718,#53719,#53720,#53721,#53722,
#53723,#53724,#53725,#53726,#53727,#53728,#53729,#53730,#53731,#53732,#53733,
#53734,#53735,#53736,#53737,#53738,#53739,#53740,#53741,#53742,#53743,#53744,
#53745,#53746,#53747,#53748,#53749,#53750,#53751,#53752,#53753,#53754,#53755,
#53756,#53757,#53758,#53759,#53760,#53761,#53762,#53763,#53764,#53765,#53766,
#53767,#53768,#53769,#53770,#53771,#53772,#53773,#53774,#53775,#53776,#53777,
#53778,#53779,#53780,#53781,#53782,#53783,#53784,#53785,#53786,#53787,#53788,
#53789,#53790,#53791,#53792,#53793,#53794,#53795,#53796,#53797,#53798,#53799,
#53800,#53801),.UNSPECIFIED.,.F.,.F.,(4,2,2,2,2,2,2,2,2,2,2,2,2,2,2,2,2,
2,2,2,2,2,2,2,2,2,2,2,2,2,2,2,2,2,2,2,2,2,2,2,2,2,2,2,2,2,2,2,2,2,2,2,2,
2,2,2,2,2,2,2,2,2,2,2,2,2,2,2,2,2,2,2,2,2,2,2,2,2,2,2,2,2,2,2,2,2,2,2,2,
2,2,2,2,2,2,2,2,2,2,2,2,2,2,2,2,2,2,2,2,2,2,2,2,2,2,2,2,2,2,2,2,2,2,2,2,
2,2,2,2,2,2,2,2,2,2,2,2,2,2,2,2,2,2,2,2,2,2,2,2,2,2,2,2,2,2,2,2,2,2,2,2,
2,2,2,2,2,2,2,2,2,2,2,2,2,2,2,2,2,2,2,2,2,2,2,2,2,2,2,2,2,2,2,2,2,2,2,2,
2,2,2,2,2,2,2,2,2,2,2,2,2,2,2,2,2,2,2,2,2,2,2,2,2,2,2,2,2,2,2,2,2,2,2,2,
2,2,2,2,2,2,2,2,2,2,2,2,2,2,2,2,2,2,2,2,2,2,2,2,2,2,2,2,2,2,2,2,2,2,2,2,
2,2,2,4),(-4.06084665564884,-4.0028780513959,-4.00042071920944,-3.99887522503487,
-3.99770325483983,-3.99650935743439,-3.99539454443845,-3.9938626581458,
-3.9899917009456,-3.93383984104344,-3.92080358884868,-3.86095583541986,
-3.84672535486906,-3.83806592724142,-3.83656340569911,-3.8357677761187,
-3.83511944618217,-3.83445081224778,-3.83318991971986,-3.82886834335183,
-3.75244909765839,-3.73480647265931,-3.69615736252467,-3.68491185283819,
-3.67788574330586,-3.67633496108725,-3.67516109281549,-3.67396617197069,
-3.67285297998951,-3.67132733571929,-3.66749306124244,-3.61544394587349,
-3.55821293806315,-3.53299229457196,-3.51592868449372,-3.51417556525937,
-3.51332848492551,-3.51273114960538,-3.51210170422558,-3.51121482264067,
-3.50885821992887,-3.4668078565601,-3.4348277067004,-3.38667431338305,-3.3668200882538,
-3.35601685573383,-3.3536027972697,-3.35246376412079,-3.35139595919912,
-3.35026662431209,-3.34868015515922,-3.34540643784939,-3.30985514934358,
-3.3005700992973,-3.22078252563658,-3.19747970433049,-3.1925607992896,-3.19129827756834,
-3.19055509058197,-3.18989774741418,-3.1890621439357,-3.18736680531489,
-3.17723289501793,-3.13258202339751,-3.08058586982539,-3.05976544506857,
-3.03697217692271,-3.03222675220852,-3.03043288450582,-3.02933296809575,
-3.02814049547682,-3.02657868688788,-3.02313428511907,-2.99466652576593,
-2.90315753797758,-2.87410758700642,-2.86982431227166,-2.86862134871743,
-2.86789142347827,-2.86723121591107,-2.86638620624857,-2.86459777823003,
-2.85247569190688,-2.85110979204019,-2.85069200685696,-2.84727414143885,
-2.84513313123652,-2.82636316240316,-2.75772201168065,-2.74193073828499,
-2.71497856794903,-2.71144435067359,-2.70865144481789,-2.70720887650912,
-2.70614290176253,-2.70500761431294,-2.70339977183464,-2.69906498474173,
-2.62587885863892,-2.57988900227957,-2.55141999415833,-2.54862014358062,
-2.54654932848517,-2.54564226039769,-2.54497476262775,-2.54435137631128,
-2.54348751061889,-2.54127297515948,-2.51006985440719,-2.48140761328028,
-2.43191093936057,-2.4030064846174,-2.38854961000189,-2.38590876258827,
-2.38449136636726,-2.38343174243704,-2.38210147444006,-2.37985750279757,
-2.37227965071849,-2.37029098327736,-2.366881473546,-2.32714905988595,-2.30534309580936,
-2.26611898821354,-2.23665299189941,-2.22537576825694,-2.2237684425753,
-2.22295071217099,-2.22229486916986,-2.22153942941618,-2.22025586967219,
-2.21558839374699,-2.12016188911211,-2.07244009508194,-2.0649544932126,
-2.06281599083778,-2.06150942745812,-2.06032797736067,-2.05881653432756,
-2.05572079826507,-2.03635162370017,-2.0310813328872,-2.01167690602365,
-1.96143553271675,-1.90495052660509,-1.90179129250714,-1.90067794731483,
-1.90003894762906,-1.89944499391653,-1.89862188505124,-1.8969882385081,
-1.88489180411392,-1.85859926124186,-1.78707349931804,-1.76841295810416,
-1.76337342519935,-1.74403937463855,-1.74094527104516,-1.73943415259866,
-1.73825274066622,-1.73694599922674,-1.73480670563862,-1.72731340948495,
-1.67949748196618,-1.58408696572139,-1.57944272540835,-1.57816152304118,
-1.5774065950316,-1.57675063563528,-1.57593204068365,-1.57432072956475,
-1.56292775818497,-1.53291770894004,-1.43780970500761,-1.42100691940546,
-1.41807815228675,-1.4165803315435,-1.4154003966438,-1.41408607054968,-1.41191316092933,
-1.40408607610754,-1.35247441950122,-1.2612955578568,-1.25662517075267,
-1.25534120392499,-1.25458560926862,-1.25393384482551,-1.25313455047342,
-1.25159443281484,-1.24963915897217,-1.18542342771808,-1.11665876280134,
-1.11559268784128,-1.0982783824633,-1.09532251338532,-1.09381875088855,
-1.09263801050707,-1.091326787687,-1.08916821210506,-1.08148732602759,-1.05569784653198,
-1.01223719941998,-0.979440507164036,-0.936097869553703,-0.93344378434712,
-0.932511877509622,-0.931869903682166,-0.931229692366292,-0.930405931843433,
-0.928752711667427,-0.92661632712634,-0.921753887304315,-0.90676794220684,
-0.856828288791959,-0.778147023738427,-0.773508743208243,-0.771854269118318,
-0.770706112388515,-0.769643778880089,-0.768200795315442,-0.765439601081213,
-0.748364507563801,-0.709808756004757,-0.632430689401104,-0.63046209877142,
-0.62870390076376,-0.625757180280605,-0.624980366404814,-0.612126637459858,
-0.610488505042411,-0.609651795192603,-0.609035420377114,-0.608412776176412,
-0.607527406671135,-0.605572695734177,-0.60293703929106,-0.596468565054953,
-0.575070671996718,-0.544435509044801,-0.475035657539108,-0.473386672774535,
-0.467711975043182,-0.452741656879062,-0.450168920148042,-0.448623338714239,
-0.447433273340431,-0.446155111514457,-0.44414463127366,-0.437818197101808,
-0.401657571647373,-0.359767395379664,-0.317360810816575,-0.290077606997822,
-0.28792264499455,-0.287068935790219,-0.286448182970211,-0.285822713503579,
-0.285168887176482,-0.283644376730748,-0.274415223717295,-0.255647988357035,
-0.239630346018512,-0.148702508918191,-0.147593628698093,-0.130274722700396,
-0.127318798847395,-0.125815104355112,-0.124634464223438,-0.123323401018756,
-0.121165198987564,-0.11348676927498,-0.0877030398018594,-0.000958356721493471),
 .UNSPECIFIED.);
#847=B_SPLINE_CURVE_WITH_KNOTS('',3,(#53803,#53804,#53805,#53806,#53807,
#53808,#53809,#53810,#53811,#53812,#53813,#53814,#53815,#53816,#53817,#53818,
#53819,#53820,#53821,#53822,#53823,#53824,#53825,#53826,#53827,#53828,#53829,
#53830,#53831,#53832,#53833,#53834,#53835,#53836,#53837,#53838,#53839,#53840,
#53841,#53842,#53843,#53844,#53845,#53846,#53847,#53848,#53849,#53850,#53851,
#53852,#53853,#53854,#53855,#53856,#53857,#53858,#53859,#53860,#53861,#53862,
#53863,#53864,#53865,#53866,#53867,#53868,#53869,#53870,#53871,#53872,#53873,
#53874,#53875,#53876,#53877,#53878,#53879,#53880,#53881,#53882,#53883,#53884,
#53885,#53886,#53887,#53888,#53889,#53890,#53891,#53892,#53893,#53894,#53895,
#53896,#53897,#53898,#53899,#53900,#53901,#53902,#53903,#53904,#53905,#53906,
#53907,#53908,#53909,#53910,#53911,#53912,#53913,#53914,#53915,#53916,#53917,
#53918,#53919,#53920,#53921,#53922,#53923,#53924,#53925,#53926,#53927,#53928,
#53929,#53930,#53931,#53932,#53933,#53934,#53935,#53936,#53937,#53938,#53939,
#53940,#53941,#53942,#53943,#53944,#53945,#53946,#53947,#53948,#53949,#53950,
#53951,#53952,#53953,#53954,#53955,#53956,#53957,#53958,#53959,#53960,#53961,
#53962,#53963,#53964,#53965,#53966,#53967,#53968,#53969,#53970,#53971,#53972,
#53973,#53974,#53975,#53976,#53977,#53978,#53979,#53980,#53981,#53982,#53983,
#53984,#53985,#53986,#53987,#53988,#53989,#53990,#53991,#53992,#53993,#53994,
#53995,#53996,#53997,#53998,#53999,#54000,#54001,#54002,#54003,#54004,#54005,
#54006,#54007,#54008,#54009,#54010,#54011,#54012,#54013,#54014,#54015,#54016,
#54017,#54018,#54019,#54020,#54021,#54022,#54023,#54024,#54025,#54026,#54027,
#54028,#54029,#54030,#54031,#54032,#54033,#54034,#54035,#54036,#54037,#54038,
#54039,#54040,#54041,#54042,#54043,#54044,#54045,#54046,#54047,#54048,#54049,
#54050,#54051,#54052,#54053,#54054,#54055,#54056,#54057,#54058,#54059,#54060,
#54061,#54062,#54063,#54064,#54065,#54066,#54067,#54068,#54069,#54070,#54071,
#54072,#54073,#54074,#54075,#54076,#54077,#54078,#54079,#54080,#54081,#54082,
#54083,#54084,#54085,#54086,#54087,#54088,#54089,#54090,#54091,#54092,#54093,
#54094,#54095,#54096,#54097,#54098,#54099,#54100,#54101,#54102,#54103,#54104,
#54105,#54106,#54107,#54108,#54109,#54110,#54111,#54112,#54113,#54114,#54115,
#54116,#54117,#54118,#54119,#54120,#54121,#54122,#54123,#54124,#54125,#54126,
#54127,#54128,#54129,#54130,#54131,#54132,#54133,#54134,#54135,#54136,#54137,
#54138,#54139,#54140,#54141,#54142,#54143,#54144,#54145,#54146,#54147,#54148,
#54149,#54150,#54151,#54152,#54153,#54154,#54155,#54156,#54157,#54158,#54159,
#54160,#54161,#54162,#54163,#54164,#54165,#54166,#54167,#54168,#54169,#54170,
#54171,#54172,#54173,#54174,#54175,#54176,#54177,#54178,#54179,#54180,#54181,
#54182,#54183,#54184,#54185,#54186,#54187,#54188,#54189,#54190,#54191,#54192,
#54193,#54194,#54195,#54196,#54197,#54198,#54199,#54200,#54201,#54202,#54203,
#54204,#54205,#54206,#54207,#54208,#54209,#54210,#54211,#54212,#54213,#54214,
#54215,#54216,#54217,#54218,#54219,#54220,#54221,#54222,#54223,#54224,#54225,
#54226,#54227,#54228,#54229,#54230,#54231,#54232,#54233,#54234,#54235,#54236,
#54237,#54238,#54239,#54240,#54241,#54242,#54243,#54244,#54245,#54246,#54247,
#54248,#54249,#54250,#54251,#54252,#54253,#54254,#54255,#54256,#54257,#54258,
#54259,#54260,#54261,#54262,#54263,#54264,#54265,#54266,#54267,#54268,#54269,
#54270,#54271,#54272,#54273,#54274,#54275,#54276,#54277,#54278,#54279,#54280,
#54281,#54282,#54283,#54284,#54285,#54286,#54287,#54288,#54289,#54290,#54291,
#54292,#54293,#54294,#54295,#54296,#54297,#54298,#54299,#54300,#54301,#54302,
#54303,#54304,#54305,#54306,#54307,#54308,#54309,#54310,#54311,#54312,#54313,
#54314,#54315,#54316,#54317,#54318,#54319,#54320,#54321,#54322,#54323,#54324,
#54325,#54326,#54327,#54328,#54329,#54330,#54331,#54332,#54333,#54334,#54335,
#54336),.UNSPECIFIED.,.F.,.F.,(4,2,2,2,2,2,2,2,2,2,2,2,2,2,2,2,2,2,2,2,
2,2,2,2,2,2,2,2,2,2,2,2,2,2,2,2,2,2,2,2,2,2,2,2,2,2,2,2,2,2,2,2,2,2,2,2,
2,2,2,2,2,2,2,2,2,2,2,2,2,2,2,2,2,2,2,2,2,2,2,2,2,2,2,2,2,2,2,2,2,2,2,2,
2,2,2,2,2,2,2,2,2,2,2,2,2,2,2,2,2,2,2,2,2,2,2,2,2,2,2,2,2,2,2,2,2,2,2,2,
2,2,2,2,2,2,2,2,2,2,2,2,2,2,2,2,2,2,2,2,2,2,2,2,2,2,2,2,2,2,2,2,2,2,2,2,
2,2,2,2,2,2,2,2,2,2,2,2,2,2,2,2,2,2,2,2,2,2,2,2,2,2,2,2,2,2,2,2,2,2,2,2,
2,2,2,2,2,2,2,2,2,2,2,2,2,2,2,2,2,2,2,2,2,2,2,2,2,2,2,2,2,2,2,2,2,2,2,2,
2,2,2,2,2,2,2,2,2,2,2,2,2,2,2,2,2,2,2,2,2,2,2,2,2,2,2,2,2,2,4),(-4.06037209229428,
-4.02640913549226,-4.02504603866398,-4.02418868183135,-4.02353723092419,
-4.02291060247345,-4.02228792406252,-4.02142600964768,-4.01922159591739,
-3.98868429987278,-3.98388367217803,-3.92403925518192,-3.88413301701106,
-3.86676127380683,-3.86398900393097,-3.86254414327959,-3.86148205834355,
-3.86033574298703,-3.85868660654864,-3.85408055076813,-3.85229852113474,
-3.74861586758456,-3.72193257955187,-3.70936570669668,-3.70508737885633,
-3.70221092344829,-3.70117704982093,-3.70056367975202,-3.69990033234403,
-3.69903292540613,-3.69712548783886,-3.68187895887367,-3.68122880962401,
-3.66869381646718,-3.61932981463282,-3.61314374104717,-3.60580315493032,
-3.5968202708822,-3.58518149476958,-3.54909110310954,-3.54277252429512,
-3.54076348454315,-3.53948597495551,-3.5382963327726,-3.5367510393908,-3.5341782077674,
-3.51919347886417,-3.51495083163536,-3.44437762478163,-3.40854196383101,
-3.38989915539538,-3.38377420366753,-3.38124253154513,-3.37934629172893,
-3.37847454964509,-3.37784934931223,-3.37722889397738,-3.37637576252615,
-3.37467245723807,-3.3598877648246,-3.35844118610148,-3.35460502239932,
-3.27371736841735,-3.22774720668829,-3.22042522002019,-3.2183039872667,
-3.21700147825746,-3.2158194271038,-3.2143012707974,-3.21117073383994,-3.19103648388762,
-3.18515238702846,-3.10928068650413,-3.07947728086454,-3.06057104188322,
-3.05835957185709,-3.05665988718641,-3.05582667547211,-3.05519041887597,
-3.05455387469196,-3.05345240233324,-3.05037523131688,-2.99688625709063,
-2.90357405612487,-2.89749240669817,-2.89551228981326,-2.89424127468884,
-2.89304926316966,-2.89148881197816,-2.88805047712412,-2.85975714801818,
-2.77195991838237,-2.7394119722766,-2.73639421194111,-2.73488948707351,
-2.73397300638607,-2.73317142396205,-2.73252210197848,-2.7318900687036,
-2.73099363737232,-2.72857376613876,-2.68565036073925,-2.62945420995895,
-2.58262853746982,-2.57522621292564,-2.5730965530655,-2.57179212310483,
-2.57061046215371,-2.56909577696221,-2.56598291861817,-2.54623718540984,
-2.54473181795764,-2.46928228956254,-2.41373138063906,-2.41160580883417,
-2.41068912746642,-2.41002007796818,-2.40939935053494,-2.40854525675795,
-2.4068382246516,-2.39193927397282,-2.35859793967623,-2.33141594388722,
-2.30477660417554,-2.25987678314051,-2.25511279449212,-2.2515277102166,
-2.24992277236893,-2.24872775619021,-2.24761446668442,-2.24608867520263,
-2.24225396027311,-2.1901883776986,-2.12909356783482,-2.10331941725205,
-2.09051318055266,-2.08885862139936,-2.08803128177093,-2.08743680554677,
-2.08679969794487,-2.08569564255834,-2.08260130096764,-2.03166839848904,
-1.96328263158965,-1.95698715610408,-1.95151686386301,-1.93182203520147,
-1.92871130102069,-1.92719695270389,-1.92601523826596,-1.92471042726512,
-1.92257941817028,-1.91516533044424,-1.8682064277294,-1.77172766105245,
-1.76718830661844,-1.76590318021374,-1.76515487683486,-1.76456389262974,
-1.76376743506938,-1.76226159358856,-1.75353737512461,-1.73488097787056,
-1.69112686980541,-1.6116696257496,-1.60684050115156,-1.60497095481778,
-1.6038485060017,-1.60265846984708,-1.6010854512624,-1.59767270057822,-1.53934315974291,
-1.4490957415655,-1.44445156352843,-1.44317034216603,-1.44241539511016,
-1.4417594142684,-1.44094078619409,-1.43932938935112,-1.42793501977486,
-1.39791901064057,-1.30339992452531,-1.28605971416785,-1.28310267214911,
-1.28159873893875,-1.28044232460678,-1.27916531782585,-1.27783273392812,
-1.27588213617923,-1.27244355174192,-1.24675027158748,-1.2228528709134,
-1.12609023386585,-1.12158557401631,-1.12030405986131,-1.1195564729064,
-1.11896526890078,-1.11816751267975,-1.11665598629907,-1.10781376232755,
-1.08891442821059,-1.04247108026109,-0.96567946800784,-0.961121107469808,
-0.959478555304893,-0.958333621022034,-0.957176740473526,-0.955710335608556,
-0.954113503986432,-0.951534445925017,-0.946475484320042,-0.920683521925532,
-0.877218517377548,-0.80299567884522,-0.798795782674685,-0.797548397017467,
-0.796882282142163,-0.796227178679169,-0.795423829745015,-0.793885938536731,
-0.784448233629749,-0.77172521137124,-0.729958517925943,-0.675917526938045,
-0.641539959767883,-0.637930709470467,-0.636481909022103,-0.635290303110902,
-0.634086686442692,-0.632362264141079,-0.630406783631054,-0.626956410292478,
-0.619450435106283,-0.596012373336783,-0.550961374560593,-0.490368831628682,
-0.487073050284924,-0.476917230017275,-0.47522028903973,-0.474384157934497,
-0.473726524834264,-0.472983144044041,-0.471720606754265,-0.466805406167451,
-0.443513121518276,-0.392394235644475,-0.365081507815186,-0.319217003047633,
-0.315458634800603,-0.313945552144851,-0.312835217280349,-0.311661301465675,
-0.310088981231741,-0.308345660794175,-0.305414991345334,-0.299395810212257,
-0.20874642529792,-0.164154900034783,-0.1541408492381,-0.152472106198326,
-0.151630108932222,-0.150971787274006,-0.150231838534827,-0.148984883746677,
-0.144244761686984,-0.109485172234029,-0.000957829592074313),
 .UNSPECIFIED.);
#848=B_SPLINE_CURVE_WITH_KNOTS('',3,(#54338,#54339,#54340,#54341,#54342,
#54343,#54344,#54345,#54346,#54347,#54348,#54349,#54350,#54351,#54352,#54353,
#54354,#54355,#54356,#54357,#54358,#54359,#54360,#54361,#54362,#54363,#54364,
#54365,#54366,#54367,#54368,#54369,#54370,#54371,#54372,#54373,#54374,#54375,
#54376,#54377,#54378,#54379,#54380,#54381,#54382,#54383,#54384,#54385,#54386,
#54387,#54388,#54389,#54390,#54391,#54392,#54393,#54394,#54395,#54396,#54397,
#54398,#54399,#54400,#54401,#54402,#54403,#54404,#54405,#54406,#54407,#54408,
#54409,#54410,#54411,#54412,#54413,#54414,#54415,#54416,#54417,#54418,#54419,
#54420,#54421,#54422,#54423,#54424,#54425,#54426,#54427,#54428,#54429,#54430,
#54431,#54432,#54433,#54434,#54435,#54436,#54437,#54438,#54439,#54440,#54441,
#54442,#54443,#54444,#54445,#54446,#54447,#54448,#54449,#54450,#54451,#54452,
#54453,#54454,#54455,#54456,#54457,#54458,#54459,#54460,#54461,#54462,#54463,
#54464,#54465,#54466,#54467,#54468,#54469,#54470,#54471,#54472,#54473,#54474,
#54475,#54476,#54477,#54478,#54479,#54480,#54481,#54482,#54483,#54484,#54485,
#54486,#54487,#54488,#54489,#54490,#54491,#54492,#54493,#54494,#54495,#54496,
#54497,#54498,#54499,#54500,#54501,#54502,#54503,#54504,#54505,#54506,#54507,
#54508,#54509,#54510,#54511,#54512,#54513,#54514,#54515,#54516,#54517,#54518,
#54519,#54520,#54521,#54522,#54523,#54524,#54525,#54526,#54527,#54528,#54529,
#54530,#54531,#54532,#54533,#54534,#54535,#54536,#54537,#54538,#54539,#54540,
#54541,#54542,#54543,#54544,#54545,#54546,#54547,#54548,#54549,#54550,#54551,
#54552,#54553,#54554,#54555,#54556,#54557,#54558,#54559,#54560,#54561,#54562,
#54563,#54564,#54565,#54566,#54567,#54568,#54569,#54570,#54571,#54572,#54573,
#54574,#54575,#54576,#54577,#54578,#54579,#54580,#54581,#54582,#54583,#54584,
#54585,#54586,#54587,#54588,#54589,#54590,#54591,#54592,#54593,#54594,#54595,
#54596,#54597,#54598,#54599,#54600,#54601,#54602,#54603,#54604,#54605,#54606,
#54607,#54608,#54609,#54610,#54611,#54612,#54613,#54614,#54615,#54616,#54617,
#54618,#54619,#54620,#54621,#54622,#54623,#54624,#54625,#54626,#54627,#54628,
#54629,#54630,#54631,#54632,#54633,#54634,#54635,#54636,#54637,#54638,#54639,
#54640,#54641,#54642,#54643,#54644,#54645,#54646,#54647,#54648,#54649,#54650,
#54651,#54652,#54653,#54654,#54655,#54656,#54657,#54658,#54659,#54660,#54661,
#54662,#54663,#54664,#54665,#54666,#54667,#54668,#54669,#54670,#54671,#54672,
#54673,#54674,#54675,#54676,#54677,#54678,#54679,#54680,#54681,#54682,#54683,
#54684,#54685,#54686,#54687,#54688,#54689,#54690,#54691,#54692,#54693,#54694,
#54695,#54696,#54697,#54698,#54699,#54700,#54701,#54702,#54703,#54704,#54705,
#54706,#54707,#54708,#54709,#54710,#54711,#54712,#54713,#54714,#54715,#54716,
#54717,#54718,#54719,#54720,#54721,#54722,#54723,#54724,#54725,#54726,#54727,
#54728,#54729,#54730,#54731,#54732,#54733,#54734,#54735,#54736,#54737,#54738,
#54739,#54740,#54741,#54742,#54743,#54744,#54745,#54746,#54747,#54748,#54749,
#54750,#54751,#54752,#54753,#54754,#54755,#54756,#54757,#54758,#54759,#54760,
#54761,#54762,#54763,#54764,#54765,#54766,#54767,#54768,#54769,#54770,#54771,
#54772,#54773,#54774,#54775,#54776,#54777,#54778,#54779,#54780,#54781,#54782,
#54783,#54784,#54785,#54786,#54787,#54788,#54789,#54790,#54791,#54792,#54793,
#54794,#54795,#54796,#54797,#54798,#54799,#54800,#54801,#54802,#54803,#54804,
#54805,#54806,#54807,#54808,#54809,#54810,#54811,#54812,#54813,#54814,#54815,
#54816,#54817,#54818,#54819,#54820,#54821,#54822,#54823,#54824,#54825,#54826,
#54827,#54828,#54829,#54830,#54831,#54832,#54833,#54834,#54835,#54836,#54837,
#54838,#54839,#54840,#54841,#54842,#54843,#54844,#54845,#54846,#54847,#54848,
#54849,#54850,#54851,#54852,#54853,#54854,#54855,#54856,#54857,#54858,#54859,
#54860,#54861,#54862,#54863,#54864,#54865,#54866,#54867,#54868,#54869,#54870,
#54871,#54872,#54873,#54874,#54875,#54876,#54877,#54878,#54879,#54880,#54881,
#54882,#54883,#54884,#54885),.UNSPECIFIED.,.F.,.F.,(4,2,2,2,2,2,2,2,2,2,
2,2,2,2,2,2,2,2,2,2,2,2,2,2,2,2,2,2,2,2,2,2,2,2,2,2,2,2,2,2,2,2,2,2,2,2,
2,2,2,2,2,2,2,2,2,2,2,2,2,2,2,2,2,2,2,2,2,2,2,2,2,2,2,2,2,2,2,2,2,2,2,2,
2,2,2,2,2,2,2,2,2,2,2,2,2,2,2,2,2,2,2,2,2,2,2,2,2,2,2,2,2,2,2,2,2,2,2,2,
2,2,2,2,2,2,2,2,2,2,2,2,2,2,2,2,2,2,2,2,2,2,2,2,2,2,2,2,2,2,2,2,2,2,2,2,
2,2,2,2,2,2,2,2,2,2,2,2,2,2,2,2,2,2,2,2,2,2,2,2,2,2,2,2,2,2,2,2,2,2,2,2,
2,2,2,2,2,2,2,2,2,2,2,2,2,2,2,2,2,2,2,2,2,2,2,2,2,2,2,2,2,2,2,2,2,2,2,2,
2,2,2,2,2,2,2,2,2,2,2,2,2,2,2,2,2,2,2,2,2,2,2,2,2,2,2,2,2,2,2,2,2,2,2,2,
2,2,2,2,2,2,2,2,2,2,2,4),(-4.06165407026546,-4.05740964544468,-4.05400539194529,
-4.0524781749501,-4.05131240313444,-4.05018996086548,-4.04908094134211,
-4.04757269022949,-4.04384170581745,-4.03641892777598,-3.93042213168213,
-3.89574718704119,-3.8910137597619,-3.8897674188987,-3.88902761014295,-3.88836926114119,
-3.88752703060503,-3.88585720714289,-3.87582213268271,-3.83122313814856,
-3.74048883286755,-3.7345677413575,-3.73167229838484,-3.72994353557879,
-3.72838211363205,-3.72721009201704,-3.72609708027135,-3.72457364209001,
-3.72075506851831,-3.67032219040894,-3.64596709898665,-3.61423912190594,
-3.5707475787363,-3.56782671199944,-3.56678485733794,-3.56609050411309,
-3.56542190897701,-3.5646200326619,-3.56263957493068,-3.54510307177094,
-3.45795244305617,-3.43574125061026,-3.41856748049928,-3.41219603235631,
-3.40913971441172,-3.40734464549353,-3.4057353064316,-3.40455507238027,
-3.40345379493462,-3.40197628846588,-3.39834336951894,-3.36083303398119,
-3.31247646323611,-3.29498682328827,-3.28245725928372,-3.25006695443711,
-3.24550758849709,-3.24427759259807,-3.24354153904301,-3.24288261900017,
-3.24203435416075,-3.24027628828694,-3.22884797334992,-3.15362639018163,
-3.09436451820203,-3.08883821369963,-3.08608631631904,-3.08441725337565,
-3.08290043957803,-3.0817353317018,-3.08060999758779,-3.07903937121443,
-3.07583104166304,-3.04318356447465,-2.95611042419199,-2.92697263377816,
-2.92268133746237,-2.92147736524947,-2.92074709255175,-2.92008671462688,
-2.91924170664772,-2.91745415837025,-2.90536243771982,-2.86180633726569,
-2.77143704122718,-2.76597390706601,-2.76324511150198,-2.76158563103093,
-2.760073974608,-2.75890999180129,-2.75778190457202,-2.75620124707182,-2.75203853286507,
-2.68776167341046,-2.64153826193142,-2.61194310789301,-2.6006374655522,
-2.59902896213997,-2.59821090184312,-2.59755496782113,-2.59679964666062,
-2.59551663765062,-2.59085462247898,-2.49531730542908,-2.45808649774396,
-2.44128892995578,-2.43853959175595,-2.4370992031111,-2.43603726791407,
-2.43488807738552,-2.43322960073072,-2.42856383620457,-2.35588170651182,
-2.31312004970147,-2.28166606413652,-2.27870424789595,-2.27653862753007,
-2.27561483636152,-2.27494442880766,-2.27432524226566,-2.27347741592653,
-2.27135653055447,-2.24597186350575,-2.17011162254495,-2.13498825231204,
-2.11855901736462,-2.11582520576584,-2.11438797382565,-2.11332626634158,
-2.11217528142981,-2.11051070167082,-2.10580485953711,-2.03081534233176,
-1.9586365768906,-1.95447342316307,-1.95323022550838,-1.95256491691888,
-1.95190950885699,-1.95110429127795,-1.94955878461852,-1.93995470904831,
-1.92268570516832,-1.897393739233,-1.82333119120031,-1.81567369047869,-1.79648765894569,
-1.79339925264149,-1.7918887192281,-1.79070675953333,-1.78939838312632,
-1.78725407228404,-1.77971998292058,-1.75422595681069,-1.71141794876818,
-1.63586064375099,-1.6318113298592,-1.63058152952279,-1.62991892826898,
-1.62926389575223,-1.62845553470062,-1.62689124574334,-1.61677272106587,
-1.59269104607831,-1.50287722020347,-1.47419844964061,-1.4707937429151,
-1.46935741020303,-1.46815776711736,-1.46692515368837,-1.46512088902775,
-1.46032860967519,-1.43736654712427,-1.41546954831765,-1.34284595903923,
-1.31066838506157,-1.3084423072406,-1.30757679093033,-1.30695325059003,
-1.30629960515896,-1.30542173652212,-1.30444371401243,-1.30279013778082,
-1.2623735630243,-1.16611216232519,-1.15042218510316,-1.14780965890159,
-1.14625199498803,-1.14505956892014,-1.14378564067582,-1.14179588099459,
-1.1356451969395,-1.10110282100427,-1.00240765596283,-0.987193855677619,
-0.985284903838327,-0.984416220519701,-0.983764238604498,-0.98306030625779,
-0.981955612611417,-0.980656220700224,-0.978194157829027,-0.95547247504219,
-0.93057438950738,-0.854891794714637,-0.84601465565169,-0.828427824497416,
-0.825452646625093,-0.823942490072284,-0.822758393424724,-0.821445151191329,
-0.819287150008426,-0.811647526538121,-0.785956023021821,-0.769624505543458,
-0.757708102428476,-0.70259084313062,-0.665593756811462,-0.663247552340367,
-0.662362571197941,-0.661733354881777,-0.661085221888442,-0.660231446611528,
-0.659284516030755,-0.657700729057482,-0.654455287059512,-0.645839835409615,
-0.624811803750036,-0.532107702575697,-0.523762298751068,-0.520004480876801,
-0.504716195978818,-0.502138153598254,-0.500596564254775,-0.499413821016613,
-0.498147688628208,-0.496164835837219,-0.489994672960956,-0.455126923023744,
-0.42772766814659,-0.419675561577709,-0.412813942731298,-0.4068450200568,
-0.347371747571115,-0.340932524122567,-0.339622276546277,-0.338792525752766,
-0.338168700191169,-0.337448947843508,-0.336271270044064,-0.334864202572282,
-0.332113875489203,-0.325263611732087,-0.300209541027107,-0.219742396136675,
-0.212508367882264,-0.182322803766125,-0.17916319551422,-0.177600541216223,
-0.176473531952652,-0.175276043651974,-0.173688737720666,-0.170227417512946,
-0.103878048749372,-0.0311419473554923,-0.0269734683702882,-0.0182226738461123,
-0.0167539138764466,-0.0158784160279446,-0.0152185369868466,-0.0145871428898369,
-0.0138632201451378,-0.0128415480744668,-0.00908015386448269,-0.00096178856909809),
 .UNSPECIFIED.);
#849=B_SPLINE_CURVE_WITH_KNOTS('',3,(#54887,#54888,#54889,#54890,#54891,
#54892,#54893,#54894,#54895,#54896,#54897,#54898,#54899,#54900,#54901,#54902,
#54903,#54904,#54905),.UNSPECIFIED.,.F.,.F.,(4,3,3,3,3,3,4),(14.8194310462886,
14.9820505664306,15.1443726613452,15.306670802268,15.4689507744941,15.6315623856294,
15.7079632677806),.UNSPECIFIED.);
#850=B_SPLINE_CURVE_WITH_KNOTS('',3,(#54909,#54910,#54911,#54912,#54913,
#54914,#54915,#54916,#54917,#54918,#54919,#54920,#54921,#54922,#54923,#54924,
#54925,#54926,#54927,#54928,#54929,#54930,#54931,#54932,#54933,#54934,#54935,
#54936,#54937,#54938,#54939,#54940,#54941,#54942,#54943,#54944,#54945,#54946,
#54947,#54948,#54949,#54950,#54951,#54952,#54953,#54954,#54955,#54956,#54957,
#54958,#54959,#54960,#54961,#54962,#54963,#54964,#54965,#54966,#54967,#54968,
#54969,#54970,#54971,#54972,#54973,#54974,#54975,#54976,#54977,#54978,#54979,
#54980,#54981,#54982,#54983,#54984,#54985,#54986,#54987,#54988,#54989,#54990,
#54991,#54992,#54993,#54994,#54995,#54996,#54997,#54998,#54999,#55000,#55001,
#55002,#55003,#55004,#55005,#55006,#55007,#55008,#55009,#55010,#55011,#55012,
#55013,#55014,#55015,#55016,#55017),.UNSPECIFIED.,.F.,.F.,(4,3,3,3,3,3,
3,3,3,3,3,3,3,3,3,3,3,3,3,3,3,3,3,3,3,3,3,3,3,3,3,3,3,3,3,3,4),(16.0586828769936,
16.228071424883,16.3973387439612,16.5667947821335,16.7363202110308,16.906337659739,
17.0574752807613,17.2212840646477,17.3847419026725,17.5526233481367,17.7159497278199,
17.8861087061746,18.0562676845293,18.2219517445982,18.3873187559091,18.5542540890062,
18.7195349605951,18.8872975244462,19.0550600882973,19.2208116332235,19.3862551116776,
19.5531544567745,19.7185320739229,19.8861922829941,20.0538524920653,20.2191011613401,
20.3840291050623,20.5511830527551,20.7160253663893,20.8843351311113,21.0526448958333,
21.2166948429012,21.3804312878908,21.5441304586967,21.707790871614,21.8718046546966,
21.9911485749085),.UNSPECIFIED.);
#851=B_SPLINE_CURVE_WITH_KNOTS('',3,(#55019,#55020,#55021,#55022,#55023,
#55024,#55025,#55026,#55027,#55028,#55029,#55030,#55031,#55032,#55033,#55034,
#55035,#55036,#55037,#55038,#55039,#55040,#55041,#55042,#55043,#55044,#55045,
#55046,#55047,#55048,#55049,#55050,#55051,#55052,#55053,#55054,#55055,#55056,
#55057,#55058,#55059,#55060,#55061,#55062,#55063,#55064,#55065,#55066,#55067,
#55068,#55069,#55070,#55071,#55072,#55073,#55074,#55075,#55076,#55077,#55078,
#55079,#55080,#55081,#55082,#55083,#55084,#55085,#55086,#55087,#55088,#55089,
#55090,#55091,#55092,#55093,#55094,#55095,#55096,#55097,#55098,#55099,#55100,
#55101,#55102,#55103,#55104,#55105,#55106,#55107,#55108,#55109,#55110,#55111,
#55112,#55113,#55114,#55115,#55116,#55117,#55118,#55119,#55120,#55121,#55122,
#55123,#55124,#55125,#55126,#55127,#55128,#55129,#55130,#55131,#55132,#55133,
#55134,#55135,#55136,#55137,#55138,#55139,#55140,#55141,#55142,#55143,#55144,
#55145,#55146,#55147,#55148,#55149,#55150,#55151,#55152,#55153,#55154,#55155,
#55156,#55157,#55158,#55159,#55160,#55161,#55162,#55163,#55164,#55165,#55166,
#55167,#55168,#55169,#55170,#55171,#55172,#55173,#55174,#55175,#55176,#55177,
#55178,#55179,#55180,#55181,#55182,#55183,#55184,#55185,#55186,#55187,#55188,
#55189,#55190,#55191,#55192,#55193,#55194,#55195,#55196,#55197,#55198,#55199,
#55200,#55201,#55202,#55203,#55204,#55205,#55206,#55207,#55208,#55209,#55210,
#55211,#55212,#55213,#55214,#55215,#55216,#55217,#55218,#55219,#55220,#55221,
#55222,#55223,#55224,#55225,#55226,#55227,#55228,#55229,#55230,#55231,#55232,
#55233,#55234,#55235,#55236,#55237,#55238,#55239,#55240,#55241,#55242,#55243,
#55244,#55245,#55246,#55247,#55248,#55249,#55250,#55251,#55252,#55253,#55254,
#55255,#55256,#55257,#55258,#55259,#55260,#55261,#55262,#55263,#55264,#55265,
#55266,#55267,#55268,#55269,#55270,#55271,#55272,#55273,#55274,#55275,#55276,
#55277,#55278,#55279,#55280,#55281,#55282,#55283,#55284,#55285,#55286,#55287,
#55288,#55289,#55290,#55291,#55292,#55293,#55294,#55295,#55296,#55297,#55298,
#55299,#55300,#55301,#55302,#55303,#55304,#55305,#55306,#55307,#55308,#55309,
#55310,#55311,#55312,#55313,#55314,#55315,#55316,#55317,#55318,#55319,#55320,
#55321,#55322,#55323,#55324,#55325,#55326,#55327,#55328,#55329,#55330,#55331,
#55332,#55333,#55334,#55335,#55336,#55337,#55338,#55339,#55340,#55341,#55342,
#55343,#55344,#55345,#55346,#55347,#55348,#55349,#55350,#55351,#55352,#55353,
#55354,#55355,#55356,#55357,#55358,#55359,#55360,#55361,#55362,#55363,#55364,
#55365,#55366,#55367,#55368,#55369,#55370,#55371,#55372,#55373,#55374,#55375,
#55376,#55377,#55378,#55379,#55380,#55381,#55382,#55383,#55384,#55385,#55386,
#55387,#55388,#55389,#55390,#55391,#55392,#55393,#55394,#55395,#55396,#55397,
#55398,#55399,#55400,#55401,#55402,#55403,#55404,#55405,#55406,#55407,#55408,
#55409,#55410,#55411,#55412,#55413,#55414,#55415,#55416,#55417,#55418,#55419,
#55420,#55421,#55422,#55423,#55424,#55425,#55426,#55427,#55428,#55429,#55430,
#55431,#55432,#55433,#55434,#55435,#55436,#55437,#55438,#55439,#55440,#55441,
#55442,#55443,#55444,#55445,#55446,#55447,#55448,#55449,#55450,#55451,#55452,
#55453,#55454,#55455,#55456,#55457,#55458,#55459,#55460,#55461,#55462,#55463,
#55464,#55465,#55466,#55467,#55468,#55469,#55470,#55471,#55472,#55473,#55474,
#55475,#55476,#55477,#55478,#55479,#55480,#55481,#55482,#55483,#55484,#55485,
#55486,#55487,#55488,#55489,#55490,#55491,#55492,#55493,#55494,#55495,#55496,
#55497,#55498,#55499,#55500,#55501,#55502,#55503,#55504,#55505,#55506,#55507,
#55508,#55509,#55510,#55511,#55512,#55513,#55514,#55515,#55516,#55517,#55518,
#55519,#55520,#55521,#55522,#55523,#55524,#55525,#55526,#55527,#55528,#55529,
#55530,#55531,#55532,#55533,#55534,#55535,#55536,#55537,#55538,#55539,#55540,
#55541,#55542,#55543,#55544,#55545,#55546,#55547,#55548,#55549,#55550,#55551,
#55552,#55553,#55554,#55555,#55556,#55557,#55558),.UNSPECIFIED.,.F.,.F.,
(4,2,2,2,2,2,2,2,2,2,2,2,2,2,2,2,2,2,2,2,2,2,2,2,2,2,2,2,2,2,2,2,2,2,2,
2,2,2,2,2,2,2,2,2,2,2,2,2,2,2,2,2,2,2,2,2,2,2,2,2,2,2,2,2,2,2,2,2,2,2,2,
2,2,2,2,2,2,2,2,2,2,2,2,2,2,2,2,2,2,2,2,2,2,2,2,2,2,2,2,2,2,2,2,2,2,2,2,
2,2,2,2,2,2,2,2,2,2,2,2,2,2,2,2,2,2,2,2,2,2,2,2,2,2,2,2,2,2,2,2,2,2,2,2,
2,2,2,2,2,2,2,2,2,2,2,2,2,2,2,2,2,2,2,2,2,2,2,2,2,2,2,2,2,2,2,2,2,2,2,2,
2,2,2,2,2,2,2,2,2,2,2,2,2,2,2,2,2,2,2,2,2,2,2,2,2,2,2,2,2,2,2,2,2,2,2,2,
2,2,2,2,2,2,2,2,2,2,2,2,2,2,2,2,2,2,2,2,2,2,2,2,2,2,2,2,2,2,2,2,2,2,2,2,
2,2,2,2,2,2,2,2,2,2,2,2,2,2,2,2,2,2,4),(-4.06062904163106,-4.04570360185412,
-4.04390479883215,-4.04286596618711,-4.04214226005793,-4.04152432695382,
-4.04089273972695,-4.04005118959283,-4.03833265676747,-4.02779688455913,
-4.02475212675819,-4.02057511193562,-3.95556552189716,-3.88599997279386,
-3.88254007503904,-3.8809567331219,-3.87976361458958,-3.87864172965352,
-3.87708779235204,-3.87395082788115,-3.84427456933291,-3.75729595410533,
-3.7315861969366,-3.72465186402193,-3.72187832226222,-3.72046333458138,
-3.71928077316759,-3.71856063837893,-3.71793479508989,-3.71710300984889,
-3.71579295430406,-3.70942190820894,-3.65247735656485,-3.64690576232457,
-3.64055415360531,-3.63318376102258,-3.62441538901417,-3.56502277266714,
-3.56022663834124,-3.55842182838225,-3.55718912501054,-3.55598961204051,
-3.554553692942,-3.55101658888885,-3.51930538088721,-3.47245882505677,-3.4261708206132,
-3.40730001512376,-3.40146679170015,-3.39902481377663,-3.39773501909049,
-3.39663793520301,-3.39593819392463,-3.39528770808305,-3.3944194258323,
-3.39250864501398,-3.37718292236751,-3.37582408706139,-3.29182806322054,
-3.24561168171937,-3.23826438270998,-3.23613951464844,-3.23483558510705,
-3.23365277735547,-3.23213439102603,-3.22900600880857,-3.20895314382336,
-3.20716332962316,-3.19428533140588,-3.11143431645357,-3.07989420077164,
-3.07692720542661,-3.07544061644637,-3.07453137827011,-3.07369302826554,
-3.07304702212045,-3.07240341640841,-3.0712677872062,-3.06794972666932,
-3.00879557124416,-2.9595658190066,-2.94192509180402,-2.91978835700861,
-2.91509817342019,-2.91330825880092,-2.91207777738029,-2.91087423098795,
-2.90942602564079,-2.90581984517675,-2.87158578710844,-2.78886111437125,
-2.75731205006472,-2.75434511715292,-2.7528587850803,-2.75194982978359,
-2.7511215338754,-2.75047514605092,-2.74983394496181,-2.74870988564432,
-2.74547330168384,-2.74500917989446,-2.68523401249009,-2.62649219500212,
-2.60084220835202,-2.59582627073307,-2.59208950713824,-2.59045691086623,
-2.58925694799464,-2.58815011363426,-2.58665011398216,-2.58372132561593,
-2.56070879580912,-2.54378188828005,-2.46926518708424,-2.44270686700676,
-2.4309344045196,-2.4293106959667,-2.428489544122,-2.42783933694991,-2.42718503162967,
-2.42599624872686,-2.42228006951242,-2.35734309009427,-2.32399520619353,
-2.28823251548006,-2.27170092880894,-2.26896224602825,-2.26752379568303,
-2.26646175367632,-2.26531095550206,-2.26364759133703,-2.25895135088672,
-2.18005319719431,-2.14259879251171,-2.10911490296156,-2.10697795909713,
-2.10605896326605,-2.10538921852708,-2.1047686137569,-2.1039157581023,-2.10176636888289,
-2.07481669973366,-2.03147697517407,-1.95250504854578,-1.94748580179032,
-1.94558551879651,-1.94445689301101,-1.94326935306538,-1.94171471229048,
-1.93839974162612,-1.89408825722172,-1.8435538926705,-1.78790421228387,
-1.78478477137643,-1.78367727278607,-1.78303931149941,-1.78244478899956,
-1.78161853530436,-1.77997025631581,-1.76739898769783,-1.74145618156212,
-1.67666002857445,-1.62821277920486,-1.62441926195705,-1.62290017041284,
-1.62178832510878,-1.62059158807168,-1.61897862350564,-1.61535168392906,
-1.57144159253841,-1.52087302829296,-1.46529490340021,-1.46220047248265,
-1.46109613483065,-1.46045879909683,-1.45986405594485,-1.45903626859684,
-1.45738055002091,-1.44455270247651,-1.41879700397575,-1.35883124267773,
-1.33488767436293,-1.30509399970225,-1.30195686754842,-1.30040384322776,
-1.29928308383072,-1.29811544908455,-1.29658055736026,-1.29488897303617,
-1.29208312021498,-1.23321401263478,-1.144302083178,-1.139868940756,-1.13859507713029,
-1.13784908546256,-1.13725751111051,-1.13645715746509,-1.13493389098948,
-1.12583770330936,-1.10668350589057,-1.0591714618927,-0.983887328247649,
-0.979411951856088,-0.977781807930227,-0.976640134521728,-0.975480974398116,
-0.97400765260036,-0.972399107054665,-0.969792376505275,-0.964659618590341,
-0.913416879026794,-0.828860645516561,-0.817919742226803,-0.816183877249544,
-0.815339837149445,-0.814681209609328,-0.81394229093811,-0.81270022400218,
-0.808014637431663,-0.773995699930228,-0.76176438252304,-0.708625793981986,
-0.660219245749986,-0.656424784839306,-0.654905277707063,-0.653793114794276,
-0.652620097273498,-0.651053692004251,-0.649318491389566,-0.646407763989167,
-0.640444556270726,-0.549713700438118,-0.505124847630551,-0.495108088602803,
-0.493438933812155,-0.492596731044865,-0.491938248640452,-0.491198113737797,
-0.489950832949214,-0.485209321070121,-0.450436217023383,-0.426532372750122,
-0.396421226157924,-0.337606682590258,-0.333715753423511,-0.332179690624836,
-0.331063142951378,-0.329892638562272,-0.328341719684826,-0.326627954801142,
-0.323769123622164,-0.317949950797744,-0.227034516771874,-0.182383601828387,
-0.172337998166678,-0.170667239338103,-0.169824637255569,-0.169166045185823,
-0.168426004895614,-0.16717938028982,-0.162446072367399,-0.127788719663138,
-0.0178688328568037,-0.0115443800013135,-0.00945485230489118,-0.00828833477619918,
-0.00712531855638712,-0.00599379196373133,-0.00457291864233748,-0.000957836357716254),
 .UNSPECIFIED.);
#852=B_SPLINE_CURVE_WITH_KNOTS('',3,(#55560,#55561,#55562,#55563,#55564,
#55565,#55566,#55567,#55568,#55569,#55570,#55571,#55572,#55573,#55574,#55575,
#55576,#55577,#55578,#55579,#55580,#55581,#55582,#55583,#55584,#55585,#55586,
#55587,#55588,#55589,#55590,#55591,#55592,#55593,#55594,#55595,#55596,#55597,
#55598,#55599,#55600,#55601,#55602,#55603,#55604,#55605,#55606,#55607,#55608,
#55609,#55610,#55611,#55612,#55613,#55614,#55615,#55616,#55617,#55618,#55619,
#55620,#55621,#55622,#55623,#55624,#55625,#55626,#55627,#55628,#55629,#55630,
#55631,#55632,#55633,#55634,#55635,#55636,#55637,#55638,#55639,#55640,#55641,
#55642,#55643,#55644,#55645,#55646,#55647,#55648,#55649,#55650,#55651,#55652,
#55653,#55654,#55655,#55656,#55657,#55658,#55659,#55660,#55661,#55662,#55663,
#55664,#55665,#55666,#55667,#55668,#55669,#55670,#55671,#55672,#55673,#55674,
#55675,#55676,#55677,#55678,#55679,#55680,#55681,#55682,#55683,#55684,#55685,
#55686,#55687,#55688,#55689,#55690,#55691,#55692,#55693,#55694,#55695,#55696,
#55697,#55698,#55699,#55700,#55701,#55702,#55703,#55704,#55705,#55706,#55707,
#55708,#55709,#55710,#55711,#55712,#55713,#55714,#55715,#55716,#55717,#55718,
#55719,#55720,#55721,#55722,#55723,#55724,#55725,#55726,#55727,#55728,#55729,
#55730,#55731,#55732,#55733,#55734,#55735,#55736,#55737,#55738,#55739,#55740,
#55741,#55742,#55743,#55744,#55745,#55746,#55747,#55748,#55749,#55750,#55751,
#55752,#55753,#55754,#55755,#55756,#55757,#55758,#55759,#55760,#55761,#55762,
#55763,#55764,#55765,#55766,#55767,#55768,#55769,#55770,#55771,#55772,#55773,
#55774,#55775,#55776,#55777,#55778,#55779,#55780,#55781,#55782,#55783,#55784,
#55785,#55786,#55787,#55788,#55789,#55790,#55791,#55792,#55793,#55794,#55795,
#55796,#55797,#55798,#55799,#55800,#55801,#55802,#55803,#55804,#55805,#55806,
#55807,#55808,#55809,#55810,#55811,#55812,#55813,#55814,#55815,#55816,#55817,
#55818,#55819,#55820,#55821,#55822,#55823,#55824,#55825,#55826,#55827,#55828,
#55829,#55830,#55831,#55832,#55833,#55834,#55835,#55836,#55837,#55838,#55839,
#55840,#55841,#55842,#55843,#55844,#55845,#55846,#55847,#55848,#55849,#55850,
#55851,#55852,#55853,#55854,#55855,#55856,#55857,#55858,#55859,#55860,#55861,
#55862,#55863,#55864,#55865,#55866,#55867,#55868,#55869,#55870,#55871,#55872,
#55873,#55874,#55875,#55876,#55877,#55878,#55879,#55880,#55881,#55882,#55883,
#55884,#55885,#55886,#55887,#55888,#55889,#55890,#55891,#55892,#55893,#55894,
#55895,#55896,#55897,#55898,#55899,#55900,#55901,#55902,#55903,#55904,#55905,
#55906,#55907,#55908,#55909,#55910,#55911,#55912,#55913,#55914,#55915,#55916,
#55917,#55918,#55919,#55920,#55921,#55922,#55923,#55924,#55925,#55926,#55927,
#55928,#55929,#55930,#55931,#55932,#55933,#55934,#55935,#55936,#55937,#55938,
#55939,#55940,#55941,#55942,#55943,#55944,#55945,#55946,#55947,#55948,#55949,
#55950,#55951,#55952,#55953,#55954,#55955,#55956,#55957,#55958,#55959,#55960,
#55961,#55962,#55963,#55964,#55965,#55966,#55967,#55968,#55969,#55970,#55971,
#55972,#55973,#55974,#55975,#55976,#55977,#55978,#55979,#55980,#55981,#55982,
#55983,#55984,#55985,#55986,#55987,#55988,#55989,#55990,#55991,#55992,#55993,
#55994,#55995,#55996,#55997,#55998,#55999,#56000,#56001,#56002,#56003,#56004,
#56005,#56006,#56007,#56008,#56009,#56010,#56011,#56012,#56013,#56014,#56015,
#56016,#56017,#56018,#56019,#56020,#56021,#56022,#56023,#56024,#56025,#56026,
#56027,#56028,#56029,#56030,#56031,#56032,#56033,#56034,#56035,#56036,#56037,
#56038,#56039,#56040,#56041,#56042,#56043,#56044,#56045,#56046,#56047,#56048,
#56049,#56050,#56051,#56052,#56053,#56054,#56055,#56056,#56057,#56058,#56059,
#56060,#56061,#56062,#56063,#56064,#56065,#56066,#56067,#56068,#56069,#56070,
#56071,#56072,#56073,#56074,#56075,#56076,#56077,#56078,#56079,#56080,#56081,
#56082,#56083,#56084,#56085,#56086,#56087,#56088,#56089,#56090,#56091,#56092,
#56093),.UNSPECIFIED.,.F.,.F.,(4,2,2,2,2,2,2,2,2,2,2,2,2,2,2,2,2,2,2,2,
2,2,2,2,2,2,2,2,2,2,2,2,2,2,2,2,2,2,2,2,2,2,2,2,2,2,2,2,2,2,2,2,2,2,2,2,
2,2,2,2,2,2,2,2,2,2,2,2,2,2,2,2,2,2,2,2,2,2,2,2,2,2,2,2,2,2,2,2,2,2,2,2,
2,2,2,2,2,2,2,2,2,2,2,2,2,2,2,2,2,2,2,2,2,2,2,2,2,2,2,2,2,2,2,2,2,2,2,2,
2,2,2,2,2,2,2,2,2,2,2,2,2,2,2,2,2,2,2,2,2,2,2,2,2,2,2,2,2,2,2,2,2,2,2,2,
2,2,2,2,2,2,2,2,2,2,2,2,2,2,2,2,2,2,2,2,2,2,2,2,2,2,2,2,2,2,2,2,2,2,2,2,
2,2,2,2,2,2,2,2,2,2,2,2,2,2,2,2,2,2,2,2,2,2,2,2,2,2,2,2,2,2,2,2,2,2,2,2,
2,2,2,2,2,2,2,2,2,2,2,2,2,2,2,2,2,2,2,2,2,2,2,2,2,2,2,2,2,2,4),(-4.06064425517163,
-4.05296410003843,-3.94672613835459,-3.91290974138407,-3.90982817367382,
-3.90759311330821,-3.90665714968852,-3.90598433074735,-3.90536761780485,
-3.90452991114187,-3.90288823337092,-3.88994164328037,-3.88923479658141,
-3.8888496971427,-3.81580461233557,-3.75180985328595,-3.74895640602316,
-3.74724504606555,-3.74569574611307,-3.74452575290477,-3.74340916632325,
-3.7418720093438,-3.73797272524807,-3.67711571784792,-3.61318095284064,
-3.58922058650699,-3.58539996295065,-3.58424570667373,-3.58352653706374,
-3.58286281456234,-3.58199518353242,-3.58008831861781,-3.56488463684256,
-3.56133858435174,-3.46549597030189,-3.4295816746418,-3.42650248000174,
-3.42469799407264,-3.42308168298624,-3.42189979392784,-3.42079983151505,
-3.41932776334154,-3.4158021287258,-3.3818918259257,-3.31795507364913,-3.302363586632,
-3.27693668371665,-3.26363201118395,-3.26196312442044,-3.26113268239232,
-3.26053759258747,-3.25990138556735,-3.25880265704849,-3.25574640415757,
-3.20032557994589,-3.1497432485707,-3.10659725780123,-3.1037152656533,-3.10199210514405,
-3.10043441316532,-3.09934223519345,-3.09824147695676,-3.09676621172103,
-3.09322276854617,-3.05858274861475,-2.97902836439941,-2.9449760657488,
-2.94188310706846,-2.93964150988172,-2.93870445394111,-2.93803145074841,
-2.93741500549012,-2.93657828822805,-2.9349404059872,-2.92209901734225,
-2.92131518620934,-2.92071440131782,-2.83936312339982,-2.78840430260704,
-2.78328690807435,-2.78068596175113,-2.77907991030517,-2.77760688181741,
-2.7764485949315,-2.77530620846294,-2.77367308634269,-2.76917727782508,
-2.69336270630096,-2.64615398749984,-2.62706490027276,-2.6181052545071,
-2.61658828552802,-2.61578934036829,-2.61514055230356,-2.61447343446265,
-2.61322114832562,-2.60897888032015,-2.53444309444672,-2.49124612813746,
-2.46558517549526,-2.460565659559,-2.45682660954906,-2.45519341085603,-2.45399315818889,
-2.45288616410474,-2.45138611160395,-2.44845770158678,-2.42546649641701,
-2.35658341025406,-2.32163066022849,-2.30654519623683,-2.2956295550279,
-2.29403439703826,-2.29321905585137,-2.29256322549915,-2.29190407891758,
-2.29069134203691,-2.28678328140576,-2.18352486079379,-2.14197088536682,
-2.13507991615464,-2.13300448494649,-2.13171183708642,-2.13052648596604,
-2.1290122267874,-2.12582022176927,-2.10431017386536,-2.03045972163131,
-1.9965528404156,-1.97369492010131,-1.97162356687346,-1.9707842467643,-1.97016718679459,
-1.9694948547294,-1.9685610832051,-1.96633833059885,-1.96327811573176,-1.9298978486507,
-1.84283708775814,-1.81475224998551,-1.81131923743569,-1.80975932830531,
-1.80856695515276,-1.80729480237645,-1.80531136292772,-1.79920759370235,
-1.76508705677307,-1.66838573118981,-1.65077879345792,-1.64879631290665,
-1.64799408576513,-1.64732538816017,-1.64663114419488,-1.64558981965511,
-1.64267277887198,-1.58001750174665,-1.50962490411154,-1.50857569369179,
-1.49134761577209,-1.48839605337645,-1.48689310294381,-1.48571232492881,
-1.48440036336656,-1.4822389698576,-1.47453169167166,-1.44869599340569,
-1.4051494839862,-1.33864283932188,-1.32777635012069,-1.32604402214284,
-1.32520080279432,-1.32454239999897,-1.32381820112596,-1.32261722005126,
-1.32117610379163,-1.31833241182128,-1.2890854999383,-1.20185222291373,
-1.19580780068877,-1.18818435108172,-1.16887652984217,-1.16578306136782,
-1.1642718143428,-1.16309010111076,-1.16178282079033,-1.15964217715774,
-1.15213950678408,-1.10422872324986,-1.01769456895971,-1.00518409047303,
-1.00355824665588,-1.00272461344346,-1.00210894143622,-1.00144920850849,
-1.00053666576166,-0.999510640934306,-0.997739686801674,-0.993971735812353,
-0.930979557123285,-0.849183363239738,-0.844039575339781,-0.842119746146725,
-0.840987269418947,-0.839919915458461,-0.838439551967217,-0.835499190509757,
-0.813289963621546,-0.794480429412944,-0.698841334603281,-0.696248501497367,
-0.695790285575151,-0.69400985109842,-0.682349134146024,-0.680580318391485,
-0.67972979910098,-0.679070459812087,-0.67835017053872,-0.677168291943857,
-0.675754030672242,-0.67298299125,-0.666058629994212,-0.640456317861474,
-0.553893475679808,-0.523975492498826,-0.520834931563955,-0.519281001841084,
-0.518159958519205,-0.516968510203523,-0.515388703432245,-0.511941772297602,
-0.445576812260463,-0.438678104798247,-0.432780132679777,-0.383078962686884,
-0.360182081410214,-0.358109641621491,-0.357270043848103,-0.356652838783945,
-0.356029613478544,-0.355146197413434,-0.353194309542699,-0.350568145909762,
-0.344131841931772,-0.323424997182118,-0.305118591753579,-0.235147781033413,
-0.224359710638494,-0.218294647550135,-0.200626646264396,-0.19765187304851,
-0.196143849355795,-0.19496236885282,-0.1936530005663,-0.191503594643511,
-0.183916981307173,-0.158316629533491,-0.0683540926283739,-0.0637523387064982,
-0.0375946310101134,-0.035458969575932,-0.0346083804467672,-0.0339882948652247,
-0.0333631832269334,-0.0327082914623046,-0.0318421738770758,-0.0304587988341439,
-0.000956382887790925),.UNSPECIFIED.);
#853=B_SPLINE_CURVE_WITH_KNOTS('',3,(#56095,#56096,#56097,#56098,#56099,
#56100,#56101,#56102,#56103,#56104,#56105,#56106,#56107,#56108,#56109,#56110,
#56111,#56112,#56113,#56114,#56115,#56116,#56117,#56118,#56119,#56120,#56121,
#56122,#56123,#56124,#56125,#56126,#56127,#56128,#56129,#56130,#56131,#56132,
#56133,#56134,#56135,#56136,#56137,#56138,#56139,#56140,#56141,#56142,#56143,
#56144,#56145,#56146,#56147,#56148,#56149,#56150,#56151,#56152,#56153,#56154,
#56155,#56156,#56157,#56158,#56159,#56160,#56161,#56162,#56163,#56164,#56165,
#56166,#56167,#56168,#56169,#56170,#56171,#56172,#56173,#56174,#56175,#56176,
#56177,#56178,#56179,#56180,#56181,#56182,#56183,#56184,#56185,#56186,#56187,
#56188,#56189,#56190,#56191,#56192,#56193,#56194,#56195,#56196,#56197,#56198,
#56199,#56200,#56201,#56202,#56203,#56204,#56205,#56206,#56207,#56208,#56209,
#56210,#56211,#56212,#56213,#56214,#56215,#56216,#56217,#56218,#56219,#56220,
#56221,#56222,#56223,#56224,#56225,#56226,#56227,#56228,#56229,#56230,#56231,
#56232,#56233,#56234,#56235,#56236,#56237,#56238,#56239,#56240,#56241,#56242,
#56243,#56244,#56245,#56246,#56247,#56248,#56249,#56250,#56251,#56252,#56253,
#56254,#56255,#56256,#56257,#56258,#56259,#56260,#56261,#56262,#56263,#56264,
#56265,#56266,#56267,#56268,#56269,#56270,#56271,#56272,#56273,#56274,#56275,
#56276,#56277,#56278,#56279,#56280,#56281,#56282,#56283,#56284,#56285,#56286,
#56287,#56288,#56289,#56290,#56291,#56292,#56293,#56294,#56295,#56296,#56297,
#56298,#56299,#56300,#56301,#56302,#56303,#56304,#56305,#56306,#56307,#56308,
#56309,#56310,#56311,#56312,#56313,#56314,#56315,#56316,#56317,#56318,#56319,
#56320,#56321,#56322,#56323,#56324,#56325,#56326,#56327,#56328,#56329,#56330,
#56331,#56332,#56333,#56334,#56335,#56336,#56337,#56338,#56339,#56340,#56341,
#56342,#56343,#56344,#56345,#56346,#56347,#56348,#56349,#56350,#56351,#56352,
#56353,#56354,#56355,#56356,#56357,#56358,#56359,#56360,#56361,#56362,#56363,
#56364,#56365,#56366,#56367,#56368,#56369,#56370,#56371,#56372,#56373,#56374,
#56375,#56376,#56377,#56378,#56379,#56380,#56381,#56382,#56383,#56384,#56385,
#56386,#56387,#56388,#56389,#56390,#56391,#56392,#56393,#56394,#56395,#56396,
#56397,#56398,#56399,#56400,#56401,#56402,#56403,#56404,#56405,#56406,#56407,
#56408,#56409,#56410,#56411,#56412,#56413,#56414,#56415,#56416,#56417,#56418,
#56419,#56420,#56421,#56422,#56423,#56424,#56425,#56426,#56427,#56428,#56429,
#56430,#56431,#56432,#56433,#56434,#56435,#56436,#56437,#56438,#56439,#56440,
#56441,#56442,#56443,#56444,#56445,#56446,#56447,#56448,#56449,#56450,#56451,
#56452,#56453,#56454,#56455,#56456,#56457,#56458,#56459,#56460,#56461,#56462,
#56463,#56464,#56465,#56466,#56467,#56468,#56469,#56470,#56471,#56472,#56473,
#56474,#56475,#56476,#56477,#56478,#56479,#56480,#56481,#56482,#56483,#56484,
#56485,#56486,#56487,#56488,#56489,#56490,#56491,#56492,#56493,#56494,#56495,
#56496,#56497,#56498,#56499,#56500,#56501,#56502,#56503,#56504,#56505,#56506,
#56507,#56508,#56509,#56510,#56511,#56512,#56513,#56514,#56515,#56516,#56517,
#56518,#56519,#56520,#56521,#56522,#56523,#56524,#56525,#56526,#56527,#56528,
#56529,#56530,#56531,#56532,#56533,#56534,#56535,#56536,#56537,#56538,#56539,
#56540,#56541,#56542,#56543,#56544,#56545,#56546,#56547,#56548,#56549,#56550,
#56551,#56552,#56553,#56554,#56555,#56556,#56557,#56558,#56559,#56560,#56561,
#56562,#56563,#56564,#56565,#56566,#56567,#56568,#56569,#56570,#56571,#56572,
#56573,#56574,#56575,#56576,#56577,#56578,#56579,#56580,#56581,#56582,#56583,
#56584,#56585,#56586,#56587,#56588,#56589,#56590,#56591,#56592,#56593,#56594,
#56595,#56596,#56597,#56598,#56599,#56600,#56601,#56602,#56603,#56604,#56605,
#56606,#56607,#56608,#56609,#56610,#56611,#56612,#56613,#56614,#56615,#56616,
#56617,#56618,#56619,#56620,#56621,#56622,#56623,#56624,#56625,#56626,#56627,
#56628),.UNSPECIFIED.,.F.,.F.,(4,2,2,2,2,2,2,2,2,2,2,2,2,2,2,2,2,2,2,2,
2,2,2,2,2,2,2,2,2,2,2,2,2,2,2,2,2,2,2,2,2,2,2,2,2,2,2,2,2,2,2,2,2,2,2,2,
2,2,2,2,2,2,2,2,2,2,2,2,2,2,2,2,2,2,2,2,2,2,2,2,2,2,2,2,2,2,2,2,2,2,2,2,
2,2,2,2,2,2,2,2,2,2,2,2,2,2,2,2,2,2,2,2,2,2,2,2,2,2,2,2,2,2,2,2,2,2,2,2,
2,2,2,2,2,2,2,2,2,2,2,2,2,2,2,2,2,2,2,2,2,2,2,2,2,2,2,2,2,2,2,2,2,2,2,2,
2,2,2,2,2,2,2,2,2,2,2,2,2,2,2,2,2,2,2,2,2,2,2,2,2,2,2,2,2,2,2,2,2,2,2,2,
2,2,2,2,2,2,2,2,2,2,2,2,2,2,2,2,2,2,2,2,2,2,2,2,2,2,2,2,2,2,2,2,2,2,2,2,
2,2,2,2,2,2,2,2,2,2,2,2,2,2,2,2,2,2,2,2,2,2,2,2,2,2,2,2,2,2,4),(-4.06120447951431,
-4.01260665686555,-3.93887131362229,-3.93540604210493,-3.93382296588376,
-3.93263117358277,-3.93151136039023,-3.92996160091044,-3.92683714135233,
-3.89750678502528,-3.81787782242457,-3.80243128736636,-3.78338932151216,
-3.77422208004284,-3.77270043372142,-3.77204684702149,-3.77142105707436,
-3.77079986614458,-3.76994466312798,-3.76823396344177,-3.75323657077867,
-3.75227926538786,-3.74668664122066,-3.70696599683707,-3.67376842843106,
-3.62199772577786,-3.61415562910771,-3.61198087711131,-3.6106659202612,
-3.60948572874616,-3.60798800366273,-3.60506073607164,-3.58829361111022,
-3.5824149941432,-3.51058703376588,-3.47819074083318,-3.46299987916976,
-3.45553954999855,-3.45261299812562,-3.45114140243028,-3.44991917302459,
-3.44919039258122,-3.44853281544024,-3.44769729173634,-3.44600338661094,
-3.43590700968378,-3.36412796441999,-3.29364695386967,-3.2901886820578,
-3.28860686756102,-3.28741522477499,-3.28629496536932,-3.28443776215458,
-3.2796859589146,-3.20060132336445,-3.15075079035032,-3.13607631970201,
-3.13128797754732,-3.12917558798084,-3.12753701072295,-3.12675653454788,
-3.12610832434285,-3.12547223796761,-3.12437420245592,-3.12132283834259,
-3.06713031505546,-3.06240608985419,-3.01437324688398,-2.97080273742987,
-2.96749480807397,-2.96594148108525,-2.96475408993239,-2.96362496256596,
-2.96204057941722,-2.95877695904907,-2.92373859070982,-2.84177486273639,
-2.81029361137534,-2.80732995225721,-2.80584472516268,-2.80493616102164,
-2.80410774773889,-2.80346128976041,-2.8028196407536,-2.80169395057468,
-2.79812208241094,-2.74074619701058,-2.69098903370517,-2.67110805544016,
-2.64764931588654,-2.64467358885685,-2.64318591269066,-2.64211741402926,
-2.640987539141,-2.6394006268126,-2.63612701265303,-2.60064322121399,-2.51909405544329,
-2.48764379548256,-2.48315909396866,-2.48193598520474,-2.48120133747992,
-2.48054187057482,-2.47969043388984,-2.47791702511518,-2.46615349489035,
-2.38205408096663,-2.33125874606431,-2.32349896453561,-2.32133213217007,
-2.32001882616276,-2.31883809833027,-2.31733693608956,-2.31439430635057,
-2.29733950700057,-2.29363051800344,-2.27529568818749,-2.19943762137914,
-2.172724448719,-2.16113677390182,-2.15951860234089,-2.15869842186024,-2.15804213204117,
-2.15728786505847,-2.15601017984342,-2.15140212121821,-2.05541532624224,
-2.03139406804066,-2.0028918646598,-1.99944517987408,-1.99788250010006,
-1.99668942894802,-1.99541790584765,-1.99343827550916,-1.98736788184511,
-1.89430345183146,-1.85084311801432,-1.8385861340834,-1.83696953526359,
-1.83613822857712,-1.83552309026127,-1.83484872564573,-1.83390484445389,
-1.83162342259734,-1.82846128305234,-1.79295204685174,-1.69815887357967,
-1.69580455480164,-1.67928829809879,-1.676633090897,-1.67506306522859,-1.67386876695179,
-1.67260015218366,-1.6706336640036,-1.66466853844555,-1.63180185792013,
-1.54003786222529,-1.536745482764,-1.53220038220944,-1.53173192821666,-1.53134270883874,
-1.52839018459887,-1.51579191155756,-1.51416286966213,-1.51332834613226,
-1.51271238266444,-1.5120387287282,-1.51109869415273,-1.50884016515445,
-1.50571800939087,-1.47106684709087,-1.40868175071105,-1.3860678051899,
-1.3573639958444,-1.35391074054749,-1.35234671730259,-1.35115329390594,
-1.34990792850022,-1.34799704106151,-1.34577492326821,-1.34165223899833,
-1.30655363753438,-1.23650156783843,-1.19440426308996,-1.19175888947053,
-1.19082803736432,-1.19018618886753,-1.18959257696181,-1.1887744737123,
-1.18716659005905,-1.17589180189729,-1.14645093040212,-1.05382101032975,
-1.03408129129811,-1.03096714434445,-1.02945156299714,-1.02826908018954,
-1.02716723730698,-1.02527107053875,-1.01981028025,-0.977114693117432,-0.926062068477467,
-0.882444024580411,-0.87038321409291,-0.868596883765736,-0.86775206170295,
-0.86709164283985,-0.866361096031581,-0.865156253922068,-0.86085758448151,
-0.831641875039946,-0.751344132820681,-0.750926753098481,-0.746984466294774,
-0.712196411366071,-0.708623433978229,-0.70715620423306,-0.706057308189376,
-0.704849946483502,-0.703211604329819,-0.699417452192986,-0.694260697959506,
-0.6813601458361,-0.661529662386007,-0.622040845859146,-0.589860823682174,
-0.548610061946015,-0.546293173491164,-0.545412391612473,-0.544784350831595,
-0.544119213380871,-0.543227554244988,-0.54124257409324,-0.493928781643987,
-0.437350207339252,-0.418815322744822,-0.389420111347358,-0.386293389671841,
-0.384742898303089,-0.383622741175249,-0.382430754638513,-0.381263102836175,
-0.378573637781362,-0.362942223505265,-0.351675082976487,-0.31576092867744,
-0.228857596800781,-0.224267620798758,-0.222991796692276,-0.222237937732807,
-0.221581558224078,-0.220760693292927,-0.219139338763125,-0.207455658227395,
-0.180828827667497,-0.122231133032375,-0.115094672208138,-0.0961741127566374,
-0.0667481036950851,-0.0636202284095314,-0.0620693413285802,-0.0609489808032809,
-0.0597568544353694,-0.0585890903058442,-0.0570568356257562,-0.0546319021202795,
-0.000956654129082594),.UNSPECIFIED.);
#854=B_SPLINE_CURVE_WITH_KNOTS('',3,(#56630,#56631,#56632,#56633,#56634,
#56635,#56636,#56637,#56638,#56639),.UNSPECIFIED.,.F.,.F.,(4,1,1,1,1,1,
1,4),(59.6902669190053,60.0055486427859,61.0043410465539,62.0031334503219,
63.0019258540899,64.0007182578579,64.9995106616259,65.9734422249333),
 .UNSPECIFIED.);
#855=B_SPLINE_CURVE_WITH_KNOTS('',3,(#56641,#56642,#56643,#56644,#56645,
#56646,#56647,#56648,#56649,#56650,#56651,#56652,#56653,#56654,#56655,#56656,
#56657,#56658,#56659,#56660,#56661,#56662,#56663,#56664,#56665,#56666,#56667,
#56668,#56669,#56670,#56671,#56672,#56673,#56674,#56675,#56676,#56677,#56678,
#56679,#56680,#56681,#56682,#56683,#56684,#56685,#56686,#56687,#56688,#56689,
#56690,#56691,#56692,#56693,#56694,#56695,#56696,#56697,#56698,#56699,#56700,
#56701,#56702,#56703,#56704,#56705,#56706,#56707,#56708,#56709,#56710,#56711,
#56712,#56713,#56714,#56715,#56716,#56717,#56718,#56719,#56720,#56721,#56722,
#56723,#56724,#56725,#56726,#56727,#56728,#56729,#56730,#56731,#56732,#56733,
#56734,#56735,#56736,#56737,#56738,#56739,#56740,#56741,#56742,#56743,#56744,
#56745,#56746,#56747,#56748,#56749,#56750,#56751,#56752,#56753,#56754,#56755,
#56756,#56757,#56758),.UNSPECIFIED.,.F.,.F.,(4,3,3,3,3,3,3,3,3,3,3,3,3,
3,3,3,3,3,3,3,3,3,3,3,3,3,3,3,3,3,3,3,3,3,3,3,3,3,3,4),(65.9734457253865,
65.9983030653939,66.1637658780536,66.3289121646202,66.4959579907556,66.6610242971856,
66.8290598831738,66.997095469162,67.1625582818218,67.3277045683883,67.4947503945237,
67.6598167009538,67.8278522869419,67.99588787293,68.1613506855898,68.3264969721563,
68.4935427982917,68.6586091047218,68.8266446907099,68.994680276698,69.1601430893578,
69.3252893759243,69.4923352020597,69.6574015084897,69.8254370944779,69.993472680466,
70.1589354931258,70.3240817796923,70.4911276058277,70.6561939122578,70.8242294982459,
70.992265084234,71.1577278968938,71.3228741834603,71.4899200095957,71.6549863160257,
71.8230219020139,71.991057488002,72.200388695361,72.2566310324091),
 .UNSPECIFIED.);
#856=B_SPLINE_CURVE_WITH_KNOTS('',3,(#56760,#56761,#56762,#56763,#56764,
#56765,#56766,#56767,#56768,#56769,#56770,#56771,#56772,#56773,#56774,#56775,
#56776,#56777,#56778,#56779,#56780,#56781,#56782,#56783,#56784,#56785,#56786,
#56787,#56788,#56789,#56790,#56791,#56792,#56793,#56794,#56795,#56796,#56797,
#56798,#56799,#56800,#56801,#56802,#56803,#56804,#56805,#56806,#56807,#56808,
#56809,#56810,#56811,#56812,#56813,#56814,#56815,#56816,#56817,#56818,#56819,
#56820,#56821,#56822,#56823,#56824,#56825,#56826,#56827,#56828,#56829,#56830,
#56831,#56832,#56833,#56834,#56835,#56836,#56837,#56838,#56839,#56840,#56841,
#56842,#56843,#56844,#56845,#56846,#56847,#56848,#56849,#56850,#56851,#56852,
#56853,#56854,#56855,#56856,#56857,#56858,#56859,#56860,#56861,#56862,#56863,
#56864,#56865,#56866,#56867,#56868,#56869,#56870,#56871,#56872,#56873,#56874,
#56875,#56876,#56877,#56878,#56879,#56880,#56881,#56882,#56883,#56884,#56885,
#56886,#56887,#56888,#56889,#56890,#56891,#56892,#56893,#56894,#56895,#56896,
#56897,#56898,#56899,#56900,#56901,#56902,#56903,#56904,#56905,#56906,#56907,
#56908,#56909,#56910,#56911,#56912,#56913,#56914,#56915,#56916,#56917,#56918,
#56919,#56920,#56921,#56922,#56923,#56924,#56925,#56926,#56927,#56928,#56929,
#56930,#56931,#56932,#56933,#56934,#56935,#56936,#56937,#56938,#56939,#56940,
#56941,#56942,#56943,#56944,#56945,#56946,#56947,#56948,#56949,#56950,#56951,
#56952,#56953,#56954,#56955,#56956,#56957,#56958,#56959,#56960,#56961,#56962,
#56963,#56964,#56965,#56966,#56967,#56968,#56969,#56970,#56971,#56972,#56973,
#56974,#56975,#56976,#56977,#56978,#56979,#56980,#56981,#56982,#56983,#56984,
#56985,#56986,#56987,#56988,#56989,#56990,#56991,#56992,#56993,#56994,#56995,
#56996,#56997,#56998,#56999,#57000,#57001,#57002,#57003,#57004,#57005,#57006,
#57007,#57008,#57009,#57010,#57011,#57012,#57013,#57014,#57015,#57016,#57017,
#57018,#57019,#57020,#57021,#57022,#57023,#57024,#57025,#57026,#57027,#57028,
#57029,#57030,#57031,#57032,#57033,#57034,#57035,#57036,#57037,#57038,#57039,
#57040,#57041,#57042,#57043,#57044,#57045,#57046,#57047,#57048,#57049,#57050,
#57051,#57052,#57053,#57054,#57055,#57056,#57057,#57058,#57059,#57060,#57061,
#57062,#57063,#57064,#57065,#57066,#57067,#57068,#57069,#57070,#57071,#57072,
#57073,#57074,#57075,#57076,#57077,#57078,#57079,#57080,#57081,#57082,#57083,
#57084,#57085,#57086,#57087,#57088,#57089,#57090,#57091,#57092,#57093,#57094,
#57095,#57096,#57097,#57098,#57099,#57100,#57101,#57102,#57103,#57104,#57105,
#57106,#57107,#57108,#57109,#57110,#57111,#57112,#57113,#57114,#57115,#57116,
#57117,#57118,#57119,#57120,#57121,#57122,#57123,#57124,#57125,#57126,#57127,
#57128,#57129,#57130,#57131,#57132,#57133,#57134,#57135,#57136,#57137,#57138,
#57139,#57140,#57141,#57142,#57143,#57144,#57145,#57146,#57147,#57148,#57149,
#57150,#57151,#57152,#57153,#57154,#57155,#57156,#57157,#57158,#57159,#57160,
#57161,#57162,#57163,#57164,#57165,#57166,#57167,#57168,#57169,#57170,#57171,
#57172,#57173,#57174,#57175,#57176,#57177,#57178,#57179,#57180,#57181,#57182,
#57183,#57184,#57185,#57186,#57187,#57188,#57189,#57190,#57191,#57192,#57193,
#57194,#57195,#57196,#57197,#57198,#57199,#57200,#57201,#57202,#57203,#57204,
#57205,#57206,#57207,#57208,#57209,#57210,#57211,#57212,#57213,#57214,#57215,
#57216,#57217,#57218,#57219,#57220,#57221,#57222,#57223,#57224,#57225,#57226,
#57227,#57228,#57229,#57230,#57231,#57232,#57233,#57234,#57235,#57236,#57237,
#57238,#57239,#57240,#57241,#57242,#57243,#57244,#57245,#57246,#57247,#57248,
#57249,#57250,#57251,#57252,#57253,#57254,#57255,#57256,#57257,#57258,#57259,
#57260,#57261,#57262,#57263,#57264,#57265,#57266,#57267,#57268,#57269,#57270,
#57271,#57272,#57273,#57274,#57275,#57276,#57277,#57278,#57279,#57280,#57281,
#57282,#57283,#57284,#57285,#57286,#57287,#57288,#57289,#57290,#57291,#57292,
#57293,#57294,#57295,#57296,#57297,#57298,#57299,#57300,#57301,#57302,#57303),
 .UNSPECIFIED.,.F.,.F.,(4,2,2,2,2,2,2,2,2,2,2,2,2,2,2,2,2,2,2,2,2,2,2,2,
2,2,2,2,2,2,2,2,2,2,2,2,2,2,2,2,2,2,2,2,2,2,2,2,2,2,2,2,2,2,2,2,2,2,2,2,
2,2,2,2,2,2,2,2,2,2,2,2,2,2,2,2,2,2,2,2,2,2,2,2,2,2,2,2,2,2,2,2,2,2,2,2,
2,2,2,2,2,2,2,2,2,2,2,2,2,2,2,2,2,2,2,2,2,2,2,2,2,2,2,2,2,2,2,2,2,2,2,2,
2,2,2,2,2,2,2,2,2,2,2,2,2,2,2,2,2,2,2,2,2,2,2,2,2,2,2,2,2,2,2,2,2,2,2,2,
2,2,2,2,2,2,2,2,2,2,2,2,2,2,2,2,2,2,2,2,2,2,2,2,2,2,2,2,2,2,2,2,2,2,2,2,
2,2,2,2,2,2,2,2,2,2,2,2,2,2,2,2,2,2,2,2,2,2,2,2,2,2,2,2,2,2,2,2,2,2,2,2,
2,2,2,2,2,2,2,2,2,2,2,2,2,2,2,2,2,2,2,2,2,2,2,2,2,2,2,2,2,2,2,4),(-4.06072099708927,
-3.99335883250795,-3.98986432731804,-3.98789113213452,-3.98654908115576,
-3.98524506280465,-3.98406271280404,-3.98254566511379,-3.97942270971339,
-3.95947578699461,-3.95391800962889,-3.91051859611513,-3.89505923928516,
-3.88056463606732,-3.84577748398674,-3.83314679121407,-3.82617200163564,
-3.82515357337312,-3.82423535193232,-3.82356587981738,-3.8229452778733,
-3.82209211660086,-3.82038927715486,-3.80563200668368,-3.74626137690391,
-3.7218834894641,-3.69245200208607,-3.67599833664372,-3.66982528611993,
-3.66544295850923,-3.66410013502624,-3.66279558392796,-3.66161338479511,
-3.66009741314531,-3.65697979802827,-3.63714848328601,-3.63163495430244,
-3.62471755983852,-3.6114546325119,-3.58526836572976,-3.51307499914043,
-3.50386602177083,-3.50233033768937,-3.50152749444441,-3.50093581596219,
-3.50028688677812,-3.4991245490177,-3.49561052448371,-3.43663258663599,
-3.39932239147558,-3.36653982717003,-3.3456908627346,-3.3424351978904,-3.3412026907319,
-3.33997251023921,-3.33876864411134,-3.33731931251696,-3.3337064342559,
-3.2992001267201,-3.2827255089068,-3.22500814929884,-3.20364408112494,-3.1823684717428,
-3.180194822064,-3.1792586535416,-3.17858588274869,-3.17796935610548,-3.17713210630159,
-3.17549192901851,-3.16258191564604,-3.16233608692326,-3.15930888062328,
-3.15842195058216,-3.1527272898174,-3.13846155992828,-3.08939200134123,
-3.05170411821848,-3.03236852671488,-3.02177486032964,-3.01938833865428,
-3.01824865641427,-3.01718031326076,-3.01605073694866,-3.01446446263209,
-3.01119287165909,-2.97577992317334,-2.97193228414542,-2.89135490638498,
-2.86248329602656,-2.85827740918681,-2.85704328117893,-2.85630625014124,
-2.8556474395333,-2.85480064370919,-2.85305029026807,-2.84179356387293,
-2.83822496429671,-2.83404092847237,-2.82944305127106,-2.81746956660634,
-2.74374768937198,-2.70503105063669,-2.70066263319988,-2.69734431409533,
-2.69579478259173,-2.69460320964923,-2.69348274980362,-2.6919307419077,
-2.68794289329454,-2.61977813425535,-2.57574433637417,-2.54047889482085,
-2.53570313449774,-2.53445303813546,-2.5337124404429,-2.53305432837918,
-2.53221365111005,-2.53049402119961,-2.51988415264725,-2.42252893770577,
-2.3783820321245,-2.37475266874645,-2.37313934502629,-2.37194262644947,
-2.37083100092052,-2.36931252291292,-2.36552214855692,-2.31731812633353,
-2.29253682582188,-2.24659114260684,-2.21727369035603,-2.21296733247813,
-2.21176195853327,-2.21103143410059,-2.21037126755577,-2.20952707959449,
-2.20774323554686,-2.19573123724008,-2.19427053656808,-2.19384302215281,
-2.15501915411242,-2.06164504275828,-2.05344270724838,-2.0512336373799,
-2.04991117758355,-2.04873263205055,-2.04724828292767,-2.0449315707945,
-2.0339625014908,-2.03209838231703,-2.03113092655583,-2.00381465955611,
-1.89716199242147,-1.89064747166278,-1.8893268086618,-1.88849130111971,
-1.88783371837105,-1.88708991301324,-1.88582552530768,-1.88088945973974,
-1.85755214598733,-1.81083269690741,-1.76235190115433,-1.7328539702797,
-1.72972467606081,-1.72817360178935,-1.72705334746834,-1.72586155826572,
-1.72427929289465,-1.72081901356831,-1.64966873624368,-1.57884786197904,
-1.56841732286664,-1.56670653881582,-1.56586757035643,-1.56520957304588,
-1.56446778710064,-1.56321263209929,-1.55838175820877,-1.52234578556094,
-1.43853473970214,-1.41008171286273,-1.40663665951705,-1.40507432079703,
-1.40388134562564,-1.40260976573028,-1.40062971990445,-1.39455555294364,
-1.3014081309899,-1.24789902350362,-1.24461783379485,-1.24348722478367,
-1.24284455802936,-1.2422512457827,-1.24145159462075,-1.23991044877817,
-1.23795369381672,-1.17231776782399,-1.10614949839837,-1.08677397701938,
-1.08367686565386,-1.08216470517731,-1.0809826726965,-1.07967544281879,
-1.07753579769192,-1.07004566605452,-1.02227931115542,-0.941977310151469,
-0.938514206695889,-0.923226949943139,-0.921317038015533,-0.920448756366965,
-0.919784845110124,-0.919170988122657,-0.918136522100213,-0.91525467365338,
-0.910969376460969,-0.885221855109396,-0.838361221338347,-0.791575463267311,
-0.764578602480926,-0.761519157616712,-0.759985496037017,-0.758869665614673,
-0.757674936584945,-0.75607560739648,-0.752524570562522,-0.703291855299055,
-0.634137888300082,-0.622056766666631,-0.614079229067929,-0.613298404318261,
-0.600446788120734,-0.59880824768054,-0.597971258372075,-0.5973546429039,
-0.596681484532904,-0.595763127177067,-0.593757364493382,-0.572264728431434,
-0.533756983152834,-0.464307329652044,-0.441649550359683,-0.43873280338078,
-0.4372355455115,-0.436129058403392,-0.434927851403497,-0.433290669199081,
-0.42953076741507,-0.390277941080532,-0.353032736615377,-0.317602269526929,
-0.287824194276457,-0.277625251695785,-0.275925833882827,-0.275089084212629,
-0.274431247352916,-0.273814825758799,-0.273083750482211,-0.270851228684327,
-0.241438404009671,-0.221724876065615,-0.146254067552353,-0.119252101270172,
-0.116192588404928,-0.114658937128221,-0.113543135266999,-0.112348456630963,
-0.110749229159927,-0.107198558774455,-0.0587031010197374,-0.000958174941626183),
 .UNSPECIFIED.);
#857=B_SPLINE_CURVE_WITH_KNOTS('',3,(#57305,#57306,#57307,#57308,#57309,
#57310,#57311,#57312,#57313,#57314,#57315,#57316,#57317,#57318,#57319,#57320,
#57321,#57322,#57323,#57324,#57325,#57326,#57327,#57328,#57329,#57330,#57331,
#57332,#57333,#57334,#57335,#57336,#57337,#57338,#57339,#57340,#57341,#57342,
#57343,#57344,#57345,#57346,#57347,#57348,#57349,#57350,#57351,#57352,#57353,
#57354,#57355,#57356,#57357,#57358,#57359,#57360,#57361,#57362,#57363,#57364,
#57365,#57366,#57367,#57368,#57369,#57370,#57371,#57372,#57373,#57374,#57375,
#57376,#57377,#57378,#57379,#57380,#57381,#57382,#57383,#57384,#57385,#57386,
#57387,#57388,#57389,#57390,#57391,#57392,#57393,#57394,#57395,#57396,#57397,
#57398,#57399,#57400,#57401,#57402,#57403,#57404,#57405,#57406,#57407,#57408,
#57409,#57410,#57411,#57412,#57413,#57414,#57415,#57416,#57417,#57418,#57419,
#57420,#57421,#57422,#57423,#57424,#57425,#57426,#57427,#57428,#57429,#57430,
#57431,#57432,#57433,#57434,#57435,#57436,#57437,#57438,#57439,#57440,#57441,
#57442,#57443,#57444,#57445,#57446,#57447,#57448,#57449,#57450,#57451,#57452,
#57453,#57454,#57455,#57456,#57457,#57458,#57459,#57460,#57461,#57462,#57463,
#57464,#57465,#57466,#57467,#57468,#57469,#57470,#57471,#57472,#57473,#57474,
#57475,#57476,#57477,#57478,#57479,#57480,#57481,#57482,#57483,#57484,#57485,
#57486,#57487,#57488,#57489,#57490,#57491,#57492,#57493,#57494,#57495,#57496,
#57497,#57498,#57499,#57500,#57501,#57502,#57503,#57504,#57505,#57506,#57507,
#57508,#57509,#57510,#57511,#57512,#57513,#57514,#57515,#57516,#57517,#57518,
#57519,#57520,#57521,#57522,#57523,#57524,#57525,#57526,#57527,#57528,#57529,
#57530,#57531,#57532,#57533,#57534,#57535,#57536,#57537,#57538,#57539,#57540,
#57541,#57542,#57543,#57544,#57545,#57546,#57547,#57548,#57549,#57550,#57551,
#57552,#57553,#57554,#57555,#57556,#57557,#57558,#57559,#57560,#57561,#57562,
#57563,#57564,#57565,#57566,#57567,#57568,#57569,#57570,#57571,#57572,#57573,
#57574,#57575,#57576,#57577,#57578,#57579,#57580,#57581,#57582,#57583,#57584,
#57585,#57586,#57587,#57588,#57589,#57590,#57591,#57592,#57593,#57594,#57595,
#57596,#57597,#57598,#57599,#57600,#57601,#57602,#57603,#57604,#57605,#57606,
#57607,#57608,#57609,#57610,#57611,#57612,#57613,#57614,#57615,#57616,#57617,
#57618,#57619,#57620,#57621,#57622,#57623,#57624,#57625,#57626,#57627,#57628,
#57629,#57630,#57631,#57632,#57633,#57634,#57635,#57636,#57637,#57638,#57639,
#57640,#57641,#57642,#57643,#57644,#57645,#57646,#57647,#57648,#57649,#57650,
#57651,#57652,#57653,#57654,#57655,#57656,#57657,#57658,#57659,#57660,#57661,
#57662,#57663,#57664,#57665,#57666,#57667,#57668,#57669,#57670,#57671,#57672,
#57673,#57674,#57675,#57676,#57677,#57678,#57679,#57680,#57681,#57682,#57683,
#57684,#57685,#57686,#57687,#57688,#57689,#57690,#57691,#57692,#57693,#57694,
#57695,#57696,#57697,#57698,#57699,#57700,#57701,#57702,#57703,#57704,#57705,
#57706,#57707,#57708,#57709,#57710,#57711,#57712,#57713,#57714,#57715,#57716,
#57717,#57718,#57719,#57720,#57721,#57722,#57723,#57724,#57725,#57726,#57727,
#57728,#57729,#57730,#57731,#57732,#57733,#57734,#57735,#57736,#57737,#57738,
#57739,#57740,#57741,#57742,#57743,#57744,#57745,#57746,#57747,#57748,#57749,
#57750,#57751,#57752,#57753,#57754,#57755,#57756,#57757,#57758,#57759,#57760,
#57761,#57762,#57763,#57764,#57765,#57766,#57767,#57768,#57769,#57770,#57771,
#57772,#57773,#57774,#57775,#57776,#57777,#57778,#57779,#57780,#57781,#57782,
#57783,#57784,#57785,#57786,#57787,#57788,#57789,#57790,#57791,#57792,#57793,
#57794,#57795,#57796,#57797,#57798,#57799,#57800,#57801,#57802,#57803,#57804,
#57805,#57806,#57807,#57808,#57809,#57810,#57811,#57812,#57813,#57814,#57815,
#57816,#57817,#57818,#57819,#57820,#57821,#57822,#57823,#57824,#57825,#57826,
#57827,#57828,#57829,#57830,#57831,#57832,#57833,#57834,#57835,#57836,#57837,
#57838,#57839,#57840,#57841,#57842,#57843,#57844,#57845,#57846,#57847,#57848,
#57849,#57850,#57851,#57852,#57853,#57854,#57855,#57856,#57857,#57858,#57859,
#57860,#57861,#57862,#57863,#57864,#57865,#57866,#57867,#57868,#57869,#57870,
#57871,#57872,#57873,#57874),.UNSPECIFIED.,.F.,.F.,(4,2,2,2,2,2,2,2,2,2,
2,2,2,2,2,2,2,2,2,2,2,2,2,2,2,2,2,2,2,2,2,2,2,2,2,2,2,2,2,2,2,2,2,2,2,2,
2,2,2,2,2,2,2,2,2,2,2,2,2,2,2,2,2,2,2,2,2,2,2,2,2,2,2,2,2,2,2,2,2,2,2,2,
2,2,2,2,2,2,2,2,2,2,2,2,2,2,2,2,2,2,2,2,2,2,2,2,2,2,2,2,2,2,2,2,2,2,2,2,
2,2,2,2,2,2,2,2,2,2,2,2,2,2,2,2,2,2,2,2,2,2,2,2,2,2,2,2,2,2,2,2,2,2,2,2,
2,2,2,2,2,2,2,2,2,2,2,2,2,2,2,2,2,2,2,2,2,2,2,2,2,2,2,2,2,2,2,2,2,2,2,2,
2,2,2,2,2,2,2,2,2,2,2,2,2,2,2,2,2,2,2,2,2,2,2,2,2,2,2,2,2,2,2,2,2,2,2,2,
2,2,2,2,2,2,2,2,2,2,2,2,2,2,2,2,2,2,2,2,2,2,2,2,2,2,2,2,2,2,2,2,2,2,2,2,
2,2,2,2,2,2,2,2,2,2,2,2,2,2,2,2,2,2,2,2,2,2,4),(-4.06035509702412,-4.0166517298775,
-4.01441449234829,-4.01320321613188,-4.01240935392366,-4.01177839014718,
-4.0111858386207,-4.01054102551551,-4.00959901378349,-4.00687614329751,
-3.96344012068408,-3.95513263774935,-3.94863346869362,-3.93572197765867,
-3.90829480679015,-3.86137867262917,-3.85396675872054,-3.85183550429672,
-3.85053035090128,-3.84934820007201,-3.847833116488,-3.84472024791505,-3.82499486328965,
-3.82346699629693,-3.74850398268308,-3.72815146569418,-3.70583639151684,
-3.69183241693507,-3.69015179062701,-3.68948116859182,-3.68880710987465,
-3.68819199372132,-3.68736035237359,-3.68574203743482,-3.6734309756206,
-3.67222603324444,-3.64471275551412,-3.5922979514002,-3.58458122203527,
-3.57475404198815,-3.53764502462112,-3.53121598294735,-3.52919321337834,
-3.52791224228308,-3.52672303600258,-3.52518347544333,-3.52263130483662,
-3.50803028184044,-3.50329310646057,-3.4361361105773,-3.39556471690477,
-3.38043522305897,-3.37293486249413,-3.36999684142157,-3.36786083453126,
-3.36694416536503,-3.36627148530115,-3.36565476527854,-3.36481685584832,
-3.3631742066735,-3.35019625601309,-3.34951295106431,-3.34902277559775,
-3.34171194001412,-3.32962865690209,-3.25180446507136,-3.23479466859309,
-3.21279733839221,-3.20812474648994,-3.2063374640299,-3.2051074860625,-3.20390341064808,
-3.20245333480698,-3.198836011597,-3.16414790006469,-3.15733380195568,-3.13225216005585,
-3.0813190479429,-3.05038336568593,-3.04744865076373,-3.04531489290246,
-3.04439845024177,-3.04372584797718,-3.04310911212548,-3.0422710559909,
-3.04062774696895,-3.02762913093425,-3.02747655949292,-3.02421289170875,
-2.93810625912863,-2.88864527961295,-2.88508082159158,-2.88347941107379,
-2.88228472433674,-2.88117008518121,-2.87963985990916,-2.87578052407747,
-2.82118886006901,-2.75040744906852,-2.72693675992932,-2.72443191548218,
-2.72311777253637,-2.72200460026686,-2.7213002316465,-2.72063656833257,
-2.71976872169285,-2.71786020901982,-2.7026006608473,-2.70196056742692,
-2.69958336163531,-2.69266171760252,-2.60185446692245,-2.56921604551337,
-2.56327651588692,-2.56131359441477,-2.56004600226084,-2.55885174992778,
-2.55728045008014,-2.55462011011217,-2.53799412256239,-2.44262326924299,
-2.40222025441417,-2.39997775357103,-2.39904059871654,-2.39836762626695,
-2.39775128309192,-2.39691481027123,-2.3952777203941,-2.38245512716111,
-2.37972931604978,-2.37938816853435,-2.37857158427384,-2.37538078043006,
-2.35711854414599,-2.31814068582426,-2.27463360217371,-2.24878665111095,
-2.24107033546701,-2.23890805706653,-2.23759590711746,-2.2364151844756,
-2.2349126127234,-2.23196276270387,-2.21476624792574,-2.20939448666436,
-2.13392782457848,-2.07949095587983,-2.07736505156232,-2.07644803888323,
-2.0757786753869,-2.07515760031897,-2.07430294230389,-2.07259451754829,
-2.05767098581951,-2.03154886797263,-1.93614392775167,-1.9197190911341,
-1.9170689067251,-1.91550048566944,-1.91430661639961,-1.91303769610962,
-1.91106918151433,-1.90508626731136,-1.87205682183273,-1.77964714656913,
-1.77495063079604,-1.77255254756129,-1.76933163515013,-1.75628317340285,
-1.75447920012865,-1.75361827412503,-1.75295559992204,-1.75223333896791,
-1.75106523868195,-1.74711857620357,-1.72182763167177,-1.6738899684977,
-1.59973192467694,-1.5950120821501,-1.59334523239723,-1.59219347735758,
-1.59113167848084,-1.58969525509982,-1.58696608281538,-1.570652055203,-1.53640182220655,
-1.44435135822236,-1.43342768418569,-1.43169272570572,-1.4308489015717,
-1.43019033883438,-1.42945138233257,-1.42820899750609,-1.42351932570883,
-1.38944364031986,-1.30983829910646,-1.27531095273964,-1.27169693654138,
-1.27024723482255,-1.26904309343857,-1.26783726527603,-1.2661028795937,
-1.26413351599843,-1.26064886122142,-1.23435704145997,-1.21025274677618,
-1.1145723884373,-1.1099200977961,-1.10863768251027,-1.10788225772218,-1.10722600480482,
-1.1064072159987,-1.10479606883131,-1.0934251569476,-1.06352934077086,-0.967697851666491,
-0.951413573628203,-0.948770166264878,-0.947203517049197,-0.946033568845979,
-0.944889420162937,-0.943084769295693,-0.941015624822096,-0.937281524752191,
-0.928932122532361,-0.904179144784289,-0.813229092305789,-0.806386242894336,
-0.804281506391321,-0.803229847509772,-0.788077388513619,-0.786171658095859,
-0.785304112533975,-0.78464027461973,-0.783920793555731,-0.782765650913222,
-0.778938672909169,-0.754919845777028,-0.702637641047084,-0.672052490261681,
-0.629972130168234,-0.626274618518567,-0.624771829041888,-0.623663897109187,
-0.622487666411461,-0.620999104013068,-0.619289460046474,-0.616440508327956,
-0.610648527030055,-0.595556253810271,-0.558732409586937,-0.482579963217482,
-0.478522044160389,-0.465289498241768,-0.463454652120675,-0.462600412727027,
-0.461938551423845,-0.461212638893719,-0.460028933877112,-0.455938237779528,
-0.429085467490673,-0.381173378458307,-0.355607585829613,-0.307417295202559,
-0.303625800914895,-0.30210666669628,-0.300994486561671,-0.299821039252192,
-0.298260289225738,-0.296527288122433,-0.293622078010773,-0.287674529661808,
-0.272031490896816,-0.252134646705724,-0.202282707677591,-0.144874251914233,
-0.141446793513763,-0.140295367026057,-0.139648407793025,-0.139055925684922,
-0.138248129782516,-0.136690136117058,-0.126777301712368,-0.104030397732436,
-0.000958019755019555),.UNSPECIFIED.);
#858=B_SPLINE_CURVE_WITH_KNOTS('',3,(#57876,#57877,#57878,#57879,#57880,
#57881,#57882,#57883,#57884,#57885,#57886,#57887,#57888,#57889,#57890,#57891,
#57892,#57893,#57894,#57895,#57896,#57897,#57898,#57899,#57900,#57901,#57902,
#57903,#57904,#57905,#57906,#57907,#57908,#57909,#57910,#57911,#57912,#57913,
#57914,#57915,#57916,#57917,#57918,#57919,#57920,#57921,#57922,#57923,#57924,
#57925,#57926,#57927,#57928,#57929,#57930,#57931,#57932,#57933,#57934,#57935,
#57936,#57937,#57938,#57939,#57940,#57941,#57942,#57943,#57944,#57945,#57946,
#57947,#57948,#57949,#57950,#57951,#57952,#57953,#57954,#57955,#57956,#57957,
#57958,#57959,#57960,#57961,#57962,#57963,#57964,#57965,#57966,#57967,#57968,
#57969,#57970,#57971,#57972,#57973,#57974,#57975,#57976,#57977,#57978,#57979,
#57980,#57981,#57982,#57983,#57984,#57985,#57986,#57987,#57988,#57989,#57990,
#57991,#57992,#57993,#57994,#57995,#57996,#57997,#57998,#57999,#58000,#58001,
#58002,#58003,#58004,#58005,#58006,#58007,#58008,#58009,#58010,#58011,#58012,
#58013,#58014,#58015,#58016,#58017,#58018,#58019,#58020,#58021,#58022,#58023,
#58024,#58025,#58026,#58027,#58028,#58029,#58030,#58031,#58032,#58033,#58034,
#58035,#58036,#58037,#58038,#58039,#58040,#58041,#58042,#58043,#58044,#58045,
#58046,#58047,#58048,#58049,#58050,#58051,#58052,#58053,#58054,#58055,#58056,
#58057,#58058,#58059,#58060,#58061,#58062,#58063,#58064,#58065,#58066,#58067,
#58068,#58069,#58070,#58071,#58072,#58073,#58074,#58075,#58076,#58077,#58078,
#58079,#58080,#58081,#58082,#58083,#58084,#58085,#58086,#58087,#58088,#58089,
#58090,#58091,#58092,#58093,#58094,#58095,#58096,#58097,#58098,#58099,#58100,
#58101,#58102,#58103,#58104,#58105,#58106,#58107,#58108,#58109,#58110,#58111,
#58112,#58113,#58114,#58115,#58116,#58117,#58118,#58119,#58120,#58121,#58122,
#58123,#58124,#58125,#58126,#58127,#58128,#58129,#58130,#58131,#58132,#58133,
#58134,#58135,#58136,#58137,#58138,#58139,#58140,#58141,#58142,#58143,#58144,
#58145,#58146,#58147,#58148,#58149,#58150,#58151,#58152,#58153,#58154,#58155,
#58156,#58157,#58158,#58159,#58160,#58161,#58162,#58163,#58164,#58165,#58166,
#58167,#58168,#58169,#58170,#58171,#58172,#58173,#58174,#58175,#58176,#58177,
#58178,#58179,#58180,#58181,#58182,#58183,#58184,#58185,#58186,#58187,#58188,
#58189,#58190,#58191,#58192,#58193,#58194,#58195,#58196,#58197,#58198,#58199,
#58200,#58201,#58202,#58203,#58204,#58205,#58206,#58207,#58208,#58209,#58210,
#58211,#58212,#58213,#58214,#58215,#58216,#58217,#58218,#58219,#58220,#58221,
#58222,#58223,#58224,#58225,#58226,#58227,#58228,#58229,#58230,#58231,#58232,
#58233,#58234,#58235,#58236,#58237,#58238,#58239,#58240,#58241,#58242,#58243,
#58244,#58245,#58246,#58247,#58248,#58249,#58250,#58251,#58252,#58253,#58254,
#58255,#58256,#58257,#58258,#58259,#58260,#58261,#58262,#58263,#58264,#58265,
#58266,#58267,#58268,#58269,#58270,#58271,#58272,#58273,#58274,#58275,#58276,
#58277,#58278,#58279,#58280,#58281,#58282,#58283,#58284,#58285,#58286,#58287,
#58288,#58289,#58290,#58291,#58292,#58293,#58294,#58295,#58296,#58297,#58298,
#58299,#58300,#58301,#58302,#58303,#58304,#58305,#58306,#58307,#58308,#58309,
#58310,#58311,#58312,#58313,#58314,#58315,#58316,#58317,#58318,#58319,#58320,
#58321,#58322,#58323,#58324,#58325,#58326,#58327,#58328,#58329,#58330,#58331,
#58332,#58333,#58334,#58335,#58336,#58337,#58338,#58339,#58340,#58341,#58342,
#58343,#58344,#58345,#58346,#58347,#58348,#58349,#58350,#58351,#58352,#58353,
#58354,#58355,#58356,#58357,#58358,#58359,#58360,#58361,#58362,#58363,#58364,
#58365,#58366,#58367,#58368,#58369,#58370,#58371,#58372,#58373,#58374,#58375,
#58376,#58377,#58378,#58379,#58380,#58381,#58382,#58383,#58384,#58385,#58386,
#58387,#58388,#58389,#58390,#58391,#58392,#58393,#58394,#58395,#58396,#58397,
#58398,#58399,#58400,#58401,#58402,#58403,#58404,#58405,#58406,#58407,#58408,
#58409,#58410,#58411,#58412,#58413,#58414,#58415,#58416,#58417,#58418,#58419,
#58420,#58421,#58422,#58423,#58424,#58425,#58426,#58427,#58428,#58429,#58430,
#58431,#58432,#58433,#58434,#58435),.UNSPECIFIED.,.F.,.F.,(4,2,2,2,2,2,
2,2,2,2,2,2,2,2,2,2,2,2,2,2,2,2,2,2,2,2,2,2,2,2,2,2,2,2,2,2,2,2,2,2,2,2,
2,2,2,2,2,2,2,2,2,2,2,2,2,2,2,2,2,2,2,2,2,2,2,2,2,2,2,2,2,2,2,2,2,2,2,2,
2,2,2,2,2,2,2,2,2,2,2,2,2,2,2,2,2,2,2,2,2,2,2,2,2,2,2,2,2,2,2,2,2,2,2,2,
2,2,2,2,2,2,2,2,2,2,2,2,2,2,2,2,2,2,2,2,2,2,2,2,2,2,2,2,2,2,2,2,2,2,2,2,
2,2,2,2,2,2,2,2,2,2,2,2,2,2,2,2,2,2,2,2,2,2,2,2,2,2,2,2,2,2,2,2,2,2,2,2,
2,2,2,2,2,2,2,2,2,2,2,2,2,2,2,2,2,2,2,2,2,2,2,2,2,2,2,2,2,2,2,2,2,2,2,2,
2,2,2,2,2,2,2,2,2,2,2,2,2,2,2,2,2,2,2,2,2,2,2,2,2,2,2,2,2,2,2,2,2,2,2,2,
2,2,2,2,2,2,2,2,2,2,2,2,2,2,2,2,2,2,2,2,2,4),(-4.06157938018324,-4.04929940099998,
-4.04313669884873,-4.04131232596992,-4.04003165241435,-4.03892991937186,
-4.03780813755122,-4.03632507831366,-4.03401321255865,-4.02310497446659,
-4.02139406885323,-4.02028008704974,-4.01356621420751,-3.90805438721962,
-3.88890260317504,-3.87978560112757,-3.8782613086838,-3.87746069641896,
-3.87686905537172,-3.87612314488593,-3.87484980277311,-3.87042193660157,
-3.78150287143677,-3.74386351870886,-3.72864913477018,-3.72282242989663,
-3.71996095138317,-3.71824617285081,-3.71669608891183,-3.71552538733439,
-3.71440954869489,-3.71287570741085,-3.70899694799184,-3.65204502404822,
-3.62708797663248,-3.61977440704627,-3.59500091758243,-3.56125084780741,
-3.55817238413721,-3.55593906894415,-3.55500335238149,-3.55433053383106,
-3.55371369247524,-3.55287562628584,-3.55123269384663,-3.53825350179553,
-3.53567362604543,-3.53428025433594,-3.5329163138851,-3.53156634385107,
-3.43909181058316,-3.41331882454522,-3.40314883353897,-3.39882591626416,
-3.39652617792721,-3.39504676601777,-3.39366584656413,-3.392515069685,-3.39114562703312,
-3.3887898333872,-3.37990578129682,-3.37612199512405,-3.37416965822323,
-3.27668455367688,-3.26254713810166,-3.24340234081891,-3.23427885059627,
-3.23275432905304,-3.2319536932878,-3.23130470981491,-3.2306384335494,-3.22939072103251,
-3.22518952237327,-3.15099584662564,-3.10756812923709,-3.08178807186003,
-3.07673025862297,-3.07415139383303,-3.07255448945885,-3.07108889421372,
-3.06993075953537,-3.06878539104258,-3.06714197739563,-3.062579710284,-2.98548767011597,
-2.93924193559961,-2.91600125356003,-2.91110905808973,-2.90984836153644,
-2.90910528813776,-2.90844742682768,-2.90761033645685,-2.90590917358895,
-2.89567051310861,-2.8204966298444,-2.75462558842416,-2.75176271239363,
-2.75004736479306,-2.74849554299325,-2.74732502098873,-2.74620912478893,
-2.74467500893042,-2.74079453020509,-2.683567348571,-2.61678080054094,-2.59774647492763,
-2.58882834480926,-2.58731303494897,-2.58651434407189,-2.58592290940046,
-2.58517564088467,-2.583896128718,-2.57941182824167,-2.48251434544779,-2.43084873181743,
-2.42731766836566,-2.42572216289348,-2.42452819124415,-2.42341154579004,
-2.42187437694899,-2.4179755298692,-2.35733522124522,-2.3263200895269,-2.29458188990736,
-2.26939329355178,-2.2654565459147,-2.26428949363732,-2.26356745093017,
-2.26290467449152,-2.26204320330842,-2.26023662725417,-2.24712245277621,
-2.24466784325711,-2.24429446543634,-2.24338296534809,-2.15819662764129,
-2.10817288312619,-2.10465025365646,-2.10305638775078,-2.10186275969647,
-2.10074579435196,-2.09920717801928,-2.09529933977342,-2.03084478645711,
-1.957000782158,-1.95370122822266,-1.94364921999502,-1.94197856353996,-1.94113616255659,
-1.94047780080694,-1.93973809712531,-1.93849222053185,-1.93376382991103,
-1.8991626165271,-1.84121037601963,-1.78612514958083,-1.7822608191165,-1.7807295182096,
-1.77961441375779,-1.77841952817089,-1.77681837260095,-1.77325663088332,
-1.7685316229984,-1.72427175975269,-1.63143879327304,-1.62096599449034,
-1.61925292262388,-1.61841342881897,-1.61775529863996,-1.6170136631592,
-1.6157594598391,-1.61094044978144,-1.57507911925762,-1.47935487149066,
-1.46186741121067,-1.45890189822566,-1.45739581777379,-1.45621451913527,
-1.45490397437831,-1.45274948678109,-1.44511322580062,-1.4194135619701,
-1.37612437444694,-1.32092242972616,-1.31667255096297,-1.31280623304216,
-1.31172084910497,-1.30943952881608,-1.29829376465542,-1.29654840007514,
-1.29570252906064,-1.29505906466221,-1.29434119459483,-1.29358732000092,
-1.29247189912089,-1.2904785917702,-1.27475569666923,-1.2557275134402,-1.16771063580113,
-1.13986211622061,-1.13643602005204,-1.13487719828291,-1.13368480470536,
-1.13241180352474,-1.1304253354784,-1.12429909491525,-1.0298526904658,-0.977628311817583,
-0.974405073116387,-0.973282601625687,-0.972641563368027,-0.971994872609418,
-0.971164815782008,-0.970254000503845,-0.968763426002787,-0.965785298004453,
-0.934033265607395,-0.849456122746227,-0.843525608270362,-0.835817114406746,
-0.816557359610101,-0.81346577064542,-0.811954739114466,-0.810772873511582,
-0.809465096477722,-0.807322894047626,-0.79980738511717,-0.751761812465428,
-0.740128041908324,-0.656499929790048,-0.651980566136304,-0.650697229765164,
-0.649949105456,-0.649304983865417,-0.648498982449435,-0.647621507404035,
-0.64621097044235,-0.643450014753405,-0.615681081428755,-0.530832711525216,
-0.525760435977595,-0.515414580338789,-0.493967875588897,-0.490777911785087,
-0.489263796717977,-0.488078194231609,-0.486784902593373,-0.48470762996452,
-0.477803351052211,-0.436116845752842,-0.393385536315315,-0.371882380492645,
-0.35991336209724,-0.330832676303123,-0.328648583552053,-0.327789716192758,
-0.327167496906952,-0.326512345553086,-0.32562651982592,-0.324637764769449,
-0.322958270023982,-0.319452894459693,-0.274882886790835,-0.201068384060724,
-0.171784825943187,-0.168661151373046,-0.167111434905487,-0.165991493052065,
-0.164799415412777,-0.163215709158981,-0.159748056324509,-0.0851461990511898,
-0.0100209562745193,-0.00639465879684327,-0.0052174293180658,-0.0045653640992891,
-0.00391770964333854,-0.00328293326089312,-0.00247679621787721,-0.000957169744583153),
 .UNSPECIFIED.);
#859=B_SPLINE_CURVE_WITH_KNOTS('',3,(#58437,#58438,#58439,#58440,#58441,
#58442,#58443,#58444,#58445,#58446,#58447,#58448,#58449,#58450,#58451,#58452,
#58453,#58454,#58455,#58456,#58457,#58458,#58459,#58460,#58461,#58462,#58463,
#58464,#58465,#58466,#58467,#58468,#58469,#58470,#58471,#58472,#58473,#58474,
#58475,#58476,#58477,#58478,#58479,#58480,#58481,#58482,#58483,#58484,#58485,
#58486,#58487,#58488,#58489,#58490,#58491,#58492,#58493,#58494,#58495,#58496,
#58497,#58498,#58499,#58500,#58501,#58502,#58503,#58504,#58505,#58506,#58507,
#58508,#58509,#58510,#58511,#58512,#58513,#58514,#58515,#58516,#58517,#58518,
#58519,#58520,#58521,#58522,#58523,#58524,#58525,#58526,#58527,#58528,#58529,
#58530,#58531,#58532,#58533,#58534,#58535,#58536,#58537,#58538,#58539,#58540,
#58541,#58542,#58543,#58544,#58545,#58546,#58547,#58548,#58549,#58550,#58551),
 .UNSPECIFIED.,.F.,.F.,(4,3,3,3,3,3,3,3,3,3,3,3,3,3,3,3,3,3,3,3,3,3,3,3,
3,3,3,3,3,3,3,3,3,3,3,3,3,3,4),(109.955742875847,110.120897363818,110.285736432889,
110.450546875869,110.615309592152,110.780469619239,110.943961234955,111.109424047615,
111.274570334181,111.441616160317,111.606682466747,111.774718052735,111.942753638723,
112.108216451383,112.273362737949,112.440408564085,112.605474870515,112.773510456503,
112.941546042491,113.107008855151,113.272155141717,113.439200967853,113.604267274283,
113.772302860271,113.940338446259,114.105801258919,114.270947545485,114.437993371621,
114.603059678051,114.771095264039,114.939130850027,115.104593662687,115.269739949253,
115.436785775389,115.601852081819,115.769887667807,115.937923253795,116.137885025419,
116.238928182531),.UNSPECIFIED.);
#860=B_SPLINE_CURVE_WITH_KNOTS('',3,(#58553,#58554,#58555,#58556,#58557,
#58558,#58559,#58560,#58561,#58562,#58563,#58564,#58565,#58566,#58567,#58568,
#58569,#58570,#58571,#58572,#58573,#58574,#58575,#58576,#58577,#58578,#58579,
#58580,#58581,#58582,#58583,#58584,#58585,#58586,#58587,#58588,#58589,#58590,
#58591,#58592,#58593,#58594,#58595,#58596,#58597,#58598,#58599,#58600,#58601,
#58602,#58603,#58604,#58605,#58606,#58607,#58608,#58609,#58610,#58611,#58612,
#58613,#58614,#58615,#58616,#58617,#58618,#58619,#58620,#58621,#58622,#58623,
#58624,#58625,#58626,#58627,#58628,#58629,#58630,#58631,#58632,#58633,#58634,
#58635,#58636,#58637,#58638,#58639,#58640,#58641,#58642,#58643,#58644,#58645,
#58646,#58647,#58648,#58649,#58650,#58651,#58652,#58653,#58654,#58655,#58656,
#58657,#58658,#58659,#58660,#58661,#58662,#58663,#58664,#58665,#58666,#58667,
#58668,#58669,#58670),.UNSPECIFIED.,.F.,.F.,(4,3,3,3,3,3,3,3,3,3,3,3,3,
3,3,3,3,3,3,3,3,3,3,3,3,3,3,3,3,3,3,3,3,3,3,3,3,3,3,4),(116.238928182823,
116.402979220447,116.567099493634,116.731267675343,116.895801311704,116.936715657563,
117.102178470223,117.267324756789,117.434370582925,117.599436889355,117.767472475343,
117.935508061331,118.100970873991,118.266117160557,118.433162986693,118.598229293123,
118.766264879111,118.934300465099,119.099763277759,119.264909564325,119.431955390461,
119.597021696891,119.765057282879,119.933092868867,120.098555681527,120.263701968093,
120.430747794229,120.595814100659,120.763849686647,120.931885272635,121.097348085295,
121.262494371861,121.429540197997,121.594606504427,121.762642090415,121.930677676403,
122.098914915071,122.266779046469,122.434399504567,122.522113490003),
 .UNSPECIFIED.);
#861=B_SPLINE_CURVE_WITH_KNOTS('',3,(#58672,#58673,#58674,#58675,#58676,
#58677,#58678,#58679,#58680,#58681,#58682,#58683,#58684,#58685,#58686,#58687,
#58688,#58689,#58690,#58691,#58692,#58693,#58694,#58695,#58696,#58697,#58698,
#58699,#58700,#58701,#58702,#58703,#58704,#58705,#58706,#58707,#58708,#58709,
#58710,#58711,#58712,#58713,#58714,#58715,#58716,#58717,#58718,#58719,#58720,
#58721,#58722,#58723,#58724,#58725,#58726,#58727,#58728,#58729,#58730,#58731,
#58732,#58733,#58734,#58735,#58736,#58737,#58738,#58739,#58740,#58741,#58742,
#58743,#58744,#58745,#58746,#58747,#58748,#58749,#58750,#58751,#58752,#58753,
#58754,#58755,#58756,#58757,#58758,#58759,#58760,#58761,#58762,#58763,#58764,
#58765,#58766,#58767,#58768,#58769,#58770,#58771,#58772,#58773,#58774,#58775,
#58776,#58777,#58778,#58779,#58780,#58781,#58782,#58783,#58784,#58785,#58786,
#58787,#58788,#58789,#58790,#58791,#58792,#58793,#58794,#58795,#58796,#58797,
#58798,#58799,#58800,#58801,#58802,#58803,#58804,#58805,#58806,#58807,#58808,
#58809,#58810,#58811,#58812,#58813,#58814,#58815,#58816,#58817,#58818,#58819,
#58820,#58821,#58822,#58823,#58824,#58825,#58826,#58827,#58828,#58829,#58830,
#58831,#58832,#58833,#58834,#58835,#58836,#58837,#58838,#58839,#58840,#58841,
#58842,#58843,#58844,#58845,#58846,#58847,#58848,#58849,#58850,#58851,#58852,
#58853,#58854,#58855,#58856,#58857,#58858,#58859,#58860,#58861,#58862,#58863,
#58864,#58865,#58866,#58867,#58868,#58869,#58870,#58871,#58872,#58873,#58874,
#58875,#58876,#58877,#58878,#58879,#58880,#58881,#58882,#58883,#58884,#58885,
#58886,#58887,#58888,#58889,#58890,#58891,#58892,#58893,#58894,#58895,#58896,
#58897,#58898,#58899,#58900,#58901,#58902,#58903,#58904,#58905,#58906,#58907,
#58908,#58909,#58910,#58911,#58912,#58913,#58914,#58915,#58916,#58917,#58918,
#58919,#58920,#58921,#58922,#58923,#58924,#58925,#58926,#58927,#58928,#58929,
#58930,#58931,#58932,#58933,#58934,#58935,#58936,#58937,#58938,#58939,#58940,
#58941,#58942,#58943,#58944,#58945,#58946,#58947,#58948,#58949,#58950,#58951,
#58952,#58953,#58954,#58955,#58956,#58957,#58958,#58959,#58960,#58961,#58962,
#58963,#58964,#58965,#58966,#58967,#58968,#58969,#58970,#58971,#58972,#58973,
#58974,#58975,#58976,#58977,#58978,#58979,#58980,#58981,#58982,#58983,#58984,
#58985,#58986,#58987,#58988,#58989,#58990,#58991,#58992,#58993,#58994,#58995,
#58996,#58997,#58998,#58999,#59000,#59001,#59002,#59003,#59004,#59005,#59006,
#59007,#59008,#59009,#59010,#59011,#59012,#59013,#59014,#59015,#59016,#59017,
#59018,#59019,#59020,#59021,#59022,#59023,#59024,#59025,#59026,#59027,#59028,
#59029,#59030,#59031,#59032,#59033,#59034,#59035,#59036,#59037,#59038,#59039,
#59040,#59041,#59042,#59043,#59044,#59045,#59046,#59047,#59048,#59049,#59050,
#59051,#59052,#59053,#59054,#59055,#59056,#59057,#59058,#59059,#59060,#59061,
#59062,#59063,#59064,#59065,#59066,#59067,#59068,#59069,#59070,#59071,#59072,
#59073,#59074,#59075,#59076,#59077,#59078,#59079,#59080,#59081,#59082,#59083,
#59084,#59085,#59086,#59087,#59088,#59089,#59090,#59091,#59092,#59093,#59094,
#59095,#59096,#59097,#59098,#59099,#59100,#59101,#59102,#59103,#59104,#59105,
#59106,#59107,#59108,#59109,#59110,#59111,#59112,#59113,#59114,#59115,#59116,
#59117,#59118,#59119,#59120,#59121,#59122,#59123,#59124,#59125,#59126,#59127,
#59128,#59129,#59130,#59131,#59132,#59133,#59134,#59135,#59136,#59137,#59138,
#59139,#59140,#59141,#59142,#59143,#59144,#59145,#59146,#59147,#59148,#59149,
#59150,#59151,#59152,#59153,#59154,#59155,#59156,#59157,#59158,#59159,#59160,
#59161,#59162,#59163,#59164,#59165,#59166,#59167,#59168,#59169,#59170,#59171,
#59172,#59173,#59174,#59175,#59176,#59177,#59178,#59179,#59180,#59181,#59182,
#59183,#59184,#59185,#59186,#59187,#59188,#59189,#59190,#59191,#59192,#59193,
#59194,#59195,#59196,#59197,#59198,#59199,#59200,#59201,#59202,#59203,#59204,
#59205,#59206,#59207,#59208,#59209,#59210,#59211,#59212,#59213),
 .UNSPECIFIED.,.F.,.F.,(4,2,2,2,2,2,2,2,2,2,2,2,2,2,2,2,2,2,2,2,2,2,2,2,
2,2,2,2,2,2,2,2,2,2,2,2,2,2,2,2,2,2,2,2,2,2,2,2,2,2,2,2,2,2,2,2,2,2,2,2,
2,2,2,2,2,2,2,2,2,2,2,2,2,2,2,2,2,2,2,2,2,2,2,2,2,2,2,2,2,2,2,2,2,2,2,2,
2,2,2,2,2,2,2,2,2,2,2,2,2,2,2,2,2,2,2,2,2,2,2,2,2,2,2,2,2,2,2,2,2,2,2,2,
2,2,2,2,2,2,2,2,2,2,2,2,2,2,2,2,2,2,2,2,2,2,2,2,2,2,2,2,2,2,2,2,2,2,2,2,
2,2,2,2,2,2,2,2,2,2,2,2,2,2,2,2,2,2,2,2,2,2,2,2,2,2,2,2,2,2,2,2,2,2,2,2,
2,2,2,2,2,2,2,2,2,2,2,2,2,2,2,2,2,2,2,2,2,2,2,2,2,2,2,2,2,2,2,2,2,2,2,2,
2,2,2,2,2,2,2,2,2,2,2,2,2,2,2,2,2,2,2,2,2,2,2,2,2,2,2,2,2,2,4),(-4.05964741638998,
-3.96771229126991,-3.94150414541432,-3.93094429280988,-3.92936219553924,
-3.92854966160014,-3.92795695033789,-3.92731296325643,-3.92617504777717,
-3.92284664434187,-3.8648582764161,-3.81524979992763,-3.792800589541,-3.77908159504651,
-3.77368464773745,-3.76974918824406,-3.76808607126964,-3.76698046514721,
-3.76577679679464,-3.76432797633504,-3.76071780657895,-3.71015855344816,
-3.68610806425633,-3.64110350011837,-3.61833275389342,-3.60842068353853,
-3.60686343850952,-3.60605609903267,-3.6054639815529,-3.60481744882046,
-3.60366685587539,-3.60024237368457,-3.54292283090896,-3.49313517667065,
-3.4737707172032,-3.45777677408279,-3.45173155455545,-3.44879163046223,
-3.44704457637554,-3.44546961706033,-3.44429540565269,-3.44318603656636,
-3.44167617936555,-3.43793550282111,-3.39321776437008,-3.36394521822187,
-3.31305615860536,-3.28904017461946,-3.28521462158442,-3.28405999859921,
-3.28334086270451,-3.28267735823723,-3.28181026970665,-3.27990562676699,
-3.26476514025276,-3.2190110895415,-3.16969887049525,-3.14102808116928,
-3.13162673130971,-3.12754905153014,-3.12534471108212,-3.12344521573008,
-3.12220309086274,-3.12100883422539,-3.11943771402838,-3.11677809055926,
-3.1001673370388,-3.00461560865409,-2.97477944604189,-2.96342359530593,
-2.96181335210144,-2.96099491036414,-2.96034489323205,-2.95959187004256,
-2.95831909188324,-2.95375585972012,-2.85749620001157,-2.80660749120145,
-2.80361217178845,-2.80184223584783,-2.80025078183398,-2.79907358275466,
-2.79796818669785,-2.79647406933887,-2.79282381167851,-2.75320019014866,
-2.67908456860427,-2.65253511008579,-2.64074982339514,-2.63912561218791,
-2.63830431981327,-2.63764810111837,-2.63689498376993,-2.63562169306295,
-2.63105321088003,-2.5348350736172,-2.48774411415948,-2.4803162640277,-2.47818348671641,
-2.4768780689198,-2.47569611594782,-2.47418189352805,-2.47107293877906,
-2.45142772286948,-2.44434385311394,-2.37011369653049,-2.36539503371552,
-2.34608695847689,-2.3271350577283,-2.31792870084004,-2.31640093189904,
-2.31559978112025,-2.31500829712149,-2.31426332157452,-2.31299331878772,
-2.30859270326235,-2.22327091505121,-2.1603539009291,-2.15659628645676,
-2.15495999908904,-2.15375940965304,-2.15265346301431,-2.15115689336974,
-2.14824135194245,-2.12558733384093,-2.10978650655946,-2.10105107139752,
-2.03017404498582,-2.0203502428717,-2.01782256634113,-2.01569296517961,
-2.01240743623537,-2.00965183280716,-2.00924011927456,-2.00793231192996,
-1.99574131449827,-1.99412823246604,-1.9932979943166,-1.99268328292312,
-1.99200900686524,-1.99106457642466,-1.98877858804073,-1.93679367794855,
-1.86475012865124,-1.83730324110417,-1.83389066365808,-1.83233460959198,
-1.83114292716277,-1.829869317681,-1.82787907134717,-1.82171924122576,-1.78708768356907,
-1.68814030881204,-1.67322900787048,-1.67152105273368,-1.67066653830971,
-1.67004552331697,-1.66937617952708,-1.66845911641212,-1.66633275164356,
-1.61069468857292,-1.53540209617109,-1.53395808323956,-1.51413432127003,
-1.51101682807647,-1.5095007963325,-1.50831849616965,-1.50701377849806,
-1.50488459078559,-1.49749303646297,-1.45078689121974,-1.36373313256029,
-1.36142065094032,-1.35030682318781,-1.34856303831821,-1.34771751752846,
-1.34705882554826,-1.34633588248368,-1.34514305956238,-1.3437121208279,
-1.34089600478512,-1.31214660044174,-1.24100184839937,-1.22390690020138,
-1.19212069868279,-1.18857858356026,-1.18714082784542,-1.18593985645542,
-1.18470573259045,-1.18289898532629,-1.17809850576683,-1.11864321824673,
-1.04511964565717,-1.02800063807625,-1.02603282290231,-1.02515393054467,
-1.0244883493741,-1.02377401220692,-1.0226642332556,-1.01921195057052,-0.974640679061058,
-0.925454618227494,-0.870059336861939,-0.866192405283044,-0.864660643989419,
-0.863545404928706,-0.86235056409264,-0.8607497957851,-0.857190262767763,
-0.829458600875901,-0.805606869339249,-0.742893449047942,-0.727737038477988,
-0.722951424643649,-0.705424934252106,-0.70344459236857,-0.702642668464635,
-0.701973997833251,-0.701279533861291,-0.7002584142616,-0.697472879945731,
-0.693367244688429,-0.681498816352566,-0.665552064240402,-0.626455091227633,
-0.614253972735603,-0.575093365147055,-0.546770142444156,-0.543328856613729,
-0.541767119389444,-0.540574146475342,-0.539302126462858,-0.537320484874904,
-0.53123445412487,-0.436793619122999,-0.412785742341316,-0.383120021847698,
-0.380926487465927,-0.380065944303145,-0.379443236356708,-0.378774752214637,
-0.378114064819476,-0.377231998908609,-0.373079144838368,-0.366196798443717,
-0.340885499502995,-0.315743134760332,-0.246335292556876,-0.223713824583821,
-0.220798472693206,-0.219301595709063,-0.218195225749841,-0.21699398689879,
-0.215356476855426,-0.211594576082469,-0.193456395079492,-0.146609572933761,
-0.129604422682245,-0.121071321008588,-0.111362890677887,-0.104328173526239,
-0.0612248244022761,-0.0585113140628138,-0.0575704700533938,-0.0569258502208856,
-0.0563329889305497,-0.0557015798871949,-0.0549066667988391,-0.053693128986409,
-0.0514504190834883,-0.000956747946955143),.UNSPECIFIED.);
#862=B_SPLINE_CURVE_WITH_KNOTS('',3,(#59215,#59216,#59217,#59218,#59219,
#59220,#59221,#59222,#59223,#59224,#59225,#59226,#59227,#59228,#59229,#59230,
#59231,#59232,#59233,#59234,#59235,#59236,#59237,#59238,#59239,#59240,#59241,
#59242,#59243,#59244,#59245,#59246,#59247,#59248,#59249,#59250,#59251,#59252,
#59253,#59254,#59255,#59256,#59257,#59258,#59259,#59260,#59261,#59262,#59263,
#59264,#59265,#59266,#59267,#59268,#59269,#59270,#59271,#59272,#59273,#59274,
#59275,#59276,#59277,#59278,#59279,#59280,#59281,#59282,#59283,#59284,#59285,
#59286,#59287,#59288,#59289,#59290,#59291,#59292,#59293,#59294,#59295,#59296,
#59297,#59298,#59299,#59300,#59301,#59302,#59303,#59304,#59305,#59306,#59307,
#59308,#59309,#59310,#59311,#59312,#59313,#59314,#59315,#59316,#59317,#59318,
#59319,#59320,#59321,#59322,#59323,#59324,#59325,#59326,#59327,#59328,#59329,
#59330,#59331,#59332,#59333,#59334,#59335,#59336,#59337,#59338,#59339,#59340,
#59341,#59342,#59343,#59344,#59345,#59346,#59347,#59348,#59349,#59350,#59351,
#59352,#59353,#59354,#59355,#59356,#59357,#59358,#59359,#59360,#59361,#59362,
#59363,#59364,#59365,#59366,#59367,#59368,#59369,#59370,#59371,#59372,#59373,
#59374,#59375,#59376,#59377,#59378,#59379,#59380,#59381,#59382,#59383,#59384,
#59385,#59386,#59387,#59388,#59389,#59390,#59391,#59392,#59393,#59394,#59395,
#59396,#59397,#59398,#59399,#59400,#59401,#59402,#59403,#59404,#59405,#59406,
#59407,#59408,#59409,#59410,#59411,#59412,#59413,#59414,#59415,#59416,#59417,
#59418,#59419,#59420,#59421,#59422,#59423,#59424,#59425,#59426,#59427,#59428,
#59429,#59430,#59431,#59432,#59433,#59434,#59435,#59436,#59437,#59438,#59439,
#59440,#59441,#59442,#59443,#59444,#59445,#59446,#59447,#59448,#59449,#59450,
#59451,#59452,#59453,#59454,#59455,#59456,#59457,#59458,#59459,#59460,#59461,
#59462,#59463,#59464,#59465,#59466,#59467,#59468,#59469,#59470,#59471,#59472,
#59473,#59474,#59475,#59476,#59477,#59478,#59479,#59480,#59481,#59482,#59483,
#59484,#59485,#59486,#59487,#59488,#59489,#59490,#59491,#59492,#59493,#59494,
#59495,#59496,#59497,#59498,#59499,#59500,#59501,#59502,#59503,#59504,#59505,
#59506,#59507,#59508,#59509,#59510,#59511,#59512,#59513,#59514,#59515,#59516,
#59517,#59518,#59519,#59520,#59521,#59522,#59523,#59524,#59525,#59526,#59527,
#59528,#59529,#59530,#59531,#59532,#59533,#59534,#59535,#59536,#59537,#59538,
#59539,#59540,#59541,#59542,#59543,#59544,#59545,#59546,#59547,#59548,#59549,
#59550,#59551,#59552,#59553,#59554,#59555,#59556,#59557,#59558,#59559,#59560,
#59561,#59562,#59563,#59564,#59565,#59566,#59567,#59568,#59569,#59570,#59571,
#59572,#59573,#59574,#59575,#59576,#59577,#59578,#59579,#59580,#59581,#59582,
#59583,#59584,#59585,#59586,#59587,#59588,#59589,#59590,#59591,#59592,#59593,
#59594,#59595,#59596,#59597,#59598,#59599,#59600,#59601,#59602,#59603,#59604,
#59605,#59606,#59607,#59608,#59609,#59610,#59611,#59612,#59613,#59614,#59615,
#59616,#59617,#59618,#59619,#59620,#59621,#59622,#59623,#59624,#59625,#59626,
#59627,#59628,#59629,#59630,#59631,#59632,#59633,#59634,#59635,#59636,#59637,
#59638,#59639,#59640,#59641,#59642,#59643,#59644,#59645,#59646,#59647,#59648,
#59649,#59650,#59651,#59652,#59653,#59654,#59655,#59656,#59657,#59658,#59659,
#59660,#59661,#59662,#59663,#59664,#59665,#59666,#59667,#59668,#59669,#59670,
#59671,#59672,#59673,#59674,#59675,#59676,#59677,#59678,#59679,#59680,#59681,
#59682,#59683,#59684,#59685,#59686,#59687,#59688,#59689,#59690,#59691,#59692,
#59693,#59694,#59695,#59696,#59697,#59698,#59699,#59700,#59701,#59702,#59703,
#59704,#59705,#59706,#59707,#59708,#59709,#59710,#59711,#59712,#59713,#59714,
#59715,#59716,#59717,#59718,#59719,#59720,#59721,#59722,#59723,#59724,#59725,
#59726,#59727,#59728,#59729,#59730,#59731,#59732,#59733,#59734,#59735,#59736,
#59737,#59738,#59739,#59740),.UNSPECIFIED.,.F.,.F.,(4,2,2,2,2,2,2,2,2,2,
2,2,2,2,2,2,2,2,2,2,2,2,2,2,2,2,2,2,2,2,2,2,2,2,2,2,2,2,2,2,2,2,2,2,2,2,
2,2,2,2,2,2,2,2,2,2,2,2,2,2,2,2,2,2,2,2,2,2,2,2,2,2,2,2,2,2,2,2,2,2,2,2,
2,2,2,2,2,2,2,2,2,2,2,2,2,2,2,2,2,2,2,2,2,2,2,2,2,2,2,2,2,2,2,2,2,2,2,2,
2,2,2,2,2,2,2,2,2,2,2,2,2,2,2,2,2,2,2,2,2,2,2,2,2,2,2,2,2,2,2,2,2,2,2,2,
2,2,2,2,2,2,2,2,2,2,2,2,2,2,2,2,2,2,2,2,2,2,2,2,2,2,2,2,2,2,2,2,2,2,2,2,
2,2,2,2,2,2,2,2,2,2,2,2,2,2,2,2,2,2,2,2,2,2,2,2,2,2,2,2,2,2,2,2,2,2,2,2,
2,2,2,2,2,2,2,2,2,2,2,2,2,2,2,2,2,2,2,2,2,2,2,2,2,2,2,2,2,2,2,2,2,2,2,2,
4),(-4.06114224698561,-4.00001303158136,-3.96528985380881,-3.959118626996,
-3.95712662291717,-3.95585237803074,-3.95466044648186,-3.95310456183611,
-3.95049748498737,-3.93490221555494,-3.92983053850339,-3.92821890119364,
-3.85262336244111,-3.83150826821505,-3.79897703100541,-3.79607454941721,
-3.79528181464072,-3.79465108344775,-3.79405855594289,-3.79341287334194,
-3.7924680859699,-3.78972696349286,-3.74440205570379,-3.71004024964133,
-3.67042696822791,-3.64457976068527,-3.63686433379437,-3.63470190137461,
-3.63338957264201,-3.63220863409026,-3.63070571216941,-3.62775493710997,
-3.61054768063997,-3.6094901380153,-3.53902604148103,-3.49812184619457,
-3.48202430360799,-3.47689974011342,-3.47359373374267,-3.47249849170568,
-3.47188261771507,-3.47122420957702,-3.47038172863594,-3.46865349226174,
-3.45787418778024,-3.42814344596467,-3.36427505272666,-3.33605139278129,
-3.31551897369797,-3.31262995128466,-3.31115999022718,-3.31009392816273,
-3.30895700237288,-3.30734427372795,-3.30298176152018,-3.23311418678964,
-3.1853722183985,-3.16182022701342,-3.15516852601445,-3.15247811999766,
-3.15051705649481,-3.14961512860368,-3.14894508542379,-3.14832471740542,
-3.14747299955162,-3.14533066318468,-3.11879577598211,-3.04448852433188,
-2.99390205281782,-2.99032252751395,-2.98871805885583,-2.98752258107513,
-2.98640827745896,-2.98488018612651,-2.98103494843924,-2.9280843670292,
-2.86508267184413,-2.84661426088346,-2.83110406606961,-2.82817669725758,
-2.82713361063186,-2.8265196115286,-2.82585673517008,-2.82499487006355,
-2.82355656835764,-2.81516819735642,-2.71424617545012,-2.67071867008357,
-2.66741109118186,-2.66585780917715,-2.66467040098836,-2.6635412187936,
-2.66195669583781,-2.65869258461702,-2.62363440047175,-2.55779579698852,
-2.50720989183457,-2.50508955252923,-2.50417349864469,-2.50350428200063,
-2.50288293201163,-2.50202728820265,-2.50031502419303,-2.48527276429107,
-2.44453476750168,-2.39351253240482,-2.34878880014281,-2.34503670495141,
-2.34340109613744,-2.34220033998085,-2.34109377277499,-2.33959565383928,
-2.33667500769443,-2.31389988141551,-2.29823112953338,-2.21890685638057,
-2.19403202459556,-2.18375362864259,-2.18218168756151,-2.18137111019561,
-2.18071550783119,-2.18005350831207,-2.17882691282501,-2.17480515329745,
-2.10030382621504,-2.05692714523976,-2.03117461525432,-2.02366086652744,
-2.02142375927547,-2.02009472513819,-2.0190344970597,-2.01761425589761,
-2.01496156572746,-2.00028367548369,-1.97099808392245,-1.92115105916958,
-1.86378704739135,-1.86300850996411,-1.86017785106389,-1.85911413743264,
-1.85848477272725,-1.85788680338899,-1.85703769178822,-1.85527600282917,
-1.83780101911226,-1.81865185858543,-1.73484232555152,-1.72761076611245,
-1.72215181902474,-1.70249246601315,-1.69938220727608,-1.69786746831221,
-1.69668516593646,-1.69537941702786,-1.6932462226591,-1.68581813519658,
-1.63872427347712,-1.55210306882951,-1.5501045547725,-1.53867470255187,
-1.53691617974683,-1.53606766137065,-1.53540852959051,-1.53467221650713,
-1.53344173538332,-1.52887998342651,-1.49647240665228,-1.40025392101122,
-1.39660920896643,-1.37947947046207,-1.37653288547301,-1.37503089896113,
-1.37385010855601,-1.37253733826996,-1.37041602830899,-1.36304824917662,
-1.31633468132226,-1.24245971127869,-1.21653207090875,-1.21440063136174,
-1.21355078928561,-1.21293091682349,-1.21226052724157,-1.21133811382842,
-1.20935081154521,-1.18617746785199,-1.16360025720917,-1.09483637160338,
-1.07996115238234,-1.05724080802097,-1.05432200839922,-1.05282431012563,
-1.05171779793573,-1.0505168542246,-1.04888055013317,-1.0452274786955,-1.04029765039158,
-0.992644272547453,-0.937048251885136,-0.894691841960536,-0.892004654175016,
-0.891067679287383,-0.890424162169914,-0.88983106874731,-0.889016787497805,
-0.887459009777875,-0.879396112447043,-0.862067764628417,-0.79601548088594,
-0.735676717232088,-0.731779323973176,-0.730242368410367,-0.729125751834298,
-0.727931692835962,-0.726335868815505,-0.722919528044963,-0.700375873421387,
-0.680524479667042,-0.631226351387264,-0.57274738391304,-0.569531998340495,
-0.568410581942753,-0.567769759554352,-0.567175948158349,-0.566355826027135,
-0.565474202695044,-0.561322210745656,-0.532548018902344,-0.482280282293101,
-0.461658274880054,-0.446902437031573,-0.412562908864718,-0.40895326461438,
-0.407504219745201,-0.406300191464685,-0.405069438788336,-0.403836222115316,
-0.402130094620727,-0.392366567468876,-0.375034081561154,-0.342880070155488,
-0.316554158052441,-0.250709848203937,-0.247060423852895,-0.245880168433941,
-0.245227489125309,-0.24463624563698,-0.243839638718882,-0.242990778729422,
-0.241648628012149,-0.226759001258927,-0.192580550022399,-0.178973385328588,
-0.164474901946467,-0.0910876980290721,-0.0867414813788719,-0.0851312652438351,
-0.0839949960333603,-0.082928656904803,-0.0814569148344321,-0.0798804066408968,
-0.0773501622759522,-0.00095726213492795),.UNSPECIFIED.);
#863=B_SPLINE_CURVE_WITH_KNOTS('',3,(#59742,#59743,#59744,#59745,#59746,
#59747,#59748,#59749,#59750,#59751,#59752,#59753,#59754,#59755,#59756,#59757,
#59758,#59759,#59760,#59761,#59762,#59763,#59764,#59765,#59766,#59767,#59768,
#59769,#59770,#59771,#59772,#59773,#59774,#59775,#59776,#59777,#59778,#59779,
#59780,#59781,#59782,#59783,#59784,#59785,#59786,#59787,#59788,#59789,#59790,
#59791,#59792,#59793,#59794,#59795,#59796,#59797,#59798,#59799,#59800,#59801,
#59802,#59803,#59804,#59805,#59806,#59807,#59808,#59809,#59810,#59811,#59812,
#59813,#59814,#59815,#59816,#59817,#59818,#59819,#59820,#59821,#59822,#59823,
#59824,#59825,#59826,#59827,#59828,#59829,#59830,#59831,#59832,#59833,#59834,
#59835,#59836,#59837,#59838,#59839,#59840,#59841,#59842,#59843,#59844,#59845,
#59846,#59847,#59848,#59849,#59850,#59851,#59852,#59853,#59854,#59855,#59856,
#59857,#59858,#59859,#59860,#59861,#59862,#59863,#59864,#59865,#59866,#59867,
#59868,#59869,#59870,#59871,#59872,#59873,#59874,#59875,#59876,#59877,#59878,
#59879,#59880,#59881,#59882,#59883,#59884,#59885,#59886,#59887,#59888,#59889,
#59890,#59891,#59892,#59893,#59894,#59895,#59896,#59897,#59898,#59899,#59900,
#59901,#59902,#59903,#59904,#59905,#59906,#59907,#59908,#59909,#59910,#59911,
#59912,#59913,#59914,#59915,#59916,#59917,#59918,#59919,#59920,#59921,#59922,
#59923,#59924,#59925,#59926,#59927,#59928,#59929,#59930,#59931,#59932,#59933,
#59934,#59935,#59936,#59937,#59938,#59939,#59940,#59941,#59942,#59943,#59944,
#59945,#59946,#59947,#59948,#59949,#59950,#59951,#59952,#59953,#59954,#59955,
#59956,#59957,#59958,#59959,#59960,#59961,#59962,#59963,#59964,#59965,#59966,
#59967,#59968,#59969,#59970,#59971,#59972,#59973,#59974,#59975,#59976,#59977,
#59978,#59979,#59980,#59981,#59982,#59983,#59984,#59985,#59986,#59987,#59988,
#59989,#59990,#59991,#59992,#59993,#59994,#59995,#59996,#59997,#59998,#59999,
#60000,#60001,#60002,#60003,#60004,#60005,#60006,#60007,#60008,#60009,#60010,
#60011,#60012,#60013,#60014,#60015,#60016,#60017,#60018,#60019,#60020,#60021,
#60022,#60023,#60024,#60025,#60026,#60027,#60028,#60029,#60030,#60031,#60032,
#60033,#60034,#60035,#60036,#60037,#60038,#60039,#60040,#60041,#60042,#60043,
#60044,#60045,#60046,#60047,#60048,#60049,#60050,#60051,#60052,#60053,#60054,
#60055,#60056,#60057,#60058,#60059,#60060,#60061,#60062,#60063,#60064,#60065,
#60066,#60067,#60068,#60069,#60070,#60071,#60072,#60073,#60074,#60075,#60076,
#60077,#60078,#60079,#60080,#60081,#60082,#60083,#60084,#60085,#60086,#60087,
#60088,#60089,#60090,#60091,#60092,#60093,#60094,#60095,#60096,#60097,#60098,
#60099,#60100,#60101,#60102,#60103,#60104,#60105,#60106,#60107,#60108,#60109,
#60110,#60111,#60112,#60113,#60114,#60115,#60116,#60117,#60118,#60119,#60120,
#60121,#60122,#60123,#60124,#60125,#60126,#60127,#60128,#60129,#60130,#60131,
#60132,#60133,#60134,#60135,#60136,#60137,#60138,#60139,#60140,#60141,#60142,
#60143,#60144,#60145,#60146,#60147,#60148,#60149,#60150,#60151,#60152,#60153,
#60154,#60155,#60156,#60157,#60158,#60159,#60160,#60161,#60162,#60163,#60164,
#60165,#60166,#60167,#60168,#60169,#60170,#60171,#60172,#60173,#60174,#60175,
#60176,#60177,#60178,#60179,#60180,#60181,#60182,#60183,#60184,#60185,#60186,
#60187,#60188,#60189,#60190,#60191,#60192,#60193,#60194,#60195,#60196,#60197,
#60198,#60199,#60200,#60201,#60202,#60203,#60204,#60205,#60206,#60207,#60208,
#60209,#60210,#60211,#60212,#60213,#60214,#60215,#60216,#60217,#60218,#60219,
#60220,#60221,#60222,#60223,#60224,#60225,#60226,#60227,#60228,#60229,#60230,
#60231,#60232,#60233,#60234,#60235,#60236,#60237,#60238,#60239,#60240,#60241,
#60242,#60243,#60244,#60245,#60246,#60247,#60248,#60249,#60250,#60251,#60252,
#60253,#60254,#60255,#60256,#60257,#60258,#60259,#60260,#60261,#60262,#60263,
#60264,#60265,#60266,#60267,#60268,#60269,#60270,#60271,#60272,#60273,#60274,
#60275,#60276,#60277,#60278,#60279,#60280,#60281,#60282,#60283),
 .UNSPECIFIED.,.F.,.F.,(4,2,2,2,2,2,2,2,2,2,2,2,2,2,2,2,2,2,2,2,2,2,2,2,
2,2,2,2,2,2,2,2,2,2,2,2,2,2,2,2,2,2,2,2,2,2,2,2,2,2,2,2,2,2,2,2,2,2,2,2,
2,2,2,2,2,2,2,2,2,2,2,2,2,2,2,2,2,2,2,2,2,2,2,2,2,2,2,2,2,2,2,2,2,2,2,2,
2,2,2,2,2,2,2,2,2,2,2,2,2,2,2,2,2,2,2,2,2,2,2,2,2,2,2,2,2,2,2,2,2,2,2,2,
2,2,2,2,2,2,2,2,2,2,2,2,2,2,2,2,2,2,2,2,2,2,2,2,2,2,2,2,2,2,2,2,2,2,2,2,
2,2,2,2,2,2,2,2,2,2,2,2,2,2,2,2,2,2,2,2,2,2,2,2,2,2,2,2,2,2,2,2,2,2,2,2,
2,2,2,2,2,2,2,2,2,2,2,2,2,2,2,2,2,2,2,2,2,2,2,2,2,2,2,2,2,2,2,2,2,2,2,2,
2,2,2,2,2,2,2,2,2,2,2,2,2,2,2,2,2,2,2,2,2,2,2,2,2,2,2,2,2,2,4),(-4.05869209090443,
-3.99347258329797,-3.98346120577144,-3.98208998989009,-3.98092451464955,
-3.98020309274606,-3.97954063639963,-3.97867924005389,-3.97687161016431,
-3.96371109793033,-3.90330803197401,-3.88941211170496,-3.87624746347955,
-3.83715160599044,-3.82354092163575,-3.82168028279355,-3.82038502854958,
-3.81911343292964,-3.81792135991715,-3.81636152330673,-3.81292736988021,
-3.78478033641603,-3.74368455190069,-3.71872396463521,-3.69443095110323,
-3.67053686034673,-3.6638476086542,-3.65978456155156,-3.65890867439712,
-3.65809280794549,-3.65743725174819,-3.6567789718537,-3.65556946147614,
-3.65168459272487,-3.58622242948792,-3.53618493112009,-3.50251232365159,
-3.49908882405575,-3.49749477855142,-3.49630162099827,-3.49518553492371,
-3.49364881906767,-3.48974944812107,-3.42835259914059,-3.37827520698967,
-3.35648731837807,-3.34413012705425,-3.33990362330514,-3.33705462975647,
-3.3360131527021,-3.33531912081921,-3.33465087535234,-3.33384947320327,
-3.33187047351668,-3.31435871924742,-3.31382632047267,-3.3125988638393,
-3.30854524847308,-3.28356320945582,-3.24019468590367,-3.20230389615886,
-3.18025010728797,-3.1767512160406,-3.17514500253715,-3.17394980917278,
-3.17283690956727,-3.17131251484101,-3.16748578571744,-3.11619593857404,
-3.04558135936149,-3.01900253211695,-3.01631127234367,-3.014308405995,-3.01341173944794,
-3.01274607162127,-3.01211996984645,-3.01124563256016,-3.0089672390449,
-2.9722445492164,-2.90871398816466,-2.85933728395486,-2.8547410468211,-2.85296761210967,
-2.85173329621102,-2.8505335193074,-2.84909883931475,-2.84557274001998,
-2.81431629949973,-2.73026740070147,-2.69715718415143,-2.69411100829313,
-2.69191249499498,-2.69097380915784,-2.69030069604425,-2.68968491886818,
-2.68885020798521,-2.68721950567013,-2.67456346912241,-2.67364163046961,
-2.67152532678081,-2.58650640212305,-2.54022047085763,-2.53286843056385,
-2.53074384441092,-2.52944045390558,-2.52825837622549,-2.52674126404126,
-2.52361670736036,-2.50362107215227,-2.49803349926442,-2.49106017750256,
-2.42408106944974,-2.40938055692036,-2.3747786175866,-2.37165999457705,
-2.36940385937669,-2.3684645821546,-2.36779138447463,-2.36717577572786,
-2.36634164429621,-2.36429900219243,-2.34269448234719,-2.32577188766398,
-2.3044653320574,-2.26378635877624,-2.21778784599914,-2.21046274708313,
-2.20834091785456,-2.20703810852483,-2.20585582779685,-2.20433743613603,
-2.20120662294794,-2.18107557005975,-2.17518809458094,-2.16809225126649,
-2.08376849980179,-2.05205266781258,-2.04754746600594,-2.0463227676784,
-2.04558798297482,-2.0449289364761,-2.04407878345783,-2.04231068430796,
-2.03065364045763,-2.00419858862673,-1.93092385407595,-1.91720484133572,
-1.89009050337525,-1.8866888911869,-1.88513496052345,-1.88394370547852,
-1.88266938439029,-1.88067560285052,-1.8744859227434,-1.83957993519644,
-1.73929276459037,-1.7375876994948,-1.72584766613721,-1.72407567310284,
-1.72322466373908,-1.72256541454763,-1.72183088768666,-1.72060770990543,
-1.71611983870235,-1.68462950451055,-1.60238725051932,-1.56771372954905,
-1.56409698447731,-1.56264708351932,-1.56144312909577,-1.56021325160227,
-1.55842607341528,-1.55375352080345,-1.53175274533621,-1.5147471883378,
-1.43424825479234,-1.40393268570916,-1.40173035145221,-1.40086847269809,
-1.40024554654462,-1.39957757221406,-1.39866821012499,-1.39658506680723,
-1.39376449718957,-1.36493221022214,-1.27610191022616,-1.24492844691205,
-1.24140390423043,-1.23982714316561,-1.23863192639957,-1.23739206812402,
-1.23553672083929,-1.23336869885897,-1.22938368883327,-1.13765909431138,
-1.12749760261023,-1.08196819024256,-1.07922875452862,-1.07828431096571,
-1.0776387945916,-1.0770463633003,-1.07623673967627,-1.07466884839031,-1.06448897261829,
-1.04010870110007,-0.939603093648809,-0.938552483257593,-0.921333857077579,
-0.918383186266903,-0.916880593927318,-0.915700050302603,-0.914414776111133,
-0.912459832095758,-0.910080233292249,-0.905548931503627,-0.894711326258798,
-0.859207650419671,-0.76130582002647,-0.75689293812503,-0.755621468557156,
-0.754876101976212,-0.754284574964159,-0.753483711848289,-0.751957616907415,
-0.742792813056688,-0.723726030183432,-0.680291557784628,-0.623314637256144,
-0.618189956915694,-0.598861164980214,-0.595766585476366,-0.594255066479902,
-0.593073264135499,-0.591971443730137,-0.590069670801379,-0.584577625832007,
-0.576374678789233,-0.552196945338399,-0.518410522256117,-0.438426681111395,
-0.434254081621596,-0.433009775291891,-0.43234423675009,-0.431689013672621,
-0.430884522809926,-0.429341446107404,-0.419783446657282,-0.406008561488972,
-0.36213950823656,-0.31736657151772,-0.303685341310649,-0.276741440802165,
-0.273683882194079,-0.272150807996261,-0.271035234906337,-0.269908404751917,
-0.268747950612618,-0.266234986174628,-0.253179862043125,-0.227573960953151,
-0.210980423150055,-0.11633706344912,-0.111685449240086,-0.110403127475343,
-0.10964773761638,-0.108991502158835,-0.108172718567571,-0.10656152904128,
-0.0951882948480381,-0.0652806265416462,-0.00095819449416442),
 .UNSPECIFIED.);
#864=B_SPLINE_CURVE_WITH_KNOTS('',3,(#60285,#60286,#60287,#60288,#60289,
#60290,#60291,#60292,#60293,#60294),.UNSPECIFIED.,.F.,.F.,(4,1,1,1,1,1,
1,4),(160.22122533308,160.883581423355,161.882373827123,162.881166230891,
163.879958634659,164.878751038427,165.877543442195,166.50441064026),
 .UNSPECIFIED.);
#865=B_SPLINE_CURVE_WITH_KNOTS('',3,(#60296,#60297,#60298,#60299,#60300,
#60301,#60302,#60303,#60304,#60305,#60306,#60307,#60308,#60309,#60310,#60311,
#60312,#60313,#60314,#60315,#60316,#60317,#60318,#60319,#60320,#60321,#60322,
#60323,#60324,#60325,#60326,#60327,#60328,#60329,#60330,#60331,#60332,#60333,
#60334,#60335,#60336,#60337,#60338,#60339,#60340,#60341,#60342,#60343,#60344,
#60345,#60346,#60347,#60348,#60349,#60350,#60351,#60352,#60353,#60354,#60355,
#60356,#60357,#60358,#60359,#60360,#60361,#60362,#60363,#60364,#60365,#60366,
#60367,#60368,#60369,#60370,#60371,#60372,#60373,#60374,#60375,#60376,#60377,
#60378,#60379,#60380,#60381,#60382,#60383,#60384,#60385,#60386,#60387,#60388,
#60389,#60390,#60391,#60392,#60393,#60394,#60395,#60396,#60397,#60398,#60399,
#60400,#60401,#60402,#60403,#60404,#60405,#60406,#60407,#60408,#60409,#60410,
#60411,#60412,#60413,#60414,#60415,#60416,#60417,#60418,#60419,#60420,#60421,
#60422,#60423,#60424,#60425,#60426,#60427,#60428,#60429,#60430,#60431,#60432,
#60433,#60434,#60435,#60436,#60437,#60438,#60439,#60440,#60441,#60442,#60443,
#60444,#60445,#60446,#60447,#60448,#60449,#60450,#60451,#60452,#60453,#60454,
#60455,#60456,#60457,#60458,#60459,#60460,#60461,#60462,#60463,#60464,#60465,
#60466,#60467,#60468,#60469,#60470,#60471,#60472,#60473,#60474,#60475,#60476,
#60477,#60478,#60479,#60480,#60481,#60482,#60483,#60484,#60485,#60486,#60487,
#60488,#60489,#60490,#60491,#60492,#60493,#60494,#60495,#60496,#60497,#60498,
#60499,#60500,#60501,#60502,#60503,#60504,#60505,#60506,#60507,#60508,#60509,
#60510,#60511,#60512,#60513,#60514,#60515,#60516,#60517,#60518,#60519,#60520,
#60521,#60522,#60523,#60524,#60525,#60526,#60527,#60528,#60529,#60530,#60531,
#60532,#60533,#60534,#60535,#60536,#60537,#60538,#60539,#60540,#60541,#60542,
#60543,#60544,#60545,#60546,#60547,#60548,#60549,#60550,#60551,#60552,#60553,
#60554,#60555,#60556,#60557,#60558,#60559,#60560,#60561,#60562,#60563,#60564,
#60565,#60566,#60567,#60568,#60569,#60570,#60571,#60572,#60573,#60574,#60575,
#60576,#60577,#60578,#60579,#60580,#60581,#60582,#60583,#60584,#60585,#60586,
#60587,#60588,#60589,#60590,#60591,#60592,#60593,#60594,#60595,#60596,#60597,
#60598,#60599,#60600,#60601,#60602,#60603,#60604,#60605,#60606,#60607,#60608,
#60609,#60610,#60611,#60612,#60613,#60614,#60615,#60616,#60617,#60618,#60619,
#60620,#60621,#60622,#60623,#60624,#60625,#60626,#60627,#60628,#60629,#60630,
#60631,#60632,#60633,#60634,#60635,#60636,#60637,#60638,#60639,#60640,#60641,
#60642,#60643,#60644,#60645,#60646,#60647,#60648,#60649,#60650,#60651,#60652,
#60653,#60654,#60655,#60656,#60657,#60658,#60659,#60660,#60661,#60662,#60663,
#60664,#60665,#60666,#60667,#60668,#60669,#60670,#60671,#60672,#60673,#60674,
#60675,#60676,#60677,#60678,#60679,#60680,#60681,#60682,#60683,#60684,#60685,
#60686,#60687,#60688,#60689,#60690,#60691,#60692,#60693,#60694,#60695,#60696,
#60697,#60698,#60699,#60700,#60701,#60702,#60703,#60704,#60705,#60706,#60707,
#60708,#60709,#60710,#60711,#60712,#60713,#60714,#60715,#60716,#60717,#60718,
#60719,#60720,#60721,#60722,#60723,#60724,#60725,#60726,#60727,#60728,#60729,
#60730,#60731,#60732,#60733,#60734,#60735,#60736,#60737,#60738,#60739,#60740,
#60741,#60742,#60743,#60744,#60745,#60746,#60747,#60748,#60749,#60750,#60751,
#60752,#60753,#60754,#60755,#60756,#60757,#60758,#60759,#60760,#60761,#60762,
#60763,#60764,#60765,#60766,#60767,#60768,#60769,#60770,#60771,#60772,#60773,
#60774,#60775,#60776,#60777,#60778,#60779,#60780,#60781,#60782,#60783,#60784,
#60785,#60786,#60787,#60788,#60789,#60790,#60791,#60792,#60793,#60794,#60795,
#60796,#60797,#60798,#60799,#60800,#60801,#60802,#60803,#60804,#60805,#60806,
#60807,#60808,#60809,#60810,#60811,#60812,#60813,#60814,#60815,#60816,#60817,
#60818,#60819),.UNSPECIFIED.,.F.,.F.,(4,2,2,2,2,2,2,2,2,2,2,2,2,2,2,2,2,
2,2,2,2,2,2,2,2,2,2,2,2,2,2,2,2,2,2,2,2,2,2,2,2,2,2,2,2,2,2,2,2,2,2,2,2,
2,2,2,2,2,2,2,2,2,2,2,2,2,2,2,2,2,2,2,2,2,2,2,2,2,2,2,2,2,2,2,2,2,2,2,2,
2,2,2,2,2,2,2,2,2,2,2,2,2,2,2,2,2,2,2,2,2,2,2,2,2,2,2,2,2,2,2,2,2,2,2,2,
2,2,2,2,2,2,2,2,2,2,2,2,2,2,2,2,2,2,2,2,2,2,2,2,2,2,2,2,2,2,2,2,2,2,2,2,
2,2,2,2,2,2,2,2,2,2,2,2,2,2,2,2,2,2,2,2,2,2,2,2,2,2,2,2,2,2,2,2,2,2,2,2,
2,2,2,2,2,2,2,2,2,2,2,2,2,2,2,2,2,2,2,2,2,2,2,2,2,2,2,2,2,2,2,2,2,2,2,2,
2,2,2,2,2,2,2,2,2,2,2,2,2,2,2,2,2,2,2,2,2,2,2,2,2,2,2,2,4),(-4.06096447082831,
-4.00218619815695,-3.94477647938606,-3.94253132446907,-3.94159355959484,
-3.94092033114405,-3.94030388564263,-3.93946746319739,-3.93783103262021,
-3.92503600526774,-3.92421528180793,-3.92384404994144,-3.92091631400899,
-3.91936481455205,-3.91258690982016,-3.83258152742667,-3.81363505663347,
-3.79449492223586,-3.78759300721156,-3.78280477880188,-3.78100146097245,
-3.77990095384434,-3.77870891521173,-3.77715297966182,-3.77374301963086,
-3.74640823523031,-3.69806326678204,-3.65951927375612,-3.63286771916824,
-3.62120232266677,-3.61958165477234,-3.61876097136293,-3.61810465559998,
-3.61735077774152,-3.61607471325399,-3.61148185493626,-3.52449023872323,
-3.48367139400823,-3.46942556509153,-3.46387560092107,-3.45985061544652,
-3.45817174346589,-3.45706703643878,-3.45586669751534,-3.45443160820636,
-3.45090584531046,-3.37392507615069,-3.32691600444757,-3.30161928590703,
-3.29767236744177,-3.29650417531516,-3.29578185452777,-3.29511912296023,
-3.29425811965844,-3.29245397534329,-3.27940438196209,-3.27619211305589,
-3.27127246523667,-3.19059316537041,-3.1453069782317,-3.14051838099005,
-3.13804073358735,-3.1359519726925,-3.13466593904349,-3.13348511219617,
-3.131982728221,-3.12903425580655,-3.11186844919232,-3.01612324975095,-2.97991181478353,
-2.97506901227411,-2.97381269649704,-2.97307059878349,-2.97241256541246,
-2.97157387445079,-2.96986475617299,-2.95947000414462,-2.87448059752547,
-2.82314947137994,-2.81801133204022,-2.81540252962181,-2.81379308992444,
-2.8123173458174,-2.81115816706667,-2.81001633651661,-2.80838570988961,
-2.80390740195913,-2.72833995387676,-2.68094284014332,-2.66179922003237,
-2.65278611138067,-2.65126652046725,-2.65046692997369,-2.64987541720512,
-2.64912883379502,-2.64785236033582,-2.64339567427571,-2.54598670059336,
-2.49980145970686,-2.49245734782595,-2.49033289184346,-2.4890291048637,
-2.48784635453783,-2.48632794242201,-2.483199157835,-2.46313571648298,-2.4574954764943,
-2.45202725289263,-2.36598701959304,-2.33398727655881,-2.32945840855069,
-2.32823107073707,-2.32749547474342,-2.32683621274415,-2.32598647905774,
-2.32422172579294,-2.31265302249965,-2.22873157693695,-2.18837152038456,
-2.17089175140843,-2.16811331468741,-2.16666640337302,-2.16549066861251,
-2.16414199577729,-2.16187552442417,-2.15385961439457,-2.15190754881952,
-2.05316758066489,-2.03066949219596,-2.02885137315661,-2.02393503293034,
-2.02071318300825,-2.00766199684392,-2.00585763963675,-2.00499652960808,
-2.00433371339276,-2.00361129727941,-2.00244294526099,-1.9984954249464,
-1.97319893352562,-1.92525083697928,-1.8510603639767,-1.84635179450875,
-1.84468640984145,-1.84353491495814,-1.8424727738264,-1.84103500967911,
-1.83830037014701,-1.82187124566366,-1.78678273244212,-1.69581062178425,
-1.68475214244394,-1.68301055622251,-1.68216531106741,-1.68150646991398,
-1.68076808598611,-1.67952868788944,-1.67487314505085,-1.6412568690676,
-1.53617931582387,-1.52487048793311,-1.52252859795815,-1.5210361244916,
-1.51985627315952,-1.51853773410441,-1.51634783376683,-1.5083534570595,
-1.45472595018595,-1.40249205000551,-1.37276629193726,-1.36191379794683,
-1.36018191338134,-1.35933868162962,-1.35868016350463,-1.35794081087457,
-1.35672168331944,-1.35224917882957,-1.3207772346126,-1.24485977429493,
-1.23313866151306,-1.2036113627,-1.20048095296736,-1.19892949155482,-1.19780903512143,
-1.19661710284132,-1.19503476998065,-1.19167731122357,-1.14056506878807,
-1.07107161587476,-1.04001100918898,-1.03779766557423,-1.03693376739693,
-1.03631018419738,-1.0356423012306,-1.03498269910086,-1.03340585903183,
-1.02285790269602,-0.996665709950003,-0.938832095524279,-0.881642903737174,
-0.877762424009881,-0.876228265704909,-0.875112323616314,-0.873917709857394,
-0.872318940869264,-0.868863293324374,-0.790051523509473,-0.74833230944164,
-0.717311327989627,-0.71509847592135,-0.714234645701145,-0.713611068238389,
-0.712943148479055,-0.712283496309154,-0.710706317102811,-0.700150731074761,
-0.685545466164838,-0.632432026131966,-0.559510763708878,-0.555209752309043,
-0.553606833484714,-0.552472536521956,-0.551405490517319,-0.549928747396166,
-0.548345328634094,-0.540816664643569,-0.507161542245567,-0.452574164137795,
-0.396157054923731,-0.39435466387973,-0.392282472882878,-0.391465448273148,
-0.390792767079811,-0.390103407430586,-0.389408364851707,-0.388436928662513,
-0.382613521948706,-0.37178156362884,-0.341796723288487,-0.316457124211684,
-0.237435799224814,-0.232692414017665,-0.230836305217791,-0.229716055112962,
-0.228523929692737,-0.226940637619189,-0.225209784927132,-0.222309520217191,
-0.203920827161043,-0.163957449155886,-0.149379467111453,-0.134468359562708,
-0.0738342822100937,-0.0702103412711332,-0.0690333851441698,-0.0683813659741074,
-0.0677900038366501,-0.0669921883173715,-0.066141646527258,-0.0647954905755286,
-0.054637818555212,-0.000957111951693946),.UNSPECIFIED.);
#866=B_SPLINE_CURVE_WITH_KNOTS('',3,(#60821,#60822,#60823,#60824,#60825,
#60826,#60827,#60828,#60829,#60830,#60831,#60832,#60833,#60834,#60835,#60836,
#60837,#60838,#60839,#60840,#60841,#60842,#60843,#60844,#60845,#60846,#60847,
#60848,#60849,#60850,#60851,#60852,#60853,#60854,#60855,#60856,#60857,#60858,
#60859,#60860,#60861,#60862,#60863,#60864,#60865,#60866,#60867,#60868,#60869,
#60870,#60871,#60872,#60873,#60874,#60875,#60876,#60877,#60878,#60879,#60880,
#60881,#60882,#60883,#60884,#60885,#60886,#60887,#60888,#60889,#60890,#60891,
#60892,#60893,#60894,#60895,#60896,#60897,#60898,#60899,#60900,#60901,#60902,
#60903,#60904,#60905,#60906,#60907,#60908,#60909,#60910,#60911,#60912,#60913,
#60914,#60915,#60916,#60917,#60918,#60919,#60920,#60921,#60922,#60923,#60924,
#60925,#60926,#60927,#60928,#60929,#60930,#60931,#60932,#60933,#60934,#60935,
#60936,#60937,#60938,#60939,#60940,#60941,#60942,#60943,#60944,#60945,#60946,
#60947,#60948,#60949,#60950,#60951,#60952,#60953,#60954,#60955,#60956,#60957,
#60958,#60959,#60960,#60961,#60962,#60963,#60964,#60965,#60966,#60967,#60968,
#60969,#60970,#60971,#60972,#60973,#60974,#60975,#60976,#60977,#60978,#60979,
#60980,#60981,#60982,#60983,#60984,#60985,#60986,#60987,#60988,#60989,#60990,
#60991,#60992,#60993,#60994,#60995,#60996,#60997,#60998,#60999,#61000,#61001,
#61002,#61003,#61004,#61005,#61006,#61007,#61008,#61009,#61010,#61011,#61012,
#61013,#61014,#61015,#61016,#61017,#61018,#61019,#61020,#61021,#61022,#61023,
#61024,#61025,#61026,#61027,#61028,#61029,#61030,#61031,#61032,#61033,#61034,
#61035,#61036,#61037,#61038,#61039,#61040,#61041,#61042,#61043,#61044,#61045,
#61046,#61047,#61048,#61049,#61050,#61051,#61052,#61053,#61054,#61055,#61056,
#61057,#61058,#61059,#61060,#61061,#61062,#61063,#61064,#61065,#61066,#61067,
#61068,#61069,#61070,#61071,#61072,#61073,#61074,#61075,#61076,#61077,#61078,
#61079,#61080,#61081,#61082,#61083,#61084,#61085,#61086,#61087,#61088,#61089,
#61090,#61091,#61092,#61093,#61094,#61095,#61096,#61097,#61098,#61099,#61100,
#61101,#61102,#61103,#61104,#61105,#61106,#61107,#61108,#61109,#61110,#61111,
#61112,#61113,#61114,#61115,#61116,#61117,#61118,#61119,#61120,#61121,#61122,
#61123,#61124,#61125,#61126,#61127,#61128,#61129,#61130,#61131,#61132,#61133,
#61134,#61135,#61136,#61137,#61138,#61139,#61140,#61141,#61142,#61143,#61144,
#61145,#61146,#61147,#61148,#61149,#61150,#61151,#61152,#61153,#61154,#61155,
#61156,#61157,#61158,#61159,#61160,#61161,#61162,#61163,#61164,#61165,#61166,
#61167,#61168,#61169,#61170,#61171,#61172,#61173,#61174,#61175,#61176,#61177,
#61178,#61179,#61180,#61181,#61182,#61183,#61184,#61185,#61186,#61187,#61188,
#61189,#61190,#61191,#61192,#61193,#61194,#61195,#61196,#61197,#61198,#61199,
#61200,#61201,#61202,#61203,#61204,#61205,#61206,#61207,#61208,#61209,#61210,
#61211,#61212,#61213,#61214,#61215,#61216,#61217,#61218,#61219,#61220,#61221,
#61222,#61223,#61224,#61225,#61226,#61227,#61228,#61229,#61230,#61231,#61232,
#61233,#61234,#61235,#61236,#61237,#61238,#61239,#61240,#61241,#61242,#61243,
#61244,#61245,#61246,#61247,#61248,#61249,#61250,#61251,#61252,#61253,#61254,
#61255,#61256,#61257,#61258,#61259,#61260,#61261,#61262,#61263,#61264,#61265,
#61266,#61267,#61268,#61269,#61270,#61271,#61272,#61273,#61274,#61275,#61276,
#61277,#61278,#61279,#61280,#61281,#61282,#61283,#61284,#61285,#61286,#61287,
#61288,#61289,#61290,#61291,#61292,#61293,#61294,#61295,#61296,#61297,#61298,
#61299,#61300,#61301,#61302,#61303,#61304,#61305,#61306,#61307,#61308,#61309,
#61310,#61311,#61312,#61313,#61314,#61315,#61316,#61317,#61318,#61319,#61320,
#61321,#61322,#61323,#61324,#61325,#61326,#61327,#61328,#61329,#61330,#61331,
#61332,#61333,#61334,#61335,#61336,#61337,#61338,#61339,#61340,#61341,#61342,
#61343,#61344,#61345,#61346,#61347,#61348),.UNSPECIFIED.,.F.,.F.,(4,2,2,
2,2,2,2,2,2,2,2,2,2,2,2,2,2,2,2,2,2,2,2,2,2,2,2,2,2,2,2,2,2,2,2,2,2,2,2,
2,2,2,2,2,2,2,2,2,2,2,2,2,2,2,2,2,2,2,2,2,2,2,2,2,2,2,2,2,2,2,2,2,2,2,2,
2,2,2,2,2,2,2,2,2,2,2,2,2,2,2,2,2,2,2,2,2,2,2,2,2,2,2,2,2,2,2,2,2,2,2,2,
2,2,2,2,2,2,2,2,2,2,2,2,2,2,2,2,2,2,2,2,2,2,2,2,2,2,2,2,2,2,2,2,2,2,2,2,
2,2,2,2,2,2,2,2,2,2,2,2,2,2,2,2,2,2,2,2,2,2,2,2,2,2,2,2,2,2,2,2,2,2,2,2,
2,2,2,2,2,2,2,2,2,2,2,2,2,2,2,2,2,2,2,2,2,2,2,2,2,2,2,2,2,2,2,2,2,2,2,2,
2,2,2,2,2,2,2,2,2,2,2,2,2,2,2,2,2,2,2,2,2,2,2,2,2,2,2,2,2,2,2,2,2,2,2,2,
2,2,2,2,2,2,2,2,4),(-4.06131869556804,-4.03569863910276,-3.9909247024884,
-3.97862060287754,-3.973641496883,-3.97109218908225,-3.96893113293521,-3.96761920361655,
-3.96643834324285,-3.96493513530557,-3.96198258332817,-3.94473755005551,
-3.94369087588502,-3.87455289302399,-3.85164534667204,-3.82177684670054,
-3.81190432096129,-3.80798881762499,-3.80712260526249,-3.8063135864326,
-3.8057211682998,-3.80507523640384,-3.80392809998666,-3.80052866251502,
-3.74387154325791,-3.70410143400313,-3.66646156166628,-3.65535791910726,
-3.64839952728795,-3.64685259361792,-3.6454022500706,-3.64433880479701,
-3.64319358507599,-3.641550383398,-3.63698869523099,-3.55865323911149,-3.51129861408268,
-3.49541932059155,-3.48603278702949,-3.48450035759345,-3.48369150845678,
-3.48309908098602,-3.48245300560784,-3.48150679816215,-3.47875578525753,
-3.42965437464634,-3.37622728375723,-3.35357150572134,-3.32804046310582,
-3.32463311606416,-3.32303905463316,-3.32184531422547,-3.3207282684827,
-3.31918958026955,-3.31528176495629,-3.25113314273419,-3.20099699126577,
-3.17419434676126,-3.16351302825318,-3.16193145578828,-3.16127139516624,
-3.16060330039048,-3.15998022934258,-3.15911810222608,-3.15691488123021,
-3.12656252666364,-3.06939784441054,-3.00888646940935,-3.0029096689483,
-3.00092262834493,-2.9996494589355,-2.99845704838277,-2.99689840610967,
-2.99347352437931,-2.9656665358806,-2.94232157084541,-2.87427741624493,
-2.84455319416342,-2.84168339304578,-2.83957264692708,-2.83866868810316,
-2.83799829410187,-2.83737847642198,-2.83652879637264,-2.83439820875131,
-2.80851542731251,-2.71928243170916,-2.68617904722715,-2.68021318597376,
-2.6782307809838,-2.67695868592617,-2.67576593709756,-2.6742049171214,-2.6715803005839,
-2.65565216358661,-2.65090332695905,-2.63438260868126,-2.54640469844639,
-2.52130847075577,-2.51738025194337,-2.51621407557219,-2.51549219709238,
-2.51482930559271,-2.5139673216949,-2.5121583817277,-2.49898586244086,-2.49843295858623,
-2.41253509376591,-2.36522158649048,-2.35777229496608,-2.35563691815514,
-2.35433068449459,-2.35314849971841,-2.35163468389678,-2.34852904358714,
-2.32896851302666,-2.32353606397736,-2.30467290179328,-2.23382782656863,
-2.20721949574438,-2.19550009001742,-2.19387771982011,-2.19305670131569,
-2.19240037749282,-2.19164677939242,-2.19037185099724,-2.18578950879352,
-2.08963527085972,-2.03864313074189,-2.0342141389977,-2.03246470567244,
-2.03124236597178,-2.03001660696279,-2.02825029438574,-2.02371415791498,
-1.96749169832077,-1.87657162270288,-1.87207513104574,-1.87079431379922,
-1.87004676870704,-1.86945538972021,-1.86865712709353,-1.86714376701672,
-1.85826747585291,-1.83930544008547,-1.79257604003289,-1.74409091328136,
-1.71458792360639,-1.711458113297,-1.70990678492543,-1.70878634788007,-1.70759436502605,
-1.70601184381665,-1.70255101001824,-1.63139273241994,-1.56370711464608,
-1.56214191974715,-1.55024054192167,-1.54846099971433,-1.54760831924798,
-1.54694865777873,-1.54621459971359,-1.54499428290201,-1.54053914613007,
-1.5094599330364,-1.42135597296793,-1.39180812308225,-1.38867715145079,
-1.38712554551831,-1.38600504733111,-1.38481312875505,-1.38323091301578,
-1.37988284870221,-1.36295648228376,-1.32075011352674,-1.2386392744335,
-1.22742267705983,-1.22567384535582,-1.22482721382252,-1.22416826974383,
-1.2234308096263,-1.22222010272727,-1.21786103246147,-1.18771586860836,
-1.11990263055763,-1.06969992951049,-1.06588229069133,-1.06435880953691,
-1.06324561824641,-1.06204920324017,-1.06043976576669,-1.05693302528263,
-1.05224560753613,-1.00859471534161,-0.942822426554163,-0.927204026504941,
-0.919086579621284,-0.918484199093398,-0.917698385617313,-0.904853502731454,
-0.903215209423113,-0.902378285369261,-0.901761688312629,-0.901088519373151,
-0.900419587839021,-0.898756233310041,-0.885450446991834,-0.86003378349266,
-0.810699060081097,-0.747164025227985,-0.743256605043414,-0.741717833837789,
-0.740600644362787,-0.739406672159888,-0.737812168563272,-0.734403362734202,
-0.708880510765015,-0.686224876365195,-0.632786461502381,-0.583596107392925,
-0.580842910186204,-0.57989628003352,-0.579250011864593,-0.578657482502376,
-0.577848608093183,-0.576316500275781,-0.56694299960962,-0.550478284461759,
-0.50358876610826,-0.425393255384568,-0.420832955564247,-0.419189778872074,
-0.418044431345235,-0.416980754281111,-0.415529921172911,-0.413982379816667,
-0.407018250335395,-0.395902507449545,-0.358182890253443,-0.318506204301113,
-0.261761201589244,-0.258355853819562,-0.257207716837274,-0.256561490603367,
-0.255968972722374,-0.255160073741072,-0.254294097540713,-0.250384052523628,
-0.240514951347302,-0.210607965309897,-0.187683494692836,-0.118658155605018,
-0.117613936309703,-0.100335826894927,-0.0973810513441103,-0.0958771694253617,
-0.0946960042762633,-0.0933839680649612,-0.091223268034337,-0.0886745600925323,
-0.0836973545416452,-0.0713997823159879,-0.0269275451426486,-0.00095762347367935),
 .UNSPECIFIED.);
#867=B_SPLINE_CURVE_WITH_KNOTS('',3,(#61350,#61351,#61352,#61353,#61354,
#61355,#61356,#61357,#61358,#61359,#61360,#61361,#61362,#61363,#61364,#61365,
#61366,#61367,#61368,#61369,#61370,#61371,#61372,#61373,#61374,#61375,#61376,
#61377,#61378,#61379,#61380,#61381,#61382,#61383,#61384,#61385,#61386,#61387,
#61388,#61389,#61390,#61391,#61392,#61393,#61394,#61395,#61396,#61397,#61398,
#61399,#61400,#61401,#61402,#61403,#61404,#61405,#61406,#61407,#61408,#61409,
#61410,#61411,#61412,#61413,#61414,#61415,#61416,#61417,#61418,#61419,#61420,
#61421,#61422,#61423,#61424,#61425,#61426,#61427,#61428,#61429,#61430,#61431,
#61432,#61433,#61434,#61435,#61436,#61437,#61438,#61439,#61440,#61441,#61442,
#61443,#61444,#61445,#61446,#61447,#61448,#61449,#61450,#61451,#61452,#61453,
#61454,#61455,#61456,#61457,#61458,#61459,#61460,#61461,#61462,#61463,#61464,
#61465,#61466,#61467,#61468,#61469,#61470,#61471,#61472,#61473,#61474,#61475,
#61476,#61477,#61478,#61479,#61480,#61481,#61482,#61483,#61484,#61485,#61486,
#61487,#61488,#61489,#61490,#61491,#61492,#61493,#61494,#61495,#61496,#61497,
#61498,#61499,#61500,#61501,#61502,#61503,#61504,#61505,#61506,#61507,#61508,
#61509,#61510,#61511,#61512,#61513,#61514,#61515,#61516,#61517,#61518,#61519,
#61520,#61521,#61522,#61523,#61524,#61525,#61526,#61527,#61528,#61529,#61530,
#61531,#61532,#61533,#61534,#61535,#61536,#61537,#61538,#61539,#61540,#61541,
#61542,#61543,#61544,#61545,#61546,#61547,#61548,#61549,#61550,#61551,#61552,
#61553,#61554,#61555,#61556,#61557,#61558,#61559,#61560,#61561,#61562,#61563,
#61564,#61565,#61566,#61567,#61568,#61569,#61570,#61571,#61572,#61573,#61574,
#61575,#61576,#61577,#61578,#61579,#61580,#61581,#61582,#61583,#61584,#61585,
#61586,#61587,#61588,#61589,#61590,#61591,#61592,#61593,#61594,#61595,#61596,
#61597,#61598,#61599,#61600,#61601,#61602,#61603,#61604,#61605,#61606,#61607,
#61608,#61609,#61610,#61611,#61612,#61613,#61614,#61615,#61616,#61617,#61618,
#61619,#61620,#61621,#61622,#61623,#61624,#61625,#61626,#61627,#61628,#61629,
#61630,#61631,#61632,#61633,#61634,#61635,#61636,#61637,#61638,#61639,#61640,
#61641,#61642,#61643,#61644,#61645,#61646,#61647,#61648,#61649,#61650,#61651,
#61652,#61653,#61654,#61655,#61656,#61657,#61658,#61659,#61660,#61661,#61662,
#61663,#61664,#61665,#61666,#61667,#61668,#61669,#61670,#61671,#61672,#61673,
#61674,#61675,#61676,#61677,#61678,#61679,#61680,#61681,#61682,#61683,#61684,
#61685,#61686,#61687,#61688,#61689,#61690,#61691,#61692,#61693,#61694,#61695,
#61696,#61697,#61698,#61699,#61700,#61701,#61702,#61703,#61704,#61705,#61706,
#61707,#61708,#61709,#61710,#61711,#61712,#61713,#61714,#61715,#61716,#61717,
#61718,#61719,#61720,#61721,#61722,#61723,#61724,#61725,#61726,#61727,#61728,
#61729,#61730,#61731,#61732,#61733,#61734,#61735,#61736,#61737,#61738,#61739,
#61740,#61741,#61742,#61743,#61744,#61745,#61746,#61747,#61748,#61749,#61750,
#61751,#61752,#61753,#61754,#61755,#61756,#61757,#61758,#61759,#61760,#61761,
#61762,#61763,#61764,#61765,#61766,#61767,#61768,#61769,#61770,#61771,#61772,
#61773,#61774,#61775,#61776,#61777,#61778,#61779,#61780,#61781,#61782,#61783,
#61784,#61785,#61786,#61787,#61788,#61789,#61790,#61791,#61792,#61793,#61794,
#61795,#61796,#61797,#61798,#61799,#61800,#61801,#61802,#61803,#61804,#61805,
#61806,#61807,#61808,#61809,#61810,#61811,#61812,#61813,#61814,#61815,#61816,
#61817,#61818,#61819,#61820,#61821,#61822,#61823,#61824,#61825,#61826,#61827,
#61828,#61829,#61830,#61831,#61832,#61833,#61834,#61835,#61836,#61837,#61838,
#61839,#61840,#61841,#61842,#61843,#61844,#61845,#61846,#61847,#61848,#61849,
#61850,#61851,#61852,#61853,#61854,#61855,#61856,#61857,#61858,#61859,#61860,
#61861,#61862,#61863,#61864,#61865,#61866,#61867,#61868,#61869,#61870,#61871,
#61872,#61873,#61874,#61875,#61876,#61877,#61878,#61879,#61880,#61881,#61882,
#61883,#61884,#61885,#61886,#61887,#61888,#61889,#61890,#61891,#61892,#61893,
#61894,#61895,#61896,#61897,#61898,#61899,#61900,#61901),.UNSPECIFIED.,
 .F.,.F.,(4,2,2,2,2,2,2,2,2,2,2,2,2,2,2,2,2,2,2,2,2,2,2,2,2,2,2,2,2,2,2,
2,2,2,2,2,2,2,2,2,2,2,2,2,2,2,2,2,2,2,2,2,2,2,2,2,2,2,2,2,2,2,2,2,2,2,2,
2,2,2,2,2,2,2,2,2,2,2,2,2,2,2,2,2,2,2,2,2,2,2,2,2,2,2,2,2,2,2,2,2,2,2,2,
2,2,2,2,2,2,2,2,2,2,2,2,2,2,2,2,2,2,2,2,2,2,2,2,2,2,2,2,2,2,2,2,2,2,2,2,
2,2,2,2,2,2,2,2,2,2,2,2,2,2,2,2,2,2,2,2,2,2,2,2,2,2,2,2,2,2,2,2,2,2,2,2,
2,2,2,2,2,2,2,2,2,2,2,2,2,2,2,2,2,2,2,2,2,2,2,2,2,2,2,2,2,2,2,2,2,2,2,2,
2,2,2,2,2,2,2,2,2,2,2,2,2,2,2,2,2,2,2,2,2,2,2,2,2,2,2,2,2,2,2,2,2,2,2,2,
2,2,2,2,2,2,2,2,2,2,2,2,2,2,2,2,2,2,2,2,2,2,2,2,2,2,2,2,4),(-4.06102915371521,
-4.00733943593029,-3.99716016596606,-3.99580480695467,-3.9949504102,-3.99414983477194,
-3.99355820236957,-3.99290768106946,-3.99173817561084,-3.98817165157536,
-3.92742560176029,-3.91252780523285,-3.89796188468783,-3.85798693922934,
-3.83963195849921,-3.83675661705982,-3.83503605346045,-3.83346015784654,
-3.83226914759206,-3.83114666528226,-3.82927915338896,-3.82446627265448,
-3.74513178642116,-3.71783312479859,-3.68573795207312,-3.67788349767447,
-3.67329525877463,-3.67238693041042,-3.67171643459974,-3.6710423505235,
-3.67042677706451,-3.6695938991768,-3.66797136173466,-3.65555775000817,
-3.65478127186798,-3.60932695647417,-3.55482133755643,-3.52125899810746,
-3.51366418584821,-3.51207661153792,-3.51059682767539,-3.50952929691238,
-3.50839607940177,-3.50679730927733,-3.50252253148154,-3.42955600199011,
-3.37623725490668,-3.36171349326885,-3.35120957181207,-3.34963419436093,
-3.34897469493649,-3.34830683990842,-3.34768304398592,-3.34681849411808,
-3.34460158712089,-3.31329412359299,-3.27159898642495,-3.19311887365023,
-3.1896576357764,-3.18805774882761,-3.18686288646319,-3.1857471352634,-3.18421390120989,
-3.18033922854664,-3.12402869754315,-3.06717190593994,-3.0413120806648,
-3.02860448202687,-3.02695778801249,-3.02612484009397,-3.02552923419839,
-3.02489370774551,-3.02379911704159,-3.02077236884465,-2.96695184145353,
-2.87382065025079,-2.86777086006729,-2.86577850808278,-2.86450408299875,
-2.86331201277833,-2.86175598994524,-2.85834565283953,-2.83100062857812,
-2.81409668608624,-2.73591224284481,-2.70905607729515,-2.7049804435879,
-2.70380107809911,-2.70307078825265,-2.7024102228172,-2.70156471264444,
-2.699775066108,-2.68764002322005,-2.68628112875578,-2.68356662075688,-2.67876007285917,
-2.67005486353434,-2.60470557591073,-2.57260116358125,-2.54951353833579,
-2.54470263240534,-2.54289407771874,-2.54165938086559,-2.54045836217543,
-2.53902115730969,-2.53548352684915,-2.5038804613039,-2.48656745162599,
-2.42374609865796,-2.38369548820815,-2.38168407973732,-2.38078747672822,
-2.38012144642017,-2.37949469195182,-2.37861896810163,-2.37682659522316,
-2.35894580044785,-2.35851693795969,-2.31478670737558,-2.27807710143261,
-2.23026019743436,-2.22276401309483,-2.22062352250683,-2.21931596729519,
-2.21813376532547,-2.21662156067946,-2.21352496520746,-2.19416770114435,
-2.18895088245867,-2.17548222963585,-2.09869525847194,-2.0644668122392,
-2.06136488515132,-2.0591179788927,-2.05817983692009,-2.05750646693748,
-2.05688998557783,-2.05605364868231,-2.05441778292071,-2.04164300068632,
-2.03886444312354,-2.03841120256686,-2.03740178355526,-2.03327875330647,
-2.03144781779701,-2.00920037979788,-1.9056413164506,-1.90449912440638,
-1.8994322961333,-1.89752424492679,-1.89639391422296,-1.89532543022547,
-1.8938384848014,-1.89086681759855,-1.86756711302524,-1.84771271482242,
-1.79800189317953,-1.74013642267774,-1.73996109416646,-1.73672493907313,
-1.7356006519438,-1.73495922546185,-1.7343655292388,-1.73354659020148,-1.73193456287823,
-1.72053491817359,-1.69049906955036,-1.5959482742005,-1.59496663003824,
-1.5785799831447,-1.57593138994919,-1.5743632675347,-1.57316925249797,-1.57189981823352,
-1.569929773153,-1.56393669682915,-1.53082049102495,-1.43808197957827,-1.4362701610064,
-1.43172475487711,-1.42893888336086,-1.42849726943842,-1.42689683370545,
-1.41503509845552,-1.41325728642984,-1.41240494518431,-1.41174532502459,
-1.41101108030882,-1.40978993211521,-1.40532620399357,-1.37414189396467,
-1.29584050206474,-1.2569814159065,-1.25334532376706,-1.25185339619462,
-1.25074829256064,-1.24957056019521,-1.24797587704692,-1.24620158559183,
-1.24319612859928,-1.1916146639028,-1.0960804660733,-1.09141450991743,-1.090130584307,
-1.08937475840956,-1.08871846896896,-1.08790003546813,-1.08629085912563,
-1.0749825197842,-1.04538691813522,-0.948932539611661,-0.932865072291202,
-0.930232730238419,-0.928669245188569,-0.927475857842218,-0.926229968492027,
-0.924317611371169,-0.922093497209466,-0.917965782788841,-0.908409746899213,
-0.879290315483234,-0.829577782899801,-0.771700054523462,-0.771161052022005,
-0.768204747292225,-0.767121546425524,-0.766488275933347,-0.765891822122101,
-0.765053067584421,-0.76334382578701,-0.748440415181851,-0.720937547816619,
-0.629287628851472,-0.624755913173499,-0.609992243447726,-0.607430427895019,
-0.60588779909447,-0.604697861919676,-0.60344344125612,-0.601565883206071,
-0.599337367352461,-0.59519824348891,-0.585606370726419,-0.556399448175455,
-0.506617238973183,-0.449017904541551,-0.445606806245524,-0.444457853245045,
-0.44381147346478,-0.443219008642684,-0.442410471143043,-0.440848484764004,
-0.430829263660783,-0.407359071390185,-0.365989160381794,-0.315908814486658,
-0.288281557522388,-0.284861984073732,-0.283304186065663,-0.282111768643872,
-0.281011157685621,-0.279209870485887,-0.274435765373547,-0.26755916794571,
-0.248512933410093,-0.229473094424572,-0.151451708380495,-0.124658018962657,
-0.122510880889271,-0.121658270280633,-0.121037610923996,-0.120367614628153,
-0.119447880578009,-0.117307428956169,-0.0834569910630557,-0.000958237941546336),
 .UNSPECIFIED.);
#868=B_SPLINE_CURVE_WITH_KNOTS('',3,(#61903,#61904,#61905,#61906,#61907,
#61908,#61909,#61910,#61911,#61912),.UNSPECIFIED.,.F.,.F.,(4,1,1,1,1,1,
1,4),(204.203522483337,204.830447189148,205.829239592916,206.828031996684,
207.826824400452,208.82561680422,209.824409207988,210.486707790517),
 .UNSPECIFIED.);
#869=B_SPLINE_CURVE_WITH_KNOTS('',3,(#61914,#61915,#61916,#61917,#61918,
#61919,#61920,#61921,#61922,#61923,#61924,#61925,#61926,#61927,#61928,#61929,
#61930,#61931,#61932,#61933,#61934,#61935,#61936,#61937,#61938,#61939,#61940,
#61941,#61942,#61943,#61944,#61945,#61946,#61947,#61948,#61949,#61950,#61951,
#61952,#61953,#61954,#61955,#61956,#61957,#61958,#61959,#61960,#61961,#61962,
#61963,#61964,#61965,#61966,#61967,#61968,#61969,#61970,#61971,#61972,#61973,
#61974,#61975,#61976,#61977,#61978,#61979,#61980,#61981,#61982,#61983,#61984,
#61985,#61986,#61987,#61988,#61989,#61990,#61991,#61992,#61993,#61994,#61995,
#61996,#61997,#61998,#61999,#62000,#62001,#62002,#62003,#62004,#62005,#62006,
#62007,#62008,#62009,#62010,#62011,#62012,#62013,#62014,#62015,#62016,#62017,
#62018,#62019,#62020,#62021,#62022,#62023,#62024,#62025,#62026,#62027,#62028,
#62029,#62030,#62031,#62032,#62033,#62034,#62035,#62036,#62037,#62038,#62039,
#62040,#62041,#62042,#62043,#62044,#62045,#62046,#62047,#62048,#62049,#62050,
#62051,#62052,#62053,#62054,#62055,#62056,#62057,#62058,#62059,#62060,#62061,
#62062,#62063,#62064,#62065,#62066,#62067,#62068,#62069,#62070,#62071,#62072,
#62073,#62074,#62075,#62076,#62077,#62078,#62079,#62080,#62081,#62082,#62083,
#62084,#62085,#62086,#62087,#62088,#62089,#62090,#62091,#62092,#62093,#62094,
#62095,#62096,#62097,#62098,#62099,#62100,#62101,#62102,#62103,#62104,#62105,
#62106,#62107,#62108,#62109,#62110,#62111,#62112,#62113,#62114,#62115,#62116,
#62117,#62118,#62119,#62120,#62121,#62122,#62123,#62124,#62125,#62126,#62127,
#62128,#62129,#62130,#62131,#62132,#62133,#62134,#62135,#62136,#62137,#62138,
#62139,#62140,#62141,#62142,#62143,#62144,#62145,#62146,#62147,#62148,#62149,
#62150,#62151,#62152,#62153,#62154,#62155,#62156,#62157,#62158,#62159,#62160,
#62161,#62162,#62163,#62164,#62165,#62166,#62167,#62168,#62169,#62170,#62171,
#62172,#62173,#62174,#62175,#62176,#62177,#62178,#62179,#62180,#62181,#62182,
#62183,#62184,#62185,#62186,#62187,#62188,#62189,#62190,#62191,#62192,#62193,
#62194,#62195,#62196,#62197,#62198,#62199,#62200,#62201,#62202,#62203,#62204,
#62205,#62206,#62207,#62208,#62209,#62210,#62211,#62212,#62213,#62214,#62215,
#62216,#62217,#62218,#62219,#62220,#62221,#62222,#62223,#62224,#62225,#62226,
#62227,#62228,#62229,#62230,#62231,#62232,#62233,#62234,#62235,#62236,#62237,
#62238,#62239,#62240,#62241,#62242,#62243,#62244,#62245,#62246,#62247,#62248,
#62249,#62250,#62251,#62252,#62253,#62254,#62255,#62256,#62257,#62258,#62259,
#62260,#62261,#62262,#62263,#62264,#62265,#62266,#62267,#62268,#62269,#62270,
#62271,#62272,#62273,#62274,#62275,#62276,#62277,#62278,#62279,#62280,#62281,
#62282,#62283,#62284,#62285,#62286,#62287,#62288,#62289,#62290,#62291,#62292,
#62293,#62294,#62295,#62296,#62297,#62298,#62299,#62300,#62301,#62302,#62303,
#62304,#62305,#62306,#62307,#62308,#62309,#62310,#62311,#62312,#62313,#62314,
#62315,#62316,#62317,#62318,#62319,#62320,#62321,#62322,#62323,#62324,#62325,
#62326,#62327,#62328,#62329,#62330,#62331,#62332,#62333,#62334,#62335,#62336,
#62337,#62338,#62339,#62340,#62341,#62342,#62343,#62344,#62345,#62346,#62347,
#62348,#62349,#62350,#62351,#62352,#62353,#62354,#62355,#62356,#62357,#62358,
#62359,#62360,#62361,#62362,#62363,#62364,#62365,#62366,#62367,#62368,#62369,
#62370,#62371,#62372,#62373,#62374,#62375,#62376,#62377,#62378,#62379,#62380,
#62381,#62382,#62383,#62384,#62385,#62386,#62387,#62388,#62389,#62390,#62391,
#62392,#62393,#62394,#62395,#62396,#62397,#62398,#62399,#62400,#62401,#62402,
#62403,#62404,#62405,#62406,#62407,#62408,#62409,#62410,#62411,#62412,#62413,
#62414,#62415,#62416,#62417,#62418,#62419,#62420,#62421,#62422,#62423,#62424,
#62425,#62426,#62427,#62428,#62429,#62430,#62431,#62432,#62433,#62434,#62435,
#62436,#62437,#62438,#62439,#62440,#62441,#62442,#62443,#62444,#62445,#62446,
#62447,#62448,#62449,#62450,#62451,#62452,#62453,#62454,#62455,#62456,#62457,
#62458,#62459,#62460,#62461,#62462,#62463),.UNSPECIFIED.,.F.,.F.,(4,2,2,
2,2,2,2,2,2,2,2,2,2,2,2,2,2,2,2,2,2,2,2,2,2,2,2,2,2,2,2,2,2,2,2,2,2,2,2,
2,2,2,2,2,2,2,2,2,2,2,2,2,2,2,2,2,2,2,2,2,2,2,2,2,2,2,2,2,2,2,2,2,2,2,2,
2,2,2,2,2,2,2,2,2,2,2,2,2,2,2,2,2,2,2,2,2,2,2,2,2,2,2,2,2,2,2,2,2,2,2,2,
2,2,2,2,2,2,2,2,2,2,2,2,2,2,2,2,2,2,2,2,2,2,2,2,2,2,2,2,2,2,2,2,2,2,2,2,
2,2,2,2,2,2,2,2,2,2,2,2,2,2,2,2,2,2,2,2,2,2,2,2,2,2,2,2,2,2,2,2,2,2,2,2,
2,2,2,2,2,2,2,2,2,2,2,2,2,2,2,2,2,2,2,2,2,2,2,2,2,2,2,2,2,2,2,2,2,2,2,2,
2,2,2,2,2,2,2,2,2,2,2,2,2,2,2,2,2,2,2,2,2,2,2,2,2,2,2,2,2,2,2,2,2,2,2,2,
2,2,2,2,2,2,2,2,2,2,2,2,2,2,2,2,2,2,2,4),(-4.06049657891224,-3.98971205792811,
-3.96625604543254,-3.95483641893174,-3.95322370018519,-3.95240461080479,
-3.95175437644203,-3.95100143850387,-3.94972957284891,-3.94517701314423,
-3.84881143108739,-3.82766435633166,-3.79657451171058,-3.79316968208567,
-3.79192248935369,-3.79082197477453,-3.78962905374788,-3.78806764794247,
-3.78462816818222,-3.75636230042786,-3.74444863908848,-3.70251564154461,
-3.66436601142297,-3.6356582212257,-3.63284459407056,-3.63076550651394,
-3.62985675190409,-3.62918876984315,-3.6285654962427,-3.6277026290837,-3.62549510167175,
-3.59484061183983,-3.54261933495207,-3.50827714133197,-3.48855632216326,
-3.47824711353032,-3.4738802481785,-3.47056799467337,-3.46901652871813,
-3.46789493764059,-3.46678739537104,-3.46528563748001,-3.46235105681029,
-3.43920151261024,-3.42885175141428,-3.3496950636264,-3.3105005101393,-3.30822261330623,
-3.30727930826882,-3.30660503795583,-3.30598975707241,-3.30515793335222,
-3.3035393818741,-3.29123108981414,-3.20103188379539,-3.16650419057776,
-3.15575920909221,-3.15125607801153,-3.14888699257951,-3.14693917976173,
-3.14565534873104,-3.14447397626,-3.14296736835865,-3.13999944075464,-3.12246577289303,
-3.02299541359719,-2.99055402879725,-2.98598993881807,-2.98475916396203,
-2.98402274399093,-2.98336356084332,-2.98251503926993,-2.98075672743739,
-2.96933412776831,-2.87666251348363,-2.83321092591174,-2.82853559650572,
-2.82610078466645,-2.82404533456081,-2.82276522441222,-2.82158294491178,
-2.82006938032845,-2.81696556698497,-2.79745014349672,-2.79203852421539,
-2.77325061675747,-2.70223777430702,-2.67560264228216,-2.66391184551348,
-2.66229023919452,-2.66146931637408,-2.66081892501236,-2.66006727329548,
-2.65880091497487,-2.65429990751109,-2.55755637135215,-2.51081588477976,
-2.50341956840764,-2.50128959481028,-2.49998452362602,-2.49880198704553,
-2.49728576892938,-2.49416830593207,-2.47435509144533,-2.46884712381461,
-2.45592709430216,-2.37938272439594,-2.3451672256626,-2.34206615059194,
-2.33981980719672,-2.33888184857659,-2.33820859136882,-2.33759219959382,
-2.33675596467168,-2.33512024044937,-2.32234425885274,-2.31956925691279,
-2.31922798582844,-2.26071001490321,-2.18295413425186,-2.17948170413756,
-2.17789705401794,-2.17670477615157,-2.17558501850019,-2.17403614659422,
-2.17091599780379,-2.14176647354427,-2.12969103856988,-2.05681360748445,
-2.03037373286562,-2.01865824001209,-2.01688695171465,-2.01603592856054,
-2.01537650911459,-2.0146416243322,-2.01341747238458,-2.00892195781575,
-1.97734432841322,-1.89425190193827,-1.88289619612652,-1.85993098471858,
-1.85700321945561,-1.85550322624516,-1.85439614563031,-1.85319567339058,
-1.85156195369865,-1.84782074366267,-1.84279759363904,-1.81711854060672,
-1.77387153635517,-1.71013265430017,-1.70973583963201,-1.70904989344843,
-1.69607010992939,-1.69442716024068,-1.69358909100762,-1.6929722491954,
-1.69229943142584,-1.69136371791093,-1.68913041767247,-1.68605210125461,
-1.65231053568945,-1.61779096137798,-1.53939364852726,-1.53475049940659,
-1.53309496739072,-1.53194628043425,-1.53088361488174,-1.52944042066184,
-1.52667963041437,-1.50963100387274,-1.4712083935111,-1.38536091296174,
-1.37328446361084,-1.37149736185187,-1.37065235190876,-1.36999186518111,
-1.36926132743611,-1.36805668545317,-1.3638526398519,-1.33555526487758,
-1.24927803481731,-1.21504113622242,-1.21143406220145,-1.20998545731942,
-1.20878156113753,-1.2075507053953,-1.20579605508432,-1.20132456283697,
-1.14679701555565,-1.08506050590719,-1.07539727748638,-1.07203844495038,
-1.06514349730385,-1.06352564073989,-1.05062481200013,-1.04898461878447,
-1.04814724378296,-1.04753056705026,-1.04685757210219,-1.04592098544587,
-1.04375031904111,-1.0407455760875,-1.00847699734796,-0.9422377587332,-0.941400112120224,
-0.925726967205936,-0.915296816215335,-0.909685975295693,-0.908606304480574,
-0.891454919976999,-0.888506986584862,-0.887004626773872,-0.885823696792347,
-0.884510930295395,-0.882389979490946,-0.875039506142504,-0.86311575095035,
-0.818097840061453,-0.775445501820224,-0.729381807882283,-0.726650853413126,
-0.725707491712472,-0.725062177231477,-0.724469501574668,-0.723658901347221,
-0.722118480586721,-0.712512260016122,-0.694379890664134,-0.633906409190096,
-0.570322814450785,-0.566415723232065,-0.564877101131939,-0.563760026732863,
-0.562566183907004,-0.560971864090938,-0.557550342704471,-0.523826241750137,
-0.473709151203545,-0.407891756969277,-0.404252083875212,-0.403073094854276,
-0.402420672121827,-0.401829388378052,-0.401032328587121,-0.400182836402296,
-0.396518897683616,-0.390677591280717,-0.371780069704382,-0.343698357389322,
-0.316739747637345,-0.285973126794533,-0.282585089649083,-0.247212079072741,
-0.243940513122593,-0.242353981159195,-0.241224101376784,-0.240155374211044,
-0.238667022523693,-0.237067556795919,-0.234482650685707,-0.216375519981168,
-0.182169082583788,-0.169702923985518,-0.156297498125755,-0.0981423875346418,
-0.0829063260632253,-0.0809981108166153,-0.0801301315670966,-0.0794662546876113,
-0.0787470322045957,-0.0775929299122855,-0.0762385391647315,-0.0662546035110392,
-0.000957508011488563),.UNSPECIFIED.);
#870=B_SPLINE_CURVE_WITH_KNOTS('',3,(#62465,#62466,#62467,#62468,#62469,
#62470,#62471,#62472,#62473,#62474,#62475,#62476,#62477,#62478,#62479,#62480,
#62481,#62482,#62483,#62484,#62485,#62486,#62487,#62488,#62489,#62490,#62491,
#62492,#62493,#62494,#62495,#62496,#62497,#62498,#62499,#62500,#62501,#62502,
#62503,#62504,#62505,#62506,#62507,#62508,#62509,#62510,#62511,#62512,#62513,
#62514,#62515,#62516,#62517,#62518,#62519,#62520,#62521,#62522,#62523,#62524,
#62525,#62526,#62527,#62528,#62529,#62530,#62531,#62532,#62533,#62534,#62535,
#62536,#62537,#62538,#62539,#62540,#62541,#62542,#62543,#62544,#62545,#62546,
#62547,#62548,#62549,#62550,#62551,#62552,#62553,#62554,#62555,#62556,#62557,
#62558,#62559,#62560,#62561,#62562,#62563,#62564,#62565,#62566,#62567,#62568,
#62569,#62570,#62571,#62572,#62573,#62574,#62575,#62576,#62577,#62578,#62579,
#62580,#62581,#62582,#62583,#62584,#62585,#62586,#62587,#62588,#62589,#62590,
#62591,#62592,#62593,#62594,#62595,#62596,#62597,#62598,#62599,#62600,#62601,
#62602,#62603,#62604,#62605,#62606,#62607,#62608,#62609,#62610,#62611,#62612,
#62613,#62614,#62615,#62616,#62617,#62618,#62619,#62620,#62621,#62622,#62623,
#62624,#62625,#62626,#62627,#62628,#62629,#62630,#62631,#62632,#62633,#62634,
#62635,#62636,#62637,#62638,#62639,#62640,#62641,#62642,#62643,#62644,#62645,
#62646,#62647,#62648,#62649,#62650,#62651,#62652,#62653,#62654,#62655,#62656,
#62657,#62658,#62659,#62660,#62661,#62662,#62663,#62664,#62665,#62666,#62667,
#62668,#62669,#62670,#62671,#62672,#62673,#62674,#62675,#62676,#62677,#62678,
#62679,#62680,#62681,#62682,#62683,#62684,#62685,#62686,#62687,#62688,#62689,
#62690,#62691,#62692,#62693,#62694,#62695,#62696,#62697,#62698,#62699,#62700,
#62701,#62702,#62703,#62704,#62705,#62706,#62707,#62708,#62709,#62710,#62711,
#62712,#62713,#62714,#62715,#62716,#62717,#62718,#62719,#62720,#62721,#62722,
#62723,#62724,#62725,#62726,#62727,#62728,#62729,#62730,#62731,#62732,#62733,
#62734,#62735,#62736,#62737,#62738,#62739,#62740,#62741,#62742,#62743,#62744,
#62745,#62746,#62747,#62748,#62749,#62750,#62751,#62752,#62753,#62754,#62755,
#62756,#62757,#62758,#62759,#62760,#62761,#62762,#62763,#62764,#62765,#62766,
#62767,#62768,#62769,#62770,#62771,#62772,#62773,#62774,#62775,#62776,#62777,
#62778,#62779,#62780,#62781,#62782,#62783,#62784,#62785,#62786,#62787,#62788,
#62789,#62790,#62791,#62792,#62793,#62794,#62795,#62796,#62797,#62798,#62799,
#62800,#62801,#62802,#62803,#62804,#62805,#62806,#62807,#62808,#62809,#62810,
#62811,#62812,#62813,#62814,#62815,#62816,#62817,#62818,#62819,#62820,#62821,
#62822,#62823,#62824,#62825,#62826,#62827,#62828,#62829,#62830,#62831,#62832,
#62833,#62834,#62835,#62836,#62837,#62838,#62839,#62840,#62841,#62842,#62843,
#62844,#62845,#62846,#62847,#62848,#62849,#62850,#62851,#62852,#62853,#62854,
#62855,#62856,#62857,#62858,#62859,#62860,#62861,#62862,#62863,#62864,#62865,
#62866,#62867,#62868,#62869,#62870,#62871,#62872,#62873,#62874,#62875,#62876,
#62877,#62878,#62879,#62880,#62881,#62882,#62883,#62884,#62885,#62886,#62887,
#62888,#62889,#62890,#62891,#62892,#62893,#62894,#62895,#62896,#62897,#62898,
#62899,#62900,#62901,#62902,#62903,#62904,#62905,#62906,#62907,#62908,#62909,
#62910,#62911,#62912,#62913,#62914,#62915,#62916,#62917,#62918,#62919,#62920,
#62921,#62922,#62923,#62924,#62925,#62926,#62927,#62928,#62929,#62930,#62931,
#62932,#62933,#62934,#62935,#62936,#62937,#62938,#62939,#62940,#62941,#62942,
#62943,#62944,#62945,#62946,#62947,#62948,#62949,#62950,#62951,#62952,#62953,
#62954,#62955,#62956,#62957,#62958,#62959,#62960,#62961,#62962,#62963,#62964,
#62965,#62966,#62967,#62968,#62969,#62970,#62971,#62972,#62973,#62974,#62975,
#62976,#62977,#62978,#62979,#62980,#62981,#62982,#62983,#62984,#62985,#62986,
#62987,#62988,#62989,#62990,#62991,#62992,#62993,#62994,#62995,#62996),
 .UNSPECIFIED.,.F.,.F.,(4,2,2,2,2,2,2,2,2,2,2,2,2,2,2,2,2,2,2,2,2,2,2,2,
2,2,2,2,2,2,2,2,2,2,2,2,2,2,2,2,2,2,2,2,2,2,2,2,2,2,2,2,2,2,2,2,2,2,2,2,
2,2,2,2,2,2,2,2,2,2,2,2,2,2,2,2,2,2,2,2,2,2,2,2,2,2,2,2,2,2,2,2,2,2,2,2,
2,2,2,2,2,2,2,2,2,2,2,2,2,2,2,2,2,2,2,2,2,2,2,2,2,2,2,2,2,2,2,2,2,2,2,2,
2,2,2,2,2,2,2,2,2,2,2,2,2,2,2,2,2,2,2,2,2,2,2,2,2,2,2,2,2,2,2,2,2,2,2,2,
2,2,2,2,2,2,2,2,2,2,2,2,2,2,2,2,2,2,2,2,2,2,2,2,2,2,2,2,2,2,2,2,2,2,2,2,
2,2,2,2,2,2,2,2,2,2,2,2,2,2,2,2,2,2,2,2,2,2,2,2,2,2,2,2,2,2,2,2,2,2,2,2,
2,2,2,2,2,2,2,2,2,2,2,2,2,2,2,2,2,2,2,2,2,2,2,2,2,4),(-4.06151371944992,
-3.98512772967926,-3.98259757323507,-3.98102106276342,-3.97954928378014,
-3.97848288548137,-3.97734652293743,-3.97573612284057,-3.97138910350108,
-3.89794537359405,-3.88348754773806,-3.86993036953823,-3.83605836290238,
-3.82096867995507,-3.81953415603881,-3.81864665669649,-3.81782229926178,
-3.81717159195894,-3.81651855312469,-3.81533662561074,-3.81167493976928,
-3.74443235264209,-3.70806150464538,-3.67883633606832,-3.66713263832581,
-3.65988550560989,-3.65831945020771,-3.65685522166278,-3.65578982277248,
-3.65465030490257,-3.65302839201582,-3.64860746349398,-3.58004365421,-3.52975879651499,
-3.50097983344832,-3.49682941166829,-3.49594779392835,-3.49512765855346,
-3.49453377962682,-3.49389282570049,-3.49277103518101,-3.48955353550529,
-3.43112016523926,-3.38181983635296,-3.36197267371988,-3.33938729313599,
-3.33599700736088,-3.33440605332477,-3.33321262385723,-3.33209440201768,
-3.3305517840918,-3.32662173070605,-3.26610327247955,-3.19997768644188,
-3.1827970314216,-3.17478830020052,-3.17323279859951,-3.17241891013092,
-3.17182577239953,-3.17118187832659,-3.17024380923783,-3.16754983918248,
-3.12502988638493,-3.06921765356264,-3.02194919054577,-3.01704106414756,
-3.01340077806828,-3.01176660624983,-3.01056585285235,-3.00945854786686,
-3.00795830378961,-3.00503019691679,-2.98206764730743,-2.96740115683939,
-2.89860465057851,-2.87601356231537,-2.85283235039043,-2.8508450987227,
-2.84992370337539,-2.84925338686956,-2.84863308923869,-2.84778194261741,
-2.8456435003422,-2.81934656432651,-2.74530862085288,-2.69911020929803,
-2.69426584937583,-2.69065771016551,-2.68903300826618,-2.68783391781903,
-2.68672439773346,-2.68521541659526,-2.68148237467049,-2.63733823261918,
-2.60715733754165,-2.55333643021045,-2.53893405303632,-2.52936702454637,
-2.52782326621996,-2.52701850628826,-2.52636310908942,-2.52569743251024,
-2.52445297841195,-2.52028083215,-2.4176797366519,-2.37147597069743,-2.36782265180503,
-2.36620466940427,-2.36500685952995,-2.36389590594072,-2.36238094571682,
-2.35861264328418,-2.31206555053525,-2.28669448063043,-2.24030580974222,
-2.2166598042577,-2.20661172753485,-2.20504866077235,-2.20423992187869,
-2.20364746147161,-2.203001236692,-2.20185294651217,-2.19844621702278,-2.14086705997772,
-2.09113097900259,-2.06192773154901,-2.04730029167468,-2.04465002230972,
-2.04323024984365,-2.04217001209396,-2.04084049672412,-2.0386014520073,
-2.03107154402968,-2.00528069771464,-1.9618158144137,-1.88738490256459,
-1.88336335739162,-1.88213670630677,-1.88147464932939,-1.88081897229186,
-1.88000827713126,-1.87843602751664,-1.86815282362126,-1.84325958684407,
-1.76344045258801,-1.75053923520712,-1.74506547906303,-1.7253518505943,
-1.7222388183663,-1.72072342160264,-1.71954092035503,-1.71823527210264,
-1.71610296578969,-1.70868502493469,-1.66170449585513,-1.60873048778164,
-1.56306618116939,-1.56032773237834,-1.55938326581525,-1.55873762789598,
-1.55814500055396,-1.55733498271432,-1.55576590239949,-1.54556441064946,
-1.52108085455418,-1.43728854171577,-1.4255493091801,-1.40286543265996,
-1.39994794362398,-1.39845057231878,-1.39734413242912,-1.39614310346215,
-1.39450639054982,-1.39074855873075,-1.30813586907975,-1.25149220788208,
-1.24963054633628,-1.23879017245977,-1.23705885398049,-1.23621572310077,
-1.23555720283631,-1.23483267260556,-1.23362942733197,-1.23218596063727,
-1.22933614284275,-1.19998323530304,-1.13593269534862,-1.0811690989687,
-1.07730704232857,-1.07577601865248,-1.07466089641787,-1.07346578476392,
-1.07186396755439,-1.06829927604034,-1.01937261360948,-0.943968968419398,
-0.916784754200208,-0.914630825293692,-0.913777075686765,-0.913156135410346,
-0.912486388015048,-0.911586393908492,-0.909635882158193,-0.906963362616315,
-0.90037239370779,-0.877396017037223,-0.829282053511521,-0.78429203997342,
-0.776324157434589,-0.757221241323316,-0.754136664865288,-0.752626856172148,
-0.75144493837064,-0.750136070607724,-0.747989731015974,-0.740436351969627,
-0.714901060391101,-0.672615355651724,-0.628293906667524,-0.618465867825959,
-0.614601332848636,-0.609743060308636,-0.60836457801826,-0.593725152995518,
-0.592025549668843,-0.591173008688977,-0.590552381900024,-0.589882402487084,
-0.589219044505901,-0.587607504730847,-0.576051348864818,-0.563162145589931,
-0.522875005716314,-0.452613780709759,-0.451496070038381,-0.43441463991666,
-0.431470271181607,-0.429968606292793,-0.428787672356814,-0.427474332769528,
-0.425307895873875,-0.417554179171333,-0.366824468445903,-0.342463153414464,
-0.316259115670658,-0.272343795696258,-0.269608474124362,-0.268664442477199,
-0.268018914218223,-0.267426237621165,-0.266795281734187,-0.26600197410379,
-0.263093698105171,-0.230492159776364,-0.209351413165981,-0.133776513955677,
-0.131677902535982,-0.111966237724981,-0.10885325950652,-0.107337858498801,
-0.106155340078874,-0.104849658754597,-0.102717266555907,-0.0952987163971223,
-0.048312173861197,-0.000957996441563316),.UNSPECIFIED.);
#871=B_SPLINE_CURVE_WITH_KNOTS('',3,(#62998,#62999,#63000,#63001,#63002,
#63003,#63004,#63005,#63006,#63007,#63008,#63009,#63010,#63011,#63012,#63013,
#63014,#63015,#63016,#63017,#63018,#63019,#63020,#63021,#63022,#63023,#63024,
#63025,#63026,#63027,#63028,#63029,#63030,#63031,#63032,#63033,#63034,#63035,
#63036,#63037,#63038,#63039,#63040,#63041,#63042,#63043,#63044,#63045,#63046,
#63047,#63048,#63049,#63050,#63051,#63052,#63053,#63054,#63055,#63056,#63057,
#63058,#63059,#63060,#63061,#63062,#63063,#63064,#63065,#63066,#63067,#63068,
#63069,#63070,#63071,#63072,#63073,#63074,#63075,#63076,#63077,#63078,#63079,
#63080,#63081,#63082,#63083,#63084,#63085,#63086,#63087,#63088,#63089,#63090,
#63091,#63092,#63093,#63094,#63095,#63096,#63097,#63098,#63099,#63100,#63101,
#63102,#63103,#63104,#63105,#63106,#63107,#63108,#63109,#63110,#63111,#63112,
#63113,#63114,#63115,#63116,#63117,#63118,#63119,#63120,#63121,#63122,#63123,
#63124,#63125,#63126,#63127,#63128,#63129,#63130,#63131,#63132,#63133,#63134,
#63135,#63136,#63137,#63138,#63139,#63140,#63141,#63142,#63143,#63144,#63145,
#63146,#63147,#63148,#63149,#63150,#63151,#63152,#63153,#63154,#63155,#63156,
#63157,#63158,#63159,#63160,#63161,#63162,#63163,#63164,#63165,#63166,#63167,
#63168,#63169,#63170,#63171,#63172,#63173,#63174,#63175,#63176,#63177,#63178,
#63179,#63180,#63181,#63182,#63183,#63184,#63185,#63186,#63187,#63188,#63189,
#63190,#63191,#63192,#63193,#63194,#63195,#63196,#63197,#63198,#63199,#63200,
#63201,#63202,#63203,#63204,#63205,#63206,#63207,#63208,#63209,#63210,#63211,
#63212,#63213,#63214,#63215,#63216,#63217,#63218,#63219,#63220,#63221,#63222,
#63223,#63224,#63225,#63226,#63227,#63228,#63229,#63230,#63231,#63232,#63233,
#63234,#63235,#63236,#63237,#63238,#63239,#63240,#63241,#63242,#63243,#63244,
#63245,#63246,#63247,#63248,#63249,#63250,#63251,#63252,#63253,#63254,#63255,
#63256,#63257,#63258,#63259,#63260,#63261,#63262,#63263,#63264,#63265,#63266,
#63267,#63268,#63269,#63270,#63271,#63272,#63273,#63274,#63275,#63276,#63277,
#63278,#63279,#63280,#63281,#63282,#63283,#63284,#63285,#63286,#63287,#63288,
#63289,#63290,#63291,#63292,#63293,#63294,#63295,#63296,#63297,#63298,#63299,
#63300,#63301,#63302,#63303,#63304,#63305,#63306,#63307,#63308,#63309,#63310,
#63311,#63312,#63313,#63314,#63315,#63316,#63317,#63318,#63319,#63320,#63321,
#63322,#63323,#63324,#63325,#63326,#63327,#63328,#63329,#63330,#63331,#63332,
#63333,#63334,#63335,#63336,#63337,#63338,#63339,#63340,#63341,#63342,#63343,
#63344,#63345,#63346,#63347,#63348,#63349,#63350,#63351,#63352,#63353,#63354,
#63355,#63356,#63357,#63358,#63359,#63360,#63361,#63362,#63363,#63364,#63365,
#63366,#63367,#63368,#63369,#63370,#63371,#63372,#63373,#63374,#63375,#63376,
#63377,#63378,#63379,#63380,#63381,#63382,#63383,#63384,#63385,#63386,#63387,
#63388,#63389,#63390,#63391,#63392,#63393,#63394,#63395,#63396,#63397,#63398,
#63399,#63400,#63401,#63402,#63403,#63404,#63405,#63406,#63407,#63408,#63409,
#63410,#63411,#63412,#63413,#63414,#63415,#63416,#63417,#63418,#63419,#63420,
#63421,#63422,#63423,#63424,#63425,#63426,#63427,#63428,#63429,#63430,#63431,
#63432,#63433,#63434,#63435,#63436,#63437,#63438,#63439,#63440,#63441,#63442,
#63443,#63444,#63445,#63446,#63447,#63448,#63449,#63450,#63451,#63452,#63453,
#63454,#63455,#63456,#63457,#63458,#63459,#63460,#63461,#63462,#63463,#63464,
#63465,#63466,#63467,#63468,#63469,#63470,#63471,#63472,#63473,#63474,#63475,
#63476,#63477,#63478,#63479,#63480,#63481,#63482,#63483,#63484,#63485,#63486,
#63487,#63488,#63489,#63490,#63491,#63492,#63493,#63494,#63495,#63496,#63497,
#63498,#63499,#63500,#63501,#63502,#63503,#63504,#63505,#63506,#63507,#63508,
#63509,#63510,#63511,#63512,#63513,#63514,#63515,#63516,#63517,#63518,#63519,
#63520,#63521,#63522,#63523,#63524,#63525,#63526,#63527,#63528,#63529),
 .UNSPECIFIED.,.F.,.F.,(4,2,2,2,2,2,2,2,2,2,2,2,2,2,2,2,2,2,2,2,2,2,2,2,
2,2,2,2,2,2,2,2,2,2,2,2,2,2,2,2,2,2,2,2,2,2,2,2,2,2,2,2,2,2,2,2,2,2,2,2,
2,2,2,2,2,2,2,2,2,2,2,2,2,2,2,2,2,2,2,2,2,2,2,2,2,2,2,2,2,2,2,2,2,2,2,2,
2,2,2,2,2,2,2,2,2,2,2,2,2,2,2,2,2,2,2,2,2,2,2,2,2,2,2,2,2,2,2,2,2,2,2,2,
2,2,2,2,2,2,2,2,2,2,2,2,2,2,2,2,2,2,2,2,2,2,2,2,2,2,2,2,2,2,2,2,2,2,2,2,
2,2,2,2,2,2,2,2,2,2,2,2,2,2,2,2,2,2,2,2,2,2,2,2,2,2,2,2,2,2,2,2,2,2,2,2,
2,2,2,2,2,2,2,2,2,2,2,2,2,2,2,2,2,2,2,2,2,2,2,2,2,2,2,2,2,2,2,2,2,2,2,2,
2,2,2,2,2,2,2,2,2,2,2,2,2,2,2,2,2,2,2,2,2,2,2,2,2,4),(-4.05932996479639,
-4.00703982614242,-4.00563635672431,-4.00476205512462,-4.00410446570224,
-4.00343791005599,-4.00281349106476,-4.00194531211603,-4.00018194533193,
-3.98334890264101,-3.97717005467382,-3.96452440677062,-3.94885813133185,
-3.93917667015674,-3.93067217108731,-3.91372058995674,-3.86700643780568,
-3.84888488142342,-3.84512283213122,-3.84348601181196,-3.84228556881662,
-3.84118013424965,-3.83968482992644,-3.83677343411346,-3.81421717048654,
-3.7448386342237,-3.71946790158547,-3.69429661730345,-3.68743692680702,
-3.68329543363733,-3.68241453214386,-3.68175451860975,-3.68108663303139,
-3.68046422333629,-3.67960370664482,-3.67740823265023,-3.64752124479994,
-3.62358499529834,-3.54363701481488,-3.52575002923593,-3.52244444515951,
-3.52089206562346,-3.5197053325659,-3.518576781307,-3.51667495397654,-3.51164241961022,
-3.43101402734289,-3.3833267904943,-3.36853178856557,-3.3637154724233,-3.36055970608928,
-3.35948786740035,-3.35887336566448,-3.35821371367795,-3.35737196586634,
-3.35559983403549,-3.34384623511312,-3.34216037694053,-3.33987442472209,
-3.31806982684442,-3.2567797742728,-3.23260411217912,-3.20351352799144,
-3.20006783564887,-3.1984887786853,-3.19729797129602,-3.1961775853651,-3.19462465320913,
-3.19062858379612,-3.1255126203354,-3.07076593674566,-3.04257219390286,
-3.03978816080786,-3.03774392632649,-3.03684310929708,-3.03617358557071,
-3.03555347672019,-3.0347017888063,-3.03255783649128,-3.00587177076776,
-2.91961628152862,-2.88471028454306,-2.8785204599378,-2.87652693090985,
-2.87525284681774,-2.87406186657044,-2.87250837019673,-2.86910801587083,
-2.84201495880432,-2.82863283523943,-2.75956901914329,-2.71822665751334,
-2.71638673408371,-2.71492263703646,-2.71413901188669,-2.71354783552038,
-2.71280228181256,-2.7115290054986,-2.70709647026816,-2.62509949603952,
-2.55897030408486,-2.55520132234405,-2.55356332929277,-2.55236273374501,
-2.5512576547487,-2.54976358350078,-2.5468567941117,-2.52442209582214,-2.42991088108071,
-2.39472555220532,-2.39264219885133,-2.39173297694854,-2.39106519613794,
-2.39044251849916,-2.38958108590613,-2.38738042625372,-2.35714166928091,
-2.31807715787911,-2.27996889340665,-2.2357947233799,-2.23248214006755,
-2.23092828926107,-2.22974121118285,-2.2286129170372,-2.22671293677503,
-2.22169306693046,-2.22048316405023,-2.1165075637908,-2.07238023472366,
-2.07012748202891,-2.06918867542096,-2.06851547433938,-2.06789961569855,
-2.06706479296895,-2.06543386796836,-2.05277593847135,-2.0522653880507,
-2.04923681714071,-2.04422863701577,-2.04117262619971,-2.03108909889942,
-1.96173427887808,-1.94283109231867,-1.91339387453022,-1.91026685162819,
-1.90871655690413,-1.90759670367404,-1.90640519080956,-1.90482303626466,
-1.90136197853318,-1.82948368626787,-1.75250924151542,-1.74821170334011,
-1.74695323335772,-1.74628492799194,-1.74563631421854,-1.74483947506058,
-1.74333211891183,-1.73457834702299,-1.71585620321083,-1.67078418641421,
-1.59263607492646,-1.5879148235483,-1.58624794881998,-1.58509631753747,
-1.58403474176386,-1.5825987844117,-1.57987104296965,-1.56358086213379,
-1.52950955754347,-1.4368886148485,-1.42632976694317,-1.42461269646842,
-1.42377253323136,-1.42311448054266,-1.42237357930586,-1.42112211651503,
-1.41633117323276,-1.38085949954155,-1.28632861348975,-1.28164732181547,
-1.26700715675596,-1.26445289308245,-1.26291276883899,-1.26172354668411,
-1.2604685750393,-1.25866846685609,-1.25648906401622,-1.25247510317897,
-1.21892622159933,-1.1245112041976,-1.12119813395443,-1.10395819216122,
-1.10198623560193,-1.1011066286737,-1.10044096875315,-1.09972701367949,
-1.09859604350529,-1.09497895173494,-1.07311070175187,-1.04867700039954,
-1.00948764941425,-0.94608805912035,-0.942181673646234,-0.940643291526206,
-0.939526378121796,-0.938358169899059,-0.936813034429958,-0.935105563345423,
-0.9322614742094,-0.926482301456736,-0.835552549137356,-0.790903601742188,
-0.78085098166428,-0.779159189046723,-0.778324030107459,-0.777666420327303,
-0.776922257893027,-0.775656496547922,-0.770705761192523,-0.747332565313931,
-0.696882939047241,-0.667674657542121,-0.623166883433151,-0.619428536663269,
-0.617918801550849,-0.616809227325592,-0.615634522203932,-0.614058427383091,
-0.612309915683628,-0.609366856694525,-0.603313429467553,-0.587290614074345,
-0.567986456094639,-0.518152993509329,-0.460742313680543,-0.457316669132169,
-0.456165675239484,-0.455518912550233,-0.454926581013473,-0.454118946596125,
-0.452561117978147,-0.4426447448664,-0.419858258998069,-0.374874099501909,
-0.350830450129026,-0.300214648501835,-0.297004049647198,-0.295432608608637,
-0.29430682899995,-0.293173060519748,-0.291670417036584,-0.288596339061355,
-0.284616940313561,-0.275520234167969,-0.248733762062387,-0.144802768233036,
-0.1354406663,-0.133806334307815,-0.132971565735155,-0.132313828212072,
-0.131569049363713,-0.130301129756311,-0.125328418052534,-0.101900466247598,
-0.000958141822577317),.UNSPECIFIED.);
#872=B_SPLINE_CURVE_WITH_KNOTS('',3,(#63531,#63532,#63533,#63534,#63535,
#63536,#63537,#63538,#63539,#63540,#63541,#63542,#63543,#63544,#63545,#63546,
#63547,#63548,#63549,#63550,#63551,#63552,#63553,#63554,#63555,#63556,#63557,
#63558,#63559,#63560,#63561,#63562,#63563,#63564,#63565,#63566,#63567,#63568,
#63569,#63570,#63571,#63572,#63573,#63574,#63575,#63576,#63577,#63578,#63579,
#63580,#63581,#63582,#63583,#63584,#63585,#63586,#63587,#63588,#63589,#63590,
#63591,#63592,#63593,#63594,#63595,#63596,#63597,#63598,#63599,#63600,#63601,
#63602,#63603,#63604,#63605,#63606,#63607,#63608,#63609,#63610,#63611,#63612,
#63613,#63614,#63615,#63616,#63617,#63618,#63619,#63620,#63621,#63622,#63623,
#63624,#63625,#63626,#63627,#63628,#63629,#63630,#63631,#63632,#63633,#63634,
#63635,#63636,#63637,#63638,#63639,#63640,#63641,#63642,#63643,#63644,#63645,
#63646,#63647,#63648),.UNSPECIFIED.,.F.,.F.,(4,3,3,3,3,3,3,3,3,3,3,3,3,
3,3,3,3,3,3,3,3,3,3,3,3,3,3,3,3,3,3,3,3,3,3,3,3,3,3,4),(248.185819633594,
248.353498579193,248.521277971523,248.689527055698,248.77731295494,248.9427757676,
249.107922054166,249.274967880302,249.440034186732,249.60806977272,249.776105358708,
249.941568171368,250.106714457934,250.27376028407,250.4388265905,250.606862176488,
250.774897762476,250.940360575136,251.105506861702,251.272552687838,251.437618994268,
251.605654580256,251.773690166244,251.939152978904,252.10429926547,252.271345091606,
252.436411398036,252.604446984024,252.772482570012,252.937945382672,253.103091669238,
253.270137495374,253.435203801804,253.603239387792,253.77127497378,253.935826065977,
254.100044847577,254.264077257094,254.428142795537,254.469004940774),
 .UNSPECIFIED.);
#873=B_SPLINE_CURVE_WITH_KNOTS('',3,(#63650,#63651,#63652,#63653,#63654,
#63655,#63656,#63657,#63658,#63659,#63660,#63661,#63662,#63663,#63664,#63665,
#63666,#63667,#63668,#63669,#63670,#63671,#63672,#63673,#63674,#63675,#63676,
#63677,#63678,#63679,#63680,#63681,#63682,#63683,#63684,#63685,#63686,#63687,
#63688,#63689,#63690,#63691,#63692,#63693,#63694,#63695,#63696,#63697,#63698,
#63699,#63700,#63701,#63702,#63703,#63704,#63705,#63706,#63707,#63708,#63709,
#63710,#63711,#63712,#63713,#63714,#63715,#63716,#63717,#63718,#63719,#63720,
#63721,#63722,#63723,#63724,#63725,#63726,#63727,#63728,#63729,#63730,#63731,
#63732,#63733,#63734,#63735,#63736,#63737,#63738,#63739,#63740,#63741,#63742,
#63743,#63744,#63745,#63746,#63747,#63748,#63749,#63750,#63751,#63752,#63753,
#63754,#63755,#63756,#63757,#63758,#63759,#63760,#63761,#63762,#63763,#63764,
#63765,#63766,#63767,#63768,#63769,#63770,#63771,#63772,#63773,#63774,#63775,
#63776,#63777,#63778,#63779,#63780,#63781,#63782,#63783,#63784,#63785,#63786,
#63787,#63788,#63789,#63790,#63791,#63792,#63793,#63794,#63795,#63796,#63797,
#63798,#63799,#63800,#63801,#63802,#63803,#63804,#63805,#63806,#63807,#63808,
#63809,#63810,#63811,#63812,#63813,#63814,#63815,#63816,#63817,#63818,#63819,
#63820,#63821,#63822,#63823,#63824,#63825,#63826,#63827,#63828,#63829,#63830,
#63831,#63832,#63833,#63834,#63835,#63836,#63837,#63838,#63839,#63840,#63841,
#63842,#63843,#63844,#63845,#63846,#63847,#63848,#63849,#63850,#63851,#63852,
#63853,#63854,#63855,#63856,#63857,#63858,#63859,#63860,#63861,#63862,#63863,
#63864,#63865,#63866,#63867,#63868,#63869,#63870,#63871,#63872,#63873,#63874,
#63875,#63876,#63877,#63878,#63879,#63880,#63881,#63882,#63883,#63884,#63885,
#63886,#63887,#63888,#63889,#63890,#63891,#63892,#63893,#63894,#63895,#63896,
#63897,#63898,#63899,#63900,#63901,#63902,#63903,#63904,#63905,#63906,#63907,
#63908,#63909,#63910,#63911,#63912,#63913,#63914,#63915,#63916,#63917,#63918,
#63919,#63920,#63921,#63922,#63923,#63924,#63925,#63926,#63927,#63928,#63929,
#63930,#63931,#63932,#63933,#63934,#63935,#63936,#63937,#63938,#63939,#63940,
#63941,#63942,#63943,#63944,#63945,#63946,#63947,#63948,#63949,#63950,#63951,
#63952,#63953,#63954,#63955,#63956,#63957,#63958,#63959,#63960,#63961,#63962,
#63963,#63964,#63965,#63966,#63967,#63968,#63969,#63970,#63971,#63972,#63973,
#63974,#63975,#63976,#63977,#63978,#63979,#63980,#63981,#63982,#63983,#63984,
#63985,#63986,#63987,#63988,#63989,#63990,#63991,#63992,#63993,#63994,#63995,
#63996,#63997,#63998,#63999,#64000,#64001,#64002,#64003,#64004,#64005,#64006,
#64007,#64008,#64009,#64010,#64011,#64012,#64013,#64014,#64015,#64016,#64017,
#64018,#64019,#64020,#64021,#64022,#64023,#64024,#64025,#64026,#64027,#64028,
#64029,#64030,#64031,#64032,#64033,#64034,#64035,#64036,#64037,#64038,#64039,
#64040,#64041,#64042,#64043,#64044,#64045,#64046,#64047,#64048,#64049,#64050,
#64051,#64052,#64053,#64054,#64055,#64056,#64057,#64058,#64059,#64060,#64061,
#64062,#64063,#64064,#64065,#64066,#64067,#64068,#64069,#64070,#64071,#64072,
#64073,#64074,#64075,#64076,#64077,#64078,#64079,#64080,#64081,#64082,#64083,
#64084,#64085,#64086,#64087,#64088,#64089,#64090,#64091,#64092,#64093,#64094,
#64095,#64096,#64097,#64098,#64099,#64100,#64101,#64102,#64103,#64104,#64105,
#64106,#64107,#64108,#64109,#64110,#64111,#64112,#64113,#64114,#64115,#64116,
#64117,#64118,#64119,#64120,#64121,#64122,#64123,#64124,#64125,#64126,#64127,
#64128,#64129,#64130,#64131,#64132,#64133,#64134,#64135,#64136,#64137,#64138,
#64139,#64140,#64141,#64142,#64143,#64144,#64145,#64146,#64147,#64148,#64149,
#64150,#64151,#64152,#64153,#64154,#64155,#64156,#64157,#64158,#64159,#64160,
#64161,#64162,#64163,#64164,#64165,#64166,#64167,#64168,#64169,#64170,#64171,
#64172,#64173,#64174,#64175),.UNSPECIFIED.,.F.,.F.,(4,2,2,2,2,2,2,2,2,2,
2,2,2,2,2,2,2,2,2,2,2,2,2,2,2,2,2,2,2,2,2,2,2,2,2,2,2,2,2,2,2,2,2,2,2,2,
2,2,2,2,2,2,2,2,2,2,2,2,2,2,2,2,2,2,2,2,2,2,2,2,2,2,2,2,2,2,2,2,2,2,2,2,
2,2,2,2,2,2,2,2,2,2,2,2,2,2,2,2,2,2,2,2,2,2,2,2,2,2,2,2,2,2,2,2,2,2,2,2,
2,2,2,2,2,2,2,2,2,2,2,2,2,2,2,2,2,2,2,2,2,2,2,2,2,2,2,2,2,2,2,2,2,2,2,2,
2,2,2,2,2,2,2,2,2,2,2,2,2,2,2,2,2,2,2,2,2,2,2,2,2,2,2,2,2,2,2,2,2,2,2,2,
2,2,2,2,2,2,2,2,2,2,2,2,2,2,2,2,2,2,2,2,2,2,2,2,2,2,2,2,2,2,2,2,2,2,2,2,
2,2,2,2,2,2,2,2,2,2,2,2,2,2,2,2,2,2,2,2,2,2,2,2,2,2,2,2,2,2,2,2,2,2,2,2,
4),(-4.06003765655308,-4.00423323853758,-3.9775885287128,-3.96592804501213,
-3.96430790737641,-3.96348747859677,-3.96283135961083,-3.96207770015301,
-3.9608019878455,-3.95621022710372,-3.86881393128048,-3.84672550835414,
-3.81256410512827,-3.80551531040521,-3.80396309607576,-3.80278850837579,
-3.80159301238478,-3.8004797286445,-3.79895464865576,-3.79512537359173,
-3.74366120825391,-3.70737379642536,-3.67097216501958,-3.65204456085692,
-3.6431898036797,-3.641677865137,-3.64088009303478,-3.64023149272111,-3.63956388833052,
-3.63830872623847,-3.63403976594128,-3.55922856444301,-3.52535529128013,
-3.50307352407948,-3.48431666131623,-3.48148792495554,-3.4803091431868,
-3.47911136883844,-3.47800156490333,-3.47648989053705,-3.47273849798057,
-3.42731063642589,-3.35677709939312,-3.32467510535317,-3.32013882191028,
-3.31891106924827,-3.3181755486514,-3.31751656887546,-3.31666749097112,
-3.31490513377514,-3.30337968200422,-3.26168742496592,-3.17085396910647,
-3.16431232364196,-3.15972055188708,-3.15795023183699,-3.15671643151351,
-3.15551586057287,-3.15407868472972,-3.1505385252423,-3.1187928567134,-3.03616188309034,
-2.99915565177217,-2.99688171779778,-2.99593930368405,-2.99526539983568,
-2.99465025836384,-2.99381834563154,-2.99219880649293,-2.97985150458162,
-2.95135294555784,-2.89169905793147,-2.84177160305828,-2.8386478302614,
-2.83612795362345,-2.8347420099736,-2.83368260110756,-2.83251980208,-2.83044709474672,
-2.82424815698305,-2.71192978605101,-2.67933551979252,-2.6747599490895,
-2.67352829696475,-2.67279179983287,-2.67213284323163,-2.67128501445439,
-2.66952955211513,-2.65816254402649,-2.65472269592798,-2.64805313184364,
-2.64466083950641,-2.5533927976318,-2.520640056549,-2.51468736079452,-2.5127225879152,
-2.51145445534932,-2.51026016356363,-2.50868949525341,-2.50603174446617,
-2.4894615691651,-2.39450738704549,-2.36756162523348,-2.35366808946732,
-2.35138621218681,-2.35044231620384,-2.34976800368468,-2.34915295815784,
-2.34832184192608,-2.34670580799768,-2.33446057106395,-2.2937078594994,
-2.24108978181261,-2.21934384448944,-2.19646360760062,-2.19167904642637,
-2.18987462004845,-2.18864092952215,-2.18743948903697,-2.18600010460584,
-2.18258400239798,-2.15361988057456,-2.08468387265484,-2.03065533724721,
-2.02885595946918,-2.02797856515932,-2.02735141510452,-2.02668574155726,
-2.02579090960959,-2.02378879854155,-1.96663009573278,-1.92865181113395,
-1.87266012022273,-1.86878835266972,-1.86725572573166,-1.86614022545783,
-1.8649454521817,-1.86334537567978,-1.85978985331268,-1.80752926875823,
-1.72232565715337,-1.71954689995726,-1.70761040629583,-1.7058293196915,
-1.70497633006638,-1.70431662365299,-1.70358271973112,-1.70236311598163,
-1.697915440332,-1.66692755409178,-1.59256917397857,-1.59133912298184,-1.57289532837151,
-1.56778615902482,-1.54862850687657,-1.54554145412597,-1.54403120387796,
-1.54284929285635,-1.54154079352943,-1.5393958795344,-1.53185568931526,
-1.50634800179568,-1.46349892424954,-1.38832031359065,-1.38402637410402,
-1.3827679654152,-1.38209948606301,-1.38145057325746,-1.3806531816044,-1.37914423188577,
-1.37053478152417,-1.35211878308866,-1.3268524956792,-1.23015706199185,
-1.22403187801211,-1.22196871244141,-1.22080754026395,-1.21974736891938,
-1.21835718618358,-1.21582252395606,-1.2126746980832,-1.19071019677127,
-1.17314264993399,-1.10852564953798,-1.06358363181037,-1.06083841929929,
-1.05989296892876,-1.05924705087823,-1.05865447947678,-1.057845005684,-1.05627855329976,
-1.04634157642698,-1.02332687356086,-0.944432269165112,-0.930660698989446,
-0.903632101823023,-0.900232004006861,-0.898677890553498,-0.897486130474042,
-0.896210913164362,-0.894254873758918,-0.888340314457047,-0.879329905375872,
-0.852017773563202,-0.801380849424833,-0.753755829162131,-0.753199119556926,
-0.752463250163929,-0.739552052868511,-0.73791148369758,-0.737074009902193,
-0.736457305675226,-0.735784327476104,-0.734847846166601,-0.732610158506311,
-0.729524249635282,-0.72150488685021,-0.686512005705855,-0.631860928771763,
-0.581750218193201,-0.57793509965139,-0.576412093885637,-0.575299062142194,
-0.574102640533274,-0.572926744583817,-0.570379919166202,-0.555869492164762,
-0.526818612471642,-0.49140153106653,-0.432889805969842,-0.432522067889638,
-0.430036324468666,-0.418478404806516,-0.415616991911007,-0.41454843570457,
-0.41391809443866,-0.41332050927828,-0.412474021156023,-0.410725749948347,
-0.399194352705144,-0.367404137958462,-0.343231570135268,-0.3162103712397,
-0.259244935838322,-0.255365884115638,-0.253831950644351,-0.252716052891383,
-0.251521374489583,-0.250348749371768,-0.24880276565047,-0.241855192666256,
-0.203240702388004,-0.179565560509696,-0.104341712672523,-0.0941031145889821,
-0.0924018679918587,-0.0915647213533804,-0.090906809568289,-0.0901636703847361,
-0.0889028445459993,-0.0873917716374819,-0.0843575726311591,-0.00095786616459987),
 .UNSPECIFIED.);
#874=B_SPLINE_CURVE_WITH_KNOTS('',3,(#64177,#64178,#64179,#64180,#64181,
#64182,#64183,#64184,#64185,#64186,#64187,#64188,#64189,#64190,#64191,#64192,
#64193,#64194,#64195,#64196,#64197,#64198,#64199,#64200,#64201,#64202,#64203,
#64204,#64205,#64206,#64207,#64208,#64209,#64210,#64211,#64212,#64213,#64214,
#64215,#64216,#64217,#64218,#64219,#64220,#64221,#64222,#64223,#64224,#64225,
#64226,#64227,#64228,#64229,#64230,#64231,#64232,#64233,#64234,#64235,#64236,
#64237,#64238,#64239,#64240,#64241,#64242,#64243,#64244,#64245,#64246,#64247,
#64248,#64249,#64250,#64251,#64252,#64253,#64254,#64255,#64256,#64257,#64258,
#64259,#64260,#64261,#64262,#64263,#64264,#64265,#64266,#64267,#64268,#64269,
#64270,#64271,#64272,#64273,#64274,#64275,#64276,#64277,#64278,#64279,#64280,
#64281,#64282,#64283,#64284,#64285,#64286,#64287,#64288,#64289,#64290,#64291,
#64292,#64293,#64294,#64295,#64296,#64297,#64298,#64299,#64300,#64301,#64302,
#64303,#64304,#64305,#64306,#64307,#64308,#64309,#64310,#64311,#64312,#64313,
#64314,#64315,#64316,#64317,#64318,#64319,#64320,#64321,#64322,#64323,#64324,
#64325,#64326,#64327,#64328,#64329,#64330,#64331,#64332,#64333,#64334,#64335,
#64336,#64337,#64338,#64339,#64340,#64341,#64342,#64343,#64344,#64345,#64346,
#64347,#64348,#64349,#64350,#64351,#64352,#64353,#64354,#64355,#64356,#64357,
#64358,#64359,#64360,#64361,#64362,#64363,#64364,#64365,#64366,#64367,#64368,
#64369,#64370,#64371,#64372,#64373,#64374,#64375,#64376,#64377,#64378,#64379,
#64380,#64381,#64382,#64383,#64384,#64385,#64386,#64387,#64388,#64389,#64390,
#64391,#64392,#64393,#64394,#64395,#64396,#64397,#64398,#64399,#64400,#64401,
#64402,#64403,#64404,#64405,#64406,#64407,#64408,#64409,#64410,#64411,#64412,
#64413,#64414,#64415,#64416,#64417,#64418,#64419,#64420,#64421,#64422,#64423,
#64424,#64425,#64426,#64427,#64428,#64429,#64430,#64431,#64432,#64433,#64434,
#64435,#64436,#64437,#64438,#64439,#64440,#64441,#64442,#64443,#64444,#64445,
#64446,#64447,#64448,#64449,#64450,#64451,#64452,#64453,#64454,#64455,#64456,
#64457,#64458,#64459,#64460,#64461,#64462,#64463,#64464,#64465,#64466,#64467,
#64468,#64469,#64470,#64471,#64472,#64473,#64474,#64475,#64476,#64477,#64478,
#64479,#64480,#64481,#64482,#64483,#64484,#64485,#64486,#64487,#64488,#64489,
#64490,#64491,#64492,#64493,#64494,#64495,#64496,#64497,#64498,#64499,#64500,
#64501,#64502,#64503,#64504,#64505,#64506,#64507,#64508,#64509,#64510,#64511,
#64512,#64513,#64514,#64515,#64516,#64517,#64518,#64519,#64520,#64521,#64522,
#64523,#64524,#64525,#64526,#64527,#64528,#64529,#64530,#64531,#64532,#64533,
#64534,#64535,#64536,#64537,#64538,#64539,#64540,#64541,#64542,#64543,#64544,
#64545,#64546,#64547,#64548,#64549,#64550,#64551,#64552,#64553,#64554,#64555,
#64556,#64557,#64558,#64559,#64560,#64561,#64562,#64563,#64564,#64565,#64566,
#64567,#64568,#64569,#64570,#64571,#64572,#64573,#64574,#64575,#64576,#64577,
#64578,#64579,#64580,#64581,#64582,#64583,#64584,#64585,#64586,#64587,#64588,
#64589,#64590,#64591,#64592,#64593,#64594,#64595,#64596,#64597,#64598,#64599,
#64600,#64601,#64602,#64603,#64604,#64605,#64606,#64607,#64608,#64609,#64610,
#64611,#64612,#64613,#64614,#64615,#64616,#64617,#64618,#64619,#64620,#64621,
#64622,#64623,#64624,#64625,#64626,#64627,#64628,#64629,#64630,#64631,#64632,
#64633,#64634,#64635,#64636,#64637,#64638,#64639,#64640,#64641,#64642,#64643,
#64644,#64645,#64646,#64647,#64648,#64649,#64650,#64651,#64652,#64653,#64654,
#64655,#64656,#64657,#64658,#64659,#64660,#64661,#64662,#64663,#64664,#64665,
#64666,#64667,#64668,#64669,#64670,#64671,#64672,#64673,#64674,#64675,#64676,
#64677,#64678,#64679,#64680,#64681,#64682,#64683,#64684,#64685,#64686,#64687,
#64688,#64689,#64690,#64691,#64692,#64693,#64694,#64695,#64696,#64697,#64698,
#64699,#64700,#64701,#64702,#64703,#64704),.UNSPECIFIED.,.F.,.F.,(4,2,2,
2,2,2,2,2,2,2,2,2,2,2,2,2,2,2,2,2,2,2,2,2,2,2,2,2,2,2,2,2,2,2,2,2,2,2,2,
2,2,2,2,2,2,2,2,2,2,2,2,2,2,2,2,2,2,2,2,2,2,2,2,2,2,2,2,2,2,2,2,2,2,2,2,
2,2,2,2,2,2,2,2,2,2,2,2,2,2,2,2,2,2,2,2,2,2,2,2,2,2,2,2,2,2,2,2,2,2,2,2,
2,2,2,2,2,2,2,2,2,2,2,2,2,2,2,2,2,2,2,2,2,2,2,2,2,2,2,2,2,2,2,2,2,2,2,2,
2,2,2,2,2,2,2,2,2,2,2,2,2,2,2,2,2,2,2,2,2,2,2,2,2,2,2,2,2,2,2,2,2,2,2,2,
2,2,2,2,2,2,2,2,2,2,2,2,2,2,2,2,2,2,2,2,2,2,2,2,2,2,2,2,2,2,2,2,2,2,2,2,
2,2,2,2,2,2,2,2,2,2,2,2,2,2,2,2,2,2,2,2,2,2,2,2,2,2,2,2,2,2,2,2,2,2,2,2,
2,2,2,2,2,2,2,2,4),(-4.06038590671169,-3.99533115978584,-3.99288451615544,
-3.99134341032541,-3.99017287297142,-3.98897961717822,-3.98786307860057,
-3.98632517332637,-3.98241979227162,-3.91886260821685,-3.90119545165806,
-3.88452875331077,-3.83915093933452,-3.83058095787481,-3.82907456383882,
-3.82827802040948,-3.82762953684154,-3.82696126726956,-3.82570257818847,
-3.8214018101828,-3.74614728588927,-3.7208503082374,-3.68832738513958,-3.67731598887521,
-3.67040291837945,-3.66885943099757,-3.6676880530777,-3.66649435788101,
-3.6653785945957,-3.66384361784815,-3.65995547818127,-3.60116494648335,
-3.54620435551938,-3.51955836072467,-3.50826639038863,-3.50665127275837,
-3.50583196500646,-3.50517603930975,-3.50451941198775,-3.50331848235849,
-3.49950404823833,-3.43357947647393,-3.38879027493756,-3.36453950423955,
-3.34903401280407,-3.34635056778719,-3.34518393980045,-3.34399273117545,
-3.34287257243987,-3.34132091578194,-3.33818820688385,-3.30853087914805,
-3.28787768837631,-3.21719027501515,-3.19547295422153,-3.18571897675306,
-3.18414377748797,-3.18333272647675,-3.182740235025,-3.18209563033733,-3.18115416285461,
-3.1784344875749,-3.13022316242323,-3.07845876830885,-3.03278772268032,
-3.02797645367114,-3.0243916887075,-3.02279012163587,-3.021589922032,-3.02048357087056,
-3.01898529309025,-3.01606300887088,-2.99322330893292,-2.98170133891302,
-2.89951413922132,-2.88897140780225,-2.86612785263719,-2.86243802535101,
-2.86128495050293,-2.86056616352924,-2.85990254225026,-2.85903469582242,
-2.85712596413958,-2.84185665231,-2.84123050729425,-2.83885125461131,-2.83192990478553,
-2.76341658478353,-2.73448352958715,-2.70770601607517,-2.70418487854436,
-2.70140095946039,-2.699959918848,-2.69889409011143,-2.69775803604036,-2.6961475779052,
-2.6917974291399,-2.6184276668183,-2.56859383444668,-2.54951070661052,-2.54055478622066,
-2.5390381817123,-2.538239397899,-2.53759072504984,-2.53692371165883,-2.53567158114221,
-2.53142949248462,-2.45690138500186,-2.41371548288173,-2.38806071896264,
-2.38304262582197,-2.37930455642501,-2.37767170294239,-2.37647167184569,
-2.37536485949717,-2.37386501882376,-2.37018189195767,-2.31913591187493,
-2.29422451502291,-2.24580699105114,-2.22687874109205,-2.21802365829361,
-2.21651168278256,-2.21571389333632,-2.21506528004273,-2.21439766328819,
-2.21314248082997,-2.20887347621438,-2.1340612618785,-2.09106008450369,
-2.06549021339839,-2.057914419542,-2.05576651701238,-2.05445772866599,-2.05327655330566,
-2.05176861829506,-2.04879306091321,-2.03110452184611,-1.98742809340207,
-1.8995917320736,-1.89501699559509,-1.89374303253049,-1.89298975211511,
-1.89233354118016,-1.89151245397762,-1.88988927285698,-1.87813654855862,
-1.85157472971377,-1.79129114485283,-1.73818167604261,-1.73433567324719,
-1.73280764484916,-1.7316935159328,-1.7304983472386,-1.72889450670342,-1.72531726610269,
-1.67587512379374,-1.58430610411295,-1.57312948655571,-1.57138276296661,
-1.57053665320079,-1.56987788627118,-1.56914038108417,-1.56790427173414,
-1.56328138192024,-1.53008432777748,-1.44726166379064,-1.44098101010954,
-1.43381993741566,-1.41423397001383,-1.41112730629537,-1.40961335922946,
-1.40843123904355,-1.40712524707561,-1.40499065081702,-1.39754786078178,
-1.35029219345686,-1.26306858931603,-1.25050895106294,-1.24888120344901,
-1.2480470462768,-1.24743120827324,-1.24677168968778,-1.24585971065689,
-1.24376238628546,-1.24088484071129,-1.2110237191372,-1.14883359296096,
-1.0927995609803,-1.08892758415155,-1.08739494992516,-1.08627947089618,
-1.08508474536429,-1.08348477604279,-1.07992966953421,-1.02993200486211,
-0.941374290409813,-0.940435776942215,-0.927789621217176,-0.926158554940047,
-0.925323492209265,-0.924707373701481,-0.924084798603714,-0.923197366954174,
-0.921221998688909,-0.918557925163082,-0.892459960234906,-0.845165487382356,
-0.771150630036447,-0.766487904222883,-0.764829341003457,-0.763679738270363,
-0.76261714889549,-0.761175458119865,-0.758422244573456,-0.741559916201148,
-0.704027631937379,-0.633542480812273,-0.605678782390739,-0.603513354421616,
-0.602657630643331,-0.602036173225907,-0.601410143291156,-0.60053908972563,
-0.598711417293119,-0.59625822323979,-0.590391929139022,-0.571427828814243,
-0.538277446886927,-0.468894489325305,-0.446303785723019,-0.443389492276724,
-0.441892861812162,-0.440786528475238,-0.439585188463481,-0.437947288396691,
-0.434183386407426,-0.429122409831035,-0.40332631888975,-0.35847569032206,
-0.317948250199433,-0.305946417234263,-0.298902685152201,-0.295635185601995,
-0.294588555524527,-0.282426574417055,-0.280635801625219,-0.279790080904281,
-0.279129495504108,-0.278514743861476,-0.277796405396636,-0.275649395382003,
-0.248817718028,-0.229763844089698,-0.139484360858154,-0.123137138790546,
-0.120490509893527,-0.118922931077595,-0.117728970396443,-0.116459247698824,
-0.114488047529457,-0.10848613054866,-0.07529142213324,-0.000958271623644713),
 .UNSPECIFIED.);
#875=B_SPLINE_CURVE_WITH_KNOTS('',3,(#64706,#64707,#64708,#64709,#64710,
#64711,#64712,#64713,#64714,#64715,#64716,#64717,#64718,#64719,#64720,#64721,
#64722,#64723,#64724,#64725,#64726,#64727,#64728,#64729,#64730,#64731,#64732,
#64733,#64734,#64735,#64736,#64737,#64738,#64739,#64740,#64741,#64742,#64743,
#64744,#64745,#64746,#64747,#64748,#64749,#64750,#64751,#64752,#64753,#64754,
#64755,#64756,#64757,#64758,#64759,#64760,#64761,#64762,#64763,#64764,#64765,
#64766,#64767,#64768,#64769,#64770,#64771,#64772,#64773,#64774,#64775,#64776,
#64777,#64778,#64779,#64780,#64781,#64782,#64783,#64784,#64785,#64786,#64787,
#64788,#64789,#64790,#64791,#64792,#64793,#64794,#64795,#64796,#64797,#64798,
#64799,#64800,#64801,#64802,#64803,#64804,#64805,#64806,#64807,#64808,#64809,
#64810,#64811,#64812,#64813,#64814,#64815,#64816,#64817,#64818,#64819,#64820,
#64821,#64822,#64823,#64824,#64825,#64826,#64827,#64828,#64829,#64830,#64831,
#64832,#64833,#64834,#64835,#64836,#64837,#64838,#64839,#64840,#64841,#64842,
#64843,#64844,#64845,#64846,#64847,#64848,#64849,#64850,#64851,#64852,#64853,
#64854,#64855,#64856,#64857,#64858,#64859,#64860,#64861,#64862,#64863,#64864,
#64865,#64866,#64867,#64868,#64869,#64870,#64871,#64872,#64873,#64874,#64875,
#64876,#64877,#64878,#64879,#64880,#64881,#64882,#64883,#64884,#64885,#64886,
#64887,#64888,#64889,#64890,#64891,#64892,#64893,#64894,#64895,#64896,#64897,
#64898,#64899,#64900,#64901,#64902,#64903,#64904,#64905,#64906,#64907,#64908,
#64909,#64910,#64911,#64912,#64913,#64914,#64915,#64916,#64917,#64918,#64919,
#64920,#64921,#64922,#64923,#64924,#64925,#64926,#64927,#64928,#64929,#64930,
#64931,#64932,#64933,#64934,#64935,#64936,#64937,#64938,#64939,#64940,#64941,
#64942,#64943,#64944,#64945,#64946,#64947,#64948,#64949,#64950,#64951,#64952,
#64953,#64954,#64955,#64956,#64957,#64958,#64959,#64960,#64961,#64962,#64963,
#64964,#64965,#64966,#64967,#64968,#64969,#64970,#64971,#64972,#64973,#64974,
#64975,#64976,#64977,#64978,#64979,#64980,#64981,#64982,#64983,#64984,#64985,
#64986,#64987,#64988,#64989,#64990,#64991,#64992,#64993,#64994,#64995,#64996,
#64997,#64998,#64999,#65000,#65001,#65002,#65003,#65004,#65005,#65006,#65007,
#65008,#65009,#65010,#65011,#65012,#65013,#65014,#65015,#65016,#65017,#65018,
#65019,#65020,#65021,#65022,#65023,#65024,#65025,#65026,#65027,#65028,#65029,
#65030,#65031,#65032,#65033,#65034,#65035,#65036,#65037,#65038,#65039,#65040,
#65041,#65042,#65043,#65044,#65045,#65046,#65047,#65048,#65049,#65050,#65051,
#65052,#65053,#65054,#65055,#65056,#65057,#65058,#65059,#65060,#65061,#65062,
#65063,#65064,#65065,#65066,#65067,#65068,#65069,#65070,#65071,#65072,#65073,
#65074,#65075,#65076,#65077,#65078,#65079,#65080,#65081,#65082,#65083,#65084,
#65085,#65086,#65087,#65088,#65089,#65090,#65091,#65092,#65093,#65094,#65095,
#65096,#65097,#65098,#65099,#65100,#65101,#65102,#65103,#65104,#65105,#65106,
#65107,#65108,#65109,#65110,#65111,#65112,#65113,#65114,#65115,#65116,#65117,
#65118,#65119,#65120,#65121,#65122,#65123,#65124,#65125,#65126,#65127,#65128,
#65129,#65130,#65131,#65132,#65133,#65134,#65135,#65136,#65137,#65138,#65139,
#65140,#65141,#65142,#65143,#65144,#65145,#65146,#65147,#65148,#65149,#65150,
#65151,#65152,#65153,#65154,#65155,#65156,#65157,#65158,#65159,#65160,#65161,
#65162,#65163,#65164,#65165,#65166,#65167,#65168,#65169,#65170,#65171,#65172,
#65173,#65174,#65175,#65176,#65177,#65178,#65179,#65180,#65181,#65182,#65183,
#65184,#65185,#65186,#65187,#65188,#65189,#65190,#65191,#65192,#65193,#65194,
#65195,#65196,#65197,#65198,#65199,#65200,#65201,#65202,#65203,#65204,#65205,
#65206,#65207,#65208,#65209,#65210,#65211,#65212,#65213,#65214,#65215,#65216,
#65217,#65218,#65219,#65220,#65221,#65222,#65223,#65224,#65225,#65226,#65227,
#65228,#65229,#65230,#65231,#65232,#65233,#65234,#65235,#65236,#65237,#65238,
#65239,#65240,#65241,#65242,#65243,#65244,#65245,#65246,#65247,#65248,#65249,
#65250,#65251,#65252,#65253),.UNSPECIFIED.,.F.,.F.,(4,2,2,2,2,2,2,2,2,2,
2,2,2,2,2,2,2,2,2,2,2,2,2,2,2,2,2,2,2,2,2,2,2,2,2,2,2,2,2,2,2,2,2,2,2,2,
2,2,2,2,2,2,2,2,2,2,2,2,2,2,2,2,2,2,2,2,2,2,2,2,2,2,2,2,2,2,2,2,2,2,2,2,
2,2,2,2,2,2,2,2,2,2,2,2,2,2,2,2,2,2,2,2,2,2,2,2,2,2,2,2,2,2,2,2,2,2,2,2,
2,2,2,2,2,2,2,2,2,2,2,2,2,2,2,2,2,2,2,2,2,2,2,2,2,2,2,2,2,2,2,2,2,2,2,2,
2,2,2,2,2,2,2,2,2,2,2,2,2,2,2,2,2,2,2,2,2,2,2,2,2,2,2,2,2,2,2,2,2,2,2,2,
2,2,2,2,2,2,2,2,2,2,2,2,2,2,2,2,2,2,2,2,2,2,2,2,2,2,2,2,2,2,2,2,2,2,2,2,
2,2,2,2,2,2,2,2,2,2,2,2,2,2,2,2,2,2,2,2,2,2,2,2,2,2,2,2,2,2,2,2,2,2,2,2,
2,2,2,2,2,2,2,2,2,2,2,4),(-4.06054173240988,-4.02058570238127,-4.01875545172079,
-4.01770545766817,-4.016978695896,-4.01636305788412,-4.01570464905039,-4.01486107357676,
-4.01312680093112,-4.00221193031645,-3.999924470005,-3.99674131556362,-3.97461839182422,
-3.96933614986905,-3.91205726126169,-3.86601400458494,-3.85868367516395,
-3.8565608411054,-3.85525752746501,-3.85407486318991,-3.8525560823871,-3.84942483471692,
-3.82930070060744,-3.82329163044152,-3.7473505980948,-3.7215458154747,-3.70694023010225,
-3.69992368131608,-3.69712584876673,-3.69506931722858,-3.69435889293425,
-3.69374497577411,-3.69308230207342,-3.69222118828335,-3.69041615491519,
-3.67734103291924,-3.67397582543777,-3.66720433544192,-3.65453252885351,
-3.60623937532244,-3.59981345960569,-3.56975130937846,-3.54392055922187,
-3.53621314668269,-3.5340516621585,-3.5327396336653,-3.53155878784385,-3.53005574073782,
-3.52710395333014,-3.50987351271807,-3.50882361005823,-3.43834778113679,
-3.39878957717023,-3.38431000332136,-3.37734627277779,-3.37456386876616,
-3.37251851069903,-3.37161833006428,-3.37094865912725,-3.370327977555,-3.36947486093409,
-3.36732397145806,-3.34029185485344,-3.26703533429014,-3.22085873452279,
-3.21351565049087,-3.21139139895943,-3.21008771697486,-3.20890504843565,
-3.20738672254149,-3.2042580489153,-3.18419356396322,-3.17796355599614,
-3.10200852367228,-3.05298995397825,-3.0510792522122,-3.04957054151396,
-3.0487764214578,-3.04812086195007,-3.04745893223393,-3.04623254057066,
-3.04221205371738,-2.9674289482759,-2.89304952306376,-2.8895826808681,-2.88799920623245,
-2.88680724568932,-2.88568737085695,-2.88413767893281,-2.88101383134194,
-2.85171580498124,-2.82959418464685,-2.76208704384754,-2.73219371986278,
-2.72931480815302,-2.72721133757102,-2.72630151059308,-2.72564245326429,
-2.72502624102431,-2.72419045316517,-2.72255620574681,-2.70981568283167,
-2.70799357505028,-2.70015767492631,-2.68473016274241,-2.62048216674927,
-2.58570086725821,-2.56931808134276,-2.56658586586715,-2.56514878405913,
-2.56408689617126,-2.56293543189889,-2.56126966927437,-2.5565572727695,
-2.48237962277254,-2.43439051107804,-2.40909187569006,-2.40514488526984,
-2.40397673514042,-2.40325445473263,-2.40259177033796,-2.40173084213492,
-2.39992690406947,-2.38688016150908,-2.38366191290005,-2.38151071381351,
-2.37461971462848,-2.35832772674211,-2.32828775473404,-2.29940612344123,
-2.25300654105434,-2.24564222570681,-2.24351563429889,-2.24221135282333,
-2.24102868986355,-2.23951113697194,-2.23638677399111,-2.21642123894337,
-2.21085514458431,-2.16743681442079,-2.11778017265357,-2.0934905409715,
-2.08332731900652,-2.08175986211478,-2.08095024555145,-2.08035772900889,
-2.07971202804921,-2.07876716282358,-2.07602546714092,-2.03164749009595,
-1.9353431972879,-1.92829460028116,-1.92267213925653,-1.92068042923444,
-1.9195337321908,-1.91847077824902,-1.91702394905577,-1.9142452400809,-1.89675049413491,
-1.85631167696801,-1.77177850251612,-1.76082942520942,-1.75909336191206,
-1.75824936021085,-1.75759082505384,-1.75685207677666,-1.75561044824367,
-1.75092823831163,-1.71694991556723,-1.63531349669321,-1.62647952944112,
-1.62127327998383,-1.60193394884238,-1.5988387768399,-1.59732710024486,
-1.59614523480706,-1.5948379738486,-1.59269778808553,-1.58520093141039,
-1.53735728958329,-1.44201115415768,-1.43733670299921,-1.43605204393648,
-1.43529613306126,-1.43463999104861,-1.43382202550577,-1.43221466933165,
-1.42095331918417,-1.38688105792138,-1.2831161430962,-1.28167296674716,
-1.27683524940639,-1.27496392129631,-1.27384085499594,-1.27267430091801,
-1.27114938890705,-1.26946921101127,-1.26669083658375,-1.21030353114819,
-1.12619232831601,-1.11521635008148,-1.1134789012282,-1.11263457891498,
-1.11197595651617,-1.11123728411188,-1.10999618093828,-1.10532045578578,
-1.07143114986391,-0.990394934343854,-0.95704562975981,-0.953461841862194,
-0.95201711454946,-0.950814270858487,-0.949606907521943,-0.947866065420648,
-0.945887002110378,-0.942378227593677,-0.934700707455248,-0.912584835536502,
-0.868237212244875,-0.795516726407038,-0.791623855581194,-0.790412856038334,
-0.789753988390567,-0.789097994646529,-0.788281801986684,-0.786682937855588,
-0.775667433433133,-0.74741577790899,-0.701347966776549,-0.635036239808415,
-0.631088831508773,-0.629543414468046,-0.628424552098376,-0.627255582417368,
-0.625748251891298,-0.624064291845193,-0.621276971015926,-0.615654207189192,
-0.601154475927136,-0.567080705902515,-0.483230526948228,-0.480100403342687,
-0.469782925850279,-0.468077676793534,-0.467239737234692,-0.466581755411169,
-0.46583913376575,-0.46458057795939,-0.45971306857014,-0.43653864768605,
-0.386154887574586,-0.359580447511575,-0.312114852168862,-0.310265566614375,
-0.307867135672493,-0.306357207318808,-0.305221085814658,-0.303951933507669,
-0.301939409682461,-0.299571157082405,-0.295070370780411,-0.284332911011669,
-0.249914683940878,-0.158683821464179,-0.14714091930333,-0.145377018848626,
-0.144527327768726,-0.143867932392595,-0.143132009382931,-0.141903726810655,
-0.137367016506054,-0.105281344936748,-0.000957917344321264),
 .UNSPECIFIED.);
#876=B_SPLINE_CURVE_WITH_KNOTS('',3,(#65255,#65256,#65257,#65258,#65259,
#65260,#65261,#65262,#65263,#65264,#65265,#65266,#65267,#65268,#65269,#65270,
#65271,#65272,#65273,#65274,#65275,#65276,#65277,#65278,#65279,#65280,#65281,
#65282,#65283,#65284,#65285,#65286,#65287,#65288,#65289,#65290,#65291,#65292,
#65293,#65294,#65295,#65296,#65297,#65298,#65299,#65300,#65301,#65302,#65303,
#65304,#65305,#65306,#65307,#65308,#65309,#65310,#65311,#65312,#65313,#65314,
#65315,#65316,#65317,#65318,#65319,#65320,#65321,#65322,#65323,#65324,#65325,
#65326,#65327,#65328,#65329,#65330,#65331,#65332,#65333,#65334,#65335,#65336,
#65337,#65338,#65339,#65340,#65341,#65342,#65343,#65344,#65345,#65346,#65347,
#65348,#65349,#65350,#65351,#65352,#65353,#65354,#65355,#65356,#65357,#65358,
#65359,#65360,#65361,#65362,#65363,#65364,#65365,#65366,#65367,#65368,#65369,
#65370,#65371,#65372,#65373,#65374,#65375,#65376,#65377,#65378,#65379,#65380,
#65381,#65382,#65383,#65384,#65385,#65386,#65387,#65388,#65389,#65390,#65391,
#65392,#65393,#65394,#65395,#65396,#65397,#65398,#65399,#65400,#65401,#65402,
#65403,#65404,#65405,#65406,#65407,#65408,#65409,#65410,#65411,#65412,#65413,
#65414,#65415,#65416,#65417,#65418,#65419,#65420,#65421,#65422,#65423,#65424,
#65425,#65426,#65427,#65428,#65429,#65430,#65431,#65432,#65433,#65434,#65435,
#65436,#65437,#65438,#65439,#65440,#65441,#65442,#65443,#65444,#65445,#65446,
#65447,#65448,#65449,#65450,#65451,#65452,#65453,#65454,#65455,#65456,#65457,
#65458,#65459,#65460,#65461,#65462,#65463,#65464,#65465,#65466,#65467,#65468,
#65469,#65470,#65471,#65472,#65473,#65474,#65475,#65476,#65477,#65478,#65479,
#65480,#65481,#65482,#65483,#65484,#65485,#65486,#65487,#65488,#65489,#65490,
#65491,#65492,#65493,#65494,#65495,#65496,#65497,#65498,#65499,#65500,#65501,
#65502,#65503,#65504,#65505,#65506,#65507,#65508,#65509,#65510,#65511,#65512,
#65513,#65514,#65515,#65516,#65517,#65518,#65519,#65520,#65521,#65522,#65523,
#65524,#65525,#65526,#65527,#65528,#65529,#65530,#65531,#65532,#65533,#65534,
#65535,#65536,#65537,#65538,#65539,#65540,#65541,#65542,#65543,#65544,#65545,
#65546,#65547,#65548,#65549,#65550,#65551,#65552,#65553,#65554,#65555,#65556,
#65557,#65558,#65559,#65560,#65561,#65562,#65563,#65564,#65565,#65566,#65567,
#65568,#65569,#65570,#65571,#65572,#65573,#65574,#65575,#65576,#65577,#65578,
#65579,#65580,#65581,#65582,#65583,#65584,#65585,#65586,#65587,#65588,#65589,
#65590,#65591,#65592,#65593,#65594,#65595,#65596,#65597,#65598,#65599,#65600,
#65601,#65602,#65603,#65604,#65605,#65606,#65607,#65608,#65609,#65610,#65611,
#65612,#65613,#65614,#65615,#65616,#65617,#65618,#65619,#65620,#65621,#65622,
#65623,#65624,#65625,#65626,#65627,#65628,#65629,#65630,#65631,#65632,#65633,
#65634,#65635,#65636,#65637,#65638,#65639,#65640,#65641,#65642,#65643,#65644,
#65645,#65646,#65647,#65648,#65649,#65650,#65651,#65652,#65653,#65654,#65655,
#65656,#65657,#65658,#65659,#65660,#65661,#65662,#65663,#65664,#65665,#65666,
#65667,#65668,#65669,#65670,#65671,#65672,#65673,#65674,#65675,#65676,#65677,
#65678,#65679,#65680,#65681,#65682,#65683,#65684,#65685,#65686,#65687,#65688,
#65689,#65690,#65691,#65692,#65693,#65694,#65695,#65696,#65697,#65698,#65699,
#65700,#65701,#65702,#65703,#65704,#65705,#65706,#65707,#65708,#65709,#65710,
#65711,#65712,#65713,#65714,#65715,#65716,#65717,#65718,#65719,#65720,#65721,
#65722,#65723,#65724,#65725,#65726,#65727,#65728,#65729,#65730,#65731,#65732,
#65733,#65734,#65735,#65736,#65737,#65738,#65739,#65740,#65741,#65742,#65743,
#65744,#65745,#65746,#65747,#65748,#65749,#65750,#65751,#65752,#65753,#65754,
#65755,#65756,#65757,#65758,#65759,#65760,#65761,#65762,#65763,#65764,#65765,
#65766,#65767,#65768,#65769,#65770,#65771,#65772,#65773,#65774,#65775,#65776,
#65777,#65778,#65779,#65780,#65781,#65782,#65783,#65784,#65785,#65786,#65787,
#65788,#65789,#65790,#65791,#65792,#65793,#65794,#65795,#65796,#65797,#65798,
#65799,#65800,#65801,#65802),.UNSPECIFIED.,.F.,.F.,(4,2,2,2,2,2,2,2,2,2,
2,2,2,2,2,2,2,2,2,2,2,2,2,2,2,2,2,2,2,2,2,2,2,2,2,2,2,2,2,2,2,2,2,2,2,2,
2,2,2,2,2,2,2,2,2,2,2,2,2,2,2,2,2,2,2,2,2,2,2,2,2,2,2,2,2,2,2,2,2,2,2,2,
2,2,2,2,2,2,2,2,2,2,2,2,2,2,2,2,2,2,2,2,2,2,2,2,2,2,2,2,2,2,2,2,2,2,2,2,
2,2,2,2,2,2,2,2,2,2,2,2,2,2,2,2,2,2,2,2,2,2,2,2,2,2,2,2,2,2,2,2,2,2,2,2,
2,2,2,2,2,2,2,2,2,2,2,2,2,2,2,2,2,2,2,2,2,2,2,2,2,2,2,2,2,2,2,2,2,2,2,2,
2,2,2,2,2,2,2,2,2,2,2,2,2,2,2,2,2,2,2,2,2,2,2,2,2,2,2,2,2,2,2,2,2,2,2,2,
2,2,2,2,2,2,2,2,2,2,2,2,2,2,2,2,2,2,2,2,2,2,2,2,2,2,2,2,2,2,2,2,2,2,2,2,
2,2,2,2,2,2,2,2,2,2,2,4),(-4.06119598324708,-4.04831213485074,-4.04613216796598,
-4.0447032789022,-4.0435695858176,-4.04241134613562,-4.04108248347896,-4.03884564966487,
-4.03133266086793,-4.02913402067733,-4.02226911079524,-3.91185697649888,
-3.89286452981374,-3.88397315721871,-3.88245903351183,-3.88166057909371,
-3.88106915056492,-3.88032166421199,-3.87904124063376,-3.87454882418137,
-3.78599732559944,-3.74811169684466,-3.73287020459906,-3.72703583866328,
-3.72417159316184,-3.72245567057437,-3.72090411274886,-3.71973344540439,
-3.71861775919585,-3.71708448499482,-3.71320903293776,-3.65672615559556,
-3.63036541331377,-3.62268870331163,-3.59821812146691,-3.57196980179826,
-3.56139951422218,-3.55981662924339,-3.55900376794863,-3.55841085008741,
-3.55776667046272,-3.55662849576664,-3.55329986138373,-3.49528807827662,
-3.44566369845203,-3.42583664661937,-3.41038524812807,-3.40449164447257,
-3.4016060101805,-3.39988123352774,-3.3983227302198,-3.39715105238165,-3.39603706641129,
-3.39451027206645,-3.39067278295422,-3.33859720518647,-3.28947302144958,
-3.27770195672611,-3.24294795508707,-3.23820875971718,-3.23696184576256,
-3.23622188177811,-3.23556351871944,-3.2347214280468,-3.23305236783941,
-3.22303324262004,-3.17848047476073,-3.0878010906804,-3.08183977120618,
-3.07892980232035,-3.07719500042003,-3.07562948631269,-3.07445658035381,
-3.07334468761864,-3.07182572137609,-3.06803349556223,-3.01970685160269,
-2.95489343224616,-2.92022493582164,-2.9154921082358,-2.91424582110855,
-2.9135060233453,-2.91284767419626,-2.91200542132921,-2.91027818003952,
-2.89951759804377,-2.82386997055,-2.75904561575592,-2.7561872791134,-2.75447387592398,
-2.75292337466126,-2.75175321153512,-2.75063707188765,-2.7491017027941,
-2.74521322884299,-2.68661337893046,-2.63639824644016,-2.60468183355031,
-2.59345516003901,-2.59184917015406,-2.59103156441559,-2.59043812285857,
-2.58979626910084,-2.5886694798217,-2.58541465028248,-2.52940490180812,
-2.47909580399444,-2.43561341913953,-2.43199120511317,-2.43037900862065,
-2.42918231173339,-2.42807012366431,-2.42654997558329,-2.42275079702834,
-2.3738994737391,-2.35868228349457,-2.33387987752456,-2.31109816538221,
-2.27511212623186,-2.27028541379398,-2.26903070053604,-2.26828905298795,
-2.26763109808349,-2.26679207879462,-2.26508082902035,-2.25463918114359,
-2.16155426094268,-2.11756558024354,-2.11285724236001,-2.1093056135218,
-2.10770646639083,-2.10651205460603,-2.10539665045518,-2.10386377803796,
-2.10080651930832,-2.07385997440993,-2.06017827746862,-2.03093944879856,
-1.95172518779088,-1.94756236716279,-1.94631924002593,-1.94565396275599,
-1.94499875922123,-1.94419394926238,-1.94264922557405,-1.93305016168607,
-1.91576176969738,-1.89047118732563,-1.81638810307692,-1.80902375511383,
-1.78955767135633,-1.78645664177325,-1.78494383418346,-1.78376187249125,
-1.78245530954921,-1.78031809037149,-1.77284958067353,-1.72531401690485,
-1.62959765373666,-1.62495074811905,-1.62366899216035,-1.62291377666702,
-1.62225759108585,-1.6214387390334,-1.61982699959438,-1.60843389140765,
-1.57842822327829,-1.4834096111169,-1.46652407837208,-1.46359002810906,
-1.46209076776547,-1.46091031939734,-1.45959606425452,-1.45742475703102,
-1.44961885609579,-1.39826972063741,-1.3066025801482,-1.30209966064335,
-1.30081810752998,-1.30007037774205,-1.29942620051062,-1.2986196542456,
-1.29774138718091,-1.29632895847721,-1.29356292091741,-1.26570495741673,
-1.18044578342886,-1.14476346729518,-1.14148519071065,-1.13989708953866,
-1.13876685690014,-1.1376984185932,-1.13621146183489,-1.13323949844945,
-1.10992419252317,-1.09006511377496,-1.04034555643182,-0.982556257018479,
-0.979154360057,-0.978006778257242,-0.977360698283811,-0.976715330821373,
-0.975896758639818,-0.975001931838431,-0.973549776997043,-0.970676345182222,
-0.940891509829287,-0.849400214579552,-0.821728963188047,-0.818308426466099,
-0.816750609661067,-0.815558352199623,-0.814284881599966,-0.812296410671139,
-0.806154164872239,-0.771689339545847,-0.756754354086426,-0.745142588021295,
-0.661194890293366,-0.656665019158565,-0.655395623826028,-0.654643293109446,
-0.653999718288247,-0.653199821391288,-0.652330724473448,-0.650940208704385,
-0.648232940268742,-0.641524772982774,-0.617497692152871,-0.527929709181589,
-0.499043405954087,-0.495629617301253,-0.494190651428808,-0.492989320742526,
-0.49175549807956,-0.489950427590264,-0.485161554695287,-0.462244339077295,
-0.427908411380341,-0.41813426046919,-0.409990329352877,-0.402997640182685,
-0.388979831589526,-0.34825753485031,-0.334943683653466,-0.333105859760514,
-0.33225122229192,-0.331605368496845,-0.330899696399484,-0.33016296767771,
-0.329088852740455,-0.327198820235607,-0.323082202484467,-0.31116969197251,
-0.29192970666293,-0.203992326073534,-0.176370337764317,-0.172951638971376,
-0.1713942602897,-0.17020217250957,-0.168928722126584,-0.166939949800652,
-0.160794192577671,-0.126295168089752,-0.0223944647338021,-0.0163729017965301,
-0.0113135017104637,-0.00999015043440988,-0.00922523504495427,-0.00863391393677181,
-0.00801091682884623,-0.00724723259923413,-0.00610832021660343,-0.00100602066474334),
 .UNSPECIFIED.);
#877=B_SPLINE_CURVE_WITH_KNOTS('',3,(#65804,#65805,#65806,#65807,#65808,
#65809,#65810,#65811,#65812,#65813),.UNSPECIFIED.,.F.,.F.,(4,1,1,1,1,1,
1,4),(304.734490891393,305.708479969717,306.707272373485,307.706064777253,
308.704857181021,309.703649584789,310.702441988557,311.017666207308),
 .UNSPECIFIED.);
#878=B_SPLINE_CURVE_WITH_KNOTS('',3,(#65815,#65816,#65817,#65818,#65819,
#65820,#65821,#65822,#65823,#65824,#65825,#65826,#65827,#65828,#65829,#65830,
#65831,#65832,#65833,#65834,#65835,#65836,#65837,#65838,#65839,#65840,#65841,
#65842,#65843,#65844,#65845,#65846,#65847,#65848,#65849,#65850,#65851,#65852,
#65853,#65854,#65855,#65856,#65857,#65858,#65859,#65860,#65861,#65862,#65863,
#65864,#65865,#65866,#65867,#65868,#65869,#65870,#65871,#65872,#65873,#65874,
#65875,#65876,#65877,#65878,#65879,#65880,#65881,#65882,#65883,#65884,#65885,
#65886,#65887,#65888,#65889,#65890,#65891,#65892,#65893,#65894,#65895,#65896,
#65897,#65898,#65899,#65900,#65901,#65902,#65903,#65904,#65905,#65906,#65907,
#65908,#65909,#65910,#65911,#65912,#65913,#65914,#65915,#65916,#65917,#65918,
#65919,#65920,#65921,#65922,#65923,#65924,#65925,#65926,#65927,#65928,#65929,
#65930,#65931,#65932,#65933,#65934,#65935,#65936,#65937,#65938,#65939,#65940,
#65941,#65942,#65943,#65944,#65945,#65946,#65947,#65948,#65949,#65950,#65951,
#65952,#65953,#65954,#65955,#65956,#65957,#65958,#65959,#65960,#65961,#65962,
#65963,#65964,#65965,#65966,#65967,#65968,#65969,#65970,#65971,#65972,#65973,
#65974,#65975,#65976,#65977,#65978,#65979,#65980,#65981,#65982,#65983,#65984,
#65985,#65986,#65987,#65988,#65989,#65990,#65991,#65992,#65993,#65994,#65995,
#65996,#65997,#65998,#65999,#66000,#66001,#66002,#66003,#66004,#66005,#66006,
#66007,#66008,#66009,#66010,#66011,#66012,#66013,#66014,#66015,#66016,#66017,
#66018,#66019,#66020,#66021,#66022,#66023,#66024,#66025,#66026,#66027,#66028,
#66029,#66030,#66031,#66032,#66033,#66034,#66035,#66036,#66037,#66038,#66039,
#66040,#66041,#66042,#66043,#66044,#66045,#66046,#66047,#66048,#66049,#66050,
#66051,#66052,#66053,#66054,#66055,#66056,#66057,#66058,#66059,#66060,#66061,
#66062,#66063,#66064,#66065,#66066,#66067,#66068,#66069,#66070,#66071,#66072,
#66073,#66074,#66075,#66076,#66077,#66078,#66079,#66080,#66081,#66082,#66083,
#66084,#66085,#66086,#66087,#66088,#66089,#66090,#66091,#66092,#66093,#66094,
#66095,#66096,#66097,#66098,#66099,#66100,#66101,#66102,#66103,#66104,#66105,
#66106,#66107,#66108,#66109,#66110,#66111,#66112,#66113,#66114,#66115,#66116,
#66117,#66118,#66119,#66120,#66121,#66122,#66123,#66124,#66125,#66126,#66127,
#66128,#66129,#66130,#66131,#66132,#66133,#66134,#66135,#66136,#66137,#66138,
#66139,#66140,#66141,#66142,#66143,#66144,#66145,#66146,#66147,#66148,#66149,
#66150,#66151,#66152,#66153,#66154,#66155,#66156,#66157,#66158,#66159,#66160,
#66161,#66162,#66163,#66164,#66165,#66166,#66167,#66168,#66169,#66170,#66171,
#66172,#66173,#66174,#66175,#66176,#66177,#66178,#66179,#66180,#66181,#66182,
#66183,#66184,#66185,#66186,#66187,#66188,#66189,#66190,#66191,#66192,#66193,
#66194,#66195,#66196,#66197,#66198,#66199,#66200,#66201,#66202,#66203,#66204,
#66205,#66206,#66207,#66208,#66209,#66210,#66211,#66212,#66213,#66214,#66215,
#66216,#66217,#66218,#66219,#66220,#66221,#66222,#66223,#66224,#66225,#66226,
#66227,#66228,#66229,#66230,#66231,#66232,#66233,#66234,#66235,#66236,#66237,
#66238,#66239,#66240,#66241,#66242,#66243,#66244,#66245,#66246,#66247,#66248,
#66249,#66250,#66251,#66252,#66253,#66254,#66255,#66256,#66257,#66258,#66259,
#66260,#66261,#66262,#66263,#66264,#66265,#66266,#66267,#66268,#66269,#66270,
#66271,#66272,#66273,#66274,#66275,#66276,#66277,#66278,#66279,#66280,#66281,
#66282,#66283,#66284,#66285,#66286,#66287,#66288,#66289,#66290,#66291,#66292,
#66293,#66294,#66295,#66296,#66297,#66298,#66299,#66300,#66301,#66302,#66303,
#66304,#66305,#66306,#66307,#66308,#66309,#66310,#66311,#66312,#66313,#66314,
#66315,#66316,#66317,#66318,#66319,#66320,#66321,#66322,#66323,#66324,#66325,
#66326,#66327,#66328,#66329,#66330,#66331,#66332,#66333,#66334,#66335,#66336,
#66337,#66338,#66339,#66340,#66341,#66342,#66343,#66344,#66345,#66346,#66347,
#66348,#66349,#66350),.UNSPECIFIED.,.F.,.F.,(4,2,2,2,2,2,2,2,2,2,2,2,2,
2,2,2,2,2,2,2,2,2,2,2,2,2,2,2,2,2,2,2,2,2,2,2,2,2,2,2,2,2,2,2,2,2,2,2,2,
2,2,2,2,2,2,2,2,2,2,2,2,2,2,2,2,2,2,2,2,2,2,2,2,2,2,2,2,2,2,2,2,2,2,2,2,
2,2,2,2,2,2,2,2,2,2,2,2,2,2,2,2,2,2,2,2,2,2,2,2,2,2,2,2,2,2,2,2,2,2,2,2,
2,2,2,2,2,2,2,2,2,2,2,2,2,2,2,2,2,2,2,2,2,2,2,2,2,2,2,2,2,2,2,2,2,2,2,2,
2,2,2,2,2,2,2,2,2,2,2,2,2,2,2,2,2,2,2,2,2,2,2,2,2,2,2,2,2,2,2,2,2,2,2,2,
2,2,2,2,2,2,2,2,2,2,2,2,2,2,2,2,2,2,2,2,2,2,2,2,2,2,2,2,2,2,2,2,2,2,2,2,
2,2,2,2,2,2,2,2,2,2,2,2,2,2,2,2,2,2,2,2,2,2,2,2,2,2,2,2,2,2,2,2,2,2,2,2,
2,2,4),(-4.06080606694336,-4.00717255232006,-4.0047483802516,-4.00321666452518,
-4.00204936916829,-4.00085773774574,-3.99973792161758,-3.99818791373868,
-3.9950621925593,-3.96567738302845,-3.94671800235698,-3.93958039481456,
-3.87039716115203,-3.85137641269848,-3.84246594045836,-3.84095138336434,
-3.8401530259413,-3.83956181069048,-3.83881478269707,-3.83753559479031,
-3.8330516310455,-3.74727275620697,-3.71866671116966,-3.69898629847681,
-3.68333149825631,-3.6806415774336,-3.67947416247776,-3.67828247504177,
-3.67716279529695,-3.67561327584829,-3.67248947249685,-3.64317490838713,
-3.62443646244887,-3.56672948021867,-3.55863577978085,-3.53093908446463,
-3.52004935454113,-3.51845536725507,-3.5176403710051,-3.51698469096027,
-3.5163255873877,-3.51511263069805,-3.51120150821404,-3.4384698843406,-3.39650433651383,
-3.37283344665796,-3.36475891739992,-3.35933187642299,-3.35744081558777,
-3.35633953030525,-3.3551571491848,-3.35363932993903,-3.35051218926495,
-3.33047039431957,-3.32484796131439,-3.3193609166491,-3.31161587996121,
-3.23584994889392,-3.20920342764072,-3.19754598338155,-3.19592596360619,
-3.19510556674154,-3.1944494595678,-3.19369579842393,-3.19242004826655,
-3.18782781124516,-3.10082316149683,-3.06622252926881,-3.04157224076184,
-3.03821357469777,-3.03553721628582,-3.03411816734862,-3.03294271497257,
-3.03176927726416,-3.02964360842558,-3.02304316668977,-3.01694730574734,
-2.92659565795725,-2.875625914849,-2.87350494970679,-2.87258887738458,-2.87191974391799,
-2.87129854301787,-2.87044321070968,-2.86873189684117,-2.85371290167005,
-2.85206295001582,-2.84897482984182,-2.84690299858028,-2.83493600444057,
-2.76834181078234,-2.74454869528609,-2.71908574205562,-2.71566438587501,
-2.71294415301269,-2.71151708982905,-2.71045304966401,-2.70931078535952,
-2.70767789881456,-2.70318312066917,-2.6274618114087,-2.57999225754786,
-2.56100584430165,-2.55211729444739,-2.55060365242198,-2.54980545212675,
-2.54915674747659,-2.54848925227222,-2.54723492120474,-2.54297419876359,
-2.46825245337991,-2.42518176196537,-2.39958028004199,-2.39457957936221,
-2.39085184157743,-2.38922074391765,-2.38802093522189,-2.38691357520513,
-2.38541184504491,-2.38247667044703,-2.35929748178034,-2.31414790645294,
-2.2819212021583,-2.23071364865202,-2.22844550226923,-2.22750401836176,
-2.22683024931546,-2.22621484794584,-2.22538203818414,-2.2237591490883,
-2.21132399982757,-2.16807127052786,-2.07508815950537,-2.06902094982162,
-2.06704206294794,-2.06577094108367,-2.06457819216111,-2.063015855784,-2.05956960918846,
-2.03105717956733,-2.00702157703462,-1.91104810427369,-1.90643614223651,
-1.90515820225468,-1.90440396505848,-1.90374781561744,-1.90292795987113,
-1.90131090314939,-1.88974973895514,-1.86303615956141,-1.78708628620946,
-1.77050865476943,-1.768066239237,-1.74835512299657,-1.7452427821876,-1.74372775713779,
-1.74254556189619,-1.74124026775414,-1.73910857642669,-1.73169313223271,
-1.6847308934884,-1.58824861224914,-1.58371127302196,-1.58244111285369,
-1.58168862202532,-1.58103841231353,-1.5802188904055,-1.57860382618543,
-1.567109268723,-1.54103214993805,-1.45498255754657,-1.42610875346996,-1.42269540566677,
-1.42125654028859,-1.42005525691236,-1.41882144519868,-1.41701632136877,
-1.41222690598796,-1.38930497769127,-1.36747994346505,-1.30893316381916,
-1.26336342523369,-1.2605951854004,-1.25964650128379,-1.25899973285973,
-1.2583546245898,-1.25753775615542,-1.25664527292953,-1.25519867888632,
-1.25234023328002,-1.22282720796652,-1.1308768098669,-1.10336912046584,
-1.099954050715,-1.09839733624122,-1.09720534590314,-1.09593159984851,-1.09394153857412,
-1.08778537776143,-1.05319185522816,-0.954433927690995,-0.939271681188969,
-0.937365789773948,-0.936498282402379,-0.935834520564802,-0.935129764184481,
-0.934015247787698,-0.9326992359398,-0.930189792521849,-0.906652854563262,
-0.858764365074775,-0.810255190078082,-0.780751228228655,-0.777621407962522,
-0.776070082383189,-0.774949650967242,-0.773757677457121,-0.772175174364369,
-0.768714402940023,-0.69757279831974,-0.626581586851115,-0.616278170201482,
-0.614573646300439,-0.613735856085354,-0.613077894237505,-0.612350165405804,
-0.611133045536139,-0.609669120482026,-0.606763805025855,-0.599378371739643,
-0.584169490896696,-0.551745190069182,-0.479834604328143,-0.474486626748439,
-0.457267742756472,-0.454316107312384,-0.452812902396344,-0.451631818085496,
-0.450319406434124,-0.448157019163733,-0.440443618830817,-0.414593179621914,
-0.365307984260105,-0.343551717664757,-0.312535330181327,-0.311562542197397,
-0.294071376256208,-0.292091891959814,-0.291290060812106,-0.290621365244334,
-0.290006759448331,-0.289047561039487,-0.286679245035633,-0.28332756548136,
-0.274348609237957,-0.249983084694278,-0.166218929541401,-0.160422800612661,
-0.154834242937302,-0.134827997608625,-0.131701641017142,-0.130183645579306,
-0.129000875424188,-0.127696717029503,-0.125570869464186,-0.118214375946852,
-0.0718901686108905,-0.000958363168410272),.UNSPECIFIED.);
#879=B_SPLINE_CURVE_WITH_KNOTS('',3,(#66352,#66353,#66354,#66355,#66356,
#66357,#66358,#66359,#66360,#66361,#66362,#66363,#66364,#66365,#66366,#66367,
#66368,#66369,#66370,#66371,#66372,#66373,#66374,#66375,#66376,#66377,#66378,
#66379,#66380,#66381,#66382,#66383,#66384,#66385,#66386,#66387,#66388,#66389,
#66390,#66391,#66392,#66393,#66394,#66395,#66396,#66397,#66398,#66399,#66400,
#66401,#66402,#66403,#66404,#66405,#66406,#66407,#66408,#66409,#66410,#66411,
#66412,#66413,#66414,#66415,#66416,#66417,#66418,#66419,#66420,#66421,#66422,
#66423,#66424,#66425,#66426,#66427,#66428,#66429,#66430,#66431,#66432,#66433,
#66434,#66435,#66436,#66437,#66438,#66439,#66440,#66441,#66442,#66443,#66444,
#66445,#66446,#66447,#66448,#66449,#66450,#66451,#66452,#66453,#66454,#66455,
#66456,#66457,#66458,#66459,#66460,#66461,#66462,#66463,#66464,#66465,#66466,
#66467,#66468,#66469,#66470,#66471,#66472,#66473,#66474,#66475,#66476,#66477,
#66478,#66479,#66480,#66481,#66482,#66483,#66484,#66485,#66486,#66487,#66488,
#66489,#66490,#66491,#66492,#66493,#66494,#66495,#66496,#66497,#66498,#66499,
#66500,#66501,#66502,#66503,#66504,#66505,#66506,#66507,#66508,#66509,#66510,
#66511,#66512,#66513,#66514,#66515,#66516,#66517,#66518,#66519,#66520,#66521,
#66522,#66523,#66524,#66525,#66526,#66527,#66528,#66529,#66530,#66531,#66532,
#66533,#66534,#66535,#66536,#66537,#66538,#66539,#66540,#66541,#66542,#66543,
#66544,#66545,#66546,#66547,#66548,#66549,#66550,#66551,#66552,#66553,#66554,
#66555,#66556,#66557,#66558,#66559,#66560,#66561,#66562,#66563,#66564,#66565,
#66566,#66567,#66568,#66569,#66570,#66571,#66572,#66573,#66574,#66575,#66576,
#66577,#66578,#66579,#66580,#66581,#66582,#66583,#66584,#66585,#66586,#66587,
#66588,#66589,#66590,#66591,#66592,#66593,#66594,#66595,#66596,#66597,#66598,
#66599,#66600,#66601,#66602,#66603,#66604,#66605,#66606,#66607,#66608,#66609,
#66610,#66611,#66612,#66613,#66614,#66615,#66616,#66617,#66618,#66619,#66620,
#66621,#66622,#66623,#66624,#66625,#66626,#66627,#66628,#66629,#66630,#66631,
#66632,#66633,#66634,#66635,#66636,#66637,#66638,#66639,#66640,#66641,#66642,
#66643,#66644,#66645,#66646,#66647,#66648,#66649,#66650,#66651,#66652,#66653,
#66654,#66655,#66656,#66657,#66658,#66659,#66660,#66661,#66662,#66663,#66664,
#66665,#66666,#66667,#66668,#66669,#66670,#66671,#66672,#66673,#66674,#66675,
#66676,#66677,#66678,#66679,#66680,#66681,#66682,#66683,#66684,#66685,#66686,
#66687,#66688,#66689,#66690,#66691,#66692,#66693,#66694,#66695,#66696,#66697,
#66698,#66699,#66700,#66701,#66702,#66703,#66704,#66705,#66706,#66707,#66708,
#66709,#66710,#66711,#66712,#66713,#66714,#66715,#66716,#66717,#66718,#66719,
#66720,#66721,#66722,#66723,#66724,#66725,#66726,#66727,#66728,#66729,#66730,
#66731,#66732,#66733,#66734,#66735,#66736,#66737,#66738,#66739,#66740,#66741,
#66742,#66743,#66744,#66745,#66746,#66747,#66748,#66749,#66750,#66751,#66752,
#66753,#66754,#66755,#66756,#66757,#66758,#66759,#66760,#66761,#66762,#66763,
#66764,#66765,#66766,#66767,#66768,#66769,#66770,#66771,#66772,#66773,#66774,
#66775,#66776,#66777,#66778,#66779,#66780,#66781,#66782,#66783,#66784,#66785,
#66786,#66787,#66788,#66789,#66790,#66791,#66792,#66793,#66794,#66795,#66796,
#66797,#66798,#66799,#66800,#66801,#66802,#66803,#66804,#66805,#66806,#66807,
#66808,#66809,#66810,#66811,#66812,#66813,#66814,#66815,#66816,#66817,#66818,
#66819,#66820,#66821,#66822,#66823,#66824,#66825,#66826,#66827,#66828,#66829,
#66830,#66831,#66832,#66833,#66834,#66835,#66836,#66837,#66838,#66839,#66840,
#66841,#66842,#66843,#66844,#66845,#66846,#66847,#66848,#66849,#66850,#66851,
#66852,#66853,#66854,#66855,#66856,#66857,#66858,#66859,#66860,#66861,#66862,
#66863,#66864,#66865,#66866,#66867,#66868,#66869,#66870,#66871,#66872,#66873,
#66874,#66875),.UNSPECIFIED.,.F.,.F.,(4,2,2,2,2,2,2,2,2,2,2,2,2,2,2,2,2,
2,2,2,2,2,2,2,2,2,2,2,2,2,2,2,2,2,2,2,2,2,2,2,2,2,2,2,2,2,2,2,2,2,2,2,2,
2,2,2,2,2,2,2,2,2,2,2,2,2,2,2,2,2,2,2,2,2,2,2,2,2,2,2,2,2,2,2,2,2,2,2,2,
2,2,2,2,2,2,2,2,2,2,2,2,2,2,2,2,2,2,2,2,2,2,2,2,2,2,2,2,2,2,2,2,2,2,2,2,
2,2,2,2,2,2,2,2,2,2,2,2,2,2,2,2,2,2,2,2,2,2,2,2,2,2,2,2,2,2,2,2,2,2,2,2,
2,2,2,2,2,2,2,2,2,2,2,2,2,2,2,2,2,2,2,2,2,2,2,2,2,2,2,2,2,2,2,2,2,2,2,2,
2,2,2,2,2,2,2,2,2,2,2,2,2,2,2,2,2,2,2,2,2,2,2,2,2,2,2,2,2,2,2,2,2,2,2,2,
2,2,2,2,2,2,2,2,2,2,2,2,2,2,2,2,2,2,2,2,2,2,2,2,2,2,2,2,4),(-4.0592502292357,
-4.02971377170784,-4.02833269367985,-4.02746777430755,-4.02681359033491,
-4.02618885191426,-4.02556907401911,-4.02471842136597,-4.02258008547932,
-3.99619692647021,-3.99159020568108,-3.92268324987285,-3.87624072683285,
-3.86887460694005,-3.86674882885036,-3.86544533951018,-3.86426358736687,
-3.86274747144284,-3.85962701790925,-3.83971133977558,-3.82304306502926,
-3.75513412111111,-3.73670470144439,-3.71631718798715,-3.7098965427674,
-3.70727566583918,-3.70532732615901,-3.70444490606196,-3.70382204043842,
-3.70320515508762,-3.70236569461928,-3.70029210282313,-3.67728266226473,
-3.62864470595126,-3.62291915087168,-3.61624333686055,-3.54916689486743,
-3.54541358994127,-3.54377844458771,-3.54257841023991,-3.54147277627322,
-3.53997632801371,-3.53706013624253,-3.5143664509238,-3.5052048861805,-3.41996440525756,
-3.39460006666537,-3.38771279179005,-3.38495326888161,-3.38354357269005,
-3.38236500195798,-3.38164576818019,-3.3809867545542,-3.38013578421831,
-3.37836292286758,-3.36659149151968,-3.3636358336911,-3.2778147509822,-3.23134723132067,
-3.22397866204519,-3.22185258015306,-3.22054899309389,-3.21936721048809,
-3.2178511364515,-3.21473105609792,-3.19482525808929,-3.18825160183172,
-3.11370804105403,-3.06668622824333,-3.0631138819864,-3.06141123410297,
-3.06041321938472,-3.0595207907915,-3.05886477210674,-3.05824478785809,
-3.05739344426438,-3.0552512575727,-3.02865686272347,-2.95230316484772,
-2.90388431078029,-2.90033793925088,-2.89874025406815,-2.89754656823444,
-2.89643157732694,-2.89489885865933,-2.89102271432198,-2.83407452147374,
-2.7667328697092,-2.74237768966846,-2.73981910032576,-2.7384847442697,-2.73735689928254,
-2.73664973245552,-2.73598741618292,-2.73512677991275,-2.73332279376308,
-2.7202622809692,-2.71964177312284,-2.68191441981314,-2.61253353497769,
-2.58680342430162,-2.5791449196508,-2.57698914262429,-2.57567887487318,
-2.57449851244917,-2.57299456888179,-2.57003624549943,-2.55265920153993,
-2.45741639898088,-2.43142372570276,-2.41695347429834,-2.41525540123041,
-2.41441925148273,-2.41382352781453,-2.41318995664229,-2.41210369268551,
-2.40912387498563,-2.35756011545445,-2.32850505275292,-2.29693371639008,
-2.26245477784835,-2.2563114507617,-2.25432343355344,-2.25305045845657,
-2.25185880975524,-2.25030199594488,-2.24688450374002,-2.21927023589699,
-2.13137524934467,-2.09503498197563,-2.09295846718097,-2.0920503966135,
-2.09138274518819,-2.09075965091689,-2.08989683886026,-2.08768843487486,
-2.05691851562357,-2.03119195075069,-1.95735863467018,-1.93586025489425,
-1.93266915324815,-1.9311552378453,-1.92997011807192,-1.92867768443113,
-1.92660251406883,-1.91971167549072,-1.8781458032303,-1.77487154754452,
-1.77096377132384,-1.76975113397566,-1.76909204296414,-1.76843626896615,
-1.76762100008687,-1.76602598860223,-1.75511136260808,-1.72730942662431,
-1.66994103917675,-1.64308089446468,-1.61364135102043,-1.61051385077805,
-1.60896330027604,-1.60784325334014,-1.60665152606785,-1.60506907267428,
-1.60160730478632,-1.52967363334016,-1.45273193869247,-1.448430641462,-1.44717160899822,
-1.44650311679914,-1.44585439215727,-1.44505751695631,-1.44355038913142,
-1.43480570025145,-1.41610331917782,-1.37136114636524,-1.29271074443671,
-1.28807249694865,-1.28641781882221,-1.28526945479591,-1.2841128575556,
-1.28265385833431,-1.28106721332884,-1.27851257388335,-1.27351909193643,
-1.24793397391805,-1.20489056377862,-1.13003927289164,-1.12577025917861,
-1.12451486847455,-1.12384709686803,-1.12319830560107,-1.12240025803603,
-1.1208876758493,-1.11202581912504,-1.09308930954775,-1.04646452103335,
-0.969930824152034,-0.965385320340384,-0.96374438552121,-0.962599800057412,
-0.961442595319757,-0.9599747409644,-0.958375981601473,-0.955792497741351,
-0.950721935870888,-0.924899515604346,-0.881376751963629,-0.807278818911658,
-0.803095157629477,-0.801849542657765,-0.801183726072711,-0.800528500246564,
-0.799724396747227,-0.798183239424336,-0.78867194895334,-0.775982822829522,
-0.770383974634293,-0.716610071917506,-0.646715215280458,-0.642573382785571,
-0.640995997405014,-0.63986869899485,-0.638704119463013,-0.637189273524821,
-0.635525592149643,-0.632786857356244,-0.579740233152768,-0.485086588406905,
-0.480433681635539,-0.479151226984352,-0.478395807306426,-0.477739576910882,
-0.47692083945773,-0.475309867177421,-0.463943027569456,-0.434065962925085,
-0.388476760758934,-0.323616948547831,-0.319708153250979,-0.318169182260372,
-0.317051950443698,-0.315881899024113,-0.314333558453753,-0.312623608305136,
-0.30977383667544,-0.246378726847262,-0.181458022257683,-0.17686737633803,
-0.172939757871662,-0.172074784825208,-0.170796326286433,-0.158563831078692,
-0.156948577082422,-0.156117568360779,-0.155502457131242,-0.154827920537826,
-0.153883441010261,-0.151598853725842,-0.0880982192293773,-0.0144811591141122,
-0.000957555802355253),.UNSPECIFIED.);
#880=B_SPLINE_CURVE_WITH_KNOTS('',3,(#66877,#66878,#66879,#66880,#66881,
#66882,#66883,#66884,#66885,#66886,#66887,#66888,#66889,#66890,#66891,#66892,
#66893,#66894,#66895,#66896,#66897,#66898,#66899,#66900,#66901,#66902,#66903,
#66904,#66905,#66906,#66907,#66908,#66909,#66910,#66911,#66912,#66913,#66914,
#66915,#66916,#66917,#66918,#66919,#66920,#66921,#66922,#66923,#66924,#66925,
#66926,#66927,#66928,#66929,#66930,#66931,#66932,#66933,#66934,#66935,#66936,
#66937,#66938,#66939,#66940,#66941,#66942,#66943,#66944,#66945,#66946,#66947,
#66948,#66949,#66950,#66951,#66952,#66953,#66954,#66955,#66956,#66957,#66958,
#66959,#66960,#66961,#66962,#66963,#66964,#66965,#66966,#66967,#66968,#66969,
#66970,#66971,#66972,#66973,#66974,#66975,#66976,#66977,#66978,#66979,#66980,
#66981,#66982,#66983,#66984,#66985,#66986,#66987,#66988,#66989,#66990,#66991,
#66992,#66993,#66994,#66995,#66996,#66997,#66998,#66999,#67000,#67001,#67002,
#67003,#67004,#67005,#67006,#67007,#67008,#67009,#67010,#67011,#67012,#67013,
#67014,#67015,#67016,#67017,#67018,#67019,#67020,#67021,#67022,#67023,#67024,
#67025,#67026,#67027,#67028,#67029,#67030,#67031,#67032,#67033,#67034,#67035,
#67036,#67037,#67038,#67039,#67040,#67041,#67042,#67043,#67044,#67045,#67046,
#67047,#67048,#67049,#67050,#67051,#67052,#67053,#67054,#67055,#67056,#67057,
#67058,#67059,#67060,#67061,#67062,#67063,#67064,#67065,#67066,#67067,#67068,
#67069,#67070,#67071,#67072,#67073,#67074,#67075,#67076,#67077,#67078,#67079,
#67080,#67081,#67082,#67083,#67084,#67085,#67086,#67087,#67088,#67089,#67090,
#67091,#67092,#67093,#67094,#67095,#67096,#67097,#67098,#67099,#67100,#67101,
#67102,#67103,#67104,#67105,#67106,#67107,#67108,#67109,#67110,#67111,#67112,
#67113,#67114,#67115,#67116,#67117,#67118,#67119,#67120,#67121,#67122,#67123,
#67124,#67125,#67126,#67127,#67128,#67129,#67130,#67131,#67132,#67133,#67134,
#67135,#67136,#67137,#67138,#67139,#67140,#67141,#67142,#67143,#67144,#67145,
#67146,#67147,#67148,#67149,#67150,#67151,#67152,#67153,#67154,#67155,#67156,
#67157,#67158,#67159,#67160,#67161,#67162,#67163,#67164,#67165,#67166,#67167,
#67168,#67169,#67170,#67171,#67172,#67173,#67174,#67175,#67176,#67177,#67178,
#67179,#67180,#67181,#67182,#67183,#67184,#67185,#67186,#67187,#67188,#67189,
#67190,#67191,#67192,#67193,#67194,#67195,#67196,#67197,#67198,#67199,#67200,
#67201,#67202,#67203,#67204,#67205,#67206,#67207,#67208,#67209,#67210,#67211,
#67212,#67213,#67214,#67215,#67216,#67217,#67218,#67219,#67220,#67221,#67222,
#67223,#67224,#67225,#67226,#67227,#67228,#67229,#67230,#67231,#67232,#67233,
#67234,#67235,#67236,#67237,#67238,#67239,#67240,#67241,#67242,#67243,#67244,
#67245,#67246,#67247,#67248,#67249,#67250,#67251,#67252,#67253,#67254,#67255,
#67256,#67257,#67258,#67259,#67260,#67261,#67262,#67263,#67264,#67265,#67266,
#67267,#67268,#67269,#67270,#67271,#67272,#67273,#67274,#67275,#67276,#67277,
#67278,#67279,#67280,#67281,#67282,#67283,#67284,#67285,#67286,#67287,#67288,
#67289,#67290,#67291,#67292,#67293,#67294,#67295,#67296,#67297,#67298,#67299,
#67300,#67301,#67302,#67303,#67304,#67305,#67306,#67307,#67308,#67309,#67310,
#67311,#67312,#67313,#67314,#67315,#67316,#67317,#67318,#67319,#67320,#67321,
#67322,#67323,#67324,#67325,#67326,#67327,#67328,#67329,#67330,#67331,#67332,
#67333,#67334,#67335,#67336,#67337,#67338,#67339,#67340,#67341,#67342,#67343,
#67344,#67345,#67346,#67347,#67348,#67349,#67350,#67351,#67352,#67353,#67354,
#67355,#67356,#67357,#67358,#67359,#67360,#67361,#67362,#67363,#67364,#67365,
#67366,#67367,#67368,#67369,#67370,#67371,#67372,#67373,#67374,#67375,#67376,
#67377,#67378,#67379,#67380,#67381,#67382,#67383,#67384,#67385,#67386,#67387,
#67388,#67389,#67390,#67391,#67392,#67393,#67394,#67395,#67396,#67397,#67398,
#67399,#67400,#67401,#67402,#67403,#67404,#67405,#67406,#67407,#67408,#67409,
#67410,#67411,#67412,#67413,#67414,#67415,#67416,#67417,#67418),
 .UNSPECIFIED.,.F.,.F.,(4,2,2,2,2,2,2,2,2,2,2,2,2,2,2,2,2,2,2,2,2,2,2,2,
2,2,2,2,2,2,2,2,2,2,2,2,2,2,2,2,2,2,2,2,2,2,2,2,2,2,2,2,2,2,2,2,2,2,2,2,
2,2,2,2,2,2,2,2,2,2,2,2,2,2,2,2,2,2,2,2,2,2,2,2,2,2,2,2,2,2,2,2,2,2,2,2,
2,2,2,2,2,2,2,2,2,2,2,2,2,2,2,2,2,2,2,2,2,2,2,2,2,2,2,2,2,2,2,2,2,2,2,2,
2,2,2,2,2,2,2,2,2,2,2,2,2,2,2,2,2,2,2,2,2,2,2,2,2,2,2,2,2,2,2,2,2,2,2,2,
2,2,2,2,2,2,2,2,2,2,2,2,2,2,2,2,2,2,2,2,2,2,2,2,2,2,2,2,2,2,2,2,2,2,2,2,
2,2,2,2,2,2,2,2,2,2,2,2,2,2,2,2,2,2,2,2,2,2,2,2,2,2,2,2,2,2,2,2,2,2,2,2,
2,2,2,2,2,2,2,2,2,2,2,2,2,2,2,2,2,2,2,2,2,2,2,2,2,2,2,2,2,2,4),(-4.06075182852026,
-4.05713602550796,-4.05572147461755,-4.05459203620983,-4.0534262098459,
-4.05225574680044,-4.0501453121058,-4.04365868504524,-3.93391486943271,
-3.89929173805632,-3.89456217807212,-3.8933161697968,-3.89257642336149,
-3.89191804550264,-3.89107565595412,-3.88940512112919,-3.87935627056182,
-3.83475399024018,-3.74391097474562,-3.73808824921845,-3.73522832452903,
-3.73351427019815,-3.73196323873318,-3.73079301518622,-3.72967701783565,
-3.7281421547425,-3.72425659274861,-3.66619413419257,-3.6363178160674,-3.62747131263969,
-3.5996676191543,-3.58172716477806,-3.57239894599916,-3.5708656880108,-3.57006329542363,
-3.5694715979636,-3.56882229406063,-3.56765835910751,-3.56413407376746,
-3.50389499509457,-3.45509133257403,-3.43817666677135,-3.42189973085289,
-3.4157753982106,-3.41280697835267,-3.4110480498888,-3.40946460323284,-3.40828903924013,
-3.40718159558842,-3.40567985639861,-3.40198686785289,-3.36009545553401,
-3.30118335719606,-3.28918429248858,-3.2540962543738,-3.24933314381725,
-3.24808416229119,-3.24734379640251,-3.2466856119475,-3.24584446897499,
-3.24412260257951,-3.23346870618805,-3.14870615885526,-3.09745153153282,
-3.09231801730517,-3.08971107510054,-3.08810251736758,-3.08662922778336,
-3.08547022964981,-3.08432882997043,-3.08269926861627,-3.07822669187297,
-3.0029671837174,-2.95540075120341,-2.93626788314443,-2.92713838241178,
-2.92561382195227,-2.92481327492123,-2.92422177103945,-2.92347615173796,
-2.922203586898,-2.9177809451957,-2.82886227321155,-2.7750063201366,-2.76973573344294,
-2.76707794289168,-2.76544812931981,-2.76395787734161,-2.7627969803059,
-2.76166129666719,-2.76005249720835,-2.75571279887429,-2.68771464048416,
-2.64300429590222,-2.61654839721385,-2.60464128573738,-2.60301319471541,
-2.60219109673491,-2.60154079080291,-2.60079038371751,-2.59952871334197,
-2.59506884112714,-2.5041145795129,-2.44635922355543,-2.44294910763652,
-2.44137646058749,-2.44018635208269,-2.43906357260995,-2.43719285820363,
-2.43235742893389,-2.3556186039616,-2.31463915416349,-2.29464276974331,
-2.28199443833417,-2.28034404794254,-2.27951741639506,-2.27892289654618,
-2.27828520280973,-2.27717881467369,-2.27406612251968,-2.21848179217728,
-2.16798442556103,-2.12365006701894,-2.12033520914686,-2.11878068161532,
-2.11759325401149,-2.11646475329001,-2.11456472847643,-2.10954640706296,
-2.03056631304233,-1.98625197267401,-1.96020852560816,-1.95807541347298,
-1.95722540624879,-1.9566055912339,-1.95593544386434,-1.95501367391308,
-1.95286030009851,-1.91733023238687,-1.82973793937463,-1.80119276547675,
-1.79774541700403,-1.7961828540386,-1.79499004423848,-1.79371896620784,
-1.79174037100798,-1.78567576394416,-1.69272447714349,-1.63900010488334,
-1.63575159526142,-1.63462576434238,-1.63398414622884,-1.6333907204264,
-1.63257283279629,-1.63096523114785,-1.61968703672752,-1.59022259506031,
-1.49518191015856,-1.49267422447255,-1.47752745360438,-1.47494503232474,
-1.47339660143541,-1.47220609673132,-1.47092918442724,-1.46892427052881,
-1.46264409090269,-1.42690999405084,-1.32154755052495,-1.3146200421444,
-1.31251930649618,-1.31167479258714,-1.3110563284359,-1.31039906930294,
-1.30949922829901,-1.30849058227328,-1.30676236431469,-1.257671083213,-1.18186317266664,
-1.17475107311608,-1.155135983372,-1.15202787791082,-1.15051360792592,-1.14933140816592,
-1.14802550415524,-1.14589144944102,-1.13845443727308,-1.09126263659276,
-1.01569115322376,-0.991932213817203,-0.98984229359769,-0.988999638701811,
-0.988381639070366,-0.987723788123036,-0.986822593831915,-0.985811346896852,
-0.984076772760184,-0.980413871624433,-0.955831890316237,-0.906774771954784,
-0.86096833305819,-0.833014917578596,-0.829585267799973,-0.828025701130271,
-0.826833098888544,-0.82556022544062,-0.823574680047915,-0.817456864744306,
-0.783215387031529,-0.768835710602314,-0.683196082462364,-0.682162536409167,
-0.680308173655444,-0.668726863554091,-0.666961477934312,-0.666120676476328,
-0.66548236205044,-0.664770917480712,-0.663625614522972,-0.662266381104344,
-0.659642642599554,-0.653214775777888,-0.632740345273278,-0.583319172724665,
-0.535379122049546,-0.529824524948346,-0.509872094008693,-0.506747968409015,
-0.505230323206139,-0.504047494304743,-0.502742934345031,-0.500615673948938,
-0.49324697151785,-0.446795938016764,-0.4361108543253,-0.427447163777085,
-0.420143277630098,-0.413835415115689,-0.408291773102417,-0.350202709489139,
-0.345362526340499,-0.344060842045815,-0.343300938166315,-0.342646684094746,
-0.34185101991378,-0.340331163160333,-0.33840631424111,-0.334186616723762,
-0.321861649607299,-0.300194475951382,-0.204487071698002,-0.186940368902747,
-0.183971731609116,-0.182464963680236,-0.181283563882519,-0.179973357195922,
-0.17782045512056,-0.170200196877061,-0.14453194325761,-0.116681991627422,
-0.0410510682472698,-0.0368848661310568,-0.0355407581861974,-0.0233865722114733,
-0.021596184330195,-0.0207505582788536,-0.0201095965444524,-0.0194954147846064,
-0.0187829799930978,-0.0177682625203108,-0.0160252307618027,-0.000956555014723939),
 .UNSPECIFIED.);
#881=B_SPLINE_CURVE_WITH_KNOTS('',3,(#67420,#67421,#67422,#67423,#67424,
#67425,#67426,#67427,#67428,#67429,#67430,#67431,#67432,#67433,#67434,#67435,
#67436,#67437,#67438,#67439,#67440,#67441,#67442,#67443,#67444,#67445,#67446,
#67447,#67448,#67449,#67450,#67451,#67452,#67453,#67454,#67455,#67456,#67457,
#67458,#67459,#67460,#67461,#67462,#67463,#67464,#67465,#67466,#67467,#67468,
#67469,#67470,#67471,#67472,#67473,#67474,#67475,#67476,#67477,#67478,#67479,
#67480,#67481,#67482,#67483,#67484,#67485,#67486,#67487,#67488,#67489,#67490,
#67491,#67492,#67493,#67494,#67495,#67496,#67497,#67498,#67499,#67500,#67501,
#67502,#67503,#67504,#67505,#67506,#67507,#67508,#67509,#67510,#67511,#67512,
#67513,#67514,#67515,#67516,#67517,#67518,#67519,#67520,#67521,#67522,#67523,
#67524,#67525,#67526,#67527,#67528,#67529,#67530,#67531,#67532,#67533,#67534,
#67535,#67536,#67537,#67538,#67539,#67540,#67541,#67542,#67543,#67544,#67545,
#67546,#67547,#67548,#67549,#67550,#67551,#67552,#67553,#67554,#67555,#67556,
#67557,#67558,#67559,#67560,#67561,#67562,#67563,#67564,#67565,#67566,#67567,
#67568,#67569,#67570,#67571,#67572,#67573,#67574,#67575,#67576,#67577,#67578,
#67579,#67580,#67581,#67582,#67583,#67584,#67585,#67586,#67587,#67588,#67589,
#67590,#67591,#67592,#67593,#67594,#67595,#67596,#67597,#67598,#67599,#67600,
#67601,#67602,#67603,#67604,#67605,#67606,#67607,#67608,#67609,#67610,#67611,
#67612,#67613,#67614,#67615,#67616,#67617,#67618,#67619,#67620,#67621,#67622,
#67623,#67624,#67625,#67626,#67627,#67628,#67629,#67630,#67631,#67632,#67633,
#67634,#67635,#67636,#67637,#67638,#67639,#67640,#67641,#67642,#67643,#67644,
#67645,#67646,#67647,#67648,#67649,#67650,#67651,#67652,#67653,#67654,#67655,
#67656,#67657,#67658,#67659,#67660,#67661,#67662,#67663,#67664,#67665,#67666,
#67667,#67668,#67669,#67670,#67671,#67672,#67673,#67674,#67675,#67676,#67677,
#67678,#67679,#67680,#67681,#67682,#67683,#67684,#67685,#67686,#67687,#67688,
#67689,#67690,#67691,#67692,#67693,#67694,#67695,#67696,#67697,#67698,#67699,
#67700,#67701,#67702,#67703,#67704,#67705,#67706,#67707,#67708,#67709,#67710,
#67711,#67712,#67713,#67714,#67715,#67716,#67717,#67718,#67719,#67720,#67721,
#67722,#67723,#67724,#67725,#67726,#67727,#67728,#67729,#67730,#67731,#67732,
#67733,#67734,#67735,#67736,#67737,#67738,#67739,#67740,#67741,#67742,#67743,
#67744,#67745,#67746,#67747,#67748,#67749,#67750,#67751,#67752,#67753,#67754,
#67755,#67756,#67757,#67758,#67759,#67760,#67761,#67762,#67763,#67764,#67765,
#67766,#67767,#67768,#67769,#67770,#67771,#67772,#67773,#67774,#67775,#67776,
#67777,#67778,#67779,#67780,#67781,#67782,#67783,#67784,#67785,#67786,#67787,
#67788,#67789,#67790,#67791,#67792,#67793,#67794,#67795,#67796,#67797,#67798,
#67799,#67800,#67801,#67802,#67803,#67804,#67805,#67806,#67807,#67808,#67809,
#67810,#67811,#67812,#67813,#67814,#67815,#67816,#67817,#67818,#67819,#67820,
#67821,#67822,#67823,#67824,#67825,#67826,#67827,#67828,#67829,#67830,#67831,
#67832,#67833,#67834,#67835,#67836,#67837,#67838,#67839,#67840,#67841,#67842,
#67843,#67844,#67845,#67846,#67847,#67848,#67849,#67850,#67851,#67852,#67853,
#67854,#67855,#67856,#67857,#67858,#67859,#67860,#67861,#67862,#67863,#67864,
#67865,#67866,#67867,#67868,#67869,#67870,#67871,#67872,#67873,#67874,#67875,
#67876,#67877,#67878,#67879,#67880,#67881,#67882,#67883,#67884,#67885,#67886,
#67887,#67888,#67889,#67890,#67891,#67892,#67893,#67894,#67895,#67896,#67897,
#67898,#67899,#67900,#67901,#67902,#67903,#67904,#67905,#67906,#67907,#67908,
#67909,#67910,#67911,#67912,#67913,#67914,#67915,#67916,#67917,#67918,#67919,
#67920,#67921,#67922,#67923,#67924,#67925,#67926,#67927,#67928,#67929,#67930,
#67931,#67932,#67933,#67934,#67935,#67936,#67937,#67938,#67939,#67940,#67941,
#67942,#67943,#67944,#67945,#67946,#67947,#67948,#67949),.UNSPECIFIED.,
 .F.,.F.,(4,2,2,2,2,2,2,2,2,2,2,2,2,2,2,2,2,2,2,2,2,2,2,2,2,2,2,2,2,2,2,
2,2,2,2,2,2,2,2,2,2,2,2,2,2,2,2,2,2,2,2,2,2,2,2,2,2,2,2,2,2,2,2,2,2,2,2,
2,2,2,2,2,2,2,2,2,2,2,2,2,2,2,2,2,2,2,2,2,2,2,2,2,2,2,2,2,2,2,2,2,2,2,2,
2,2,2,2,2,2,2,2,2,2,2,2,2,2,2,2,2,2,2,2,2,2,2,2,2,2,2,2,2,2,2,2,2,2,2,2,
2,2,2,2,2,2,2,2,2,2,2,2,2,2,2,2,2,2,2,2,2,2,2,2,2,2,2,2,2,2,2,2,2,2,2,2,
2,2,2,2,2,2,2,2,2,2,2,2,2,2,2,2,2,2,2,2,2,2,2,2,2,2,2,2,2,2,2,2,2,2,2,2,
2,2,2,2,2,2,2,2,2,2,2,2,2,2,2,2,2,2,2,2,2,2,2,2,2,2,2,2,2,2,2,2,2,2,2,2,
2,2,2,2,2,2,2,2,2,2,2,2,2,2,2,2,2,4),(-4.06084443590171,-3.97731844721829,
-3.93012302769939,-3.92268671047794,-3.92055359085664,-3.91924841914854,
-3.91806698699717,-3.91655384555902,-3.91344856904977,-3.89386413803157,
-3.88842159406268,-3.88089843136169,-3.79607080323638,-3.78292953552254,
-3.76765849608381,-3.76272957180426,-3.76057197191954,-3.75890746928953,
-3.75808042143403,-3.75744175032905,-3.75680184122872,-3.75587690222132,
-3.75326843823274,-3.69679524389133,-3.65912322151103,-3.6188521365159,
-3.6013974109016,-3.59862125802278,-3.59717535706437,-3.59611291663646,
-3.5949666115149,-3.59331816108274,-3.58871831869473,-3.58692534334826,
-3.48321037349395,-3.45341045788923,-3.44305029103678,-3.43933112039623,
-3.43757725524908,-3.43655829868936,-3.43565087655506,-3.43499188242287,
-3.43437530588361,-3.43353751199936,-3.43189485329819,-3.41890703208826,
-3.37418909144057,-3.33029027840057,-3.27997440763444,-3.27645134742111,
-3.27485771137402,-3.27366442825823,-3.27254791114154,-3.27101010929729,
-3.26710538130226,-3.20394976652324,-3.12055093104217,-3.11680133934631,
-3.11503688294052,-3.11401358039626,-3.11310367186522,-3.11244391816564,
-3.1118280258814,-3.11099313167253,-3.10936199057641,-3.0966993724259,-3.09381984545065,
-3.093478029282,-2.99528169901182,-2.9608008203631,-2.95465709029732,-2.95266892414645,
-2.9513958489468,-2.95020410319279,-2.94864715778687,-2.94522935727576,
-2.91761183553983,-2.82958504033269,-2.81039042432415,-2.79460568111286,
-2.79260839411531,-2.79149151042415,-2.79073712703266,-2.7900189074072,
-2.78937618016919,-2.78853174954314,-2.78679278594318,-2.77577492449043,
-2.70487375518483,-2.66572993117447,-2.64004815008967,-2.63502120430159,
-2.63127786836222,-2.62964410642004,-2.62844394520468,-2.62733739106485,
-2.62583847580987,-2.62291388032471,-2.60001453652611,-2.58450843031352,
-2.50841007158774,-2.48167750172757,-2.47013015376645,-2.46851372447391,
-2.46769406938381,-2.46703802300443,-2.46628383865707,-2.46500584022129,
-2.46039222868414,-2.36602724824773,-2.34292561561298,-2.3175308128802,
-2.30980485047108,-2.30764189774675,-2.30632976751042,-2.30514933912842,
-2.30364752055451,-2.30070034169906,-2.28354619511033,-2.18872419607834,
-2.15878715882718,-2.14741069613728,-2.14579986480449,-2.1449813418037,
-2.14438786971759,-2.14374660745554,-2.14262241561173,-2.13938528123742,
-2.08114588283808,-2.03157579402172,-2.01307693557964,-2.00797983300827,
-1.98878667378008,-1.98569870450949,-1.98418858696784,-1.98300704543098,
-1.98169922705864,-1.979556047706,-1.9720280966689,-1.92383814060439,-1.82889908868079,
-1.82422440359268,-1.82293983081376,-1.8221840032555,-1.82152795431853,
-1.82071013145765,-1.81910314005874,-1.80784754246262,-1.77418251211763,
-1.67006548941637,-1.66862339036771,-1.66375430990932,-1.66187806205275,
-1.66075414973902,-1.65956446989974,-1.65799513476366,-1.65460292151076,
-1.60011961093511,-1.50588822765113,-1.50134050655198,-1.50006927380101,
-1.4993165517208,-1.49866014642657,-1.49783793492101,-1.49620969997124,
-1.48430465313199,-1.45785444564072,-1.38333629801203,-1.36645709435033,
-1.34347683540578,-1.34054864286672,-1.33904858522402,-1.33794153254176,
-1.33676559664923,-1.33518246050896,-1.33342205990064,-1.33045010742261,
-1.28128841473332,-1.20976804633029,-1.18020074706501,-1.17800887442522,
-1.17714867511123,-1.17652610644557,-1.17585766267407,-1.17494621394699,
-1.17285201891497,-1.13082007825071,-1.02988316365458,-1.02267070891844,
-1.01813299353101,-1.01649348720987,-1.01534933406244,-1.014202716672,-1.01273950696304,
-1.0098500321605,-1.00616495475597,-0.946074159473671,-0.860317693906782,
-0.855845311144342,-0.854567174623528,-0.853820254104679,-0.853228834796903,
-0.85242983429433,-0.850912863838098,-0.841955917945522,-0.822874644488806,
-0.777053495135603,-0.702006106977066,-0.695914900793396,-0.693856525683937,
-0.692696400998567,-0.691538152374137,-0.690101798401045,-0.687340255289911,
-0.683854370429263,-0.676244259994933,-0.654390455663302,-0.61481570883021,
-0.537397001801655,-0.533130306169542,-0.531875107490516,-0.53120733567724,
-0.530558479526669,-0.529760259996369,-0.528247077842323,-0.519374398651029,
-0.500418614801332,-0.475702843733456,-0.468574661030553,-0.462436211239311,
-0.408134104551966,-0.401992201293512,-0.394546586384605,-0.375124342614916,
-0.372024920205923,-0.370512250711903,-0.369330102597084,-0.368228095799293,
-0.366327224538797,-0.360835064555212,-0.352636062866895,-0.3284755498035,
-0.307074065932593,-0.22567827891349,-0.225069469539524,-0.22427579642959,
-0.211441321875502,-0.209803396543811,-0.208966564655551,-0.208349988887942,
-0.207676794989064,-0.206739388591995,-0.204496551838612,-0.165878030590847,
-0.0945384025142255,-0.0877800856059834,-0.0532014966570062,-0.0495858368248017,
-0.0481357412690161,-0.0469313773131904,-0.045825218747467,-0.0446218283110119,
-0.0429926733844762,-0.0403368641217892,-0.000956521092448796),
 .UNSPECIFIED.);
#882=B_SPLINE_CURVE_WITH_KNOTS('',3,(#67951,#67952,#67953,#67954,#67955,
#67956,#67957,#67958,#67959,#67960,#67961,#67962,#67963,#67964,#67965,#67966,
#67967,#67968,#67969,#67970,#67971,#67972,#67973,#67974,#67975,#67976,#67977,
#67978,#67979,#67980,#67981,#67982,#67983,#67984,#67985,#67986,#67987,#67988,
#67989,#67990,#67991,#67992,#67993,#67994,#67995,#67996,#67997,#67998,#67999,
#68000,#68001,#68002,#68003,#68004,#68005,#68006,#68007,#68008,#68009,#68010,
#68011,#68012,#68013,#68014,#68015,#68016,#68017,#68018,#68019,#68020,#68021,
#68022,#68023,#68024,#68025,#68026,#68027,#68028,#68029,#68030,#68031,#68032,
#68033,#68034,#68035,#68036,#68037,#68038,#68039,#68040,#68041,#68042,#68043,
#68044,#68045,#68046,#68047,#68048,#68049,#68050,#68051,#68052,#68053,#68054,
#68055,#68056,#68057,#68058,#68059,#68060,#68061,#68062,#68063,#68064,#68065,
#68066,#68067,#68068,#68069,#68070,#68071,#68072,#68073,#68074,#68075,#68076,
#68077,#68078,#68079,#68080,#68081,#68082,#68083,#68084,#68085,#68086,#68087,
#68088,#68089,#68090,#68091,#68092,#68093,#68094,#68095,#68096,#68097,#68098,
#68099,#68100,#68101,#68102,#68103,#68104,#68105,#68106,#68107,#68108,#68109,
#68110,#68111,#68112,#68113,#68114,#68115,#68116,#68117,#68118,#68119,#68120,
#68121,#68122,#68123,#68124,#68125,#68126,#68127,#68128,#68129,#68130,#68131,
#68132,#68133,#68134,#68135,#68136,#68137,#68138,#68139,#68140,#68141,#68142,
#68143,#68144,#68145,#68146,#68147,#68148,#68149,#68150,#68151,#68152,#68153,
#68154,#68155,#68156,#68157,#68158,#68159,#68160,#68161,#68162,#68163,#68164,
#68165,#68166,#68167,#68168,#68169,#68170,#68171,#68172,#68173,#68174,#68175,
#68176,#68177,#68178,#68179,#68180,#68181,#68182,#68183,#68184,#68185,#68186,
#68187,#68188,#68189,#68190,#68191,#68192,#68193,#68194,#68195,#68196,#68197,
#68198,#68199,#68200,#68201,#68202,#68203,#68204,#68205,#68206,#68207,#68208,
#68209,#68210,#68211,#68212,#68213,#68214,#68215,#68216,#68217,#68218,#68219,
#68220,#68221,#68222,#68223,#68224,#68225,#68226,#68227,#68228,#68229,#68230,
#68231,#68232,#68233,#68234,#68235,#68236,#68237,#68238,#68239,#68240,#68241,
#68242,#68243,#68244,#68245,#68246,#68247,#68248,#68249,#68250,#68251,#68252,
#68253,#68254,#68255,#68256,#68257,#68258,#68259,#68260,#68261,#68262,#68263,
#68264,#68265,#68266,#68267,#68268,#68269,#68270,#68271,#68272,#68273,#68274,
#68275,#68276,#68277,#68278,#68279,#68280,#68281,#68282,#68283,#68284,#68285,
#68286,#68287,#68288,#68289,#68290,#68291,#68292,#68293,#68294,#68295,#68296,
#68297,#68298,#68299,#68300,#68301,#68302,#68303,#68304,#68305,#68306,#68307,
#68308,#68309,#68310,#68311,#68312,#68313,#68314,#68315,#68316,#68317,#68318,
#68319,#68320,#68321,#68322,#68323,#68324,#68325,#68326,#68327,#68328,#68329,
#68330,#68331,#68332,#68333,#68334,#68335,#68336,#68337,#68338,#68339,#68340,
#68341,#68342,#68343,#68344,#68345,#68346,#68347,#68348,#68349,#68350,#68351,
#68352,#68353,#68354,#68355,#68356,#68357,#68358,#68359,#68360,#68361,#68362,
#68363,#68364,#68365,#68366,#68367,#68368,#68369,#68370,#68371,#68372,#68373,
#68374,#68375,#68376,#68377,#68378,#68379,#68380,#68381,#68382,#68383,#68384,
#68385,#68386,#68387,#68388,#68389,#68390,#68391,#68392,#68393,#68394,#68395,
#68396,#68397,#68398,#68399,#68400,#68401,#68402,#68403,#68404,#68405,#68406,
#68407,#68408,#68409,#68410,#68411,#68412,#68413,#68414,#68415,#68416,#68417,
#68418,#68419,#68420,#68421,#68422,#68423,#68424,#68425,#68426,#68427,#68428,
#68429,#68430,#68431,#68432,#68433,#68434,#68435,#68436,#68437,#68438,#68439,
#68440,#68441,#68442,#68443,#68444,#68445,#68446,#68447,#68448,#68449,#68450,
#68451,#68452,#68453,#68454,#68455,#68456,#68457,#68458,#68459,#68460,#68461,
#68462,#68463,#68464,#68465,#68466,#68467,#68468,#68469,#68470,#68471,#68472,
#68473,#68474,#68475,#68476,#68477,#68478,#68479,#68480,#68481,#68482,#68483,
#68484,#68485,#68486,#68487,#68488,#68489,#68490,#68491,#68492,#68493,#68494,
#68495,#68496,#68497,#68498,#68499,#68500,#68501,#68502),.UNSPECIFIED.,
 .F.,.F.,(4,2,2,2,2,2,2,2,2,2,2,2,2,2,2,2,2,2,2,2,2,2,2,2,2,2,2,2,2,2,2,
2,2,2,2,2,2,2,2,2,2,2,2,2,2,2,2,2,2,2,2,2,2,2,2,2,2,2,2,2,2,2,2,2,2,2,2,
2,2,2,2,2,2,2,2,2,2,2,2,2,2,2,2,2,2,2,2,2,2,2,2,2,2,2,2,2,2,2,2,2,2,2,2,
2,2,2,2,2,2,2,2,2,2,2,2,2,2,2,2,2,2,2,2,2,2,2,2,2,2,2,2,2,2,2,2,2,2,2,2,
2,2,2,2,2,2,2,2,2,2,2,2,2,2,2,2,2,2,2,2,2,2,2,2,2,2,2,2,2,2,2,2,2,2,2,2,
2,2,2,2,2,2,2,2,2,2,2,2,2,2,2,2,2,2,2,2,2,2,2,2,2,2,2,2,2,2,2,2,2,2,2,2,
2,2,2,2,2,2,2,2,2,2,2,2,2,2,2,2,2,2,2,2,2,2,2,2,2,2,2,2,2,2,2,2,2,2,2,2,
2,2,2,2,2,2,2,2,2,2,2,2,2,2,2,2,2,2,2,2,2,2,2,2,2,2,2,2,4),(-4.06011575675384,
-3.98757700257165,-3.95179295117725,-3.94861885117166,-3.94633076893291,
-3.94538589119552,-3.94471144585061,-3.94409668820049,-3.94326654170211,
-3.94165409237231,-3.9294847635718,-3.92815873945996,-3.8371688991084,-3.81600790057753,
-3.78989226159108,-3.78616584462785,-3.78488556839697,-3.78378401734363,
-3.78260194174737,-3.78108739400615,-3.77797717769672,-3.75830867887014,
-3.75126249675961,-3.74522684226998,-3.70026359103249,-3.66294429751494,
-3.62904013491075,-3.62436444415706,-3.62312358873041,-3.62238511183924,
-3.62172669405768,-3.62088267751096,-3.61914600486653,-3.60817875336548,
-3.534204661898,-3.50011203236926,-3.48153218048321,-3.4711617681877,-3.46456192409247,
-3.46254687397687,-3.46126826934228,-3.46008609530097,-3.45857051990397,
-3.45545500749174,-3.43567052689144,-3.43017071591548,-3.34240908177447,
-3.30658352529893,-3.30176815741044,-3.30051450987388,-3.29977312798081,
-3.29911517319415,-3.29827583921713,-3.29656287114189,-3.28608566833394,
-3.19298388606223,-3.14905271954859,-3.14434807955539,-3.1408234020704,
-3.13923539261104,-3.1380590030997,-3.13695285958045,-3.13545582989029,
-3.13178905497669,-3.09138338920161,-3.01262550483756,-2.98329290309546,
-2.97898508725235,-2.97777949802357,-2.97704888398538,-2.97638866411616,
-2.97554444467752,-2.97376066980215,-2.96175290085045,-2.92069757376718,
-2.85571352021303,-2.82475412584975,-2.82092423448123,-2.81881722971635,
-2.81705683755318,-2.81581670580873,-2.81462140651379,-2.81304480258912,
-2.8095217278567,-2.77841076753186,-2.69335461663846,-2.65802227558515,
-2.65578290342084,-2.6548462207046,-2.65417328206735,-2.65355674813457,
-2.65271969856161,-2.65108053710975,-2.63820379829682,-2.63744615582557,
-2.63450514595683,-2.55770344715032,-2.5157261156125,-2.49790757702579,
-2.49511594211743,-2.49366637466137,-2.4926030644969,-2.4914575737486,-2.4898132755788,
-2.48524404129061,-2.41046298206508,-2.3626967212315,-2.33756644554804,
-2.33363522436984,-2.33246880727037,-2.3317469284101,-2.33108414115988,
-2.33022243572056,-2.32841458727274,-2.31526623985899,-2.31224590514854,
-2.30847676164208,-2.30643466094583,-2.30396204516384,-2.21246096227134,
-2.17965017689615,-2.17369100507901,-2.17172542755749,-2.17045712463039,
-2.16926292244687,-2.16769273560219,-2.16503660768012,-2.14849761943066,
-2.0531487337881,-2.0304385676575,-2.02855419268785,-2.02554854596311,-2.02457276282454,
-2.01197596165693,-2.01034713486672,-2.00951272663943,-2.0088968507714,
-2.00822329522742,-2.00728340251416,-2.0050252360139,-2.00190359451685,
-1.96725877699995,-1.91300194891421,-1.85430688137431,-1.85041792491926,
-1.84888245597491,-1.84776627522264,-1.84657207737013,-1.84497502417979,
-1.84143544803906,-1.83674695449518,-1.79307319778345,-1.70001592127376,
-1.68914489406369,-1.6874120736328,-1.68656864404352,-1.68591009071925,
-1.68517082599969,-1.68392719157903,-1.67922448193481,-1.6449754465871,
-1.53591198361227,-1.52857662093458,-1.52636040423623,-1.52503611631389,
-1.52397534737126,-1.52254879379158,-1.51986618239382,-1.50457141420902,
-1.47584647183738,-1.38520397836188,-1.38252745292843,-1.38071950166956,
-1.37985698306795,-1.37858484437319,-1.36634664710396,-1.36473132157762,
-1.3639003473568,-1.3632852967005,-1.36261086306937,-1.36166659250757,-1.35943583542082,
-1.35633503006023,-1.32212998844326,-1.24415999997894,-1.2275810356317,
-1.2074179944024,-1.2042845458431,-1.20276515978735,-1.20158223274631,-1.20027884091198,
-1.19819876358201,-1.19124424286824,-1.14876100407268,-1.07984632646153,
-1.06680786533071,-1.04415446176051,-1.042087245498,-1.04124852029701,-1.04063150433497,
-1.0399588148753,-1.03902383731458,-1.03686232211116,-1.03387335306232,
-1.00191178713765,-0.940581954475832,-0.885973531995667,-0.882112962732701,
-0.880582232716324,-0.879467220111196,-0.878272127677422,-0.876670165898123,
-0.873197286235571,-0.849273271456177,-0.83064978468061,-0.772638226546301,
-0.761543247602596,-0.731816544990858,-0.720968354552017,-0.71923673911755,
-0.718393585078587,-0.71773510295712,-0.716995764373869,-0.716227361141434,
-0.713582327241202,-0.709737068389898,-0.698893396978624,-0.682418563074156,
-0.631929507295326,-0.591124604455596,-0.562677562324951,-0.559232353497958,
-0.557669862960634,-0.556476738326142,-0.555204966663074,-0.553224555489426,
-0.54727617640514,-0.513769534126682,-0.461111344103762,-0.400772719599086,
-0.397349708037988,-0.396199057993426,-0.395552345444014,-0.394959969307072,
-0.394152139281111,-0.393287639585438,-0.389404893637406,-0.383104203831881,
-0.380657451845361,-0.34823028593471,-0.317500596304946,-0.272270897944792,
-0.266112004474246,-0.259428211114443,-0.239576022223285,-0.236456531740176,
-0.234939822637774,-0.233757127401935,-0.232452109154229,-0.231108815591459,
-0.229133120753417,-0.212888424794893,-0.172097567544964,-0.157913890404894,
-0.143347691792025,-0.0865974685278843,-0.0757781157366671,-0.0740478200476607,
-0.0732048887942819,-0.0725463861762182,-0.0718068166944389,-0.0710381076872037,
-0.069887180503094,-0.0678043440310872,-0.0631073317543311,-0.000957274032640893),
 .UNSPECIFIED.);
#883=B_SPLINE_CURVE_WITH_KNOTS('',3,(#68504,#68505,#68506,#68507,#68508,
#68509,#68510,#68511,#68512,#68513,#68514,#68515,#68516,#68517,#68518,#68519,
#68520,#68521,#68522,#68523,#68524,#68525,#68526,#68527,#68528,#68529,#68530,
#68531,#68532,#68533,#68534,#68535,#68536,#68537,#68538,#68539,#68540,#68541,
#68542,#68543,#68544,#68545,#68546,#68547,#68548,#68549,#68550,#68551,#68552,
#68553,#68554,#68555,#68556,#68557,#68558,#68559,#68560,#68561,#68562,#68563,
#68564,#68565,#68566,#68567,#68568,#68569,#68570,#68571,#68572,#68573,#68574,
#68575,#68576,#68577,#68578,#68579,#68580,#68581,#68582,#68583,#68584,#68585,
#68586,#68587,#68588,#68589,#68590,#68591,#68592,#68593,#68594,#68595,#68596,
#68597,#68598,#68599,#68600,#68601,#68602,#68603,#68604,#68605,#68606,#68607,
#68608,#68609,#68610,#68611,#68612,#68613,#68614,#68615,#68616,#68617,#68618,
#68619,#68620,#68621,#68622,#68623,#68624,#68625,#68626,#68627,#68628,#68629,
#68630,#68631,#68632,#68633,#68634,#68635,#68636,#68637,#68638,#68639,#68640,
#68641,#68642,#68643,#68644,#68645,#68646,#68647,#68648,#68649,#68650,#68651,
#68652,#68653,#68654,#68655,#68656,#68657,#68658,#68659,#68660,#68661,#68662,
#68663,#68664,#68665,#68666,#68667,#68668,#68669,#68670,#68671,#68672,#68673,
#68674,#68675,#68676,#68677,#68678,#68679,#68680,#68681,#68682,#68683,#68684,
#68685,#68686,#68687,#68688,#68689,#68690,#68691,#68692,#68693,#68694,#68695,
#68696,#68697,#68698,#68699,#68700,#68701,#68702,#68703,#68704,#68705,#68706,
#68707,#68708,#68709,#68710,#68711,#68712,#68713,#68714,#68715,#68716,#68717,
#68718,#68719,#68720,#68721,#68722,#68723,#68724,#68725,#68726,#68727,#68728,
#68729,#68730,#68731,#68732,#68733,#68734,#68735,#68736,#68737,#68738,#68739,
#68740,#68741,#68742,#68743,#68744,#68745,#68746,#68747,#68748,#68749,#68750,
#68751,#68752,#68753,#68754,#68755,#68756,#68757,#68758,#68759,#68760,#68761,
#68762,#68763,#68764,#68765,#68766,#68767,#68768,#68769,#68770,#68771,#68772,
#68773,#68774,#68775,#68776,#68777,#68778,#68779,#68780,#68781,#68782,#68783,
#68784,#68785,#68786,#68787,#68788,#68789,#68790,#68791,#68792,#68793,#68794,
#68795,#68796,#68797,#68798,#68799,#68800,#68801,#68802,#68803,#68804,#68805,
#68806,#68807,#68808,#68809,#68810,#68811,#68812,#68813,#68814,#68815,#68816,
#68817,#68818,#68819,#68820,#68821,#68822,#68823,#68824,#68825,#68826,#68827,
#68828,#68829,#68830,#68831,#68832,#68833,#68834,#68835,#68836,#68837,#68838,
#68839,#68840,#68841,#68842,#68843,#68844,#68845,#68846,#68847,#68848,#68849,
#68850,#68851,#68852,#68853,#68854,#68855,#68856,#68857,#68858,#68859,#68860,
#68861,#68862,#68863,#68864,#68865,#68866,#68867,#68868,#68869,#68870,#68871,
#68872,#68873,#68874,#68875,#68876,#68877,#68878,#68879,#68880,#68881,#68882,
#68883,#68884,#68885,#68886,#68887,#68888,#68889,#68890,#68891,#68892,#68893,
#68894,#68895,#68896,#68897,#68898,#68899,#68900,#68901,#68902,#68903,#68904,
#68905,#68906,#68907,#68908,#68909,#68910,#68911,#68912,#68913,#68914,#68915,
#68916,#68917,#68918,#68919,#68920,#68921,#68922,#68923,#68924,#68925,#68926,
#68927,#68928,#68929,#68930,#68931,#68932,#68933,#68934,#68935,#68936,#68937,
#68938,#68939,#68940,#68941,#68942,#68943,#68944,#68945,#68946,#68947,#68948,
#68949,#68950,#68951,#68952,#68953,#68954,#68955,#68956,#68957,#68958,#68959,
#68960,#68961,#68962,#68963,#68964,#68965,#68966,#68967,#68968,#68969,#68970,
#68971,#68972,#68973,#68974,#68975,#68976,#68977,#68978,#68979,#68980,#68981,
#68982,#68983,#68984,#68985,#68986,#68987,#68988,#68989,#68990,#68991,#68992,
#68993,#68994,#68995,#68996,#68997,#68998,#68999,#69000,#69001,#69002,#69003,
#69004,#69005,#69006,#69007,#69008,#69009,#69010,#69011,#69012,#69013,#69014,
#69015,#69016,#69017,#69018,#69019,#69020,#69021,#69022,#69023,#69024,#69025,
#69026,#69027,#69028,#69029,#69030,#69031,#69032,#69033,#69034,#69035,#69036,
#69037,#69038,#69039),.UNSPECIFIED.,.F.,.F.,(4,2,2,2,2,2,2,2,2,2,2,2,2,
2,2,2,2,2,2,2,2,2,2,2,2,2,2,2,2,2,2,2,2,2,2,2,2,2,2,2,2,2,2,2,2,2,2,2,2,
2,2,2,2,2,2,2,2,2,2,2,2,2,2,2,2,2,2,2,2,2,2,2,2,2,2,2,2,2,2,2,2,2,2,2,2,
2,2,2,2,2,2,2,2,2,2,2,2,2,2,2,2,2,2,2,2,2,2,2,2,2,2,2,2,2,2,2,2,2,2,2,2,
2,2,2,2,2,2,2,2,2,2,2,2,2,2,2,2,2,2,2,2,2,2,2,2,2,2,2,2,2,2,2,2,2,2,2,2,
2,2,2,2,2,2,2,2,2,2,2,2,2,2,2,2,2,2,2,2,2,2,2,2,2,2,2,2,2,2,2,2,2,2,2,2,
2,2,2,2,2,2,2,2,2,2,2,2,2,2,2,2,2,2,2,2,2,2,2,2,2,2,2,2,2,2,2,2,2,2,2,2,
2,2,2,2,2,2,2,2,2,2,2,2,2,2,2,2,2,2,2,2,2,2,2,2,2,2,2,2,2,2,2,2,2,2,2,2,
2,2,4),(-4.06100195960022,-3.97862899521379,-3.975726211888,-3.97399450084426,
-3.97241069470506,-3.97121883560045,-3.97009931297994,-3.9682455270532,
-3.96351385378274,-3.88450523397763,-3.87102826455039,-3.85862758370722,
-3.82721889707641,-3.81688445820489,-3.81230049299831,-3.81139301648855,
-3.81072297947515,-3.81004928207542,-3.80943384896562,-3.80860085773195,
-3.80697720747016,-3.79452034828951,-3.79343651670533,-3.79265394528713,
-3.74355949624964,-3.70412651921958,-3.67004977845332,-3.65934447765577,
-3.65258031504339,-3.65104663765605,-3.64960591595634,-3.64854374960308,
-3.64739432248811,-3.64573552695692,-3.64106900295924,-3.56702032070852,
-3.52008512077055,-3.49199828347988,-3.48931196432979,-3.48853761920477,
-3.487794153824,-3.48713659060821,-3.48630073692835,-3.48460498843525,-3.47447073051979,
-3.4298234015499,-3.37824996769656,-3.35670039542035,-3.33234988232163,
-3.32893566749388,-3.32734043032294,-3.326146651058,-3.32503017944141,-3.3234932403519,
-3.31959492563555,-3.2589082594984,-3.20794941930971,-3.17902172502668,
-3.17159441385538,-3.16723800355652,-3.16600309071061,-3.16526025329817,
-3.16460256402472,-3.16376564346453,-3.16206465917049,-3.15182327288676,
-3.121932906067,-3.06177317081537,-3.01497428168572,-3.00760173456035,-3.00545688269464,
-3.00414864410296,-3.0029671135387,-3.00145754966638,-2.99837260032162,
-2.97924519558001,-2.97611557523412,-2.96755722429297,-2.95015561030973,
-2.88087076760129,-2.84914898335842,-2.84617294660422,-2.84401224332467,
-2.84309270843413,-2.8424194752211,-2.84180336428273,-2.84096788074587,
-2.83933472216725,-2.82662224290997,-2.82574073141467,-2.82536810031513,
-2.81781353991909,-2.73947889040378,-2.69240103249051,-2.68499915694957,
-2.68285341278672,-2.68154498750054,-2.68036352084798,-2.67885435969665,
-2.6757713553391,-2.65668405106025,-2.64867288027682,-2.55788468760732,
-2.52362255340759,-2.52135176543623,-2.52040975057213,-2.51973580573709,
-2.51912039121322,-2.51828777363767,-2.51666587637117,-2.50426233389479,
-2.41723490725594,-2.3697152588366,-2.36224731954546,-2.36011016997924,
-2.35880362887595,-2.35762167338357,-2.35610885494249,-2.35300773732636,
-2.33353905516213,-2.32815347891129,-2.30937354338989,-2.27545181797462,
-2.22803466344111,-2.20888777219725,-2.19986547228952,-2.1983457270625,
-2.19754621477197,-2.19695482889031,-2.19620849758587,-2.1949326737715,
-2.19048023761434,-2.10172838425506,-2.04775783822248,-2.03973639725366,
-2.03754434992121,-2.03622559749815,-2.03504624151239,-2.0335553224936,
-2.03121765742446,-2.01759028407343,-1.99057914725422,-1.88690433179769,
-1.87730510045499,-1.87565793686551,-1.87482055450431,-1.87416272281584,
-1.8734199605097,-1.87216044280701,-1.86728058781452,-1.84407759867751,
-1.79801636916948,-1.75408599160187,-1.71937799571806,-1.715806871268,-1.71433995229095,
-1.71324112016464,-1.7120336612542,-1.71036136535635,-1.7063998721415,-1.65612314841707,
-1.56594781731917,-1.55474359554411,-1.55299533303979,-1.55214881284511,
-1.55148988008721,-1.55075235259725,-1.54951657773581,-1.54489908216215,
-1.51177779063074,-1.42589358949798,-1.39636497592263,-1.39323445933923,
-1.39168294766779,-1.390562456198,-1.38937048781632,-1.38778810902263,-1.38432807756073,
-1.36673379967075,-1.35061402519731,-1.30531227803955,-1.24422311397194,
-1.23210107052551,-1.23031204068527,-1.22946666986523,-1.22880614675318,
-1.22807583025985,-1.22689626393047,-1.22284184182671,-1.19617980012805,
-1.1284526045915,-1.07437601000282,-1.07052003403702,-1.0689900616717,-1.06787522581011,
-1.0666799690242,-1.0650771733889,-1.06150707000265,-1.05676838840711,-1.01229101143329,
-0.943429311678271,-0.93141617378817,-0.929278532842363,-0.924753906773191,
-0.909602926568883,-0.90769735812237,-0.906829883771583,-0.906166099287072,
-0.905446675041333,-0.904314803233453,-0.900679453593819,-0.894897069443431,
-0.876176506298365,-0.821707988418639,-0.75238293335182,-0.748045292673333,
-0.746436558509093,-0.745300694707331,-0.744234222110286,-0.742761489522267,
-0.739859193975525,-0.719320944712954,-0.689516220297427,-0.633298405655588,
-0.588200843627052,-0.585456242761711,-0.584510892211894,-0.583865010115297,
-0.583272445978597,-0.582641719848806,-0.581347539870029,-0.576073715852917,
-0.566593280987147,-0.541810763526414,-0.508511272998862,-0.430038070900999,
-0.425472286470002,-0.423828339898572,-0.422682822785653,-0.421619276202319,
-0.420169061877189,-0.417375078376827,-0.399832948230513,-0.359096910092,
-0.318631021463136,-0.274005810371374,-0.263971419869908,-0.262301571293539,
-0.261459305973149,-0.260800916626039,-0.260061038955666,-0.259291871724942,
-0.258139799704044,-0.246234842469268,-0.218053254730235,-0.196473021979129,
-0.127113466610081,-0.125487720877041,-0.120143229730793,-0.104830416061291,
-0.102238367774451,-0.100686838965146,-0.0994955297405637,-0.0982192981729564,
-0.096218672422179,-0.0939009296580686,-0.0844466177707292,-0.00095780636328563),
 .UNSPECIFIED.);
#884=B_SPLINE_CURVE_WITH_KNOTS('',3,(#69041,#69042,#69043,#69044,#69045,
#69046,#69047,#69048,#69049,#69050,#69051,#69052,#69053,#69054,#69055,#69056,
#69057,#69058,#69059,#69060,#69061,#69062,#69063,#69064,#69065,#69066,#69067,
#69068,#69069,#69070,#69071,#69072,#69073,#69074,#69075,#69076,#69077,#69078,
#69079,#69080,#69081,#69082,#69083,#69084,#69085,#69086,#69087,#69088,#69089,
#69090,#69091,#69092,#69093,#69094,#69095,#69096,#69097,#69098,#69099,#69100,
#69101,#69102,#69103,#69104,#69105,#69106,#69107,#69108,#69109,#69110,#69111,
#69112,#69113,#69114,#69115,#69116,#69117,#69118,#69119,#69120,#69121,#69122,
#69123,#69124,#69125,#69126,#69127,#69128,#69129,#69130,#69131,#69132,#69133,
#69134,#69135,#69136,#69137,#69138,#69139,#69140,#69141,#69142,#69143,#69144,
#69145,#69146,#69147,#69148,#69149,#69150,#69151,#69152,#69153,#69154,#69155,
#69156,#69157,#69158,#69159,#69160,#69161,#69162,#69163,#69164,#69165,#69166,
#69167,#69168,#69169,#69170,#69171,#69172,#69173,#69174,#69175,#69176,#69177,
#69178,#69179,#69180,#69181,#69182,#69183,#69184,#69185,#69186,#69187,#69188,
#69189,#69190,#69191,#69192,#69193,#69194,#69195,#69196,#69197,#69198,#69199,
#69200,#69201,#69202,#69203,#69204,#69205,#69206,#69207,#69208,#69209,#69210,
#69211,#69212,#69213,#69214,#69215,#69216,#69217,#69218,#69219,#69220,#69221,
#69222,#69223,#69224,#69225,#69226,#69227,#69228,#69229,#69230,#69231,#69232,
#69233,#69234,#69235,#69236,#69237,#69238,#69239,#69240,#69241,#69242,#69243,
#69244,#69245,#69246,#69247,#69248,#69249,#69250,#69251,#69252,#69253,#69254,
#69255,#69256,#69257,#69258,#69259,#69260,#69261,#69262,#69263,#69264,#69265,
#69266,#69267,#69268,#69269,#69270,#69271,#69272,#69273,#69274,#69275,#69276,
#69277,#69278,#69279,#69280,#69281,#69282,#69283,#69284,#69285,#69286,#69287,
#69288,#69289,#69290,#69291,#69292,#69293,#69294,#69295,#69296,#69297,#69298,
#69299,#69300,#69301,#69302,#69303,#69304,#69305,#69306,#69307,#69308,#69309,
#69310,#69311,#69312,#69313,#69314,#69315,#69316,#69317,#69318,#69319,#69320,
#69321,#69322,#69323,#69324,#69325,#69326,#69327,#69328,#69329,#69330,#69331,
#69332,#69333,#69334,#69335,#69336,#69337,#69338,#69339,#69340,#69341,#69342,
#69343,#69344,#69345,#69346,#69347,#69348,#69349,#69350,#69351,#69352,#69353,
#69354,#69355,#69356,#69357,#69358,#69359,#69360,#69361,#69362,#69363,#69364,
#69365,#69366,#69367,#69368,#69369,#69370,#69371,#69372,#69373,#69374,#69375,
#69376,#69377,#69378,#69379,#69380,#69381,#69382,#69383,#69384,#69385,#69386,
#69387,#69388,#69389,#69390,#69391,#69392,#69393,#69394,#69395,#69396,#69397,
#69398,#69399,#69400,#69401,#69402,#69403,#69404,#69405,#69406,#69407,#69408,
#69409,#69410,#69411,#69412,#69413,#69414,#69415,#69416,#69417,#69418,#69419,
#69420,#69421,#69422,#69423,#69424,#69425,#69426,#69427,#69428,#69429,#69430,
#69431,#69432,#69433,#69434,#69435,#69436,#69437,#69438,#69439,#69440,#69441,
#69442,#69443,#69444,#69445,#69446,#69447,#69448,#69449,#69450,#69451,#69452,
#69453,#69454,#69455,#69456,#69457,#69458,#69459,#69460,#69461,#69462,#69463,
#69464,#69465,#69466,#69467,#69468,#69469,#69470,#69471,#69472,#69473,#69474,
#69475,#69476,#69477,#69478,#69479,#69480,#69481,#69482,#69483,#69484,#69485,
#69486,#69487,#69488,#69489,#69490,#69491,#69492,#69493,#69494,#69495,#69496,
#69497,#69498,#69499,#69500,#69501,#69502,#69503,#69504,#69505,#69506,#69507,
#69508,#69509,#69510,#69511,#69512,#69513,#69514,#69515,#69516,#69517,#69518,
#69519,#69520,#69521,#69522,#69523,#69524,#69525,#69526,#69527,#69528,#69529,
#69530,#69531,#69532,#69533,#69534,#69535,#69536,#69537,#69538,#69539,#69540,
#69541,#69542,#69543,#69544,#69545,#69546,#69547,#69548,#69549,#69550,#69551,
#69552,#69553,#69554,#69555,#69556,#69557,#69558,#69559,#69560,#69561,#69562,
#69563,#69564,#69565,#69566),.UNSPECIFIED.,.F.,.F.,(4,2,2,2,2,2,2,2,2,2,
2,2,2,2,2,2,2,2,2,2,2,2,2,2,2,2,2,2,2,2,2,2,2,2,2,2,2,2,2,2,2,2,2,2,2,2,
2,2,2,2,2,2,2,2,2,2,2,2,2,2,2,2,2,2,2,2,2,2,2,2,2,2,2,2,2,2,2,2,2,2,2,2,
2,2,2,2,2,2,2,2,2,2,2,2,2,2,2,2,2,2,2,2,2,2,2,2,2,2,2,2,2,2,2,2,2,2,2,2,
2,2,2,2,2,2,2,2,2,2,2,2,2,2,2,2,2,2,2,2,2,2,2,2,2,2,2,2,2,2,2,2,2,2,2,2,
2,2,2,2,2,2,2,2,2,2,2,2,2,2,2,2,2,2,2,2,2,2,2,2,2,2,2,2,2,2,2,2,2,2,2,2,
2,2,2,2,2,2,2,2,2,2,2,2,2,2,2,2,2,2,2,2,2,2,2,2,2,2,2,2,2,2,2,2,2,2,2,2,
2,2,2,2,2,2,2,2,2,2,2,2,2,2,2,2,2,2,2,2,2,2,2,2,2,2,2,2,2,2,2,2,2,2,2,2,
4),(-4.05837967880851,-4.00114997962759,-3.99885786767353,-3.99762552912259,
-3.9968230236056,-3.99618974499812,-3.99559634508342,-3.99495669272019,
-3.99383912483112,-3.99064763807603,-3.93486593044823,-3.92562478079503,
-3.9177941050812,-3.90206842493183,-3.85787989888074,-3.83986311131241,
-3.83693028810942,-3.8354521413208,-3.83438575770854,-3.83325372643113,
-3.83133322295104,-3.82617954040288,-3.74423570466487,-3.72164401947659,
-3.69693646754935,-3.68295670012722,-3.67833511550716,-3.67527997458224,
-3.67447698972937,-3.67384354395003,-3.67325004887753,-3.67261057582201,
-3.67149401834921,-3.66831022658899,-3.61575703947775,-3.55873903585013,
-3.52326972702981,-3.51606349064379,-3.51393903226155,-3.51263593240743,
-3.51145425774148,-3.50993785711651,-3.50681545538903,-3.48685168599715,
-3.48128191897757,-3.47363585076932,-3.42895771502899,-3.37983569981381,
-3.36480205136965,-3.35757572516932,-3.35326806809867,-3.35206477311877,
-3.35132947919183,-3.35067091860498,-3.34982267463912,-3.34806308764843,
-3.33658332861734,-3.31098042527118,-3.26459306558094,-3.19598542264968,
-3.192557372488,-3.19096473634342,-3.18977203488181,-3.18865594071235,-3.18711853085315,
-3.18321379086585,-3.11886334614989,-3.05648873116259,-3.03436856739687,
-3.03074516316081,-3.02961509163815,-3.02889651243075,-3.0282332986454,
-3.02736628258029,-3.02546056866849,-3.01025878225391,-3.00680051026876,
-3.00378788423812,-2.93647193934366,-2.8766535399211,-2.87105717568062,
-2.86907633029981,-2.86780523232915,-2.86661341576706,-2.86505361211981,
-2.86161829918681,-2.83341231061393,-2.815004636839,-2.73990169365395,-2.71257500815404,
-2.70845844726987,-2.70727562505949,-2.70654498179522,-2.70588530443346,
-2.70504253310068,-2.70326460044982,-2.69137289692048,-2.6877317867718,
-2.68737613379298,-2.68429807624357,-2.63314262600088,-2.58250911237497,
-2.55674143124803,-2.54906285762393,-2.54690523274297,-2.54559464938686,
-2.54441452442639,-2.54291159956409,-2.53995754234237,-2.5226575879747,
-2.5191350607216,-2.42067527257305,-2.38752228907476,-2.38538930504742,
-2.38447133717972,-2.38380207756533,-2.38318169309282,-2.38232886095255,
-2.38062677085322,-2.3658801709741,-2.35939375785636,-2.35734266875868,
-2.31700919515784,-2.28179809527985,-2.2513664799281,-2.2280157565012,-2.22504431493079,
-2.22355802214818,-2.22249021865752,-2.22136080331619,-2.21945477307557,
-2.21439592966997,-2.13352045214246,-2.12430573290513,-2.09851889040651,
-2.06510833763195,-2.06297302656451,-2.06205461606913,-2.0613852467922,
-2.06076491858795,-2.05991239625014,-2.0577635704893,-2.03080139871175,
-1.98370736019489,-1.90830253150715,-1.90348917916552,-1.90162239558283,
-1.90050062103354,-1.89931056244168,-1.89773626739029,-1.89431584255193,
-1.83425328504353,-1.74563975339823,-1.74116314654907,-1.73988490510131,
-1.7391381705834,-1.73854703916434,-1.73774860741926,-1.73623329897262,
-1.72730188506405,-1.70825709689502,-1.66120989655085,-1.58549595068009,
-1.58084248980402,-1.57918589124235,-1.5780372497445,-1.57697523735169,
-1.57553385715438,-1.57277965170257,-1.55586440902599,-1.51804879986678,
-1.4232609877706,-1.41859394327791,-1.41731037572708,-1.41655490287901,
-1.41589901077637,-1.41508118940544,-1.41347358625866,-1.40219037402685,
-1.37269913975616,-1.27694991347926,-1.26020459675332,-1.25727909565672,
-1.25578199647074,-1.25460216174129,-1.25331414678017,-1.25122068988163,
-1.2487318234765,-1.24391272763347,-1.19810329257103,-1.10022234669614,
-1.09580824655952,-1.09453670633292,-1.09379136187305,-1.09319988876281,
-1.09239914529803,-1.09087343062266,-1.08171516639059,-1.06263818577135,
-1.0151427816789,-0.939786839406562,-0.935373431755597,-0.933753071190259,
-0.9326142666752,-0.931455592388888,-0.930062482405305,-0.928486024192247,
-0.925955481012324,-0.921025987709515,-0.873367884512564,-0.777824541968153,
-0.77316343434182,-0.771880296305007,-0.771124815659568,-0.770468750426268,
-0.769650499400428,-0.76804137382139,-0.756721636735015,-0.727063697712971,
-0.685810661766175,-0.616606839776575,-0.612535849646385,-0.610970079098724,
-0.609845919125714,-0.608713315289243,-0.607207532235838,-0.604115197254895,
-0.600107654068119,-0.590923698141503,-0.562977806945251,-0.514144239050153,
-0.453867872614956,-0.450316554562721,-0.449149216138912,-0.448499203394114,
-0.447907599998148,-0.447106427231515,-0.445579068966624,-0.436387808020264,
-0.41738512345892,-0.371366899622648,-0.348027623676495,-0.30869990580444,
-0.292253558609206,-0.289601929278322,-0.288032938038533,-0.28683879994682,
-0.285738265939946,-0.283951240467609,-0.279262048675758,-0.27254205137593,
-0.254080987998467,-0.235082400694175,-0.131592404963221,-0.127688789537731,
-0.126476362980388,-0.125817145815021,-0.125161086886395,-0.124345229269591,
-0.122748329517448,-0.111794078331155,-0.0838223294241255,-0.000958211236916205),
 .UNSPECIFIED.);
#885=B_SPLINE_CURVE_WITH_KNOTS('',3,(#69568,#69569,#69570,#69571,#69572,
#69573,#69574,#69575,#69576,#69577,#69578,#69579,#69580,#69581,#69582,#69583,
#69584,#69585,#69586,#69587,#69588,#69589,#69590,#69591,#69592,#69593,#69594,
#69595,#69596,#69597,#69598,#69599,#69600,#69601,#69602,#69603,#69604,#69605,
#69606,#69607,#69608,#69609,#69610,#69611,#69612,#69613,#69614,#69615,#69616,
#69617,#69618,#69619,#69620,#69621,#69622,#69623,#69624,#69625,#69626,#69627,
#69628,#69629,#69630,#69631,#69632,#69633,#69634,#69635,#69636,#69637,#69638,
#69639,#69640,#69641,#69642,#69643,#69644,#69645,#69646,#69647,#69648,#69649,
#69650,#69651,#69652,#69653,#69654,#69655,#69656,#69657,#69658,#69659,#69660,
#69661,#69662,#69663,#69664,#69665,#69666,#69667,#69668,#69669,#69670,#69671,
#69672,#69673,#69674,#69675,#69676,#69677,#69678,#69679,#69680,#69681,#69682,
#69683,#69684,#69685,#69686,#69687,#69688,#69689,#69690,#69691,#69692,#69693,
#69694,#69695,#69696,#69697,#69698,#69699,#69700,#69701,#69702,#69703,#69704,
#69705,#69706,#69707,#69708,#69709,#69710,#69711,#69712,#69713,#69714,#69715,
#69716,#69717,#69718,#69719,#69720,#69721,#69722,#69723,#69724,#69725,#69726,
#69727,#69728,#69729,#69730,#69731,#69732,#69733,#69734,#69735,#69736,#69737,
#69738,#69739,#69740,#69741,#69742,#69743,#69744,#69745,#69746,#69747,#69748,
#69749,#69750,#69751,#69752,#69753,#69754,#69755,#69756,#69757,#69758,#69759,
#69760,#69761,#69762,#69763,#69764,#69765,#69766,#69767,#69768,#69769,#69770,
#69771,#69772,#69773,#69774,#69775,#69776,#69777,#69778,#69779,#69780,#69781,
#69782,#69783,#69784,#69785,#69786,#69787,#69788,#69789,#69790,#69791,#69792,
#69793,#69794,#69795,#69796,#69797,#69798,#69799,#69800,#69801,#69802,#69803,
#69804,#69805,#69806,#69807,#69808,#69809,#69810,#69811,#69812,#69813,#69814,
#69815,#69816,#69817,#69818,#69819,#69820,#69821,#69822,#69823,#69824,#69825,
#69826,#69827,#69828,#69829,#69830,#69831,#69832,#69833,#69834,#69835,#69836,
#69837,#69838,#69839,#69840,#69841,#69842,#69843,#69844,#69845,#69846,#69847,
#69848,#69849,#69850,#69851,#69852,#69853,#69854,#69855,#69856,#69857,#69858,
#69859,#69860,#69861,#69862,#69863,#69864,#69865,#69866,#69867,#69868,#69869,
#69870,#69871,#69872,#69873,#69874,#69875,#69876,#69877,#69878,#69879,#69880,
#69881,#69882,#69883,#69884,#69885,#69886,#69887,#69888,#69889,#69890,#69891,
#69892,#69893,#69894,#69895,#69896,#69897,#69898,#69899,#69900,#69901,#69902,
#69903,#69904,#69905,#69906,#69907,#69908,#69909,#69910,#69911,#69912,#69913,
#69914,#69915,#69916,#69917,#69918,#69919,#69920,#69921,#69922,#69923,#69924,
#69925,#69926,#69927,#69928,#69929,#69930,#69931,#69932,#69933,#69934,#69935,
#69936,#69937,#69938,#69939,#69940,#69941,#69942,#69943,#69944,#69945,#69946,
#69947,#69948,#69949,#69950,#69951,#69952,#69953,#69954,#69955,#69956,#69957,
#69958,#69959,#69960,#69961,#69962,#69963,#69964,#69965,#69966,#69967,#69968,
#69969,#69970,#69971,#69972,#69973,#69974,#69975,#69976,#69977,#69978,#69979,
#69980,#69981,#69982,#69983,#69984,#69985,#69986,#69987,#69988,#69989,#69990,
#69991,#69992,#69993,#69994,#69995,#69996,#69997,#69998,#69999,#70000,#70001,
#70002,#70003,#70004,#70005,#70006,#70007,#70008,#70009,#70010,#70011,#70012,
#70013,#70014,#70015,#70016,#70017,#70018,#70019,#70020,#70021,#70022,#70023,
#70024,#70025,#70026,#70027,#70028,#70029,#70030,#70031,#70032,#70033,#70034,
#70035,#70036,#70037,#70038,#70039,#70040,#70041,#70042,#70043,#70044,#70045,
#70046,#70047,#70048,#70049,#70050,#70051,#70052,#70053,#70054,#70055,#70056,
#70057,#70058,#70059,#70060,#70061,#70062,#70063,#70064,#70065,#70066,#70067,
#70068,#70069,#70070,#70071,#70072,#70073,#70074,#70075,#70076,#70077,#70078,
#70079,#70080,#70081,#70082,#70083,#70084,#70085,#70086,#70087,#70088,#70089,
#70090,#70091,#70092,#70093,#70094,#70095),.UNSPECIFIED.,.F.,.F.,(4,2,2,
2,2,2,2,2,2,2,2,2,2,2,2,2,2,2,2,2,2,2,2,2,2,2,2,2,2,2,2,2,2,2,2,2,2,2,2,
2,2,2,2,2,2,2,2,2,2,2,2,2,2,2,2,2,2,2,2,2,2,2,2,2,2,2,2,2,2,2,2,2,2,2,2,
2,2,2,2,2,2,2,2,2,2,2,2,2,2,2,2,2,2,2,2,2,2,2,2,2,2,2,2,2,2,2,2,2,2,2,2,
2,2,2,2,2,2,2,2,2,2,2,2,2,2,2,2,2,2,2,2,2,2,2,2,2,2,2,2,2,2,2,2,2,2,2,2,
2,2,2,2,2,2,2,2,2,2,2,2,2,2,2,2,2,2,2,2,2,2,2,2,2,2,2,2,2,2,2,2,2,2,2,2,
2,2,2,2,2,2,2,2,2,2,2,2,2,2,2,2,2,2,2,2,2,2,2,2,2,2,2,2,2,2,2,2,2,2,2,2,
2,2,2,2,2,2,2,2,2,2,2,2,2,2,2,2,2,2,2,2,2,2,2,2,2,2,2,2,2,2,2,2,2,2,2,2,
2,2,2,2,2,2,2,2,4),(-4.06120156146985,-4.03210757396722,-4.02898962223826,
-4.02716923153719,-4.02589021951178,-4.02478870107512,-4.02360620612062,
-4.02208890672558,-4.01896520012184,-3.9990073799305,-3.99251745116898,
-3.98587636646403,-3.90492614531435,-3.87687630781146,-3.86590705178375,
-3.86430996816114,-3.86349421197578,-3.86283833298179,-3.86217937966733,
-3.86096766763953,-3.85706816786919,-3.75355810273542,-3.72233241612452,
-3.71193739985365,-3.70754385493776,-3.70421038782226,-3.70265777093699,
-3.70153674915908,-3.70042994104384,-3.69893038731804,-3.69600367842245,
-3.67305405653463,-3.61133036129914,-3.60472086317543,-3.59707456127475,
-3.54399453666206,-3.54187001850888,-3.54095330337529,-3.54028404202883,
-3.5396629762727,-3.53880820490921,-3.53709916588012,-3.5221526334199,-3.52113650057503,
-3.52009181161374,-3.51874348920431,-3.5143740386739,-3.42162329407878,
-3.39650004326749,-3.38805641206967,-3.38429131185362,-3.3813495959608,
-3.37987624134638,-3.3787336160924,-3.37759496928168,-3.37564322543333,
-3.37029052139437,-3.36298556912049,-3.25915209091068,-3.2245225180134,
-3.21979274183245,-3.21854680863072,-3.21780713268899,-3.21714883445646,
-3.21630656947934,-3.21463635321678,-3.20459111334289,-3.15999698161363,
-3.069175260887,-3.0633442102124,-3.06048136102256,-3.05876615550513,-3.05721650914028,
-3.05604599358132,-3.05493075006046,-3.05339845558342,-3.04952742355869,
-2.9935117479299,-2.93679635755297,-2.90188242769568,-2.89713209289675,
-2.89588434381003,-2.89514429430316,-2.89448612186026,-2.89364463297165,
-2.89192081389984,-2.88122545896731,-2.78889099056695,-2.74088725901194,
-2.73793223075628,-2.73617892301259,-2.73460039378158,-2.73342538628342,
-2.73231727455111,-2.73081241588302,-2.72710067123767,-2.68416031586473,
-2.61382134399594,-2.58599886270908,-2.57508077374812,-2.57348567875365,
-2.57267041044276,-2.57201465909501,-2.57135560923095,-2.5701430982173,
-2.56623614249461,-2.46297033493821,-2.4171649235412,-2.41351736121602,
-2.41190085425706,-2.41070371274285,-2.40959307686894,-2.40807808403072,
-2.40430561535023,-2.35739818734881,-2.32243777142454,-2.29081059076187,
-2.26425096416842,-2.26182673534768,-2.2523498306447,-2.25081056107775,
-2.25000704140691,-2.24935208326961,-2.24868635861321,-2.2474403980938,
-2.24325120571912,-2.16489884879582,-2.0943380880748,-2.09088060328921,
-2.08929921653918,-2.08810792401065,-2.08698801442365,-2.08543722359272,
-2.082307886553,-2.05277444455319,-2.03089391965558,-1.93366913198929,-1.92920708808078,
-1.92793030522512,-1.92718381571344,-1.92659253274293,-1.92579345413335,
-1.9242754851656,-1.91528957935169,-1.89617921795791,-1.84891360244464,
-1.80729748762842,-1.77201419985588,-1.76874558330729,-1.767160082276,-1.76603075518482,
-1.76496240284194,-1.76347433697782,-1.76049566222153,-1.73690710647679,
-1.71703078689443,-1.66717080638795,-1.60974807636699,-1.60644110870235,
-1.60530711256131,-1.6046638834551,-1.60407093025589,-1.60325665295594,
-1.60166633036362,-1.59088223098859,-1.56366616301844,-1.48148523758425,
-1.47555659102584,-1.46794113588852,-1.44863083767028,-1.44553747319105,
-1.44402633731195,-1.4428447385262,-1.44153761296112,-1.43939728664751,
-1.43189635997558,-1.38400122075942,-1.28871555710387,-1.28406442637754,
-1.28278235878451,-1.28202714487373,-1.28138499384764,-1.28058955198037,
-1.27972680600245,-1.27835135481755,-1.27568418191224,-1.2495287345976,
-1.20066870967902,-1.12778343313502,-1.12351067297052,-1.12191250764918,
-1.12077966932391,-1.11971245657581,-1.11823305138376,-1.11529734185162,
-1.09324603946533,-1.05861260428938,-0.966055005163889,-0.961370678346296,
-0.960085047261387,-0.959328940478198,-0.958687231744595,-0.957893015902392,
-0.95703193160292,-0.955660542804421,-0.953004339971197,-0.927037404740657,
-0.878358327099164,-0.805153349665185,-0.800815022830284,-0.799206257082382,
-0.798070443248395,-0.797004075573314,-0.795531578903331,-0.792630071959325,
-0.771706381770003,-0.740582406387014,-0.695463179798476,-0.68895080292122,
-0.640955160043092,-0.638241416235582,-0.637300594714132,-0.636656020582063,
-0.636011195459987,-0.63518996880752,-0.634291356655268,-0.632830073313045,
-0.629931780106595,-0.622570278351487,-0.59408512482129,-0.499234711943945,
-0.496242225825804,-0.480245119230678,-0.477616947653999,-0.476054907710212,
-0.474862021359495,-0.473590401293034,-0.471610015611962,-0.46553268557093,
-0.372314046198989,-0.331458232353176,-0.327697006359998,-0.316686748383605,
-0.314948012015827,-0.314103472062978,-0.313460612642792,-0.312742031671555,
-0.31198730133634,-0.310869802223092,-0.308871244738963,-0.304430255999315,
-0.291203734391308,-0.266470356942769,-0.166067276683062,-0.16396932658475,
-0.156270181840844,-0.154012157762357,-0.152678592687857,-0.151619138598524,
-0.150205529603611,-0.147583083518611,-0.13348898393143,-0.105349081958357,
-0.00100413960794193),.UNSPECIFIED.);
#886=B_SPLINE_CURVE_WITH_KNOTS('',3,(#70097,#70098,#70099,#70100,#70101,
#70102,#70103,#70104,#70105,#70106,#70107),.UNSPECIFIED.,.F.,.F.,(4,1,1,
1,1,1,1,1,4),(411.548637620263,411.580474769127,412.579267172895,413.578059576663,
414.576851980431,415.575644384199,416.574436787967,417.573229191735,417.831820549658),
 .UNSPECIFIED.);
#887=B_SPLINE_CURVE_WITH_KNOTS('',3,(#70109,#70110,#70111,#70112,#70113,
#70114,#70115,#70116,#70117,#70118,#70119,#70120,#70121,#70122,#70123,#70124,
#70125,#70126,#70127,#70128,#70129,#70130,#70131,#70132,#70133,#70134,#70135,
#70136,#70137,#70138,#70139,#70140,#70141,#70142,#70143,#70144,#70145,#70146,
#70147,#70148,#70149,#70150,#70151,#70152,#70153,#70154,#70155,#70156,#70157,
#70158,#70159,#70160,#70161,#70162,#70163,#70164,#70165,#70166,#70167,#70168,
#70169,#70170,#70171,#70172,#70173,#70174,#70175,#70176,#70177,#70178,#70179,
#70180,#70181,#70182,#70183,#70184,#70185,#70186,#70187,#70188,#70189,#70190,
#70191,#70192,#70193,#70194,#70195,#70196,#70197,#70198,#70199,#70200,#70201,
#70202,#70203,#70204,#70205,#70206,#70207,#70208,#70209,#70210,#70211,#70212,
#70213,#70214,#70215,#70216,#70217,#70218,#70219,#70220,#70221,#70222,#70223,
#70224,#70225,#70226,#70227,#70228,#70229,#70230,#70231,#70232,#70233,#70234,
#70235,#70236,#70237,#70238,#70239,#70240,#70241,#70242,#70243,#70244,#70245,
#70246,#70247,#70248,#70249,#70250,#70251,#70252,#70253,#70254,#70255,#70256,
#70257,#70258,#70259,#70260,#70261,#70262,#70263,#70264,#70265,#70266,#70267,
#70268,#70269,#70270,#70271,#70272,#70273,#70274,#70275,#70276,#70277,#70278,
#70279,#70280,#70281,#70282,#70283,#70284,#70285,#70286,#70287,#70288,#70289,
#70290,#70291,#70292,#70293,#70294,#70295,#70296,#70297,#70298,#70299,#70300,
#70301,#70302,#70303,#70304,#70305,#70306,#70307,#70308,#70309,#70310,#70311,
#70312,#70313,#70314,#70315,#70316,#70317,#70318,#70319,#70320,#70321,#70322,
#70323,#70324,#70325,#70326,#70327,#70328,#70329,#70330,#70331,#70332,#70333,
#70334,#70335,#70336,#70337,#70338,#70339,#70340,#70341,#70342,#70343,#70344,
#70345,#70346,#70347,#70348,#70349,#70350,#70351,#70352,#70353,#70354,#70355,
#70356,#70357,#70358,#70359,#70360,#70361,#70362,#70363,#70364,#70365,#70366,
#70367,#70368,#70369,#70370,#70371,#70372,#70373,#70374,#70375,#70376,#70377,
#70378,#70379,#70380,#70381,#70382,#70383,#70384,#70385,#70386,#70387,#70388,
#70389,#70390,#70391,#70392,#70393,#70394,#70395,#70396,#70397,#70398,#70399,
#70400,#70401,#70402,#70403,#70404,#70405,#70406,#70407,#70408,#70409,#70410,
#70411,#70412,#70413,#70414,#70415,#70416,#70417,#70418,#70419,#70420,#70421,
#70422,#70423,#70424,#70425,#70426,#70427,#70428,#70429,#70430,#70431,#70432,
#70433,#70434,#70435,#70436,#70437,#70438,#70439,#70440,#70441,#70442,#70443,
#70444,#70445,#70446,#70447,#70448,#70449,#70450,#70451,#70452,#70453,#70454,
#70455,#70456,#70457,#70458,#70459,#70460,#70461,#70462,#70463,#70464,#70465,
#70466,#70467,#70468,#70469,#70470,#70471,#70472,#70473,#70474,#70475,#70476,
#70477,#70478,#70479,#70480,#70481,#70482,#70483,#70484,#70485,#70486,#70487,
#70488,#70489,#70490,#70491,#70492,#70493,#70494,#70495,#70496,#70497,#70498,
#70499,#70500,#70501,#70502,#70503,#70504,#70505,#70506,#70507,#70508,#70509,
#70510,#70511,#70512,#70513,#70514,#70515,#70516,#70517,#70518,#70519,#70520,
#70521,#70522,#70523,#70524,#70525,#70526,#70527,#70528,#70529,#70530,#70531,
#70532,#70533,#70534,#70535,#70536,#70537,#70538,#70539,#70540,#70541,#70542,
#70543,#70544,#70545,#70546,#70547,#70548,#70549,#70550,#70551,#70552,#70553,
#70554,#70555,#70556,#70557,#70558,#70559,#70560,#70561,#70562,#70563,#70564,
#70565,#70566,#70567,#70568,#70569,#70570,#70571,#70572,#70573,#70574,#70575,
#70576,#70577,#70578,#70579,#70580,#70581,#70582,#70583,#70584,#70585,#70586,
#70587,#70588,#70589,#70590,#70591,#70592,#70593,#70594,#70595,#70596,#70597,
#70598,#70599,#70600,#70601,#70602,#70603,#70604,#70605,#70606,#70607,#70608,
#70609,#70610,#70611,#70612,#70613,#70614,#70615,#70616,#70617,#70618,#70619,
#70620,#70621,#70622,#70623,#70624,#70625,#70626,#70627,#70628,#70629,#70630,
#70631,#70632,#70633,#70634,#70635,#70636,#70637,#70638,#70639,#70640,#70641,
#70642,#70643,#70644,#70645,#70646,#70647,#70648,#70649,#70650,#70651,#70652,
#70653,#70654,#70655,#70656,#70657,#70658,#70659,#70660,#70661,#70662,#70663,
#70664,#70665,#70666),.UNSPECIFIED.,.F.,.F.,(4,2,2,2,2,2,2,2,2,2,2,2,2,
2,2,2,2,2,2,2,2,2,2,2,2,2,2,2,2,2,2,2,2,2,2,2,2,2,2,2,2,2,2,2,2,2,2,2,2,
2,2,2,2,2,2,2,2,2,2,2,2,2,2,2,2,2,2,2,2,2,2,2,2,2,2,2,2,2,2,2,2,2,2,2,2,
2,2,2,2,2,2,2,2,2,2,2,2,2,2,2,2,2,2,2,2,2,2,2,2,2,2,2,2,2,2,2,2,2,2,2,2,
2,2,2,2,2,2,2,2,2,2,2,2,2,2,2,2,2,2,2,2,2,2,2,2,2,2,2,2,2,2,2,2,2,2,2,2,
2,2,2,2,2,2,2,2,2,2,2,2,2,2,2,2,2,2,2,2,2,2,2,2,2,2,2,2,2,2,2,2,2,2,2,2,
2,2,2,2,2,2,2,2,2,2,2,2,2,2,2,2,2,2,2,2,2,2,2,2,2,2,2,2,2,2,2,2,2,2,2,2,
2,2,2,2,2,2,2,2,2,2,2,2,2,2,2,2,2,2,2,2,2,2,2,2,2,2,2,2,2,2,2,2,2,2,2,2,
2,2,2,2,2,2,2,2,2,2,2,2,2,4),(-4.06049910102836,-3.98885752482128,-3.98628571019544,
-3.98469195091486,-3.98320785462953,-3.98214011736032,-3.9810093730988,
-3.97941850301221,-3.97519186879429,-3.90584130610861,-3.89048237730222,
-3.87601308438949,-3.83994592728347,-3.82475055393006,-3.82328769351999,
-3.82205961830065,-3.82132402914361,-3.82066507049597,-3.81981613209028,
-3.8180544617547,-3.8065440587236,-3.80463201303284,-3.74452665069794,-3.71401735447342,
-3.68094396614464,-3.67031011533946,-3.66358104600662,-3.66204983183634,
-3.66088270039567,-3.65969114215245,-3.6585711253673,-3.65702041234628,
-3.6538919375063,-3.62440639169627,-3.60547728889943,-3.57970784813515,
-3.50454695758624,-3.50065847777196,-3.49979412513344,-3.49898646866834,
-3.4983942741377,-3.49774781264562,-3.49659774668816,-3.49317735950503,
-3.43577708954707,-3.39818249297175,-3.35941524947579,-3.34231305900054,
-3.33955954318896,-3.33838531284719,-3.33718995189852,-3.33607614731679,
-3.33454934771791,-3.330710524477,-3.27841791799949,-3.22220749706289,-3.20118990040303,
-3.18238133233035,-3.17819929710273,-3.17699573014311,-3.1762655865804,
-3.17560528023819,-3.17476027025618,-3.17297230734869,-3.16086617571934,
-3.15829614981815,-3.15289177171601,-3.12080639242039,-3.05789909109812,
-3.02435686494712,-3.01834472207156,-3.01637595085011,-3.01509808306824,
-3.01390780363821,-3.01236125089029,-3.00912157059228,-2.98541029678503,
-2.97593596687526,-2.96791131043136,-2.88978496784511,-2.85999150429394,
-2.85570655511072,-2.85446452580222,-2.8537257345788,-2.8530672878009,-2.85222357263386,
-2.85048869651388,-2.83956215441281,-2.83728759360666,-2.83410228178253,
-2.8162338862243,-2.7416067843407,-2.70249494515861,-2.69810030260833,-2.69476602185416,
-2.6932133266055,-2.69202126468134,-2.69090176758201,-2.68935334751774,
-2.68538686174789,-2.61778475726787,-2.57376432014592,-2.54489019247849,
-2.53374011603199,-2.53213685814006,-2.53131986292278,-2.53066394368582,
-2.53000576025179,-2.52879769656697,-2.52492737844062,-2.42262746359116,
-2.37581983736633,-2.37216122534024,-2.37054264092001,-2.36934507155384,
-2.36823482956124,-2.36672159202005,-2.36296140621004,-2.31688755773626,
-2.29268467759209,-2.24969069604329,-2.22378449648682,-2.21115359728144,
-2.20950378823812,-2.20867730418549,-2.20808283274479,-2.20744513494251,
-2.20652858199373,-2.20397682426801,-2.20275491099092,-2.14250844297962,
-2.09370324500228,-2.070439592343,-2.0520335572599,-2.04921974607596,-2.04776570837877,
-2.04670202316632,-2.04555890540741,-2.04358455769836,-2.03807977099596,
-2.03091957374525,-2.0088737925009,-1.96460962312695,-1.89201062909916,
-1.88790816209106,-1.88667220203356,-1.88600842877215,-1.88535319867153,
-1.88454617224062,-1.88299056578486,-1.87312112517939,-1.85068301791431,
-1.76329320216655,-1.75416049926012,-1.7490647448628,-1.72987149661922,
-1.72678373944993,-1.7252737530139,-1.72409232657149,-1.72278464840351,
-1.72064172793675,-1.7131149752923,-1.66493477361444,-1.56983484418296,
-1.56529755976216,-1.56401247269335,-1.56326406995635,-1.56267293719772,
-1.56187618556825,-1.56036948442738,-1.55163231260533,-1.53294639006951,
-1.45375183039616,-1.40828474145392,-1.40453208640381,-1.40302006536907,
-1.40191006474474,-1.40071213340248,-1.39909196526675,-1.3954251179766,
-1.34786659278294,-1.24663285367013,-1.24246159355445,-1.24121738462658,
-1.24055183401719,-1.23989655780716,-1.2391081559464,-1.23761938106537,
-1.23574417883147,-1.1908037710805,-1.1293734115829,-1.11151490207392,-1.10348120616627,
-1.09802719382188,-1.09603595836976,-1.09307498461364,-1.09110670233415,
-1.08308579972866,-1.08081876610682,-1.0794699487634,-1.0782942069575,-1.0768474390265,
-1.07406974893305,-1.05660942503629,-1.01633193898139,-0.940996949372963,
-0.937395956764601,-0.93454042075786,-0.933992201958512,-0.920808756031269,
-0.91899932210531,-0.918137208769172,-0.917474265716635,-0.916860245296265,
-0.915817349368871,-0.912876367626713,-0.908478066816871,-0.882596613499722,
-0.835420366930702,-0.800808312108693,-0.793162479332177,-0.787691040513085,
-0.781983520004337,-0.761880625849114,-0.758749679727123,-0.757230697762973,
-0.756047719895461,-0.754743901503228,-0.752619887647664,-0.745282053454694,
-0.69915887202195,-0.633861981779868,-0.621714483177402,-0.618939913866563,
-0.616040596135668,-0.598422963831734,-0.596439795397862,-0.595637331722109,
-0.594968453735436,-0.594353789719638,-0.593395318234527,-0.591036614993808,
-0.587699413217694,-0.578773695082703,-0.556463444922131,-0.525893291528445,
-0.457582848829746,-0.456197936212814,-0.438994727746949,-0.436043903744468,
-0.43454086463401,-0.433359789442815,-0.43204726287174,-0.429884398786693,
-0.422166357163926,-0.396306967814914,-0.354576703673571,-0.317909442154778,
-0.276434382547346,-0.274056119835759,-0.273165317344658,-0.272534510490315,
-0.271937099890703,-0.271296460826856,-0.270471889413739,-0.267408673664023,
-0.237730563324097,-0.217684110991243,-0.142968757481856,-0.136548772213743,
-0.11657231593272,-0.113447187371181,-0.111929381906384,-0.110746576003267,
-0.109442191602947,-0.107315555633617,-0.0999522814260519,-0.053557751782706,
-0.000958120265015606),.UNSPECIFIED.);
#888=B_SPLINE_CURVE_WITH_KNOTS('',3,(#70668,#70669,#70670,#70671,#70672,
#70673,#70674,#70675,#70676,#70677,#70678,#70679,#70680,#70681,#70682,#70683,
#70684,#70685,#70686,#70687,#70688,#70689,#70690,#70691,#70692,#70693,#70694,
#70695,#70696,#70697,#70698,#70699,#70700,#70701,#70702,#70703,#70704,#70705,
#70706,#70707,#70708,#70709,#70710,#70711,#70712,#70713,#70714,#70715,#70716,
#70717,#70718,#70719,#70720,#70721,#70722,#70723,#70724,#70725,#70726,#70727,
#70728,#70729,#70730,#70731,#70732,#70733,#70734,#70735,#70736,#70737,#70738,
#70739,#70740,#70741,#70742,#70743,#70744,#70745,#70746,#70747,#70748,#70749,
#70750,#70751,#70752,#70753,#70754,#70755,#70756,#70757,#70758,#70759,#70760,
#70761,#70762,#70763,#70764,#70765,#70766,#70767,#70768,#70769,#70770,#70771,
#70772,#70773,#70774,#70775,#70776,#70777,#70778,#70779,#70780,#70781,#70782,
#70783,#70784,#70785,#70786,#70787,#70788,#70789,#70790,#70791,#70792,#70793,
#70794,#70795,#70796,#70797,#70798,#70799,#70800,#70801,#70802,#70803,#70804,
#70805,#70806,#70807,#70808,#70809,#70810,#70811,#70812,#70813,#70814,#70815,
#70816,#70817,#70818,#70819,#70820,#70821,#70822,#70823,#70824,#70825,#70826,
#70827,#70828,#70829,#70830,#70831,#70832,#70833,#70834,#70835,#70836,#70837,
#70838,#70839,#70840,#70841,#70842,#70843,#70844,#70845,#70846,#70847,#70848,
#70849,#70850,#70851,#70852,#70853,#70854,#70855,#70856,#70857,#70858,#70859,
#70860,#70861,#70862,#70863,#70864,#70865,#70866,#70867,#70868,#70869,#70870,
#70871,#70872,#70873,#70874,#70875,#70876,#70877,#70878,#70879,#70880,#70881,
#70882,#70883,#70884,#70885,#70886,#70887,#70888,#70889,#70890,#70891,#70892,
#70893,#70894,#70895,#70896,#70897,#70898,#70899,#70900,#70901,#70902,#70903,
#70904,#70905,#70906,#70907,#70908,#70909,#70910,#70911,#70912,#70913,#70914,
#70915,#70916,#70917,#70918,#70919,#70920,#70921,#70922,#70923,#70924,#70925,
#70926,#70927,#70928,#70929,#70930,#70931,#70932,#70933,#70934,#70935,#70936,
#70937,#70938,#70939,#70940,#70941,#70942,#70943,#70944,#70945,#70946,#70947,
#70948,#70949,#70950,#70951,#70952,#70953,#70954,#70955,#70956,#70957,#70958,
#70959,#70960,#70961,#70962,#70963,#70964,#70965,#70966,#70967,#70968,#70969,
#70970,#70971,#70972,#70973,#70974,#70975,#70976,#70977,#70978,#70979,#70980,
#70981,#70982,#70983,#70984,#70985,#70986,#70987,#70988,#70989,#70990,#70991,
#70992,#70993,#70994,#70995,#70996,#70997,#70998,#70999,#71000,#71001,#71002,
#71003,#71004,#71005,#71006,#71007,#71008,#71009,#71010,#71011,#71012,#71013,
#71014,#71015,#71016,#71017,#71018,#71019,#71020,#71021,#71022,#71023,#71024,
#71025,#71026,#71027,#71028,#71029,#71030,#71031,#71032,#71033,#71034,#71035,
#71036,#71037,#71038,#71039,#71040,#71041,#71042,#71043,#71044,#71045,#71046,
#71047,#71048,#71049,#71050,#71051,#71052,#71053,#71054,#71055,#71056,#71057,
#71058,#71059,#71060,#71061,#71062,#71063,#71064,#71065,#71066,#71067,#71068,
#71069,#71070,#71071,#71072,#71073,#71074,#71075,#71076,#71077,#71078,#71079,
#71080,#71081,#71082,#71083,#71084,#71085,#71086,#71087,#71088,#71089,#71090,
#71091,#71092,#71093,#71094,#71095,#71096,#71097,#71098,#71099,#71100,#71101,
#71102,#71103,#71104,#71105,#71106,#71107,#71108,#71109,#71110,#71111,#71112,
#71113,#71114,#71115,#71116,#71117,#71118,#71119,#71120,#71121,#71122,#71123,
#71124,#71125,#71126,#71127,#71128,#71129,#71130,#71131,#71132,#71133,#71134,
#71135,#71136,#71137,#71138,#71139,#71140,#71141,#71142,#71143,#71144,#71145,
#71146,#71147,#71148,#71149,#71150,#71151,#71152,#71153,#71154,#71155,#71156,
#71157,#71158,#71159,#71160,#71161,#71162,#71163,#71164,#71165,#71166,#71167,
#71168,#71169,#71170,#71171,#71172,#71173,#71174,#71175,#71176,#71177,#71178,
#71179,#71180,#71181,#71182,#71183,#71184,#71185,#71186,#71187,#71188,#71189,
#71190,#71191,#71192,#71193,#71194,#71195,#71196,#71197,#71198,#71199,#71200,
#71201),.UNSPECIFIED.,.F.,.F.,(4,2,2,2,2,2,2,2,2,2,2,2,2,2,2,2,2,2,2,2,
2,2,2,2,2,2,2,2,2,2,2,2,2,2,2,2,2,2,2,2,2,2,2,2,2,2,2,2,2,2,2,2,2,2,2,2,
2,2,2,2,2,2,2,2,2,2,2,2,2,2,2,2,2,2,2,2,2,2,2,2,2,2,2,2,2,2,2,2,2,2,2,2,
2,2,2,2,2,2,2,2,2,2,2,2,2,2,2,2,2,2,2,2,2,2,2,2,2,2,2,2,2,2,2,2,2,2,2,2,
2,2,2,2,2,2,2,2,2,2,2,2,2,2,2,2,2,2,2,2,2,2,2,2,2,2,2,2,2,2,2,2,2,2,2,2,
2,2,2,2,2,2,2,2,2,2,2,2,2,2,2,2,2,2,2,2,2,2,2,2,2,2,2,2,2,2,2,2,2,2,2,2,
2,2,2,2,2,2,2,2,2,2,2,2,2,2,2,2,2,2,2,2,2,2,2,2,2,2,2,2,2,2,2,2,2,2,2,2,
2,2,2,2,2,2,2,2,2,2,2,2,2,2,2,2,2,2,2,2,2,2,2,2,2,2,2,2,2,2,4),(-4.05995377572391,
-4.01400246747446,-4.01177154444041,-4.01056281431475,-4.00977009445503,
-4.00913956836879,-4.00854729014005,-4.00790213991193,-4.00695856989801,
-4.00422396151782,-3.95855758109048,-3.94974625837205,-3.94211776551452,
-3.92741103186041,-3.89376938653784,-3.85747901825741,-3.85113851675836,
-3.84912662567192,-3.84784832654309,-3.84665866287938,-3.84511435293067,
-3.84254534276043,-3.82763516026328,-3.82190593181161,-3.82005063205414,
-3.74452293753362,-3.71125939823236,-3.69624643017317,-3.69137826647667,
-3.68819647998594,-3.68738314770942,-3.68674632972713,-3.68615106200478,
-3.68551601504203,-3.68460889888909,-3.68211844133079,-3.6400014950322,
-3.58836716214006,-3.58068159176122,-3.55199496804809,-3.5303112652294,
-3.52738719040587,-3.525910422878,-3.52484382715423,-3.5237104454478,-3.52178488726442,
-3.516601769143,-3.43425896573359,-3.39147744723565,-3.3770460237176,-3.37010233023217,
-3.36732603006827,-3.36528527798725,-3.36438559122186,-3.36371616443874,
-3.36309561792888,-3.36224255261446,-3.36053996521379,-3.34578761395255,
-3.34084897727765,-3.33872045605109,-3.3267222450338,-3.26009308420307,
-3.20873038533377,-3.20517671471311,-3.20357739193803,-3.20238314927038,
-3.20126812007694,-3.19973610230576,-3.19586567633618,-3.13986222297861,
-3.09135204547227,-3.04584090507054,-3.04306545438893,-3.04204617534767,
-3.04143280730987,-3.04076736907386,-3.03988817812,-3.03791766483837,-3.02071296851616,
-3.01929473866048,-2.93599591256572,-2.89100460269533,-2.88623486374829,
-2.8826462213513,-2.88104051895364,-2.87984526450297,-2.87873199072358,
-2.8772065900912,-2.87337477368271,-2.82161048964312,-2.75110192876342,
-2.72483912826716,-2.72216619863406,-2.72018481375698,-2.71929714934193,
-2.7186298596449,-2.71800618246504,-2.71714118322686,-2.71491985330561,
-2.68320058823522,-2.60427179187408,-2.5762213926229,-2.56216410406148,
-2.55954413243011,-2.55813129763701,-2.55696883133844,-2.55559783189003,
-2.55323396547082,-2.54426183583299,-2.54057346086215,-2.53861963074762,
-2.44801699085874,-2.4235795518854,-2.40172973975032,-2.39811519434472,
-2.39698470232759,-2.39627097185911,-2.39560546454292,-2.39472598014229,
-2.39275396679636,-2.37549944454451,-2.37324268897085,-2.36955568888835,
-2.35729532833842,-2.31903765467566,-2.27905061989296,-2.24459663141503,
-2.2384555718358,-2.23646758360399,-2.23519444708779,-2.23400252002539,
-2.23244515985288,-2.22902572873452,-2.20136674129527,-2.1098761421412,
-2.080063628466,-2.07571501422694,-2.07450537978201,-2.07377386619003,-2.07311388027818,
-2.07227134675223,-2.07049624015617,-2.0586869921538,-2.03151183110093,
-1.93768582828269,-1.91773894619717,-1.9146160265192,-1.91309900710585,
-1.91191668402246,-1.9106127003078,-1.9084864209234,-1.90112151627912,-1.85469715316082,
-1.75754713182159,-1.75308027059876,-1.75180281420884,-1.75105608935098,
-1.75046471014248,-1.74966561687974,-1.7481479941862,-1.73917429703633,
-1.72007457800104,-1.6728486127334,-1.59747311081948,-1.59273564553788,
-1.59088074985169,-1.58976090372091,-1.58856896044566,-1.58698548805259,
-1.58351856837576,-1.50913360032373,-1.43456899114881,-1.43032760249357,
-1.42907534677448,-1.42840819590629,-1.42775934481914,-1.42696027801401,
-1.4254429456969,-1.4164774746771,-1.39738627488976,-1.35019021136672,-1.27439697017666,
-1.26991985430255,-1.26828950197514,-1.26714781367578,-1.26598873624409,
-1.26451305503826,-1.26290364082852,-1.26029476076451,-1.25515611370009,
-1.20380233072963,-1.11878046657677,-1.10839277852334,-1.10668407267769,
-1.10584548448627,-1.1051874858975,-1.10444537597366,-1.10318892273092,
-1.09834419291398,-1.0621105099933,-0.967320426640924,-0.966246121807509,
-0.949271459751717,-0.946333226743836,-0.944833057224183,-0.943677226015442,
-0.94239752142191,-0.941061394927552,-0.939102687463249,-0.935644433181199,
-0.928115537650841,-0.905649194183061,-0.861229863714368,-0.836503950591983,
-0.787270204849993,-0.784517322255822,-0.783570859245963,-0.7829247223026,
-0.782332326887393,-0.781523655669347,-0.779960644602817,-0.769910391568304,
-0.746247913068194,-0.698323535060005,-0.628453073134337,-0.624373580611973,
-0.622806405755344,-0.621681864659135,-0.620516052873785,-0.619004516850361,
-0.617335132726419,-0.6145826687902,-0.60905502830531,-0.59488530601837,
-0.562267698950175,-0.466966483521416,-0.46229035383612,-0.461005510610261,
-0.460249551268411,-0.459593405381632,-0.458775484052763,-0.457168370057543,
-0.445914597657873,-0.412535385543892,-0.373207296041935,-0.308192821483237,
-0.30682643585624,-0.301953614440325,-0.300076428659167,-0.29895210150243,
-0.297819315679176,-0.296313071123386,-0.293217396221707,-0.28920593574069,
-0.280010478350127,-0.253529604370361,-0.150423073130263,-0.140168445430379,
-0.138466201320709,-0.137628779896677,-0.136970753884912,-0.136227595512537,
-0.134966993683787,-0.130078008043466,-0.106848936157074,-0.000958066444032279),
 .UNSPECIFIED.);
#889=B_SPLINE_CURVE_WITH_KNOTS('',3,(#71202,#71203,#71204,#71205,#71206,
#71207,#71208,#71209,#71210,#71211,#71212,#71213,#71214,#71215,#71216,#71217,
#71218,#71219,#71220,#71221,#71222,#71223,#71224,#71225,#71226,#71227,#71228,
#71229,#71230,#71231,#71232,#71233,#71234,#71235,#71236,#71237,#71238,#71239,
#71240,#71241,#71242,#71243,#71244,#71245,#71246,#71247,#71248,#71249,#71250,
#71251,#71252,#71253,#71254,#71255,#71256,#71257,#71258,#71259,#71260,#71261,
#71262,#71263,#71264,#71265,#71266,#71267,#71268,#71269,#71270,#71271,#71272,
#71273,#71274,#71275,#71276,#71277,#71278,#71279,#71280,#71281,#71282,#71283,
#71284,#71285,#71286,#71287,#71288,#71289,#71290,#71291,#71292,#71293,#71294,
#71295,#71296,#71297,#71298,#71299,#71300,#71301,#71302,#71303,#71304,#71305,
#71306,#71307,#71308,#71309,#71310,#71311,#71312,#71313,#71314,#71315,#71316,
#71317,#71318,#71319,#71320,#71321,#71322,#71323,#71324,#71325,#71326,#71327,
#71328,#71329,#71330,#71331,#71332,#71333,#71334,#71335,#71336,#71337,#71338,
#71339,#71340,#71341,#71342,#71343,#71344,#71345,#71346,#71347,#71348,#71349,
#71350,#71351,#71352,#71353,#71354,#71355,#71356,#71357,#71358,#71359,#71360,
#71361,#71362,#71363,#71364,#71365,#71366,#71367,#71368,#71369,#71370,#71371,
#71372,#71373,#71374,#71375,#71376,#71377,#71378,#71379,#71380,#71381,#71382,
#71383,#71384,#71385,#71386,#71387,#71388,#71389,#71390,#71391,#71392,#71393,
#71394,#71395,#71396,#71397,#71398,#71399,#71400,#71401,#71402,#71403,#71404,
#71405,#71406,#71407,#71408,#71409,#71410,#71411,#71412,#71413,#71414,#71415,
#71416,#71417,#71418,#71419,#71420,#71421,#71422,#71423,#71424,#71425,#71426,
#71427,#71428,#71429,#71430,#71431,#71432,#71433,#71434,#71435,#71436,#71437,
#71438,#71439,#71440,#71441,#71442,#71443,#71444,#71445,#71446,#71447,#71448,
#71449,#71450,#71451,#71452,#71453,#71454,#71455,#71456,#71457,#71458,#71459,
#71460,#71461,#71462,#71463,#71464,#71465,#71466,#71467,#71468,#71469,#71470,
#71471,#71472,#71473,#71474,#71475,#71476,#71477,#71478,#71479,#71480,#71481,
#71482,#71483,#71484,#71485,#71486,#71487,#71488,#71489,#71490,#71491,#71492,
#71493,#71494,#71495,#71496,#71497,#71498,#71499,#71500,#71501,#71502,#71503,
#71504,#71505,#71506,#71507,#71508,#71509,#71510,#71511,#71512,#71513,#71514,
#71515,#71516,#71517,#71518,#71519,#71520,#71521,#71522,#71523,#71524,#71525,
#71526,#71527,#71528,#71529,#71530,#71531,#71532,#71533,#71534,#71535,#71536,
#71537,#71538,#71539,#71540,#71541,#71542,#71543,#71544,#71545,#71546,#71547,
#71548,#71549,#71550,#71551,#71552,#71553,#71554,#71555,#71556,#71557,#71558,
#71559,#71560,#71561,#71562,#71563,#71564,#71565,#71566,#71567,#71568,#71569,
#71570,#71571,#71572,#71573,#71574,#71575,#71576,#71577,#71578,#71579,#71580,
#71581,#71582,#71583,#71584,#71585,#71586,#71587,#71588,#71589,#71590,#71591,
#71592,#71593,#71594,#71595,#71596,#71597,#71598,#71599,#71600,#71601,#71602,
#71603,#71604,#71605,#71606,#71607,#71608,#71609,#71610,#71611,#71612,#71613,
#71614,#71615,#71616,#71617,#71618,#71619,#71620,#71621,#71622,#71623,#71624,
#71625,#71626,#71627,#71628,#71629,#71630,#71631,#71632,#71633,#71634,#71635,
#71636,#71637,#71638,#71639,#71640,#71641,#71642,#71643,#71644,#71645,#71646,
#71647,#71648,#71649,#71650,#71651,#71652,#71653,#71654,#71655,#71656,#71657,
#71658,#71659,#71660,#71661,#71662,#71663,#71664,#71665,#71666,#71667,#71668,
#71669,#71670,#71671,#71672,#71673,#71674,#71675,#71676,#71677,#71678,#71679,
#71680,#71681,#71682,#71683,#71684,#71685,#71686,#71687,#71688,#71689,#71690,
#71691,#71692,#71693,#71694,#71695,#71696,#71697,#71698,#71699,#71700,#71701,
#71702,#71703,#71704,#71705,#71706,#71707,#71708,#71709,#71710,#71711,#71712,
#71713,#71714,#71715,#71716,#71717,#71718,#71719,#71720,#71721,#71722,#71723,
#71724,#71725,#71726,#71727,#71728,#71729,#71730,#71731,#71732,#71733,#71734,
#71735,#71736,#71737,#71738,#71739,#71740,#71741,#71742,#71743,#71744,#71745,
#71746,#71747,#71748,#71749,#71750,#71751,#71752,#71753),.UNSPECIFIED.,
 .F.,.F.,(4,2,2,2,2,2,2,2,2,2,2,2,2,2,2,2,2,2,2,2,2,2,2,2,2,2,2,2,2,2,2,
2,2,2,2,2,2,2,2,2,2,2,2,2,2,2,2,2,2,2,2,2,2,2,2,2,2,2,2,2,2,2,2,2,2,2,2,
2,2,2,2,2,2,2,2,2,2,2,2,2,2,2,2,2,2,2,2,2,2,2,2,2,2,2,2,2,2,2,2,2,2,2,2,
2,2,2,2,2,2,2,2,2,2,2,2,2,2,2,2,2,2,2,2,2,2,2,2,2,2,2,2,2,2,2,2,2,2,2,2,
2,2,2,2,2,2,2,2,2,2,2,2,2,2,2,2,2,2,2,2,2,2,2,2,2,2,2,2,2,2,2,2,2,2,2,2,
2,2,2,2,2,2,2,2,2,2,2,2,2,2,2,2,2,2,2,2,2,2,2,2,2,2,2,2,2,2,2,2,2,2,2,2,
2,2,2,2,2,2,2,2,2,2,2,2,2,2,2,2,2,2,2,2,2,2,2,2,2,2,2,2,2,2,2,2,2,2,2,2,
2,2,2,2,2,2,2,2,2,2,2,2,2,2,2,2,2,2,2,2,2,2,2,2,2,2,2,2,4),(-4.06264891370286,
-4.04466481678739,-4.04171944035511,-4.03996985759614,-4.03871927843569,
-4.03761859860726,-4.03642671242435,-4.03487264716332,-4.03227246129462,
-4.01681467878756,-4.01014125613746,-3.90573478602837,-3.8871846779329,
-3.87850842302826,-3.87700395232275,-3.87620740433803,-3.87561599675183,
-3.87496292345712,-3.87378138823818,-3.87012395580404,-3.80980203232441,
-3.76104296925034,-3.73316357016784,-3.72399629271692,-3.71999348829215,
-3.71690092715767,-3.71539616443503,-3.71426245673253,-3.7131369394838,
-3.71156744014438,-3.70747653186516,-3.64881087907444,-3.62401254388835,
-3.61656188127699,-3.60789424833173,-3.59740056822543,-3.56736416612173,
-3.55596378725396,-3.55435136909462,-3.55353220732303,-3.55288180596164,
-3.5521285504499,-3.55085586509878,-3.54629764461666,-3.45204318794294,
-3.41364352788284,-3.40242957146284,-3.39778104250459,-3.39535627288935,
-3.3938239864202,-3.39240498643094,-3.39125143545477,-3.38991201369727,
-3.38762951064948,-3.37971709624268,-3.37747988972333,-3.3746353645517,
-3.37263237261971,-3.36720801473551,-3.28252509320965,-3.27084231774962,
-3.23709310366739,-3.23401418446853,-3.23178044683541,-3.23084446535944,
-3.23017142411008,-3.22955435515529,-3.22871594608443,-3.22707224142077,
-3.21408280073917,-3.21258201094603,-3.13144330822818,-3.08047434810702,
-3.07535528653699,-3.07275338730131,-3.07114668987156,-3.06967411033925,
-3.06851480809128,-3.06737197226251,-3.06573842047608,-3.06124276196288,
-2.98549381977511,-2.93819581239956,-2.9190780865949,-2.91009694569104,
-2.9085784733559,-2.90777898152405,-2.90718732933246,-2.90644028681986,
-2.90516235469261,-2.90069445661373,-2.80352244961704,-2.77972659583146,
-2.75427434874244,-2.75085308393796,-2.74890909770608,-2.74757892818489,
-2.74630379729038,-2.7451475854759,-2.74363936600893,-2.740664919527,-2.72301519728503,
-2.71692084504026,-2.70649715419583,-2.68570361411242,-2.62591533664153,
-2.59152072844372,-2.58680738603405,-2.58556264122349,-2.58482305240464,
-2.58416442844553,-2.58332120437218,-2.58158982747912,-2.57075243747133,
-2.47770335757685,-2.43401398621811,-2.42932359070342,-2.42578259617335,
-2.42418506236398,-2.42299056965065,-2.42187415897067,-2.42033844524547,
-2.41644924676154,-2.35792623016082,-2.32567410053728,-2.29273912264715,
-2.27373897086213,-2.26453994747926,-2.26301199780479,-2.26221059521409,
-2.2616188576344,-2.26087347288027,-2.25960256010805,-2.25519688990326,
-2.1572357926411,-2.10651633922664,-2.10298966090939,-2.10139490091177,
-2.10020098467784,-2.09908402647144,-2.09754585470916,-2.09364144259511,
-2.03143342376781,-1.94568588945432,-1.94121698804714,-1.93993908572206,
-1.93919213110808,-1.93860058744174,-1.93780129439016,-1.93628336519513,
-1.92730983372192,-1.9082076668517,-1.86097829719755,-1.81750874641717,
-1.80678277047357,-1.80099151151946,-1.80001860086326,-1.78295564961322,
-1.78001214956565,-1.77851062024225,-1.77732964203715,-1.77601609720063,
-1.77384896224531,-1.76608904582066,-1.71528954659117,-1.63723895592994,
-1.61967407370476,-1.61769219268508,-1.61688987243586,-1.61622096245566,
-1.61552635018331,-1.61448420297336,-1.61156312607422,-1.56827757619857,
-1.46434374419021,-1.46271710076099,-1.45798394544778,-1.45612947616272,
-1.45500951206666,-1.45381715969488,-1.45223266033903,-1.44876155980102,
-1.37235721928435,-1.29937739262119,-1.2954602912155,-1.29424619105613,
-1.29358662310028,-1.29294348821077,-1.29215074485718,-1.29129178900118,
-1.28992563280379,-1.24556146210342,-1.14140955031371,-1.14001302734392,
-1.13510811926426,-1.1332257918778,-1.13210048334515,-1.13091099351039,
-1.12934470803984,-1.12596994972009,-1.07434393310633,-1.00208523049849,
-0.974195601435886,-0.972029966830966,-0.971174235177764,-0.970552785005667,
-0.969896912539696,-0.969023552505082,-0.968038602582755,-0.961778676708886,
-0.949855964905436,-0.930587346958811,-0.842672860523167,-0.815039886352264,
-0.811620300002119,-0.81006256115565,-0.808870216021372,-0.807596508539697,
-0.805607371545677,-0.799460772993834,-0.764958629994796,-0.749888589531647,
-0.738227608248846,-0.654482738438058,-0.649959783302609,-0.648676001491574,
-0.647927745510757,-0.647283587130959,-0.646477620639891,-0.6456002326701,
-0.644189950782242,-0.606020150324919,-0.560186106112749,-0.518588038663505,
-0.511559193756308,-0.491891115511732,-0.488779975478132,-0.487264866943717,
-0.48608230319546,-0.48477629321908,-0.482642734719899,-0.475213988144116,
-0.428120201063305,-0.416854710770204,-0.407719220631319,-0.399998861959737,
-0.393305527808217,-0.371011617528432,-0.352438741898368,-0.328724171930144,
-0.326635097231675,-0.325792516975249,-0.325174475984557,-0.324516105602696,
-0.323613095556591,-0.322600375285419,-0.315647102101332,-0.301857080080799,
-0.275421913256252,-0.186220713459997,-0.169003008704053,-0.166051551319051,
-0.164548433991943,-0.163367416991245,-0.162055078578265,-0.159892808409297,
-0.152179789379607,-0.126330690551008,-0.097875296897731,-0.0372463253441361,
-0.00709930852854725,-0.00423362856377661,-0.00316447147116906,-0.00253401405903737,
-0.00190190014399343,-0.00125763970154655),.UNSPECIFIED.);
#890=B_SPLINE_CURVE_WITH_KNOTS('',3,(#71792,#71793,#71794,#71795,#71796,
#71797,#71798,#71799,#71800,#71801,#71802,#71803,#71804,#71805,#71806,#71807,
#71808,#71809,#71810,#71811,#71812,#71813,#71814,#71815,#71816,#71817,#71818,
#71819,#71820,#71821,#71822,#71823,#71824,#71825,#71826,#71827,#71828,#71829,
#71830,#71831,#71832,#71833,#71834,#71835,#71836,#71837,#71838,#71839,#71840,
#71841,#71842,#71843,#71844,#71845,#71846,#71847,#71848,#71849,#71850,#71851,
#71852),.UNSPECIFIED.,.F.,.F.,(4,3,3,3,3,3,3,3,3,3,3,3,3,3,3,3,3,3,3,3,
4),(-0.733313182989362,-0.716294493786964,-0.670821266456911,-0.640789190757952,
-0.62133617984982,-0.569925089098463,-0.543537875173823,-0.523380244131678,
-0.461289689980783,-0.415691816844391,-0.398550463653533,-0.341537216799208,
-0.279356146584203,-0.262754828049987,-0.241371242852862,-0.181974595834089,
-0.136653796141601,-0.117467040668732,-0.0607494647494775,-0.00403188883022294,
0.),.UNSPECIFIED.);
#891=B_SPLINE_CURVE_WITH_KNOTS('',3,(#71854,#71855,#71856,#71857),
 .UNSPECIFIED.,.F.,.F.,(4,4),(0.,0.0148351583007577),.UNSPECIFIED.);
#892=B_SPLINE_CURVE_WITH_KNOTS('',3,(#71858,#71859,#71860,#71861,#71862,
#71863,#71864,#71865,#71866,#71867,#71868,#71869,#71870,#71871,#71872,#71873,
#71874,#71875,#71876,#71877,#71878,#71879,#71880,#71881,#71882,#71883,#71884,
#71885,#71886,#71887,#71888,#71889,#71890,#71891,#71892,#71893,#71894,#71895,
#71896,#71897,#71898,#71899,#71900,#71901,#71902,#71903,#71904,#71905,#71906,
#71907,#71908,#71909,#71910,#71911,#71912,#71913,#71914,#71915,#71916,#71917,
#71918),.UNSPECIFIED.,.F.,.F.,(4,3,3,3,3,3,3,3,3,3,3,3,3,3,3,3,3,3,3,3,
4),(-0.744397949170595,-0.723616735492759,-0.67829295687754,-0.65916345595812,
-0.604538037765455,-0.577309499118107,-0.555880865424909,-0.495420190252057,
-0.44066178318746,-0.425583850132311,-0.378804123990258,-0.331770874270554,
-0.304228573210021,-0.284737624550849,-0.222500848162153,-0.158731754394471,
-0.15102870873837,-0.135594328587619,-0.0696436621400311,-0.00369299569244323,
0.),.UNSPECIFIED.);
#893=B_SPLINE_CURVE_WITH_KNOTS('',3,(#73751,#73752,#73753,#73754,#73755,
#73756,#73757,#73758,#73759,#73760,#73761,#73762,#73763,#73764,#73765,#73766,
#73767,#73768,#73769,#73770,#73771,#73772,#73773,#73774,#73775,#73776,#73777,
#73778,#73779,#73780,#73781,#73782,#73783,#73784,#73785,#73786,#73787,#73788,
#73789,#73790,#73791,#73792,#73793,#73794,#73795,#73796,#73797,#73798,#73799,
#73800,#73801,#73802,#73803,#73804,#73805,#73806,#73807,#73808,#73809,#73810,
#73811,#73812,#73813,#73814),.UNSPECIFIED.,.F.,.F.,(4,3,3,3,3,3,3,3,3,3,
3,3,3,3,3,3,3,3,3,3,3,4),(-0.744397949170525,-0.723616735492616,-0.667849821071476,
-0.659163469387309,-0.641214414426581,-0.591076386810976,-0.569755772081005,
-0.54382354565886,-0.483363318569143,-0.440662303964159,-0.421846140318383,
-0.37880412399009,-0.325805172793596,-0.300222673925967,-0.279280379085805,
-0.216042753422732,-0.166808319204116,-0.15102867511565,-0.104251465971131,
-0.0393806484926011,-0.00369301913285791,0.),.UNSPECIFIED.);
#894=B_SPLINE_CURVE_WITH_KNOTS('',3,(#73816,#73817,#73818,#73819,#73820,
#73821,#73822,#73823,#73824,#73825,#73826,#73827,#73828,#73829,#73830,#73831,
#73832,#73833,#73834,#73835,#73836,#73837,#73838,#73839,#73840,#73841,#73842,
#73843,#73844,#73845,#73846,#73847,#73848,#73849,#73850,#73851,#73852,#73853,
#73854,#73855,#73856,#73857,#73858,#73859,#73860,#73861,#73862,#73863,#73864,
#73865,#73866,#73867,#73868,#73869,#73870,#73871,#73872,#73873,#73874,#73875,
#73876,#73877,#73878,#73879,#73880,#73881,#73882),.UNSPECIFIED.,.F.,.F.,
(4,3,3,3,3,3,3,3,3,3,3,3,3,3,3,3,3,3,3,3,3,3,4),(-0.733313036857812,-0.71629449378717,
-0.650953385595915,-0.640774184990949,-0.621184304739324,-0.570131565600329,
-0.547731071725486,-0.528561181480364,-0.466083910280972,-0.429328908955862,
-0.40653620544786,-0.387326345085585,-0.341537216799262,-0.27727496749461,
-0.259045768830733,-0.236144865812168,-0.178116580240476,-0.147890161229715,
-0.127897896546065,-0.109092903344164,-0.0531230889165709,-0.00403172352540138,
-8.60864227220048E-14),.UNSPECIFIED.);
#1080=PLANE('',#10489);
#1081=PLANE('',#10490);
#1082=PLANE('',#10491);
#1083=PLANE('',#10492);
#1084=PLANE('',#10493);
#1085=PLANE('',#10494);
#1086=PLANE('',#10495);
#1087=PLANE('',#10496);
#1088=PLANE('',#10497);
#1089=PLANE('',#10498);
#1090=PLANE('',#10503);
#1469=LINE('',#71757,#2005);
#1470=LINE('',#71759,#2006);
#1471=LINE('',#71761,#2007);
#1472=LINE('',#71762,#2008);
#1473=LINE('',#71765,#2009);
#1474=LINE('',#71767,#2010);
#1475=LINE('',#71768,#2011);
#1476=LINE('',#71771,#2012);
#1477=LINE('',#71773,#2013);
#1478=LINE('',#71774,#2014);
#1479=LINE('',#71777,#2015);
#1480=LINE('',#71779,#2016);
#1481=LINE('',#71780,#2017);
#1482=LINE('',#71783,#2018);
#1483=LINE('',#71785,#2019);
#1484=LINE('',#71786,#2020);
#1485=LINE('',#71788,#2021);
#1486=LINE('',#71789,#2022);
#1487=LINE('',#75719,#2023);
#1488=LINE('',#75722,#2024);
#2005=VECTOR('',#12013,0.999999999999999);
#2006=VECTOR('',#12014,1.);
#2007=VECTOR('',#12015,0.999999999999999);
#2008=VECTOR('',#12016,1.);
#2009=VECTOR('',#12019,1.);
#2010=VECTOR('',#12020,1.);
#2011=VECTOR('',#12021,1.);
#2012=VECTOR('',#12024,1.);
#2013=VECTOR('',#12025,1.);
#2014=VECTOR('',#12026,1.);
#2015=VECTOR('',#12029,1.);
#2016=VECTOR('',#12030,1.);
#2017=VECTOR('',#12031,1.);
#2018=VECTOR('',#12034,1.);
#2019=VECTOR('',#12035,1.);
#2020=VECTOR('',#12036,1.);
#2021=VECTOR('',#12039,1.);
#2022=VECTOR('',#12040,1.);
#2023=VECTOR('',#12053,0.375);
#2024=VECTOR('',#12056,0.38);
#2326=CYLINDRICAL_SURFACE('',#10481,0.3933);
#2327=CYLINDRICAL_SURFACE('',#10486,0.322275);
#2666=FACE_OUTER_BOUND('',#3218,.T.);
#2667=FACE_OUTER_BOUND('',#3221,.T.);
#2668=FACE_OUTER_BOUND('',#3222,.T.);
#2669=FACE_OUTER_BOUND('',#3223,.T.);
#2670=FACE_OUTER_BOUND('',#3224,.T.);
#2671=FACE_OUTER_BOUND('',#3225,.T.);
#2672=FACE_OUTER_BOUND('',#3226,.T.);
#2673=FACE_OUTER_BOUND('',#3227,.T.);
#2674=FACE_OUTER_BOUND('',#3228,.T.);
#2675=FACE_OUTER_BOUND('',#3229,.T.);
#2676=FACE_OUTER_BOUND('',#3230,.T.);
#2677=FACE_OUTER_BOUND('',#3231,.T.);
#2678=FACE_OUTER_BOUND('',#3232,.T.);
#2679=FACE_OUTER_BOUND('',#3233,.T.);
#2680=FACE_OUTER_BOUND('',#3234,.T.);
#2681=FACE_OUTER_BOUND('',#3235,.T.);
#2682=FACE_OUTER_BOUND('',#3236,.T.);
#3218=EDGE_LOOP('',(#7725));
#3219=EDGE_LOOP('',(#7726,#7727,#7728,#7729,#7730,#7731,#7732,#7733,#7734,
#7735,#7736,#7737,#7738,#7739,#7740,#7741,#7742,#7743,#7744,#7745,#7746,
#7747,#7748,#7749,#7750,#7751,#7752,#7753,#7754,#7755,#7756,#7757,#7758,
#7759,#7760,#7761,#7762,#7763,#7764,#7765,#7766,#7767,#7768,#7769,#7770,
#7771,#7772,#7773,#7774,#7775,#7776,#7777,#7778,#7779,#7780,#7781,#7782,
#7783,#7784,#7785,#7786,#7787,#7788,#7789,#7790,#7791,#7792,#7793,#7794,
#7795,#7796,#7797,#7798,#7799,#7800,#7801,#7802,#7803,#7804,#7805,#7806,
#7807,#7808,#7809,#7810,#7811,#7812,#7813,#7814,#7815,#7816,#7817,#7818,
#7819,#7820,#7821,#7822,#7823,#7824,#7825,#7826,#7827,#7828,#7829,#7830,
#7831,#7832,#7833,#7834,#7835,#7836,#7837,#7838,#7839,#7840,#7841,#7842,
#7843,#7844,#7845,#7846,#7847,#7848,#7849,#7850,#7851,#7852,#7853,#7854,
#7855,#7856,#7857,#7858,#7859,#7860,#7861,#7862,#7863,#7864,#7865,#7866,
#7867,#7868,#7869,#7870,#7871,#7872,#7873,#7874,#7875));
#3220=EDGE_LOOP('',(#7876));
#3221=EDGE_LOOP('',(#7877,#7878,#7879,#7880,#7881,#7882,#7883,#7884,#7885,
#7886,#7887,#7888,#7889,#7890,#7891,#7892,#7893,#7894,#7895,#7896,#7897,
#7898,#7899,#7900,#7901,#7902,#7903,#7904,#7905,#7906,#7907,#7908,#7909,
#7910,#7911,#7912,#7913,#7914,#7915,#7916,#7917,#7918,#7919,#7920,#7921,
#7922,#7923,#7924,#7925,#7926,#7927,#7928,#7929,#7930,#7931,#7932,#7933,
#7934,#7935,#7936,#7937,#7938,#7939,#7940,#7941,#7942,#7943,#7944,#7945,
#7946,#7947,#7948,#7949,#7950,#7951,#7952,#7953,#7954,#7955,#7956,#7957,
#7958,#7959));
#3222=EDGE_LOOP('',(#7960,#7961,#7962,#7963));
#3223=EDGE_LOOP('',(#7964,#7965,#7966,#7967));
#3224=EDGE_LOOP('',(#7968,#7969,#7970,#7971));
#3225=EDGE_LOOP('',(#7972,#7973,#7974,#7975));
#3226=EDGE_LOOP('',(#7976,#7977,#7978,#7979));
#3227=EDGE_LOOP('',(#7980,#7981,#7982,#7983));
#3228=EDGE_LOOP('',(#7984,#7985,#7986,#7987,#7988,#7989));
#3229=EDGE_LOOP('',(#7990,#7991,#7992,#7993,#7994));
#3230=EDGE_LOOP('',(#7995,#7996,#7997,#7998,#7999,#8000,#8001,#8002,#8003,
#8004,#8005,#8006,#8007,#8008,#8009,#8010,#8011,#8012,#8013,#8014,#8015,
#8016,#8017,#8018,#8019,#8020,#8021,#8022,#8023,#8024,#8025,#8026,#8027,
#8028,#8029,#8030,#8031,#8032,#8033,#8034,#8035,#8036,#8037,#8038,#8039,
#8040,#8041,#8042,#8043,#8044,#8045,#8046,#8047,#8048,#8049,#8050,#8051,
#8052,#8053,#8054,#8055,#8056,#8057,#8058,#8059,#8060,#8061,#8062,#8063,
#8064,#8065,#8066,#8067,#8068,#8069,#8070,#8071,#8072,#8073,#8074,#8075,
#8076,#8077,#8078,#8079,#8080,#8081,#8082,#8083,#8084,#8085,#8086,#8087,
#8088,#8089,#8090,#8091,#8092,#8093,#8094,#8095,#8096,#8097,#8098,#8099,
#8100,#8101,#8102,#8103,#8104,#8105,#8106,#8107,#8108,#8109,#8110));
#3231=EDGE_LOOP('',(#8111,#8112,#8113,#8114));
#3232=EDGE_LOOP('',(#8115,#8116,#8117,#8118,#8119,#8120,#8121,#8122,#8123,
#8124,#8125,#8126,#8127,#8128,#8129,#8130,#8131,#8132,#8133,#8134,#8135,
#8136,#8137,#8138,#8139,#8140,#8141,#8142,#8143,#8144,#8145,#8146,#8147,
#8148,#8149,#8150,#8151,#8152,#8153,#8154,#8155,#8156,#8157,#8158,#8159,
#8160,#8161,#8162,#8163,#8164,#8165,#8166,#8167,#8168,#8169,#8170,#8171,
#8172,#8173,#8174,#8175,#8176,#8177,#8178,#8179,#8180,#8181,#8182,#8183,
#8184,#8185,#8186,#8187,#8188,#8189,#8190,#8191,#8192,#8193,#8194,#8195,
#8196,#8197,#8198,#8199,#8200,#8201,#8202,#8203,#8204,#8205,#8206,#8207,
#8208,#8209,#8210,#8211,#8212,#8213,#8214,#8215,#8216,#8217,#8218,#8219,
#8220,#8221,#8222,#8223,#8224,#8225,#8226,#8227,#8228,#8229,#8230,#8231,
#8232));
#3233=EDGE_LOOP('',(#8233));
#3234=EDGE_LOOP('',(#8234,#8235,#8236,#8237));
#3235=EDGE_LOOP('',(#8238,#8239,#8240,#8241));
#3236=EDGE_LOOP('',(#8242));
#3237=EDGE_LOOP('',(#8243,#8244,#8245,#8246,#8247,#8248));
#3692=CIRCLE('',#10482,0.3933);
#3693=CIRCLE('',#10483,0.3933);
#3694=CIRCLE('',#10484,0.3933);
#3695=CIRCLE('',#10485,0.3933);
#3696=CIRCLE('',#10487,0.322275);
#3697=CIRCLE('',#10488,0.322275);
#3698=CIRCLE('',#10499,0.35);
#3699=CIRCLE('',#10502,0.36);
#4301=VERTEX_POINT('',#23894);
#4302=VERTEX_POINT('',#23896);
#4303=VERTEX_POINT('',#23897);
#4304=VERTEX_POINT('',#23899);
#4305=VERTEX_POINT('',#23906);
#4306=VERTEX_POINT('',#23917);
#4307=VERTEX_POINT('',#24051);
#4308=VERTEX_POINT('',#24188);
#4309=VERTEX_POINT('',#24322);
#4310=VERTEX_POINT('',#24456);
#4311=VERTEX_POINT('',#24468);
#4312=VERTEX_POINT('',#24602);
#4313=VERTEX_POINT('',#24613);
#4314=VERTEX_POINT('',#24750);
#4315=VERTEX_POINT('',#24884);
#4316=VERTEX_POINT('',#25018);
#4317=VERTEX_POINT('',#25029);
#4318=VERTEX_POINT('',#25163);
#4319=VERTEX_POINT('',#25174);
#4320=VERTEX_POINT('',#25308);
#4321=VERTEX_POINT('',#25320);
#4322=VERTEX_POINT('',#25451);
#4323=VERTEX_POINT('',#25462);
#4324=VERTEX_POINT('',#25593);
#4325=VERTEX_POINT('',#25606);
#4326=VERTEX_POINT('',#25740);
#4327=VERTEX_POINT('',#25751);
#4328=VERTEX_POINT('',#25885);
#4329=VERTEX_POINT('',#26019);
#4330=VERTEX_POINT('',#26030);
#4331=VERTEX_POINT('',#26164);
#4332=VERTEX_POINT('',#26301);
#4333=VERTEX_POINT('',#26435);
#4334=VERTEX_POINT('',#26446);
#4335=VERTEX_POINT('',#26580);
#4336=VERTEX_POINT('',#26591);
#4337=VERTEX_POINT('',#26725);
#4338=VERTEX_POINT('',#26862);
#4339=VERTEX_POINT('',#26996);
#4340=VERTEX_POINT('',#27007);
#4341=VERTEX_POINT('',#27141);
#4342=VERTEX_POINT('',#27153);
#4343=VERTEX_POINT('',#27287);
#4344=VERTEX_POINT('',#27298);
#4345=VERTEX_POINT('',#27435);
#4346=VERTEX_POINT('',#27566);
#4347=VERTEX_POINT('',#27700);
#4348=VERTEX_POINT('',#27711);
#4349=VERTEX_POINT('',#27845);
#4350=VERTEX_POINT('',#27856);
#4351=VERTEX_POINT('',#27867);
#4352=VERTEX_POINT('',#28001);
#4353=VERTEX_POINT('',#28012);
#4354=VERTEX_POINT('',#28146);
#4355=VERTEX_POINT('',#28277);
#4356=VERTEX_POINT('',#28414);
#4357=VERTEX_POINT('',#28425);
#4358=VERTEX_POINT('',#28559);
#4359=VERTEX_POINT('',#28571);
#4360=VERTEX_POINT('',#28705);
#4361=VERTEX_POINT('',#28716);
#4362=VERTEX_POINT('',#28850);
#4363=VERTEX_POINT('',#28987);
#4364=VERTEX_POINT('',#29121);
#4365=VERTEX_POINT('',#29132);
#4366=VERTEX_POINT('',#29266);
#4367=VERTEX_POINT('',#29277);
#4368=VERTEX_POINT('',#29411);
#4369=VERTEX_POINT('',#29548);
#4370=VERTEX_POINT('',#29682);
#4371=VERTEX_POINT('',#29693);
#4372=VERTEX_POINT('',#29827);
#4373=VERTEX_POINT('',#29961);
#4374=VERTEX_POINT('',#29972);
#4375=VERTEX_POINT('',#30106);
#4376=VERTEX_POINT('',#30118);
#4377=VERTEX_POINT('',#30198);
#4378=VERTEX_POINT('',#30203);
#4379=VERTEX_POINT('',#30205);
#4380=VERTEX_POINT('',#30212);
#4381=VERTEX_POINT('',#30224);
#4382=VERTEX_POINT('',#30235);
#4383=VERTEX_POINT('',#30369);
#4384=VERTEX_POINT('',#30381);
#4385=VERTEX_POINT('',#30515);
#4386=VERTEX_POINT('',#30526);
#4387=VERTEX_POINT('',#30660);
#4388=VERTEX_POINT('',#30797);
#4389=VERTEX_POINT('',#30931);
#4390=VERTEX_POINT('',#30942);
#4391=VERTEX_POINT('',#31076);
#4392=VERTEX_POINT('',#31087);
#4393=VERTEX_POINT('',#31221);
#4394=VERTEX_POINT('',#31358);
#4395=VERTEX_POINT('',#31492);
#4396=VERTEX_POINT('',#31503);
#4397=VERTEX_POINT('',#31637);
#4398=VERTEX_POINT('',#31771);
#4399=VERTEX_POINT('',#31782);
#4400=VERTEX_POINT('',#31916);
#4401=VERTEX_POINT('',#31928);
#4402=VERTEX_POINT('',#32059);
#4403=VERTEX_POINT('',#32070);
#4404=VERTEX_POINT('',#32201);
#4405=VERTEX_POINT('',#32213);
#4406=VERTEX_POINT('',#32347);
#4407=VERTEX_POINT('',#32358);
#4408=VERTEX_POINT('',#32492);
#4409=VERTEX_POINT('',#32503);
#4410=VERTEX_POINT('',#32637);
#4411=VERTEX_POINT('',#32771);
#4412=VERTEX_POINT('',#32908);
#4413=VERTEX_POINT('',#32919);
#4414=VERTEX_POINT('',#33053);
#4415=VERTEX_POINT('',#33065);
#4416=VERTEX_POINT('',#33199);
#4417=VERTEX_POINT('',#33333);
#4418=VERTEX_POINT('',#33470);
#4419=VERTEX_POINT('',#33604);
#4420=VERTEX_POINT('',#33738);
#4421=VERTEX_POINT('',#33872);
#4422=VERTEX_POINT('',#33884);
#4423=VERTEX_POINT('',#34018);
#4424=VERTEX_POINT('',#34029);
#4425=VERTEX_POINT('',#34166);
#4426=VERTEX_POINT('',#34177);
#4427=VERTEX_POINT('',#34311);
#4428=VERTEX_POINT('',#34322);
#4429=VERTEX_POINT('',#34456);
#4430=VERTEX_POINT('',#34590);
#4431=VERTEX_POINT('',#34721);
#4432=VERTEX_POINT('',#34733);
#4433=VERTEX_POINT('',#34864);
#4434=VERTEX_POINT('',#34998);
#4435=VERTEX_POINT('',#35129);
#4436=VERTEX_POINT('',#35142);
#4437=VERTEX_POINT('',#35276);
#4438=VERTEX_POINT('',#35287);
#4439=VERTEX_POINT('',#35299);
#4440=VERTEX_POINT('',#35433);
#4441=VERTEX_POINT('',#35444);
#4442=VERTEX_POINT('',#35578);
#4443=VERTEX_POINT('',#35591);
#4444=VERTEX_POINT('',#35725);
#4445=VERTEX_POINT('',#35736);
#4446=VERTEX_POINT('',#35870);
#4447=VERTEX_POINT('',#35881);
#4448=VERTEX_POINT('',#36015);
#4449=VERTEX_POINT('',#36027);
#4450=VERTEX_POINT('',#36161);
#4451=VERTEX_POINT('',#36172);
#4452=VERTEX_POINT('',#36247);
#4453=VERTEX_POINT('',#36250);
#4454=VERTEX_POINT('',#36251);
#4455=VERTEX_POINT('',#36758);
#4456=VERTEX_POINT('',#36760);
#4457=VERTEX_POINT('',#36861);
#4458=VERTEX_POINT('',#37408);
#4459=VERTEX_POINT('',#37527);
#4460=VERTEX_POINT('',#38058);
#4461=VERTEX_POINT('',#38070);
#4462=VERTEX_POINT('',#38605);
#4463=VERTEX_POINT('',#39160);
#4464=VERTEX_POINT('',#39691);
#4465=VERTEX_POINT('',#40230);
#4466=VERTEX_POINT('',#40769);
#4467=VERTEX_POINT('',#41314);
#4468=VERTEX_POINT('',#41863);
#4469=VERTEX_POINT('',#42414);
#4470=VERTEX_POINT('',#42426);
#4471=VERTEX_POINT('',#42957);
#4472=VERTEX_POINT('',#43482);
#4473=VERTEX_POINT('',#44023);
#4474=VERTEX_POINT('',#44558);
#4475=VERTEX_POINT('',#45075);
#4476=VERTEX_POINT('',#45610);
#4477=VERTEX_POINT('',#46167);
#4478=VERTEX_POINT('',#46722);
#4479=VERTEX_POINT('',#46734);
#4480=VERTEX_POINT('',#47267);
#4481=VERTEX_POINT('',#47800);
#4482=VERTEX_POINT('',#48349);
#4483=VERTEX_POINT('',#48884);
#4484=VERTEX_POINT('',#49433);
#4485=VERTEX_POINT('',#50000);
#4486=VERTEX_POINT('',#50543);
#4487=VERTEX_POINT('',#51080);
#4488=VERTEX_POINT('',#51091);
#4489=VERTEX_POINT('',#51658);
#4490=VERTEX_POINT('',#52195);
#4491=VERTEX_POINT('',#52734);
#4492=VERTEX_POINT('',#53255);
#4493=VERTEX_POINT('',#53802);
#4494=VERTEX_POINT('',#54337);
#4495=VERTEX_POINT('',#54886);
#4496=VERTEX_POINT('',#54906);
#4497=VERTEX_POINT('',#54908);
#4498=VERTEX_POINT('',#55018);
#4499=VERTEX_POINT('',#55559);
#4500=VERTEX_POINT('',#56094);
#4501=VERTEX_POINT('',#56629);
#4502=VERTEX_POINT('',#56640);
#4503=VERTEX_POINT('',#56759);
#4504=VERTEX_POINT('',#57304);
#4505=VERTEX_POINT('',#57875);
#4506=VERTEX_POINT('',#58436);
#4507=VERTEX_POINT('',#58552);
#4508=VERTEX_POINT('',#58671);
#4509=VERTEX_POINT('',#59214);
#4510=VERTEX_POINT('',#59741);
#4511=VERTEX_POINT('',#60284);
#4512=VERTEX_POINT('',#60295);
#4513=VERTEX_POINT('',#60820);
#4514=VERTEX_POINT('',#61349);
#4515=VERTEX_POINT('',#61902);
#4516=VERTEX_POINT('',#61913);
#4517=VERTEX_POINT('',#62464);
#4518=VERTEX_POINT('',#62997);
#4519=VERTEX_POINT('',#63530);
#4520=VERTEX_POINT('',#63649);
#4521=VERTEX_POINT('',#64176);
#4522=VERTEX_POINT('',#64705);
#4523=VERTEX_POINT('',#65254);
#4524=VERTEX_POINT('',#65803);
#4525=VERTEX_POINT('',#65814);
#4526=VERTEX_POINT('',#66351);
#4527=VERTEX_POINT('',#66876);
#4528=VERTEX_POINT('',#67419);
#4529=VERTEX_POINT('',#67950);
#4530=VERTEX_POINT('',#68503);
#4531=VERTEX_POINT('',#69040);
#4532=VERTEX_POINT('',#69567);
#4533=VERTEX_POINT('',#70096);
#4534=VERTEX_POINT('',#70108);
#4535=VERTEX_POINT('',#70667);
#4536=VERTEX_POINT('',#71755);
#4537=VERTEX_POINT('',#71756);
#4538=VERTEX_POINT('',#71758);
#4539=VERTEX_POINT('',#71760);
#4540=VERTEX_POINT('',#71764);
#4541=VERTEX_POINT('',#71766);
#4542=VERTEX_POINT('',#71770);
#4543=VERTEX_POINT('',#71772);
#4544=VERTEX_POINT('',#71776);
#4545=VERTEX_POINT('',#71778);
#4546=VERTEX_POINT('',#71782);
#4547=VERTEX_POINT('',#71784);
#4548=VERTEX_POINT('',#71853);
#4549=VERTEX_POINT('',#75716);
#4550=VERTEX_POINT('',#75721);
#5590=EDGE_CURVE('',#4301,#4301,#3692,.T.);
#5591=EDGE_CURVE('',#4302,#4303,#3693,.T.);
#5592=EDGE_CURVE('',#4303,#4304,#661,.T.);
#5593=EDGE_CURVE('',#4304,#4305,#662,.T.);
#5594=EDGE_CURVE('',#4305,#4306,#663,.T.);
#5595=EDGE_CURVE('',#4306,#4307,#664,.T.);
#5596=EDGE_CURVE('',#4307,#4308,#665,.T.);
#5597=EDGE_CURVE('',#4308,#4309,#666,.T.);
#5598=EDGE_CURVE('',#4309,#4310,#667,.T.);
#5599=EDGE_CURVE('',#4310,#4311,#668,.T.);
#5600=EDGE_CURVE('',#4311,#4312,#669,.T.);
#5601=EDGE_CURVE('',#4312,#4313,#670,.T.);
#5602=EDGE_CURVE('',#4313,#4314,#671,.T.);
#5603=EDGE_CURVE('',#4314,#4315,#672,.T.);
#5604=EDGE_CURVE('',#4315,#4316,#673,.T.);
#5605=EDGE_CURVE('',#4316,#4317,#674,.T.);
#5606=EDGE_CURVE('',#4317,#4318,#675,.T.);
#5607=EDGE_CURVE('',#4318,#4319,#676,.T.);
#5608=EDGE_CURVE('',#4319,#4320,#677,.T.);
#5609=EDGE_CURVE('',#4320,#4321,#678,.T.);
#5610=EDGE_CURVE('',#4321,#4322,#679,.T.);
#5611=EDGE_CURVE('',#4322,#4323,#680,.T.);
#5612=EDGE_CURVE('',#4323,#4324,#681,.T.);
#5613=EDGE_CURVE('',#4324,#4325,#682,.T.);
#5614=EDGE_CURVE('',#4325,#4326,#683,.T.);
#5615=EDGE_CURVE('',#4326,#4327,#684,.T.);
#5616=EDGE_CURVE('',#4327,#4328,#685,.T.);
#5617=EDGE_CURVE('',#4328,#4329,#686,.T.);
#5618=EDGE_CURVE('',#4329,#4330,#687,.T.);
#5619=EDGE_CURVE('',#4330,#4331,#688,.T.);
#5620=EDGE_CURVE('',#4331,#4332,#689,.T.);
#5621=EDGE_CURVE('',#4332,#4333,#690,.T.);
#5622=EDGE_CURVE('',#4333,#4334,#691,.T.);
#5623=EDGE_CURVE('',#4334,#4335,#692,.T.);
#5624=EDGE_CURVE('',#4335,#4336,#693,.T.);
#5625=EDGE_CURVE('',#4336,#4337,#694,.T.);
#5626=EDGE_CURVE('',#4337,#4338,#695,.T.);
#5627=EDGE_CURVE('',#4338,#4339,#696,.T.);
#5628=EDGE_CURVE('',#4339,#4340,#697,.T.);
#5629=EDGE_CURVE('',#4340,#4341,#698,.T.);
#5630=EDGE_CURVE('',#4341,#4342,#699,.T.);
#5631=EDGE_CURVE('',#4342,#4343,#700,.T.);
#5632=EDGE_CURVE('',#4343,#4344,#701,.T.);
#5633=EDGE_CURVE('',#4344,#4345,#702,.T.);
#5634=EDGE_CURVE('',#4345,#4346,#703,.T.);
#5635=EDGE_CURVE('',#4346,#4347,#704,.T.);
#5636=EDGE_CURVE('',#4347,#4348,#705,.T.);
#5637=EDGE_CURVE('',#4348,#4349,#706,.T.);
#5638=EDGE_CURVE('',#4349,#4350,#707,.T.);
#5639=EDGE_CURVE('',#4350,#4351,#708,.T.);
#5640=EDGE_CURVE('',#4351,#4352,#709,.T.);
#5641=EDGE_CURVE('',#4352,#4353,#710,.T.);
#5642=EDGE_CURVE('',#4353,#4354,#711,.T.);
#5643=EDGE_CURVE('',#4354,#4355,#712,.T.);
#5644=EDGE_CURVE('',#4355,#4356,#713,.T.);
#5645=EDGE_CURVE('',#4356,#4357,#714,.T.);
#5646=EDGE_CURVE('',#4357,#4358,#715,.T.);
#5647=EDGE_CURVE('',#4358,#4359,#716,.T.);
#5648=EDGE_CURVE('',#4359,#4360,#717,.T.);
#5649=EDGE_CURVE('',#4360,#4361,#718,.T.);
#5650=EDGE_CURVE('',#4361,#4362,#719,.T.);
#5651=EDGE_CURVE('',#4362,#4363,#720,.T.);
#5652=EDGE_CURVE('',#4363,#4364,#721,.T.);
#5653=EDGE_CURVE('',#4364,#4365,#722,.T.);
#5654=EDGE_CURVE('',#4365,#4366,#723,.T.);
#5655=EDGE_CURVE('',#4366,#4367,#724,.T.);
#5656=EDGE_CURVE('',#4367,#4368,#725,.T.);
#5657=EDGE_CURVE('',#4368,#4369,#726,.T.);
#5658=EDGE_CURVE('',#4369,#4370,#727,.T.);
#5659=EDGE_CURVE('',#4370,#4371,#728,.T.);
#5660=EDGE_CURVE('',#4371,#4372,#729,.T.);
#5661=EDGE_CURVE('',#4372,#4373,#730,.T.);
#5662=EDGE_CURVE('',#4373,#4374,#731,.T.);
#5663=EDGE_CURVE('',#4374,#4375,#732,.T.);
#5664=EDGE_CURVE('',#4375,#4376,#733,.T.);
#5665=EDGE_CURVE('',#4376,#4377,#734,.T.);
#5666=EDGE_CURVE('',#4377,#4378,#3694,.T.);
#5667=EDGE_CURVE('',#4378,#4379,#735,.T.);
#5668=EDGE_CURVE('',#4379,#4380,#736,.T.);
#5669=EDGE_CURVE('',#4380,#4381,#737,.T.);
#5670=EDGE_CURVE('',#4381,#4382,#738,.T.);
#5671=EDGE_CURVE('',#4382,#4383,#739,.T.);
#5672=EDGE_CURVE('',#4383,#4384,#740,.T.);
#5673=EDGE_CURVE('',#4384,#4385,#741,.T.);
#5674=EDGE_CURVE('',#4385,#4386,#742,.T.);
#5675=EDGE_CURVE('',#4386,#4387,#743,.T.);
#5676=EDGE_CURVE('',#4387,#4388,#744,.T.);
#5677=EDGE_CURVE('',#4388,#4389,#745,.T.);
#5678=EDGE_CURVE('',#4389,#4390,#746,.T.);
#5679=EDGE_CURVE('',#4390,#4391,#747,.T.);
#5680=EDGE_CURVE('',#4391,#4392,#748,.T.);
#5681=EDGE_CURVE('',#4392,#4393,#749,.T.);
#5682=EDGE_CURVE('',#4393,#4394,#750,.T.);
#5683=EDGE_CURVE('',#4394,#4395,#751,.T.);
#5684=EDGE_CURVE('',#4395,#4396,#752,.T.);
#5685=EDGE_CURVE('',#4396,#4397,#753,.T.);
#5686=EDGE_CURVE('',#4397,#4398,#754,.T.);
#5687=EDGE_CURVE('',#4398,#4399,#755,.T.);
#5688=EDGE_CURVE('',#4399,#4400,#756,.T.);
#5689=EDGE_CURVE('',#4400,#4401,#757,.T.);
#5690=EDGE_CURVE('',#4401,#4402,#758,.T.);
#5691=EDGE_CURVE('',#4402,#4403,#759,.T.);
#5692=EDGE_CURVE('',#4403,#4404,#760,.T.);
#5693=EDGE_CURVE('',#4404,#4405,#761,.T.);
#5694=EDGE_CURVE('',#4405,#4406,#762,.T.);
#5695=EDGE_CURVE('',#4406,#4407,#763,.T.);
#5696=EDGE_CURVE('',#4407,#4408,#764,.T.);
#5697=EDGE_CURVE('',#4408,#4409,#765,.T.);
#5698=EDGE_CURVE('',#4409,#4410,#766,.T.);
#5699=EDGE_CURVE('',#4410,#4411,#767,.T.);
#5700=EDGE_CURVE('',#4411,#4412,#768,.T.);
#5701=EDGE_CURVE('',#4412,#4413,#769,.T.);
#5702=EDGE_CURVE('',#4413,#4414,#770,.T.);
#5703=EDGE_CURVE('',#4414,#4415,#771,.T.);
#5704=EDGE_CURVE('',#4415,#4416,#772,.T.);
#5705=EDGE_CURVE('',#4416,#4417,#773,.T.);
#5706=EDGE_CURVE('',#4417,#4418,#774,.T.);
#5707=EDGE_CURVE('',#4418,#4419,#775,.T.);
#5708=EDGE_CURVE('',#4419,#4420,#776,.T.);
#5709=EDGE_CURVE('',#4420,#4421,#777,.T.);
#5710=EDGE_CURVE('',#4421,#4422,#778,.T.);
#5711=EDGE_CURVE('',#4422,#4423,#779,.T.);
#5712=EDGE_CURVE('',#4423,#4424,#780,.T.);
#5713=EDGE_CURVE('',#4424,#4425,#781,.T.);
#5714=EDGE_CURVE('',#4425,#4426,#782,.T.);
#5715=EDGE_CURVE('',#4426,#4427,#783,.T.);
#5716=EDGE_CURVE('',#4427,#4428,#784,.T.);
#5717=EDGE_CURVE('',#4428,#4429,#785,.T.);
#5718=EDGE_CURVE('',#4429,#4430,#786,.T.);
#5719=EDGE_CURVE('',#4430,#4431,#787,.T.);
#5720=EDGE_CURVE('',#4431,#4432,#788,.T.);
#5721=EDGE_CURVE('',#4432,#4433,#789,.T.);
#5722=EDGE_CURVE('',#4433,#4434,#790,.T.);
#5723=EDGE_CURVE('',#4434,#4435,#791,.T.);
#5724=EDGE_CURVE('',#4435,#4436,#792,.T.);
#5725=EDGE_CURVE('',#4436,#4437,#793,.T.);
#5726=EDGE_CURVE('',#4437,#4438,#794,.T.);
#5727=EDGE_CURVE('',#4438,#4439,#795,.T.);
#5728=EDGE_CURVE('',#4439,#4440,#796,.T.);
#5729=EDGE_CURVE('',#4440,#4441,#797,.T.);
#5730=EDGE_CURVE('',#4441,#4442,#798,.T.);
#5731=EDGE_CURVE('',#4442,#4443,#799,.T.);
#5732=EDGE_CURVE('',#4443,#4444,#800,.T.);
#5733=EDGE_CURVE('',#4444,#4445,#801,.T.);
#5734=EDGE_CURVE('',#4445,#4446,#802,.T.);
#5735=EDGE_CURVE('',#4446,#4447,#803,.T.);
#5736=EDGE_CURVE('',#4447,#4448,#804,.T.);
#5737=EDGE_CURVE('',#4448,#4449,#805,.T.);
#5738=EDGE_CURVE('',#4449,#4450,#806,.T.);
#5739=EDGE_CURVE('',#4450,#4451,#807,.T.);
#5740=EDGE_CURVE('',#4451,#4302,#808,.T.);
#5741=EDGE_CURVE('',#4452,#4452,#3695,.F.);
#5742=EDGE_CURVE('',#4453,#4454,#809,.T.);
#5743=EDGE_CURVE('',#4455,#4454,#3696,.T.);
#5744=EDGE_CURVE('',#4456,#4455,#810,.T.);
#5745=EDGE_CURVE('',#4457,#4456,#811,.F.);
#5746=EDGE_CURVE('',#4458,#4457,#812,.T.);
#5747=EDGE_CURVE('',#4459,#4458,#813,.F.);
#5748=EDGE_CURVE('',#4460,#4459,#814,.T.);
#5749=EDGE_CURVE('',#4461,#4460,#815,.F.);
#5750=EDGE_CURVE('',#4462,#4461,#816,.F.);
#5751=EDGE_CURVE('',#4463,#4462,#817,.F.);
#5752=EDGE_CURVE('',#4464,#4463,#818,.F.);
#5753=EDGE_CURVE('',#4465,#4464,#819,.F.);
#5754=EDGE_CURVE('',#4466,#4465,#820,.F.);
#5755=EDGE_CURVE('',#4467,#4466,#821,.F.);
#5756=EDGE_CURVE('',#4468,#4467,#822,.F.);
#5757=EDGE_CURVE('',#4469,#4468,#823,.T.);
#5758=EDGE_CURVE('',#4470,#4469,#824,.F.);
#5759=EDGE_CURVE('',#4471,#4470,#825,.F.);
#5760=EDGE_CURVE('',#4472,#4471,#826,.F.);
#5761=EDGE_CURVE('',#4473,#4472,#827,.F.);
#5762=EDGE_CURVE('',#4474,#4473,#828,.F.);
#5763=EDGE_CURVE('',#4475,#4474,#829,.F.);
#5764=EDGE_CURVE('',#4476,#4475,#830,.F.);
#5765=EDGE_CURVE('',#4477,#4476,#831,.F.);
#5766=EDGE_CURVE('',#4478,#4477,#832,.T.);
#5767=EDGE_CURVE('',#4479,#4478,#833,.F.);
#5768=EDGE_CURVE('',#4480,#4479,#834,.F.);
#5769=EDGE_CURVE('',#4481,#4480,#835,.F.);
#5770=EDGE_CURVE('',#4482,#4481,#836,.F.);
#5771=EDGE_CURVE('',#4483,#4482,#837,.F.);
#5772=EDGE_CURVE('',#4484,#4483,#838,.F.);
#5773=EDGE_CURVE('',#4485,#4484,#839,.F.);
#5774=EDGE_CURVE('',#4486,#4485,#840,.F.);
#5775=EDGE_CURVE('',#4487,#4486,#841,.T.);
#5776=EDGE_CURVE('',#4488,#4487,#842,.F.);
#5777=EDGE_CURVE('',#4489,#4488,#843,.F.);
#5778=EDGE_CURVE('',#4490,#4489,#844,.F.);
#5779=EDGE_CURVE('',#4491,#4490,#845,.F.);
#5780=EDGE_CURVE('',#4492,#4491,#846,.F.);
#5781=EDGE_CURVE('',#4493,#4492,#847,.F.);
#5782=EDGE_CURVE('',#4494,#4493,#848,.F.);
#5783=EDGE_CURVE('',#4495,#4494,#849,.T.);
#5784=EDGE_CURVE('',#4496,#4495,#3697,.T.);
#5785=EDGE_CURVE('',#4496,#4497,#850,.T.);
#5786=EDGE_CURVE('',#4497,#4498,#851,.T.);
#5787=EDGE_CURVE('',#4498,#4499,#852,.T.);
#5788=EDGE_CURVE('',#4499,#4500,#853,.T.);
#5789=EDGE_CURVE('',#4500,#4501,#854,.T.);
#5790=EDGE_CURVE('',#4501,#4502,#855,.T.);
#5791=EDGE_CURVE('',#4502,#4503,#856,.T.);
#5792=EDGE_CURVE('',#4503,#4504,#857,.T.);
#5793=EDGE_CURVE('',#4504,#4505,#858,.T.);
#5794=EDGE_CURVE('',#4505,#4506,#859,.T.);
#5795=EDGE_CURVE('',#4506,#4507,#860,.T.);
#5796=EDGE_CURVE('',#4507,#4508,#861,.T.);
#5797=EDGE_CURVE('',#4508,#4509,#862,.T.);
#5798=EDGE_CURVE('',#4509,#4510,#863,.T.);
#5799=EDGE_CURVE('',#4510,#4511,#864,.T.);
#5800=EDGE_CURVE('',#4511,#4512,#865,.T.);
#5801=EDGE_CURVE('',#4512,#4513,#866,.T.);
#5802=EDGE_CURVE('',#4513,#4514,#867,.T.);
#5803=EDGE_CURVE('',#4514,#4515,#868,.T.);
#5804=EDGE_CURVE('',#4515,#4516,#869,.T.);
#5805=EDGE_CURVE('',#4516,#4517,#870,.T.);
#5806=EDGE_CURVE('',#4517,#4518,#871,.T.);
#5807=EDGE_CURVE('',#4518,#4519,#872,.T.);
#5808=EDGE_CURVE('',#4519,#4520,#873,.T.);
#5809=EDGE_CURVE('',#4520,#4521,#874,.T.);
#5810=EDGE_CURVE('',#4521,#4522,#875,.T.);
#5811=EDGE_CURVE('',#4522,#4523,#876,.T.);
#5812=EDGE_CURVE('',#4523,#4524,#877,.T.);
#5813=EDGE_CURVE('',#4524,#4525,#878,.T.);
#5814=EDGE_CURVE('',#4525,#4526,#879,.T.);
#5815=EDGE_CURVE('',#4526,#4527,#880,.T.);
#5816=EDGE_CURVE('',#4527,#4528,#881,.T.);
#5817=EDGE_CURVE('',#4528,#4529,#882,.T.);
#5818=EDGE_CURVE('',#4529,#4530,#883,.T.);
#5819=EDGE_CURVE('',#4530,#4531,#884,.T.);
#5820=EDGE_CURVE('',#4531,#4532,#885,.T.);
#5821=EDGE_CURVE('',#4532,#4533,#886,.T.);
#5822=EDGE_CURVE('',#4533,#4534,#887,.T.);
#5823=EDGE_CURVE('',#4534,#4535,#888,.T.);
#5824=EDGE_CURVE('',#4535,#4453,#889,.T.);
#5825=EDGE_CURVE('',#4536,#4537,#1469,.T.);
#5826=EDGE_CURVE('',#4536,#4538,#1470,.T.);
#5827=EDGE_CURVE('',#4538,#4539,#1471,.T.);
#5828=EDGE_CURVE('',#4537,#4539,#1472,.T.);
#5829=EDGE_CURVE('',#4540,#4536,#1473,.T.);
#5830=EDGE_CURVE('',#4540,#4541,#1474,.T.);
#5831=EDGE_CURVE('',#4541,#4538,#1475,.T.);
#5832=EDGE_CURVE('',#4542,#4540,#1476,.T.);
#5833=EDGE_CURVE('',#4542,#4543,#1477,.T.);
#5834=EDGE_CURVE('',#4543,#4541,#1478,.T.);
#5835=EDGE_CURVE('',#4544,#4542,#1479,.T.);
#5836=EDGE_CURVE('',#4544,#4545,#1480,.T.);
#5837=EDGE_CURVE('',#4545,#4543,#1481,.T.);
#5838=EDGE_CURVE('',#4546,#4544,#1482,.T.);
#5839=EDGE_CURVE('',#4546,#4547,#1483,.T.);
#5840=EDGE_CURVE('',#4547,#4545,#1484,.T.);
#5841=EDGE_CURVE('',#4537,#4546,#1485,.T.);
#5842=EDGE_CURVE('',#4539,#4547,#1486,.T.);
#5843=EDGE_CURVE('',#4302,#4455,#890,.T.);
#5844=EDGE_CURVE('',#4454,#4548,#891,.T.);
#5845=EDGE_CURVE('',#4548,#4303,#892,.T.);
#5846=EDGE_CURVE('',#4495,#4378,#893,.T.);
#5847=EDGE_CURVE('',#4377,#4496,#894,.T.);
#5848=EDGE_CURVE('',#4549,#4549,#3698,.T.);
#5849=EDGE_CURVE('',#4301,#4549,#1487,.T.);
#5850=EDGE_CURVE('',#4452,#4550,#1488,.T.);
#5851=EDGE_CURVE('',#4550,#4550,#3699,.T.);
#7725=ORIENTED_EDGE('',*,*,#5590,.T.);
#7726=ORIENTED_EDGE('',*,*,#5591,.T.);
#7727=ORIENTED_EDGE('',*,*,#5592,.T.);
#7728=ORIENTED_EDGE('',*,*,#5593,.T.);
#7729=ORIENTED_EDGE('',*,*,#5594,.T.);
#7730=ORIENTED_EDGE('',*,*,#5595,.T.);
#7731=ORIENTED_EDGE('',*,*,#5596,.T.);
#7732=ORIENTED_EDGE('',*,*,#5597,.T.);
#7733=ORIENTED_EDGE('',*,*,#5598,.T.);
#7734=ORIENTED_EDGE('',*,*,#5599,.T.);
#7735=ORIENTED_EDGE('',*,*,#5600,.T.);
#7736=ORIENTED_EDGE('',*,*,#5601,.T.);
#7737=ORIENTED_EDGE('',*,*,#5602,.T.);
#7738=ORIENTED_EDGE('',*,*,#5603,.T.);
#7739=ORIENTED_EDGE('',*,*,#5604,.T.);
#7740=ORIENTED_EDGE('',*,*,#5605,.T.);
#7741=ORIENTED_EDGE('',*,*,#5606,.T.);
#7742=ORIENTED_EDGE('',*,*,#5607,.T.);
#7743=ORIENTED_EDGE('',*,*,#5608,.T.);
#7744=ORIENTED_EDGE('',*,*,#5609,.T.);
#7745=ORIENTED_EDGE('',*,*,#5610,.T.);
#7746=ORIENTED_EDGE('',*,*,#5611,.T.);
#7747=ORIENTED_EDGE('',*,*,#5612,.T.);
#7748=ORIENTED_EDGE('',*,*,#5613,.T.);
#7749=ORIENTED_EDGE('',*,*,#5614,.T.);
#7750=ORIENTED_EDGE('',*,*,#5615,.T.);
#7751=ORIENTED_EDGE('',*,*,#5616,.T.);
#7752=ORIENTED_EDGE('',*,*,#5617,.T.);
#7753=ORIENTED_EDGE('',*,*,#5618,.T.);
#7754=ORIENTED_EDGE('',*,*,#5619,.T.);
#7755=ORIENTED_EDGE('',*,*,#5620,.T.);
#7756=ORIENTED_EDGE('',*,*,#5621,.T.);
#7757=ORIENTED_EDGE('',*,*,#5622,.T.);
#7758=ORIENTED_EDGE('',*,*,#5623,.T.);
#7759=ORIENTED_EDGE('',*,*,#5624,.T.);
#7760=ORIENTED_EDGE('',*,*,#5625,.T.);
#7761=ORIENTED_EDGE('',*,*,#5626,.T.);
#7762=ORIENTED_EDGE('',*,*,#5627,.T.);
#7763=ORIENTED_EDGE('',*,*,#5628,.T.);
#7764=ORIENTED_EDGE('',*,*,#5629,.T.);
#7765=ORIENTED_EDGE('',*,*,#5630,.T.);
#7766=ORIENTED_EDGE('',*,*,#5631,.T.);
#7767=ORIENTED_EDGE('',*,*,#5632,.T.);
#7768=ORIENTED_EDGE('',*,*,#5633,.T.);
#7769=ORIENTED_EDGE('',*,*,#5634,.T.);
#7770=ORIENTED_EDGE('',*,*,#5635,.T.);
#7771=ORIENTED_EDGE('',*,*,#5636,.T.);
#7772=ORIENTED_EDGE('',*,*,#5637,.T.);
#7773=ORIENTED_EDGE('',*,*,#5638,.T.);
#7774=ORIENTED_EDGE('',*,*,#5639,.T.);
#7775=ORIENTED_EDGE('',*,*,#5640,.T.);
#7776=ORIENTED_EDGE('',*,*,#5641,.T.);
#7777=ORIENTED_EDGE('',*,*,#5642,.T.);
#7778=ORIENTED_EDGE('',*,*,#5643,.T.);
#7779=ORIENTED_EDGE('',*,*,#5644,.T.);
#7780=ORIENTED_EDGE('',*,*,#5645,.T.);
#7781=ORIENTED_EDGE('',*,*,#5646,.T.);
#7782=ORIENTED_EDGE('',*,*,#5647,.T.);
#7783=ORIENTED_EDGE('',*,*,#5648,.T.);
#7784=ORIENTED_EDGE('',*,*,#5649,.T.);
#7785=ORIENTED_EDGE('',*,*,#5650,.T.);
#7786=ORIENTED_EDGE('',*,*,#5651,.T.);
#7787=ORIENTED_EDGE('',*,*,#5652,.T.);
#7788=ORIENTED_EDGE('',*,*,#5653,.T.);
#7789=ORIENTED_EDGE('',*,*,#5654,.T.);
#7790=ORIENTED_EDGE('',*,*,#5655,.T.);
#7791=ORIENTED_EDGE('',*,*,#5656,.T.);
#7792=ORIENTED_EDGE('',*,*,#5657,.T.);
#7793=ORIENTED_EDGE('',*,*,#5658,.T.);
#7794=ORIENTED_EDGE('',*,*,#5659,.T.);
#7795=ORIENTED_EDGE('',*,*,#5660,.T.);
#7796=ORIENTED_EDGE('',*,*,#5661,.T.);
#7797=ORIENTED_EDGE('',*,*,#5662,.T.);
#7798=ORIENTED_EDGE('',*,*,#5663,.T.);
#7799=ORIENTED_EDGE('',*,*,#5664,.T.);
#7800=ORIENTED_EDGE('',*,*,#5665,.T.);
#7801=ORIENTED_EDGE('',*,*,#5666,.T.);
#7802=ORIENTED_EDGE('',*,*,#5667,.T.);
#7803=ORIENTED_EDGE('',*,*,#5668,.T.);
#7804=ORIENTED_EDGE('',*,*,#5669,.T.);
#7805=ORIENTED_EDGE('',*,*,#5670,.T.);
#7806=ORIENTED_EDGE('',*,*,#5671,.T.);
#7807=ORIENTED_EDGE('',*,*,#5672,.T.);
#7808=ORIENTED_EDGE('',*,*,#5673,.T.);
#7809=ORIENTED_EDGE('',*,*,#5674,.T.);
#7810=ORIENTED_EDGE('',*,*,#5675,.T.);
#7811=ORIENTED_EDGE('',*,*,#5676,.T.);
#7812=ORIENTED_EDGE('',*,*,#5677,.T.);
#7813=ORIENTED_EDGE('',*,*,#5678,.T.);
#7814=ORIENTED_EDGE('',*,*,#5679,.T.);
#7815=ORIENTED_EDGE('',*,*,#5680,.T.);
#7816=ORIENTED_EDGE('',*,*,#5681,.T.);
#7817=ORIENTED_EDGE('',*,*,#5682,.T.);
#7818=ORIENTED_EDGE('',*,*,#5683,.T.);
#7819=ORIENTED_EDGE('',*,*,#5684,.T.);
#7820=ORIENTED_EDGE('',*,*,#5685,.T.);
#7821=ORIENTED_EDGE('',*,*,#5686,.T.);
#7822=ORIENTED_EDGE('',*,*,#5687,.T.);
#7823=ORIENTED_EDGE('',*,*,#5688,.T.);
#7824=ORIENTED_EDGE('',*,*,#5689,.T.);
#7825=ORIENTED_EDGE('',*,*,#5690,.T.);
#7826=ORIENTED_EDGE('',*,*,#5691,.T.);
#7827=ORIENTED_EDGE('',*,*,#5692,.T.);
#7828=ORIENTED_EDGE('',*,*,#5693,.T.);
#7829=ORIENTED_EDGE('',*,*,#5694,.T.);
#7830=ORIENTED_EDGE('',*,*,#5695,.T.);
#7831=ORIENTED_EDGE('',*,*,#5696,.T.);
#7832=ORIENTED_EDGE('',*,*,#5697,.T.);
#7833=ORIENTED_EDGE('',*,*,#5698,.T.);
#7834=ORIENTED_EDGE('',*,*,#5699,.T.);
#7835=ORIENTED_EDGE('',*,*,#5700,.T.);
#7836=ORIENTED_EDGE('',*,*,#5701,.T.);
#7837=ORIENTED_EDGE('',*,*,#5702,.T.);
#7838=ORIENTED_EDGE('',*,*,#5703,.T.);
#7839=ORIENTED_EDGE('',*,*,#5704,.T.);
#7840=ORIENTED_EDGE('',*,*,#5705,.T.);
#7841=ORIENTED_EDGE('',*,*,#5706,.T.);
#7842=ORIENTED_EDGE('',*,*,#5707,.T.);
#7843=ORIENTED_EDGE('',*,*,#5708,.T.);
#7844=ORIENTED_EDGE('',*,*,#5709,.T.);
#7845=ORIENTED_EDGE('',*,*,#5710,.T.);
#7846=ORIENTED_EDGE('',*,*,#5711,.T.);
#7847=ORIENTED_EDGE('',*,*,#5712,.T.);
#7848=ORIENTED_EDGE('',*,*,#5713,.T.);
#7849=ORIENTED_EDGE('',*,*,#5714,.T.);
#7850=ORIENTED_EDGE('',*,*,#5715,.T.);
#7851=ORIENTED_EDGE('',*,*,#5716,.T.);
#7852=ORIENTED_EDGE('',*,*,#5717,.T.);
#7853=ORIENTED_EDGE('',*,*,#5718,.T.);
#7854=ORIENTED_EDGE('',*,*,#5719,.T.);
#7855=ORIENTED_EDGE('',*,*,#5720,.T.);
#7856=ORIENTED_EDGE('',*,*,#5721,.T.);
#7857=ORIENTED_EDGE('',*,*,#5722,.T.);
#7858=ORIENTED_EDGE('',*,*,#5723,.T.);
#7859=ORIENTED_EDGE('',*,*,#5724,.T.);
#7860=ORIENTED_EDGE('',*,*,#5725,.T.);
#7861=ORIENTED_EDGE('',*,*,#5726,.T.);
#7862=ORIENTED_EDGE('',*,*,#5727,.T.);
#7863=ORIENTED_EDGE('',*,*,#5728,.T.);
#7864=ORIENTED_EDGE('',*,*,#5729,.T.);
#7865=ORIENTED_EDGE('',*,*,#5730,.T.);
#7866=ORIENTED_EDGE('',*,*,#5731,.T.);
#7867=ORIENTED_EDGE('',*,*,#5732,.T.);
#7868=ORIENTED_EDGE('',*,*,#5733,.T.);
#7869=ORIENTED_EDGE('',*,*,#5734,.T.);
#7870=ORIENTED_EDGE('',*,*,#5735,.T.);
#7871=ORIENTED_EDGE('',*,*,#5736,.T.);
#7872=ORIENTED_EDGE('',*,*,#5737,.T.);
#7873=ORIENTED_EDGE('',*,*,#5738,.T.);
#7874=ORIENTED_EDGE('',*,*,#5739,.T.);
#7875=ORIENTED_EDGE('',*,*,#5740,.T.);
#7876=ORIENTED_EDGE('',*,*,#5741,.F.);
#7877=ORIENTED_EDGE('',*,*,#5742,.T.);
#7878=ORIENTED_EDGE('',*,*,#5743,.F.);
#7879=ORIENTED_EDGE('',*,*,#5744,.F.);
#7880=ORIENTED_EDGE('',*,*,#5745,.F.);
#7881=ORIENTED_EDGE('',*,*,#5746,.F.);
#7882=ORIENTED_EDGE('',*,*,#5747,.F.);
#7883=ORIENTED_EDGE('',*,*,#5748,.F.);
#7884=ORIENTED_EDGE('',*,*,#5749,.F.);
#7885=ORIENTED_EDGE('',*,*,#5750,.F.);
#7886=ORIENTED_EDGE('',*,*,#5751,.F.);
#7887=ORIENTED_EDGE('',*,*,#5752,.F.);
#7888=ORIENTED_EDGE('',*,*,#5753,.F.);
#7889=ORIENTED_EDGE('',*,*,#5754,.F.);
#7890=ORIENTED_EDGE('',*,*,#5755,.F.);
#7891=ORIENTED_EDGE('',*,*,#5756,.F.);
#7892=ORIENTED_EDGE('',*,*,#5757,.F.);
#7893=ORIENTED_EDGE('',*,*,#5758,.F.);
#7894=ORIENTED_EDGE('',*,*,#5759,.F.);
#7895=ORIENTED_EDGE('',*,*,#5760,.F.);
#7896=ORIENTED_EDGE('',*,*,#5761,.F.);
#7897=ORIENTED_EDGE('',*,*,#5762,.F.);
#7898=ORIENTED_EDGE('',*,*,#5763,.F.);
#7899=ORIENTED_EDGE('',*,*,#5764,.F.);
#7900=ORIENTED_EDGE('',*,*,#5765,.F.);
#7901=ORIENTED_EDGE('',*,*,#5766,.F.);
#7902=ORIENTED_EDGE('',*,*,#5767,.F.);
#7903=ORIENTED_EDGE('',*,*,#5768,.F.);
#7904=ORIENTED_EDGE('',*,*,#5769,.F.);
#7905=ORIENTED_EDGE('',*,*,#5770,.F.);
#7906=ORIENTED_EDGE('',*,*,#5771,.F.);
#7907=ORIENTED_EDGE('',*,*,#5772,.F.);
#7908=ORIENTED_EDGE('',*,*,#5773,.F.);
#7909=ORIENTED_EDGE('',*,*,#5774,.F.);
#7910=ORIENTED_EDGE('',*,*,#5775,.F.);
#7911=ORIENTED_EDGE('',*,*,#5776,.F.);
#7912=ORIENTED_EDGE('',*,*,#5777,.F.);
#7913=ORIENTED_EDGE('',*,*,#5778,.F.);
#7914=ORIENTED_EDGE('',*,*,#5779,.F.);
#7915=ORIENTED_EDGE('',*,*,#5780,.F.);
#7916=ORIENTED_EDGE('',*,*,#5781,.F.);
#7917=ORIENTED_EDGE('',*,*,#5782,.F.);
#7918=ORIENTED_EDGE('',*,*,#5783,.F.);
#7919=ORIENTED_EDGE('',*,*,#5784,.F.);
#7920=ORIENTED_EDGE('',*,*,#5785,.T.);
#7921=ORIENTED_EDGE('',*,*,#5786,.T.);
#7922=ORIENTED_EDGE('',*,*,#5787,.T.);
#7923=ORIENTED_EDGE('',*,*,#5788,.T.);
#7924=ORIENTED_EDGE('',*,*,#5789,.T.);
#7925=ORIENTED_EDGE('',*,*,#5790,.T.);
#7926=ORIENTED_EDGE('',*,*,#5791,.T.);
#7927=ORIENTED_EDGE('',*,*,#5792,.T.);
#7928=ORIENTED_EDGE('',*,*,#5793,.T.);
#7929=ORIENTED_EDGE('',*,*,#5794,.T.);
#7930=ORIENTED_EDGE('',*,*,#5795,.T.);
#7931=ORIENTED_EDGE('',*,*,#5796,.T.);
#7932=ORIENTED_EDGE('',*,*,#5797,.T.);
#7933=ORIENTED_EDGE('',*,*,#5798,.T.);
#7934=ORIENTED_EDGE('',*,*,#5799,.T.);
#7935=ORIENTED_EDGE('',*,*,#5800,.T.);
#7936=ORIENTED_EDGE('',*,*,#5801,.T.);
#7937=ORIENTED_EDGE('',*,*,#5802,.T.);
#7938=ORIENTED_EDGE('',*,*,#5803,.T.);
#7939=ORIENTED_EDGE('',*,*,#5804,.T.);
#7940=ORIENTED_EDGE('',*,*,#5805,.T.);
#7941=ORIENTED_EDGE('',*,*,#5806,.T.);
#7942=ORIENTED_EDGE('',*,*,#5807,.T.);
#7943=ORIENTED_EDGE('',*,*,#5808,.T.);
#7944=ORIENTED_EDGE('',*,*,#5809,.T.);
#7945=ORIENTED_EDGE('',*,*,#5810,.T.);
#7946=ORIENTED_EDGE('',*,*,#5811,.T.);
#7947=ORIENTED_EDGE('',*,*,#5812,.T.);
#7948=ORIENTED_EDGE('',*,*,#5813,.T.);
#7949=ORIENTED_EDGE('',*,*,#5814,.T.);
#7950=ORIENTED_EDGE('',*,*,#5815,.T.);
#7951=ORIENTED_EDGE('',*,*,#5816,.T.);
#7952=ORIENTED_EDGE('',*,*,#5817,.T.);
#7953=ORIENTED_EDGE('',*,*,#5818,.T.);
#7954=ORIENTED_EDGE('',*,*,#5819,.T.);
#7955=ORIENTED_EDGE('',*,*,#5820,.T.);
#7956=ORIENTED_EDGE('',*,*,#5821,.T.);
#7957=ORIENTED_EDGE('',*,*,#5822,.T.);
#7958=ORIENTED_EDGE('',*,*,#5823,.T.);
#7959=ORIENTED_EDGE('',*,*,#5824,.T.);
#7960=ORIENTED_EDGE('',*,*,#5825,.F.);
#7961=ORIENTED_EDGE('',*,*,#5826,.T.);
#7962=ORIENTED_EDGE('',*,*,#5827,.T.);
#7963=ORIENTED_EDGE('',*,*,#5828,.F.);
#7964=ORIENTED_EDGE('',*,*,#5829,.F.);
#7965=ORIENTED_EDGE('',*,*,#5830,.T.);
#7966=ORIENTED_EDGE('',*,*,#5831,.T.);
#7967=ORIENTED_EDGE('',*,*,#5826,.F.);
#7968=ORIENTED_EDGE('',*,*,#5832,.F.);
#7969=ORIENTED_EDGE('',*,*,#5833,.T.);
#7970=ORIENTED_EDGE('',*,*,#5834,.T.);
#7971=ORIENTED_EDGE('',*,*,#5830,.F.);
#7972=ORIENTED_EDGE('',*,*,#5835,.F.);
#7973=ORIENTED_EDGE('',*,*,#5836,.T.);
#7974=ORIENTED_EDGE('',*,*,#5837,.T.);
#7975=ORIENTED_EDGE('',*,*,#5833,.F.);
#7976=ORIENTED_EDGE('',*,*,#5838,.F.);
#7977=ORIENTED_EDGE('',*,*,#5839,.T.);
#7978=ORIENTED_EDGE('',*,*,#5840,.T.);
#7979=ORIENTED_EDGE('',*,*,#5836,.F.);
#7980=ORIENTED_EDGE('',*,*,#5841,.F.);
#7981=ORIENTED_EDGE('',*,*,#5828,.T.);
#7982=ORIENTED_EDGE('',*,*,#5842,.T.);
#7983=ORIENTED_EDGE('',*,*,#5839,.F.);
#7984=ORIENTED_EDGE('',*,*,#5842,.F.);
#7985=ORIENTED_EDGE('',*,*,#5827,.F.);
#7986=ORIENTED_EDGE('',*,*,#5831,.F.);
#7987=ORIENTED_EDGE('',*,*,#5834,.F.);
#7988=ORIENTED_EDGE('',*,*,#5837,.F.);
#7989=ORIENTED_EDGE('',*,*,#5840,.F.);
#7990=ORIENTED_EDGE('',*,*,#5591,.F.);
#7991=ORIENTED_EDGE('',*,*,#5843,.T.);
#7992=ORIENTED_EDGE('',*,*,#5743,.T.);
#7993=ORIENTED_EDGE('',*,*,#5844,.T.);
#7994=ORIENTED_EDGE('',*,*,#5845,.T.);
#7995=ORIENTED_EDGE('',*,*,#5843,.F.);
#7996=ORIENTED_EDGE('',*,*,#5740,.F.);
#7997=ORIENTED_EDGE('',*,*,#5739,.F.);
#7998=ORIENTED_EDGE('',*,*,#5738,.F.);
#7999=ORIENTED_EDGE('',*,*,#5737,.F.);
#8000=ORIENTED_EDGE('',*,*,#5736,.F.);
#8001=ORIENTED_EDGE('',*,*,#5735,.F.);
#8002=ORIENTED_EDGE('',*,*,#5734,.F.);
#8003=ORIENTED_EDGE('',*,*,#5733,.F.);
#8004=ORIENTED_EDGE('',*,*,#5732,.F.);
#8005=ORIENTED_EDGE('',*,*,#5731,.F.);
#8006=ORIENTED_EDGE('',*,*,#5730,.F.);
#8007=ORIENTED_EDGE('',*,*,#5729,.F.);
#8008=ORIENTED_EDGE('',*,*,#5728,.F.);
#8009=ORIENTED_EDGE('',*,*,#5727,.F.);
#8010=ORIENTED_EDGE('',*,*,#5726,.F.);
#8011=ORIENTED_EDGE('',*,*,#5725,.F.);
#8012=ORIENTED_EDGE('',*,*,#5724,.F.);
#8013=ORIENTED_EDGE('',*,*,#5723,.F.);
#8014=ORIENTED_EDGE('',*,*,#5722,.F.);
#8015=ORIENTED_EDGE('',*,*,#5721,.F.);
#8016=ORIENTED_EDGE('',*,*,#5720,.F.);
#8017=ORIENTED_EDGE('',*,*,#5719,.F.);
#8018=ORIENTED_EDGE('',*,*,#5718,.F.);
#8019=ORIENTED_EDGE('',*,*,#5717,.F.);
#8020=ORIENTED_EDGE('',*,*,#5716,.F.);
#8021=ORIENTED_EDGE('',*,*,#5715,.F.);
#8022=ORIENTED_EDGE('',*,*,#5714,.F.);
#8023=ORIENTED_EDGE('',*,*,#5713,.F.);
#8024=ORIENTED_EDGE('',*,*,#5712,.F.);
#8025=ORIENTED_EDGE('',*,*,#5711,.F.);
#8026=ORIENTED_EDGE('',*,*,#5710,.F.);
#8027=ORIENTED_EDGE('',*,*,#5709,.F.);
#8028=ORIENTED_EDGE('',*,*,#5708,.F.);
#8029=ORIENTED_EDGE('',*,*,#5707,.F.);
#8030=ORIENTED_EDGE('',*,*,#5706,.F.);
#8031=ORIENTED_EDGE('',*,*,#5705,.F.);
#8032=ORIENTED_EDGE('',*,*,#5704,.F.);
#8033=ORIENTED_EDGE('',*,*,#5703,.F.);
#8034=ORIENTED_EDGE('',*,*,#5702,.F.);
#8035=ORIENTED_EDGE('',*,*,#5701,.F.);
#8036=ORIENTED_EDGE('',*,*,#5700,.F.);
#8037=ORIENTED_EDGE('',*,*,#5699,.F.);
#8038=ORIENTED_EDGE('',*,*,#5698,.F.);
#8039=ORIENTED_EDGE('',*,*,#5697,.F.);
#8040=ORIENTED_EDGE('',*,*,#5696,.F.);
#8041=ORIENTED_EDGE('',*,*,#5695,.F.);
#8042=ORIENTED_EDGE('',*,*,#5694,.F.);
#8043=ORIENTED_EDGE('',*,*,#5693,.F.);
#8044=ORIENTED_EDGE('',*,*,#5692,.F.);
#8045=ORIENTED_EDGE('',*,*,#5691,.F.);
#8046=ORIENTED_EDGE('',*,*,#5690,.F.);
#8047=ORIENTED_EDGE('',*,*,#5689,.F.);
#8048=ORIENTED_EDGE('',*,*,#5688,.F.);
#8049=ORIENTED_EDGE('',*,*,#5687,.F.);
#8050=ORIENTED_EDGE('',*,*,#5686,.F.);
#8051=ORIENTED_EDGE('',*,*,#5685,.F.);
#8052=ORIENTED_EDGE('',*,*,#5684,.F.);
#8053=ORIENTED_EDGE('',*,*,#5683,.F.);
#8054=ORIENTED_EDGE('',*,*,#5682,.F.);
#8055=ORIENTED_EDGE('',*,*,#5681,.F.);
#8056=ORIENTED_EDGE('',*,*,#5680,.F.);
#8057=ORIENTED_EDGE('',*,*,#5679,.F.);
#8058=ORIENTED_EDGE('',*,*,#5678,.F.);
#8059=ORIENTED_EDGE('',*,*,#5677,.F.);
#8060=ORIENTED_EDGE('',*,*,#5676,.F.);
#8061=ORIENTED_EDGE('',*,*,#5675,.F.);
#8062=ORIENTED_EDGE('',*,*,#5674,.F.);
#8063=ORIENTED_EDGE('',*,*,#5673,.F.);
#8064=ORIENTED_EDGE('',*,*,#5672,.F.);
#8065=ORIENTED_EDGE('',*,*,#5671,.F.);
#8066=ORIENTED_EDGE('',*,*,#5670,.F.);
#8067=ORIENTED_EDGE('',*,*,#5669,.F.);
#8068=ORIENTED_EDGE('',*,*,#5668,.F.);
#8069=ORIENTED_EDGE('',*,*,#5667,.F.);
#8070=ORIENTED_EDGE('',*,*,#5846,.F.);
#8071=ORIENTED_EDGE('',*,*,#5783,.T.);
#8072=ORIENTED_EDGE('',*,*,#5782,.T.);
#8073=ORIENTED_EDGE('',*,*,#5781,.T.);
#8074=ORIENTED_EDGE('',*,*,#5780,.T.);
#8075=ORIENTED_EDGE('',*,*,#5779,.T.);
#8076=ORIENTED_EDGE('',*,*,#5778,.T.);
#8077=ORIENTED_EDGE('',*,*,#5777,.T.);
#8078=ORIENTED_EDGE('',*,*,#5776,.T.);
#8079=ORIENTED_EDGE('',*,*,#5775,.T.);
#8080=ORIENTED_EDGE('',*,*,#5774,.T.);
#8081=ORIENTED_EDGE('',*,*,#5773,.T.);
#8082=ORIENTED_EDGE('',*,*,#5772,.T.);
#8083=ORIENTED_EDGE('',*,*,#5771,.T.);
#8084=ORIENTED_EDGE('',*,*,#5770,.T.);
#8085=ORIENTED_EDGE('',*,*,#5769,.T.);
#8086=ORIENTED_EDGE('',*,*,#5768,.T.);
#8087=ORIENTED_EDGE('',*,*,#5767,.T.);
#8088=ORIENTED_EDGE('',*,*,#5766,.T.);
#8089=ORIENTED_EDGE('',*,*,#5765,.T.);
#8090=ORIENTED_EDGE('',*,*,#5764,.T.);
#8091=ORIENTED_EDGE('',*,*,#5763,.T.);
#8092=ORIENTED_EDGE('',*,*,#5762,.T.);
#8093=ORIENTED_EDGE('',*,*,#5761,.T.);
#8094=ORIENTED_EDGE('',*,*,#5760,.T.);
#8095=ORIENTED_EDGE('',*,*,#5759,.T.);
#8096=ORIENTED_EDGE('',*,*,#5758,.T.);
#8097=ORIENTED_EDGE('',*,*,#5757,.T.);
#8098=ORIENTED_EDGE('',*,*,#5756,.T.);
#8099=ORIENTED_EDGE('',*,*,#5755,.T.);
#8100=ORIENTED_EDGE('',*,*,#5754,.T.);
#8101=ORIENTED_EDGE('',*,*,#5753,.T.);
#8102=ORIENTED_EDGE('',*,*,#5752,.T.);
#8103=ORIENTED_EDGE('',*,*,#5751,.T.);
#8104=ORIENTED_EDGE('',*,*,#5750,.T.);
#8105=ORIENTED_EDGE('',*,*,#5749,.T.);
#8106=ORIENTED_EDGE('',*,*,#5748,.T.);
#8107=ORIENTED_EDGE('',*,*,#5747,.T.);
#8108=ORIENTED_EDGE('',*,*,#5746,.T.);
#8109=ORIENTED_EDGE('',*,*,#5745,.T.);
#8110=ORIENTED_EDGE('',*,*,#5744,.T.);
#8111=ORIENTED_EDGE('',*,*,#5666,.F.);
#8112=ORIENTED_EDGE('',*,*,#5847,.T.);
#8113=ORIENTED_EDGE('',*,*,#5784,.T.);
#8114=ORIENTED_EDGE('',*,*,#5846,.T.);
#8115=ORIENTED_EDGE('',*,*,#5845,.F.);
#8116=ORIENTED_EDGE('',*,*,#5844,.F.);
#8117=ORIENTED_EDGE('',*,*,#5742,.F.);
#8118=ORIENTED_EDGE('',*,*,#5824,.F.);
#8119=ORIENTED_EDGE('',*,*,#5823,.F.);
#8120=ORIENTED_EDGE('',*,*,#5822,.F.);
#8121=ORIENTED_EDGE('',*,*,#5821,.F.);
#8122=ORIENTED_EDGE('',*,*,#5820,.F.);
#8123=ORIENTED_EDGE('',*,*,#5819,.F.);
#8124=ORIENTED_EDGE('',*,*,#5818,.F.);
#8125=ORIENTED_EDGE('',*,*,#5817,.F.);
#8126=ORIENTED_EDGE('',*,*,#5816,.F.);
#8127=ORIENTED_EDGE('',*,*,#5815,.F.);
#8128=ORIENTED_EDGE('',*,*,#5814,.F.);
#8129=ORIENTED_EDGE('',*,*,#5813,.F.);
#8130=ORIENTED_EDGE('',*,*,#5812,.F.);
#8131=ORIENTED_EDGE('',*,*,#5811,.F.);
#8132=ORIENTED_EDGE('',*,*,#5810,.F.);
#8133=ORIENTED_EDGE('',*,*,#5809,.F.);
#8134=ORIENTED_EDGE('',*,*,#5808,.F.);
#8135=ORIENTED_EDGE('',*,*,#5807,.F.);
#8136=ORIENTED_EDGE('',*,*,#5806,.F.);
#8137=ORIENTED_EDGE('',*,*,#5805,.F.);
#8138=ORIENTED_EDGE('',*,*,#5804,.F.);
#8139=ORIENTED_EDGE('',*,*,#5803,.F.);
#8140=ORIENTED_EDGE('',*,*,#5802,.F.);
#8141=ORIENTED_EDGE('',*,*,#5801,.F.);
#8142=ORIENTED_EDGE('',*,*,#5800,.F.);
#8143=ORIENTED_EDGE('',*,*,#5799,.F.);
#8144=ORIENTED_EDGE('',*,*,#5798,.F.);
#8145=ORIENTED_EDGE('',*,*,#5797,.F.);
#8146=ORIENTED_EDGE('',*,*,#5796,.F.);
#8147=ORIENTED_EDGE('',*,*,#5795,.F.);
#8148=ORIENTED_EDGE('',*,*,#5794,.F.);
#8149=ORIENTED_EDGE('',*,*,#5793,.F.);
#8150=ORIENTED_EDGE('',*,*,#5792,.F.);
#8151=ORIENTED_EDGE('',*,*,#5791,.F.);
#8152=ORIENTED_EDGE('',*,*,#5790,.F.);
#8153=ORIENTED_EDGE('',*,*,#5789,.F.);
#8154=ORIENTED_EDGE('',*,*,#5788,.F.);
#8155=ORIENTED_EDGE('',*,*,#5787,.F.);
#8156=ORIENTED_EDGE('',*,*,#5786,.F.);
#8157=ORIENTED_EDGE('',*,*,#5785,.F.);
#8158=ORIENTED_EDGE('',*,*,#5847,.F.);
#8159=ORIENTED_EDGE('',*,*,#5665,.F.);
#8160=ORIENTED_EDGE('',*,*,#5664,.F.);
#8161=ORIENTED_EDGE('',*,*,#5663,.F.);
#8162=ORIENTED_EDGE('',*,*,#5662,.F.);
#8163=ORIENTED_EDGE('',*,*,#5661,.F.);
#8164=ORIENTED_EDGE('',*,*,#5660,.F.);
#8165=ORIENTED_EDGE('',*,*,#5659,.F.);
#8166=ORIENTED_EDGE('',*,*,#5658,.F.);
#8167=ORIENTED_EDGE('',*,*,#5657,.F.);
#8168=ORIENTED_EDGE('',*,*,#5656,.F.);
#8169=ORIENTED_EDGE('',*,*,#5655,.F.);
#8170=ORIENTED_EDGE('',*,*,#5654,.F.);
#8171=ORIENTED_EDGE('',*,*,#5653,.F.);
#8172=ORIENTED_EDGE('',*,*,#5652,.F.);
#8173=ORIENTED_EDGE('',*,*,#5651,.F.);
#8174=ORIENTED_EDGE('',*,*,#5650,.F.);
#8175=ORIENTED_EDGE('',*,*,#5649,.F.);
#8176=ORIENTED_EDGE('',*,*,#5648,.F.);
#8177=ORIENTED_EDGE('',*,*,#5647,.F.);
#8178=ORIENTED_EDGE('',*,*,#5646,.F.);
#8179=ORIENTED_EDGE('',*,*,#5645,.F.);
#8180=ORIENTED_EDGE('',*,*,#5644,.F.);
#8181=ORIENTED_EDGE('',*,*,#5643,.F.);
#8182=ORIENTED_EDGE('',*,*,#5642,.F.);
#8183=ORIENTED_EDGE('',*,*,#5641,.F.);
#8184=ORIENTED_EDGE('',*,*,#5640,.F.);
#8185=ORIENTED_EDGE('',*,*,#5639,.F.);
#8186=ORIENTED_EDGE('',*,*,#5638,.F.);
#8187=ORIENTED_EDGE('',*,*,#5637,.F.);
#8188=ORIENTED_EDGE('',*,*,#5636,.F.);
#8189=ORIENTED_EDGE('',*,*,#5635,.F.);
#8190=ORIENTED_EDGE('',*,*,#5634,.F.);
#8191=ORIENTED_EDGE('',*,*,#5633,.F.);
#8192=ORIENTED_EDGE('',*,*,#5632,.F.);
#8193=ORIENTED_EDGE('',*,*,#5631,.F.);
#8194=ORIENTED_EDGE('',*,*,#5630,.F.);
#8195=ORIENTED_EDGE('',*,*,#5629,.F.);
#8196=ORIENTED_EDGE('',*,*,#5628,.F.);
#8197=ORIENTED_EDGE('',*,*,#5627,.F.);
#8198=ORIENTED_EDGE('',*,*,#5626,.F.);
#8199=ORIENTED_EDGE('',*,*,#5625,.F.);
#8200=ORIENTED_EDGE('',*,*,#5624,.F.);
#8201=ORIENTED_EDGE('',*,*,#5623,.F.);
#8202=ORIENTED_EDGE('',*,*,#5622,.F.);
#8203=ORIENTED_EDGE('',*,*,#5621,.F.);
#8204=ORIENTED_EDGE('',*,*,#5620,.F.);
#8205=ORIENTED_EDGE('',*,*,#5619,.F.);
#8206=ORIENTED_EDGE('',*,*,#5618,.F.);
#8207=ORIENTED_EDGE('',*,*,#5617,.F.);
#8208=ORIENTED_EDGE('',*,*,#5616,.F.);
#8209=ORIENTED_EDGE('',*,*,#5615,.F.);
#8210=ORIENTED_EDGE('',*,*,#5614,.F.);
#8211=ORIENTED_EDGE('',*,*,#5613,.F.);
#8212=ORIENTED_EDGE('',*,*,#5612,.F.);
#8213=ORIENTED_EDGE('',*,*,#5611,.F.);
#8214=ORIENTED_EDGE('',*,*,#5610,.F.);
#8215=ORIENTED_EDGE('',*,*,#5609,.F.);
#8216=ORIENTED_EDGE('',*,*,#5608,.F.);
#8217=ORIENTED_EDGE('',*,*,#5607,.F.);
#8218=ORIENTED_EDGE('',*,*,#5606,.F.);
#8219=ORIENTED_EDGE('',*,*,#5605,.F.);
#8220=ORIENTED_EDGE('',*,*,#5604,.F.);
#8221=ORIENTED_EDGE('',*,*,#5603,.F.);
#8222=ORIENTED_EDGE('',*,*,#5602,.F.);
#8223=ORIENTED_EDGE('',*,*,#5601,.F.);
#8224=ORIENTED_EDGE('',*,*,#5600,.F.);
#8225=ORIENTED_EDGE('',*,*,#5599,.F.);
#8226=ORIENTED_EDGE('',*,*,#5598,.F.);
#8227=ORIENTED_EDGE('',*,*,#5597,.F.);
#8228=ORIENTED_EDGE('',*,*,#5596,.F.);
#8229=ORIENTED_EDGE('',*,*,#5595,.F.);
#8230=ORIENTED_EDGE('',*,*,#5594,.F.);
#8231=ORIENTED_EDGE('',*,*,#5593,.F.);
#8232=ORIENTED_EDGE('',*,*,#5592,.F.);
#8233=ORIENTED_EDGE('',*,*,#5848,.F.);
#8234=ORIENTED_EDGE('',*,*,#5590,.F.);
#8235=ORIENTED_EDGE('',*,*,#5849,.T.);
#8236=ORIENTED_EDGE('',*,*,#5848,.T.);
#8237=ORIENTED_EDGE('',*,*,#5849,.F.);
#8238=ORIENTED_EDGE('',*,*,#5741,.T.);
#8239=ORIENTED_EDGE('',*,*,#5850,.T.);
#8240=ORIENTED_EDGE('',*,*,#5851,.F.);
#8241=ORIENTED_EDGE('',*,*,#5850,.F.);
#8242=ORIENTED_EDGE('',*,*,#5851,.T.);
#8243=ORIENTED_EDGE('',*,*,#5825,.T.);
#8244=ORIENTED_EDGE('',*,*,#5841,.T.);
#8245=ORIENTED_EDGE('',*,*,#5838,.T.);
#8246=ORIENTED_EDGE('',*,*,#5835,.T.);
#8247=ORIENTED_EDGE('',*,*,#5832,.T.);
#8248=ORIENTED_EDGE('',*,*,#5829,.T.);
#9644=ADVANCED_FACE('',(#2666,#437,#438),#2326,.T.);
#9645=ADVANCED_FACE('',(#2667),#2327,.T.);
#9646=ADVANCED_FACE('',(#2668),#1080,.F.);
#9647=ADVANCED_FACE('',(#2669),#1081,.F.);
#9648=ADVANCED_FACE('',(#2670),#1082,.F.);
#9649=ADVANCED_FACE('',(#2671),#1083,.F.);
#9650=ADVANCED_FACE('',(#2672),#1084,.F.);
#9651=ADVANCED_FACE('',(#2673),#1085,.F.);
#9652=ADVANCED_FACE('',(#2674),#1086,.F.);
#9653=ADVANCED_FACE('',(#2675),#1087,.F.);
#9654=ADVANCED_FACE('',(#2676),#381,.F.);
#9655=ADVANCED_FACE('',(#2677),#1088,.T.);
#9656=ADVANCED_FACE('',(#2678),#382,.F.);
#9657=ADVANCED_FACE('',(#2679),#1089,.T.);
#9658=ADVANCED_FACE('',(#2680),#163,.T.);
#9659=ADVANCED_FACE('',(#2681),#164,.T.);
#9660=ADVANCED_FACE('',(#2682,#439),#1090,.T.);
#9885=CLOSED_SHELL('',(#9644,#9645,#9646,#9647,#9648,#9649,#9650,#9651,
#9652,#9653,#9654,#9655,#9656,#9657,#9658,#9659,#9660));
#10480=AXIS2_PLACEMENT_3D('',#23892,#11993,#11994);
#10481=AXIS2_PLACEMENT_3D('',#23893,#11995,#11996);
#10482=AXIS2_PLACEMENT_3D('',#23895,#11997,#11998);
#10483=AXIS2_PLACEMENT_3D('',#23898,#11999,#12000);
#10484=AXIS2_PLACEMENT_3D('',#30204,#12001,#12002);
#10485=AXIS2_PLACEMENT_3D('',#36248,#12003,#12004);
#10486=AXIS2_PLACEMENT_3D('',#36249,#12005,#12006);
#10487=AXIS2_PLACEMENT_3D('',#36759,#12007,#12008);
#10488=AXIS2_PLACEMENT_3D('',#54907,#12009,#12010);
#10489=AXIS2_PLACEMENT_3D('',#71754,#12011,#12012);
#10490=AXIS2_PLACEMENT_3D('',#71763,#12017,#12018);
#10491=AXIS2_PLACEMENT_3D('',#71769,#12022,#12023);
#10492=AXIS2_PLACEMENT_3D('',#71775,#12027,#12028);
#10493=AXIS2_PLACEMENT_3D('',#71781,#12032,#12033);
#10494=AXIS2_PLACEMENT_3D('',#71787,#12037,#12038);
#10495=AXIS2_PLACEMENT_3D('',#71790,#12041,#12042);
#10496=AXIS2_PLACEMENT_3D('',#71791,#12043,#12044);
#10497=AXIS2_PLACEMENT_3D('',#73815,#12045,#12046);
#10498=AXIS2_PLACEMENT_3D('',#75715,#12047,#12048);
#10499=AXIS2_PLACEMENT_3D('',#75717,#12049,#12050);
#10500=AXIS2_PLACEMENT_3D('',#75718,#12051,#12052);
#10501=AXIS2_PLACEMENT_3D('',#75720,#12054,#12055);
#10502=AXIS2_PLACEMENT_3D('',#75723,#12057,#12058);
#10503=AXIS2_PLACEMENT_3D('',#75724,#12059,#12060);
#11993=DIRECTION('axis',(0.,0.,1.));
#11994=DIRECTION('refdir',(1.,0.,0.));
#11995=DIRECTION('center_axis',(0.,0.,1.));
#11996=DIRECTION('ref_axis',(1.,0.,0.));
#11997=DIRECTION('center_axis',(0.,0.,1.));
#11998=DIRECTION('ref_axis',(1.,0.,0.));
#11999=DIRECTION('center_axis',(0.,0.,1.));
#12000=DIRECTION('ref_axis',(1.,0.,0.));
#12001=DIRECTION('center_axis',(0.,0.,-1.));
#12002=DIRECTION('ref_axis',(1.,0.,0.));
#12003=DIRECTION('center_axis',(0.,0.,-1.));
#12004=DIRECTION('ref_axis',(1.,0.,0.));
#12005=DIRECTION('center_axis',(0.,0.,1.));
#12006=DIRECTION('ref_axis',(1.,-1.2787674710755E-12,0.));
#12007=DIRECTION('center_axis',(0.,0.,1.));
#12008=DIRECTION('ref_axis',(1.,-1.2787674710755E-12,0.));
#12009=DIRECTION('center_axis',(0.,0.,-1.));
#12010=DIRECTION('ref_axis',(1.,-1.2787674710755E-12,0.));
#12011=DIRECTION('center_axis',(0.866025403784438,0.5,0.));
#12012=DIRECTION('ref_axis',(0.5,-0.866025403784438,0.));
#12013=DIRECTION('',(0.5,-0.866025403784438,0.));
#12014=DIRECTION('',(0.,0.,-1.));
#12015=DIRECTION('',(0.5,-0.866025403784438,0.));
#12016=DIRECTION('',(0.,0.,-1.));
#12017=DIRECTION('center_axis',(0.,1.,0.));
#12018=DIRECTION('ref_axis',(1.,0.,0.));
#12019=DIRECTION('',(1.,0.,0.));
#12020=DIRECTION('',(0.,0.,-1.));
#12021=DIRECTION('',(1.,0.,0.));
#12022=DIRECTION('center_axis',(-0.866025403784438,0.500000000000001,0.));
#12023=DIRECTION('ref_axis',(0.500000000000001,0.866025403784438,0.));
#12024=DIRECTION('',(0.500000000000001,0.866025403784438,0.));
#12025=DIRECTION('',(0.,0.,-1.));
#12026=DIRECTION('',(0.500000000000001,0.866025403784438,0.));
#12027=DIRECTION('center_axis',(-0.866025403784439,-0.499999999999999,0.));
#12028=DIRECTION('ref_axis',(-0.499999999999999,0.866025403784439,0.));
#12029=DIRECTION('',(-0.499999999999999,0.866025403784439,0.));
#12030=DIRECTION('',(0.,0.,-1.));
#12031=DIRECTION('',(-0.499999999999999,0.866025403784439,0.));
#12032=DIRECTION('center_axis',(0.,-1.,0.));
#12033=DIRECTION('ref_axis',(-1.,0.,0.));
#12034=DIRECTION('',(-1.,0.,0.));
#12035=DIRECTION('',(0.,0.,-1.));
#12036=DIRECTION('',(-1.,0.,0.));
#12037=DIRECTION('center_axis',(0.866025403784439,-0.5,0.));
#12038=DIRECTION('ref_axis',(-0.5,-0.866025403784439,0.));
#12039=DIRECTION('',(-0.5,-0.866025403784439,0.));
#12040=DIRECTION('',(-0.5,-0.866025403784439,0.));
#12041=DIRECTION('center_axis',(0.,0.,-1.));
#12042=DIRECTION('ref_axis',(-1.,0.,0.));
#12043=DIRECTION('center_axis',(0.,0.,1.));
#12044=DIRECTION('ref_axis',(1.,0.,0.));
#12045=DIRECTION('center_axis',(0.,0.,1.));
#12046=DIRECTION('ref_axis',(1.,0.,0.));
#12047=DIRECTION('center_axis',(0.,0.,-1.));
#12048=DIRECTION('ref_axis',(-1.,0.,0.));
#12049=DIRECTION('center_axis',(0.,0.,1.));
#12050=DIRECTION('ref_axis',(1.,0.,0.));
#12051=DIRECTION('center_axis',(0.,0.,1.));
#12052=DIRECTION('ref_axis',(1.,0.,0.));
#12053=DIRECTION('',(0.707106781186549,8.65956056235496E-17,-0.707106781186546));
#12054=DIRECTION('center_axis',(0.,0.,-1.));
#12055=DIRECTION('ref_axis',(1.,0.,0.));
#12056=DIRECTION('',(0.70710678118654,-8.65956056235484E-17,0.707106781186556));
#12057=DIRECTION('center_axis',(0.,0.,1.));
#12058=DIRECTION('ref_axis',(1.,0.,0.));
#12059=DIRECTION('center_axis',(0.,0.,1.));
#12060=DIRECTION('ref_axis',(1.,0.,0.));
#23892=CARTESIAN_POINT('',(0.,0.,0.));
#23893=CARTESIAN_POINT('Origin',(0.,2.1,8.275));
#23894=CARTESIAN_POINT('',(-0.3933,2.1,3.1433));
#23895=CARTESIAN_POINT('Origin',(0.,2.1,3.1433));
#23896=CARTESIAN_POINT('',(0.384471428898077,2.18286501288886,13.3567));
#23897=CARTESIAN_POINT('',(0.29316324943834,1.83781647805639,13.3567));
#23898=CARTESIAN_POINT('Origin',(0.,2.1,13.3567));
#23899=CARTESIAN_POINT('',(-0.392808029221009,2.09981557082489,13.3087163522035));
#23900=CARTESIAN_POINT('Ctrl Pts',(0.293163249438369,1.83781647805643,13.3567));
#23901=CARTESIAN_POINT('Ctrl Pts',(0.205874279401571,1.74021340252209,13.3500765521591));
#23902=CARTESIAN_POINT('Ctrl Pts',(-0.0723649223063588,1.64076470611477,
13.3368296564771));
#23903=CARTESIAN_POINT('Ctrl Pts',(-0.357038552261128,1.85969648354392,
13.3208351072118));
#23904=CARTESIAN_POINT('Ctrl Pts',(-0.393052229550994,2.04530970055771,
13.3114640057871));
#23905=CARTESIAN_POINT('Ctrl Pts',(-0.392808029221009,2.09981557082489,
13.3087163522035));
#23906=CARTESIAN_POINT('',(-0.393251878202368,2.10034280740082,13.1837163495333));
#23907=CARTESIAN_POINT('Ctrl Pts',(-0.392808029221009,2.09981557082489,
13.3087163522035));
#23908=CARTESIAN_POINT('Ctrl Pts',(-0.392463564313855,2.1767006411361,13.3048405579462));
#23909=CARTESIAN_POINT('Ctrl Pts',(-0.333298288113736,2.38542484271478,
13.2943413158479));
#23910=CARTESIAN_POINT('Ctrl Pts',(0.00570651033598579,2.56500954775341,
13.2772186259089));
#23911=CARTESIAN_POINT('Ctrl Pts',(0.394173573742321,2.34685779795354,13.257348282386));
#23912=CARTESIAN_POINT('Ctrl Pts',(0.420885805445878,1.90223262684733,13.2374779388633));
#23913=CARTESIAN_POINT('Ctrl Pts',(0.0615726668307027,1.63903988954688,
13.2176075953405));
#23914=CARTESIAN_POINT('Ctrl Pts',(-0.313461573621718,1.7830432015364,13.1996870664539));
#23915=CARTESIAN_POINT('Ctrl Pts',(-0.392298178424971,2.00783384627357,
13.1883899854082));
#23916=CARTESIAN_POINT('Ctrl Pts',(-0.39306562301603,2.1003425921784,13.1837163522035));
#23917=CARTESIAN_POINT('',(-0.393299999901611,2.10000879729578,13.0587163522061));
#23918=CARTESIAN_POINT('Ctrl Pts',(-0.393299850553082,2.10034286283405,
13.1837163488456));
#23919=CARTESIAN_POINT('Ctrl Pts',(-0.393277891496654,2.12553221774172,
13.1824445054716));
#23920=CARTESIAN_POINT('Ctrl Pts',(-0.390832020267695,2.15061417421091,
13.1811726620976));
#23921=CARTESIAN_POINT('Ctrl Pts',(-0.386046962715129,2.17518399150367,
13.1799008187235));
#23922=CARTESIAN_POINT('Ctrl Pts',(-0.383496234992751,2.18828120369264,
13.1792228485807));
#23923=CARTESIAN_POINT('Ctrl Pts',(-0.380281645786825,2.20123326940233,
13.1785448784378));
#23924=CARTESIAN_POINT('Ctrl Pts',(-0.376421488055696,2.21398137273228,
13.1778669082949));
#23925=CARTESIAN_POINT('Ctrl Pts',(-0.370477346392613,2.23361179651466,
13.1768229223095));
#23926=CARTESIAN_POINT('Ctrl Pts',(-0.362975776245312,2.25283444432371,
13.1757789363242));
#23927=CARTESIAN_POINT('Ctrl Pts',(-0.353993350086029,2.27138727518363,
13.1747349503388));
#23928=CARTESIAN_POINT('Ctrl Pts',(-0.345027440958812,2.28990599079487,
13.1736928840519));
#23929=CARTESIAN_POINT('Ctrl Pts',(-0.334586344420496,2.30775665364154,
13.172650817765));
#23930=CARTESIAN_POINT('Ctrl Pts',(-0.322795237567398,2.32469562657917,
13.1716087514782));
#23931=CARTESIAN_POINT('Ctrl Pts',(-0.311016785982873,2.34161641909875,
13.1705678036299));
#23932=CARTESIAN_POINT('Ctrl Pts',(-0.297891595095139,2.35762684698715,
13.1695268557816));
#23933=CARTESIAN_POINT('Ctrl Pts',(-0.283588888680998,2.3725109763233,13.1684859079333));
#23934=CARTESIAN_POINT('Ctrl Pts',(-0.269278826679315,2.38740276026083,
13.1674444247469));
#23935=CARTESIAN_POINT('Ctrl Pts',(-0.253790537533736,2.40116654681418,
13.1664029415606));
#23936=CARTESIAN_POINT('Ctrl Pts',(-0.237331461545412,2.4136218540866,13.1653614583742));
#23937=CARTESIAN_POINT('Ctrl Pts',(-0.220867349369152,2.42608097246411,
13.1643196565123));
#23938=CARTESIAN_POINT('Ctrl Pts',(-0.203432467039979,2.43723039977957,
13.1632778546504));
#23939=CARTESIAN_POINT('Ctrl Pts',(-0.185264047611803,2.44693244682862,
13.1622360527885));
#23940=CARTESIAN_POINT('Ctrl Pts',(-0.167056352371871,2.45665546740126,
13.1611919987982));
#23941=CARTESIAN_POINT('Ctrl Pts',(-0.148112629136325,2.46492456641514,
13.1601479448079));
#23942=CARTESIAN_POINT('Ctrl Pts',(-0.128691628157987,2.47164950537038,
13.1591038908176));
#23943=CARTESIAN_POINT('Ctrl Pts',(-0.121825642167522,2.47402700057286,
13.1587347821357));
#23944=CARTESIAN_POINT('Ctrl Pts',(-0.114900135186391,2.47621195498811,
13.1583656734539));
#23945=CARTESIAN_POINT('Ctrl Pts',(-0.107926882296612,2.47820190120851,
13.1579965647721));
#23946=CARTESIAN_POINT('Ctrl Pts',(-0.0882047006351017,2.4838299892007,
13.1569526289518));
#23947=CARTESIAN_POINT('Ctrl Pts',(-0.067982306282485,2.48792801563734,
13.1559086931315));
#23948=CARTESIAN_POINT('Ctrl Pts',(-0.0475214463151485,2.49041849615524,
13.1548647573111));
#23949=CARTESIAN_POINT('Ctrl Pts',(-0.0270982382722515,2.49290439370915,
13.1538227425339));
#23950=CARTESIAN_POINT('Ctrl Pts',(-0.0064381506447005,2.49378847026311,
13.1527807277566));
#23951=CARTESIAN_POINT('Ctrl Pts',(0.0141862272639498,2.49304406999218,
13.1517387129793));
#23952=CARTESIAN_POINT('Ctrl Pts',(0.0347884451167996,2.49230046954908,
13.1506978178046));
#23953=CARTESIAN_POINT('Ctrl Pts',(0.0553542967653325,2.48993186339393,
13.1496569226298));
#23954=CARTESIAN_POINT('Ctrl Pts',(0.0756106380122407,2.48596362706787,
13.1486160274551));
#23955=CARTESIAN_POINT('Ctrl Pts',(0.0958773755848161,2.48199335409181,
13.1475745980533));
#23956=CARTESIAN_POINT('Ctrl Pts',(0.115833560205196,2.47642193640849,13.1465331686515));
#23957=CARTESIAN_POINT('Ctrl Pts',(0.135215165358773,2.46932607416347,13.1454917392497));
#23958=CARTESIAN_POINT('Ctrl Pts',(0.154602688013568,2.46222804544291,13.1444499918835));
#23959=CARTESIAN_POINT('Ctrl Pts',(0.173414604016691,2.45360493232044,13.1434082445174));
#23960=CARTESIAN_POINT('Ctrl Pts',(0.191406737712538,2.44358165078805,13.1423664971512));
#23961=CARTESIAN_POINT('Ctrl Pts',(0.209437763911716,2.43353670253637,13.141322497903));
#23962=CARTESIAN_POINT('Ctrl Pts',(0.226644856785306,2.42208595134131,13.1402784986548));
#23963=CARTESIAN_POINT('Ctrl Pts',(0.242812088822247,2.40939809230468,13.1392344994066));
#23964=CARTESIAN_POINT('Ctrl Pts',(0.248532971016366,2.40490840930401,13.1388650733542));
#23965=CARTESIAN_POINT('Ctrl Pts',(0.254123961662768,2.4002641822085,13.1384956473018));
#23966=CARTESIAN_POINT('Ctrl Pts',(0.259576589738731,2.39547399895695,13.1381262212494));
#23967=CARTESIAN_POINT('Ctrl Pts',(0.274985324271206,2.38193728582399,13.1370822498118));
#23968=CARTESIAN_POINT('Ctrl Pts',(0.289378219602958,2.36715166976236,13.1360382783743));
#23969=CARTESIAN_POINT('Ctrl Pts',(0.302548435357331,2.35129531285488,13.1349943069367));
#23970=CARTESIAN_POINT('Ctrl Pts',(0.315694424602928,2.3354681235918,13.1339522558764));
#23971=CARTESIAN_POINT('Ctrl Pts',(0.327621688123889,2.31857462470843,13.1329102048162));
#23972=CARTESIAN_POINT('Ctrl Pts',(0.33816025659571,2.30082960653032,13.1318681537559));
#23973=CARTESIAN_POINT('Ctrl Pts',(0.348687507651402,2.28310364480713,13.130827221759));
#23974=CARTESIAN_POINT('Ctrl Pts',(0.357828625639041,2.26452859383173,13.129786289762));
#23975=CARTESIAN_POINT('Ctrl Pts',(0.365457091351407,2.24534787367199,13.1287453577651));
#23976=CARTESIAN_POINT('Ctrl Pts',(0.373089474834909,2.22615730281952,13.1277038911739));
#23977=CARTESIAN_POINT('Ctrl Pts',(0.37920736717172,2.2063611190848,13.1266624245828));
#23978=CARTESIAN_POINT('Ctrl Pts',(0.383732340163726,2.18622285725067,13.1256209579917));
#23979=CARTESIAN_POINT('Ctrl Pts',(0.388258695777645,2.1660784420976,13.1245791731767));
#23980=CARTESIAN_POINT('Ctrl Pts',(0.391191037230872,2.14559246595596,13.1235373883617));
#23981=CARTESIAN_POINT('Ctrl Pts',(0.392502222912741,2.12503787148615,13.1224956035467));
#23982=CARTESIAN_POINT('Ctrl Pts',(0.393816242581397,2.10443885047177,13.1214515670258));
#23983=CARTESIAN_POINT('Ctrl Pts',(0.393502122194069,2.08377165141165,13.120407530505));
#23984=CARTESIAN_POINT('Ctrl Pts',(0.39158482157553,2.06330916311038,13.1193634939842));
#23985=CARTESIAN_POINT('Ctrl Pts',(0.390906801444503,2.05607295880053,13.118994288565));
#23986=CARTESIAN_POINT('Ctrl Pts',(0.390028765919873,2.04886228550099,13.1186250831458));
#23987=CARTESIAN_POINT('Ctrl Pts',(0.388953345278611,2.04168889302562,13.1182558777266));
#23988=CARTESIAN_POINT('Ctrl Pts',(0.38591248675788,2.02140541436217,13.1172119127868));
#23989=CARTESIAN_POINT('Ctrl Pts',(0.381271655761468,2.00130000996013,13.1161679478471));
#23990=CARTESIAN_POINT('Ctrl Pts',(0.375068685372782,1.9816430346252,13.1151239829074));
#23991=CARTESIAN_POINT('Ctrl Pts',(0.368877125441056,1.96202221859088,13.1140819383568));
#23992=CARTESIAN_POINT('Ctrl Pts',(0.361129292266942,1.94284890588497,13.1130398938062));
#23993=CARTESIAN_POINT('Ctrl Pts',(0.351913775661758,1.92438227737644,13.1119978492557));
#23994=CARTESIAN_POINT('Ctrl Pts',(0.342708155609275,1.90593548019913,13.1109569237578));
#23995=CARTESIAN_POINT('Ctrl Pts',(0.332038282154381,1.88819452852851,13.1099159982599));
#23996=CARTESIAN_POINT('Ctrl Pts',(0.320040337939026,1.87139756761602,13.1088750727621));
#23997=CARTESIAN_POINT('Ctrl Pts',(0.308036230796624,1.85459197868835,13.1078336125769));
#23998=CARTESIAN_POINT('Ctrl Pts',(0.294703104591166,1.83873195732152,13.1067921523918));
#23999=CARTESIAN_POINT('Ctrl Pts',(0.280220087396299,1.82402610156102,13.1057506922067));
#24000=CARTESIAN_POINT('Ctrl Pts',(0.265732644198551,1.80931575169828,13.1047089137518));
#24001=CARTESIAN_POINT('Ctrl Pts',(0.250095152073664,1.79576076800596,13.103667135297));
#24002=CARTESIAN_POINT('Ctrl Pts',(0.233522411733559,1.78353171846433,13.1026253568422));
#24003=CARTESIAN_POINT('Ctrl Pts',(0.216913848346639,1.77127623504361,13.101581326516));
#24004=CARTESIAN_POINT('Ctrl Pts',(0.199366625946405,1.76035279699869,13.1005372961899));
#24005=CARTESIAN_POINT('Ctrl Pts',(0.181123703314227,1.75088813526645,13.0994932658637));
#24006=CARTESIAN_POINT('Ctrl Pts',(0.17467169949027,1.74754075311063,13.0991240219771));
#24007=CARTESIAN_POINT('Ctrl Pts',(0.168132872239832,1.74437540547865,13.0987547780904));
#24008=CARTESIAN_POINT('Ctrl Pts',(0.161518528472187,1.7413962424065,13.0983855342038));
#24009=CARTESIAN_POINT('Ctrl Pts',(0.142817870497033,1.73297328895537,13.0973415752146));
#24010=CARTESIAN_POINT('Ctrl Pts',(0.123400847963987,1.72599199312796,13.0962976162254));
#24011=CARTESIAN_POINT('Ctrl Pts',(0.10351525561347,1.72056689409689,13.0952536572363));
#24012=CARTESIAN_POINT('Ctrl Pts',(0.0836662466095349,1.71515177557205,
13.0942116188091));
#24013=CARTESIAN_POINT('Ctrl Pts',(0.0633510650414822,1.71128741990603,
13.093169580382));
#24014=CARTESIAN_POINT('Ctrl Pts',(0.0428355866410116,1.70903964073436,
13.0921275419548));
#24015=CARTESIAN_POINT('Ctrl Pts',(0.022342142943603,1.70679427579577,13.0910866227318));
#24016=CARTESIAN_POINT('Ctrl Pts',(0.00164955404500148,1.70616214888769,
13.0900457035087));
#24017=CARTESIAN_POINT('Ctrl Pts',(-0.0189682279706726,1.70715766988822,
13.0890047842856));
#24018=CARTESIAN_POINT('Ctrl Pts',(-0.0395965976908121,1.70815370211164,
13.0879633305267));
#24019=CARTESIAN_POINT('Ctrl Pts',(-0.0601493480777889,1.71077903267315,
13.0869218767677));
#24020=CARTESIAN_POINT('Ctrl Pts',(-0.0803541232532163,1.71499596771435,
13.0858804230087));
#24021=CARTESIAN_POINT('Ctrl Pts',(-0.100565071178656,1.71921419106912,
13.0848386510757));
#24022=CARTESIAN_POINT('Ctrl Pts',(-0.120427119989594,1.72502480129605,
13.0837968791428));
#24023=CARTESIAN_POINT('Ctrl Pts',(-0.139680579560224,1.73233952388961,
13.0827551072098));
#24024=CARTESIAN_POINT('Ctrl Pts',(-0.158975656144607,1.73967005750714,
13.0817110834511));
#24025=CARTESIAN_POINT('Ctrl Pts',(-0.177658851470548,1.74851087932031,
13.0806670596923));
#24026=CARTESIAN_POINT('Ctrl Pts',(-0.195492091675046,1.75872630911171,
13.0796230359336));
#24027=CARTESIAN_POINT('Ctrl Pts',(-0.201799888898195,1.76233960983175,
13.0792537541827));
#24028=CARTESIAN_POINT('Ctrl Pts',(-0.20800160610377,1.7661244877695,13.0788844724318));
#24029=CARTESIAN_POINT('Ctrl Pts',(-0.214087630197371,1.7700736800489,13.078515190681));
#24030=CARTESIAN_POINT('Ctrl Pts',(-0.231281785301351,1.78123088605782,
13.0774719007426));
#24031=CARTESIAN_POINT('Ctrl Pts',(-0.247652961663615,1.79376928691335,
13.0764286108042));
#24032=CARTESIAN_POINT('Ctrl Pts',(-0.262970887533086,1.80754281969823,
13.0753853208659));
#24033=CARTESIAN_POINT('Ctrl Pts',(-0.2782606347176,1.82129101484639,13.074343950152));
#24034=CARTESIAN_POINT('Ctrl Pts',(-0.29250039560478,1.83626938927644,13.0733025794381));
#24035=CARTESIAN_POINT('Ctrl Pts',(-0.305491059368287,1.85229028552348,
13.0722612087243));
#24036=CARTESIAN_POINT('Ctrl Pts',(-0.318467806746011,1.86829401921617,
13.0712209535898));
#24037=CARTESIAN_POINT('Ctrl Pts',(-0.330197629191986,1.88533750641536,
13.0701806984553));
#24038=CARTESIAN_POINT('Ctrl Pts',(-0.340520257307395,1.90319846453011,
13.0691404433208));
#24039=CARTESIAN_POINT('Ctrl Pts',(-0.350848207924016,1.9210686320216,13.0680996518152));
#24040=CARTESIAN_POINT('Ctrl Pts',(-0.359767132357192,1.93975648239246,
13.0670588603096));
#24041=CARTESIAN_POINT('Ctrl Pts',(-0.367161437262072,1.95901287651828,
13.0660180688041));
#24042=CARTESIAN_POINT('Ctrl Pts',(-0.374558056424921,1.97827529748018,
13.0649769515532));
#24043=CARTESIAN_POINT('Ctrl Pts',(-0.380428876601272,1.99810591598814,
13.0639358343023));
#24044=CARTESIAN_POINT('Ctrl Pts',(-0.384707693247568,2.01823887992367,
13.0628947170515));
#24045=CARTESIAN_POINT('Ctrl Pts',(-0.388995726059894,2.03841520835778,
13.0618513573326));
#24046=CARTESIAN_POINT('Ctrl Pts',(-0.3916848148126,2.05889445100123,13.0608079976137));
#24047=CARTESIAN_POINT('Ctrl Pts',(-0.392760317080386,2.07940331757505,
13.0597646378949));
#24048=CARTESIAN_POINT('Ctrl Pts',(-0.393120510410699,2.08627188231304,
13.0594152093319));
#24049=CARTESIAN_POINT('Ctrl Pts',(-0.393300153457839,2.09314377131058,
13.059065780769));
#24050=CARTESIAN_POINT('Ctrl Pts',(-0.393299999901611,2.10000879729578,
13.0587163522061));
#24051=CARTESIAN_POINT('',(-0.393299846364205,2.09965236528803,12.9337163522064));
#24052=CARTESIAN_POINT('Ctrl Pts',(-0.39329999990161,2.10000879734644,13.0587163522035));
#24053=CARTESIAN_POINT('Ctrl Pts',(-0.393299989427263,2.10047707045121,
13.0586925171884));
#24054=CARTESIAN_POINT('Ctrl Pts',(-0.393299142646321,2.10094534245175,
13.0586686821733));
#24055=CARTESIAN_POINT('Ctrl Pts',(-0.393297459568052,2.10141361144476,
13.0586448471582));
#24056=CARTESIAN_POINT('Ctrl Pts',(-0.393223741505037,2.12192358044329,
13.057600884333));
#24057=CARTESIAN_POINT('Ctrl Pts',(-0.391541130597174,2.14248887778938,
13.0565569215078));
#24058=CARTESIAN_POINT('Ctrl Pts',(-0.388247938399845,2.16283652065694,
13.0555129586825));
#24059=CARTESIAN_POINT('Ctrl Pts',(-0.384960804350849,2.18314673205032,
13.0544709163288));
#24060=CARTESIAN_POINT('Ctrl Pts',(-0.380069027615285,2.20323935611151,
13.053428873975));
#24061=CARTESIAN_POINT('Ctrl Pts',(-0.37362275919439,2.22284512123797,13.0523868316213));
#24062=CARTESIAN_POINT('Ctrl Pts',(-0.367183413903594,2.24242983026595,
13.0513459083948));
#24063=CARTESIAN_POINT('Ctrl Pts',(-0.359193092431404,2.26152801393411,
13.0503049851684));
#24064=CARTESIAN_POINT('Ctrl Pts',(-0.349752081724406,2.27988432763708,
13.0492640619419));
#24065=CARTESIAN_POINT('Ctrl Pts',(-0.34030622225204,2.29825006887498,13.0482226041124));
#24066=CARTESIAN_POINT('Ctrl Pts',(-0.329408507284762,2.31587251728544,
13.047181146283));
#24067=CARTESIAN_POINT('Ctrl Pts',(-0.317205992928561,2.33251934984041,
13.0461396884535));
#24068=CARTESIAN_POINT('Ctrl Pts',(-0.304999750088171,2.34917126884315,
13.0450979124061));
#24069=CARTESIAN_POINT('Ctrl Pts',(-0.29148837798416,2.36484640701149,13.0440561363587));
#24070=CARTESIAN_POINT('Ctrl Pts',(-0.276859733177765,2.37934490892933,
13.0430143603113));
#24071=CARTESIAN_POINT('Ctrl Pts',(-0.262199468123118,2.39387474978772,
13.0419703324342));
#24072=CARTESIAN_POINT('Ctrl Pts',(-0.246417671226193,2.40722240116009,
13.0409263045571));
#24073=CARTESIAN_POINT('Ctrl Pts',(-0.229736404323014,2.41922730855729,
13.0398822766799));
#24074=CARTESIAN_POINT('Ctrl Pts',(-0.223836479544724,2.42347327206983,
13.0395130189984));
#24075=CARTESIAN_POINT('Ctrl Pts',(-0.21782429496167,2.42755166837154,13.0391437613169));
#24076=CARTESIAN_POINT('Ctrl Pts',(-0.211710439165922,2.43145675426543,
13.0387745036354));
#24077=CARTESIAN_POINT('Ctrl Pts',(-0.194425398337294,2.44249717971381,
13.0377305414756));
#24078=CARTESIAN_POINT('Ctrl Pts',(-0.176222914177312,2.45221477202946,
13.0366865793157));
#24079=CARTESIAN_POINT('Ctrl Pts',(-0.157331601041175,2.46046034083352,
13.0356426171559));
#24080=CARTESIAN_POINT('Ctrl Pts',(-0.138475040730624,2.46869074092949,
13.0346005754891));
#24081=CARTESIAN_POINT('Ctrl Pts',(-0.11893280968917,2.47545414719846,13.0335585338223));
#24082=CARTESIAN_POINT('Ctrl Pts',(-0.0989584635155615,2.48064696570266,
13.0325164921555));
#24083=CARTESIAN_POINT('Ctrl Pts',(-0.0790055696679896,2.48583420715144,
13.0314755696351));
#24084=CARTESIAN_POINT('Ctrl Pts',(-0.0586221832361915,2.48945399735763,
13.0304346471147));
#24085=CARTESIAN_POINT('Ctrl Pts',(-0.0380772893152163,2.49145243649568,
13.0293937245942));
#24086=CARTESIAN_POINT('Ctrl Pts',(-0.017521844227084,2.49345190196492,
13.028352267491));
#24087=CARTESIAN_POINT('Ctrl Pts',(0.00319454329350911,2.49382826559513,
13.0273108103878));
#24088=CARTESIAN_POINT('Ctrl Pts',(0.023796928057364,2.49257941389613,13.0262693532845));
#24089=CARTESIAN_POINT('Ctrl Pts',(0.0444056076453001,2.49133018062472,
13.0252275779759));
#24090=CARTESIAN_POINT('Ctrl Pts',(0.0648994835106651,2.48845482407434,
13.0241858026673));
#24091=CARTESIAN_POINT('Ctrl Pts',(0.0850088237426345,2.48400311181798,
13.0231440273587));
#24092=CARTESIAN_POINT('Ctrl Pts',(0.1051616307887,2.47954177708039,13.0221000002282));
#24093=CARTESIAN_POINT('Ctrl Pts',(0.124927538499802,2.47349749943457,13.0210559730976));
#24094=CARTESIAN_POINT('Ctrl Pts',(0.144051343921903,2.46597008117371,13.0200119459671));
#24095=CARTESIAN_POINT('Ctrl Pts',(0.150815242582771,2.46330770864008,13.0196426840156));
#24096=CARTESIAN_POINT('Ctrl Pts',(0.157499014214537,2.46046023452778,13.0192734220641));
#24097=CARTESIAN_POINT('Ctrl Pts',(0.164092097660787,2.45743345322631,13.0189041601126));
#24098=CARTESIAN_POINT('Ctrl Pts',(0.182731804010363,2.4488762561115,13.0178601972387));
#24099=CARTESIAN_POINT('Ctrl Pts',(0.200755875449437,2.43883158084948,13.0168162343649));
#24100=CARTESIAN_POINT('Ctrl Pts',(0.217915116787653,2.42741089150397,13.0157722714911));
#24101=CARTESIAN_POINT('Ctrl Pts',(0.235042791917278,2.41601121170398,13.0147302290955));
#24102=CARTESIAN_POINT('Ctrl Pts',(0.251308156361853,2.40324089595244,13.0136881866999));
#24103=CARTESIAN_POINT('Ctrl Pts',(0.266486852156776,2.38925706149993,13.0126461443043));
#24104=CARTESIAN_POINT('Ctrl Pts',(0.28164924631423,2.37528824542599,13.0116052210429));
#24105=CARTESIAN_POINT('Ctrl Pts',(0.295726730730443,2.36010897274665,13.0105642977815));
#24106=CARTESIAN_POINT('Ctrl Pts',(0.308528378921624,2.34391623439204,13.0095233745201));
#24107=CARTESIAN_POINT('Ctrl Pts',(0.321336601720315,2.32771517985053,13.0084819166665));
#24108=CARTESIAN_POINT('Ctrl Pts',(0.332867210316033,2.31050018700096,13.0074404588128));
#24109=CARTESIAN_POINT('Ctrl Pts',(0.34296959482452,2.29250129097205,13.0063990009592));
#24110=CARTESIAN_POINT('Ctrl Pts',(0.353075066061434,2.27449689547873,13.0053572248938));
#24111=CARTESIAN_POINT('Ctrl Pts',(0.36175111619616,2.25570877877258,13.0043154488284));
#24112=CARTESIAN_POINT('Ctrl Pts',(0.368893579926101,2.23639067669495,13.003273672763));
#24113=CARTESIAN_POINT('Ctrl Pts',(0.376051482236477,2.21703081814727,13.0022296448774));
#24114=CARTESIAN_POINT('Ctrl Pts',(0.381668979991324,2.19713939590162,13.0011856169919));
#24115=CARTESIAN_POINT('Ctrl Pts',(0.385691842767505,2.17698501427295,13.0001415891064));
#24116=CARTESIAN_POINT('Ctrl Pts',(0.387114670926065,2.16985670209948,12.9997723316008));
#24117=CARTESIAN_POINT('Ctrl Pts',(0.388338492958074,2.16269556421669,12.9994030740953));
#24118=CARTESIAN_POINT('Ctrl Pts',(0.389362463971912,2.15551361679554,12.9990338165898));
#24119=CARTESIAN_POINT('Ctrl Pts',(0.392257428810782,2.13520885720969,12.9979898539379));
#24120=CARTESIAN_POINT('Ctrl Pts',(0.393568441845717,2.11461653557569,12.9969458912861));
#24121=CARTESIAN_POINT('Ctrl Pts',(0.393254330125343,2.09400651706701,12.9959019286342));
#24122=CARTESIAN_POINT('Ctrl Pts',(0.392940796247009,2.07343441288748,12.9948598864631));
#24123=CARTESIAN_POINT('Ctrl Pts',(0.391008023454439,2.05284540474457,12.993817844292));
#24124=CARTESIAN_POINT('Ctrl Pts',(0.387466669650576,2.03251318714081,12.9927758021209));
#24125=CARTESIAN_POINT('Ctrl Pts',(0.383929119201573,2.0122028059993,12.9917348790857));
#24126=CARTESIAN_POINT('Ctrl Pts',(0.378786514539462,1.99214939404301,12.9906939560505));
#24127=CARTESIAN_POINT('Ctrl Pts',(0.372101137137044,1.97262012034345,12.9896530330153));
#24128=CARTESIAN_POINT('Ctrl Pts',(0.365412326289747,1.95308081689078,12.9886115753877));
#24129=CARTESIAN_POINT('Ctrl Pts',(0.357179382852222,1.93406689080609,12.9875701177601));
#24130=CARTESIAN_POINT('Ctrl Pts',(0.347514196557822,1.9158294996728,12.9865286601325));
#24131=CARTESIAN_POINT('Ctrl Pts',(0.337846057119786,1.89758653620661,12.9854868842933));
#24132=CARTESIAN_POINT('Ctrl Pts',(0.326745179860557,1.88012121266505,12.9844451084542));
#24133=CARTESIAN_POINT('Ctrl Pts',(0.314368523790327,1.86365846482285,12.983403332615));
#24134=CARTESIAN_POINT('Ctrl Pts',(0.301965115283709,1.84716013235974,12.9823593049526));
#24135=CARTESIAN_POINT('Ctrl Pts',(0.288280910085889,1.83166925404743,12.9813152772902));
#24136=CARTESIAN_POINT('Ctrl Pts',(0.273512399539091,1.81737682809372,12.9802712496278));
#24137=CARTESIAN_POINT('Ctrl Pts',(0.268288971587627,1.81232178500157,12.9799019907742));
#24138=CARTESIAN_POINT('Ctrl Pts',(0.262930216575671,1.80741630175329,12.9795327319206));
#24139=CARTESIAN_POINT('Ctrl Pts',(0.257445780669388,1.80266759339835,12.979163473067));
#24140=CARTESIAN_POINT('Ctrl Pts',(0.2419402732851,1.78924212289936,12.9781195104829));
#24141=CARTESIAN_POINT('Ctrl Pts',(0.225335556935778,1.77699280464536,12.9770755478987));
#24142=CARTESIAN_POINT('Ctrl Pts',(0.207836251371787,1.76610034049774,12.9760315853146));
#24143=CARTESIAN_POINT('Ctrl Pts',(0.190369137693771,1.75522791422892,12.9749895432138));
#24144=CARTESIAN_POINT('Ctrl Pts',(0.17201128761171,1.74570782235724,12.973947501113));
#24145=CARTESIAN_POINT('Ctrl Pts',(0.152998597630337,1.73767925932518,12.9729054590122));
#24146=CARTESIAN_POINT('Ctrl Pts',(0.13400632700451,1.72965931885433,12.9718645360496));
#24147=CARTESIAN_POINT('Ctrl Pts',(0.114361275810847,1.72312803852619,12.970823613087));
#24148=CARTESIAN_POINT('Ctrl Pts',(0.0943217986337186,1.71817767443155,
12.9697826901245));
#24149=CARTESIAN_POINT('Ctrl Pts',(0.074272029725231,1.71322476796432,12.9687412325721));
#24150=CARTESIAN_POINT('Ctrl Pts',(0.0538281405908412,1.70985459186216,
12.9676997750198));
#24151=CARTESIAN_POINT('Ctrl Pts',(0.0332618769233426,1.70810902339613,
12.9666583174674));
#24152=CARTESIAN_POINT('Ctrl Pts',(0.0126893293803217,1.70636292158407,
12.9656165417051));
#24153=CARTESIAN_POINT('Ctrl Pts',(-0.00800493154724586,1.70624244172002,
12.9645747659428));
#24154=CARTESIAN_POINT('Ctrl Pts',(-0.0285468111130381,1.70773737168158,
12.9635329901805));
#24155=CARTESIAN_POINT('Ctrl Pts',(-0.0491330924183241,1.70923553296822,
12.9624889625963));
#24156=CARTESIAN_POINT('Ctrl Pts',(-0.0695656067424458,1.71235596399375,
12.961444935012));
#24157=CARTESIAN_POINT('Ctrl Pts',(-0.0895773950829874,1.71703684212428,
12.9604009074277));
#24158=CARTESIAN_POINT('Ctrl Pts',(-0.0966553104131074,1.71869240925874,
12.9600316481332));
#24159=CARTESIAN_POINT('Ctrl Pts',(-0.103680728015908,1.72054272172845,
12.9596623888388));
#24160=CARTESIAN_POINT('Ctrl Pts',(-0.110642359662777,1.72258357448535,
12.9592931295443));
#24161=CARTESIAN_POINT('Ctrl Pts',(-0.130324149002113,1.72835343363211,
12.9582491668622));
#24162=CARTESIAN_POINT('Ctrl Pts',(-0.149612029943242,1.73568420011201,
12.9572052041802));
#24163=CARTESIAN_POINT('Ctrl Pts',(-0.168243300725745,1.74450164309676,
12.9561612414981));
#24164=CARTESIAN_POINT('Ctrl Pts',(-0.186840297289561,1.75330286545046,
12.9551191992973));
#24165=CARTESIAN_POINT('Ctrl Pts',(-0.204782398349391,1.76358507820212,
12.9540771570964));
#24166=CARTESIAN_POINT('Ctrl Pts',(-0.221824871663632,1.77522528375593,
12.9530351148956));
#24167=CARTESIAN_POINT('Ctrl Pts',(-0.238849041637425,1.78685298791742,
12.9519941918312));
#24168=CARTESIAN_POINT('Ctrl Pts',(-0.254974881161543,1.79983540048527,
12.9509532687668));
#24169=CARTESIAN_POINT('Ctrl Pts',(-0.269984967643882,1.81400523213469,
12.9499123457024));
#24170=CARTESIAN_POINT('Ctrl Pts',(-0.285002762918998,1.8281823410437,12.9488708880468));
#24171=CARTESIAN_POINT('Ctrl Pts',(-0.298903114282888,1.84354759397336,
12.9478294303912));
#24172=CARTESIAN_POINT('Ctrl Pts',(-0.311503709712774,1.85989517115397,
12.9467879727356));
#24173=CARTESIAN_POINT('Ctrl Pts',(-0.324108155176177,1.87624774323506,
12.9457461968691));
#24174=CARTESIAN_POINT('Ctrl Pts',(-0.335411633959992,1.8935826327288,12.9447044210026));
#24175=CARTESIAN_POINT('Ctrl Pts',(-0.34527436015343,1.91166384781291,12.9436626451361));
#24176=CARTESIAN_POINT('Ctrl Pts',(-0.35515840485029,1.92978414584813,12.9426186174477));
#24177=CARTESIAN_POINT('Ctrl Pts',(-0.363595178957836,1.94865331781493,
12.9415745897594));
#24178=CARTESIAN_POINT('Ctrl Pts',(-0.370492154315508,1.96801343405235,
12.940530562071));
#24179=CARTESIAN_POINT('Ctrl Pts',(-0.372931522607136,1.97486084921953,
12.9401613033878));
#24180=CARTESIAN_POINT('Ctrl Pts',(-0.37517872820195,1.98176954231094,12.9397920447047));
#24181=CARTESIAN_POINT('Ctrl Pts',(-0.377231196270089,1.98872774577354,
12.9394227860215));
#24182=CARTESIAN_POINT('Ctrl Pts',(-0.384364369069022,2.01291037177361,
12.9381394598467));
#24183=CARTESIAN_POINT('Ctrl Pts',(-0.389176175554744,2.03780721766341,
12.936856133672));
#24184=CARTESIAN_POINT('Ctrl Pts',(-0.391557233824522,2.06301591369671,
12.9355728074972));
#24185=CARTESIAN_POINT('Ctrl Pts',(-0.392705377429683,2.07517151841772,
12.9349539890669));
#24186=CARTESIAN_POINT('Ctrl Pts',(-0.393289015992787,2.08739932130897,
12.9343351706367));
#24187=CARTESIAN_POINT('Ctrl Pts',(-0.393299846364205,2.09965236528802,
12.9337163522064));
#24188=CARTESIAN_POINT('',(-0.39329996604184,2.10016343649383,12.8087163521999));
#24189=CARTESIAN_POINT('Ctrl Pts',(-0.393299846364255,2.09965236534526,
12.9337163522035));
#24190=CARTESIAN_POINT('Ctrl Pts',(-0.393317930215556,2.12011170632657,
12.9326830891799));
#24191=CARTESIAN_POINT('Ctrl Pts',(-0.391735263661162,2.14060277128025,
12.9316498261563));
#24192=CARTESIAN_POINT('Ctrl Pts',(-0.388563460451927,2.16085496858617,
12.9306165631326));
#24193=CARTESIAN_POINT('Ctrl Pts',(-0.385390688312413,2.18111335258335,
12.9295829844653));
#24194=CARTESIAN_POINT('Ctrl Pts',(-0.380627895954077,2.20113197993515,
12.9285494057979));
#24195=CARTESIAN_POINT('Ctrl Pts',(-0.374338427906584,2.22064672143257,
12.9275158271306));
#24196=CARTESIAN_POINT('Ctrl Pts',(-0.368048185872011,2.24016386443002,
12.9264821212702));
#24197=CARTESIAN_POINT('Ctrl Pts',(-0.360231150982646,2.25917629499611,
12.9254484154098));
#24198=CARTESIAN_POINT('Ctrl Pts',(-0.350999807899556,2.27743738291148,
12.9244147095494));
#24199=CARTESIAN_POINT('Ctrl Pts',(-0.341747795418505,2.2957393582351,12.9233786891745));
#24200=CARTESIAN_POINT('Ctrl Pts',(-0.331075534220016,2.31328598694484,
12.9223426687996));
#24201=CARTESIAN_POINT('Ctrl Pts',(-0.319140661220974,2.32985675616662,
12.9213066484246));
#24202=CARTESIAN_POINT('Ctrl Pts',(-0.312404556588541,2.3392093848311,12.920721913116));
#24203=CARTESIAN_POINT('Ctrl Pts',(-0.305267016299046,2.34825170990766,
12.9201371778073));
#24204=CARTESIAN_POINT('Ctrl Pts',(-0.297761766329719,2.35694906209637,
12.9195524424987));
#24205=CARTESIAN_POINT('Ctrl Pts',(-0.284362198264628,2.3724769609825,12.9185084798591));
#24206=CARTESIAN_POINT('Ctrl Pts',(-0.269704794752743,2.3870001484392,12.9174645172196));
#24207=CARTESIAN_POINT('Ctrl Pts',(-0.253965873338599,2.40031021491012,
12.9164205545801));
#24208=CARTESIAN_POINT('Ctrl Pts',(-0.238255905369688,2.41359579607672,
12.9153785124225));
#24209=CARTESIAN_POINT('Ctrl Pts',(-0.22146888578192,2.42567217086989,12.9143364702649));
#24210=CARTESIAN_POINT('Ctrl Pts',(-0.20381808603056,2.43636747435928,12.9132944281074));
#24211=CARTESIAN_POINT('Ctrl Pts',(-0.186186242963999,2.44705129125882,
12.9122535050869));
#24212=CARTESIAN_POINT('Ctrl Pts',(-0.167693072504943,2.45635657735828,
12.9112125820665));
#24213=CARTESIAN_POINT('Ctrl Pts',(-0.148580860049953,2.46415466223408,
12.910171659046));
#24214=CARTESIAN_POINT('Ctrl Pts',(-0.129458832063715,2.47195675200183,
12.9091302014348));
#24215=CARTESIAN_POINT('Ctrl Pts',(-0.109717802104711,2.47824980126081,
12.9080887438235));
#24216=CARTESIAN_POINT('Ctrl Pts',(-0.0896205958273914,2.4829530503907,
12.9070472862123));
#24217=CARTESIAN_POINT('Ctrl Pts',(-0.0695172489793877,2.48765773656778,
12.9060055103905));
#24218=CARTESIAN_POINT('Ctrl Pts',(-0.0490582332257658,2.49077152330589,
12.9049637345686));
#24219=CARTESIAN_POINT('Ctrl Pts',(-0.0285162361747516,2.49226485220374,
12.9039219587468));
#24220=CARTESIAN_POINT('Ctrl Pts',(-0.00792983713114693,2.49376140896588,
12.9028779311029));
#24221=CARTESIAN_POINT('Ctrl Pts',(0.0127391648422252,2.49363051966932,
12.901833903459));
#24222=CARTESIAN_POINT('Ctrl Pts',(0.0332176744469679,2.49189472579295,
12.9007898758151));
#24223=CARTESIAN_POINT('Ctrl Pts',(0.0404606559185965,2.4912807981621,12.9004206168687));
#24224=CARTESIAN_POINT('Ctrl Pts',(0.0476798729945234,2.4904665786042,12.9000513579223));
#24225=CARTESIAN_POINT('Ctrl Pts',(0.0548635477976874,2.48945459443053,
12.8996820989759));
#24226=CARTESIAN_POINT('Ctrl Pts',(0.075173111794499,2.48659352987763,12.8986381363232));
#24227=CARTESIAN_POINT('Ctrl Pts',(0.0953187854656397,2.48213098626654,
12.8975941736705));
#24228=CARTESIAN_POINT('Ctrl Pts',(0.115029890446542,2.47610239869463,12.8965502110178));
#24229=CARTESIAN_POINT('Ctrl Pts',(0.13470473472776,2.4700849013586,12.8955081688468));
#24230=CARTESIAN_POINT('Ctrl Pts',(0.153945884114854,2.4625072344424,12.8944661266759));
#24231=CARTESIAN_POINT('Ctrl Pts',(0.172493383800945,2.4534556868193,12.8934240845049));
#24232=CARTESIAN_POINT('Ctrl Pts',(0.191020963765159,2.44441386041546,12.8923831614707));
#24233=CARTESIAN_POINT('Ctrl Pts',(0.208855702399793,2.43390159085845,12.8913422384366));
#24234=CARTESIAN_POINT('Ctrl Pts',(0.225758257843078,2.42205294442942,12.8903013154024));
#24235=CARTESIAN_POINT('Ctrl Pts',(0.242669493999045,2.41019821284388,12.8892598577773));
#24236=CARTESIAN_POINT('Ctrl Pts',(0.258646978794167,2.39700614239969,12.8882184001522));
#24237=CARTESIAN_POINT('Ctrl Pts',(0.273480535815841,2.38265400497761,12.8871769425271));
#24238=CARTESIAN_POINT('Ctrl Pts',(0.288318625136341,2.36829748235138,12.8861351666912));
#24239=CARTESIAN_POINT('Ctrl Pts',(0.302011587692007,2.35278072431232,12.8850933908553));
#24240=CARTESIAN_POINT('Ctrl Pts',(0.314386959518568,2.33631701099301,12.8840516150195));
#24241=CARTESIAN_POINT('Ctrl Pts',(0.326789080991684,2.31981771098439,12.8830075873615));
#24242=CARTESIAN_POINT('Ctrl Pts',(0.337867531099198,2.30236799098489,12.8819635597036));
#24243=CARTESIAN_POINT('Ctrl Pts',(0.347493431699077,2.2842096765265,12.8809195320456));
#24244=CARTESIAN_POINT('Ctrl Pts',(0.35089798625785,2.27778731930107,12.8805502731815));
#24245=CARTESIAN_POINT('Ctrl Pts',(0.354121267761971,2.27127652200698,12.8801810143173));
#24246=CARTESIAN_POINT('Ctrl Pts',(0.357159025645194,2.26468855576565,12.8798117554531));
#24247=CARTESIAN_POINT('Ctrl Pts',(0.365747325257615,2.24606316490433,12.8787677928062));
#24248=CARTESIAN_POINT('Ctrl Pts',(0.3729003558302,2.22670866641481,12.8777238301594));
#24249=CARTESIAN_POINT('Ctrl Pts',(0.378501388736522,2.20687183316723,12.8766798675126));
#24250=CARTESIAN_POINT('Ctrl Pts',(0.384092117939278,2.18707149191191,12.8756378253475));
#24251=CARTESIAN_POINT('Ctrl Pts',(0.388136261762029,2.16679126110359,12.8745957831825));
#24252=CARTESIAN_POINT('Ctrl Pts',(0.390565655198947,2.14629642512136,12.8735537410174));
#24253=CARTESIAN_POINT('Ctrl Pts',(0.392992439505489,2.12582360027092,12.8725128179893));
#24254=CARTESIAN_POINT('Ctrl Pts',(0.393807801369165,2.10513735136339,12.8714718949611));
#24255=CARTESIAN_POINT('Ctrl Pts',(0.392994906043685,2.08451149381913,12.870430971933));
#24256=CARTESIAN_POINT('Ctrl Pts',(0.392181593236339,2.06387504337163,12.8693895143139));
#24257=CARTESIAN_POINT('Ctrl Pts',(0.389738365505875,2.04329978209165,12.8683480566948));
#24258=CARTESIAN_POINT('Ctrl Pts',(0.385700503932339,2.02305839053971,12.8673065990757));
#24259=CARTESIAN_POINT('Ctrl Pts',(0.381661408616018,2.00281081436001,12.8662648232459));
#24260=CARTESIAN_POINT('Ctrl Pts',(0.376026888797889,1.9828980248649,12.865223047416));
#24261=CARTESIAN_POINT('Ctrl Pts',(0.368882916370616,1.96358048523063,12.8641812715862));
#24262=CARTESIAN_POINT('Ctrl Pts',(0.36172350208465,1.94422119029561,12.8631372439343));
#24263=CARTESIAN_POINT('Ctrl Pts',(0.353048430440259,1.92546038241904,12.8620932162823));
#24264=CARTESIAN_POINT('Ctrl Pts',(0.342991268606171,1.90753732917802,12.8610491886304));
#24265=CARTESIAN_POINT('Ctrl Pts',(0.339434182249748,1.90119818010189,12.8606799297304));
#24266=CARTESIAN_POINT('Ctrl Pts',(0.335704607486352,1.89496357446836,12.8603106708303));
#24267=CARTESIAN_POINT('Ctrl Pts',(0.331809720370535,1.88884318749416,12.8599414119303));
#24268=CARTESIAN_POINT('Ctrl Pts',(0.320798160023472,1.87153973080601,12.8588974492837));
#24269=CARTESIAN_POINT('Ctrl Pts',(0.30839661586408,1.85504839488947,12.8578534866371));
#24270=CARTESIAN_POINT('Ctrl Pts',(0.294749391624824,1.83960090987717,12.8568095239905));
#24271=CARTESIAN_POINT('Ctrl Pts',(0.281127272925502,1.82418184217854,12.8557674818258));
#24272=CARTESIAN_POINT('Ctrl Pts',(0.266264459886931,1.80980339827059,12.854725439661));
#24273=CARTESIAN_POINT('Ctrl Pts',(0.250347109415109,1.7966664957386,12.8536833974962));
#24274=CARTESIAN_POINT('Ctrl Pts',(0.234446853928001,1.78354370203386,12.8526424744684));
#24275=CARTESIAN_POINT('Ctrl Pts',(0.217494855587536,1.77166029087087,12.8516015514406));
#24276=CARTESIAN_POINT('Ctrl Pts',(0.199712230348975,1.76117863844049,12.8505606284128));
#24277=CARTESIAN_POINT('Ctrl Pts',(0.181920472417946,1.75069160290684,12.849519170794));
#24278=CARTESIAN_POINT('Ctrl Pts',(0.163297861035636,1.74160815182395,12.8484777131753));
#24279=CARTESIAN_POINT('Ctrl Pts',(0.144092769185384,1.73404622714271,12.8474362555565));
#24280=CARTESIAN_POINT('Ctrl Pts',(0.124881809342569,1.72648199196391,12.8463944797271));
#24281=CARTESIAN_POINT('Ctrl Pts',(0.105088712027454,1.72044044435186,12.8453527038977));
#24282=CARTESIAN_POINT('Ctrl Pts',(0.0849790174808098,1.71599029102379,
12.8443109280682));
#24283=CARTESIAN_POINT('Ctrl Pts',(0.0648258553731176,1.71153051858832,
12.8432669004167));
#24284=CARTESIAN_POINT('Ctrl Pts',(0.0443554591847135,1.70866910985458,
12.8422228727652));
#24285=CARTESIAN_POINT('Ctrl Pts',(0.0238413117000786,1.70742327901871,
12.8411788451136));
#24286=CARTESIAN_POINT('Ctrl Pts',(0.0165857265000572,1.70698264497427,
12.8408095862116));
#24287=CARTESIAN_POINT('Ctrl Pts',(0.00932467220683392,1.70674363352745,
12.8404403273095));
#24288=CARTESIAN_POINT('Ctrl Pts',(0.00207016844406672,1.70670544829274,
12.8400710684075));
#24289=CARTESIAN_POINT('Ctrl Pts',(-0.018439644367605,1.70659749163,12.8390271057592));
#24290=CARTESIAN_POINT('Ctrl Pts',(-0.0390190348449233,1.70809787389726,
12.8379831431109));
#24291=CARTESIAN_POINT('Ctrl Pts',(-0.05939504592475,1.71121070163957,12.8369391804626));
#24292=CARTESIAN_POINT('Ctrl Pts',(-0.0797335731368521,1.71431780299987,
12.8358971382961));
#24293=CARTESIAN_POINT('Ctrl Pts',(-0.0998687354948376,1.71903141084047,
12.8348550961295));
#24294=CARTESIAN_POINT('Ctrl Pts',(-0.119530827798182,1.72530376142016,
12.833813053963));
#24295=CARTESIAN_POINT('Ctrl Pts',(-0.139171803323475,1.73156937559392,
12.8327721309334));
#24296=CARTESIAN_POINT('Ctrl Pts',(-0.158340011223974,1.73939021415808,
12.8317312079038));
#24297=CARTESIAN_POINT('Ctrl Pts',(-0.176779228628762,1.74866825602371,
12.8306902848741));
#24298=CARTESIAN_POINT('Ctrl Pts',(-0.195227915935204,1.75795106284992,
12.8296488272536));
#24299=CARTESIAN_POINT('Ctrl Pts',(-0.21294620028672,1.76869225176188,12.828607369633));
#24300=CARTESIAN_POINT('Ctrl Pts',(-0.229700465195227,1.78074683041652,
12.8275659120124));
#24301=CARTESIAN_POINT('Ctrl Pts',(-0.246459849262177,1.79280509227054,
12.8265241361812));
#24302=CARTESIAN_POINT('Ctrl Pts',(-0.262254051887945,1.80617708403007,
12.8254823603499));
#24303=CARTESIAN_POINT('Ctrl Pts',(-0.276881561503866,1.82067672689305,
12.8244405845186));
#24304=CARTESIAN_POINT('Ctrl Pts',(-0.291540688813689,1.83520771106304,
12.8233965568652));
#24305=CARTESIAN_POINT('Ctrl Pts',(-0.305027607840395,1.85087065448245,
12.8223525292119));
#24306=CARTESIAN_POINT('Ctrl Pts',(-0.317179803406605,1.86744492628423,
12.8213085015585));
#24307=CARTESIAN_POINT('Ctrl Pts',(-0.321477875633597,1.87330702889159,
12.8209392426672));
#24308=CARTESIAN_POINT('Ctrl Pts',(-0.325609380499227,1.87928287195875,
12.820569983776));
#24309=CARTESIAN_POINT('Ctrl Pts',(-0.329568481179749,1.885361918074,12.8202007248847));
#24310=CARTESIAN_POINT('Ctrl Pts',(-0.340996590095234,1.90290933773148,
12.8191348437243));
#24311=CARTESIAN_POINT('Ctrl Pts',(-0.351050771947492,1.9214196059709,12.818068962564));
#24312=CARTESIAN_POINT('Ctrl Pts',(-0.359575330480823,1.94065612120446,
12.8170030814036));
#24313=CARTESIAN_POINT('Ctrl Pts',(-0.368081184057702,1.95985042684109,
12.815939539046));
#24314=CARTESIAN_POINT('Ctrl Pts',(-0.375063746194578,1.97976721269897,
12.8148759966883));
#24315=CARTESIAN_POINT('Ctrl Pts',(-0.380412644867909,2.00014455635969,
12.8138124543307));
#24316=CARTESIAN_POINT('Ctrl Pts',(-0.385752843557379,2.02048875627031,
12.8127506418247));
#24317=CARTESIAN_POINT('Ctrl Pts',(-0.389464444032076,2.0412913688329,12.8116888293188));
#24318=CARTESIAN_POINT('Ctrl Pts',(-0.391486464389773,2.06227417065729,
12.8106270168128));
#24319=CARTESIAN_POINT('Ctrl Pts',(-0.392699297074441,2.07485991331397,
12.8099901286097));
#24320=CARTESIAN_POINT('Ctrl Pts',(-0.393305224118923,2.08751018874901,
12.8093532404066));
#24321=CARTESIAN_POINT('Ctrl Pts',(-0.39329996604187,2.10016343642201,12.8087163522035));
#24322=CARTESIAN_POINT('',(-0.39342120080697,2.10027707468048,12.6837163522035));
#24323=CARTESIAN_POINT('Ctrl Pts',(-0.39329996604184,2.10016343649382,12.8087163521999));
#24324=CARTESIAN_POINT('Ctrl Pts',(-0.393290593258356,2.12271846896977,
12.8075810678464));
#24325=CARTESIAN_POINT('Ctrl Pts',(-0.391336792531897,2.14521105601326,
12.8064457834928));
#24326=CARTESIAN_POINT('Ctrl Pts',(-0.387495400099244,2.16732165254899,
12.8053104991393));
#24327=CARTESIAN_POINT('Ctrl Pts',(-0.38362857989576,2.1895786082999,12.8041676998675));
#24328=CARTESIAN_POINT('Ctrl Pts',(-0.377849299340276,2.21144802287218,
12.8030249005957));
#24329=CARTESIAN_POINT('Ctrl Pts',(-0.370265105169706,2.23262217723166,
12.8018821013238));
#24330=CARTESIAN_POINT('Ctrl Pts',(-0.366832438914899,2.24220576693271,
12.8013648613365));
#24331=CARTESIAN_POINT('Ctrl Pts',(-0.363030680309679,2.25164721999182,
12.8008476213493));
#24332=CARTESIAN_POINT('Ctrl Pts',(-0.358872916032692,2.26091960768717,
12.800330381362));
#24333=CARTESIAN_POINT('Ctrl Pts',(-0.350481162284677,2.27963437577207,
12.7992864187145));
#24334=CARTESIAN_POINT('Ctrl Pts',(-0.34059653621493,2.29774670930704,12.7982424560671));
#24335=CARTESIAN_POINT('Ctrl Pts',(-0.32932829007445,2.31500643561679,12.7971984934196));
#24336=CARTESIAN_POINT('Ctrl Pts',(-0.318080773087009,2.3322344108001,12.796156451254));
#24337=CARTESIAN_POINT('Ctrl Pts',(-0.305455036274669,2.34861225044094,
12.7951144090883));
#24338=CARTESIAN_POINT('Ctrl Pts',(-0.291606203295323,2.36391421371288,
12.7940723669227));
#24339=CARTESIAN_POINT('Ctrl Pts',(-0.27777224374508,2.37919974291661,12.7930314438939));
#24340=CARTESIAN_POINT('Ctrl Pts',(-0.262718265589452,2.39341112747198,
12.7919905208652));
#24341=CARTESIAN_POINT('Ctrl Pts',(-0.246639560738822,2.4063557035189,12.7909495978364));
#24342=CARTESIAN_POINT('Ctrl Pts',(-0.230552598284487,2.41930692756267,
12.7899081402168));
#24343=CARTESIAN_POINT('Ctrl Pts',(-0.213440420774801,2.43098956937945,
12.7888666825971));
#24344=CARTESIAN_POINT('Ctrl Pts',(-0.19553172014492,2.44125098742299,12.7878252249774));
#24345=CARTESIAN_POINT('Ctrl Pts',(-0.177617547626279,2.45151554077709,
12.786783449147));
#24346=CARTESIAN_POINT('Ctrl Pts',(-0.15890702334585,2.460357671781,12.7857416733166));
#24347=CARTESIAN_POINT('Ctrl Pts',(-0.139652950420971,2.46767097171074,
12.7846998974863));
#24348=CARTESIAN_POINT('Ctrl Pts',(-0.120357259380547,2.47500007950423,
12.7836558698338));
#24349=CARTESIAN_POINT('Ctrl Pts',(-0.10051638103565,2.48079355231629,12.7826118421813));
#24350=CARTESIAN_POINT('Ctrl Pts',(-0.0803984287066173,2.48499478264193,
12.7815678145288));
#24351=CARTESIAN_POINT('Ctrl Pts',(-0.0732829726542685,2.48648070274249,
12.7811985556322));
#24352=CARTESIAN_POINT('Ctrl Pts',(-0.0661329291528956,2.48776791378742,
12.7808292967356));
#24353=CARTESIAN_POINT('Ctrl Pts',(-0.0589603065575513,2.48885546447316,
12.7804600378391));
#24354=CARTESIAN_POINT('Ctrl Pts',(-0.0386819865373434,2.49193016979197,
12.7794160751914));
#24355=CARTESIAN_POINT('Ctrl Pts',(-0.018102085510851,2.49342353262573,
12.7783721125437));
#24356=CARTESIAN_POINT('Ctrl Pts',(0.00250990663971027,2.49329199123382,
12.7773281498961));
#24357=CARTESIAN_POINT('Ctrl Pts',(0.0230839808096885,2.49316069182646,
12.7762861077302));
#24358=CARTESIAN_POINT('Ctrl Pts',(0.0436893010881905,2.49141036678333,
12.7752440655643));
#24359=CARTESIAN_POINT('Ctrl Pts',(0.0640520893075922,2.48804924926526,
12.7742020233985));
#24360=CARTESIAN_POINT('Ctrl Pts',(0.0843930082123747,2.48469174153459,
12.7731611003695));
#24361=CARTESIAN_POINT('Ctrl Pts',(0.104491185179972,2.4797269664095,12.7721201773406));
#24362=CARTESIAN_POINT('Ctrl Pts',(0.124078909947421,2.47321483639622,12.7710792543116));
#24363=CARTESIAN_POINT('Ctrl Pts',(0.14367669445982,2.46669936192269,12.7700377966917));
#24364=CARTESIAN_POINT('Ctrl Pts',(0.162762799756044,2.45863516179295,12.7689963390718));
#24365=CARTESIAN_POINT('Ctrl Pts',(0.181085087014295,2.44913189665372,12.7679548814519));
#24366=CARTESIAN_POINT('Ctrl Pts',(0.199412972530104,2.43962572785268,12.7669131056213));
#24367=CARTESIAN_POINT('Ctrl Pts',(0.216975939463557,2.42867998931199,12.7658713297907));
#24368=CARTESIAN_POINT('Ctrl Pts',(0.233547670559036,2.41644964145413,12.7648295539601));
#24369=CARTESIAN_POINT('Ctrl Pts',(0.250155221827326,2.40419285742184,12.7637855263074));
#24370=CARTESIAN_POINT('Ctrl Pts',(0.265766703446861,2.39064640317974,12.7627414986547));
#24371=CARTESIAN_POINT('Ctrl Pts',(0.280189384229086,2.37600507054278,12.761697471002));
#24372=CARTESIAN_POINT('Ctrl Pts',(0.285290497363255,2.37082662311377,12.7613282121068));
#24373=CARTESIAN_POINT('Ctrl Pts',(0.290243255177885,2.36551152913714,12.7609589532116));
#24374=CARTESIAN_POINT('Ctrl Pts',(0.295040357460439,2.36006937049491,12.7605896943164));
#24375=CARTESIAN_POINT('Ctrl Pts',(0.308602645774295,2.34468338949881,12.7595457316689));
#24376=CARTESIAN_POINT('Ctrl Pts',(0.320998564262121,2.32818782453299,12.7585017690214));
#24377=CARTESIAN_POINT('Ctrl Pts',(0.332045605689831,2.31078568675807,12.7574578063738));
#24378=CARTESIAN_POINT('Ctrl Pts',(0.343072324894443,2.29341556209079,12.7564157642081));
#24379=CARTESIAN_POINT('Ctrl Pts',(0.3527546524404,2.27514275730554,12.7553737220423));
#24380=CARTESIAN_POINT('Ctrl Pts',(0.360951309847737,2.25620192674613,12.7543316798766));
#24381=CARTESIAN_POINT('Ctrl Pts',(0.369139164173787,2.23728143834118,12.7532907568478));
#24382=CARTESIAN_POINT('Ctrl Pts',(0.375844198701232,2.21769500882111,12.7522498338189));
#24383=CARTESIAN_POINT('Ctrl Pts',(0.380971872535446,2.19770016549032,12.7512089107901));
#24384=CARTESIAN_POINT('Ctrl Pts',(0.386102179809297,2.17769505332912,12.7501674531704));
#24385=CARTESIAN_POINT('Ctrl Pts',(0.389653309617672,2.15728181703275,12.7491259955506));
#24386=CARTESIAN_POINT('Ctrl Pts',(0.391580979295629,2.1367318207264,12.7480845379308));
#24387=CARTESIAN_POINT('Ctrl Pts',(0.393509237960712,2.11617554550027,12.7470427621003));
#24388=CARTESIAN_POINT('Ctrl Pts',(0.393813016364664,2.09548316240203,12.7460009862699));
#24389=CARTESIAN_POINT('Ctrl Pts',(0.392500098385387,2.07492884590887,12.7449592104394));
#24390=CARTESIAN_POINT('Ctrl Pts',(0.391184342504103,2.05433010079415,12.7439151827868));
#24391=CARTESIAN_POINT('Ctrl Pts',(0.388245018321332,2.03387074708653,12.7428711551342));
#24392=CARTESIAN_POINT('Ctrl Pts',(0.383741581407897,2.01381828094911,12.7418271274817));
#24393=CARTESIAN_POINT('Ctrl Pts',(0.382148774800765,2.00672598651557,12.7414578685856));
#24394=CARTESIAN_POINT('Ctrl Pts',(0.380360765913862,1.99968446264585,12.7410886096896));
#24395=CARTESIAN_POINT('Ctrl Pts',(0.378381659628227,1.9927050343353,12.7407193507936));
#24396=CARTESIAN_POINT('Ctrl Pts',(0.372786363049382,1.97297290997607,12.739675388146));
#24397=CARTESIAN_POINT('Ctrl Pts',(0.36562673134054,1.953620852398,12.7386314254985));
#24398=CARTESIAN_POINT('Ctrl Pts',(0.356974665456834,1.93491221056062,12.7375874628509));
#24399=CARTESIAN_POINT('Ctrl Pts',(0.348338515980635,1.91623798528587,12.7365454206852));
#24400=CARTESIAN_POINT('Ctrl Pts',(0.33821563340283,1.89820551153,12.7355033785194));
#24401=CARTESIAN_POINT('Ctrl Pts',(0.326726842703097,1.88106060140471,12.7344613363537));
#24402=CARTESIAN_POINT('Ctrl Pts',(0.315250390784098,1.86393410464357,12.7334204133248));
#24403=CARTESIAN_POINT('Ctrl Pts',(0.302411326502362,1.84769390335969,12.732379490296));
#24404=CARTESIAN_POINT('Ctrl Pts',(0.288375006731796,1.83255889341308,12.7313385672671));
#24405=CARTESIAN_POINT('Ctrl Pts',(0.274331478273237,1.81741611051983,12.7302971096474));
#24406=CARTESIAN_POINT('Ctrl Pts',(0.259089954438587,1.80338020334509,12.7292556520276));
#24407=CARTESIAN_POINT('Ctrl Pts',(0.242854632036266,1.7906352998506,12.7282141944078));
#24408=CARTESIAN_POINT('Ctrl Pts',(0.226614349035148,1.77788650223246,12.7271724185773));
#24409=CARTESIAN_POINT('Ctrl Pts',(0.209380263580363,1.76642991905275,12.7261306427468));
#24410=CARTESIAN_POINT('Ctrl Pts',(0.191387120035008,1.7564074210861,12.7250888669163));
#24411=CARTESIAN_POINT('Ctrl Pts',(0.173355083901566,1.74636325926265,12.7240448392638));
#24412=CARTESIAN_POINT('Ctrl Pts',(0.154561383701292,1.73775967782343,12.7230008116112));
#24413=CARTESIAN_POINT('Ctrl Pts',(0.135263119372274,1.73069148596643,12.7219567839586));
#24414=CARTESIAN_POINT('Ctrl Pts',(0.128437576234481,1.72819155915417,12.7215875250627));
#24415=CARTESIAN_POINT('Ctrl Pts',(0.121549055374674,1.72588324493719,12.7212182661667));
#24416=CARTESIAN_POINT('Ctrl Pts',(0.114609301097982,1.72376922228261,12.7208490072708));
#24417=CARTESIAN_POINT('Ctrl Pts',(0.0949893425059211,1.71779249237378,
12.7198050446232));
#24418=CARTESIAN_POINT('Ctrl Pts',(0.0748421479967187,1.71333682046681,
12.7187610819756));
#24419=CARTESIAN_POINT('Ctrl Pts',(0.054428067376843,1.71048430650149,12.7177171193281));
#24420=CARTESIAN_POINT('Ctrl Pts',(0.0340515406579967,1.70763704004299,
12.7166750771623));
#24421=CARTESIAN_POINT('Ctrl Pts',(0.0134098146149503,1.70638723708833,
12.7156330349965));
#24422=CARTESIAN_POINT('Ctrl Pts',(-0.00722502278297791,1.7067663683689,
12.7145909928307));
#24423=CARTESIAN_POINT('Ctrl Pts',(-0.0278376986897041,1.70714509246843,
12.7135500698018));
#24424=CARTESIAN_POINT('Ctrl Pts',(-0.0484427681833268,1.70914929319555,
12.712509146773));
#24425=CARTESIAN_POINT('Ctrl Pts',(-0.0687666690419001,1.71275842781426,
12.7114682237441));
#24426=CARTESIAN_POINT('Ctrl Pts',(-0.0891010077262566,1.71636941599046,
12.7104267661243));
#24427=CARTESIAN_POINT('Ctrl Pts',(-0.109153162032004,1.7215868719547,12.7093853085045));
#24428=CARTESIAN_POINT('Ctrl Pts',(-0.128657778450192,1.72833877516714,
12.7083438508847));
#24429=CARTESIAN_POINT('Ctrl Pts',(-0.14816835437902,1.73509274138037,12.7073020750542));
#24430=CARTESIAN_POINT('Ctrl Pts',(-0.167130376496693,1.74338181351447,
12.7062602992237));
#24431=CARTESIAN_POINT('Ctrl Pts',(-0.185297485950494,1.75308541151974,
12.7052185233931));
#24432=CARTESIAN_POINT('Ctrl Pts',(-0.203503864023646,1.76280998407231,
12.7041744957405));
#24433=CARTESIAN_POINT('Ctrl Pts',(-0.220911278838742,1.77395478960106,
12.7031304680879));
#24434=CARTESIAN_POINT('Ctrl Pts',(-0.237300840282622,1.78635497580679,
12.7020864404353));
#24435=CARTESIAN_POINT('Ctrl Pts',(-0.243097613333569,1.79074075912809,
12.7017171815395));
#24436=CARTESIAN_POINT('Ctrl Pts',(-0.248767366062678,1.79528321860555,
12.7013479226437));
#24437=CARTESIAN_POINT('Ctrl Pts',(-0.254301488541851,1.79997392959045,
12.700978663748));
#24438=CARTESIAN_POINT('Ctrl Pts',(-0.269725217596206,1.81304705104297,
12.699949530551));
#24439=CARTESIAN_POINT('Ctrl Pts',(-0.284190372762731,1.82735715623177,
12.698920397354));
#24440=CARTESIAN_POINT('Ctrl Pts',(-0.297489980694176,1.8427363193403,12.697891264157));
#24441=CARTESIAN_POINT('Ctrl Pts',(-0.310764998574633,1.8580870474448,12.6968640337558));
#24442=CARTESIAN_POINT('Ctrl Pts',(-0.322878205604673,1.87450238736961,
12.6958368033546));
#24443=CARTESIAN_POINT('Ctrl Pts',(-0.333658479324258,1.89177678041337,
12.6948095729534));
#24444=CARTESIAN_POINT('Ctrl Pts',(-0.344434541860459,1.90904442542467,
12.6937827438273));
#24445=CARTESIAN_POINT('Ctrl Pts',(-0.353878263301965,1.92716984179229,
12.6927559147013));
#24446=CARTESIAN_POINT('Ctrl Pts',(-0.361861105604863,1.94591745637345,
12.6917290855752));
#24447=CARTESIAN_POINT('Ctrl Pts',(-0.369841686340488,1.96465975968954,
12.6907025473534));
#24448=CARTESIAN_POINT('Ctrl Pts',(-0.376361921247464,1.98402320961346,
12.6896760091316));
#24449=CARTESIAN_POINT('Ctrl Pts',(-0.38134134509607,2.00375204666945,12.6886494709098));
#24450=CARTESIAN_POINT('Ctrl Pts',(-0.386329346774736,2.02351486970789,
12.6876211643167));
#24451=CARTESIAN_POINT('Ctrl Pts',(-0.389771084541329,2.04364359186479,
12.6865928577236));
#24452=CARTESIAN_POINT('Ctrl Pts',(-0.391637110626739,2.06387156826072,
12.6855645511305));
#24453=CARTESIAN_POINT('Ctrl Pts',(-0.392755061061598,2.07599030292631,
12.6849484848215));
#24454=CARTESIAN_POINT('Ctrl Pts',(-0.393308446986103,2.08814453182548,
12.6843324185125));
#24455=CARTESIAN_POINT('Ctrl Pts',(-0.393299902462425,2.10027698925372,
12.6837163522035));
#24456=CARTESIAN_POINT('',(-0.393370510321481,2.0996853138986,12.5587163522035));
#24457=CARTESIAN_POINT('Ctrl Pts',(-0.393690665213019,2.10027726445613,
12.6837163522035));
#24458=CARTESIAN_POINT('Ctrl Pts',(-0.393827751509988,2.11741474265097,
12.6828470082107));
#24459=CARTESIAN_POINT('Ctrl Pts',(-0.385020221980793,2.26497915337671,
12.6753542163767));
#24460=CARTESIAN_POINT('Ctrl Pts',(-0.198467542194671,2.52057776709468,
12.6612379767026));
#24461=CARTESIAN_POINT('Ctrl Pts',(0.246195250088315,2.49454140760323,12.6413676331794));
#24462=CARTESIAN_POINT('Ctrl Pts',(0.465007416872288,2.10656701859771,12.6214972896568));
#24463=CARTESIAN_POINT('Ctrl Pts',(0.257238583719243,1.71256828404793,12.6016269461339));
#24464=CARTESIAN_POINT('Ctrl Pts',(-0.18651163012543,1.67398540481866,12.5817566026112));
#24465=CARTESIAN_POINT('Ctrl Pts',(-0.382777726348084,1.9275339801708,12.5674530713011));
#24466=CARTESIAN_POINT('Ctrl Pts',(-0.39377123766665,2.07884159406489,12.5597729878318));
#24467=CARTESIAN_POINT('Ctrl Pts',(-0.393589312541075,2.09968513886256,
12.5587163522035));
#24468=CARTESIAN_POINT('',(-0.393063587406926,2.09989359760973,12.4337163554286));
#24469=CARTESIAN_POINT('Ctrl Pts',(-0.393299874152304,2.09968537040569,
12.5587163522035));
#24470=CARTESIAN_POINT('Ctrl Pts',(-0.393316073204164,2.11993484843599,
12.5576890687256));
#24471=CARTESIAN_POINT('Ctrl Pts',(-0.391764136452784,2.14024179843025,
12.5566617852476));
#24472=CARTESIAN_POINT('Ctrl Pts',(-0.388643851428118,2.16033942945636,
12.5556345017697));
#24473=CARTESIAN_POINT('Ctrl Pts',(-0.385527866712678,2.18040936236277,
12.5546086340715));
#24474=CARTESIAN_POINT('Ctrl Pts',(-0.380847892929046,2.20026979672838,
12.5535827663734));
#24475=CARTESIAN_POINT('Ctrl Pts',(-0.374655546270946,2.21965831207409,
12.5525568986753));
#24476=CARTESIAN_POINT('Ctrl Pts',(-0.368461716593899,2.23905147081868,
12.5515307852898));
#24477=CARTESIAN_POINT('Ctrl Pts',(-0.360754992450185,2.25797175237034,
12.5505046719044));
#24478=CARTESIAN_POINT('Ctrl Pts',(-0.351637115186527,2.27617102265497,
12.5494785585189));
#24479=CARTESIAN_POINT('Ctrl Pts',(-0.342518065902537,2.29437263229054,
12.5484523132359));
#24480=CARTESIAN_POINT('Ctrl Pts',(-0.331987870839673,2.31185238142415,
12.5474260679528));
#24481=CARTESIAN_POINT('Ctrl Pts',(-0.320194088805975,2.32838703004705,
12.5463998226698));
#24482=CARTESIAN_POINT('Ctrl Pts',(-0.308375411432332,2.34495658144305,
12.545371411099));
#24483=CARTESIAN_POINT('Ctrl Pts',(-0.295288311023228,2.3605764668794,12.5443429995283));
#24484=CARTESIAN_POINT('Ctrl Pts',(-0.281120681691834,2.37505645297851,
12.5433145879575));
#24485=CARTESIAN_POINT('Ctrl Pts',(-0.275157080608436,2.38115153485624,
12.5428816971602));
#24486=CARTESIAN_POINT('Ctrl Pts',(-0.269002461012857,2.38704511247016,
12.5424488063629));
#24487=CARTESIAN_POINT('Ctrl Pts',(-0.262672555761914,2.39272515855236,
12.5420159155656));
#24488=CARTESIAN_POINT('Ctrl Pts',(-0.247407309456433,2.40642319968154,
12.540971952918));
#24489=CARTESIAN_POINT('Ctrl Pts',(-0.231022191321355,2.41896474513736,
12.5399279902705));
#24490=CARTESIAN_POINT('Ctrl Pts',(-0.213718587953237,2.43016549662749,
12.5388840276229));
#24491=CARTESIAN_POINT('Ctrl Pts',(-0.196446816428079,2.4413456431283,12.5378419854572));
#24492=CARTESIAN_POINT('Ctrl Pts',(-0.178260491938778,2.45118944640849,
12.5367999432914));
#24493=CARTESIAN_POINT('Ctrl Pts',(-0.159393008216892,2.45955355502563,
12.5357579011256));
#24494=CARTESIAN_POINT('Ctrl Pts',(-0.140545787876112,2.46790868072152,
12.5347169780968));
#24495=CARTESIAN_POINT('Ctrl Pts',(-0.121019518127539,2.47478694351721,
12.5336760550679));
#24496=CARTESIAN_POINT('Ctrl Pts',(-0.101070878754924,2.48009152511955,
12.5326351320391));
#24497=CARTESIAN_POINT('Ctrl Pts',(-0.081111994281074,2.48539883101675,
12.5315936744193));
#24498=CARTESIAN_POINT('Ctrl Pts',(-0.0607310137548827,2.48913063645375,
12.5305522167995));
#24499=CARTESIAN_POINT('Ctrl Pts',(-0.040198898411932,2.49124025683264,
12.5295107591797));
#24500=CARTESIAN_POINT('Ctrl Pts',(-0.0196605096126161,2.49335052179252,
12.5284689833493));
#24501=CARTESIAN_POINT('Ctrl Pts',(0.0010283709272217,2.49383757582712,
12.5274272075188));
#24502=CARTESIAN_POINT('Ctrl Pts',(0.0215935105388922,2.4927067739454,12.5263854316883));
#24503=CARTESIAN_POINT('Ctrl Pts',(0.0422031021665188,2.49157352780976,
12.5253414040357));
#24504=CARTESIAN_POINT('Ctrl Pts',(0.0626876889855271,2.4888155423744,12.5242973763831));
#24505=CARTESIAN_POINT('Ctrl Pts',(0.0827792586853799,2.48448990146882,
12.5232533487305));
#24506=CARTESIAN_POINT('Ctrl Pts',(0.0898853835329845,2.48295997897992,
12.5228840898346));
#24507=CARTESIAN_POINT('Ctrl Pts',(0.0969424688577103,2.48123441215734,
12.5225148309388));
#24508=CARTESIAN_POINT('Ctrl Pts',(0.103939153748573,2.47931720540734,12.5221455720429));
#24509=CARTESIAN_POINT('Ctrl Pts',(0.123720065635645,2.47389691016998,12.5211016093953));
#24510=CARTESIAN_POINT('Ctrl Pts',(0.143134782110379,2.46690897464314,12.5200576467478));
#24511=CARTESIAN_POINT('Ctrl Pts',(0.161919327665279,2.4584229642872,12.5190136841002));
#24512=CARTESIAN_POINT('Ctrl Pts',(0.180669317024478,2.44995256486173,12.5179716419345));
#24513=CARTESIAN_POINT('Ctrl Pts',(0.198790749121794,2.439989806198,12.5169295997687));
#24514=CARTESIAN_POINT('Ctrl Pts',(0.216036751253761,2.42865333119827,12.5158875576029));
#24515=CARTESIAN_POINT('Ctrl Pts',(0.233264231450364,2.41732903139461,12.5148466345741));
#24516=CARTESIAN_POINT('Ctrl Pts',(0.24961752059224,2.40463432211781,12.5138057115452));
#24517=CARTESIAN_POINT('Ctrl Pts',(0.264876266720187,2.39073261483428,12.5127647885164));
#24518=CARTESIAN_POINT('Ctrl Pts',(0.280142849342448,2.37682376799621,12.5117233308966));
#24519=CARTESIAN_POINT('Ctrl Pts',(0.294313211189345,2.36170716837339,12.5106818732768));
#24520=CARTESIAN_POINT('Ctrl Pts',(0.307201422802289,2.34558537380766,12.509640415657));
#24521=CARTESIAN_POINT('Ctrl Pts',(0.320093572325771,2.32945865333083,12.5085986398265));
#24522=CARTESIAN_POINT('Ctrl Pts',(0.33170236093904,2.3123267233007,12.507556863996));
#24523=CARTESIAN_POINT('Ctrl Pts',(0.341883844130885,2.29442306221817,12.5065150881655));
#24524=CARTESIAN_POINT('Ctrl Pts',(0.35208733482969,2.27648070196593,12.5054710605129));
#24525=CARTESIAN_POINT('Ctrl Pts',(0.360857048273736,2.2577639472548,12.5044270328603));
#24526=CARTESIAN_POINT('Ctrl Pts',(0.368095901662538,2.23852904814241,12.5033830052077));
#24527=CARTESIAN_POINT('Ctrl Pts',(0.370656189221089,2.23172591645258,12.5030137463118));
#24528=CARTESIAN_POINT('Ctrl Pts',(0.37302542954117,2.22485811225872,12.5026444874159));
#24529=CARTESIAN_POINT('Ctrl Pts',(0.375200839732851,2.21793735567564,12.5022752285201));
#24530=CARTESIAN_POINT('Ctrl Pts',(0.381351123473112,2.19837110704542,12.5012312658725));
#24531=CARTESIAN_POINT('Ctrl Pts',(0.385985078996909,2.17826417006023,12.5001873032249));
#24532=CARTESIAN_POINT('Ctrl Pts',(0.389018303476915,2.15787615709377,12.4991433405774));
#24533=CARTESIAN_POINT('Ctrl Pts',(0.392045948013639,2.13752565007411,12.4981012984116));
#24534=CARTESIAN_POINT('Ctrl Pts',(0.393478540779884,2.11689580423328,12.4970592562458));
#24535=CARTESIAN_POINT('Ctrl Pts',(0.393282202197022,2.0962584181072,12.4960172140801));
#24536=CARTESIAN_POINT('Ctrl Pts',(0.393086074478714,2.07564319620961,12.4949762910512));
#24537=CARTESIAN_POINT('Ctrl Pts',(0.391264466525502,2.05502118239317,12.4939353680224));
#24538=CARTESIAN_POINT('Ctrl Pts',(0.387835497127093,2.03466611010983,12.4928944449935));
#24539=CARTESIAN_POINT('Ctrl Pts',(0.38440476669937,2.01430058399189,12.4918529873737));
#24540=CARTESIAN_POINT('Ctrl Pts',(0.379365131992984,1.99420300152393,12.4908115297539));
#24541=CARTESIAN_POINT('Ctrl Pts',(0.372786260292589,1.97463934374348,12.4897700721341));
#24542=CARTESIAN_POINT('Ctrl Pts',(0.366205378460076,1.95506970841268,12.4887282963036));
#24543=CARTESIAN_POINT('Ctrl Pts',(0.358084591987923,1.93603500781878,12.4876865204731));
#24544=CARTESIAN_POINT('Ctrl Pts',(0.348542294015158,1.91778265921529,12.4866447446426));
#24545=CARTESIAN_POINT('Ctrl Pts',(0.338979370148784,1.8994908577461,12.4856007169901));
#24546=CARTESIAN_POINT('Ctrl Pts',(0.327989192021601,1.88198540815059,12.4845566893375));
#24547=CARTESIAN_POINT('Ctrl Pts',(0.315734666595995,1.86548665217196,12.4835126616849));
#24548=CARTESIAN_POINT('Ctrl Pts',(0.311400401582283,1.85965125844398,12.483143402789));
#24549=CARTESIAN_POINT('Ctrl Pts',(0.306908341447079,1.8539414922597,12.4827741438931));
#24550=CARTESIAN_POINT('Ctrl Pts',(0.302266834244163,1.8483660378327,12.4824048849973));
#24551=CARTESIAN_POINT('Ctrl Pts',(0.289144441791431,1.83260320522365,12.4813609223497));
#24552=CARTESIAN_POINT('Ctrl Pts',(0.274746613027273,1.81782264415175,12.4803169597022));
#24553=CARTESIAN_POINT('Ctrl Pts',(0.259245945908198,1.8042358548942,12.4792729970546));
#24554=CARTESIAN_POINT('Ctrl Pts',(0.243773793936582,1.79067405999955,12.4782309548888));
#24555=CARTESIAN_POINT('Ctrl Pts',(0.227203338538617,1.7783022020407,12.4771889127231));
#24556=CARTESIAN_POINT('Ctrl Pts',(0.20974477316162,1.76729589703254,12.4761468705573));
#24557=CARTESIAN_POINT('Ctrl Pts',(0.192304958009566,1.75630141262306,12.4751059475284));
#24558=CARTESIAN_POINT('Ctrl Pts',(0.173979530268808,1.74666998450989,12.4740650244996));
#24559=CARTESIAN_POINT('Ctrl Pts',(0.155008457955053,1.73853455495387,12.4730241014707));
#24560=CARTESIAN_POINT('Ctrl Pts',(0.136027642593012,1.73039494725327,12.4719826438509));
#24561=CARTESIAN_POINT('Ctrl Pts',(0.11640119009215,1.72375317781577,12.4709411862312));
#24562=CARTESIAN_POINT('Ctrl Pts',(0.0963904542310355,1.71869464948268,
12.4698997286114));
#24563=CARTESIAN_POINT('Ctrl Pts',(0.0763736042177105,1.71363457554865,
12.4688579527809));
#24564=CARTESIAN_POINT('Ctrl Pts',(0.0559729587031034,1.71015885084542,
12.4678161769504));
#24565=CARTESIAN_POINT('Ctrl Pts',(0.0354606388891938,1.7083018597318,12.4667744011199));
#24566=CARTESIAN_POINT('Ctrl Pts',(0.0149039812305196,1.70644085468974,
12.4657303734673));
#24567=CARTESIAN_POINT('Ctrl Pts',(-0.00576409621383964,1.70620557706198,
12.4646863458147));
#24568=CARTESIAN_POINT('Ctrl Pts',(-0.0262701416788386,1.70757832672472,
12.4636423181621));
#24569=CARTESIAN_POINT('Ctrl Pts',(-0.0335228611716422,1.70806385028676,
12.4632730592662));
#24570=CARTESIAN_POINT('Ctrl Pts',(-0.0407553681268636,1.70875005527154,
12.4629038003703));
#24571=CARTESIAN_POINT('Ctrl Pts',(-0.0479558417498726,1.70963462340768,
12.4625345414745));
#24572=CARTESIAN_POINT('Ctrl Pts',(-0.0683129017726483,1.7121354598227,
12.4614905788269));
#24573=CARTESIAN_POINT('Ctrl Pts',(-0.0885344670210547,1.71624042725586,
12.4604466161794));
#24574=CARTESIAN_POINT('Ctrl Pts',(-0.108349273882756,1.72191889117667,
12.4594026535318));
#24575=CARTESIAN_POINT('Ctrl Pts',(-0.128127629272081,1.72758690895121,
12.458360611366));
#24576=CARTESIAN_POINT('Ctrl Pts',(-0.147499995870457,1.73482253427522,
12.4573185692003));
#24577=CARTESIAN_POINT('Ctrl Pts',(-0.166204931077286,1.74354409685686,
12.4562765270345));
#24578=CARTESIAN_POINT('Ctrl Pts',(-0.184889777477541,1.75225629261729,
12.4552356040056));
#24579=CARTESIAN_POINT('Ctrl Pts',(-0.202907939835433,1.76245097430072,
12.4541946809768));
#24580=CARTESIAN_POINT('Ctrl Pts',(-0.220017738894964,1.77399833655095,
12.4531537579479));
#24581=CARTESIAN_POINT('Ctrl Pts',(-0.237136325101362,1.78555162922548,
12.4521123003281));
#24582=CARTESIAN_POINT('Ctrl Pts',(-0.253344997127429,1.79845859208211,
12.4510708427083));
#24583=CARTESIAN_POINT('Ctrl Pts',(-0.268430471212415,1.81254570428557,
12.4500293850885));
#24584=CARTESIAN_POINT('Ctrl Pts',(-0.283520554567386,1.82663712071593,
12.448987609258));
#24585=CARTESIAN_POINT('Ctrl Pts',(-0.297486244161894,1.8419088761414,12.4479458334275));
#24586=CARTESIAN_POINT('Ctrl Pts',(-0.310151324887868,1.8581507790579,12.4469040575971));
#24587=CARTESIAN_POINT('Ctrl Pts',(-0.322843781473253,1.87442778921615,
12.4458600299445));
#24588=CARTESIAN_POINT('Ctrl Pts',(-0.334229610884264,1.8916785187495,12.4448160022919));
#24589=CARTESIAN_POINT('Ctrl Pts',(-0.344175671320527,1.90966346312107,
12.4437719746393));
#24590=CARTESIAN_POINT('Ctrl Pts',(-0.347693462526264,1.91602450220297,
12.4434027157434));
#24591=CARTESIAN_POINT('Ctrl Pts',(-0.351031575786892,1.92247717870157,
12.4430334568475));
#24592=CARTESIAN_POINT('Ctrl Pts',(-0.354185561536747,1.92901029855895,
12.4426641979517));
#24593=CARTESIAN_POINT('Ctrl Pts',(-0.363789505481296,1.94890376729011,
12.441539797901));
#24594=CARTESIAN_POINT('Ctrl Pts',(-0.371733180364064,1.96964892991815,
12.4404153978504));
#24595=CARTESIAN_POINT('Ctrl Pts',(-0.377883062466265,1.99096201991454,
12.4392909977998));
#24596=CARTESIAN_POINT('Ctrl Pts',(-0.384000616375438,2.01216307301722,
12.4381725084026));
#24597=CARTESIAN_POINT('Ctrl Pts',(-0.388342935182014,2.03392560141778,
12.4370540190054));
#24598=CARTESIAN_POINT('Ctrl Pts',(-0.390825227665587,2.05594853668558,
12.4359355296082));
#24599=CARTESIAN_POINT('Ctrl Pts',(-0.392466916440398,2.07051362353847,
12.4351958055425));
#24600=CARTESIAN_POINT('Ctrl Pts',(-0.393296004457353,2.08519217356933,
12.4344560814769));
#24601=CARTESIAN_POINT('Ctrl Pts',(-0.393299985579107,2.09989349425388,
12.4337163574112));
#24602=CARTESIAN_POINT('',(-0.393299835296684,2.10035993832925,12.3087163506447));
#24603=CARTESIAN_POINT('Ctrl Pts',(-0.392679023151022,2.09989376574539,
12.4337163522035));
#24604=CARTESIAN_POINT('Ctrl Pts',(-0.392504708819361,2.17213770239946,
12.430075519612));
#24605=CARTESIAN_POINT('Ctrl Pts',(-0.338763420378901,2.37604995535533,
12.4198112391793));
#24606=CARTESIAN_POINT('Ctrl Pts',(-0.0106856712490616,2.5649310055368,
12.4029235109061));
#24607=CARTESIAN_POINT('Ctrl Pts',(0.385137966833689,2.3606602577738,12.3830531673834));
#24608=CARTESIAN_POINT('Ctrl Pts',(0.427649952146105,1.91726920919309,12.3631828238606));
#24609=CARTESIAN_POINT('Ctrl Pts',(0.0778513256483007,1.64150878462692,
12.3433124803378));
#24610=CARTESIAN_POINT('Ctrl Pts',(-0.30701340218317,1.77385138595576,12.3251569897854));
#24611=CARTESIAN_POINT('Ctrl Pts',(-0.39232831653515,2.0032839961273,12.313624947074));
#24612=CARTESIAN_POINT('Ctrl Pts',(-0.393198689398899,2.10035981493551,
12.3087163522035));
#24613=CARTESIAN_POINT('',(-0.393299992424556,2.09992280645213,12.183716352199));
#24614=CARTESIAN_POINT('Ctrl Pts',(-0.393299835296684,2.10035993832925,
12.3087163506447));
#24615=CARTESIAN_POINT('Ctrl Pts',(-0.393275675193132,2.1267593628298,12.3073818069068));
#24616=CARTESIAN_POINT('Ctrl Pts',(-0.390589636175855,2.15303871333908,
12.306047263169));
#24617=CARTESIAN_POINT('Ctrl Pts',(-0.38533610283396,2.17874628786639,12.3047127194312));
#24618=CARTESIAN_POINT('Ctrl Pts',(-0.383838988541392,2.18607224827196,
12.3043324107182));
#24619=CARTESIAN_POINT('Ctrl Pts',(-0.382133660681373,2.19335192324089,
12.3039521020052));
#24620=CARTESIAN_POINT('Ctrl Pts',(-0.380222989607752,2.20057518667019,
12.3035717932922));
#24621=CARTESIAN_POINT('Ctrl Pts',(-0.374978120993316,2.22040333405629,
12.3025278306446));
#24622=CARTESIAN_POINT('Ctrl Pts',(-0.368162429928449,2.23987918613092,
12.3014838679971));
#24623=CARTESIAN_POINT('Ctrl Pts',(-0.359843140920602,2.25873816155038,
12.3004399053495));
#24624=CARTESIAN_POINT('Ctrl Pts',(-0.351539156141341,2.27756244385239,
12.2993978631838));
#24625=CARTESIAN_POINT('Ctrl Pts',(-0.341737303079051,2.29577141246672,
12.298355821018));
#24626=CARTESIAN_POINT('Ctrl Pts',(-0.330554033249778,2.313117153468,12.2973137788522));
#24627=CARTESIAN_POINT('Ctrl Pts',(-0.319382774076619,2.33044426541594,
12.2962728558234));
#24628=CARTESIAN_POINT('Ctrl Pts',(-0.306833415843539,2.34690935932156,
12.2952319327945));
#24629=CARTESIAN_POINT('Ctrl Pts',(-0.293067411788011,2.36229064441546,
12.2941910097657));
#24630=CARTESIAN_POINT('Ctrl Pts',(-0.27929433787158,2.3776798289365,12.2931495521459));
#24631=CARTESIAN_POINT('Ctrl Pts',(-0.264303848523121,2.39198353363584,
12.2921080945261));
#24632=CARTESIAN_POINT('Ctrl Pts',(-0.248296846725069,2.40501404214624,
12.2910666369062));
#24633=CARTESIAN_POINT('Ctrl Pts',(-0.232284954090124,2.41804853204507,
12.2900248610757));
#24634=CARTESIAN_POINT('Ctrl Pts',(-0.215256523671905,2.42980861525563,
12.2889830852452));
#24635=CARTESIAN_POINT('Ctrl Pts',(-0.197443749790202,2.44014828482411,
12.2879413094147));
#24636=CARTESIAN_POINT('Ctrl Pts',(-0.179592473193528,2.45051030382301,
12.2868972817621));
#24637=CARTESIAN_POINT('Ctrl Pts',(-0.160954132505601,2.45944546119213,
12.2858532541095));
#24638=CARTESIAN_POINT('Ctrl Pts',(-0.14178410779799,2.46685440814569,12.2848092264569));
#24639=CARTESIAN_POINT('Ctrl Pts',(-0.13500392133518,2.4694748555684,12.284439967561));
#24640=CARTESIAN_POINT('Ctrl Pts',(-0.128157372660572,2.47190483609913,
12.2840707086652));
#24641=CARTESIAN_POINT('Ctrl Pts',(-0.121256156779108,2.4741414631435,12.2837014497693));
#24642=CARTESIAN_POINT('Ctrl Pts',(-0.101745153296427,2.4804648181583,12.2826574871218));
#24643=CARTESIAN_POINT('Ctrl Pts',(-0.0816800514438771,2.48527669371452,
12.2816135244742));
#24644=CARTESIAN_POINT('Ctrl Pts',(-0.0613197057929595,2.4884903907196,
12.2805695618267));
#24645=CARTESIAN_POINT('Ctrl Pts',(-0.0409968151918136,2.49169817578274,
12.2795275196609));
#24646=CARTESIAN_POINT('Ctrl Pts',(-0.0203804681897151,2.49331344595796,
12.2784854774951));
#24647=CARTESIAN_POINT('Ctrl Pts',(0.000257847436364005,2.49329991547762,
12.2774434353294));
#24648=CARTESIAN_POINT('Ctrl Pts',(0.0208739978356784,2.4932863995288,12.2764025123005));
#24649=CARTESIAN_POINT('Ctrl Pts',(0.0415113379529104,2.4916475272744,12.2753615892717));
#24650=CARTESIAN_POINT('Ctrl Pts',(0.0618959845834157,2.48839899213624,
12.2743206662428));
#24651=CARTESIAN_POINT('Ctrl Pts',(0.0822911002371422,2.4851487886351,12.273279208623));
#24652=CARTESIAN_POINT('Ctrl Pts',(0.102432533992589,2.48028737060078,12.2722377510032));
#24653=CARTESIAN_POINT('Ctrl Pts',(0.122053698152773,2.47388204659656,12.2711962933835));
#24654=CARTESIAN_POINT('Ctrl Pts',(0.141680857434022,2.4674747654866,12.270154517553));
#24655=CARTESIAN_POINT('Ctrl Pts',(0.160786743024064,2.45952290184056,12.2691127417225));
#24656=CARTESIAN_POINT('Ctrl Pts',(0.179122898681202,2.45014265259754,12.268070965892));
#24657=CARTESIAN_POINT('Ctrl Pts',(0.197498688354888,2.44074212773292,12.2670269382394));
#24658=CARTESIAN_POINT('Ctrl Pts',(0.215100799237128,2.42990743930654,12.2659829105868));
#24659=CARTESIAN_POINT('Ctrl Pts',(0.231707455242898,2.41779953616212,12.2649388829342));
#24660=CARTESIAN_POINT('Ctrl Pts',(0.237581011796238,2.41351712952731,12.2645696240383));
#24661=CARTESIAN_POINT('Ctrl Pts',(0.243330343440933,2.40907582118649,12.2642003651425));
#24662=CARTESIAN_POINT('Ctrl Pts',(0.24894669235926,2.4044838819435,12.2638311062466));
#24663=CARTESIAN_POINT('Ctrl Pts',(0.264825141198124,2.39150162720805,12.262787143599));
#24664=CARTESIAN_POINT('Ctrl Pts',(0.279732654505629,2.37723528550078,12.2617431809515));
#24665=CARTESIAN_POINT('Ctrl Pts',(0.29345621147571,2.36185557459471,12.2606992183039));
#24666=CARTESIAN_POINT('Ctrl Pts',(0.307154522483946,2.3465041563241,12.2596571761382));
#24667=CARTESIAN_POINT('Ctrl Pts',(0.319672671713673,2.33004393757367,12.2586151339724));
#24668=CARTESIAN_POINT('Ctrl Pts',(0.330833188202641,2.31268354798544,12.2575730918066));
#24669=CARTESIAN_POINT('Ctrl Pts',(0.341981718472226,2.29534180318291,12.2565321687778));
#24670=CARTESIAN_POINT('Ctrl Pts',(0.351775090436263,2.27710240694963,12.2554912457489));
#24671=CARTESIAN_POINT('Ctrl Pts',(0.360078241477362,2.25820414032057,12.2544503227201));
#24672=CARTESIAN_POINT('Ctrl Pts',(0.368385656800428,2.23929616803432,12.2534088651003));
#24673=CARTESIAN_POINT('Ctrl Pts',(0.375201011500912,2.21972931649054,12.2523674074805));
#24674=CARTESIAN_POINT('Ctrl Pts',(0.380436591086625,2.19976417273945,12.2513259498607));
#24675=CARTESIAN_POINT('Ctrl Pts',(0.385673770370154,2.17979292876655,12.2502841740302));
#24676=CARTESIAN_POINT('Ctrl Pts',(0.389330062134675,2.15942387061067,12.2492423981997));
#24677=CARTESIAN_POINT('Ctrl Pts',(0.391368672994078,2.13892880423099,12.2482006223692));
#24678=CARTESIAN_POINT('Ctrl Pts',(0.393411690357115,2.11838943730023,12.2471565947166));
#24679=CARTESIAN_POINT('Ctrl Pts',(0.393830031010305,2.09772425469989,12.246112567064));
#24680=CARTESIAN_POINT('Ctrl Pts',(0.392638972221088,2.07720685425029,12.2450685394114));
#24681=CARTESIAN_POINT('Ctrl Pts',(0.392217710339444,2.06995011864823,12.2446992805155));
#24682=CARTESIAN_POINT('Ctrl Pts',(0.39159559587069,2.06271181720889,12.2443300216196));
#24683=CARTESIAN_POINT('Ctrl Pts',(0.390774842289819,2.05550379079779,12.2439607627238));
#24684=CARTESIAN_POINT('Ctrl Pts',(0.388454421330812,2.03512537765745,12.2429168000762));
#24685=CARTESIAN_POINT('Ctrl Pts',(0.384528732108304,2.01486824501606,12.2418728374286));
#24686=CARTESIAN_POINT('Ctrl Pts',(0.379026005171062,1.99500391719656,12.2408288747811));
#24687=CARTESIAN_POINT('Ctrl Pts',(0.373533401092972,1.97517613194859,12.2397868326153));
#24688=CARTESIAN_POINT('Ctrl Pts',(0.366469654824172,1.95574043411958,12.2387447904496));
#24689=CARTESIAN_POINT('Ctrl Pts',(0.357914117664509,1.93695897946702,12.2377027482838));
#24690=CARTESIAN_POINT('Ctrl Pts',(0.349367769017353,1.91819769580171,12.2366618252549));
#24691=CARTESIAN_POINT('Ctrl Pts',(0.339333087298376,1.90008993856399,12.2356209022261));
#24692=CARTESIAN_POINT('Ctrl Pts',(0.327937732041783,1.8828785273095,12.2345799791972));
#24693=CARTESIAN_POINT('Ctrl Pts',(0.316536524427733,1.86565827672278,12.2335385215774));
#24694=CARTESIAN_POINT('Ctrl Pts',(0.303773639962304,1.84933591417466,12.2324970639576));
#24695=CARTESIAN_POINT('Ctrl Pts',(0.289820703463437,1.83412625205944,12.2314556063378));
#24696=CARTESIAN_POINT('Ctrl Pts',(0.27586350373417,1.81891194272936,12.2304138305073));
#24697=CARTESIAN_POINT('Ctrl Pts',(0.260716051738381,1.80481152792479,12.2293720546768));
#24698=CARTESIAN_POINT('Ctrl Pts',(0.244586969868335,1.79200307766046,12.2283302788464));
#24699=CARTESIAN_POINT('Ctrl Pts',(0.22842302462181,1.77916694164022,12.2272862511938));
#24700=CARTESIAN_POINT('Ctrl Pts',(0.211273824448557,1.76762875659117,12.2262422235412));
#24701=CARTESIAN_POINT('Ctrl Pts',(0.19337768515542,1.75752378055706,12.2251981958886));
#24702=CARTESIAN_POINT('Ctrl Pts',(0.187048055265674,1.75394978298735,12.2248289369927));
#24703=CARTESIAN_POINT('Ctrl Pts',(0.180625200015419,1.7505546446144,12.2244596780968));
#24704=CARTESIAN_POINT('Ctrl Pts',(0.174120273610395,1.74734291398323,12.224090419201));
#24705=CARTESIAN_POINT('Ctrl Pts',(0.155729653186621,1.73826276222385,12.2230464565534));
#24706=CARTESIAN_POINT('Ctrl Pts',(0.136572046861426,1.73059800008724,12.2220024939059));
#24707=CARTESIAN_POINT('Ctrl Pts',(0.11689103885316,1.72447187184469,12.2209585312583));
#24708=CARTESIAN_POINT('Ctrl Pts',(0.0972462361798775,1.71835701327518,
12.2199164890925));
#24709=CARTESIAN_POINT('Ctrl Pts',(0.0770806199719689,1.71377544319439,
12.2188744469268));
#24710=CARTESIAN_POINT('Ctrl Pts',(0.0566575697764722,1.71080235125707,
12.217832404761));
#24711=CARTESIAN_POINT('Ctrl Pts',(0.0362564536160493,1.70783245237379,
12.2167914817321));
#24712=CARTESIAN_POINT('Ctrl Pts',(0.0155991725926806,1.70646773624871,
12.2157505587033));
#24713=CARTESIAN_POINT('Ctrl Pts',(-0.00504100185119109,1.70673230707273,
12.2147096356744));
#24714=CARTESIAN_POINT('Ctrl Pts',(-0.0256917765507166,1.70699701377344,
12.2136681780547));
#24715=CARTESIAN_POINT('Ctrl Pts',(-0.0463246911948396,1.70889268576987,
12.2126267204349));
#24716=CARTESIAN_POINT('Ctrl Pts',(-0.0666662240613439,1.71239129967272,
12.2115852628151));
#24717=CARTESIAN_POINT('Ctrl Pts',(-0.0870139721529581,1.71589098255464,
12.2105434869846));
#24718=CARTESIAN_POINT('Ctrl Pts',(-0.107069442842288,1.72099442208645,
12.2095017111541));
#24719=CARTESIAN_POINT('Ctrl Pts',(-0.126569980602219,1.72762259734195,
12.2084599353236));
#24720=CARTESIAN_POINT('Ctrl Pts',(-0.146112669217038,1.73426509954868,
12.207415907671));
#24721=CARTESIAN_POINT('Ctrl Pts',(-0.165097353710535,1.74243862605138,
12.2063718800184));
#24722=CARTESIAN_POINT('Ctrl Pts',(-0.183281302045478,1.75201601427578,
12.2053278523658));
#24723=CARTESIAN_POINT('Ctrl Pts',(-0.189712726220865,1.75540341095272,
12.2049585934699));
#24724=CARTESIAN_POINT('Ctrl Pts',(-0.196044226953382,1.75896601289691,
12.2045893345741));
#24725=CARTESIAN_POINT('Ctrl Pts',(-0.202265941771804,1.76269690366206,
12.2042200756782));
#24726=CARTESIAN_POINT('Ctrl Pts',(-0.219855871078453,1.77324481637183,
12.2031761130306));
#24727=CARTESIAN_POINT('Ctrl Pts',(-0.23667089877559,1.7852038005372,12.2021321503831));
#24728=CARTESIAN_POINT('Ctrl Pts',(-0.25247554233462,1.7984357605371,12.2010881877355));
#24729=CARTESIAN_POINT('Ctrl Pts',(-0.268251111548774,1.81164337892074,
12.2000461455698));
#24730=CARTESIAN_POINT('Ctrl Pts',(-0.283019390125813,1.82611890341287,
12.199004103404));
#24731=CARTESIAN_POINT('Ctrl Pts',(-0.296574585150023,1.84168158129337,
12.1979620612382));
#24732=CARTESIAN_POINT('Ctrl Pts',(-0.310115222107724,1.85722754510232,
12.1969211382094));
#24733=CARTESIAN_POINT('Ctrl Pts',(-0.322444859331438,1.87385781134533,
12.1958802151805));
#24734=CARTESIAN_POINT('Ctrl Pts',(-0.333395302816379,1.89135565653492,
12.1948392921517));
#24735=CARTESIAN_POINT('Ctrl Pts',(-0.344351370163691,1.90886248816175,
12.1937978345319));
#24736=CARTESIAN_POINT('Ctrl Pts',(-0.35392642471822,1.92723717371848,12.1927563769121));
#24737=CARTESIAN_POINT('Ctrl Pts',(-0.361995966796987,1.94623456167684,
12.1917149192923));
#24738=CARTESIAN_POINT('Ctrl Pts',(-0.37006797447266,1.96523775416543,12.1906731434618));
#24739=CARTESIAN_POINT('Ctrl Pts',(-0.376633299803859,1.98486333703376,
12.1896313676313));
#24740=CARTESIAN_POINT('Ctrl Pts',(-0.381616204817429,2.00484768935679,
12.1885895918008));
#24741=CARTESIAN_POINT('Ctrl Pts',(-0.386609880493262,2.02487523831087,
12.1875455641482));
#24742=CARTESIAN_POINT('Ctrl Pts',(-0.390014185815633,2.04526237852428,
12.1865015364956));
#24743=CARTESIAN_POINT('Ctrl Pts',(-0.391804646116096,2.06573618115503,
12.185457508843));
#24744=CARTESIAN_POINT('Ctrl Pts',(-0.392437908455446,2.07297749677984,
12.1850882499471));
#24745=CARTESIAN_POINT('Ctrl Pts',(-0.392869764704041,2.08022963676174,
12.1847189910513));
#24746=CARTESIAN_POINT('Ctrl Pts',(-0.39310069159986,2.08748056456099,12.1843497321554));
#24747=CARTESIAN_POINT('Ctrl Pts',(-0.393232725851723,2.09162633902301,
12.1841386055047));
#24748=CARTESIAN_POINT('Ctrl Pts',(-0.393299178173347,2.0957742132399,12.1839274788541));
#24749=CARTESIAN_POINT('Ctrl Pts',(-0.393299992424539,2.09992280636392,
12.1837163522035));
#24750=CARTESIAN_POINT('',(-0.393299871729038,2.09968235566726,12.0587163522076));
#24751=CARTESIAN_POINT('Ctrl Pts',(-0.393299992424556,2.09992280645214,
12.183716352199));
#24752=CARTESIAN_POINT('Ctrl Pts',(-0.393303997505547,2.12032863526799,
12.1826778762235));
#24753=CARTESIAN_POINT('Ctrl Pts',(-0.391715603864827,2.14079812773611,
12.1816394002479));
#24754=CARTESIAN_POINT('Ctrl Pts',(-0.388531187097256,2.1610606800879,12.1806009242724));
#24755=CARTESIAN_POINT('Ctrl Pts',(-0.385352552134374,2.18128644261952,
12.1795643338118));
#24756=CARTESIAN_POINT('Ctrl Pts',(-0.380583699187246,2.2013052743376,12.1785277433511));
#24757=CARTESIAN_POINT('Ctrl Pts',(-0.374272869640994,2.22084994435537,
12.1774911528905));
#24758=CARTESIAN_POINT('Ctrl Pts',(-0.367671498009194,2.24129442463527,
12.1764068392023));
#24759=CARTESIAN_POINT('Ctrl Pts',(-0.359382669624518,2.26121911750468,
12.1753225255142));
#24760=CARTESIAN_POINT('Ctrl Pts',(-0.349520709452778,2.28033347904265,
12.174238211826));
#24761=CARTESIAN_POINT('Ctrl Pts',(-0.340097295564756,2.29859785416087,
12.173202115909));
#24762=CARTESIAN_POINT('Ctrl Pts',(-0.329238279185668,2.31612184059859,
12.1721660199919));
#24763=CARTESIAN_POINT('Ctrl Pts',(-0.317090954891824,2.33267620489812,
12.1711299240749));
#24764=CARTESIAN_POINT('Ctrl Pts',(-0.304938571797175,2.34923746332753,
12.1700933966717));
#24765=CARTESIAN_POINT('Ctrl Pts',(-0.291497287948853,2.36482772302869,
12.1690568692684));
#24766=CARTESIAN_POINT('Ctrl Pts',(-0.276954855100894,2.37925060113819,
12.1680203418652));
#24767=CARTESIAN_POINT('Ctrl Pts',(-0.262382049761107,2.39370360204435,
12.1669816496302));
#24768=CARTESIAN_POINT('Ctrl Pts',(-0.246704081486891,2.40698388492101,
12.1659429573952));
#24769=CARTESIAN_POINT('Ctrl Pts',(-0.230142255229364,2.41893484030119,
12.1649042651603));
#24770=CARTESIAN_POINT('Ctrl Pts',(-0.227884053041853,2.42056435103042,
12.164762639651));
#24771=CARTESIAN_POINT('Ctrl Pts',(-0.225609459681919,2.42216921581425,
12.1646210141418));
#24772=CARTESIAN_POINT('Ctrl Pts',(-0.223319072711738,2.4237491031079,12.1644793886326));
#24773=CARTESIAN_POINT('Ctrl Pts',(-0.206435966987021,2.43539490993406,
12.1634354259851));
#24774=CARTESIAN_POINT('Ctrl Pts',(-0.18858913326125,2.44575121162367,12.1623914633375));
#24775=CARTESIAN_POINT('Ctrl Pts',(-0.17000175783156,2.45466081307945,12.16134750069));
#24776=CARTESIAN_POINT('Ctrl Pts',(-0.151448575881872,2.4635540243633,12.1603054585242));
#24777=CARTESIAN_POINT('Ctrl Pts',(-0.132158186645935,2.47100545003735,
12.1592634163584));
#24778=CARTESIAN_POINT('Ctrl Pts',(-0.112380317171347,2.4769025793391,12.1582213741927));
#24779=CARTESIAN_POINT('Ctrl Pts',(-0.0926236888178818,2.48279337521662,
12.1571804511638));
#24780=CARTESIAN_POINT('Ctrl Pts',(-0.0723813128532868,2.48713295177294,
12.156139528135));
#24781=CARTESIAN_POINT('Ctrl Pts',(-0.0519200964590137,2.48985791460952,
12.1550986051061));
#24782=CARTESIAN_POINT('Ctrl Pts',(-0.0314483717172843,2.492584276916,12.1540571474863));
#24783=CARTESIAN_POINT('Ctrl Pts',(-0.0107583092250953,2.49369425578895,
12.1530156898665));
#24784=CARTESIAN_POINT('Ctrl Pts',(0.00987539303740517,2.49317599953756,
12.1519742322468));
#24785=CARTESIAN_POINT('Ctrl Pts',(0.0305153997955036,2.49265758493628,
12.1509324564163));
#24786=CARTESIAN_POINT('Ctrl Pts',(0.0510982780238676,2.49050999944065,
12.1498906805858));
#24787=CARTESIAN_POINT('Ctrl Pts',(0.0713527019384991,2.48677342453441,
12.1488489047553));
#24788=CARTESIAN_POINT('Ctrl Pts',(0.0916509062500565,2.48302877293671,
12.1478048771027));
#24789=CARTESIAN_POINT('Ctrl Pts',(0.111618527372682,2.47768846512622,12.1467608494501));
#24790=CARTESIAN_POINT('Ctrl Pts',(0.130996986946167,2.47084320057273,12.1457168217975));
#24791=CARTESIAN_POINT('Ctrl Pts',(0.13785089408932,2.46842212022617,12.1453475629016));
#24792=CARTESIAN_POINT('Ctrl Pts',(0.144631282693188,2.46581321920853,12.1449783040057));
#24793=CARTESIAN_POINT('Ctrl Pts',(0.151327393242926,2.46302191401388,12.1446090451099));
#24794=CARTESIAN_POINT('Ctrl Pts',(0.170258526320522,2.45513038210031,12.1435650824623));
#24795=CARTESIAN_POINT('Ctrl Pts',(0.188627103771938,2.44573049799819,12.1425211198148));
#24796=CARTESIAN_POINT('Ctrl Pts',(0.206180138369548,2.43492482819569,12.1414771571672));
#24797=CARTESIAN_POINT('Ctrl Pts',(0.223700882268574,2.42413903658717,12.1404351150014));
#24798=CARTESIAN_POINT('Ctrl Pts',(0.240408410637133,2.41195292329113,12.1393930728357));
#24799=CARTESIAN_POINT('Ctrl Pts',(0.256072940648541,2.39851555917173,12.1383510306699));
#24800=CARTESIAN_POINT('Ctrl Pts',(0.271720647200798,2.38509262657029,12.1373101076411));
#24801=CARTESIAN_POINT('Ctrl Pts',(0.286327004732961,2.37042156563308,12.1362691846122));
#24802=CARTESIAN_POINT('Ctrl Pts',(0.29969422841969,2.35469248016368,12.1352282615833));
#24803=CARTESIAN_POINT('Ctrl Pts',(0.313068317164112,2.33895531664594,12.1341868039635));
#24804=CARTESIAN_POINT('Ctrl Pts',(0.325201511946711,2.32215959327964,12.1331453463438));
#24805=CARTESIAN_POINT('Ctrl Pts',(0.335935148673514,2.3045298655104,12.132103888724));
#24806=CARTESIAN_POINT('Ctrl Pts',(0.346672064994279,2.28689475109076,12.1310621128935));
#24807=CARTESIAN_POINT('Ctrl Pts',(0.356008220552377,2.26842577171939,12.130020337063));
#24808=CARTESIAN_POINT('Ctrl Pts',(0.363830527109338,2.24937281393661,12.1289785612325));
#24809=CARTESIAN_POINT('Ctrl Pts',(0.371669741759436,2.2302786727532,12.1279345335799));
#24810=CARTESIAN_POINT('Ctrl Pts',(0.377988349443145,2.21059873429428,12.1268905059273));
#24811=CARTESIAN_POINT('Ctrl Pts',(0.38272263875999,2.19059951313661,12.1258464782747));
#24812=CARTESIAN_POINT('Ctrl Pts',(0.384397094835468,2.18352605075797,12.1254772193788));
#24813=CARTESIAN_POINT('Ctrl Pts',(0.385873831014179,2.17641273336051,12.1251079604829));
#24814=CARTESIAN_POINT('Ctrl Pts',(0.387151577261523,2.16927153978305,12.1247387015871));
#24815=CARTESIAN_POINT('Ctrl Pts',(0.390764000334346,2.14908207532537,12.1236947389395));
#24816=CARTESIAN_POINT('Ctrl Pts',(0.392803652355737,2.12854911941653,12.122650776292));
#24817=CARTESIAN_POINT('Ctrl Pts',(0.393219826507829,2.10794090934042,12.1216068136444));
#24818=CARTESIAN_POINT('Ctrl Pts',(0.393635235062723,2.0873706102874,12.1205647714786));
#24819=CARTESIAN_POINT('Ctrl Pts',(0.39243301981034,2.06672605798086,12.1195227293129));
#24820=CARTESIAN_POINT('Ctrl Pts',(0.389614136606284,2.0462811526879,12.1184806871471));
#24821=CARTESIAN_POINT('Ctrl Pts',(0.386798280838503,2.02585820490205,12.1174397641182));
#24822=CARTESIAN_POINT('Ctrl Pts',(0.382369275378471,2.00563520759659,12.1163988410894));
#24823=CARTESIAN_POINT('Ctrl Pts',(0.376379898408236,1.98588136841775,12.1153579180605));
#24824=CARTESIAN_POINT('Ctrl Pts',(0.370387445450093,1.96611738418195,12.1143164604407));
#24825=CARTESIAN_POINT('Ctrl Pts',(0.362833218095359,1.94682374823372,12.1132750028209));
#24826=CARTESIAN_POINT('Ctrl Pts',(0.353820138842289,1.92825542410421,12.1122335452011));
#24827=CARTESIAN_POINT('Ctrl Pts',(0.344804305700569,1.90968142654217,12.1111917693707));
#24828=CARTESIAN_POINT('Ctrl Pts',(0.334329086866636,1.8918338275438,12.1101499935402));
#24829=CARTESIAN_POINT('Ctrl Pts',(0.322543374710771,1.87494298182419,12.1091082177097));
#24830=CARTESIAN_POINT('Ctrl Pts',(0.310732187470628,1.85801562615826,12.1080641900571));
#24831=CARTESIAN_POINT('Ctrl Pts',(0.297605319366354,1.84204972140527,12.1070201624045));
#24832=CARTESIAN_POINT('Ctrl Pts',(0.28335237249362,1.82724310640749,12.1059761347519));
#24833=CARTESIAN_POINT('Ctrl Pts',(0.278311292008886,1.82200620076427,12.105606875856));
#24834=CARTESIAN_POINT('Ctrl Pts',(0.273129671358055,1.81691396730848,12.1052376169601));
#24835=CARTESIAN_POINT('Ctrl Pts',(0.267816895070616,1.81197395826986,12.1048683580643));
#24836=CARTESIAN_POINT('Ctrl Pts',(0.25279670175634,1.79800764636061,12.1038243954167));
#24837=CARTESIAN_POINT('Ctrl Pts',(0.236636325291627,1.78517781038189,12.1027804327692));
#24838=CARTESIAN_POINT('Ctrl Pts',(0.219533855870652,1.77367228722255,12.1017364701216));
#24839=CARTESIAN_POINT('Ctrl Pts',(0.202462848285074,1.76218792971285,12.1006944279558));
#24840=CARTESIAN_POINT('Ctrl Pts',(0.184453758238992,1.75202350463506,12.0996523857901));
#24841=CARTESIAN_POINT('Ctrl Pts',(0.165737403402908,1.74332647545232,12.0986103436243));
#24842=CARTESIAN_POINT('Ctrl Pts',(0.147041149637887,1.7346387867423,12.0975694205954));
#24843=CARTESIAN_POINT('Ctrl Pts',(0.1276397907406,1.7274156999839,12.0965284975666));
#24844=CARTESIAN_POINT('Ctrl Pts',(0.107788251103555,1.72175856529984,12.0954875745377));
#24845=CARTESIAN_POINT('Ctrl Pts',(0.0879265162331535,1.71609852525885,
12.0944461169179));
#24846=CARTESIAN_POINT('Ctrl Pts',(0.0676148419238802,1.71200626111984,
12.0934046592982));
#24847=CARTESIAN_POINT('Ctrl Pts',(0.0471233198857042,1.70953325016981,
12.0923632016784));
#24848=CARTESIAN_POINT('Ctrl Pts',(0.0266255367941799,1.70705948360713,
12.0913214258479));
#24849=CARTESIAN_POINT('Ctrl Pts',(0.00594853077608295,1.70620600733156,
12.0902796500174));
#24850=CARTESIAN_POINT('Ctrl Pts',(-0.0146334136694206,1.70697232514188,
12.0892378741869));
#24851=CARTESIAN_POINT('Ctrl Pts',(-0.0352598464549025,1.70774029936554,
12.0881938465343));
#24852=CARTESIAN_POINT('Ctrl Pts',(-0.0557900759231901,1.7101349723677,
12.0871498188817));
#24853=CARTESIAN_POINT('Ctrl Pts',(-0.0759551205932514,1.71410401705166,
12.0861057912291));
#24854=CARTESIAN_POINT('Ctrl Pts',(-0.0830872325746495,1.71550781613113,
12.0857365323332));
#24855=CARTESIAN_POINT('Ctrl Pts',(-0.0901737785218994,1.71710809756765,
12.0853672734373));
#24856=CARTESIAN_POINT('Ctrl Pts',(-0.0972033283696397,1.71890105883922,
12.0849980145415));
#24857=CARTESIAN_POINT('Ctrl Pts',(-0.117077155519838,1.72397008931346,
12.0839540518939));
#24858=CARTESIAN_POINT('Ctrl Pts',(-0.136612615100873,1.73061300115087,
12.0829100892464));
#24859=CARTESIAN_POINT('Ctrl Pts',(-0.15554454069214,1.73876491607144,12.0818661265988));
#24860=CARTESIAN_POINT('Ctrl Pts',(-0.174441638966242,1.7469018346661,12.080824084433));
#24861=CARTESIAN_POINT('Ctrl Pts',(-0.192736715404961,1.75654201306439,
12.0797820422673));
#24862=CARTESIAN_POINT('Ctrl Pts',(-0.210180834312592,1.76757120027341,
12.0787400001015));
#24863=CARTESIAN_POINT('Ctrl Pts',(-0.227606218510548,1.77858854230862,
12.0776990770726));
#24864=CARTESIAN_POINT('Ctrl Pts',(-0.24418182531333,1.7909915648636,12.0766581540438));
#24865=CARTESIAN_POINT('Ctrl Pts',(-0.259684442543274,1.80462078559758,
12.0756172310149));
#24866=CARTESIAN_POINT('Ctrl Pts',(-0.275195021513392,1.81825700594412,
12.0745757733951));
#24867=CARTESIAN_POINT('Ctrl Pts',(-0.289630946783222,1.8331202088504,12.0735343157754));
#24868=CARTESIAN_POINT('Ctrl Pts',(-0.302802729805314,1.84901116195645,
12.0724928581556));
#24869=CARTESIAN_POINT('Ctrl Pts',(-0.315978537381359,1.86490697044146,
12.0714510823251));
#24870=CARTESIAN_POINT('Ctrl Pts',(-0.327888992482206,1.88183056518122,
12.0704093064946));
#24871=CARTESIAN_POINT('Ctrl Pts',(-0.338386037167328,1.89955105425522,
12.0693675306641));
#24872=CARTESIAN_POINT('Ctrl Pts',(-0.34890577145275,1.9173098465685,12.0683235030115));
#24873=CARTESIAN_POINT('Ctrl Pts',(-0.358005671686283,1.93586831085162,
12.0672794753589));
#24874=CARTESIAN_POINT('Ctrl Pts',(-0.365584130891856,1.95497195705642,
12.0662354477063));
#24875=CARTESIAN_POINT('Ctrl Pts',(-0.368264532576321,1.96172866631324,
12.0658661888104));
#24876=CARTESIAN_POINT('Ctrl Pts',(-0.370755062659463,1.96855342228281,
12.0654969299145));
#24877=CARTESIAN_POINT('Ctrl Pts',(-0.373052731068955,1.97543455598765,
12.0651276710187));
#24878=CARTESIAN_POINT('Ctrl Pts',(-0.380724672436183,1.99841074093475,
12.0638947112988));
#24879=CARTESIAN_POINT('Ctrl Pts',(-0.386280054004908,2.02212718864926,
12.062661751579));
#24880=CARTESIAN_POINT('Ctrl Pts',(-0.38960581650926,2.04622084286498,12.0614287918592));
#24881=CARTESIAN_POINT('Ctrl Pts',(-0.392044644516216,2.06388905537695,
12.0605246453087));
#24882=CARTESIAN_POINT('Ctrl Pts',(-0.393285396653957,2.08175965223396,
12.0596204987581));
#24883=CARTESIAN_POINT('Ctrl Pts',(-0.393299871729038,2.09968235566726,
12.0587163522076));
#24884=CARTESIAN_POINT('',(-0.393117616260674,2.10022922555168,11.9337163003311));
#24885=CARTESIAN_POINT('Ctrl Pts',(-0.393299871729104,2.09968235574893,
12.0587163522035));
#24886=CARTESIAN_POINT('Ctrl Pts',(-0.393316492993478,2.12026242645436,
12.0576781494565));
#24887=CARTESIAN_POINT('Ctrl Pts',(-0.391713458209966,2.14086461331921,
12.0566399467095));
#24888=CARTESIAN_POINT('Ctrl Pts',(-0.388506753042148,2.16121595250135,
12.0556017439626));
#24889=CARTESIAN_POINT('Ctrl Pts',(-0.385298042103967,2.18158002129561,
12.0545628918274));
#24890=CARTESIAN_POINT('Ctrl Pts',(-0.380483759796851,2.20169219674375,
12.0535240396923));
#24891=CARTESIAN_POINT('Ctrl Pts',(-0.374131492706927,2.22128691670946,
12.0524851875572));
#24892=CARTESIAN_POINT('Ctrl Pts',(-0.367776788637376,2.24088915398083,
12.0514459368775));
#24893=CARTESIAN_POINT('Ctrl Pts',(-0.359883191796895,2.2599728509145,12.0504066861978));
#24894=CARTESIAN_POINT('Ctrl Pts',(-0.350567110264477,2.27829074906123,
12.0493674355182));
#24895=CARTESIAN_POINT('Ctrl Pts',(-0.341230137865095,2.29664972421785,
12.0483258543686));
#24896=CARTESIAN_POINT('Ctrl Pts',(-0.330464703739848,2.31423884457759,
12.047284273219));
#24897=CARTESIAN_POINT('Ctrl Pts',(-0.318431833598604,2.33083772947902,
12.0462426920694));
#24898=CARTESIAN_POINT('Ctrl Pts',(-0.314637357620361,2.33607206420422,
12.0459142372116));
#24899=CARTESIAN_POINT('Ctrl Pts',(-0.310717146896181,2.34120817816899,
12.0455857823537));
#24900=CARTESIAN_POINT('Ctrl Pts',(-0.306677039555868,2.34623988996352,
12.0452573274959));
#24901=CARTESIAN_POINT('Ctrl Pts',(-0.293835941137391,2.36223270919443,
12.0442133648483));
#24902=CARTESIAN_POINT('Ctrl Pts',(-0.279702205837368,2.37726600508028,
12.0431694022008));
#24903=CARTESIAN_POINT('Ctrl Pts',(-0.264444657850618,2.39112525299992,
12.0421254395532));
#24904=CARTESIAN_POINT('Ctrl Pts',(-0.249215177767485,2.4049590053396,12.0410833973875));
#24905=CARTESIAN_POINT('Ctrl Pts',(-0.232866487148554,2.41762246365465,
12.0400413552217));
#24906=CARTESIAN_POINT('Ctrl Pts',(-0.215605635461306,2.42893631595998,
12.0389993130559));
#24907=CARTESIAN_POINT('Ctrl Pts',(-0.198363321657604,2.44023801736568,
12.0379583900271));
#24908=CARTESIAN_POINT('Ctrl Pts',(-0.180211388011673,2.45019256478358,
12.0369174669982));
#24909=CARTESIAN_POINT('Ctrl Pts',(-0.161387409842751,2.45866278583685,
12.0358765439693));
#24910=CARTESIAN_POINT('Ctrl Pts',(-0.14255376416926,2.46713735697488,12.0348350863495));
#24911=CARTESIAN_POINT('Ctrl Pts',(-0.123048048815827,2.47412576219931,
12.0337936287298));
#24912=CARTESIAN_POINT('Ctrl Pts',(-0.103130063658391,2.47953798224923,
12.03275217111));
#24913=CARTESIAN_POINT('Ctrl Pts',(-0.083205992688135,2.48495185596832,
12.0317103952795));
#24914=CARTESIAN_POINT('Ctrl Pts',(-0.062870120066094,2.48878842791809,
12.030668619449));
#24915=CARTESIAN_POINT('Ctrl Pts',(-0.042393915182467,2.49100849857196,
12.0296268436185));
#24916=CARTESIAN_POINT('Ctrl Pts',(-0.0218734505173167,2.49323336795894,
12.0285828159659));
#24917=CARTESIAN_POINT('Ctrl Pts',(-0.00121278417029519,2.49383473881415,
12.0275387883133));
#24918=CARTESIAN_POINT('Ctrl Pts',(0.0193143614497235,2.49282546435,12.0264947606607));
#24919=CARTESIAN_POINT('Ctrl Pts',(0.0265745437907052,2.49246849720135,
12.0261255017648));
#24920=CARTESIAN_POINT('Ctrl Pts',(0.0338180717901917,2.4919105220603,12.0257562428689));
#24921=CARTESIAN_POINT('Ctrl Pts',(0.0410330854408241,2.49115364743181,
12.0253869839731));
#24922=CARTESIAN_POINT('Ctrl Pts',(0.0614312527895902,2.48901382399119,
12.0243430213255));
#24923=CARTESIAN_POINT('Ctrl Pts',(0.0817223634306081,2.48526772099253,
12.023299058678));
#24924=CARTESIAN_POINT('Ctrl Pts',(0.101634653634368,2.4799411627879,12.0222550960304));
#24925=CARTESIAN_POINT('Ctrl Pts',(0.121510313034625,2.47462440336105,12.0212130538647));
#24926=CARTESIAN_POINT('Ctrl Pts',(0.141007817151458,2.46773309037553,12.0201710116989));
#24927=CARTESIAN_POINT('Ctrl Pts',(0.159864317639446,2.45934424991319,12.0191289695331));
#24928=CARTESIAN_POINT('Ctrl Pts',(0.178700566542123,2.45096441893373,12.0180880465043));
#24929=CARTESIAN_POINT('Ctrl Pts',(0.196896497908281,2.44109052450962,12.0170471234754));
#24930=CARTESIAN_POINT('Ctrl Pts',(0.214208170934481,2.42984807033679,12.0160062004466));
#24931=CARTESIAN_POINT('Ctrl Pts',(0.23152873478477,2.4185998423325,12.0149647428268));
#24932=CARTESIAN_POINT('Ctrl Pts',(0.247963507187296,2.40598203764596,12.013923285207));
#24933=CARTESIAN_POINT('Ctrl Pts',(0.263296163968612,2.39216437161196,12.0128818275872));
#24934=CARTESIAN_POINT('Ctrl Pts',(0.278633505545024,2.37834248367859,12.0118400517567));
#24935=CARTESIAN_POINT('Ctrl Pts',(0.292867539228064,2.36332052359557,12.0107982759262));
#24936=CARTESIAN_POINT('Ctrl Pts',(0.305818354067898,2.34730552827465,12.0097565000958));
#24937=CARTESIAN_POINT('Ctrl Pts',(0.318797162387892,2.33125591617792,12.0087124724432));
#24938=CARTESIAN_POINT('Ctrl Pts',(0.330486797778318,2.31420959090686,12.0076684447906));
#24939=CARTESIAN_POINT('Ctrl Pts',(0.340749896564524,2.29640366083978,12.006624417138));
#24940=CARTESIAN_POINT('Ctrl Pts',(0.344379820079021,2.29010593677082,12.0062551582421));
#24941=CARTESIAN_POINT('Ctrl Pts',(0.347831717178603,2.2837134067121,12.0058858993462));
#24942=CARTESIAN_POINT('Ctrl Pts',(0.351100940695715,2.277237184142,12.0055166404504));
#24943=CARTESIAN_POINT('Ctrl Pts',(0.360343635391998,2.25892771472598,12.0044726778028));
#24944=CARTESIAN_POINT('Ctrl Pts',(0.368177789746147,2.23983875235823,12.0034287151553));
#24945=CARTESIAN_POINT('Ctrl Pts',(0.374478006718493,2.22021278003667,12.0023847525077));
#24946=CARTESIAN_POINT('Ctrl Pts',(0.380766633762833,2.200622911806,12.001342710342));
#24947=CARTESIAN_POINT('Ctrl Pts',(0.385526645695877,2.18049866901658,12.0003006681762));
#24948=CARTESIAN_POINT('Ctrl Pts',(0.388680522867616,2.16010275487327,11.9992586260104));
#24949=CARTESIAN_POINT('Ctrl Pts',(0.391831012824818,2.13972874562135,11.9982177029816));
#24950=CARTESIAN_POINT('Ctrl Pts',(0.393378652035149,2.11908436328001,11.9971767799527));
#24951=CARTESIAN_POINT('Ctrl Pts',(0.393296916688583,2.09844265506273,11.9961358569238));
#24952=CARTESIAN_POINT('Ctrl Pts',(0.393215139364874,2.07779034580209,11.9950943993041));
#24953=CARTESIAN_POINT('Ctrl Pts',(0.391502302529403,2.05714144924551,11.9940529416843));
#24954=CARTESIAN_POINT('Ctrl Pts',(0.38818400569048,2.03676972460843,11.9930114840645));
#24955=CARTESIAN_POINT('Ctrl Pts',(0.384864694967206,2.01639177552135,11.991969708234));
#24956=CARTESIAN_POINT('Ctrl Pts',(0.379939101595768,1.99629188672652,11.9909279324035));
#24957=CARTESIAN_POINT('Ctrl Pts',(0.373483916870504,1.97673340339303,11.989886156573));
#24958=CARTESIAN_POINT('Ctrl Pts',(0.367014779116969,1.95713264395397,11.9888421289204));
#24959=CARTESIAN_POINT('Ctrl Pts',(0.359009734480259,1.93807630534519,11.9877981012678));
#24960=CARTESIAN_POINT('Ctrl Pts',(0.349593790491062,1.91980823645324,11.9867540736152));
#24961=CARTESIAN_POINT('Ctrl Pts',(0.346263494523937,1.91334705993946,11.9863848147193));
#24962=CARTESIAN_POINT('Ctrl Pts',(0.34275711506805,1.90698425102751,11.9860155558234));
#24963=CARTESIAN_POINT('Ctrl Pts',(0.339081480939228,1.90072973306572,11.9856462969276));
#24964=CARTESIAN_POINT('Ctrl Pts',(0.328689788878464,1.88304706325432,11.98460233428));
#24965=CARTESIAN_POINT('Ctrl Pts',(0.316880216849635,1.86612676576232,11.9835583716324));
#24966=CARTESIAN_POINT('Ctrl Pts',(0.303788769215543,1.85020553709398,11.9825144089849));
#24967=CARTESIAN_POINT('Ctrl Pts',(0.290721404710059,1.8343135972414,11.9814723668191));
#24968=CARTESIAN_POINT('Ctrl Pts',(0.276377261527864,1.81941767773911,11.9804303246534));
#24969=CARTESIAN_POINT('Ctrl Pts',(0.260935262439899,1.80572516448833,11.9793882824876));
#24970=CARTESIAN_POINT('Ctrl Pts',(0.245509847816362,1.79204735678167,11.9783473594587));
#24971=CARTESIAN_POINT('Ctrl Pts',(0.228989446587432,1.77957089684241,11.9773064364299));
#24972=CARTESIAN_POINT('Ctrl Pts',(0.211589283921301,1.76846589175521,11.976265513401));
#24973=CARTESIAN_POINT('Ctrl Pts',(0.194180184985127,1.75735518342682,11.9752240557812));
#24974=CARTESIAN_POINT('Ctrl Pts',(0.175891033526532,1.7476177464974,11.9741825981614));
#24975=CARTESIAN_POINT('Ctrl Pts',(0.156965868671762,1.73938024725187,11.9731411405417));
#24976=CARTESIAN_POINT('Ctrl Pts',(0.138034921354045,1.7311402310912,11.9720993647112));
#24977=CARTESIAN_POINT('Ctrl Pts',(0.118468262287423,1.72440132520103,11.9710575888807));
#24978=CARTESIAN_POINT('Ctrl Pts',(0.098528831188428,1.71924159966635,11.9700158130502));
#24979=CARTESIAN_POINT('Ctrl Pts',(0.0785463005566409,1.71407072126784,
11.9689717853976));
#24980=CARTESIAN_POINT('Ctrl Pts',(0.0581901145585439,1.71048596570866,
11.967927757745));
#24981=CARTESIAN_POINT('Ctrl Pts',(0.0377329745389964,1.70851422422719,
11.9668837300924));
#24982=CARTESIAN_POINT('Ctrl Pts',(0.0304975522612305,1.70781684511029,
11.9665144711965));
#24983=CARTESIAN_POINT('Ctrl Pts',(0.0232495220501961,1.70732076830367,
11.9661452123006));
#24984=CARTESIAN_POINT('Ctrl Pts',(0.0160009241962401,1.70702562370446,
11.9657759534048));
#24985=CARTESIAN_POINT('Ctrl Pts',(-0.00449219185696926,1.70619119577152,
11.9647319907572));
#24986=CARTESIAN_POINT('Ctrl Pts',(-0.0251118156604017,1.70696163261368,
11.9636880281097));
#24987=CARTESIAN_POINT('Ctrl Pts',(-0.0455853069363327,1.70935070742222,
11.9626440654621));
#24988=CARTESIAN_POINT('Ctrl Pts',(-0.0660211350189228,1.71173538727021,
11.9616020232963));
#24989=CARTESIAN_POINT('Ctrl Pts',(-0.0863106347254772,1.71573276930209,
11.9605599811306));
#24990=CARTESIAN_POINT('Ctrl Pts',(-0.106182578148309,1.72130467378408,
11.9595179389648));
#24991=CARTESIAN_POINT('Ctrl Pts',(-0.126033179416082,1.7268705941282,11.9584770159359));
#24992=CARTESIAN_POINT('Ctrl Pts',(-0.145466402006288,1.73400751006866,
11.9574360929071));
#24993=CARTESIAN_POINT('Ctrl Pts',(-0.164222711564067,1.74262653846915,
11.9563951698782));
#24994=CARTESIAN_POINT('Ctrl Pts',(-0.182988653873587,1.75124999337798,
11.9553537122584));
#24995=CARTESIAN_POINT('Ctrl Pts',(-0.201076313335196,1.76135678882616,
11.9543122546386));
#24996=CARTESIAN_POINT('Ctrl Pts',(-0.218247083880113,1.77281029909573,
11.9532707970188));
#24997=CARTESIAN_POINT('Ctrl Pts',(-0.235423100844017,1.78426730891201,
11.9522290211883));
#24998=CARTESIAN_POINT('Ctrl Pts',(-0.251681079672283,1.79707141466158,
11.9511872453578));
#24999=CARTESIAN_POINT('Ctrl Pts',(-0.266813043620092,1.81104379267061,
11.9501454695273));
#25000=CARTESIAN_POINT('Ctrl Pts',(-0.281977715651357,1.82504637229179,
11.9491014418747));
#25001=CARTESIAN_POINT('Ctrl Pts',(-0.296011013602061,1.84022172498738,
11.9480574142221));
#25002=CARTESIAN_POINT('Ctrl Pts',(-0.308742708672144,1.85635511529731,
11.9470133865695));
#25003=CARTESIAN_POINT('Ctrl Pts',(-0.313245742334435,1.86206128397733,
11.9466441276737));
#25004=CARTESIAN_POINT('Ctrl Pts',(-0.317586342312149,1.86788702221123,
11.9462748687778));
#25005=CARTESIAN_POINT('Ctrl Pts',(-0.321758302167676,1.87382200596394,
11.945905609882));
#25006=CARTESIAN_POINT('Ctrl Pts',(-0.333683180404073,1.890786205294,11.9448501425421));
#25007=CARTESIAN_POINT('Ctrl Pts',(-0.34429731941234,1.90874491298018,11.9437946752022));
#25008=CARTESIAN_POINT('Ctrl Pts',(-0.35343870890053,1.92747183113843,11.9427392078623));
#25009=CARTESIAN_POINT('Ctrl Pts',(-0.362561452952742,1.94616055252648,
11.9416858933295));
#25010=CARTESIAN_POINT('Ctrl Pts',(-0.370217046306243,1.96561376671549,
11.9406325787968));
#25011=CARTESIAN_POINT('Ctrl Pts',(-0.376287829472357,1.98557815160127,
11.9395792642641));
#25012=CARTESIAN_POINT('Ctrl Pts',(-0.382352060450643,2.00552098895421,
11.9385270865723));
#25013=CARTESIAN_POINT('Ctrl Pts',(-0.386834628806233,2.02597323466799,
11.9374749088804));
#25014=CARTESIAN_POINT('Ctrl Pts',(-0.389666644633754,2.0466633703739,11.9364227311886));
#25015=CARTESIAN_POINT('Ctrl Pts',(-0.392094785869053,2.06440287987213,
11.9355206048602));
#25016=CARTESIAN_POINT('Ctrl Pts',(-0.393310331065654,2.08231670296114,
11.9346184785319));
#25017=CARTESIAN_POINT('Ctrl Pts',(-0.393299933737381,2.10022830280689,
11.9337163522035));
#25018=CARTESIAN_POINT('',(-0.393476660747021,2.10021501587443,11.8087164144524));
#25019=CARTESIAN_POINT('Ctrl Pts',(-0.392787134589716,2.10023089818476,
11.9337162063036));
#25020=CARTESIAN_POINT('Ctrl Pts',(-0.393054107309642,2.15099946965231,
11.9311558929888));
#25021=CARTESIAN_POINT('Ctrl Pts',(-0.360302360717907,2.33277278484366,
11.9219721318331));
#25022=CARTESIAN_POINT('Ctrl Pts',(-0.0859611737152024,2.55704015151082,
11.9061649228363));
#25023=CARTESIAN_POINT('Ctrl Pts',(0.337755205860749,2.41968178614589,11.8862945793136));
#25024=CARTESIAN_POINT('Ctrl Pts',(0.4516271652787,1.98905890273745,11.8664242357908));
#25025=CARTESIAN_POINT('Ctrl Pts',(0.15119268404004,1.66020937280082,11.846553892268));
#25026=CARTESIAN_POINT('Ctrl Pts',(-0.273919395647392,1.7324260119291,11.8273179899681));
#25027=CARTESIAN_POINT('Ctrl Pts',(-0.393020217355167,1.98223813255993,
11.8147055355092));
#25028=CARTESIAN_POINT('Ctrl Pts',(-0.393801543951838,2.10021294015016,
11.8087165288911));
#25029=CARTESIAN_POINT('',(-0.393301967689671,2.09965328553757,11.6837163511551));
#25030=CARTESIAN_POINT('Ctrl Pts',(-0.393299940606853,2.10021614496415,
11.8087163522035));
#25031=CARTESIAN_POINT('Ctrl Pts',(-0.393293081754006,2.11269659496315,
11.8080819698765));
#25032=CARTESIAN_POINT('Ctrl Pts',(-0.392692218482795,2.12516040435568,
11.8074475875494));
#25033=CARTESIAN_POINT('Ctrl Pts',(-0.391501762296877,2.1375667421856,11.8068132052223));
#25034=CARTESIAN_POINT('Ctrl Pts',(-0.389542704267171,2.15798306328373,
11.8057692425746));
#25035=CARTESIAN_POINT('Ctrl Pts',(-0.385976481415077,2.17830655986508,
11.804725279927));
#25036=CARTESIAN_POINT('Ctrl Pts',(-0.380826509869729,2.19826525011641,
11.8036813172794));
#25037=CARTESIAN_POINT('Ctrl Pts',(-0.37568601225198,2.21818722420636,11.8026392751136));
#25038=CARTESIAN_POINT('Ctrl Pts',(-0.368967673248511,2.23774500481882,
11.8015972329478));
#25039=CARTESIAN_POINT('Ctrl Pts',(-0.360746187679668,2.25667507164379,
11.8005551907821));
#25040=CARTESIAN_POINT('Ctrl Pts',(-0.352533531857171,2.27558480787437,
11.7995142677532));
#25041=CARTESIAN_POINT('Ctrl Pts',(-0.342821199442785,2.2938674856994,11.7984733447244));
#25042=CARTESIAN_POINT('Ctrl Pts',(-0.331732528447031,2.31127806220746,
11.7974324216956));
#25043=CARTESIAN_POINT('Ctrl Pts',(-0.320638162598855,2.32869758033385,
11.7963909640758));
#25044=CARTESIAN_POINT('Ctrl Pts',(-0.308166427695835,2.34524347310334,
11.7953495064561));
#25045=CARTESIAN_POINT('Ctrl Pts',(-0.294485116273548,2.36069792153632,
11.7943080488364));
#25046=CARTESIAN_POINT('Ctrl Pts',(-0.280799624614169,2.37615709197704,
11.7932662730059));
#25047=CARTESIAN_POINT('Ctrl Pts',(-0.265904335080789,2.3905236277231,11.7922244971755));
#25048=CARTESIAN_POINT('Ctrl Pts',(-0.250004682860337,2.40361579100551,
11.7911827213451));
#25049=CARTESIAN_POINT('Ctrl Pts',(-0.234070663180799,2.41673625329596,
11.7901386936925));
#25050=CARTESIAN_POINT('Ctrl Pts',(-0.217128550282337,2.42857642184816,
11.78909466604));
#25051=CARTESIAN_POINT('Ctrl Pts',(-0.19941422651103,2.43899683813423,11.7880506383874));
#25052=CARTESIAN_POINT('Ctrl Pts',(-0.193148902388196,2.44268240278632,
11.7876813794916));
#25053=CARTESIAN_POINT('Ctrl Pts',(-0.186787199084921,2.44619078777344,
11.7873121205957));
#25054=CARTESIAN_POINT('Ctrl Pts',(-0.180340188480231,2.44951724767015,
11.7869428616999));
#25055=CARTESIAN_POINT('Ctrl Pts',(-0.162113306649872,2.45892176011297,
11.7858988990524));
#25056=CARTESIAN_POINT('Ctrl Pts',(-0.143094485977205,2.46692469200966,
11.7848549364048));
#25057=CARTESIAN_POINT('Ctrl Pts',(-0.123525089214268,2.47339850339096,
11.7838109737573));
#25058=CARTESIAN_POINT('Ctrl Pts',(-0.103991692465394,2.47986040549863,
11.7827689315915));
#25059=CARTESIAN_POINT('Ctrl Pts',(-0.0839104020611678,2.48479848580899,
11.7817268894257));
#25060=CARTESIAN_POINT('Ctrl Pts',(-0.0635432242523246,2.48813290075903,
11.78068484726));
#25061=CARTESIAN_POINT('Ctrl Pts',(-0.0431979204724972,2.4914637345998,
11.7796439242311));
#25062=CARTESIAN_POINT('Ctrl Pts',(-0.0225680565905233,2.49319417546617,
11.7786030012022));
#25063=CARTESIAN_POINT('Ctrl Pts',(-0.00192643416733575,2.49329528201009,
11.7775620781733));
#25064=CARTESIAN_POINT('Ctrl Pts',(0.0187257892551426,2.4933964404797,11.7765206205535));
#25065=CARTESIAN_POINT('Ctrl Pts',(0.0393890475926803,2.49186657319596,
11.7754791629337));
#25066=CARTESIAN_POINT('Ctrl Pts',(0.059789365615982,2.48872885377759,11.7744377053139));
#25067=CARTESIAN_POINT('Ctrl Pts',(0.0801959168258219,2.48559017564915,
11.7733959294833));
#25068=CARTESIAN_POINT('Ctrl Pts',(0.100338646670289,2.48084281490468,11.7723541536528));
#25069=CARTESIAN_POINT('Ctrl Pts',(0.11995354100067,2.47456112718941,11.7713123778223));
#25070=CARTESIAN_POINT('Ctrl Pts',(0.139610833370268,2.46826586146359,11.7702683501696));
#25071=CARTESIAN_POINT('Ctrl Pts',(0.158737330916367,2.46042992677606,11.769224322517));
#25072=CARTESIAN_POINT('Ctrl Pts',(0.177088087035754,2.45117616580574,11.7681802948644));
#25073=CARTESIAN_POINT('Ctrl Pts',(0.183578508937987,2.44790323184655,11.7678110359685));
#25074=CARTESIAN_POINT('Ctrl Pts',(0.189972126797455,2.44445334999276,11.7674417770726));
#25075=CARTESIAN_POINT('Ctrl Pts',(0.196258957167312,2.44083326089394,11.7670725181768));
#25076=CARTESIAN_POINT('Ctrl Pts',(0.214032980084853,2.43059860482395,11.7660285555292));
#25077=CARTESIAN_POINT('Ctrl Pts',(0.231057219789549,2.41893937152159,11.7649845928816));
#25078=CARTESIAN_POINT('Ctrl Pts',(0.247093784372878,2.40598946342038,11.7639406302341));
#25079=CARTESIAN_POINT('Ctrl Pts',(0.263100847967622,2.39306337807054,11.7628985880683));
#25080=CARTESIAN_POINT('Ctrl Pts',(0.278123239647553,2.37885174165299,11.7618565459025));
#25081=CARTESIAN_POINT('Ctrl Pts',(0.291951996797666,2.36353163295107,11.7608145037368));
#25082=CARTESIAN_POINT('Ctrl Pts',(0.305765902079843,2.34822797780522,11.7597735807079));
#25083=CARTESIAN_POINT('Ctrl Pts',(0.318388205820068,2.33181873779631,11.7587326576791));
#25084=CARTESIAN_POINT('Ctrl Pts',(0.329646901200572,2.31451762288647,11.7576917346502));
#25085=CARTESIAN_POINT('Ctrl Pts',(0.340911378753586,2.29720762257493,11.7566502770305));
#25086=CARTESIAN_POINT('Ctrl Pts',(0.350810434049579,2.27900544019819,11.7556088194107));
#25087=CARTESIAN_POINT('Ctrl Pts',(0.359215244140055,2.26015398333292,11.7545673617909));
#25088=CARTESIAN_POINT('Ctrl Pts',(0.367622622266434,2.24129676652572,11.7535255859604));
#25089=CARTESIAN_POINT('Ctrl Pts',(0.374534579974763,2.22179056647898,11.75248381013));
#25090=CARTESIAN_POINT('Ctrl Pts',(0.379870721193706,2.20189762107024,11.7514420342995));
#25091=CARTESIAN_POINT('Ctrl Pts',(0.385218396602986,2.18196167660856,11.7503980066469));
#25092=CARTESIAN_POINT('Ctrl Pts',(0.388983321135715,2.16163804199095,11.7493539789943));
#25093=CARTESIAN_POINT('Ctrl Pts',(0.391136189093529,2.14119916966871,11.7483099513417));
#25094=CARTESIAN_POINT('Ctrl Pts',(0.391897630270952,2.13397020843597,11.7479406924459));
#25095=CARTESIAN_POINT('Ctrl Pts',(0.392457888712955,2.126726856683,11.74757143355));
#25096=CARTESIAN_POINT('Ctrl Pts',(0.392817227858228,2.11948115750609,11.7472021746541));
#25097=CARTESIAN_POINT('Ctrl Pts',(0.393833145550843,2.09899623654488,11.7461582120066));
#25098=CARTESIAN_POINT('Ctrl Pts',(0.393245381999473,2.07837059733709,11.745114249359));
#25099=CARTESIAN_POINT('Ctrl Pts',(0.391037749579127,2.05787674746542,11.7440702867115));
#25100=CARTESIAN_POINT('Ctrl Pts',(0.388834178336504,2.03742059823893,11.7430282445457));
#25101=CARTESIAN_POINT('Ctrl Pts',(0.385016672039765,2.01709648676696,11.7419862023799));
#25102=CARTESIAN_POINT('Ctrl Pts',(0.379621006461212,1.99717596850261,11.7409441602142));
#25103=CARTESIAN_POINT('Ctrl Pts',(0.374231135742727,1.97727684456193,11.7399032371853));
#25104=CARTESIAN_POINT('Ctrl Pts',(0.367266634031029,1.95778116746959,11.7388623141564));
#25105=CARTESIAN_POINT('Ctrl Pts',(0.358814082090202,1.93894924870164,11.7378213911276));
#25106=CARTESIAN_POINT('Ctrl Pts',(0.350357189138998,1.92010765835103,11.7367799335078));
#25107=CARTESIAN_POINT('Ctrl Pts',(0.340411005794053,1.90193118520857,11.735738475888));
#25108=CARTESIAN_POINT('Ctrl Pts',(0.329110038905254,1.88465963617616,11.7346970182682));
#25109=CARTESIAN_POINT('Ctrl Pts',(0.317805619078393,1.86738280993256,11.7336552424377));
#25110=CARTESIAN_POINT('Ctrl Pts',(0.305146024431257,1.85101205359708,11.7326134666072));
#25111=CARTESIAN_POINT('Ctrl Pts',(0.291308229420404,1.83575691972741,11.7315716907767));
#25112=CARTESIAN_POINT('Ctrl Pts',(0.277440523701614,1.82046881153968,11.730527663124));
#25113=CARTESIAN_POINT('Ctrl Pts',(0.26239006951038,1.80630164494062,11.7294836354714));
#25114=CARTESIAN_POINT('Ctrl Pts',(0.246370086041824,1.7934275441209,11.7284396078188));
#25115=CARTESIAN_POINT('Ctrl Pts',(0.240704027875007,1.78887414341152,11.728070348923));
#25116=CARTESIAN_POINT('Ctrl Pts',(0.234916966051311,1.78448211089951,11.7277010900271));
#25117=CARTESIAN_POINT('Ctrl Pts',(0.229019169225829,1.78025774422652,11.7273318311312));
#25118=CARTESIAN_POINT('Ctrl Pts',(0.212345015515231,1.76831468458585,11.7262878684837));
#25119=CARTESIAN_POINT('Ctrl Pts',(0.19468444174938,1.75764385551856,11.7252439058361));
#25120=CARTESIAN_POINT('Ctrl Pts',(0.176257814528997,1.74840638114798,11.7241999431886));
#25121=CARTESIAN_POINT('Ctrl Pts',(0.157865085074963,1.73918590010689,11.7231579010228));
#25122=CARTESIAN_POINT('Ctrl Pts',(0.138709723122247,1.73139391897812,11.722115858857));
#25123=CARTESIAN_POINT('Ctrl Pts',(0.1190394234298,1.72514735472522,11.7210738166913));
#25124=CARTESIAN_POINT('Ctrl Pts',(0.0993902493302116,1.71890749918419,
11.7200328936624));
#25125=CARTESIAN_POINT('Ctrl Pts',(0.0792279243557716,1.71421001464389,
11.7189919706336));
#25126=CARTESIAN_POINT('Ctrl Pts',(0.0588181907882767,1.7111230137532,11.7179510476047));
#25127=CARTESIAN_POINT('Ctrl Pts',(0.0383979753135636,1.70803442745931,
11.7169095899849));
#25128=CARTESIAN_POINT('Ctrl Pts',(0.0177308224960689,1.70655810315599,
11.7158681323651));
#25129=CARTESIAN_POINT('Ctrl Pts',(-0.00290882273925296,1.70671075688462,
11.7148266747453));
#25130=CARTESIAN_POINT('Ctrl Pts',(-0.02355477428601,1.70686345725561,11.7137848989148));
#25131=CARTESIAN_POINT('Ctrl Pts',(-0.0441724666480545,1.70864608489199,
11.7127431230843));
#25132=CARTESIAN_POINT('Ctrl Pts',(-0.0644899048119323,1.71202327108788,
11.7117013472538));
#25133=CARTESIAN_POINT('Ctrl Pts',(-0.0848512595794584,1.71540775714838,
11.7106573196013));
#25134=CARTESIAN_POINT('Ctrl Pts',(-0.104910349708517,1.72039350523695,
11.7096132919487));
#25135=CARTESIAN_POINT('Ctrl Pts',(-0.12440703069485,1.72689441077131,11.7085692642961));
#25136=CARTESIAN_POINT('Ctrl Pts',(-0.131302751201956,1.72919369584652,
11.7082000054002));
#25137=CARTESIAN_POINT('Ctrl Pts',(-0.138128291905378,1.7316820744839,11.7078307465043));
#25138=CARTESIAN_POINT('Ctrl Pts',(-0.144872799026719,1.73435432164161,
11.7074614876085));
#25139=CARTESIAN_POINT('Ctrl Pts',(-0.163940758092109,1.74190925464105,
11.7064175249609));
#25140=CARTESIAN_POINT('Ctrl Pts',(-0.182472969912289,1.7509822686813,11.7053735623134));
#25141=CARTESIAN_POINT('Ctrl Pts',(-0.200214670016784,1.76147529497824,
11.7043295996658));
#25142=CARTESIAN_POINT('Ctrl Pts',(-0.217923732352159,1.77194901822262,
11.7032875575001));
#25143=CARTESIAN_POINT('Ctrl Pts',(-0.234844513136281,1.78383724934025,
11.7022455153343));
#25144=CARTESIAN_POINT('Ctrl Pts',(-0.25074462484429,1.7969950114079,11.7012034731685));
#25145=CARTESIAN_POINT('Ctrl Pts',(-0.266627660082109,1.8101386422458,11.7001625501397));
#25146=CARTESIAN_POINT('Ctrl Pts',(-0.281491620007923,1.82454865281849,
11.6991216271108));
#25147=CARTESIAN_POINT('Ctrl Pts',(-0.29513538318823,1.84003847286505,11.6980807040819));
#25148=CARTESIAN_POINT('Ctrl Pts',(-0.308786153449707,1.85553624807947,
11.6970392464622));
#25149=CARTESIAN_POINT('Ctrl Pts',(-0.321214976608486,1.87211439918018,
11.6959977888424));
#25150=CARTESIAN_POINT('Ctrl Pts',(-0.332259235520891,1.88955121665576,
11.6949563312226));
#25151=CARTESIAN_POINT('Ctrl Pts',(-0.343306868935889,1.90699336183926,
11.6939145553921));
#25152=CARTESIAN_POINT('Ctrl Pts',(-0.352968733116018,1.92529405527396,
11.6928727795616));
#25153=CARTESIAN_POINT('Ctrl Pts',(-0.361127330886994,1.94420545296309,
11.6918310037311));
#25154=CARTESIAN_POINT('Ctrl Pts',(-0.369303563652189,1.96315772806747,
11.6907869760785));
#25155=CARTESIAN_POINT('Ctrl Pts',(-0.375969805324185,1.98272264572074,
11.6897429484259));
#25156=CARTESIAN_POINT('Ctrl Pts',(-0.381057633256767,2.00263486179976,
11.6886989207733));
#25157=CARTESIAN_POINT('Ctrl Pts',(-0.382857131306516,2.00967755162245,
11.6883296618774));
#25158=CARTESIAN_POINT('Ctrl Pts',(-0.384459646507782,2.01676359277159,
11.6879604029816));
#25159=CARTESIAN_POINT('Ctrl Pts',(-0.385863696822932,2.02388103078641,
11.6875911440857));
#25160=CARTESIAN_POINT('Ctrl Pts',(-0.390774797430378,2.04877647347876,
11.6862995467917));
#25161=CARTESIAN_POINT('Ctrl Pts',(-0.393277374005961,2.07416195048142,
11.6850079494976));
#25162=CARTESIAN_POINT('Ctrl Pts',(-0.393299847159929,2.09965326670688,
11.6837163522035));
#25163=CARTESIAN_POINT('',(-0.393051472227529,2.09996900767188,11.5587163606577));
#25164=CARTESIAN_POINT('Ctrl Pts',(-0.393452248457544,2.09965462005821,
11.6837162768534));
#25165=CARTESIAN_POINT('Ctrl Pts',(-0.392482851514261,2.20492670250052,
11.6783844514232));
#25166=CARTESIAN_POINT('Ctrl Pts',(-0.294736079347038,2.44255991631743,
11.6664291781522));
#25167=CARTESIAN_POINT('Ctrl Pts',(0.106936353373341,2.55259213405307,11.64785045704));
#25168=CARTESIAN_POINT('Ctrl Pts',(0.438434149993482,2.25508229943799,11.6279801135175));
#25169=CARTESIAN_POINT('Ctrl Pts',(0.367728301414394,1.81530556763727,11.6081097699945));
#25170=CARTESIAN_POINT('Ctrl Pts',(-0.0403182020246674,1.63669721988207,
11.5882394264718));
#25171=CARTESIAN_POINT('Ctrl Pts',(-0.347776659907118,1.84087036089522,
11.5717749611909));
#25172=CARTESIAN_POINT('Ctrl Pts',(-0.392699212427442,2.03611368051729,
11.561933943751));
#25173=CARTESIAN_POINT('Ctrl Pts',(-0.392654779593065,2.09996877097556,
11.5587163741521));
#25174=CARTESIAN_POINT('',(-0.393299835490125,2.10035972689682,11.4337163522035));
#25175=CARTESIAN_POINT('Ctrl Pts',(-0.393299998790548,2.0999691559613,11.5587163522035));
#25176=CARTESIAN_POINT('Ctrl Pts',(-0.393301690756094,2.12154382889946,
11.5576310176873));
#25177=CARTESIAN_POINT('Ctrl Pts',(-0.391523838488396,2.14308824023429,
11.5565456831711));
#25178=CARTESIAN_POINT('Ctrl Pts',(-0.388007014089908,2.16430744138149,
11.5554603486549));
#25179=CARTESIAN_POINT('Ctrl Pts',(-0.384483973544393,2.18556414843151,
11.5543730957606));
#25180=CARTESIAN_POINT('Ctrl Pts',(-0.379216005892341,2.20649387877415,
11.5532858428664));
#25181=CARTESIAN_POINT('Ctrl Pts',(-0.37229422929348,2.22681441887567,11.5521985899721));
#25182=CARTESIAN_POINT('Ctrl Pts',(-0.365349330818397,2.24720283880635,
11.5511077051595));
#25183=CARTESIAN_POINT('Ctrl Pts',(-0.356739858367749,2.26697741933563,
11.550016820347));
#25184=CARTESIAN_POINT('Ctrl Pts',(-0.346604715814774,2.2858764669746,11.5489259355344));
#25185=CARTESIAN_POINT('Ctrl Pts',(-0.345281724482195,2.28834345508944,
11.5487835368316));
#25186=CARTESIAN_POINT('Ctrl Pts',(-0.343932797815208,2.29079556406499,
11.5486411381289));
#25187=CARTESIAN_POINT('Ctrl Pts',(-0.342558298755806,2.29323224874106,
11.5484987394261));
#25188=CARTESIAN_POINT('Ctrl Pts',(-0.332481481697149,2.31109623019849,
11.5474547767786));
#25189=CARTESIAN_POINT('Ctrl Pts',(-0.320973501915486,2.3282230763783,11.546410814131));
#25190=CARTESIAN_POINT('Ctrl Pts',(-0.308166149408896,2.34437371863295,
11.5453668514835));
#25191=CARTESIAN_POINT('Ctrl Pts',(-0.295382357407313,2.36049465004083,
11.5443248093177));
#25192=CARTESIAN_POINT('Ctrl Pts',(-0.281304342812541,2.37564233522766,
11.5432827671519));
#25193=CARTESIAN_POINT('Ctrl Pts',(-0.266107326526554,2.38960625126003,
11.5422407249862));
#25194=CARTESIAN_POINT('Ctrl Pts',(-0.25092663159731,2.40355517026596,11.5411998019573));
#25195=CARTESIAN_POINT('Ctrl Pts',(-0.234629840292544,2.41632232744953,
11.5401588789284));
#25196=CARTESIAN_POINT('Ctrl Pts',(-0.217429130600451,2.42773382975569,
11.5391179558996));
#25197=CARTESIAN_POINT('Ctrl Pts',(-0.200219587072171,2.43915119271201,
11.5380764982798));
#25198=CARTESIAN_POINT('Ctrl Pts',(-0.182105801937319,2.44921108968555,
11.53703504066));
#25199=CARTESIAN_POINT('Ctrl Pts',(-0.163329532164277,2.4577825511718,11.5359935830402));
#25200=CARTESIAN_POINT('Ctrl Pts',(-0.144547525422253,2.46635663161321,
11.5349518072097));
#25201=CARTESIAN_POINT('Ctrl Pts',(-0.125103314869879,2.4734410988211,11.5339100313793));
#25202=CARTESIAN_POINT('Ctrl Pts',(-0.105258415970256,2.47895323704572,
11.5328682555488));
#25203=CARTESIAN_POINT('Ctrl Pts',(-0.0853706218713133,2.48447728988221,
11.5318242278962));
#25204=CARTESIAN_POINT('Ctrl Pts',(-0.06508113324532,2.48842208798903,11.5307802002436));
#25205=CARTESIAN_POINT('Ctrl Pts',(-0.044662132273192,2.49075591350716,
11.529736172591));
#25206=CARTESIAN_POINT('Ctrl Pts',(-0.0374401992765492,2.49158135700171,
11.5293669136951));
#25207=CARTESIAN_POINT('Ctrl Pts',(-0.0302020943018215,2.49220575312069,
11.5289976547992));
#25208=CARTESIAN_POINT('Ctrl Pts',(-0.0229598623062941,2.49262925861794,
11.5286283959034));
#25209=CARTESIAN_POINT('Ctrl Pts',(-0.00248474370291479,2.49382658636039,
11.5275844332558));
#25210=CARTESIAN_POINT('Ctrl Pts',(0.0181452926025266,2.49342154221628,
11.5265404706083));
#25211=CARTESIAN_POINT('Ctrl Pts',(0.0386578931035386,2.491395525397,11.5254965079607));
#25212=CARTESIAN_POINT('Ctrl Pts',(0.0591327584655686,2.48937323565398,
11.524454465795));
#25213=CARTESIAN_POINT('Ctrl Pts',(0.0794898870543711,2.48573590461745,
11.5234124236292));
#25214=CARTESIAN_POINT('Ctrl Pts',(0.0994574171779764,2.48051690129124,
11.5223703814634));
#25215=CARTESIAN_POINT('Ctrl Pts',(0.119403502487916,2.47530350309261,11.5213294584346));
#25216=CARTESIAN_POINT('Ctrl Pts',(0.138960104433556,2.46851196205091,11.5202885354057));
#25217=CARTESIAN_POINT('Ctrl Pts',(0.157866154841925,2.46022654976476,11.5192476123768));
#25218=CARTESIAN_POINT('Ctrl Pts',(0.176781914905033,2.45193688230681,11.518206154757));
#25219=CARTESIAN_POINT('Ctrl Pts',(0.195045775585474,2.44215209145183,11.5171646971373));
#25220=CARTESIAN_POINT('Ctrl Pts',(0.212416747963671,2.43100455462809,11.5161232395175));
#25221=CARTESIAN_POINT('Ctrl Pts',(0.229793027931236,2.41985361174585,11.515081463687));
#25222=CARTESIAN_POINT('Ctrl Pts',(0.246275277309255,2.40733952148462,11.5140396878565));
#25223=CARTESIAN_POINT('Ctrl Pts',(0.2616523841689,2.39363739519811,11.512997912026));
#25224=CARTESIAN_POINT('Ctrl Pts',(0.277062728993971,2.37990565145469,11.5119538843733));
#25225=CARTESIAN_POINT('Ctrl Pts',(0.291362652672405,2.36498127664035,11.5109098567208));
#25226=CARTESIAN_POINT('Ctrl Pts',(0.304378149127902,2.34907595695585,11.5098658290682));
#25227=CARTESIAN_POINT('Ctrl Pts',(0.308981559620264,2.34345045386649,11.5094965701723));
#25228=CARTESIAN_POINT('Ctrl Pts',(0.313424680063558,2.33770252251131,11.5091273112764));
#25229=CARTESIAN_POINT('Ctrl Pts',(0.317701122106218,2.33184237535975,11.5087580523806));
#25230=CARTESIAN_POINT('Ctrl Pts',(0.329791408371408,2.31527466418496,11.507714089733));
#25231=CARTESIAN_POINT('Ctrl Pts',(0.340618251416212,2.29770930257737,11.5066701270854));
#25232=CARTESIAN_POINT('Ctrl Pts',(0.350018581490352,2.27936522129856,11.5056261644379));
#25233=CARTESIAN_POINT('Ctrl Pts',(0.359401618644376,2.26105488593396,11.5045841222721));
#25234=CARTESIAN_POINT('Ctrl Pts',(0.367362967119777,2.24196929472217,11.5035420801064));
#25235=CARTESIAN_POINT('Ctrl Pts',(0.373783520526344,2.22235509708603,11.5025000379406));
#25236=CARTESIAN_POINT('Ctrl Pts',(0.380197178359417,2.20276196479003,11.5014591149117));
#25237=CARTESIAN_POINT('Ctrl Pts',(0.385073071051741,2.18264203984399,11.5004181918829));
#25238=CARTESIAN_POINT('Ctrl Pts',(0.38834073475305,2.16226045078106,11.499377268854));
#25239=CARTESIAN_POINT('Ctrl Pts',(0.391610076641271,2.1418683942652,11.4983358112342));
#25240=CARTESIAN_POINT('Ctrl Pts',(0.393269407093095,2.12121512911217,11.4972943536144));
#25241=CARTESIAN_POINT('Ctrl Pts',(0.393299579763786,2.10057494141412,11.4962528959946));
#25242=CARTESIAN_POINT('Ctrl Pts',(0.393329761653542,2.07992844723888,11.4952111201641));
#25243=CARTESIAN_POINT('Ctrl Pts',(0.391729829908486,2.05929577368364,11.4941693443337));
#25244=CARTESIAN_POINT('Ctrl Pts',(0.388532742588471,2.03894921837781,11.4931275685032));
#25245=CARTESIAN_POINT('Ctrl Pts',(0.385328744691665,2.01855868353097,11.4920835408506));
#25246=CARTESIAN_POINT('Ctrl Pts',(0.380520870206384,1.99845621791746,11.491039513198));
#25247=CARTESIAN_POINT('Ctrl Pts',(0.374192916047162,1.97890271852712,11.4899954855454));
#25248=CARTESIAN_POINT('Ctrl Pts',(0.371954801606327,1.97198690209526,11.4896262266495));
#25249=CARTESIAN_POINT('Ctrl Pts',(0.369526979387773,1.96513958777413,11.4892569677536));
#25250=CARTESIAN_POINT('Ctrl Pts',(0.366914578088518,1.95837167519834,11.4888877088578));
#25251=CARTESIAN_POINT('Ctrl Pts',(0.35952884031106,1.939237544619,11.4878437462102));
#25252=CARTESIAN_POINT('Ctrl Pts',(0.350620335543212,1.92062569351484,11.4867997835627));
#25253=CARTESIAN_POINT('Ctrl Pts',(0.340284872086845,1.90279174502866,11.4857558209151));
#25254=CARTESIAN_POINT('Ctrl Pts',(0.329968421829214,1.88499060401244,11.4847137787493));
#25255=CARTESIAN_POINT('Ctrl Pts',(0.318230536804764,1.86796518429359,11.4836717365836));
#25256=CARTESIAN_POINT('Ctrl Pts',(0.305214129823192,1.85194914844679,11.4826296944178));
#25257=CARTESIAN_POINT('Ctrl Pts',(0.292211702258247,1.8359503135709,11.4815887713889));
#25258=CARTESIAN_POINT('Ctrl Pts',(0.277933917944923,1.82095929677809,11.4805478483601));
#25259=CARTESIAN_POINT('Ctrl Pts',(0.26256555834549,1.80717886420082,11.4795069253312));
#25260=CARTESIAN_POINT('Ctrl Pts',(0.247189305957109,1.79339135435254,11.4784654677114));
#25261=CARTESIAN_POINT('Ctrl Pts',(0.230721896388231,1.7808161739912,11.4774240100917));
#25262=CARTESIAN_POINT('Ctrl Pts',(0.213383590033715,1.76961789772398,11.4763825524719));
#25263=CARTESIAN_POINT('Ctrl Pts',(0.196039986070725,1.75841619989516,11.4753407766414));
#25264=CARTESIAN_POINT('Ctrl Pts',(0.177825592767668,1.74859261214799,11.4742990008109));
#25265=CARTESIAN_POINT('Ctrl Pts',(0.158987203639996,1.74026682238257,11.4732572249804));
#25266=CARTESIAN_POINT('Ctrl Pts',(0.140108094906718,1.73192303623363,11.4722131973278));
#25267=CARTESIAN_POINT('Ctrl Pts',(0.120602992564972,1.72508375531778,11.4711691696752));
#25268=CARTESIAN_POINT('Ctrl Pts',(0.100736624258962,1.71981974994365,11.4701251420226));
#25269=CARTESIAN_POINT('Ctrl Pts',(0.0937101501925314,1.71795794024209,
11.4697558831267));
#25270=CARTESIAN_POINT('Ctrl Pts',(0.0866385816794043,1.71629272166694,
11.4693866242308));
#25271=CARTESIAN_POINT('Ctrl Pts',(0.0795338595838778,1.71482568208707,
11.469017365335));
#25272=CARTESIAN_POINT('Ctrl Pts',(0.0594475066971782,1.71067809203304,
11.4679734026874));
#25273=CARTESIAN_POINT('Ctrl Pts',(0.0389759944577575,1.70809359104565,
11.4669294400399));
#25274=CARTESIAN_POINT('Ctrl Pts',(0.0183861181457955,1.7071299952153,11.4658854773923));
#25275=CARTESIAN_POINT('Ctrl Pts',(-0.00216588087000324,1.70616817202332,
11.4648434352265));
#25276=CARTESIAN_POINT('Ctrl Pts',(-0.0228350878531295,1.70682142858785,
11.4638013930608));
#25277=CARTESIAN_POINT('Ctrl Pts',(-0.0433476738410554,1.70909608703344,
11.462759350895));
#25278=CARTESIAN_POINT('Ctrl Pts',(-0.0638382296338581,1.71136830253158,
11.4617184278661));
#25279=CARTESIAN_POINT('Ctrl Pts',(-0.0841717675901777,1.71525841095673,
11.4606775048373));
#25280=CARTESIAN_POINT('Ctrl Pts',(-0.104077772771117,1.72072080571826,
11.4596365818084));
#25281=CARTESIAN_POINT('Ctrl Pts',(-0.123994001157526,1.72618600582338,
11.4585951241886));
#25282=CARTESIAN_POINT('Ctrl Pts',(-0.143481544303063,1.73322492627905,
11.4575536665688));
#25283=CARTESIAN_POINT('Ctrl Pts',(-0.162282793999812,1.74174145541018,
11.4565122089491));
#25284=CARTESIAN_POINT('Ctrl Pts',(-0.181089788298018,1.75026058671226,
11.4554704331186));
#25285=CARTESIAN_POINT('Ctrl Pts',(-0.199209416969298,1.76025788917048,
11.4544286572881));
#25286=CARTESIAN_POINT('Ctrl Pts',(-0.216407450495129,1.77159064360132,
11.4533868814576));
#25287=CARTESIAN_POINT('Ctrl Pts',(-0.233642657960676,1.78294789403801,
11.452342853805));
#25288=CARTESIAN_POINT('Ctrl Pts',(-0.24995171214025,1.79564590697609,11.4512988261524));
#25289=CARTESIAN_POINT('Ctrl Pts',(-0.26513180623412,1.80950040391933,11.4502547984998));
#25290=CARTESIAN_POINT('Ctrl Pts',(-0.270500806538165,1.8144005578868,11.4498855396039));
#25291=CARTESIAN_POINT('Ctrl Pts',(-0.275728919942093,1.81944504640133,
11.449516280708));
#25292=CARTESIAN_POINT('Ctrl Pts',(-0.280808347531718,1.82462468891256,
11.4491470218122));
#25293=CARTESIAN_POINT('Ctrl Pts',(-0.294977119330179,1.83907300448438,
11.4481169953106));
#25294=CARTESIAN_POINT('Ctrl Pts',(-0.308075501102544,1.85466661177501,
11.4470869688091));
#25295=CARTESIAN_POINT('Ctrl Pts',(-0.319912636152642,1.8712188923231,11.4460569423075));
#25296=CARTESIAN_POINT('Ctrl Pts',(-0.331731227406607,1.88774524243155,
11.4450285294229));
#25297=CARTESIAN_POINT('Ctrl Pts',(-0.342291997362797,1.90522671952452,
11.4440001165382));
#25298=CARTESIAN_POINT('Ctrl Pts',(-0.351443142374184,1.92344233894232,
11.4429717036536));
#25299=CARTESIAN_POINT('Ctrl Pts',(-0.360584777984027,1.94163902962069,
11.441944359443));
#25300=CARTESIAN_POINT('Ctrl Pts',(-0.368319331334013,1.96056768695691,
11.4409170152324));
#25301=CARTESIAN_POINT('Ctrl Pts',(-0.374540414687944,1.97998180235738,
11.4398896710218));
#25302=CARTESIAN_POINT('Ctrl Pts',(-0.380770837192769,1.99942506241688,
11.4388607845521));
#25303=CARTESIAN_POINT('Ctrl Pts',(-0.385482997449294,2.01935451861674,
11.4378318980824));
#25304=CARTESIAN_POINT('Ctrl Pts',(-0.388619909072765,2.03950656008892,
11.4368030116127));
#25305=CARTESIAN_POINT('Ctrl Pts',(-0.391756820696237,2.0596586015611,11.4357741251429));
#25306=CARTESIAN_POINT('Ctrl Pts',(-0.393318427568166,2.08003246947057,
11.4347452386732));
#25307=CARTESIAN_POINT('Ctrl Pts',(-0.393299835490125,2.10035972689682,
11.4337163522035));
#25308=CARTESIAN_POINT('',(-0.393451104642905,2.0998418228525,11.3087163522035));
#25309=CARTESIAN_POINT('Ctrl Pts',(-0.393338930018346,2.10035976265415,
11.4337163522035));
#25310=CARTESIAN_POINT('Ctrl Pts',(-0.393609748993565,2.12960050264535,
11.4322364608988));
#25311=CARTESIAN_POINT('Ctrl Pts',(-0.377272507462022,2.28941218116513,
11.4241331217531));
#25312=CARTESIAN_POINT('Ctrl Pts',(-0.158959746935375,2.53704327283899,
11.4094063347668));
#25313=CARTESIAN_POINT('Ctrl Pts',(0.28142602555706,2.4702356217581,11.3895359912438));
#25314=CARTESIAN_POINT('Ctrl Pts',(0.463641732294656,2.06378719074286,11.3696656477211));
#25315=CARTESIAN_POINT('Ctrl Pts',(0.220529268774129,1.69055908229216,11.3497953041983));
#25316=CARTESIAN_POINT('Ctrl Pts',(-0.224888776497657,1.69293727549082,
11.3299249606755));
#25317=CARTESIAN_POINT('Ctrl Pts',(-0.38966566303918,1.95190924956916,11.3162319766772));
#25318=CARTESIAN_POINT('Ctrl Pts',(-0.39391722199241,2.09105853526501,11.3091624405199));
#25319=CARTESIAN_POINT('Ctrl Pts',(-0.393872410819306,2.09984165347692,
11.3087163522035));
#25320=CARTESIAN_POINT('',(-0.393214805503193,2.09972692384377,11.1837163561346));
#25321=CARTESIAN_POINT('Ctrl Pts',(-0.393299968216638,2.09984188361311,
11.3087163522035));
#25322=CARTESIAN_POINT('Ctrl Pts',(-0.393308138253223,2.12016409810585,
11.3076826968398));
#25323=CARTESIAN_POINT('Ctrl Pts',(-0.391736909333096,2.14055070961828,
11.3066490414762));
#25324=CARTESIAN_POINT('Ctrl Pts',(-0.388582538022818,2.16073303173517,
11.3056153861125));
#25325=CARTESIAN_POINT('Ctrl Pts',(-0.385433660037181,2.18088020642124,
11.3045835308554));
#25326=CARTESIAN_POINT('Ctrl Pts',(-0.380707166298691,2.20082305413041,
11.3035516755983));
#25327=CARTESIAN_POINT('Ctrl Pts',(-0.374451184500351,2.22029630262932,
11.3025198203412));
#25328=CARTESIAN_POINT('Ctrl Pts',(-0.368195759830996,2.23976781693022,
11.3014880569763));
#25329=CARTESIAN_POINT('Ctrl Pts',(-0.360411297107628,2.25876908537834,
11.3004562936115));
#25330=CARTESIAN_POINT('Ctrl Pts',(-0.35119635464645,2.27704804569112,11.2994245302467));
#25331=CARTESIAN_POINT('Ctrl Pts',(-0.341983499361973,2.29532286583479,
11.2983930005754));
#25332=CARTESIAN_POINT('Ctrl Pts',(-0.33134115609013,2.31287503586723,11.2973614709041));
#25333=CARTESIAN_POINT('Ctrl Pts',(-0.319414312760897,2.32947633168474,
11.2963299412328));
#25334=CARTESIAN_POINT('Ctrl Pts',(-0.30745977490038,2.3461161762694,11.2952960163149));
#25335=CARTESIAN_POINT('Ctrl Pts',(-0.294215240158087,2.36180013753523,
11.294262091397));
#25336=CARTESIAN_POINT('Ctrl Pts',(-0.279867280661049,2.37633167609847,
11.2932281664791));
#25337=CARTESIAN_POINT('Ctrl Pts',(-0.265787066982277,2.3905920430931,11.2922135355294));
#25338=CARTESIAN_POINT('Ctrl Pts',(-0.250644892116299,2.40374230168349,
11.2911989045796));
#25339=CARTESIAN_POINT('Ctrl Pts',(-0.234647390926508,2.41563506131509,
11.2901842736299));
#25340=CARTESIAN_POINT('Ctrl Pts',(-0.218187422205484,2.42787162558976,
11.2891403109823));
#25341=CARTESIAN_POINT('Ctrl Pts',(-0.200718650950658,2.43885363312795,
11.2880963483347));
#25342=CARTESIAN_POINT('Ctrl Pts',(-0.182458554907021,2.44841608134706,
11.2870523856872));
#25343=CARTESIAN_POINT('Ctrl Pts',(-0.164232050277696,2.45796093841225,
11.2860103435214));
#25344=CARTESIAN_POINT('Ctrl Pts',(-0.145217727279964,2.46609102957953,
11.2849683013556));
#25345=CARTESIAN_POINT('Ctrl Pts',(-0.12566117064822,2.4726850683772,11.2839262591899));
#25346=CARTESIAN_POINT('Ctrl Pts',(-0.106125617451067,2.4792720252808,11.282885336161));
#25347=CARTESIAN_POINT('Ctrl Pts',(-0.08604967116135,2.48432594355809,11.2818444131322));
#25348=CARTESIAN_POINT('Ctrl Pts',(-0.0656978257613062,2.48777401368611,
11.2808034901033));
#25349=CARTESIAN_POINT('Ctrl Pts',(-0.0453355281838982,2.49122385465308,
11.2797620324835));
#25350=CARTESIAN_POINT('Ctrl Pts',(-0.0246977711695951,2.4930660610608,
11.2787205748637));
#25351=CARTESIAN_POINT('Ctrl Pts',(-0.0040586604570363,2.49327905776343,
11.277679117244));
#25352=CARTESIAN_POINT('Ctrl Pts',(0.0165867564036378,2.49349211954584,
11.2766373414135));
#25353=CARTESIAN_POINT('Ctrl Pts',(0.0372327922934162,2.49207500922423,
11.275595565583));
#25354=CARTESIAN_POINT('Ctrl Pts',(0.0576068683316351,2.48905827162653,
11.2745537897525));
#25355=CARTESIAN_POINT('Ctrl Pts',(0.0780249833975529,2.48603501328205,
11.2735097620999));
#25356=CARTESIAN_POINT('Ctrl Pts',(0.0981692472374602,2.48140538963035,
11.2724657344473));
#25357=CARTESIAN_POINT('Ctrl Pts',(0.117778030846165,2.4752508833434,11.2714217067947));
#25358=CARTESIAN_POINT('Ctrl Pts',(0.124713400581441,2.47307411514146,11.2710524478988));
#25359=CARTESIAN_POINT('Ctrl Pts',(0.131581951273689,2.4707070398309,11.270683189003));
#25360=CARTESIAN_POINT('Ctrl Pts',(0.13837273828728,2.46815468936152,11.2703139301071));
#25361=CARTESIAN_POINT('Ctrl Pts',(0.157571539099015,2.46093872629785,11.2692699674596));
#25362=CARTESIAN_POINT('Ctrl Pts',(0.176261569184111,2.45219542977191,11.268226004812));
#25363=CARTESIAN_POINT('Ctrl Pts',(0.194186366783898,2.44201834008613,11.2671820421645));
#25364=CARTESIAN_POINT('Ctrl Pts',(0.212078189786992,2.43185997225346,11.2661399999987));
#25365=CARTESIAN_POINT('Ctrl Pts',(0.229206912610394,2.4202733542875,11.2650979578329));
#25366=CARTESIAN_POINT('Ctrl Pts',(0.245337615962998,2.40739932367133,11.2640559156672));
#25367=CARTESIAN_POINT('Ctrl Pts',(0.261450995193613,2.3945391195618,11.2630149926383));
#25368=CARTESIAN_POINT('Ctrl Pts',(0.276567892644409,2.38039468175596,11.2619740696095));
#25369=CARTESIAN_POINT('Ctrl Pts',(0.290483913393173,2.36514898841932,11.2609331465806));
#25370=CARTESIAN_POINT('Ctrl Pts',(0.304407081047498,2.34989546529193,11.2598916889608));
#25371=CARTESIAN_POINT('Ctrl Pts',(0.317127631951129,2.33354008930304,11.258850231341));
#25372=CARTESIAN_POINT('Ctrl Pts',(0.328479046946049,2.31630165444909,11.2578087737212));
#25373=CARTESIAN_POINT('Ctrl Pts',(0.339833930293128,2.29905795250178,11.2567669978907));
#25374=CARTESIAN_POINT('Ctrl Pts',(0.349818470839558,2.28093128844845,11.2557252220603));
#25375=CARTESIAN_POINT('Ctrl Pts',(0.358310799350261,2.26216738595962,11.2546834462298));
#25376=CARTESIAN_POINT('Ctrl Pts',(0.366821484221758,2.24336292486975,11.2536394185772));
#25377=CARTESIAN_POINT('Ctrl Pts',(0.373833267765141,2.22391916822786,11.2525953909246));
#25378=CARTESIAN_POINT('Ctrl Pts',(0.379273037562057,2.20410020642847,11.251551363272));
#25379=CARTESIAN_POINT('Ctrl Pts',(0.38119701283606,2.19709049942211,11.2511821043761));
#25380=CARTESIAN_POINT('Ctrl Pts',(0.382924804130471,2.19003395838695,11.2508128454802));
#25381=CARTESIAN_POINT('Ctrl Pts',(0.384454717869747,2.18294250965394,11.2504435865844));
#25382=CARTESIAN_POINT('Ctrl Pts',(0.388780064708143,2.16289368299819,11.2493996239368));
#25383=CARTESIAN_POINT('Ctrl Pts',(0.391545795438273,2.14244586667834,11.2483556612893));
#25384=CARTESIAN_POINT('Ctrl Pts',(0.392691733037251,2.12186533338873,11.2473116986417));
#25385=CARTESIAN_POINT('Ctrl Pts',(0.393835562560534,2.10132266020778,11.2462696564759));
#25386=CARTESIAN_POINT('Ctrl Pts',(0.393365413884186,2.08064847771675,11.2452276143102));
#25387=CARTESIAN_POINT('Ctrl Pts',(0.391272539628604,2.06011654813607,11.2441855721444));
#25388=CARTESIAN_POINT('Ctrl Pts',(0.389181913087094,2.03960666952521,11.2431446491156));
#25389=CARTESIAN_POINT('Ctrl Pts',(0.385472066267624,2.01923947173177,11.2421037260867));
#25390=CARTESIAN_POINT('Ctrl Pts',(0.380186207823277,1.99928586305312,11.2410628030578));
#25391=CARTESIAN_POINT('Ctrl Pts',(0.3748976346998,1.97932200672109,11.240021345438));
#25392=CARTESIAN_POINT('Ctrl Pts',(0.368031605785315,1.95977287922202,11.2389798878183));
#25393=CARTESIAN_POINT('Ctrl Pts',(0.359681947160373,1.94089692998901,11.2379384301985));
#25394=CARTESIAN_POINT('Ctrl Pts',(0.351329737350708,1.92201521333059,11.236896654368));
#25395=CARTESIAN_POINT('Ctrl Pts',(0.34149332587491,1.90380774209201,11.2358548785375));
#25396=CARTESIAN_POINT('Ctrl Pts',(0.330313351575673,1.88651000077089,11.234813102707));
#25397=CARTESIAN_POINT('Ctrl Pts',(0.319109211508281,1.86917486998937,11.2337690750544));
#25398=CARTESIAN_POINT('Ctrl Pts',(0.306556157922229,1.85275398004779,11.2327250474018));
#25399=CARTESIAN_POINT('Ctrl Pts',(0.292836665676481,1.83745176207889,11.2316810197492));
#25400=CARTESIAN_POINT('Ctrl Pts',(0.287984261100866,1.83203956816097,11.2313117608533));
#25401=CARTESIAN_POINT('Ctrl Pts',(0.282986279702331,1.82676697713963,11.2309425019574));
#25402=CARTESIAN_POINT('Ctrl Pts',(0.277851832590422,1.82164186894193,11.2305732430616));
#25403=CARTESIAN_POINT('Ctrl Pts',(0.263335808574053,1.80715224774946,11.229529280414));
#25404=CARTESIAN_POINT('Ctrl Pts',(0.247640058524564,1.79375799939032,11.2284853177665));
#25405=CARTESIAN_POINT('Ctrl Pts',(0.230955894380986,1.78165386000349,11.2274413551189));
#25406=CARTESIAN_POINT('Ctrl Pts',(0.214302422555172,1.76957198748535,11.2263993129531));
#25407=CARTESIAN_POINT('Ctrl Pts',(0.196664699784659,1.75877598836898,11.2253572707874));
#25408=CARTESIAN_POINT('Ctrl Pts',(0.178268175131284,1.74942141004425,11.2243152286216));
#25409=CARTESIAN_POINT('Ctrl Pts',(0.159891408056386,1.74007687838968,11.2232743055927));
#25410=CARTESIAN_POINT('Ctrl Pts',(0.140758096373477,1.73217105184052,11.2222333825639));
#25411=CARTESIAN_POINT('Ctrl Pts',(0.121119414254062,1.72581424734398,11.221192459535));
#25412=CARTESIAN_POINT('Ctrl Pts',(0.10147064621935,1.71945417815833,11.2201510019152));
#25413=CARTESIAN_POINT('Ctrl Pts',(0.081316684290351,1.71464496225607,11.2191095442954));
#25414=CARTESIAN_POINT('Ctrl Pts',(0.0609256271305449,1.71144761233683,
11.2180680866757));
#25415=CARTESIAN_POINT('Ctrl Pts',(0.0405283396137982,1.7082492854878,11.2170263108452));
#25416=CARTESIAN_POINT('Ctrl Pts',(0.0198945445382996,1.70666388320196,
11.2159845350147));
#25417=CARTESIAN_POINT('Ctrl Pts',(-0.000701628167408186,1.70670062583585,
11.2149427591842));
#25418=CARTESIAN_POINT('Ctrl Pts',(-0.0213423199677942,1.70673744788977,
11.2138987315316));
#25419=CARTESIAN_POINT('Ctrl Pts',(-0.0419444929620127,1.70840335566758,
11.212854703879));
#25420=CARTESIAN_POINT('Ctrl Pts',(-0.0622374808551683,1.71165558330677,
11.2118106762264));
#25421=CARTESIAN_POINT('Ctrl Pts',(-0.0694148446774901,1.71280585359336,
11.2114414173305));
#25422=CARTESIAN_POINT('Ctrl Pts',(-0.0765536312495216,1.71415409704949,
11.2110721584346));
#25423=CARTESIAN_POINT('Ctrl Pts',(-0.0836422829792746,1.71569691843804,
11.2107028995388));
#25424=CARTESIAN_POINT('Ctrl Pts',(-0.103683201993579,1.72005875756914,
11.2096589368912));
#25425=CARTESIAN_POINT('Ctrl Pts',(-0.123441718935667,1.72600547657797,
11.2086149742437));
#25426=CARTESIAN_POINT('Ctrl Pts',(-0.142650535563883,1.73348163115154,
11.2075710115961));
#25427=CARTESIAN_POINT('Ctrl Pts',(-0.161824015504042,1.74094403253317,
11.2065289694303));
#25428=CARTESIAN_POINT('Ctrl Pts',(-0.180449102885875,1.74993007623814,
11.2054869272646));
#25429=CARTESIAN_POINT('Ctrl Pts',(-0.198272971028225,1.76033440127143,
11.2044448850988));
#25430=CARTESIAN_POINT('Ctrl Pts',(-0.216077696616201,1.77072755222308,
11.20340396207));
#25431=CARTESIAN_POINT('Ctrl Pts',(-0.233082264458637,1.78253561649592,
11.2023630390411));
#25432=CARTESIAN_POINT('Ctrl Pts',(-0.249057952973691,1.79560711890625,
11.2013221160122));
#25433=CARTESIAN_POINT('Ctrl Pts',(-0.265041846185989,1.80868533449953,
11.2002806583925));
#25434=CARTESIAN_POINT('Ctrl Pts',(-0.279995224773786,1.82302783106876,
11.1992392007727));
#25435=CARTESIAN_POINT('Ctrl Pts',(-0.29372166151608,1.83844221373426,11.1981977431529));
#25436=CARTESIAN_POINT('Ctrl Pts',(-0.307452292283217,1.85386130616568,
11.1971559673224));
#25437=CARTESIAN_POINT('Ctrl Pts',(-0.319954773014172,1.87035236359677,
11.1961141914919));
#25438=CARTESIAN_POINT('Ctrl Pts',(-0.331072959584572,1.88768988382107,
11.1950724156614));
#25439=CARTESIAN_POINT('Ctrl Pts',(-0.342215178367549,1.90506487948877,
11.1940283880088));
#25440=CARTESIAN_POINT('Ctrl Pts',(-0.351966781780331,1.92328934139265,
11.1929843603562));
#25441=CARTESIAN_POINT('Ctrl Pts',(-0.360217211569774,1.94211253853172,
11.1919403327036));
#25442=CARTESIAN_POINT('Ctrl Pts',(-0.363135280441789,1.94877005663019,
11.1915710738077));
#25443=CARTESIAN_POINT('Ctrl Pts',(-0.365866007365618,1.95550230473974,
11.1912018149119));
#25444=CARTESIAN_POINT('Ctrl Pts',(-0.368405990784053,1.96229772712689,
11.190832556016));
#25445=CARTESIAN_POINT('Ctrl Pts',(-0.376614512448147,1.98425864682296,
11.1896392137192));
#25446=CARTESIAN_POINT('Ctrl Pts',(-0.382867824574344,2.00698821532882,
11.1884458714223));
#25447=CARTESIAN_POINT('Ctrl Pts',(-0.387048135574983,2.03015280429445,
11.1872525291255));
#25448=CARTESIAN_POINT('Ctrl Pts',(-0.39117723833591,2.05303363020408,11.1860738051091));
#25449=CARTESIAN_POINT('Ctrl Pts',(-0.393283661585075,2.07633860235924,
11.1848950810926));
#25450=CARTESIAN_POINT('Ctrl Pts',(-0.393299905144833,2.0997268460775,11.1837163570762));
#25451=CARTESIAN_POINT('',(-0.39323593112807,2.10028300833082,11.058716348113));
#25452=CARTESIAN_POINT('Ctrl Pts',(-0.392859536202407,2.09972724849813,
11.1837163522035));
#25453=CARTESIAN_POINT('Ctrl Pts',(-0.392322465415884,2.18398909790107,
11.1794649723));
#25454=CARTESIAN_POINT('Ctrl Pts',(-0.324387757795137,2.40031688674488,
11.1685901445557));
#25455=CARTESIAN_POINT('Ctrl Pts',(0.0321045751991462,2.56394430671225,
11.1510918689703));
#25456=CARTESIAN_POINT('Ctrl Pts',(0.407471466368896,2.32414733452502,11.1312215254476));
#25457=CARTESIAN_POINT('Ctrl Pts',(0.409038759376262,1.87872569781509,11.1113511819248));
#25458=CARTESIAN_POINT('Ctrl Pts',(0.0353686762546443,1.63629310958381,
11.091480838402));
#25459=CARTESIAN_POINT('Ctrl Pts',(-0.32322012530308,1.79783743961437,11.0739358951616));
#25460=CARTESIAN_POINT('Ctrl Pts',(-0.392314997973443,2.01510676408243,
11.0630143997621));
#25461=CARTESIAN_POINT('Ctrl Pts',(-0.39287953052133,2.10028267075746,11.0587163522035));
#25462=CARTESIAN_POINT('',(-0.393447242236147,2.10014273833465,10.9337163522035));
#25463=CARTESIAN_POINT('Ctrl Pts',(-0.393299898133711,2.1002830689187,11.0587163473789));
#25464=CARTESIAN_POINT('Ctrl Pts',(-0.393282756740734,2.12409955906082,
11.0575158255002));
#25465=CARTESIAN_POINT('Ctrl Pts',(-0.391098152989675,2.14782821277761,
11.0563153036215));
#25466=CARTESIAN_POINT('Ctrl Pts',(-0.386817917864597,2.17111109912593,
11.0551147817429));
#25467=CARTESIAN_POINT('Ctrl Pts',(-0.382807381066406,2.19292692693431,
11.0539899049474));
#25468=CARTESIAN_POINT('Ctrl Pts',(-0.376957620305677,2.21435139802366,
11.0528650281519));
#25469=CARTESIAN_POINT('Ctrl Pts',(-0.369365914877162,2.23510629491981,
11.0517401513565));
#25470=CARTESIAN_POINT('Ctrl Pts',(-0.362320292698361,2.25436825960839,
11.0506961887089));
#25471=CARTESIAN_POINT('Ctrl Pts',(-0.353742890421406,2.2731350022375,11.0496522260614));
#25472=CARTESIAN_POINT('Ctrl Pts',(-0.343724973009998,2.29114924255481,
11.0486082634138));
#25473=CARTESIAN_POINT('Ctrl Pts',(-0.333725484637158,2.3091303437359,11.0475662212481));
#25474=CARTESIAN_POINT('Ctrl Pts',(-0.322291042826342,2.32636102572852,
11.0465241790823));
#25475=CARTESIAN_POINT('Ctrl Pts',(-0.309560398683813,2.34260513095712,
11.0454821369165));
#25476=CARTESIAN_POINT('Ctrl Pts',(-0.2968434270531,2.35883179027188,11.0444412138876));
#25477=CARTESIAN_POINT('Ctrl Pts',(-0.282833445540318,2.37407338229495,
11.0434002908588));
#25478=CARTESIAN_POINT('Ctrl Pts',(-0.267711614657557,2.38812389935138,
11.0423593678299));
#25479=CARTESIAN_POINT('Ctrl Pts',(-0.252582017596578,2.40218163238717,
11.0413179102101));
#25480=CARTESIAN_POINT('Ctrl Pts',(-0.236339958445469,2.41504655576692,
11.0402764525903));
#25481=CARTESIAN_POINT('Ctrl Pts',(-0.219202747635513,2.42655021884703,
11.0392349949705));
#25482=CARTESIAN_POINT('Ctrl Pts',(-0.202060300660533,2.43805739679772,
11.03819321914));
#25483=CARTESIAN_POINT('Ctrl Pts',(-0.184022788091632,2.44820210674712,
11.0371514433095));
#25484=CARTESIAN_POINT('Ctrl Pts',(-0.165334844474637,2.45686030768712,
11.036109667479));
#25485=CARTESIAN_POINT('Ctrl Pts',(-0.146606506443435,2.46553722352494,
11.0350656398263));
#25486=CARTESIAN_POINT('Ctrl Pts',(-0.127225621076391,2.47272095954478,
11.0340216121737));
#25487=CARTESIAN_POINT('Ctrl Pts',(-0.107455620797547,2.47833606695505,
11.0329775845211));
#25488=CARTESIAN_POINT('Ctrl Pts',(-0.100463230839971,2.4803220568444,11.0326083256253));
#25489=CARTESIAN_POINT('Ctrl Pts',(-0.0934222709461556,2.48211228529378,
11.0322390667295));
#25490=CARTESIAN_POINT('Ctrl Pts',(-0.0863446519779231,2.48370495315387,
11.0318698078336));
#25491=CARTESIAN_POINT('Ctrl Pts',(-0.066334924602597,2.48820771740592,
11.0308258451861));
#25492=CARTESIAN_POINT('Ctrl Pts',(-0.0459124085568853,2.49115446087699,
11.0297818825385));
#25493=CARTESIAN_POINT('Ctrl Pts',(-0.0253428330572904,2.49248265033327,
11.028737919891));
#25494=CARTESIAN_POINT('Ctrl Pts',(-0.00481109750832695,2.49380839644193,
11.0276958777252));
#25495=CARTESIAN_POINT('Ctrl Pts',(0.015866438375116,2.49352139254206,11.0266538355594));
#25496=CARTESIAN_POINT('Ctrl Pts',(0.0364161005943682,2.49161046668533,
11.0256117933937));
#25497=CARTESIAN_POINT('Ctrl Pts',(0.0569436927992294,2.48970159313294,
11.0245708703648));
#25498=CARTESIAN_POINT('Ctrl Pts',(0.077342952400591,2.48617229899716,11.023529947336));
#25499=CARTESIAN_POINT('Ctrl Pts',(0.0973425989983654,2.48106339160334,
11.0224890243071));
#25500=CARTESIAN_POINT('Ctrl Pts',(0.117352516893378,2.47595186040784,11.0214475666873));
#25501=CARTESIAN_POINT('Ctrl Pts',(0.136961694903382,2.46925926174951,11.0204061090675));
#25502=CARTESIAN_POINT('Ctrl Pts',(0.15591086264823,2.46107712875269,11.0193646514477));
#25503=CARTESIAN_POINT('Ctrl Pts',(0.174865820189927,2.45289249575753,11.0183228756173));
#25504=CARTESIAN_POINT('Ctrl Pts',(0.193159705420792,2.44321774703808,11.0172810997868));
#25505=CARTESIAN_POINT('Ctrl Pts',(0.210555797340428,2.43219143006155,11.0162393239563));
#25506=CARTESIAN_POINT('Ctrl Pts',(0.227989491307518,2.42114127945065,11.0151952963037));
#25507=CARTESIAN_POINT('Ctrl Pts',(0.244520928612884,2.40873417014082,11.0141512686511));
#25508=CARTESIAN_POINT('Ctrl Pts',(0.259944069830627,2.39515075903662,11.0131072409985));
#25509=CARTESIAN_POINT('Ctrl Pts',(0.265399032716648,2.39034648457703,11.0127379821026));
#25510=CARTESIAN_POINT('Ctrl Pts',(0.270715687663013,2.38539540244076,11.0123687232067));
#25511=CARTESIAN_POINT('Ctrl Pts',(0.275886074348036,2.38030655358166,11.0119994643109));
#25512=CARTESIAN_POINT('Ctrl Pts',(0.290503706131458,2.36591944419209,11.0109555016633));
#25513=CARTESIAN_POINT('Ctrl Pts',(0.304036457748546,2.35034295253348,11.0099115390158));
#25514=CARTESIAN_POINT('Ctrl Pts',(0.316287906110368,2.33376665811941,11.0088675763682));
#25515=CARTESIAN_POINT('Ctrl Pts',(0.328516816612759,2.31722085758512,11.0078255342025));
#25516=CARTESIAN_POINT('Ctrl Pts',(0.339468622388193,2.29967945479898,11.0067834920367));
#25517=CARTESIAN_POINT('Ctrl Pts',(0.348985785182018,2.28136651218152,11.0057414498709));
#25518=CARTESIAN_POINT('Ctrl Pts',(0.358492726692516,2.26307323737675,11.0047005268421));
#25519=CARTESIAN_POINT('Ctrl Pts',(0.366567720806767,2.24401070398177,11.0036596038132));
#25520=CARTESIAN_POINT('Ctrl Pts',(0.373098230072271,2.22442909915666,11.0026186807844));
#25521=CARTESIAN_POINT('Ctrl Pts',(0.379632093237126,2.20483743772968,11.0015772231646));
#25522=CARTESIAN_POINT('Ctrl Pts',(0.384619638830534,2.18472686518731,11.0005357655448));
#25523=CARTESIAN_POINT('Ctrl Pts',(0.387997481800792,2.16436492924135,10.999494307925));
#25524=CARTESIAN_POINT('Ctrl Pts',(0.391376356849339,2.14399677183626,10.9984525320945));
#25525=CARTESIAN_POINT('Ctrl Pts',(0.39314446553063,2.12337782929996,10.997410756264));
#25526=CARTESIAN_POINT('Ctrl Pts',(0.393290159680905,2.10278213913533,10.9963689804335));
#25527=CARTESIAN_POINT('Ctrl Pts',(0.393436168752392,2.08214193091904,10.9953249527809));
#25528=CARTESIAN_POINT('Ctrl Pts',(0.391952814820575,2.06152580999585,10.9942809251283));
#25529=CARTESIAN_POINT('Ctrl Pts',(0.388880464581221,2.04120481085077,10.9932368974757));
#25530=CARTESIAN_POINT('Ctrl Pts',(0.387793814573136,2.03401753981557,10.9928676385798));
#25531=CARTESIAN_POINT('Ctrl Pts',(0.386508857455187,2.02686709092432,10.9924983796839));
#25532=CARTESIAN_POINT('Ctrl Pts',(0.385028885957275,2.01976505138969,10.9921291207881));
#25533=CARTESIAN_POINT('Ctrl Pts',(0.380844734998389,1.99968628259529,10.9910851581405));
#25534=CARTESIAN_POINT('Ctrl Pts',(0.375073264895953,1.97987586635585,10.990041195493));
#25535=CARTESIAN_POINT('Ctrl Pts',(0.367767550132113,1.96060158153758,10.9889972328454));
#25536=CARTESIAN_POINT('Ctrl Pts',(0.360475275017815,1.94136275384315,10.9879551906796));
#25537=CARTESIAN_POINT('Ctrl Pts',(0.351654559839988,1.9226588011806,10.9869131485139));
#25538=CARTESIAN_POINT('Ctrl Pts',(0.341408521989746,1.90474347357187,10.9858711063481));
#25539=CARTESIAN_POINT('Ctrl Pts',(0.331173488223197,1.88684738674356,10.9848301833192));
#25540=CARTESIAN_POINT('Ctrl Pts',(0.319516509061671,1.86973889334966,10.9837892602904));
#25541=CARTESIAN_POINT('Ctrl Pts',(0.306587027792332,1.85364804772549,10.9827483372615));
#25542=CARTESIAN_POINT('Ctrl Pts',(0.293650906278391,1.83754893826237,10.9817068796417));
#25543=CARTESIAN_POINT('Ctrl Pts',(0.279441425366232,1.82246910433631,10.9806654220219));
#25544=CARTESIAN_POINT('Ctrl Pts',(0.264149232488438,1.80860666964433,10.9796239644021));
#25545=CARTESIAN_POINT('Ctrl Pts',(0.248852367179039,1.7947399993742,10.9785821885716));
#25546=CARTESIAN_POINT('Ctrl Pts',(0.232472700301874,1.78209193578253,10.9775404127411));
#25547=CARTESIAN_POINT('Ctrl Pts',(0.215234342134315,1.7708206143058,10.9764986369106));
#25548=CARTESIAN_POINT('Ctrl Pts',(0.197958722864387,1.75952492961193,10.9754546092581));
#25549=CARTESIAN_POINT('Ctrl Pts',(0.179821352987357,1.74961228139096,10.9744105816055));
#25550=CARTESIAN_POINT('Ctrl Pts',(0.161071974372725,1.74119544446639,10.9733665539529));
#25551=CARTESIAN_POINT('Ctrl Pts',(0.154440564919061,1.73821851957204,10.972997295057));
#25552=CARTESIAN_POINT('Ctrl Pts',(0.147732768961565,1.73542826733806,10.9726280361611));
#25553=CARTESIAN_POINT('Ctrl Pts',(0.140960111650303,1.73282819154579,10.9722587772653));
#25554=CARTESIAN_POINT('Ctrl Pts',(0.121812566833145,1.72547730023794,10.9712148146177));
#25555=CARTESIAN_POINT('Ctrl Pts',(0.102031413115449,1.71960631937277,10.9701708519702));
#25556=CARTESIAN_POINT('Ctrl Pts',(0.0818705339385076,1.71531557651417,
10.9691268893226));
#25557=CARTESIAN_POINT('Ctrl Pts',(0.0617467428712652,1.71103272693941,
10.9680848471568));
#25558=CARTESIAN_POINT('Ctrl Pts',(0.0412453120838937,1.70832455465519,
10.9670428049911));
#25559=CARTESIAN_POINT('Ctrl Pts',(0.02063541844509,1.70724171618463,10.9660007628253));
#25560=CARTESIAN_POINT('Ctrl Pts',(4.76595082905158E-5,1.70616004066558,
10.9649598397964));
#25561=CARTESIAN_POINT('Ctrl Pts',(-0.020647601502705,1.70670030085064,
10.9639189167676));
#25562=CARTESIAN_POINT('Ctrl Pts',(-0.0411760344321745,1.70886137471679,
10.9628779937387));
#25563=CARTESIAN_POINT('Ctrl Pts',(-0.0617150102297682,1.71102355845416,
10.9618365361189));
#25564=CARTESIAN_POINT('Ctrl Pts',(-0.0820862533567069,1.71480815783761,
10.9607950784992));
#25565=CARTESIAN_POINT('Ctrl Pts',(-0.102019976961212,1.72016212102947,
10.9597536208794));
#25566=CARTESIAN_POINT('Ctrl Pts',(-0.121959791187311,1.72551772009049,
10.9587118450489));
#25567=CARTESIAN_POINT('Ctrl Pts',(-0.141461119153378,1.73244341191047,
10.9576700692184));
#25568=CARTESIAN_POINT('Ctrl Pts',(-0.160269682810538,1.74083636212471,
10.9566282933879));
#25569=CARTESIAN_POINT('Ctrl Pts',(-0.179118901604866,1.74924745389131,
10.9555842657353));
#25570=CARTESIAN_POINT('Ctrl Pts',(-0.197271719744822,1.75913178363014,
10.9545402380827));
#25571=CARTESIAN_POINT('Ctrl Pts',(-0.214498124353156,1.77034041095552,
10.9534962104301));
#25572=CARTESIAN_POINT('Ctrl Pts',(-0.220590877863647,1.77430475552057,
10.9531269515342));
#25573=CARTESIAN_POINT('Ctrl Pts',(-0.226568023053773,1.77843437650973,
10.9527576926384));
#25574=CARTESIAN_POINT('Ctrl Pts',(-0.232420375109476,1.7827214800306,10.9523884337425));
#25575=CARTESIAN_POINT('Ctrl Pts',(-0.248819573639561,1.79473460929704,
10.9513537130209));
#25576=CARTESIAN_POINT('Ctrl Pts',(-0.264337975346716,1.80806158770309,
10.9503189922992));
#25577=CARTESIAN_POINT('Ctrl Pts',(-0.278755922944686,1.8225472555132,10.9492842715776));
#25578=CARTESIAN_POINT('Ctrl Pts',(-0.293147344501958,1.83700627269144,
10.948251454528));
#25579=CARTESIAN_POINT('Ctrl Pts',(-0.306441761726816,1.8526192683248,10.9472186374785));
#25580=CARTESIAN_POINT('Ctrl Pts',(-0.318452741495019,1.86919111491473,
10.9461858204289));
#25581=CARTESIAN_POINT('Ctrl Pts',(-0.330537047765084,1.88586413189735,
10.9451466980768));
#25582=CARTESIAN_POINT('Ctrl Pts',(-0.341321657094338,1.90350719523694,
10.9441075757247));
#25583=CARTESIAN_POINT('Ctrl Pts',(-0.350657800144795,1.92188768375653,
10.9430684533726));
#25584=CARTESIAN_POINT('Ctrl Pts',(-0.35993220757721,1.94014663056317,10.9420362022584));
#25585=CARTESIAN_POINT('Ctrl Pts',(-0.367776946782641,1.95913258149407,
10.9410039511443));
#25586=CARTESIAN_POINT('Ctrl Pts',(-0.374092750276984,1.97859364023989,
10.9399717000301));
#25587=CARTESIAN_POINT('Ctrl Pts',(-0.380471616026515,1.99824901444437,
10.938929142059));
#25588=CARTESIAN_POINT('Ctrl Pts',(-0.385290591659725,2.018388300583,10.9378865840879));
#25589=CARTESIAN_POINT('Ctrl Pts',(-0.388499540705839,2.03873829196511,
10.9368440261168));
#25590=CARTESIAN_POINT('Ctrl Pts',(-0.391708489751952,2.05908828334722,
10.9358014681457));
#25591=CARTESIAN_POINT('Ctrl Pts',(-0.393307409292416,2.07964819771871,
10.9347589101746));
#25592=CARTESIAN_POINT('Ctrl Pts',(-0.393299974117743,2.10014268490739,
10.9337163522035));
#25593=CARTESIAN_POINT('',(-0.393299834164626,2.09963882680431,10.8087163522035));
#25594=CARTESIAN_POINT('Ctrl Pts',(-0.39388694406762,2.10014289785364,10.9337163522035));
#25595=CARTESIAN_POINT('Ctrl Pts',(-0.393923666401966,2.10800639674678,
10.9333169315422));
#25596=CARTESIAN_POINT('Ctrl Pts',(-0.393708632815697,2.11586784849621,
10.932917510881));
#25597=CARTESIAN_POINT('Ctrl Pts',(-0.38538959090996,2.25381922960492,10.9258946423788));
#25598=CARTESIAN_POINT('Ctrl Pts',(-0.227747813468656,2.50547004444192,
10.9126477466968));
#25599=CARTESIAN_POINT('Ctrl Pts',(0.217642466485707,2.51098270068397,10.8927774031741));
#25600=CARTESIAN_POINT('Ctrl Pts',(0.46337541278574,2.13947467929094,10.8729070596514));
#25601=CARTESIAN_POINT('Ctrl Pts',(0.284024500720983,1.73175401364076,10.8530367161285));
#25602=CARTESIAN_POINT('Ctrl Pts',(-0.155880224311077,1.66184890831106,
10.8331663726058));
#25603=CARTESIAN_POINT('Ctrl Pts',(-0.376627538569165,1.90871737413284,
10.8183929179641));
#25604=CARTESIAN_POINT('Ctrl Pts',(-0.393589382880225,2.06947046398226,
10.8102429111633));
#25605=CARTESIAN_POINT('Ctrl Pts',(-0.393310804513336,2.09963881673007,
10.8087163522035));
#25606=CARTESIAN_POINT('',(-0.393052814201458,2.10004628639809,10.6837163396379));
#25607=CARTESIAN_POINT('Ctrl Pts',(-0.393299834164626,2.09963882680431,
10.8087163522035));
#25608=CARTESIAN_POINT('Ctrl Pts',(-0.393318497199042,2.11996195274014,
10.8076879366028));
#25609=CARTESIAN_POINT('Ctrl Pts',(-0.391757613702059,2.14033015283819,
10.8066595210021));
#25610=CARTESIAN_POINT('Ctrl Pts',(-0.388622714666593,2.1604754135593,10.8056311054015));
#25611=CARTESIAN_POINT('Ctrl Pts',(-0.385488191001509,2.18061826210248,
10.8046028129425));
#25612=CARTESIAN_POINT('Ctrl Pts',(-0.380780088998554,2.20053747030646,
10.8035745204835));
#25613=CARTESIAN_POINT('Ctrl Pts',(-0.374555819724814,2.21997011257089,
10.8025462280245));
#25614=CARTESIAN_POINT('Ctrl Pts',(-0.36833302776285,2.23939814255555,10.8015181796277));
#25615=CARTESIAN_POINT('Ctrl Pts',(-0.360595024438406,2.25833911782682,
10.8004901312308));
#25616=CARTESIAN_POINT('Ctrl Pts',(-0.35144880686354,2.27654638527649,10.799462082834));
#25617=CARTESIAN_POINT('Ctrl Pts',(-0.342281589741461,2.29479545627711,
10.7984316740569));
#25618=CARTESIAN_POINT('Ctrl Pts',(-0.331700065682448,2.31230678743153,
10.7974012652799));
#25619=CARTESIAN_POINT('Ctrl Pts',(-0.31985720867979,2.3288585940173,10.7963708565029));
#25620=CARTESIAN_POINT('Ctrl Pts',(-0.308573907301469,2.34462835481243,
10.7953891328553));
#25621=CARTESIAN_POINT('Ctrl Pts',(-0.296146369165086,2.35952691372295,
10.7944074092077));
#25622=CARTESIAN_POINT('Ctrl Pts',(-0.282739281461414,2.37339237136153,
10.7934256855602));
#25623=CARTESIAN_POINT('Ctrl Pts',(-0.268482215524499,2.38813686682304,
10.7923817229126));
#25624=CARTESIAN_POINT('Ctrl Pts',(-0.253026204402658,2.40180705990591,
10.7913377602651));
#25625=CARTESIAN_POINT('Ctrl Pts',(-0.236559080309437,2.41420485598277,
10.7902937976175));
#25626=CARTESIAN_POINT('Ctrl Pts',(-0.220122249265415,2.42657984497781,
10.7892517554518));
#25627=CARTESIAN_POINT('Ctrl Pts',(-0.202678542778262,2.43768659812352,
10.788209713286));
#25628=CARTESIAN_POINT('Ctrl Pts',(-0.18445061904708,2.44736559866105,10.7871676711202));
#25629=CARTESIAN_POINT('Ctrl Pts',(-0.166242271819633,2.45703420410405,
10.7861267480914));
#25630=CARTESIAN_POINT('Ctrl Pts',(-0.147252012376544,2.46527773221188,
10.7850858250625));
#25631=CARTESIAN_POINT('Ctrl Pts',(-0.127729021236514,2.47198143385653,
10.7840449020336));
#25632=CARTESIAN_POINT('Ctrl Pts',(-0.108196003597072,2.47868857834763,
10.7830034444139));
#25633=CARTESIAN_POINT('Ctrl Pts',(-0.0881303983353836,2.48385406230473,
10.7819619867941));
#25634=CARTESIAN_POINT('Ctrl Pts',(-0.0677991812195428,2.48741213329729,
10.7809205291743));
#25635=CARTESIAN_POINT('Ctrl Pts',(-0.0474617520304963,2.49097129143566,
10.7798787533438));
#25636=CARTESIAN_POINT('Ctrl Pts',(-0.0268592798146348,2.49292196778493,
10.7788369775133));
#25637=CARTESIAN_POINT('Ctrl Pts',(-0.00626568814791708,2.49325008728802,
10.7777952016828));
#25638=CARTESIAN_POINT('Ctrl Pts',(0.014372417034512,2.49357891602885,10.7767511740302));
#25639=CARTESIAN_POINT('Ctrl Pts',(0.0350008683268066,2.4922782323283,10.7757071463776));
#25640=CARTESIAN_POINT('Ctrl Pts',(0.0553482843194677,2.48938600054816,
10.774663118725));
#25641=CARTESIAN_POINT('Ctrl Pts',(0.0625448986472379,2.48836305607817,
10.7742938598291));
#25642=CARTESIAN_POINT('Ctrl Pts',(0.0697064488265022,2.48714148611739,
10.7739246009332));
#25643=CARTESIAN_POINT('Ctrl Pts',(0.0768213189330443,2.48572448063014,
10.7735553420374));
#25644=CARTESIAN_POINT('Ctrl Pts',(0.0969363621086848,2.48171834613584,
10.7725113793898));
#25645=CARTESIAN_POINT('Ctrl Pts',(0.116797123301805,2.4761225777747,10.7714674167423));
#25646=CARTESIAN_POINT('Ctrl Pts',(0.13613536403185,2.46898787603377,10.7704234540947));
#25647=CARTESIAN_POINT('Ctrl Pts',(0.155438029984263,2.4618662993455,10.7693814119289));
#25648=CARTESIAN_POINT('Ctrl Pts',(0.174219380398024,2.45321160477635,10.7683393697632));
#25649=CARTESIAN_POINT('Ctrl Pts',(0.192224761819899,2.44312465802283,10.7672973275974));
#25650=CARTESIAN_POINT('Ctrl Pts',(0.210210805744975,2.43304854449166,10.7662564045685));
#25651=CARTESIAN_POINT('Ctrl Pts',(0.227421882342083,2.42154356505889,10.7652154815397));
#25652=CARTESIAN_POINT('Ctrl Pts',(0.24362662257272,2.40875711938967,10.7641745585108));
#25653=CARTESIAN_POINT('Ctrl Pts',(0.259839685135593,2.39596410693522,10.763133100891));
#25654=CARTESIAN_POINT('Ctrl Pts',(0.275044791222169,2.38188875656924,10.7620916432713));
#25655=CARTESIAN_POINT('Ctrl Pts',(0.289042136204373,2.36671995331886,10.7610501856515));
#25656=CARTESIAN_POINT('Ctrl Pts',(0.303043757985698,2.35154651533778,10.760008409821));
#25657=CARTESIAN_POINT('Ctrl Pts',(0.315836412059314,2.33527952417846,10.7589666339905));
#25658=CARTESIAN_POINT('Ctrl Pts',(0.327259984084065,2.31814168060528,10.75792485816));
#25659=CARTESIAN_POINT('Ctrl Pts',(0.338708248418983,2.30096679319431,10.7568808305074));
#25660=CARTESIAN_POINT('Ctrl Pts',(0.348781163692602,2.28291793841907,10.7558368028548));
#25661=CARTESIAN_POINT('Ctrl Pts',(0.357363747359534,2.26424384942259,10.7547927752022));
#25662=CARTESIAN_POINT('Ctrl Pts',(0.360399294704181,2.2576390689198,10.7544235163063));
#25663=CARTESIAN_POINT('Ctrl Pts',(0.363248853322744,2.25095625141377,10.7540542574104));
#25664=CARTESIAN_POINT('Ctrl Pts',(0.365908817484673,2.24420689056688,10.7536849985146));
#25665=CARTESIAN_POINT('Ctrl Pts',(0.373429024201246,2.2251252091293,10.752641035867));
#25666=CARTESIAN_POINT('Ctrl Pts',(0.379474990869443,2.2053968350004,10.7515970732195));
#25667=CARTESIAN_POINT('Ctrl Pts',(0.38394414503024,2.18527475298703,10.7505531105719));
#25668=CARTESIAN_POINT('Ctrl Pts',(0.388405077700381,2.16518968771178,10.7495110684061));
#25669=CARTESIAN_POINT('Ctrl Pts',(0.391294739886095,2.14471304946467,10.7484690262404));
#25670=CARTESIAN_POINT('Ctrl Pts',(0.392560092755418,2.12411355585263,10.7474269840746));
#25671=CARTESIAN_POINT('Ctrl Pts',(0.393824086655637,2.10353618577312,10.7463860610457));
#25672=CARTESIAN_POINT('Ctrl Pts',(0.393467160705411,2.08283695116777,10.7453451380169));
#25673=CARTESIAN_POINT('Ctrl Pts',(0.391488006941209,2.06229018136877,10.744304214988));
#25674=CARTESIAN_POINT('Ctrl Pts',(0.389507836735216,2.04173285928432,10.7432627573682));
#25675=CARTESIAN_POINT('Ctrl Pts',(0.385903828800499,2.0213288923701,10.7422212997484));
#25676=CARTESIAN_POINT('Ctrl Pts',(0.380726643194315,2.00134852681288,10.7411798421287));
#25677=CARTESIAN_POINT('Ctrl Pts',(0.375547875732224,1.98136205638293,10.7401380662982));
#25678=CARTESIAN_POINT('Ctrl Pts',(0.368795193113627,1.9618001475528,10.7390962904676));
#25679=CARTESIAN_POINT('Ctrl Pts',(0.360569173342583,1.94291797927501,10.7380545146372));
#25680=CARTESIAN_POINT('Ctrl Pts',(0.352325372843132,1.92399499676199,10.7370104869846));
#25681=CARTESIAN_POINT('Ctrl Pts',(0.342602223638086,1.90575533803863,10.735966459332));
#25682=CARTESIAN_POINT('Ctrl Pts',(0.331546622878107,1.88843032623241,10.7349224316794));
#25683=CARTESIAN_POINT('Ctrl Pts',(0.327636401803429,1.8823026966486,10.7345531727835));
#25684=CARTESIAN_POINT('Ctrl Pts',(0.3235598867612,1.87628920687579,10.7341839138876));
#25685=CARTESIAN_POINT('Ctrl Pts',(0.319324789981441,1.87039911040393,10.7338146549918));
#25686=CARTESIAN_POINT('Ctrl Pts',(0.307351394360173,1.85374672700571,10.7327706923442));
#25687=CARTESIAN_POINT('Ctrl Pts',(0.294036215169403,1.83798384459672,10.7317267296967));
#25688=CARTESIAN_POINT('Ctrl Pts',(0.279536442238813,1.82333365318408,10.7306827670491));
#25689=CARTESIAN_POINT('Ctrl Pts',(0.265063343202964,1.80871041237719,10.7296407248833));
#25690=CARTESIAN_POINT('Ctrl Pts',(0.249410445497218,1.79519635840129,10.7285986827176));
#25691=CARTESIAN_POINT('Ctrl Pts',(0.232774980818624,1.78298154895198,10.7275566405518));
#25692=CARTESIAN_POINT('Ctrl Pts',(0.216157382367754,1.77077985801612,10.7265157175229));
#25693=CARTESIAN_POINT('Ctrl Pts',(0.198559884838435,1.75987509804229,10.7254747944941));
#25694=CARTESIAN_POINT('Ctrl Pts',(0.180212441220589,1.75041686821399,10.7244338714652));
#25695=CARTESIAN_POINT('Ctrl Pts',(0.1618555748339,1.74095378088536,10.7233924138454));
#25696=CARTESIAN_POINT('Ctrl Pts',(0.142748639516621,1.73293905931746,10.7223509562257));
#25697=CARTESIAN_POINT('Ctrl Pts',(0.123146286305556,1.72647639677103,10.7213094986059));
#25698=CARTESIAN_POINT('Ctrl Pts',(0.103537943720977,1.72001175959945,10.7202677227754));
#25699=CARTESIAN_POINT('Ctrl Pts',(0.0834345914179953,1.71510032133677,
10.7192259469449));
#25700=CARTESIAN_POINT('Ctrl Pts',(0.0631052331196161,1.71179564717417,
10.7181841711144));
#25701=CARTESIAN_POINT('Ctrl Pts',(0.0427319324519695,1.70848382988339,
10.7171401434618));
#25702=CARTESIAN_POINT('Ctrl Pts',(0.0221323844766809,1.7067857709853,10.7160961158092));
#25703=CARTESIAN_POINT('Ctrl Pts',(0.00158060790296777,1.7067031761142,
10.7150520881566));
#25704=CARTESIAN_POINT('Ctrl Pts',(-0.005688286083539,1.70667396339093,
10.7146828292607));
#25705=CARTESIAN_POINT('Ctrl Pts',(-0.0129512272027228,1.70684635955504,
10.7143135703649));
#25706=CARTESIAN_POINT('Ctrl Pts',(-0.0201962601851129,1.70721888910675,
10.713944311469));
#25707=CARTESIAN_POINT('Ctrl Pts',(-0.0406792976923341,1.70827209849846,
10.7129003488214));
#25708=CARTESIAN_POINT('Ctrl Pts',(-0.0611407585325059,1.71093500649694,
10.7118563861739));
#25709=CARTESIAN_POINT('Ctrl Pts',(-0.081307890856511,1.71519626186267,
10.7108124235263));
#25710=CARTESIAN_POINT('Ctrl Pts',(-0.101437923567479,1.71944967818997,
10.7097703813606));
#25711=CARTESIAN_POINT('Ctrl Pts',(-0.121273978469272,1.72529551323584,
10.7087283391948));
#25712=CARTESIAN_POINT('Ctrl Pts',(-0.140549486567197,1.73267081272284,
10.707686297029));
#25713=CARTESIAN_POINT('Ctrl Pts',(-0.159804293072227,1.74003819125405,
10.7066453740002));
#25714=CARTESIAN_POINT('Ctrl Pts',(-0.178499053880445,1.74893153863871,
10.7056044509713));
#25715=CARTESIAN_POINT('Ctrl Pts',(-0.196383505611462,1.75923848702685,
10.7045635279425));
#25716=CARTESIAN_POINT('Ctrl Pts',(-0.21427714233077,1.76955072879504,10.7035220703227));
#25717=CARTESIAN_POINT('Ctrl Pts',(-0.231358993051381,1.78127766850619,
10.7024806127029));
#25718=CARTESIAN_POINT('Ctrl Pts',(-0.247404023415605,1.79426132204484,
10.7014391550831));
#25719=CARTESIAN_POINT('Ctrl Pts',(-0.263453956236107,1.80724894265568,
10.7003973792526));
#25720=CARTESIAN_POINT('Ctrl Pts',(-0.278465889309764,1.82149355093451,
10.6993556034221));
#25721=CARTESIAN_POINT('Ctrl Pts',(-0.29224916748893,1.83679795954053,10.6983138275916));
#25722=CARTESIAN_POINT('Ctrl Pts',(-0.306062238536659,1.85213544897305,
10.697269799939));
#25723=CARTESIAN_POINT('Ctrl Pts',(-0.318640904390109,1.86853672776939,
10.6962257722865));
#25724=CARTESIAN_POINT('Ctrl Pts',(-0.329835399642932,1.88577231938335,
10.6951817446339));
#25725=CARTESIAN_POINT('Ctrl Pts',(-0.333794745879168,1.89186832221732,
10.694812485738));
#25726=CARTESIAN_POINT('Ctrl Pts',(-0.337581353358565,1.89806845430745,
10.6944432268421));
#25727=CARTESIAN_POINT('Ctrl Pts',(-0.341189991104376,1.90436186473441,
10.6940739679463));
#25728=CARTESIAN_POINT('Ctrl Pts',(-0.351815332896677,1.92289230240535,
10.6929867150118));
#25729=CARTESIAN_POINT('Ctrl Pts',(-0.360953204524888,1.94233564316304,
10.6918994620774));
#25730=CARTESIAN_POINT('Ctrl Pts',(-0.368457924284301,1.96243674897668,
10.690812209143));
#25731=CARTESIAN_POINT('Ctrl Pts',(-0.375943138005039,1.98248560860926,
10.6897277821632));
#25732=CARTESIAN_POINT('Ctrl Pts',(-0.381803353160854,2.00318825710798,
10.6886433551834));
#25733=CARTESIAN_POINT('Ctrl Pts',(-0.385939644202044,2.02426704130169,
10.6875589282036));
#25734=CARTESIAN_POINT('Ctrl Pts',(-0.390065058944618,2.04529039923331,
10.686477352704));
#25735=CARTESIAN_POINT('Ctrl Pts',(-0.392475396073696,2.06668730305621,
10.6853957772043));
#25736=CARTESIAN_POINT('Ctrl Pts',(-0.393121944047708,2.0881666949608,10.6843142017047));
#25737=CARTESIAN_POINT('Ctrl Pts',(-0.393241072234284,2.09212433013901,
10.6841149185376));
#25738=CARTESIAN_POINT('Ctrl Pts',(-0.393300461280009,2.09608473789163,
10.6839156353706));
#25739=CARTESIAN_POINT('Ctrl Pts',(-0.393299997302219,2.10004606598081,
10.6837163522035));
#25740=CARTESIAN_POINT('',(-0.393315863656476,2.10034160400655,10.558716360067));
#25741=CARTESIAN_POINT('Ctrl Pts',(-0.392657465061904,2.10004663893747,
10.6837163195403));
#25742=CARTESIAN_POINT('Ctrl Pts',(-0.392722889128489,2.16297443070521,
10.680545421168));
#25743=CARTESIAN_POINT('Ctrl Pts',(-0.348724163651497,2.357260709504,10.6707510749546));
#25744=CARTESIAN_POINT('Ctrl Pts',(-0.0435775851074158,2.56300757829187,
10.6543332809008));
#25745=CARTESIAN_POINT('Ctrl Pts',(0.365715727477674,2.38727518193357,10.6344629373778));
#25746=CARTESIAN_POINT('Ctrl Pts',(0.439514647802459,1.94800691513575,10.6145925938551));
#25747=CARTESIAN_POINT('Ctrl Pts',(0.110118713284817,1.64817161171085,10.5947222503322));
#25748=CARTESIAN_POINT('Ctrl Pts',(-0.293328879552519,1.75564368824555,
10.5760968659443));
#25749=CARTESIAN_POINT('Ctrl Pts',(-0.392508382890038,1.99416607365442,
10.5640949293972));
#25750=CARTESIAN_POINT('Ctrl Pts',(-0.39348003609742,2.1003401551118,10.558716440691));
#25751=CARTESIAN_POINT('',(-0.393299933137644,2.09977066634666,10.433716352199));
#25752=CARTESIAN_POINT('Ctrl Pts',(-0.393299851525698,2.10034174532072,
10.5587163522035));
#25753=CARTESIAN_POINT('Ctrl Pts',(-0.393278507363976,2.12490581431345,
10.5574714225646));
#25754=CARTESIAN_POINT('Ctrl Pts',(-0.390954482254135,2.14937301694214,
10.5562264929256));
#25755=CARTESIAN_POINT('Ctrl Pts',(-0.386389811003518,2.17340166178409,
10.5549815632866));
#25756=CARTESIAN_POINT('Ctrl Pts',(-0.382562007298867,2.19355140109584,
10.553937600639));
#25757=CARTESIAN_POINT('Ctrl Pts',(-0.377142379728278,2.21346094894873,
10.5528936379915));
#25758=CARTESIAN_POINT('Ctrl Pts',(-0.370179250805663,2.2328616282941,10.5518496753439));
#25759=CARTESIAN_POINT('Ctrl Pts',(-0.363228931309024,2.25222661799925,
10.5508076331781));
#25760=CARTESIAN_POINT('Ctrl Pts',(-0.354740936404027,2.27108389256192,
10.5497655910124));
#25761=CARTESIAN_POINT('Ctrl Pts',(-0.344813872178568,2.2891779150779,10.5487235488466));
#25762=CARTESIAN_POINT('Ctrl Pts',(-0.334897469464141,2.30725250489794,
10.5476826258178));
#25763=CARTESIAN_POINT('Ctrl Pts',(-0.323545392451628,2.32456481430114,
10.546641702789));
#25764=CARTESIAN_POINT('Ctrl Pts',(-0.310902985619106,2.34088217769924,
10.5456007797601));
#25765=CARTESIAN_POINT('Ctrl Pts',(-0.298254085975937,2.35720792126989,
10.5445593221404));
#25766=CARTESIAN_POINT('Ctrl Pts',(-0.284313970521364,2.37253710651023,
10.5435178645206));
#25767=CARTESIAN_POINT('Ctrl Pts',(-0.269269747056953,2.38666826353799,
10.5424764069009));
#25768=CARTESIAN_POINT('Ctrl Pts',(-0.254220926926409,2.40080373825028,
10.5414346310704));
#25769=CARTESIAN_POINT('Ctrl Pts',(-0.238067887808363,2.41373997908236,
10.5403928552399));
#25770=CARTESIAN_POINT('Ctrl Pts',(-0.221031903480885,2.42531490535113,
10.5393510794095));
#25771=CARTESIAN_POINT('Ctrl Pts',(-0.203959095486683,2.43691485108571,
10.5383070517569));
#25772=CARTESIAN_POINT('Ctrl Pts',(-0.18600017194333,2.44714724308179,10.5372630241043));
#25773=CARTESIAN_POINT('Ctrl Pts',(-0.167402837751568,2.45589490009372,
10.5362189964518));
#25774=CARTESIAN_POINT('Ctrl Pts',(-0.160825204415708,2.45898883171742,
10.5358497375558));
#25775=CARTESIAN_POINT('Ctrl Pts',(-0.154167889700035,2.46189747314211,
10.5354804786599));
#25776=CARTESIAN_POINT('Ctrl Pts',(-0.147442354877446,2.46461711697093,
10.535111219764));
#25777=CARTESIAN_POINT('Ctrl Pts',(-0.128428033985807,2.47230604905385,
10.5340672571164));
#25778=CARTESIAN_POINT('Ctrl Pts',(-0.108753987352186,2.47852652715294,
10.5330232944689));
#25779=CARTESIAN_POINT('Ctrl Pts',(-0.0886722812995241,2.48317374196197,
10.5319793318213));
#25780=CARTESIAN_POINT('Ctrl Pts',(-0.0686275177090747,2.48781240771859,
10.5309372896556));
#25781=CARTESIAN_POINT('Ctrl Pts',(-0.0481772786181898,2.49088333308022,
10.5298952474898));
#25782=CARTESIAN_POINT('Ctrl Pts',(-0.0275898012882309,2.49233110106755,
10.528853205324));
#25783=CARTESIAN_POINT('Ctrl Pts',(-0.00702443458549785,2.49377731417481,
10.5278122822952));
#25784=CARTESIAN_POINT('Ctrl Pts',(0.0136771495331234,2.49360375046415,
10.5267713592663));
#25785=CARTESIAN_POINT('Ctrl Pts',(0.0342406440830859,2.49180667208813,
10.5257304362375));
#25786=CARTESIAN_POINT('Ctrl Pts',(0.0548146995078923,2.49000867077949,
10.5246889786177));
#25787=CARTESIAN_POINT('Ctrl Pts',(0.0752497892952924,2.4865855370673,10.5236475209979));
#25788=CARTESIAN_POINT('Ctrl Pts',(0.0952752291272609,2.48158553525356,
10.5226060633781));
#25789=CARTESIAN_POINT('Ctrl Pts',(0.115306787604137,2.47658400572129,10.5215642875475));
#25790=CARTESIAN_POINT('Ctrl Pts',(0.13492774245287,2.47000486212578,10.520522511717));
#25791=CARTESIAN_POINT('Ctrl Pts',(0.153882033838918,2.46194641821905,10.5194807358865));
#25792=CARTESIAN_POINT('Ctrl Pts',(0.172877295355929,2.45387055580294,10.5184367082339));
#25793=CARTESIAN_POINT('Ctrl Pts',(0.191202363562223,2.44430935001895,10.5173926805813));
#25794=CARTESIAN_POINT('Ctrl Pts',(0.208624623229872,2.43340764325701,10.5163486529287));
#25795=CARTESIAN_POINT('Ctrl Pts',(0.214786648107508,2.42955185247228,10.5159793940328));
#25796=CARTESIAN_POINT('Ctrl Pts',(0.220836010639008,2.42552876322413,10.515610135137));
#25797=CARTESIAN_POINT('Ctrl Pts',(0.226763389384609,2.4213460054751,10.5152408762411));
#25798=CARTESIAN_POINT('Ctrl Pts',(0.24352117661115,2.40952058189637,10.5141969135936));
#25799=CARTESIAN_POINT('Ctrl Pts',(0.259401382900948,2.39634554842707,10.513152950946));
#25800=CARTESIAN_POINT('Ctrl Pts',(0.27417943465761,2.38197611177338,10.5121089882984));
#25801=CARTESIAN_POINT('Ctrl Pts',(0.288930300595645,2.3676331092468,10.5110669461327));
#25802=CARTESIAN_POINT('Ctrl Pts',(0.302582473555006,2.35210052945659,10.5100249039669));
#25803=CARTESIAN_POINT('Ctrl Pts',(0.314944156270969,2.33557391288249,10.5089828618011));
#25804=CARTESIAN_POINT('Ctrl Pts',(0.32729256273389,2.31906504563497,10.5079419387722));
#25805=CARTESIAN_POINT('Ctrl Pts',(0.338352768795716,2.30156482988624,10.5069010157434));
#25806=CARTESIAN_POINT('Ctrl Pts',(0.347973144280237,2.28330188449584,10.5058600927145));
#25807=CARTESIAN_POINT('Ctrl Pts',(0.35759846053887,2.26502955973267,10.5048186350947));
#25808=CARTESIAN_POINT('Ctrl Pts',(0.365782111765119,2.24599436623121,10.5037771774749));
#25809=CARTESIAN_POINT('Ctrl Pts',(0.37241815313595,2.22645002655123,10.5027357198551));
#25810=CARTESIAN_POINT('Ctrl Pts',(0.379056222106729,2.20689971522342,10.5016939440246));
#25811=CARTESIAN_POINT('Ctrl Pts',(0.384145537763884,2.18684065577966,10.5006521681941));
#25812=CARTESIAN_POINT('Ctrl Pts',(0.387630154255204,2.16654136692379,10.4996103923636));
#25813=CARTESIAN_POINT('Ctrl Pts',(0.391122302824145,2.14619820069441,10.498566364711));
#25814=CARTESIAN_POINT('Ctrl Pts',(0.393002760346493,2.1256145017966,10.4975223370585));
#25815=CARTESIAN_POINT('Ctrl Pts',(0.393267394071057,2.10506426308162,10.4964783094059));
#25816=CARTESIAN_POINT('Ctrl Pts',(0.393360991550679,2.09779591301583,10.49610905051));
#25817=CARTESIAN_POINT('Ctrl Pts',(0.393252935323244,2.09053172978668,10.4957397916141));
#25818=CARTESIAN_POINT('Ctrl Pts',(0.392944594934099,2.08328368126421,10.4953705327183));
#25819=CARTESIAN_POINT('Ctrl Pts',(0.39207286008191,2.06279211827132,10.4943265700707));
#25820=CARTESIAN_POINT('Ctrl Pts',(0.389591298651868,2.04230787282293,10.4932826074232));
#25821=CARTESIAN_POINT('Ctrl Pts',(0.385508845475885,2.02210378661417,10.4922386447756));
#25822=CARTESIAN_POINT('Ctrl Pts',(0.381433902412427,2.00193686799911,10.4911966026099));
#25823=CARTESIAN_POINT('Ctrl Pts',(0.375763999125586,1.98204981044483,10.4901545604441));
#25824=CARTESIAN_POINT('Ctrl Pts',(0.368559726226817,1.9627097301204,10.4891125182784));
#25825=CARTESIAN_POINT('Ctrl Pts',(0.361363190603966,1.94339042073842,10.4880715952495));
#25826=CARTESIAN_POINT('Ctrl Pts',(0.3526357852584,1.92461761846187,10.4870306722207));
#25827=CARTESIAN_POINT('Ctrl Pts',(0.342487656866335,1.90664257217731,10.4859897491918));
#25828=CARTESIAN_POINT('Ctrl Pts',(0.332334316660019,1.88865829437746,10.484948291572));
#25829=CARTESIAN_POINT('Ctrl Pts',(0.320759143428588,1.87147323971675,10.4839068339522));
#25830=CARTESIAN_POINT('Ctrl Pts',(0.307918121796048,1.85531383310536,10.4828653763325));
#25831=CARTESIAN_POINT('Ctrl Pts',(0.295073176671582,1.83914948909075,10.481823600502));
#25832=CARTESIAN_POINT('Ctrl Pts',(0.280962098869543,1.82401197004405,10.4807818246715));
#25833=CARTESIAN_POINT('Ctrl Pts',(0.26578037922311,1.81009367026569,10.479740048841));
#25834=CARTESIAN_POINT('Ctrl Pts',(0.250565843945142,1.7961452857665,10.4786960211884));
#25835=CARTESIAN_POINT('Ctrl Pts',(0.234276627008033,1.78342183527605,10.4776519935358));
#25836=CARTESIAN_POINT('Ctrl Pts',(0.217140869373926,1.77207511096665,10.4766079658832));
#25837=CARTESIAN_POINT('Ctrl Pts',(0.21108017650993,1.76806192330841,10.4762387069873));
#25838=CARTESIAN_POINT('Ctrl Pts',(0.204913828401495,1.76422054528154,10.4758694480915));
#25839=CARTESIAN_POINT('Ctrl Pts',(0.198652629207673,1.76055630377207,10.4755001891956));
#25840=CARTESIAN_POINT('Ctrl Pts',(0.180951070327685,1.75019682073656,10.474456226548));
#25841=CARTESIAN_POINT('Ctrl Pts',(0.162384235955808,1.74119486982972,10.4734122639005));
#25842=CARTESIAN_POINT('Ctrl Pts',(0.143186372860344,1.73369063262442,10.4723683012529));
#25843=CARTESIAN_POINT('Ctrl Pts',(0.124023826302726,1.72620020027209,10.4713262590872));
#25844=CARTESIAN_POINT('Ctrl Pts',(0.104233211147734,1.72020233288133,10.4702842169214));
#25845=CARTESIAN_POINT('Ctrl Pts',(0.0840719222456602,1.71579067958999,
10.4692421747556));
#25846=CARTESIAN_POINT('Ctrl Pts',(0.0639322862511359,1.71138376434499,
10.4682012517268));
#25847=CARTESIAN_POINT('Ctrl Pts',(0.0434234757737663,1.70855986594305,
10.4671603286979));
#25848=CARTESIAN_POINT('Ctrl Pts',(0.0228163697618803,1.70736237664879,
10.466119405669));
#25849=CARTESIAN_POINT('Ctrl Pts',(0.00219868047744025,1.70616427235523,
10.4650779480493));
#25850=CARTESIAN_POINT('Ctrl Pts',(-0.0185166715893972,1.7065943046525,
10.4640364904295));
#25851=CARTESIAN_POINT('Ctrl Pts',(-0.0390548670247227,1.70864388677104,
10.4629950328097));
#25852=CARTESIAN_POINT('Ctrl Pts',(-0.0595993377741394,1.71069409512627,
10.4619532569792));
#25853=CARTESIAN_POINT('Ctrl Pts',(-0.079965816201812,1.7143647294148,10.4609114811487));
#25854=CARTESIAN_POINT('Ctrl Pts',(-0.0998867110149369,1.71959556395513,
10.4598697053182));
#25855=CARTESIAN_POINT('Ctrl Pts',(-0.119850665294266,1.72483770506302,
10.4588256776656));
#25856=CARTESIAN_POINT('Ctrl Pts',(-0.139366417727724,1.73164653666351,
10.457781650013));
#25857=CARTESIAN_POINT('Ctrl Pts',(-0.158182841914016,1.73991240159649,
10.4567376223604));
#25858=CARTESIAN_POINT('Ctrl Pts',(-0.164837964507673,1.74283592967638,
10.4563683634645));
#25859=CARTESIAN_POINT('Ctrl Pts',(-0.171405819580025,1.74594129823533,
10.4559991045686));
#25860=CARTESIAN_POINT('Ctrl Pts',(-0.177876079703393,1.74922230648265,
10.4556298456728));
#25861=CARTESIAN_POINT('Ctrl Pts',(-0.196168692188443,1.75849831877336,
10.4545858830252));
#25862=CARTESIAN_POINT('Ctrl Pts',(-0.213788256612227,1.76923672686017,
10.4535419203776));
#25863=CARTESIAN_POINT('Ctrl Pts',(-0.23049010379015,1.78131645468458,10.4524979577301));
#25864=CARTESIAN_POINT('Ctrl Pts',(-0.247161226120462,1.79337396054799,
10.4514559155643));
#25865=CARTESIAN_POINT('Ctrl Pts',(-0.262917357987864,1.80676751011588,
10.4504138733986));
#25866=CARTESIAN_POINT('Ctrl Pts',(-0.277540425037224,1.82133137516011,
10.4493718312328));
#25867=CARTESIAN_POINT('Ctrl Pts',(-0.292147787142294,1.83587959884206,
10.4483309082039));
#25868=CARTESIAN_POINT('Ctrl Pts',(-0.305623961160892,1.85159514665949,
10.4472899851751));
#25869=CARTESIAN_POINT('Ctrl Pts',(-0.31778583043083,1.86827374775959,10.4462490621462));
#25870=CARTESIAN_POINT('Ctrl Pts',(-0.329953945719849,1.88496091455451,
10.4452076045264));
#25871=CARTESIAN_POINT('Ctrl Pts',(-0.340805961241281,1.90261153772065,
10.4441661469066));
#25872=CARTESIAN_POINT('Ctrl Pts',(-0.350200332190293,1.92098989600079,
10.4431246892868));
#25873=CARTESIAN_POINT('Ctrl Pts',(-0.359597573529192,1.93937386967062,
10.4420829134563));
#25874=CARTESIAN_POINT('Ctrl Pts',(-0.367535981270759,1.95848535004642,
10.4410411376258));
#25875=CARTESIAN_POINT('Ctrl Pts',(-0.373921342244449,1.97806674032853,
10.4399993617953));
#25876=CARTESIAN_POINT('Ctrl Pts',(-0.380320505320784,1.99769045623009,
10.4389553341427));
#25877=CARTESIAN_POINT('Ctrl Pts',(-0.385159747222649,2.01778539386682,
10.4379113064901));
#25878=CARTESIAN_POINT('Ctrl Pts',(-0.388395330395011,2.03808104226208,
10.4368672788375));
#25879=CARTESIAN_POINT('Ctrl Pts',(-0.389539713751837,2.04525934706906,
10.4364980199417));
#25880=CARTESIAN_POINT('Ctrl Pts',(-0.390483962892018,2.05246270931861,
10.4361287610458));
#25881=CARTESIAN_POINT('Ctrl Pts',(-0.391227701128192,2.05967908892461,
10.4357595021499));
#25882=CARTESIAN_POINT('Ctrl Pts',(-0.392599429522958,2.07298876204814,
10.4350784521678));
#25883=CARTESIAN_POINT('Ctrl Pts',(-0.393292118961807,2.08636960809798,
10.4343974021856));
#25884=CARTESIAN_POINT('Ctrl Pts',(-0.393299933137593,2.09977066625803,
10.4337163522035));
#25885=CARTESIAN_POINT('',(-0.393113345386621,2.09978390338552,10.3087163551585));
#25886=CARTESIAN_POINT('Ctrl Pts',(-0.393299933137644,2.09977066634666,
10.433716352199));
#25887=CARTESIAN_POINT('Ctrl Pts',(-0.393311752893345,2.12004117204569,
10.4326861926862));
#25888=CARTESIAN_POINT('Ctrl Pts',(-0.391752186310895,2.14037481072923,
10.4316560331735));
#25889=CARTESIAN_POINT('Ctrl Pts',(-0.388618245869949,2.16050412363603,
10.4306258736607));
#25890=CARTESIAN_POINT('Ctrl Pts',(-0.385489406275611,2.18060067378317,
10.4295973908504));
#25891=CARTESIAN_POINT('Ctrl Pts',(-0.380791337052907,2.20049280953543,
10.4285689080402));
#25892=CARTESIAN_POINT('Ctrl Pts',(-0.374572916412325,2.2199167223133,10.4275404252299));
#25893=CARTESIAN_POINT('Ctrl Pts',(-0.3683544003717,2.23934093308357,10.4265119266411));
#25894=CARTESIAN_POINT('Ctrl Pts',(-0.360615672076591,2.25829617333842,
10.4254834280523));
#25895=CARTESIAN_POINT('Ctrl Pts',(-0.351455954974451,2.27653215489818,
10.4244549294635));
#25896=CARTESIAN_POINT('Ctrl Pts',(-0.342297215870464,2.29476618937202,
10.4234265406892));
#25897=CARTESIAN_POINT('Ctrl Pts',(-0.331718144692482,2.31228044926094,
10.4223981519149));
#25898=CARTESIAN_POINT('Ctrl Pts',(-0.319864204852919,2.32884881571424,
10.4213697631407));
#25899=CARTESIAN_POINT('Ctrl Pts',(-0.307983831395344,2.34545412869129,
10.4203390811173));
#25900=CARTESIAN_POINT('Ctrl Pts',(-0.294823383852538,2.36110874111289,
10.419308399094));
#25901=CARTESIAN_POINT('Ctrl Pts',(-0.280569475804279,2.37561868450254,
10.4182777170707));
#25902=CARTESIAN_POINT('Ctrl Pts',(-0.269558549170975,2.38682739453322,
10.4174815309229));
#25903=CARTESIAN_POINT('Ctrl Pts',(-0.257896023166036,2.39735367684374,
10.416685344775));
#25904=CARTESIAN_POINT('Ctrl Pts',(-0.245681167609966,2.40712481808184,
10.4158891586271));
#25905=CARTESIAN_POINT('Ctrl Pts',(-0.229664997296023,2.41993677983715,
10.4148451959796));
#25906=CARTESIAN_POINT('Ctrl Pts',(-0.212596216216608,2.43153070804052,
10.413801233332));
#25907=CARTESIAN_POINT('Ctrl Pts',(-0.194686320575257,2.44173399974376,
10.4127572706845));
#25908=CARTESIAN_POINT('Ctrl Pts',(-0.176809372116842,2.45191852139245,
10.4117152285187));
#25909=CARTESIAN_POINT('Ctrl Pts',(-0.158094983118191,2.46071707274236,
10.4106731863529));
#25910=CARTESIAN_POINT('Ctrl Pts',(-0.138784287729845,2.46799974385768,
10.4096311441872));
#25911=CARTESIAN_POINT('Ctrl Pts',(-0.119494331724977,2.47527459349864,
10.4085902211583));
#25912=CARTESIAN_POINT('Ctrl Pts',(-0.0996100154754499,2.48103650955752,
10.4075492981295));
#25913=CARTESIAN_POINT('Ctrl Pts',(-0.0793930877577652,2.48520335878116,
10.4065083751006));
#25914=CARTESIAN_POINT('Ctrl Pts',(-0.059165777152929,2.48937234798996,
10.4054669174808));
#25915=CARTESIAN_POINT('Ctrl Pts',(-0.0386062311956818,2.49194446949978,
10.404425459861));
#25916=CARTESIAN_POINT('Ctrl Pts',(-0.0179876193114655,2.49288845179199,
10.4033840022412));
#25917=CARTESIAN_POINT('Ctrl Pts',(0.00263729245758782,2.49383272251194,
10.4023422264108));
#25918=CARTESIAN_POINT('Ctrl Pts',(0.0233205700375492,2.49314786619447,
10.4013004505803));
#25919=CARTESIAN_POINT('Ctrl Pts',(0.0437887236061861,2.49085475267027,
10.4002586747498));
#25920=CARTESIAN_POINT('Ctrl Pts',(0.0643011195532388,2.48855668252915,
10.3992146470972));
#25921=CARTESIAN_POINT('Ctrl Pts',(0.0845967399894148,2.48464355437913,
10.3981706194446));
#25922=CARTESIAN_POINT('Ctrl Pts',(0.104411233674789,2.4791875318131,10.397126591792));
#25923=CARTESIAN_POINT('Ctrl Pts',(0.111419360367839,2.47725780814768,10.3967573328961));
#25924=CARTESIAN_POINT('Ctrl Pts',(0.118367451388828,2.47513552981942,10.3963880740002));
#25925=CARTESIAN_POINT('Ctrl Pts',(0.125244390719619,2.47282533791746,10.3960188151044));
#25926=CARTESIAN_POINT('Ctrl Pts',(0.144686759938549,2.46629400155344,10.3949748524568));
#25927=CARTESIAN_POINT('Ctrl Pts',(0.163674781965691,2.45821826764132,10.3939308898093));
#25928=CARTESIAN_POINT('Ctrl Pts',(0.181948842435384,2.44868253288116,10.3928869271617));
#25929=CARTESIAN_POINT('Ctrl Pts',(0.2001892858017,2.43916434013263,10.3918448849959));
#25930=CARTESIAN_POINT('Ctrl Pts',(0.217717702221878,2.42819176161839,10.3908028428302));
#25931=CARTESIAN_POINT('Ctrl Pts',(0.23429433082323,2.41589722465399,10.3897608006644));
#25932=CARTESIAN_POINT('Ctrl Pts',(0.25085315638588,2.40361589182915,10.3887198776355));
#25933=CARTESIAN_POINT('Ctrl Pts',(0.266461618244414,2.39001583198399,10.3876789546067));
#25934=CARTESIAN_POINT('Ctrl Pts',(0.280908967946815,2.37527266796225,10.3866380315778));
#25935=CARTESIAN_POINT('Ctrl Pts',(0.295363737431475,2.36052193223573,10.385596573958));
#25936=CARTESIAN_POINT('Ctrl Pts',(0.308655676963265,2.34462743373741,10.3845551163382));
#25937=CARTESIAN_POINT('Ctrl Pts',(0.320610621343578,2.32780193037304,10.3835136587185));
#25938=CARTESIAN_POINT('Ctrl Pts',(0.332569218480592,2.31097128608387,10.382471882888));
#25939=CARTESIAN_POINT('Ctrl Pts',(0.343189610904075,2.29320969087407,10.3814301070575));
#25940=CARTESIAN_POINT('Ctrl Pts',(0.352341301358908,2.27475839709929,10.380388331227));
#25941=CARTESIAN_POINT('Ctrl Pts',(0.361512773400334,2.2562672204343,10.3793443035744));
#25942=CARTESIAN_POINT('Ctrl Pts',(0.369208931250333,2.23708405241762,10.3783002759218));
#25943=CARTESIAN_POINT('Ctrl Pts',(0.375347353247155,2.21747022776157,10.3772562482692));
#25944=CARTESIAN_POINT('Ctrl Pts',(0.377518432646495,2.21053307507395,10.3768869893733));
#25945=CARTESIAN_POINT('Ctrl Pts',(0.379495110243685,2.20354216813606,10.3765177304774));
#25946=CARTESIAN_POINT('Ctrl Pts',(0.381275271048106,2.19650936580039,10.3761484715816));
#25947=CARTESIAN_POINT('Ctrl Pts',(0.386308112253202,2.17662634326987,10.375104508934));
#25948=CARTESIAN_POINT('Ctrl Pts',(0.389796450003931,2.15628933369475,10.3740605462865));
#25949=CARTESIAN_POINT('Ctrl Pts',(0.391670712609699,2.13576231094058,10.3730165836389));
#25950=CARTESIAN_POINT('Ctrl Pts',(0.39354152730744,2.11527304985668,10.3719745414731));
#25951=CARTESIAN_POINT('Ctrl Pts',(0.393804035362039,2.09459518848343,10.3709324993074));
#25952=CARTESIAN_POINT('Ctrl Pts',(0.392439797138852,2.07400200735409,10.3698904571416));
#25953=CARTESIAN_POINT('Ctrl Pts',(0.391077024086084,2.05343094297776,10.3688495341127));
#25954=CARTESIAN_POINT('Ctrl Pts',(0.388090992698617,2.03294511065555,10.3678086110839));
#25955=CARTESIAN_POINT('Ctrl Pts',(0.383515287862834,2.01281677927785,10.366767688055));
#25956=CARTESIAN_POINT('Ctrl Pts',(0.378937233064304,1.99267811051376,10.3657262304352));
#25957=CARTESIAN_POINT('Ctrl Pts',(0.372768021184381,1.97289803053894,10.3646847728154));
#25958=CARTESIAN_POINT('Ctrl Pts',(0.365092264110561,1.95373815026937,10.3636433151957));
#25959=CARTESIAN_POINT('Ctrl Pts',(0.357414161758318,1.93457241582108,10.3626015393652));
#25960=CARTESIAN_POINT('Ctrl Pts',(0.348228904812652,1.91602792730111,10.3615597635347));
#25961=CARTESIAN_POINT('Ctrl Pts',(0.337668702051527,1.89834500339729,10.3605179877042));
#25962=CARTESIAN_POINT('Ctrl Pts',(0.327085673172499,1.88062385745219,10.3594739600516));
#25963=CARTESIAN_POINT('Ctrl Pts',(0.315122191346237,1.86376859467168,10.358429932399));
#25964=CARTESIAN_POINT('Ctrl Pts',(0.301953375143129,1.84798998186645,10.3573859047464));
#25965=CARTESIAN_POINT('Ctrl Pts',(0.297295737465664,1.84240929333938,10.3570166458505));
#25966=CARTESIAN_POINT('Ctrl Pts',(0.29248766904401,1.83696296318126,10.3566473869546));
#25967=CARTESIAN_POINT('Ctrl Pts',(0.287537996131034,1.83165918912519,10.3562781280588));
#25968=CARTESIAN_POINT('Ctrl Pts',(0.273544362676087,1.81666444677083,10.3552341654112));
#25969=CARTESIAN_POINT('Ctrl Pts',(0.258332941158418,1.80272259918402,10.3541902027637));
#25970=CARTESIAN_POINT('Ctrl Pts',(0.242088025117285,1.79003503731097,10.3531462401161));
#25971=CARTESIAN_POINT('Ctrl Pts',(0.225872993349701,1.77737081557515,10.3521041979503));
#25972=CARTESIAN_POINT('Ctrl Pts',(0.208628777635873,1.76595679411621,10.3510621557846));
#25973=CARTESIAN_POINT('Ctrl Pts',(0.190575175433659,1.75595640899963,10.3500201136188));
#25974=CARTESIAN_POINT('Ctrl Pts',(0.172540962516603,1.74596676413956,10.3489791905899));
#25975=CARTESIAN_POINT('Ctrl Pts',(0.153699715169682,1.73738812160169,10.3479382675611));
#25976=CARTESIAN_POINT('Ctrl Pts',(0.134298542056594,1.73033962668218,10.3468973445322));
#25977=CARTESIAN_POINT('Ctrl Pts',(0.114887405006638,1.72328751183938,10.3458558869124));
#25978=CARTESIAN_POINT('Ctrl Pts',(0.0949164537524642,1.71776738095022,
10.3448144292927));
#25979=CARTESIAN_POINT('Ctrl Pts',(0.0746514573797654,1.71384970554061,
10.3437729716729));
#25980=CARTESIAN_POINT('Ctrl Pts',(0.0543802691671996,1.70993083311036,
10.3427311958424));
#25981=CARTESIAN_POINT('Ctrl Pts',(0.0338155856402103,1.70761549489314,
10.3416894200119));
#25982=CARTESIAN_POINT('Ctrl Pts',(0.0132310380546688,1.70692261622933,
10.3406476441814));
#25983=CARTESIAN_POINT('Ctrl Pts',(-0.00739800349760471,1.70622823989256,
10.3396036165288));
#25984=CARTESIAN_POINT('Ctrl Pts',(-0.0280462591055306,1.70716329131249,
10.3385595888762));
#25985=CARTESIAN_POINT('Ctrl Pts',(-0.0484417174146762,1.7096946195427,
10.3375155612236));
#25986=CARTESIAN_POINT('Ctrl Pts',(-0.0556553236799815,1.7105899171577,
10.3371463023277));
#25987=CARTESIAN_POINT('Ctrl Pts',(-0.0628373899030118,1.71168443024859,
10.3367770434319));
#25988=CARTESIAN_POINT('Ctrl Pts',(-0.0699762454728388,1.712975175125,10.336407784536));
#25989=CARTESIAN_POINT('Ctrl Pts',(-0.0901590999540693,1.71662434770709,
10.3353638218884));
#25990=CARTESIAN_POINT('Ctrl Pts',(-0.110115872345704,1.72186740925833,
10.3343198592409));
#25991=CARTESIAN_POINT('Ctrl Pts',(-0.129577468111601,1.72865841902934,
10.3332758965933));
#25992=CARTESIAN_POINT('Ctrl Pts',(-0.149003262174993,1.73543693600612,
10.3322338544276));
#25993=CARTESIAN_POINT('Ctrl Pts',(-0.167934981327794,1.74375756527136,
10.3311918122618));
#25994=CARTESIAN_POINT('Ctrl Pts',(-0.186116225264505,1.75352396808251,
10.330149770096));
#25995=CARTESIAN_POINT('Ctrl Pts',(-0.204277942830833,1.76327988193045,
10.3291088470672));
#25996=CARTESIAN_POINT('Ctrl Pts',(-0.221690126700608,1.77447816582868,
10.3280679240384));
#25997=CARTESIAN_POINT('Ctrl Pts',(-0.238118832990956,1.78697554189005,
10.3270270010095));
#25998=CARTESIAN_POINT('Ctrl Pts',(-0.25455597663667,1.79947933627805,10.3259855433897));
#25999=CARTESIAN_POINT('Ctrl Pts',(-0.270008038288877,1.81328312306739,
10.3249440857699));
#26000=CARTESIAN_POINT('Ctrl Pts',(-0.284271898618622,1.82820158636268,
10.3239026281501));
#26001=CARTESIAN_POINT('Ctrl Pts',(-0.298540117179546,1.8431246078989,10.3228608523196));
#26002=CARTESIAN_POINT('Ctrl Pts',(-0.311618929780691,1.85916242759387,
10.3218190764891));
#26003=CARTESIAN_POINT('Ctrl Pts',(-0.323344302114012,1.87609521601716,
10.3207773006586));
#26004=CARTESIAN_POINT('Ctrl Pts',(-0.335095019105724,1.8930646050469,10.319733273006));
#26005=CARTESIAN_POINT('Ctrl Pts',(-0.345486084981204,1.91093218828524,
10.3186892453535));
#26006=CARTESIAN_POINT('Ctrl Pts',(-0.354398128988664,1.92945130850888,
10.3176452177008));
#26007=CARTESIAN_POINT('Ctrl Pts',(-0.35755020213726,1.93600127858799,10.317275958805));
#26008=CARTESIAN_POINT('Ctrl Pts',(-0.360517698152115,1.94263256817154,
10.3169066999091));
#26009=CARTESIAN_POINT('Ctrl Pts',(-0.363296808260951,1.94933374927541,
10.3165374410132));
#26010=CARTESIAN_POINT('Ctrl Pts',(-0.372070135350239,1.97048859791629,
10.3153717336655));
#26011=CARTESIAN_POINT('Ctrl Pts',(-0.379006803815233,1.99244781540974,
10.3142060263177));
#26012=CARTESIAN_POINT('Ctrl Pts',(-0.383982339767975,2.01489739871008,
10.3130403189699));
#26013=CARTESIAN_POINT('Ctrl Pts',(-0.38891919674824,2.03717246275805,10.3118836736334));
#26014=CARTESIAN_POINT('Ctrl Pts',(-0.391925091309735,2.05992990768128,
10.3107270282968));
#26015=CARTESIAN_POINT('Ctrl Pts',(-0.392925589507551,2.08284275342185,
10.3095703829602));
#26016=CARTESIAN_POINT('Ctrl Pts',(-0.393171833720999,2.08848209958914,
10.3092857075637));
#26017=CARTESIAN_POINT('Ctrl Pts',(-0.393296832619217,2.09413077860865,
10.3090010321673));
#26018=CARTESIAN_POINT('Ctrl Pts',(-0.393299940559465,2.09978376882535,
10.3087163567708));
#26019=CARTESIAN_POINT('',(-0.393225507384553,2.10032482688042,10.1837163490571));
#26020=CARTESIAN_POINT('Ctrl Pts',(-0.392771343913059,2.09978415001449,
10.3087163522035));
#26021=CARTESIAN_POINT('Ctrl Pts',(-0.392375286529236,2.17943390890476,
10.3046999339658));
#26022=CARTESIAN_POINT('Ctrl Pts',(-0.330116542795512,2.39100262904427,
10.2940600678871));
#26023=CARTESIAN_POINT('Ctrl Pts',(0.0156496755916217,2.56479039483764,
10.2767967539677));
#26024=CARTESIAN_POINT('Ctrl Pts',(0.399275537934642,2.33844091151996,10.2569264104448));
#26025=CARTESIAN_POINT('Ctrl Pts',(0.416620450678848,1.89335435268158,10.2370560669221));
#26026=CARTESIAN_POINT('Ctrl Pts',(0.0517728176779485,1.63783704299332,
10.2171857233993));
#26027=CARTESIAN_POINT('Ctrl Pts',(-0.31718930511009,1.78856927240169,10.1994058184931));
#26028=CARTESIAN_POINT('Ctrl Pts',(-0.392294407528429,2.01055654884596,
10.1882493614278));
#26029=CARTESIAN_POINT('Ctrl Pts',(-0.392991088827784,2.10032457091715,
10.1837163522035));
#26030=CARTESIAN_POINT('',(-0.393299995369781,2.10006035006603,10.0587163522072));
#26031=CARTESIAN_POINT('Ctrl Pts',(-0.393299865795482,2.10032490807289,
10.1837163480591));
#26032=CARTESIAN_POINT('Ctrl Pts',(-0.39327953168376,2.12493926542058,10.1824743656741));
#26033=CARTESIAN_POINT('Ctrl Pts',(-0.390944445826951,2.14945349782272,
10.1812323832891));
#26034=CARTESIAN_POINT('Ctrl Pts',(-0.386374291577607,2.17348330972338,
10.1799904009042));
#26035=CARTESIAN_POINT('Ctrl Pts',(-0.383252210631985,2.1898991709326,10.179141946054));
#26036=CARTESIAN_POINT('Ctrl Pts',(-0.379088103166932,2.2060893872349,10.1782934912039));
#26037=CARTESIAN_POINT('Ctrl Pts',(-0.373920092839562,2.22193709103818,
10.1774450363537));
#26038=CARTESIAN_POINT('Ctrl Pts',(-0.367561227965505,2.24143655033984,
10.1764010737061));
#26039=CARTESIAN_POINT('Ctrl Pts',(-0.359654001645914,2.2604953601309,10.1753571110586));
#26040=CARTESIAN_POINT('Ctrl Pts',(-0.350280507675885,2.27885316866727,
10.174313148411));
#26041=CARTESIAN_POINT('Ctrl Pts',(-0.340924257258063,2.29717720603669,
10.1732711062453));
#26042=CARTESIAN_POINT('Ctrl Pts',(-0.330107371188117,2.31480212694996,
10.1722290640795));
#26043=CARTESIAN_POINT('Ctrl Pts',(-0.317960147849274,2.33148700693488,
10.1711870219137));
#26044=CARTESIAN_POINT('Ctrl Pts',(-0.305825970437466,2.34815396762081,
10.1701460988849));
#26045=CARTESIAN_POINT('Ctrl Pts',(-0.292364699674248,2.3638822828141,10.169105175856));
#26046=CARTESIAN_POINT('Ctrl Pts',(-0.277750084760658,2.37845965671071,
10.1680642528272));
#26047=CARTESIAN_POINT('Ctrl Pts',(-0.263127964161756,2.39304451716662,
10.1670227952074));
#26048=CARTESIAN_POINT('Ctrl Pts',(-0.247351825627305,2.40647672443016,
10.1659813375876));
#26049=CARTESIAN_POINT('Ctrl Pts',(-0.230632876008127,2.41858023558316,
10.1649398799678));
#26050=CARTESIAN_POINT('Ctrl Pts',(-0.213908818020965,2.43068744488648,
10.1638981041373));
#26051=CARTESIAN_POINT('Ctrl Pts',(-0.196241992178396,2.44146474808682,
10.1628563283068));
#26052=CARTESIAN_POINT('Ctrl Pts',(-0.177872485462133,2.45077951610025,
10.1618145524763));
#26053=CARTESIAN_POINT('Ctrl Pts',(-0.159463272640243,2.46011441819611,
10.1607705248237));
#26054=CARTESIAN_POINT('Ctrl Pts',(-0.140349027678615,2.46798019345056,
10.1597264971711));
#26055=CARTESIAN_POINT('Ctrl Pts',(-0.120790344968437,2.4742921086029,10.1586824695185));
#26056=CARTESIAN_POINT('Ctrl Pts',(-0.113872695264071,2.47652455025731,
10.1583132106226));
#26057=CARTESIAN_POINT('Ctrl Pts',(-0.106899571459506,2.47856307387668,
10.1579439517267));
#26058=CARTESIAN_POINT('Ctrl Pts',(-0.099882813207992,2.48040545951085,
10.1575746928309));
#26059=CARTESIAN_POINT('Ctrl Pts',(-0.080045150247591,2.48561422172605,
10.1565307301833));
#26060=CARTESIAN_POINT('Ctrl Pts',(-0.0597398372576802,2.48928256237326,
10.1554867675358));
#26061=CARTESIAN_POINT('Ctrl Pts',(-0.0392302215007405,2.49133857428192,
10.1544428048882));
#26062=CARTESIAN_POINT('Ctrl Pts',(-0.0187583353920246,2.49339080393512,
10.1534007627224));
#26063=CARTESIAN_POINT('Ctrl Pts',(0.00191638955361917,2.49383646061028,
10.1523587205567));
#26064=CARTESIAN_POINT('Ctrl Pts',(0.0225208468571737,2.49265468475091,
10.1513166783909));
#26065=CARTESIAN_POINT('Ctrl Pts',(0.0431031752972776,2.49147417810024,
10.150275755362));
#26066=CARTESIAN_POINT('Ctrl Pts',(0.0636146534114712,2.4886697218335,10.1492348323332));
#26067=CARTESIAN_POINT('Ctrl Pts',(0.0837827255047211,2.48427248783513,
10.1481939093043));
#26068=CARTESIAN_POINT('Ctrl Pts',(0.103961155394147,2.47987299553198,10.1471524516845));
#26069=CARTESIAN_POINT('Ctrl Pts',(0.123795104602177,2.47387923228649,10.1461109940647));
#26070=CARTESIAN_POINT('Ctrl Pts',(0.143022223006656,2.46637348938786,10.145069536445));
#26071=CARTESIAN_POINT('Ctrl Pts',(0.162255216134042,2.45886545315754,10.1440277606145));
#26072=CARTESIAN_POINT('Ctrl Pts',(0.180880337673762,2.4498448186313,10.142985984784));
#26073=CARTESIAN_POINT('Ctrl Pts',(0.198656107296091,2.43944166072238,10.1419442089535));
#26074=CARTESIAN_POINT('Ctrl Pts',(0.216470299647844,2.42901601615155,10.1409001813009));
#26075=CARTESIAN_POINT('Ctrl Pts',(0.233430870483884,2.41720230302976,10.1398561536483));
#26076=CARTESIAN_POINT('Ctrl Pts',(0.249325510108922,2.40417376614186,10.1388121259957));
#26077=CARTESIAN_POINT('Ctrl Pts',(0.254947235801275,2.39956574341947,10.1384428670998));
#26078=CARTESIAN_POINT('Ctrl Pts',(0.260435940870581,2.39480610574416,10.138073608204));
#26079=CARTESIAN_POINT('Ctrl Pts',(0.265783349724765,2.38990360640924,10.1377043493081));
#26080=CARTESIAN_POINT('Ctrl Pts',(0.280901455659281,2.37604334131444,10.1366603866605));
#26081=CARTESIAN_POINT('Ctrl Pts',(0.294977494970005,2.36095600967344,10.135616424013));
#26082=CARTESIAN_POINT('Ctrl Pts',(0.307808452188906,2.3448241139289,10.1345724613654));
#26083=CARTESIAN_POINT('Ctrl Pts',(0.320615805479391,2.32872189454488,10.1335304191997));
#26084=CARTESIAN_POINT('Ctrl Pts',(0.332182123772735,2.31157945765313,10.1324883770339));
#26085=CARTESIAN_POINT('Ctrl Pts',(0.342342030508542,2.29361514441615,10.1314463348681));
#26086=CARTESIAN_POINT('Ctrl Pts',(0.352491025664119,2.27567012456939,10.1304054118393));
#26087=CARTESIAN_POINT('Ctrl Pts',(0.361236222345084,2.2569056036751,10.1293644888104));
#26088=CARTESIAN_POINT('Ctrl Pts',(0.368456291107496,2.23756762534589,10.1283235657816));
#26089=CARTESIAN_POINT('Ctrl Pts',(0.375680067909047,2.21821971553502,10.1272821081618));
#26090=CARTESIAN_POINT('Ctrl Pts',(0.381376879540625,2.19829844358105,10.126240650542));
#26091=CARTESIAN_POINT('Ctrl Pts',(0.385473903130076,2.17806894392564,10.1251991929222));
#26092=CARTESIAN_POINT('Ctrl Pts',(0.389572178538849,2.15783326327616,10.1241574170917));
#26093=CARTESIAN_POINT('Ctrl Pts',(0.392069582344319,2.13728989515265,10.1231156412612));
#26094=CARTESIAN_POINT('Ctrl Pts',(0.392944766196695,2.11671229244075,10.1220738654308));
#26095=CARTESIAN_POINT('Ctrl Pts',(0.393821841778828,2.09609021077361,10.1210298377782));
#26096=CARTESIAN_POINT('Ctrl Pts',(0.393069723720385,2.07543448277302,10.1199858101256));
#26097=CARTESIAN_POINT('Ctrl Pts',(0.390719152264053,2.0550174027644,10.118941782473));
#26098=CARTESIAN_POINT('Ctrl Pts',(0.389887785950664,2.04779614918746,10.1185725235771));
#26099=CARTESIAN_POINT('Ctrl Pts',(0.388856932603512,2.0406046698185,10.1182032646812));
#26100=CARTESIAN_POINT('Ctrl Pts',(0.387629472420801,2.03345466123934,10.1178340057854));
#26101=CARTESIAN_POINT('Ctrl Pts',(0.384159217278783,2.01324027515433,10.1167900431378));
#26102=CARTESIAN_POINT('Ctrl Pts',(0.379093133122442,1.99323784405101,10.1157460804903));
#26103=CARTESIAN_POINT('Ctrl Pts',(0.372474775332054,1.97371685883961,10.1147021178427));
#26104=CARTESIAN_POINT('Ctrl Pts',(0.365868592723991,1.954231784584,10.113660075677));
#26105=CARTESIAN_POINT('Ctrl Pts',(0.35771598194294,1.93522710624149,10.1126180335112));
#26106=CARTESIAN_POINT('Ctrl Pts',(0.348111006827302,1.91696006740145,10.1115759913454));
#26107=CARTESIAN_POINT('Ctrl Pts',(0.338516347304046,1.89871264707415,10.1105350683166));
#26108=CARTESIAN_POINT('Ctrl Pts',(0.327472735148029,1.88120195491398,10.1094941452877));
#26109=CARTESIAN_POINT('Ctrl Pts',(0.315121370413706,1.86466319474297,10.1084532222588));
#26110=CARTESIAN_POINT('Ctrl Pts',(0.302763662340371,1.84811594069578,10.107411764639));
#26111=CARTESIAN_POINT('Ctrl Pts',(0.2890972872744,1.83254221501481,10.1063703070193));
#26112=CARTESIAN_POINT('Ctrl Pts',(0.274305754664904,1.81814677053878,10.1053288493995));
#26113=CARTESIAN_POINT('Ctrl Pts',(0.259509702597341,1.80374692762688,10.104287073569));
#26114=CARTESIAN_POINT('Ctrl Pts',(0.243588360667883,1.7905265694324,10.1032452977385));
#26115=CARTESIAN_POINT('Ctrl Pts',(0.226760096711288,1.77865167101806,10.102203521908));
#26116=CARTESIAN_POINT('Ctrl Pts',(0.209895458080266,1.76675110474131,10.1011594942554));
#26117=CARTESIAN_POINT('Ctrl Pts',(0.19212061705435,1.75620218027901,10.1001154666028));
#26118=CARTESIAN_POINT('Ctrl Pts',(0.173681163826441,1.74712644852314,10.0990714389502));
#26119=CARTESIAN_POINT('Ctrl Pts',(0.167159370919507,1.74391648116353,10.0987021800543));
#26120=CARTESIAN_POINT('Ctrl Pts',(0.16055462676386,1.74089036339037,10.0983329211584));
#26121=CARTESIAN_POINT('Ctrl Pts',(0.153878325158237,1.73805200505253,10.0979636622626));
#26122=CARTESIAN_POINT('Ctrl Pts',(0.135003195599921,1.73002744527012,10.096919699615));
#26123=CARTESIAN_POINT('Ctrl Pts',(0.115442430504887,1.72345942215667,10.0958757369675));
#26124=CARTESIAN_POINT('Ctrl Pts',(0.0954461999698468,1.71845719386769,
10.0948317743199));
#26125=CARTESIAN_POINT('Ctrl Pts',(0.0754867546555941,1.71346416771667,
10.0937897321541));
#26126=CARTESIAN_POINT('Ctrl Pts',(0.0550941253140348,1.7100314530493,10.0927476899884));
#26127=CARTESIAN_POINT('Ctrl Pts',(0.03453552541627,1.70821920990914,10.0917056478226));
#26128=CARTESIAN_POINT('Ctrl Pts',(0.0139990051318226,1.70640891308963,
10.0906647247937));
#26129=CARTESIAN_POINT('Ctrl Pts',(-0.00670240516006667,1.70621572585505,
10.0896238017649));
#26130=CARTESIAN_POINT('Ctrl Pts',(-0.0272945077338579,1.70764824475024,
10.088582878736));
#26131=CARTESIAN_POINT('Ctrl Pts',(-0.0478971858748285,1.7090814993498,
10.0875414211162));
#26132=CARTESIAN_POINT('Ctrl Pts',(-0.0683897090242782,1.71214209308282,
10.0864999634964));
#26133=CARTESIAN_POINT('Ctrl Pts',(-0.0885005803488368,1.71678656433011,
10.0854585058767));
#26134=CARTESIAN_POINT('Ctrl Pts',(-0.108617596421348,1.72143245466585,
10.0844167300462));
#26135=CARTESIAN_POINT('Ctrl Pts',(-0.128352020360443,1.72766298525457,
10.0833749542157));
#26136=CARTESIAN_POINT('Ctrl Pts',(-0.147446090907105,1.73538439381149,
10.0823331783852));
#26137=CARTESIAN_POINT('Ctrl Pts',(-0.166581433720556,1.74312249236823,
10.0812891507326));
#26138=CARTESIAN_POINT('Ctrl Pts',(-0.185073000898774,1.75235757353198,
10.08024512308));
#26139=CARTESIAN_POINT('Ctrl Pts',(-0.202685647866543,1.76294893836554,
10.0792010954274));
#26140=CARTESIAN_POINT('Ctrl Pts',(-0.208915010236842,1.76669496527818,
10.0788318365315));
#26141=CARTESIAN_POINT('Ctrl Pts',(-0.215034691592898,1.77061026018904,
10.0784625776356));
#26142=CARTESIAN_POINT('Ctrl Pts',(-0.221035236794658,1.77468735945997,
10.0780933187398));
#26143=CARTESIAN_POINT('Ctrl Pts',(-0.237929542875462,1.78616627690643,
10.0770536844065));
#26144=CARTESIAN_POINT('Ctrl Pts',(-0.253979647592879,1.79900042839638,
10.0760140500733));
#26145=CARTESIAN_POINT('Ctrl Pts',(-0.268959324569773,1.81304047022799,
10.0749744157401));
#26146=CARTESIAN_POINT('Ctrl Pts',(-0.283911446583697,1.8270546855459,10.0739366938036));
#26147=CARTESIAN_POINT('Ctrl Pts',(-0.297796471253918,1.84226993153282,
10.0728989718671));
#26148=CARTESIAN_POINT('Ctrl Pts',(-0.310420097793868,1.85849585327443,
10.0718612499306));
#26149=CARTESIAN_POINT('Ctrl Pts',(-0.323030379202652,1.87470462170014,
10.0708246250272));
#26150=CARTESIAN_POINT('Ctrl Pts',(-0.334381432834109,1.89192137966887,
10.0697880001237));
#26151=CARTESIAN_POINT('Ctrl Pts',(-0.34431848351851,1.90992193207128,10.0687513752203));
#26152=CARTESIAN_POINT('Ctrl Pts',(-0.354260684373736,1.9279318137931,10.0677142130553));
#26153=CARTESIAN_POINT('Ctrl Pts',(-0.362787047567585,1.94672565788657,
10.0666770508903));
#26154=CARTESIAN_POINT('Ctrl Pts',(-0.369788047242238,1.9660534057291,10.0656398887253));
#26155=CARTESIAN_POINT('Ctrl Pts',(-0.376791509495614,1.98538795204368,
10.0646023617419));
#26156=CARTESIAN_POINT('Ctrl Pts',(-0.382268325512055,2.00525606498279,
10.0635648347585));
#26157=CARTESIAN_POINT('Ctrl Pts',(-0.386158716662584,2.02539212142471,
10.0625273077751));
#26158=CARTESIAN_POINT('Ctrl Pts',(-0.390057259454706,2.04557036948923,
10.0614876068334));
#26159=CARTESIAN_POINT('Ctrl Pts',(-0.392362666939148,2.06601694301546,
10.0604479058917));
#26160=CARTESIAN_POINT('Ctrl Pts',(-0.393066867638244,2.08646014900158,
10.05940820495));
#26161=CARTESIAN_POINT('Ctrl Pts',(-0.393223067421461,2.09099468631091,
10.0591775873691));
#26162=CARTESIAN_POINT('Ctrl Pts',(-0.393300690674402,2.09552906580875,
10.0589469697881));
#26163=CARTESIAN_POINT('Ctrl Pts',(-0.393299995369781,2.10006035006604,
10.0587163522072));
#26164=CARTESIAN_POINT('',(-0.393299837194678,2.09964214159272,9.93371635220721));
#26165=CARTESIAN_POINT('Ctrl Pts',(-0.393299995369769,2.10006035013941,
10.0587163522035));
#26166=CARTESIAN_POINT('Ctrl Pts',(-0.393299499530562,2.10329171894644,
10.058551893208));
#26167=CARTESIAN_POINT('Ctrl Pts',(-0.393259180895846,2.10652274228517,
10.0583874342125));
#26168=CARTESIAN_POINT('Ctrl Pts',(-0.39317906021876,2.10975277424596,10.058222975217));
#26169=CARTESIAN_POINT('Ctrl Pts',(-0.392670465392941,2.13025656430656,
10.0571790125694));
#26170=CARTESIAN_POINT('Ctrl Pts',(-0.390552166972687,2.15078155567138,
10.0561350499219));
#26171=CARTESIAN_POINT('Ctrl Pts',(-0.386828265061194,2.17105479118079,
10.0550910872743));
#26172=CARTESIAN_POINT('Ctrl Pts',(-0.383111213668542,2.19129073188892,
10.0540490451085));
#26173=CARTESIAN_POINT('Ctrl Pts',(-0.377794494658613,2.21127510979819,
10.0530070029428));
#26174=CARTESIAN_POINT('Ctrl Pts',(-0.370933957234741,2.23073977730658,
10.051964960777));
#26175=CARTESIAN_POINT('Ctrl Pts',(-0.364080787920287,2.25018354006785,
10.0509240377481));
#26176=CARTESIAN_POINT('Ctrl Pts',(-0.355687307860049,2.26910800047918,
10.0498831147193));
#26177=CARTESIAN_POINT('Ctrl Pts',(-0.345859195631034,2.28725999785713,
10.0488421916904));
#26178=CARTESIAN_POINT('Ctrl Pts',(-0.33602603593973,2.30542131762784,10.0478007340706));
#26179=CARTESIAN_POINT('Ctrl Pts',(-0.324757108285042,2.32280872711126,
10.0467592764508));
#26180=CARTESIAN_POINT('Ctrl Pts',(-0.312204361749858,2.33919307369647,
10.045717818831));
#26181=CARTESIAN_POINT('Ctrl Pts',(-0.299647779803347,2.35558242641387,
10.0446760430005));
#26182=CARTESIAN_POINT('Ctrl Pts',(-0.285807073895645,2.37096754453505,
10.04363426717));
#26183=CARTESIAN_POINT('Ctrl Pts',(-0.270874295963819,2.38515260087558,
10.0425924913395));
#26184=CARTESIAN_POINT('Ctrl Pts',(-0.255909240493629,2.39936831853728,
10.041548463687));
#26185=CARTESIAN_POINT('Ctrl Pts',(-0.239847972583205,2.41237833213905,
10.0405044360344));
#26186=CARTESIAN_POINT('Ctrl Pts',(-0.222915908432341,2.42402683186394,
10.0394604083818));
#26187=CARTESIAN_POINT('Ctrl Pts',(-0.216927259283587,2.42814675353092,
10.0390911494859));
#26188=CARTESIAN_POINT('Ctrl Pts',(-0.210829927902349,2.43209676418458,
10.03872189059));
#26189=CARTESIAN_POINT('Ctrl Pts',(-0.204634622387762,2.43587134638164,
10.0383526316942));
#26190=CARTESIAN_POINT('Ctrl Pts',(-0.187119357028162,2.44654278278578,
10.0373086690466));
#26191=CARTESIAN_POINT('Ctrl Pts',(-0.168714903591213,2.45587222823603,
10.0362647063991));
#26192=CARTESIAN_POINT('Ctrl Pts',(-0.149652988803798,2.46371537353003,
10.0352207437515));
#26193=CARTESIAN_POINT('Ctrl Pts',(-0.130626140462668,2.47154409051312,
10.0341787015857));
#26194=CARTESIAN_POINT('Ctrl Pts',(-0.110944881641507,2.47789160283408,
10.03313665942));
#26195=CARTESIAN_POINT('Ctrl Pts',(-0.0908649078280011,2.48265971636091,
10.0320946172542));
#26196=CARTESIAN_POINT('Ctrl Pts',(-0.070806499590917,2.48742270900871,
10.0310536942253));
#26197=CARTESIAN_POINT('Ctrl Pts',(-0.0503509320291084,2.49060947305793,
10.0300127711965));
#26198=CARTESIAN_POINT('Ctrl Pts',(-0.0297682729011165,2.49217182449595,
10.0289718481676));
#26199=CARTESIAN_POINT('Ctrl Pts',(-0.00917504305586029,2.49373497831695,
10.0279303905478));
#26200=CARTESIAN_POINT('Ctrl Pts',(0.0115446763047099,2.49367198110561,
10.0268889329281));
#26201=CARTESIAN_POINT('Ctrl Pts',(0.0321159567783998,2.49198654992258,
10.0258474753083));
#26202=CARTESIAN_POINT('Ctrl Pts',(0.0526935226751098,2.49030060376684,
10.0248056994778));
#26203=CARTESIAN_POINT('Ctrl Pts',(0.0731218296459621,2.48699133286079,
10.0237639236473));
#26204=CARTESIAN_POINT('Ctrl Pts',(0.0931322615044203,2.48211421311837,
10.0227221478168));
#26205=CARTESIAN_POINT('Ctrl Pts',(0.113185946365438,2.47722655137095,10.0216781201642));
#26206=CARTESIAN_POINT('Ctrl Pts',(0.132819253266682,2.47076450518345,10.0206340925116));
#26207=CARTESIAN_POINT('Ctrl Pts',(0.151779152662418,2.46283326586337,10.019590064859));
#26208=CARTESIAN_POINT('Ctrl Pts',(0.158485020557026,2.46002809047658,10.0192208059631));
#26209=CARTESIAN_POINT('Ctrl Pts',(0.165106855885699,2.45703955722122,10.0188515470672));
#26210=CARTESIAN_POINT('Ctrl Pts',(0.171634222995775,2.45387368296701,10.0184822881714));
#26211=CARTESIAN_POINT('Ctrl Pts',(0.190088287409788,2.4449231755988,10.0174383255238));
#26212=CARTESIAN_POINT('Ctrl Pts',(0.207895315375127,2.4344985790232,10.0163943628763));
#26213=CARTESIAN_POINT('Ctrl Pts',(0.22480853126639,2.42271661604239,10.0153504002287));
#26214=CARTESIAN_POINT('Ctrl Pts',(0.241690633474522,2.41095632725205,10.0143083580629));
#26215=CARTESIAN_POINT('Ctrl Pts',(0.257681556499956,2.39784399556599,10.0132663158972));
#26216=CARTESIAN_POINT('Ctrl Pts',(0.272560324370808,2.38354146007045,10.0122242737314));
#26217=CARTESIAN_POINT('Ctrl Pts',(0.287423112678699,2.36925428527334,10.0111833507025));
#26218=CARTESIAN_POINT('Ctrl Pts',(0.301175569278181,2.35377993078405,10.0101424276737));
#26219=CARTESIAN_POINT('Ctrl Pts',(0.313630987631237,2.33731939153271,10.0091015046448));
#26220=CARTESIAN_POINT('Ctrl Pts',(0.326092802762532,2.32085039857742,10.008060047025));
#26221=CARTESIAN_POINT('Ctrl Pts',(0.337255792050764,2.30339478603645,10.0070185894052));
#26222=CARTESIAN_POINT('Ctrl Pts',(0.346974257155323,2.28518573074487,10.0059771317855));
#26223=CARTESIAN_POINT('Ctrl Pts',(0.356695691674663,2.26697111179305,10.004935355955));
#26224=CARTESIAN_POINT('Ctrl Pts',(0.364971409125805,2.24800325739952,10.0038935801245));
#26225=CARTESIAN_POINT('Ctrl Pts',(0.371702647855097,2.22853805497793,10.002851804294));
#26226=CARTESIAN_POINT('Ctrl Pts',(0.378448436309655,2.20903077807958,10.0018077766414));
#26227=CARTESIAN_POINT('Ctrl Pts',(0.383642895953234,2.18902471975168,10.0007637489888));
#26228=CARTESIAN_POINT('Ctrl Pts',(0.387237504055506,2.16878957372206,9.99971972133617));
#26229=CARTESIAN_POINT('Ctrl Pts',(0.388508869824041,2.16163266780869,9.99935046244031));
#26230=CARTESIAN_POINT('Ctrl Pts',(0.389580576667465,2.15444716305399,9.99898120354444));
#26231=CARTESIAN_POINT('Ctrl Pts',(0.390452034670221,2.14724509098186,9.99861194464858));
#26232=CARTESIAN_POINT('Ctrl Pts',(0.392915806332796,2.12688351185009,9.99756798200102));
#26233=CARTESIAN_POINT('Ctrl Pts',(0.393789884876273,2.10626802142608,9.99652401935347));
#26234=CARTESIAN_POINT('Ctrl Pts',(0.393038828817571,2.08566929723592,9.99548005670592));
#26235=CARTESIAN_POINT('Ctrl Pts',(0.392289154407419,2.06510846661853,9.99443801454015));
#26236=CARTESIAN_POINT('Ctrl Pts',(0.389920246728875,2.04456507016466,9.99339597237438));
#26237=CARTESIAN_POINT('Ctrl Pts',(0.385948564696898,2.02431251484952,9.99235393020861));
#26238=CARTESIAN_POINT('Ctrl Pts',(0.38198114818903,2.00408171046063,9.99131300717976));
#26239=CARTESIAN_POINT('Ctrl Pts',(0.376414487124075,1.98414185103363,9.99027208415091));
#26240=CARTESIAN_POINT('Ctrl Pts',(0.369316514015366,1.96475872495596,9.98923116112205));
#26241=CARTESIAN_POINT('Ctrl Pts',(0.362214895572662,1.94536564420992,9.98818970350226));
#26242=CARTESIAN_POINT('Ctrl Pts',(0.353580631820356,1.92653056447859,9.98714824588247));
#26243=CARTESIAN_POINT('Ctrl Pts',(0.343530912871894,1.90850221436945,9.98610678826268));
#26244=CARTESIAN_POINT('Ctrl Pts',(0.333478123296164,1.8904683558134,9.98506501243218));
#26245=CARTESIAN_POINT('Ctrl Pts',(0.322009407103362,1.87324234209825,9.98402323660169));
#26246=CARTESIAN_POINT('Ctrl Pts',(0.309286457544761,1.85704573027129,9.98298146077119));
#26247=CARTESIAN_POINT('Ctrl Pts',(0.296536007041966,1.8408141091003,9.98193743311859));
#26248=CARTESIAN_POINT('Ctrl Pts',(0.282526409866713,1.82561687356895,9.980893405466));
#26249=CARTESIAN_POINT('Ctrl Pts',(0.267458163103384,1.8116408125456,9.9798493778134));
#26250=CARTESIAN_POINT('Ctrl Pts',(0.26212872173407,1.80669766295641,9.97948011891753));
#26251=CARTESIAN_POINT('Ctrl Pts',(0.256667154963148,1.80190690909666,9.97911086002167));
#26252=CARTESIAN_POINT('Ctrl Pts',(0.251083259779382,1.7972755598592,9.9787416011258));
#26253=CARTESIAN_POINT('Ctrl Pts',(0.23529656360233,1.78418188583857,9.97769763847825));
#26254=CARTESIAN_POINT('Ctrl Pts',(0.218435844655353,1.77228740748459,9.9766536758307));
#26255=CARTESIAN_POINT('Ctrl Pts',(0.200709508333495,1.76176844726648,9.97560971318314));
#26256=CARTESIAN_POINT('Ctrl Pts',(0.183015781517424,1.75126883780917,9.97456767101737));
#26257=CARTESIAN_POINT('Ctrl Pts',(0.164460193432313,1.74214014610303,9.9735256288516));
#26258=CARTESIAN_POINT('Ctrl Pts',(0.145281539066169,1.7345165333335,9.97248358668583));
#26259=CARTESIAN_POINT('Ctrl Pts',(0.126123482273526,1.72690110820432,9.97144266365698));
#26260=CARTESIAN_POINT('Ctrl Pts',(0.106344357238756,1.72078785029713,9.97040174062812));
#26261=CARTESIAN_POINT('Ctrl Pts',(0.0862044166937409,1.71626351679506,
9.96936081759927));
#26262=CARTESIAN_POINT('Ctrl Pts',(0.0660541328001721,1.71173685971323,
9.96831935997948));
#26263=CARTESIAN_POINT('Ctrl Pts',(0.0455433775512048,1.70880093428048,
9.96727790235969));
#26264=CARTESIAN_POINT('Ctrl Pts',(0.0249447235392476,1.70749184624068,
9.9662364447399));
#26265=CARTESIAN_POINT('Ctrl Pts',(0.00433977574046094,1.70618235821742,
9.9651946689094));
#26266=CARTESIAN_POINT('Ctrl Pts',(-0.0163523883141121,1.7065007076543,
9.9641528930789));
#26267=CARTESIAN_POINT('Ctrl Pts',(-0.036857952013767,1.7084308728036,9.9631111172484));
#26268=CARTESIAN_POINT('Ctrl Pts',(-0.0574078389546922,1.71036521004867,
9.9620670895958));
#26269=CARTESIAN_POINT('Ctrl Pts',(-0.0777695947749148,1.71391819199709,
9.96102306194321));
#26270=CARTESIAN_POINT('Ctrl Pts',(-0.0976776313550497,1.71902234930003,
9.95997903429061));
#26271=CARTESIAN_POINT('Ctrl Pts',(-0.104718842943808,1.72082762283405,
9.95960977539474));
#26272=CARTESIAN_POINT('Ctrl Pts',(-0.111703439341944,1.72282648433332,
9.95924051649888));
#26273=CARTESIAN_POINT('Ctrl Pts',(-0.118620224059825,1.72501449035463,
9.95887125760301));
#26274=CARTESIAN_POINT('Ctrl Pts',(-0.138175243498682,1.73120038481633,
9.95782729495546));
#26275=CARTESIAN_POINT('Ctrl Pts',(-0.157303345681881,1.73893848313514,
9.9567833323079));
#26276=CARTESIAN_POINT('Ctrl Pts',(-0.175743461914374,1.74814900086208,
9.95573936966035));
#26277=CARTESIAN_POINT('Ctrl Pts',(-0.194149655566013,1.75734257484917,
9.95469732749458));
#26278=CARTESIAN_POINT('Ctrl Pts',(-0.211869698104813,1.76800291977198,
9.95365528532881));
#26279=CARTESIAN_POINT('Ctrl Pts',(-0.228661520362214,1.78000187640294,
9.95261324316304));
#26280=CARTESIAN_POINT('Ctrl Pts',(-0.245435308466308,1.79198794634298,
9.95157232013418));
#26281=CARTESIAN_POINT('Ctrl Pts',(-0.261282242936222,1.80530937184055,
9.95053139710533));
#26282=CARTESIAN_POINT('Ctrl Pts',(-0.275988497272819,1.81979429096985,
9.94949047407648));
#26283=CARTESIAN_POINT('Ctrl Pts',(-0.290702304358352,1.83428664917609,
9.94844901645669));
#26284=CARTESIAN_POINT('Ctrl Pts',(-0.304273725450247,1.84994318993631,
9.94740755883689));
#26285=CARTESIAN_POINT('Ctrl Pts',(-0.316524853723257,1.86655427402612,
9.9463661012171));
#26286=CARTESIAN_POINT('Ctrl Pts',(-0.328779725250061,1.88317043352631,
9.9453243253866));
#26287=CARTESIAN_POINT('Ctrl Pts',(-0.3397130936301,1.90074110384625,9.9442825495561));
#26288=CARTESIAN_POINT('Ctrl Pts',(-0.349190208356797,1.9190273822156,9.9432407737256));
#26289=CARTESIAN_POINT('Ctrl Pts',(-0.358687808082036,1.93735318679062,
9.94219674607301));
#26290=CARTESIAN_POINT('Ctrl Pts',(-0.366722583584917,1.95639700897595,
9.94115271842041));
#26291=CARTESIAN_POINT('Ctrl Pts',(-0.37320749665403,1.97589901514802,9.94010869076781));
#26292=CARTESIAN_POINT('Ctrl Pts',(-0.375501125403926,1.98279661910357,
9.93973943187195));
#26293=CARTESIAN_POINT('Ctrl Pts',(-0.377601335100905,1.98975141265669,
9.93937017297608));
#26294=CARTESIAN_POINT('Ctrl Pts',(-0.379505801009439,1.99675157628233,
9.93900091408021));
#26295=CARTESIAN_POINT('Ctrl Pts',(-0.386317014682717,2.02178726213446,
9.93768028070514));
#26296=CARTESIAN_POINT('Ctrl Pts',(-0.390653742797625,2.0475233829174,9.93635964733007));
#26297=CARTESIAN_POINT('Ctrl Pts',(-0.392408023018093,2.07352674045321,
9.935039013955));
#26298=CARTESIAN_POINT('Ctrl Pts',(-0.392993681229854,2.08220783922894,
9.93459812670574));
#26299=CARTESIAN_POINT('Ctrl Pts',(-0.393291899704221,2.09091854130528,
9.93415723945647));
#26300=CARTESIAN_POINT('Ctrl Pts',(-0.393299837194678,2.09964214159272,
9.93371635220721));
#26301=CARTESIAN_POINT('',(-0.393067570229214,2.10012154744265,9.80871631880887));
#26302=CARTESIAN_POINT('Ctrl Pts',(-0.393299837194745,2.09964214166643,
9.93371635220349));
#26303=CARTESIAN_POINT('Ctrl Pts',(-0.39331839913374,2.12004241434374,9.93268533062886));
#26304=CARTESIAN_POINT('Ctrl Pts',(-0.391745421875908,2.14047972199369,
9.93165430905423));
#26305=CARTESIAN_POINT('Ctrl Pts',(-0.388590103262886,2.16068460798373,
9.93062328747959));
#26306=CARTESIAN_POINT('Ctrl Pts',(-0.385434358167012,2.18089222493012,
9.92959212654882));
#26307=CARTESIAN_POINT('Ctrl Pts',(-0.380695920873502,2.20086660921189,
9.92856096561805));
#26308=CARTESIAN_POINT('Ctrl Pts',(-0.37443578397093,2.22034422994924,9.92752980468727));
#26309=CARTESIAN_POINT('Ctrl Pts',(-0.368175768378373,2.23982147324589,
9.92649866373852));
#26310=CARTESIAN_POINT('Ctrl Pts',(-0.360394362374816,2.25880126237412,
9.92546752278976));
#26311=CARTESIAN_POINT('Ctrl Pts',(-0.351201875568091,2.27703709384605,
9.924436381841));
#26312=CARTESIAN_POINT('Ctrl Pts',(-0.341988688502122,2.29531398998818,
9.92340291889979));
#26313=CARTESIAN_POINT('Ctrl Pts',(-0.331358451623212,2.31284292897447,
9.92236945595858));
#26314=CARTESIAN_POINT('Ctrl Pts',(-0.31946694191771,2.32940305800435,9.92133599301738));
#26315=CARTESIAN_POINT('Ctrl Pts',(-0.311008066570381,2.34118289678585,
9.92060085219739));
#26316=CARTESIAN_POINT('Ctrl Pts',(-0.30191195304697,2.35247308549262,9.91986571137741));
#26317=CARTESIAN_POINT('Ctrl Pts',(-0.29224647058237,2.36320503496732,9.91913057055742));
#26318=CARTESIAN_POINT('Ctrl Pts',(-0.278520661336955,2.3784453183014,9.91808660790987));
#26319=CARTESIAN_POINT('Ctrl Pts',(-0.263558603338637,2.39265444491696,
9.91704264526232));
#26320=CARTESIAN_POINT('Ctrl Pts',(-0.247540993614156,2.40562779075293,
9.91599868261476));
#26321=CARTESIAN_POINT('Ctrl Pts',(-0.231552850008755,2.41857727072128,
9.914956640449));
#26322=CARTESIAN_POINT('Ctrl Pts',(-0.214513536950555,2.43029497834499,
9.91391459828323));
#26323=CARTESIAN_POINT('Ctrl Pts',(-0.196639922175481,2.44061360954434,
9.91287255611746));
#26324=CARTESIAN_POINT('Ctrl Pts',(-0.17878550338189,2.45092115869587,9.9118316330886));
#26325=CARTESIAN_POINT('Ctrl Pts',(-0.160099181221913,2.45983222336371,
9.91079071005975));
#26326=CARTESIAN_POINT('Ctrl Pts',(-0.140825914952268,2.46722329947575,
9.9097497870309));
#26327=CARTESIAN_POINT('Ctrl Pts',(-0.121542750435389,2.47461817145185,
9.90870832941111));
#26328=CARTESIAN_POINT('Ctrl Pts',(-0.101672720823039,2.48049121684875,
9.90766687179132));
#26329=CARTESIAN_POINT('Ctrl Pts',(-0.0814803051101876,2.48476726716179,
9.90662541417152));
#26330=CARTESIAN_POINT('Ctrl Pts',(-0.0612817197340254,2.48904462399462,
9.90558363834103));
#26331=CARTESIAN_POINT('Ctrl Pts',(-0.0407612788656792,2.49172389743974,
9.90454186251053));
#26332=CARTESIAN_POINT('Ctrl Pts',(-0.0201922355651711,2.49278131781295,
9.90350008668003));
#26333=CARTESIAN_POINT('Ctrl Pts',(0.000421268189205144,2.4938410238243,
9.90245605902744));
#26334=CARTESIAN_POINT('Ctrl Pts',(0.0210828479149291,2.49327189813925,
9.90141203137484));
#26335=CARTESIAN_POINT('Ctrl Pts',(0.041519947680011,2.49110226788482,9.90036800372224));
#26336=CARTESIAN_POINT('Ctrl Pts',(0.0487482819824797,2.49033489810281,
9.89999874482638));
#26337=CARTESIAN_POINT('Ctrl Pts',(0.0559486102473542,2.48936778538109,
9.89962948593051));
#26338=CARTESIAN_POINT('Ctrl Pts',(0.0631092108396671,2.48820370619971,
9.89926022703464));
#26339=CARTESIAN_POINT('Ctrl Pts',(0.0833535424890364,2.48491264077719,
9.89821626438709));
#26340=CARTESIAN_POINT('Ctrl Pts',(0.103400062894784,2.4800239315054,9.89717230173954));
#26341=CARTESIAN_POINT('Ctrl Pts',(0.122978905917147,2.47357874497811,9.89612833909198));
#26342=CARTESIAN_POINT('Ctrl Pts',(0.14252173154802,2.46714541506595,9.89508629692621));
#26343=CARTESIAN_POINT('Ctrl Pts',(0.161597877955621,2.45916146243047,9.89404425476044));
#26344=CARTESIAN_POINT('Ctrl Pts',(0.179949278450231,2.44971866862557,9.89300221259468));
#26345=CARTESIAN_POINT('Ctrl Pts',(0.198280969829021,2.44028601623286,9.89196128956582));
#26346=CARTESIAN_POINT('Ctrl Pts',(0.215888796374484,2.42939794231108,9.89092036653697));
#26347=CARTESIAN_POINT('Ctrl Pts',(0.23253631277975,2.41719355800331,9.88987944350811));
#26348=CARTESIAN_POINT('Ctrl Pts',(0.249192378915542,2.40498290584185,9.88883798588832));
#26349=CARTESIAN_POINT('Ctrl Pts',(0.26488654669633,2.39145501477568,9.88779652826853));
#26350=CARTESIAN_POINT('Ctrl Pts',(0.279412445838746,2.37679157340933,9.88675507064874));
#26351=CARTESIAN_POINT('Ctrl Pts',(0.293942783276634,2.36212365172235,9.88571329481824));
#26352=CARTESIAN_POINT('Ctrl Pts',(0.307303649782911,2.34632003676162,9.88467151898774));
#26353=CARTESIAN_POINT('Ctrl Pts',(0.319327142562771,2.32959761763288,9.88362974315724));
#26354=CARTESIAN_POINT('Ctrl Pts',(0.33137662439511,2.31283905261574,9.88258571550464));
#26355=CARTESIAN_POINT('Ctrl Pts',(0.342082579765853,2.29515834843272,9.88154168785205));
#26356=CARTESIAN_POINT('Ctrl Pts',(0.351321287179832,2.27680000897711,9.88049766019945));
#26357=CARTESIAN_POINT('Ctrl Pts',(0.354588896893459,2.27030690494824,9.88012840130359));
#26358=CARTESIAN_POINT('Ctrl Pts',(0.357673398992924,2.26372922443483,9.87975914240772));
#26359=CARTESIAN_POINT('Ctrl Pts',(0.360570782859558,2.25707832615624,9.87938988351185));
#26360=CARTESIAN_POINT('Ctrl Pts',(0.368762218641469,2.23827501646417,9.8783459208643));
#26361=CARTESIAN_POINT('Ctrl Pts',(0.375503248069686,2.21877319652422,9.87730195821674));
#26362=CARTESIAN_POINT('Ctrl Pts',(0.380682401335698,2.19882205883954,9.87625799556919));
#26363=CARTESIAN_POINT('Ctrl Pts',(0.385852026991192,2.1789076234225,9.87521595340342));
#26364=CARTESIAN_POINT('Ctrl Pts',(0.389465239402053,2.15854620015387,9.87417391123765));
#26365=CARTESIAN_POINT('Ctrl Pts',(0.391459513979982,2.13800445914042,9.87313186907188));
#26366=CARTESIAN_POINT('Ctrl Pts',(0.393451646738343,2.11748477963413,9.87209094604303));
#26367=CARTESIAN_POINT('Ctrl Pts',(0.393828193902946,2.09678589266856,9.87105002301418));
#26368=CARTESIAN_POINT('Ctrl Pts',(0.392578130496698,2.07618190906648,9.87000909998532));
#26369=CARTESIAN_POINT('Ctrl Pts',(0.391327425090465,2.05556734379542,9.86896764236553));
#26370=CARTESIAN_POINT('Ctrl Pts',(0.38844846866883,2.03504851466331,9.86792618474574));
#26371=CARTESIAN_POINT('Ctrl Pts',(0.383982316300243,2.0148972928239,9.86688472712595));
#26372=CARTESIAN_POINT('Ctrl Pts',(0.379514799327402,1.99473991390771,9.86584295129545));
#26373=CARTESIAN_POINT('Ctrl Pts',(0.373459315369822,1.97495107579972,9.86480117546495));
#26374=CARTESIAN_POINT('Ctrl Pts',(0.365907339854241,1.95578936016787,9.86375939963446));
#26375=CARTESIAN_POINT('Ctrl Pts',(0.358339040572202,1.93658622605283,9.86271537198186));
#26376=CARTESIAN_POINT('Ctrl Pts',(0.349268115019523,1.91801358244924,9.86167134432926));
#26377=CARTESIAN_POINT('Ctrl Pts',(0.338833173766516,1.90030781098072,9.86062731667666));
#26378=CARTESIAN_POINT('Ctrl Pts',(0.335142471823961,1.89404551169519,9.8602580577808));
#26379=CARTESIAN_POINT('Ctrl Pts',(0.331281536998818,1.88789138979079,9.85988879888493));
#26380=CARTESIAN_POINT('Ctrl Pts',(0.327257748885349,1.88185496614753,9.85951953998906));
#26381=CARTESIAN_POINT('Ctrl Pts',(0.315881761633185,1.86478888898893,9.85847557734151));
#26382=CARTESIAN_POINT('Ctrl Pts',(0.303133323291774,1.84856422324269,9.85743161469396));
#26383=CARTESIAN_POINT('Ctrl Pts',(0.289161618757924,1.83340958712419,9.85638765204641));
#26384=CARTESIAN_POINT('Ctrl Pts',(0.275215616680097,1.81828282959182,9.85534560988064));
#26385=CARTESIAN_POINT('Ctrl Pts',(0.2600512646017,1.80422276958154,9.85430356771487));
#26386=CARTESIAN_POINT('Ctrl Pts',(0.24385893783366,1.79142633223387,9.8532615255491));
#26387=CARTESIAN_POINT('Ctrl Pts',(0.227684001370201,1.7786436380589,9.85222060252025));
#26388=CARTESIAN_POINT('Ctrl Pts',(0.210483838392706,1.76712234894144,9.85117967949139));
#26389=CARTESIAN_POINT('Ctrl Pts',(0.192482958169429,1.75702011602086,9.85013875646254));
#26390=CARTESIAN_POINT('Ctrl Pts',(0.174472833163229,1.74691269485675,9.84909729884275));
#26391=CARTESIAN_POINT('Ctrl Pts',(0.155661803121502,1.73822616000108,9.84805584122296));
#26392=CARTESIAN_POINT('Ctrl Pts',(0.136300686028357,1.73107316038515,9.84701438360317));
#26393=CARTESIAN_POINT('Ctrl Pts',(0.116933653269857,1.72391797521599,9.84597260777267));
#26394=CARTESIAN_POINT('Ctrl Pts',(0.0970169009997988,1.71829747891776,
9.84493083194217));
#26395=CARTESIAN_POINT('Ctrl Pts',(0.0768173666156927,1.71427473224297,
9.84388905611167));
#26396=CARTESIAN_POINT('Ctrl Pts',(0.0565741704796338,1.71024329030996,
9.84284502845908));
#26397=CARTESIAN_POINT('Ctrl Pts',(0.0360477033031119,1.70781657935499,
9.84180100080648));
#26398=CARTESIAN_POINT('Ctrl Pts',(0.0155117513937795,1.70700601077281,
9.84075697315388));
#26399=CARTESIAN_POINT('Ctrl Pts',(0.00824845438361141,1.70671932329003,
9.84038771425801));
#26400=CARTESIAN_POINT('Ctrl Pts',(0.000983964717090274,1.70663432903389,
9.84001845536215));
#26401=CARTESIAN_POINT('Ctrl Pts',(-0.00626971757168497,1.70674997693379,
9.83964919646628));
#26402=CARTESIAN_POINT('Ctrl Pts',(-0.0267772082548701,1.70707693476506,
9.83860523381873));
#26403=CARTESIAN_POINT('Ctrl Pts',(-0.0473201577308162,1.70901334524591,
9.83756127117117));
#26404=CARTESIAN_POINT('Ctrl Pts',(-0.0676255832305279,1.71255752621488,
9.83651730852362));
#26405=CARTESIAN_POINT('Ctrl Pts',(-0.0878936547119969,1.71609518728106,
9.83547526635785));
#26406=CARTESIAN_POINT('Ctrl Pts',(-0.107924342687827,1.72123468148423,
9.83443322419208));
#26407=CARTESIAN_POINT('Ctrl Pts',(-0.127449015378381,1.72792253699118,
9.83339118202631));
#26408=CARTESIAN_POINT('Ctrl Pts',(-0.146952718877181,1.73460320984638,
9.83235025899746));
#26409=CARTESIAN_POINT('Ctrl Pts',(-0.165950784055656,1.7428287328604,9.83130933596861));
#26410=CARTESIAN_POINT('Ctrl Pts',(-0.184189124089649,1.75249567403112,
9.83026841293975));
#26411=CARTESIAN_POINT('Ctrl Pts',(-0.202436830859749,1.76216757989087,
9.82922695531996));
#26412=CARTESIAN_POINT('Ctrl Pts',(-0.21992337534878,1.77328205247676,9.82818549770017));
#26413=CARTESIAN_POINT('Ctrl Pts',(-0.236418268011613,1.78568917843894,
9.82714404008038));
#26414=CARTESIAN_POINT('Ctrl Pts',(-0.252918200583262,1.798100095319,9.82610226424988));
#26415=CARTESIAN_POINT('Ctrl Pts',(-0.268425312378988,1.81180398102266,
9.82506048841938));
#26416=CARTESIAN_POINT('Ctrl Pts',(-0.28274208275248,1.82661052573153,9.82401871258888));
#26417=CARTESIAN_POINT('Ctrl Pts',(-0.297089799150026,1.84144907512279,
9.82297468493629));
#26418=CARTESIAN_POINT('Ctrl Pts',(-0.310241568742107,1.85739447375073,
9.82193065728369));
#26419=CARTESIAN_POINT('Ctrl Pts',(-0.322039591148359,1.87422269438006,
9.8208866296311));
#26420=CARTESIAN_POINT('Ctrl Pts',(-0.326212397027945,1.88017461543658,
9.82051737073523));
#26421=CARTESIAN_POINT('Ctrl Pts',(-0.330216261237806,1.88623671948787,
9.82014811183935));
#26422=CARTESIAN_POINT('Ctrl Pts',(-0.334045571701636,1.89239834772689,
9.81977885294348));
#26423=CARTESIAN_POINT('Ctrl Pts',(-0.345174432997193,1.91030546355741,
9.81870570124343));
#26424=CARTESIAN_POINT('Ctrl Pts',(-0.354888865172677,1.92915663330112,
9.81763254954337));
#26425=CARTESIAN_POINT('Ctrl Pts',(-0.363036937996751,1.94870865308967,
9.81655939784331));
#26426=CARTESIAN_POINT('Ctrl Pts',(-0.371166121038456,1.96821534517844,
9.81548873404469));
#26427=CARTESIAN_POINT('Ctrl Pts',(-0.37773584337263,1.98841906398911,9.81441807024606));
#26428=CARTESIAN_POINT('Ctrl Pts',(-0.38264005286215,2.00905232303324,9.81334740644744));
#26429=CARTESIAN_POINT('Ctrl Pts',(-0.38753456325213,2.02964477549401,9.81227886011032));
#26430=CARTESIAN_POINT('Ctrl Pts',(-0.390769912254042,2.05066443284332,
9.81121031377319));
#26431=CARTESIAN_POINT('Ctrl Pts',(-0.392289769156809,2.07182861354322,
9.81014176743606));
#26432=CARTESIAN_POINT('Ctrl Pts',(-0.392965586731042,2.08123945033659,
9.80966662902521));
#26433=CARTESIAN_POINT('Ctrl Pts',(-0.393302885292492,2.09067869849534,
9.80919149061435));
#26434=CARTESIAN_POINT('Ctrl Pts',(-0.393299981400419,2.10012095631365,
9.80871635220349));
#26435=CARTESIAN_POINT('',(-0.393383546135126,2.10030552476621,9.68371639062669));
#26436=CARTESIAN_POINT('Ctrl Pts',(-0.392686993440875,2.10012251542529,
9.80871626412467));
#26437=CARTESIAN_POINT('Ctrl Pts',(-0.392846725206061,2.15837609996444,
9.80578034589002));
#26438=CARTESIAN_POINT('Ctrl Pts',(-0.353358128587013,2.34784367211105,
9.79622097981441));
#26439=CARTESIAN_POINT('Ctrl Pts',(-0.0599518019945944,2.5611732916345,
9.78003816589791));
#26440=CARTESIAN_POINT('Ctrl Pts',(0.355309766950069,2.40004998415162,9.76016782237512));
#26441=CARTESIAN_POINT('Ctrl Pts',(0.444622995774978,1.96367166432625,9.74029747885231));
#26442=CARTESIAN_POINT('Ctrl Pts',(0.126055155931373,1.65235603305462,9.72042713532955));
#26443=CARTESIAN_POINT('Ctrl Pts',(-0.286080276586348,1.7466434788202,9.7015668080763));
#26444=CARTESIAN_POINT('Ctrl Pts',(-0.392665020011803,1.98959023483791,
9.68932992866398));
#26445=CARTESIAN_POINT('Ctrl Pts',(-0.393615372483065,2.10030360545593,
9.68371649709261));
#26446=CARTESIAN_POINT('',(-0.393409004503689,2.09971354421981,9.55871630428717));
#26447=CARTESIAN_POINT('Ctrl Pts',(-0.393299880791846,2.10030621743879,
9.68371635220349));
#26448=CARTESIAN_POINT('Ctrl Pts',(-0.39328438428292,2.12020964010897,9.68270638423031));
#26449=CARTESIAN_POINT('Ctrl Pts',(-0.391757774685968,2.14005558435781,
9.68169641625714));
#26450=CARTESIAN_POINT('Ctrl Pts',(-0.388747481156827,2.15966813131164,
9.68068644828397));
#26451=CARTESIAN_POINT('Ctrl Pts',(-0.38563586367384,2.17994082013638,9.67964248563642));
#26452=CARTESIAN_POINT('Ctrl Pts',(-0.380924912859241,2.20002985697604,
9.67859852298887));
#26453=CARTESIAN_POINT('Ctrl Pts',(-0.374653403290349,2.21966502163522,
9.67755456034132));
#26454=CARTESIAN_POINT('Ctrl Pts',(-0.368393430839102,2.23926406529322,
9.67651251817555));
#26455=CARTESIAN_POINT('Ctrl Pts',(-0.360578762777487,2.25841018303383,
9.67547047600978));
#26456=CARTESIAN_POINT('Ctrl Pts',(-0.35129889117364,2.27684450531518,9.67442843384401));
#26457=CARTESIAN_POINT('Ctrl Pts',(-0.342028986006111,2.295259029424,9.67338751081515));
#26458=CARTESIAN_POINT('Ctrl Pts',(-0.331297304606908,2.31296260882839,
9.6723465877863));
#26459=CARTESIAN_POINT('Ctrl Pts',(-0.319240858292976,2.32971757528836,
9.67130566475744));
#26460=CARTESIAN_POINT('Ctrl Pts',(-0.30717822010245,2.34648114666242,9.67026420713765));
#26461=CARTESIAN_POINT('Ctrl Pts',(-0.29378987444691,2.36229452516412,9.66922274951785));
#26462=CARTESIAN_POINT('Ctrl Pts',(-0.279255674830849,2.37694973925745,
9.66818129189805));
#26463=CARTESIAN_POINT('Ctrl Pts',(-0.264717034383171,2.39160943115759,
9.66713951606755));
#26464=CARTESIAN_POINT('Ctrl Pts',(-0.249032386357423,2.40510975766971,
9.66609774023705));
#26465=CARTESIAN_POINT('Ctrl Pts',(-0.232417124113025,2.41728090144071,
9.66505596440655));
#26466=CARTESIAN_POINT('Ctrl Pts',(-0.215765947602234,2.42947835341517,
9.66401193675395));
#26467=CARTESIAN_POINT('Ctrl Pts',(-0.198180767506498,2.44034049969521,
9.66296790910135));
#26468=CARTESIAN_POINT('Ctrl Pts',(-0.179904982235449,2.44974145788977,
9.66192388144875));
#26469=CARTESIAN_POINT('Ctrl Pts',(-0.173441076539635,2.45306645357771,
9.66155462255288));
#26470=CARTESIAN_POINT('Ctrl Pts',(-0.166890975759392,2.45620909799058,
9.66118536365702));
#26471=CARTESIAN_POINT('Ctrl Pts',(-0.1602660026435,2.45916528005456,9.66081610476116));
#26472=CARTESIAN_POINT('Ctrl Pts',(-0.141535988142762,2.46752294912835,
9.6597721421136));
#26473=CARTESIAN_POINT('Ctrl Pts',(-0.122094643488743,2.47443645596392,
9.65872817946605));
#26474=CARTESIAN_POINT('Ctrl Pts',(-0.102190164039155,2.47979212784581,
9.65768421681849));
#26475=CARTESIAN_POINT('Ctrl Pts',(-0.0823223010243468,2.48513794739217,
9.65664217465272));
#26476=CARTESIAN_POINT('Ctrl Pts',(-0.0619936814047709,2.48893137405054,
9.65560013248695));
#26477=CARTESIAN_POINT('Ctrl Pts',(-0.04147041099965,2.4911075235936,9.65455809032118));
#26478=CARTESIAN_POINT('Ctrl Pts',(-0.0209691822645188,2.49328133598625,
9.65351716729233));
#26479=CARTESIAN_POINT('Ctrl Pts',(-0.000274442679066934,2.49384121353664,
9.65247624426348));
#26480=CARTESIAN_POINT('Ctrl Pts',(0.0203398053437122,2.49277370370046,
9.65143532123462));
#26481=CARTESIAN_POINT('Ctrl Pts',(0.0409646403069961,2.49170564561906,
9.65039386361483));
#26482=CARTESIAN_POINT('Ctrl Pts',(0.0615081654954153,2.4890085523944,9.64935240599504));
#26483=CARTESIAN_POINT('Ctrl Pts',(0.0816981567661531,2.48472106932297,
9.64831094837525));
#26484=CARTESIAN_POINT('Ctrl Pts',(0.101894316959437,2.48043227623855,9.64726917254476));
#26485=CARTESIAN_POINT('Ctrl Pts',(0.121736016585802,2.47455231403098,9.64622739671426));
#26486=CARTESIAN_POINT('Ctrl Pts',(0.140963873856919,2.46717036409173,9.64518562088376));
#26487=CARTESIAN_POINT('Ctrl Pts',(0.16023329257786,2.45977245790016,9.64414159323117));
#26488=CARTESIAN_POINT('Ctrl Pts',(0.178885555380011,2.45086639967178,9.64309756557857));
#26489=CARTESIAN_POINT('Ctrl Pts',(0.196683062138064,2.44058870073447,9.64205353792598));
#26490=CARTESIAN_POINT('Ctrl Pts',(0.202977806993071,2.43695361333788,9.64168427903011));
#26491=CARTESIAN_POINT('Ctrl Pts',(0.209165886587755,2.43314734153095,9.64131502013425));
#26492=CARTESIAN_POINT('Ctrl Pts',(0.21523771504915,2.42917718028506,9.64094576123838));
#26493=CARTESIAN_POINT('Ctrl Pts',(0.232403888124444,2.4179528060266,9.63990179859083));
#26494=CARTESIAN_POINT('Ctrl Pts',(0.248740839597912,2.40534858152543,9.63885783594327));
#26495=CARTESIAN_POINT('Ctrl Pts',(0.2640186387834,2.39151166078728,9.63781387329572));
#26496=CARTESIAN_POINT('Ctrl Pts',(0.279268332811009,2.37770019455585,9.63677183112995));
#26497=CARTESIAN_POINT('Ctrl Pts',(0.293462162979261,2.36266097760134,9.63572978896418));
#26498=CARTESIAN_POINT('Ctrl Pts',(0.306401525579946,2.34658263345638,9.63468774679841));
#26499=CARTESIAN_POINT('Ctrl Pts',(0.319326991508474,2.33052155720044,9.63364682376956));
#26500=CARTESIAN_POINT('Ctrl Pts',(0.331000183044926,2.3134241214648,9.6326059007407));
#26501=CARTESIAN_POINT('Ctrl Pts',(0.34126146659212,2.29551343027883,9.63156497771185));
#26502=CARTESIAN_POINT('Ctrl Pts',(0.351528020067099,2.27759354062869,9.63052352009206));
#26503=CARTESIAN_POINT('Ctrl Pts',(0.360380837176447,2.25886019153521,9.62948206247227));
#26504=CARTESIAN_POINT('Ctrl Pts',(0.367705051730088,2.23956319332895,9.62844060485247));
#26505=CARTESIAN_POINT('Ctrl Pts',(0.375031504150583,2.22026029904846,9.62739882902198));
#26506=CARTESIAN_POINT('Ctrl Pts',(0.380828197173872,2.20039411296208,9.62635705319148));
#26507=CARTESIAN_POINT('Ctrl Pts',(0.385029708061865,2.1802310034201,9.62531527736098));
#26508=CARTESIAN_POINT('Ctrl Pts',(0.389240300610986,2.16002431085928,9.62427124970838));
#26509=CARTESIAN_POINT('Ctrl Pts',(0.391848734274883,2.13952014409667,9.62322722205578));
#26510=CARTESIAN_POINT('Ctrl Pts',(0.392841172981202,2.1189921776201,9.62218319440319));
#26511=CARTESIAN_POINT('Ctrl Pts',(0.393192185542986,2.11173170495285,9.62181393550732));
#26512=CARTESIAN_POINT('Ctrl Pts',(0.393341523354874,2.10446825313182,9.62144467661145));
#26513=CARTESIAN_POINT('Ctrl Pts',(0.393290131153164,2.09721383103047,9.62107541771558));
#26514=CARTESIAN_POINT('Ctrl Pts',(0.393144835969863,2.07670424876133,9.62003145506803));
#26515=CARTESIAN_POINT('Ctrl Pts',(0.391390465360976,2.05614495299302,9.61898749242048));
#26516=CARTESIAN_POINT('Ctrl Pts',(0.388026283414218,2.03580893068542,9.61794352977292));
#26517=CARTESIAN_POINT('Ctrl Pts',(0.384668290242663,2.0155103186822,9.61690148760715));
#26518=CARTESIAN_POINT('Ctrl Pts',(0.379706424095702,1.99543489226606,9.61585944544138));
#26519=CARTESIAN_POINT('Ctrl Pts',(0.373191775240968,1.97585174631718,9.61481740327561));
#26520=CARTESIAN_POINT('Ctrl Pts',(0.36668412301676,1.95628963235939,9.61377648024676));
#26521=CARTESIAN_POINT('Ctrl Pts',(0.358627202431044,1.93721945301948,9.6127355572179));
#26522=CARTESIAN_POINT('Ctrl Pts',(0.349122190795714,1.91889620132642,9.61169463418905));
#26523=CARTESIAN_POINT('Ctrl Pts',(0.339612297634139,1.90056353928885,9.61065317656926));
#26524=CARTESIAN_POINT('Ctrl Pts',(0.328653152168805,1.88297923180463,9.60961171894947));
#26525=CARTESIAN_POINT('Ctrl Pts',(0.316392620254153,1.86637508726869,9.60857026132967));
#26526=CARTESIAN_POINT('Ctrl Pts',(0.304128342212484,1.84976586944272,9.60752848549918));
#26527=CARTESIAN_POINT('Ctrl Pts',(0.29056235193232,1.83413798067474,9.60648670966868));
#26528=CARTESIAN_POINT('Ctrl Pts',(0.275883202181507,1.8196906195753,9.60544493383818));
#26529=CARTESIAN_POINT('Ctrl Pts',(0.261172323115398,1.805212030177,9.60440090618558));
#26530=CARTESIAN_POINT('Ctrl Pts',(0.245344044860583,1.79191953649461,9.60335687853298));
#26531=CARTESIAN_POINT('Ctrl Pts',(0.228620988110442,1.77997291709075,9.60231285088039));
#26532=CARTESIAN_POINT('Ctrl Pts',(0.22270626213964,1.77574755440096,9.60194359198452));
#26533=CARTESIAN_POINT('Ctrl Pts',(0.216679861056863,1.77169015078198,9.60157433308866));
#26534=CARTESIAN_POINT('Ctrl Pts',(0.210552393540732,1.76780641250279,9.60120507419279));
#26535=CARTESIAN_POINT('Ctrl Pts',(0.193228918649381,1.75682637182742,9.60016111154524));
#26536=CARTESIAN_POINT('Ctrl Pts',(0.174992622155822,1.74717235976401,9.59911714889769));
#26537=CARTESIAN_POINT('Ctrl Pts',(0.156072638020975,1.73899276785475,9.59807318625014));
#26538=CARTESIAN_POINT('Ctrl Pts',(0.137187459235691,1.73082822318621,9.59703114408437));
#26539=CARTESIAN_POINT('Ctrl Pts',(0.117621733466298,1.72413305802274,9.5959891019186));
#26540=CARTESIAN_POINT('Ctrl Pts',(0.0976293765910314,1.71900998067345,
9.59494705975283));
#26541=CARTESIAN_POINT('Ctrl Pts',(0.0776584911929713,1.71389240542875,
9.59390613672398));
#26542=CARTESIAN_POINT('Ctrl Pts',(0.0572625862718146,1.71034377585844,
9.59286521369513));
#26543=CARTESIAN_POINT('Ctrl Pts',(0.0367108336389134,1.70841705260119,
9.59182429066628));
#26544=CARTESIAN_POINT('Ctrl Pts',(0.0161485261615035,1.7064893398291,9.59078283304649));
#26545=CARTESIAN_POINT('Ctrl Pts',(-0.00456905786697798,1.7061852821836,
9.5897413754267));
#26546=CARTESIAN_POINT('Ctrl Pts',(-0.0251669673389064,1.70750603347954,
9.58869991780691));
#26547=CARTESIAN_POINT('Ctrl Pts',(-0.0457711703701748,1.70882718832258,
9.58765814197641));
#26548=CARTESIAN_POINT('Ctrl Pts',(-0.0662548947145264,1.71177405727269,
9.58661636614591));
#26549=CARTESIAN_POINT('Ctrl Pts',(-0.0863485835935361,1.7162959315939,
9.58557459031542));
#26550=CARTESIAN_POINT('Ctrl Pts',(-0.106485705437037,1.72082758004908,
9.58453056266282));
#26551=CARTESIAN_POINT('Ctrl Pts',(-0.126230405137249,1.72694081279087,
9.58348653501023));
#26552=CARTESIAN_POINT('Ctrl Pts',(-0.145327829414169,1.73453493737737,
9.58244250735763));
#26553=CARTESIAN_POINT('Ctrl Pts',(-0.152082338056697,1.73722087970174,
9.58207324846176));
#26554=CARTESIAN_POINT('Ctrl Pts',(-0.158756075461235,1.7400916397396,9.58170398956589));
#26555=CARTESIAN_POINT('Ctrl Pts',(-0.165338501025232,1.74314138643052,
9.58133473067002));
#26556=CARTESIAN_POINT('Ctrl Pts',(-0.183948225790025,1.75176357987102,
9.58029076802246));
#26557=CARTESIAN_POINT('Ctrl Pts',(-0.201937128783059,1.76187109330564,
9.5792468053749));
#26558=CARTESIAN_POINT('Ctrl Pts',(-0.219056405385582,1.77335159382059,
9.57820284272735));
#26559=CARTESIAN_POINT('Ctrl Pts',(-0.236144189234087,1.78481097471775,
9.57716080056158));
#26560=CARTESIAN_POINT('Ctrl Pts',(-0.252364884865585,1.79763797338003,
9.57611875839581));
#26561=CARTESIAN_POINT('Ctrl Pts',(-0.267494684041996,1.81167469065434,
9.57507671623003));
#26562=CARTESIAN_POINT('Ctrl Pts',(-0.282608234051773,1.8256963327148,9.57403579320118));
#26563=CARTESIAN_POINT('Ctrl Pts',(-0.296632657194975,1.84092463744261,
9.57299487017232));
#26564=CARTESIAN_POINT('Ctrl Pts',(-0.309377715653273,1.85716194891006,
9.57195394714347));
#26565=CARTESIAN_POINT('Ctrl Pts',(-0.322129319641413,1.87340759943747,
9.57091248952367));
#26566=CARTESIAN_POINT('Ctrl Pts',(-0.333599779331321,1.89066272312678,
9.56987103190388));
#26567=CARTESIAN_POINT('Ctrl Pts',(-0.343639288572217,1.90869676074467,
9.56882957428409));
#26568=CARTESIAN_POINT('Ctrl Pts',(-0.353681865320874,1.92673630854728,
9.56778779845359));
#26569=CARTESIAN_POINT('Ctrl Pts',(-0.362292295250751,1.94555458413378,
9.56674602262309));
#26570=CARTESIAN_POINT('Ctrl Pts',(-0.369367299220206,1.96489748978361,
9.56570424679258));
#26571=CARTESIAN_POINT('Ctrl Pts',(-0.376457595971295,1.98428220556294,
9.56466021913999));
#26572=CARTESIAN_POINT('Ctrl Pts',(-0.382005643140109,2.00419310592989,
9.56361619148739));
#26573=CARTESIAN_POINT('Ctrl Pts',(-0.385958148049284,2.02436139904541,
9.56257216383479));
#26574=CARTESIAN_POINT('Ctrl Pts',(-0.387356097227164,2.03149465995919,
9.56220290493893));
#26575=CARTESIAN_POINT('Ctrl Pts',(-0.388554925431945,2.03866005213765,
9.56183364604307));
#26576=CARTESIAN_POINT('Ctrl Pts',(-0.389553829705013,2.04584555639509,
9.56146438714721));
#26577=CARTESIAN_POINT('Ctrl Pts',(-0.392031787472687,2.06367046371548,
9.56054837549931));
#26578=CARTESIAN_POINT('Ctrl Pts',(-0.39328671362501,2.08166924724648,9.5596323638514));
#26579=CARTESIAN_POINT('Ctrl Pts',(-0.393299895050531,2.09971267920167,
9.55871635220349));
#26580=CARTESIAN_POINT('',(-0.393077129544589,2.09984967721303,9.43371639324307));
#26581=CARTESIAN_POINT('Ctrl Pts',(-0.393666275384297,2.09971558385956,
9.55871619130454));
#26582=CARTESIAN_POINT('Ctrl Pts',(-0.392741356830577,2.21224405877622,
9.5530088087445));
#26583=CARTESIAN_POINT('Ctrl Pts',(-0.283104739668165,2.45693363482398,
9.54067797834354));
#26584=CARTESIAN_POINT('Ctrl Pts',(0.132384636875694,2.54581311263665,9.52172370010165));
#26585=CARTESIAN_POINT('Ctrl Pts',(0.446509843093515,2.2300153202515,9.50185335657885));
#26586=CARTESIAN_POINT('Ctrl Pts',(0.351023055099136,1.79494617152333,9.48198301305608));
#26587=CARTESIAN_POINT('Ctrl Pts',(-0.0664795984751189,1.63972238109351,
9.46211266953325));
#26588=CARTESIAN_POINT('Ctrl Pts',(-0.355148157932989,1.85592482976135,
9.44602381903774));
#26589=CARTESIAN_POINT('Ctrl Pts',(-0.392897886971203,2.0434661290281,9.43655841638312));
#26590=CARTESIAN_POINT('Ctrl Pts',(-0.392706122236906,2.09984846278313,
9.43371646156944));
#26591=CARTESIAN_POINT('',(-0.39329984275683,2.10035169226946,9.30871635220092));
#26592=CARTESIAN_POINT('Ctrl Pts',(-0.393299971550761,2.09985040664878,
9.43371635220349));
#26593=CARTESIAN_POINT('Ctrl Pts',(-0.393308015136027,2.12099801668889,
9.43265201369966));
#26594=CARTESIAN_POINT('Ctrl Pts',(-0.391606066910142,2.14213467488965,
9.43158767519583));
#26595=CARTESIAN_POINT('Ctrl Pts',(-0.388225481374075,2.1629751189905,9.430523336692));
#26596=CARTESIAN_POINT('Ctrl Pts',(-0.384842081218753,2.18383291449827,
9.42945811203764));
#26597=CARTESIAN_POINT('Ctrl Pts',(-0.379777418637733,2.20439333155889,
9.42839288738329));
#26598=CARTESIAN_POINT('Ctrl Pts',(-0.373113810665123,2.22438237130297,
9.42732766272893));
#26599=CARTESIAN_POINT('Ctrl Pts',(-0.366430817956512,2.24442956006482,
9.42625933928804));
#26600=CARTESIAN_POINT('Ctrl Pts',(-0.358139858177786,2.26390141332144,
9.42519101584714));
#26601=CARTESIAN_POINT('Ctrl Pts',(-0.348371642207012,2.28254338910514,
9.42412269240625));
#26602=CARTESIAN_POINT('Ctrl Pts',(-0.343035769838522,2.29272653859486,
9.42353912243339));
#26603=CARTESIAN_POINT('Ctrl Pts',(-0.337259910800024,2.30266250215418,
9.42295555246054));
#26604=CARTESIAN_POINT('Ctrl Pts',(-0.331070784138775,2.31231350849566,
9.42237198248769));
#26605=CARTESIAN_POINT('Ctrl Pts',(-0.319998903548804,2.32957843061383,
9.42132801984014));
#26606=CARTESIAN_POINT('Ctrl Pts',(-0.307539881826998,2.3460263860022,9.42028405719258));
#26607=CARTESIAN_POINT('Ctrl Pts',(-0.29383883054216,2.36142614954441,9.41924009454503));
#26608=CARTESIAN_POINT('Ctrl Pts',(-0.280162983817534,2.37679758356217,
9.41819805237926));
#26609=CARTESIAN_POINT('Ctrl Pts',(-0.265250081977773,2.39112407022735,
9.41715601021349));
#26610=CARTESIAN_POINT('Ctrl Pts',(-0.249286981977645,2.4042053428467,9.41611396804772));
#26611=CARTESIAN_POINT('Ctrl Pts',(-0.233341026096144,2.41727256638475,
9.41507304501887));
#26612=CARTESIAN_POINT('Ctrl Pts',(-0.216347659082994,2.42909674445078,
9.41403212199002));
#26613=CARTESIAN_POINT('Ctrl Pts',(-0.198528562223755,2.43951627351479,
9.41299119896117));
#26614=CARTESIAN_POINT('Ctrl Pts',(-0.180700313940784,2.44994115377736,
9.41194974134137));
#26615=CARTESIAN_POINT('Ctrl Pts',(-0.162046115631449,2.45895955854018,
9.41090828372158));
#26616=CARTESIAN_POINT('Ctrl Pts',(-0.142814750372396,2.46645441336689,
9.40986682610179));
#26617=CARTESIAN_POINT('Ctrl Pts',(-0.123577509092841,2.4739515581985,9.40882505027129));
#26618=CARTESIAN_POINT('Ctrl Pts',(-0.10376344790945,2.47992399313295,9.4077832744408));
#26619=CARTESIAN_POINT('Ctrl Pts',(-0.083638345225797,2.48430393857973,
9.4067414986103));
#26620=CARTESIAN_POINT('Ctrl Pts',(-0.0634697416759932,2.48869335137798,
9.4056974709577));
#26621=CARTESIAN_POINT('Ctrl Pts',(-0.042989484103173,2.49148330309068,
9.40465344330511));
#26622=CARTESIAN_POINT('Ctrl Pts',(-0.0224711137025956,2.49265753405349,
9.40360941565251));
#26623=CARTESIAN_POINT('Ctrl Pts',(-0.0152140350416648,2.4930728441535,
9.40324015675664));
#26624=CARTESIAN_POINT('Ctrl Pts',(-0.00795219096330203,2.49328651380395,
9.40287089786078));
#26625=CARTESIAN_POINT('Ctrl Pts',(-0.000697598238044414,2.49329938133272,
9.40250163896491));
#26626=CARTESIAN_POINT('Ctrl Pts',(0.0198124664162429,2.49333576019738,
9.40145767631736));
#26627=CARTESIAN_POINT('Ctrl Pts',(0.0403864953755422,2.49176356710999,
9.40041371366981));
#26628=CARTESIAN_POINT('Ctrl Pts',(0.0607515189078829,2.48857964814229,
9.39936975102225));
#26629=CARTESIAN_POINT('Ctrl Pts',(0.0810790787849739,2.48540158633661,
9.39832770885648));
#26630=CARTESIAN_POINT('Ctrl Pts',(0.101197668504876,2.48061773755848,9.39728566669072));
#26631=CARTESIAN_POINT('Ctrl Pts',(0.12083775120033,2.47427680650135,9.39624362452495));
#26632=CARTESIAN_POINT('Ctrl Pts',(0.140456740755505,2.46794268550456,9.39520270149609));
#26633=CARTESIAN_POINT('Ctrl Pts',(0.159597537992918,2.46005499950062,9.39416177846724));
#26634=CARTESIAN_POINT('Ctrl Pts',(0.178004263685736,2.45071266317272,9.39312085543838));
#26635=CARTESIAN_POINT('Ctrl Pts',(0.196420442593136,2.44136552886436,9.39207939781859));
#26636=CARTESIAN_POINT('Ctrl Pts',(0.214101133391507,2.4305625703843,9.3910379401988));
#26637=CARTESIAN_POINT('Ctrl Pts',(0.230813227024003,2.41844959448988,9.38999648257901));
#26638=CARTESIAN_POINT('Ctrl Pts',(0.247530426929695,2.40633291755323,9.38895470674851));
#26639=CARTESIAN_POINT('Ctrl Pts',(0.263277866491292,2.39290588709676,9.38791293091801));
#26640=CARTESIAN_POINT('Ctrl Pts',(0.27785468476336,2.37835528404371,9.38687115508751));
#26641=CARTESIAN_POINT('Ctrl Pts',(0.292463011158912,2.36377322953197,9.38582712743492));
#26642=CARTESIAN_POINT('Ctrl Pts',(0.30589518599026,2.34806331355167,9.38478309978232));
#26643=CARTESIAN_POINT('Ctrl Pts',(0.317989465048927,2.33144673278726,9.38373907212972));
#26644=CARTESIAN_POINT('Ctrl Pts',(0.322267053023165,2.32556966597691,9.38336981323386));
#26645=CARTESIAN_POINT('Ctrl Pts',(0.326377677703724,2.3195794406995,9.38300055433799));
#26646=CARTESIAN_POINT('Ctrl Pts',(0.33031553907667,2.31348661467288,9.38263129544212));
#26647=CARTESIAN_POINT('Ctrl Pts',(0.34144859566814,2.29626107762825,9.38158733279456));
#26648=CARTESIAN_POINT('Ctrl Pts',(0.351263761195903,2.27811100918802,9.38054337014701));
#26649=CARTESIAN_POINT('Ctrl Pts',(0.359610620332432,2.25926421991183,9.37949940749946));
#26650=CARTESIAN_POINT('Ctrl Pts',(0.367942124522152,2.24045210133538,9.37845736533369));
#26651=CARTESIAN_POINT('Ctrl Pts',(0.374810334952862,2.22094644710565,9.37741532316792));
#26652=CARTESIAN_POINT('Ctrl Pts',(0.380110298226388,2.20100025337714,9.37637328100215));
#26653=CARTESIAN_POINT('Ctrl Pts',(0.385404569422622,2.18107548154733,9.37533235797329));
#26654=CARTESIAN_POINT('Ctrl Pts',(0.389133721203222,2.16071180957053,9.37429143494444));
#26655=CARTESIAN_POINT('Ctrl Pts',(0.391242410755887,2.1401779295873,9.37325051191559));
#26656=CARTESIAN_POINT('Ctrl Pts',(0.393352183276546,2.1196335039385,9.37220905429579));
#26657=CARTESIAN_POINT('Ctrl Pts',(0.393839739765151,2.09891942593101,9.371167596676));
#26658=CARTESIAN_POINT('Ctrl Pts',(0.392701491009382,2.07831062566582,9.37012613905621));
#26659=CARTESIAN_POINT('Ctrl Pts',(0.391562894468995,2.05769552851368,9.36908436322571));
#26660=CARTESIAN_POINT('Ctrl Pts',(0.388797580431339,2.03718650518495,9.36804258739521));
#26661=CARTESIAN_POINT('Ctrl Pts',(0.384453867981806,2.01705355104751,9.36700081156471));
#26662=CARTESIAN_POINT('Ctrl Pts',(0.380100766499244,1.99687707907284,9.36595678391212));
#26663=CARTESIAN_POINT('Ctrl Pts',(0.374162666806837,1.97707900459952,9.36491275625952));
#26664=CARTESIAN_POINT('Ctrl Pts',(0.366737999974684,1.95791506281604,9.36386872860693));
#26665=CARTESIAN_POINT('Ctrl Pts',(0.364111992636864,1.95113702780348,9.36349946971106));
#26666=CARTESIAN_POINT('Ctrl Pts',(0.361300459386208,1.94443812379475,9.3631302108152));
#26667=CARTESIAN_POINT('Ctrl Pts',(0.358309137688568,1.93782894262886,9.36276095191933));
#26668=CARTESIAN_POINT('Ctrl Pts',(0.349852122423335,1.91914357486826,9.36171698927178));
#26669=CARTESIAN_POINT('Ctrl Pts',(0.33990434636196,1.9010658479604,9.36067302662422));
#26670=CARTESIAN_POINT('Ctrl Pts',(0.328575934167167,1.88384555177796,9.35962906397667));
#26671=CARTESIAN_POINT('Ctrl Pts',(0.31726836180732,1.86665693418596,9.3585870218109));
#26672=CARTESIAN_POINT('Ctrl Pts',(0.304585544901078,1.85032325680539,9.35754497964513));
#26673=CARTESIAN_POINT('Ctrl Pts',(0.290683393974063,1.83506971772234,9.35650293747936));
#26674=CARTESIAN_POINT('Ctrl Pts',(0.276796173738736,1.81983256070063,9.35546201445051));
#26675=CARTESIAN_POINT('Ctrl Pts',(0.26169269098198,1.8056737995261,9.35442109142165));
#26676=CARTESIAN_POINT('Ctrl Pts',(0.245568908802071,1.79278541533684,9.3533801683928));
#26677=CARTESIAN_POINT('Ctrl Pts',(0.229436845867876,1.77989041200937,9.35233871077301));
#26678=CARTESIAN_POINT('Ctrl Pts',(0.212284001343244,1.76826756107926,9.35129725315322));
#26679=CARTESIAN_POINT('Ctrl Pts',(0.194339598474054,1.75806870505181,9.35025579553342));
#26680=CARTESIAN_POINT('Ctrl Pts',(0.176389712807485,1.74786673282922,9.34921401970293));
#26681=CARTESIAN_POINT('Ctrl Pts',(0.157648444336629,1.73908995348095,9.34817224387243));
#26682=CARTESIAN_POINT('Ctrl Pts',(0.138368965994907,1.73184389282602,9.34713046804193));
#26683=CARTESIAN_POINT('Ctrl Pts',(0.119047814623232,1.72458216964655,9.34608644038933));
#26684=CARTESIAN_POINT('Ctrl Pts',(0.0991868384755821,1.71885797474502,
9.34504241273674));
#26685=CARTESIAN_POINT('Ctrl Pts',(0.0790543467939964,1.71472697959372,
9.34399838508414));
#26686=CARTESIAN_POINT('Ctrl Pts',(0.0719337483779574,1.71326590075678,
9.34362912618827));
#26687=CARTESIAN_POINT('Ctrl Pts',(0.0647792561978769,1.71200365047125,
9.34325986729241));
#26688=CARTESIAN_POINT('Ctrl Pts',(0.0576028818555596,1.71094113812697,
9.34289060839654));
#26689=CARTESIAN_POINT('Ctrl Pts',(0.0373139549208018,1.70793722078765,
9.34184664574899));
#26690=CARTESIAN_POINT('Ctrl Pts',(0.0167289675391714,1.70651568878983,
9.34080268310143));
#26691=CARTESIAN_POINT('Ctrl Pts',(-0.00388244002228689,1.7067191631169,
9.33975872045388));
#26692=CARTESIAN_POINT('Ctrl Pts',(-0.0244559306785246,1.70692226313101,
9.33871667828811));
#26693=CARTESIAN_POINT('Ctrl Pts',(-0.0450550170198653,1.70874448796688,
9.33767463612234));
#26694=CARTESIAN_POINT('Ctrl Pts',(-0.0654059512788471,1.71217664905616,
9.33663259395657));
#26695=CARTESIAN_POINT('Ctrl Pts',(-0.0857350289541158,1.71560512405834,
9.33559167092772));
#26696=CARTESIAN_POINT('Ctrl Pts',(-0.105815756972389,1.72064000952241,
9.33455074789886));
#26697=CARTESIAN_POINT('Ctrl Pts',(-0.125380635789518,1.72722045902569,
9.33350982487001));
#26698=CARTESIAN_POINT('Ctrl Pts',(-0.144955562618521,1.73380428807634,
9.33246836725022));
#26699=CARTESIAN_POINT('Ctrl Pts',(-0.164013408453982,1.74193504764372,
9.33142690963042));
#26700=CARTESIAN_POINT('Ctrl Pts',(-0.182302418713991,1.75150219781033,
9.33038545201063));
#26701=CARTESIAN_POINT('Ctrl Pts',(-0.200597017063961,1.76107227115841,
9.32934367618013));
#26702=CARTESIAN_POINT('Ctrl Pts',(-0.218121677539342,1.77207923599203,
9.32830190034963));
#26703=CARTESIAN_POINT('Ctrl Pts',(-0.234650625058717,1.78436734300844,
9.32726012451913));
#26704=CARTESIAN_POINT('Ctrl Pts',(-0.251215300273235,1.796682011047,9.32621609686654));
#26705=CARTESIAN_POINT('Ctrl Pts',(-0.26677941108841,1.81028286526066,9.32517206921394));
#26706=CARTESIAN_POINT('Ctrl Pts',(-0.281150907292824,1.82497444240867,
9.32412804156134));
#26707=CARTESIAN_POINT('Ctrl Pts',(-0.286233917122273,1.83017066067233,
9.32375878266548));
#26708=CARTESIAN_POINT('Ctrl Pts',(-0.29116809565268,1.83550300690712,9.32338952376961));
#26709=CARTESIAN_POINT('Ctrl Pts',(-0.295946176155712,1.84096187381234,
9.32302026487375));
#26710=CARTESIAN_POINT('Ctrl Pts',(-0.309342113939787,1.85626648020972,
9.32198500203293));
#26711=CARTESIAN_POINT('Ctrl Pts',(-0.321591288173481,1.87266297689702,
9.32094973919211));
#26712=CARTESIAN_POINT('Ctrl Pts',(-0.332512749399159,1.88995200194476,
9.3199144763513));
#26713=CARTESIAN_POINT('Ctrl Pts',(-0.343414206542394,1.90720935988541,
9.31888110972956));
#26714=CARTESIAN_POINT('Ctrl Pts',(-0.352992325725242,1.92535541064501,
9.31784774310783));
#26715=CARTESIAN_POINT('Ctrl Pts',(-0.36110725838568,1.94415893371393,9.3168143764861));
#26716=CARTESIAN_POINT('Ctrl Pts',(-0.369213280638338,1.96294181002394,
9.31578214452788));
#26717=CARTESIAN_POINT('Ctrl Pts',(-0.375858982692616,1.98238005234684,
9.31474991256966));
#26718=CARTESIAN_POINT('Ctrl Pts',(-0.380951273679245,2.00221954652303,
9.31371768061144));
#26719=CARTESIAN_POINT('Ctrl Pts',(-0.386045781822523,2.0220676787104,9.31268499922486));
#26720=CARTESIAN_POINT('Ctrl Pts',(-0.389585330442199,2.04231668851366,
9.31165231783829));
#26721=CARTESIAN_POINT('Ctrl Pts',(-0.391527158554774,2.0626988724832,9.31061963645172));
#26722=CARTESIAN_POINT('Ctrl Pts',(-0.392720121168889,2.07522067259115,
9.30998520836897));
#26723=CARTESIAN_POINT('Ctrl Pts',(-0.393311073280722,2.08779251965456,
9.30935078028623));
#26724=CARTESIAN_POINT('Ctrl Pts',(-0.393299842756876,2.10035169221859,
9.30871635220349));
#26725=CARTESIAN_POINT('',(-0.393299999141086,2.09997400728266,9.18371635220034));
#26726=CARTESIAN_POINT('Ctrl Pts',(-0.39329984275683,2.10035169226946,9.30871635220092));
#26727=CARTESIAN_POINT('Ctrl Pts',(-0.393276918768292,2.1259877436425,9.30742134404343));
#26728=CARTESIAN_POINT('Ctrl Pts',(-0.390743538263717,2.15151131211032,
9.30612633588594));
#26729=CARTESIAN_POINT('Ctrl Pts',(-0.385788147102442,2.17650095133568,
9.30483132772845));
#26730=CARTESIAN_POINT('Ctrl Pts',(-0.3836434948974,2.18731625998109,9.30427085893595));
#26731=CARTESIAN_POINT('Ctrl Pts',(-0.381045787453246,2.19803185263539,
9.30371039014345));
#26732=CARTESIAN_POINT('Ctrl Pts',(-0.378004906977851,2.20861482541838,
9.30314992135095));
#26733=CARTESIAN_POINT('Ctrl Pts',(-0.372340781384306,2.22832730260418,
9.3021059587034));
#26734=CARTESIAN_POINT('Ctrl Pts',(-0.36511365658114,2.24765425595428,9.30106199605585));
#26735=CARTESIAN_POINT('Ctrl Pts',(-0.35639635214647,2.26633258903982,9.30001803340831));
#26736=CARTESIAN_POINT('Ctrl Pts',(-0.347695084132652,2.28497656131894,
9.29897599124254));
#26737=CARTESIAN_POINT('Ctrl Pts',(-0.337509331717907,2.30297359744135,
9.29793394907677));
#26738=CARTESIAN_POINT('Ctrl Pts',(-0.325960777005166,2.32007830845903,
9.29689190691101));
#26739=CARTESIAN_POINT('Ctrl Pts',(-0.314424625258767,2.33716464928578,
9.29585098388216));
#26740=CARTESIAN_POINT('Ctrl Pts',(-0.301528962527767,2.35335994465526,
9.29481006085331));
#26741=CARTESIAN_POINT('Ctrl Pts',(-0.287439908603183,2.36844587711901,
9.29376913782447));
#26742=CARTESIAN_POINT('Ctrl Pts',(-0.273343618907707,2.38353955732448,
9.29272768020468));
#26743=CARTESIAN_POINT('Ctrl Pts',(-0.258053204014208,2.3975221876711,9.29168622258489));
#26744=CARTESIAN_POINT('Ctrl Pts',(-0.241773502075295,2.4102103539443,9.29064476496511));
#26745=CARTESIAN_POINT('Ctrl Pts',(-0.225488825977706,2.42290239700545,
9.28960298913462));
#26746=CARTESIAN_POINT('Ctrl Pts',(-0.208214863174154,2.43429876522881,
9.28856121330412));
#26747=CARTESIAN_POINT('Ctrl Pts',(-0.190186851712651,2.44425840793745,
9.28751943747363));
#26748=CARTESIAN_POINT('Ctrl Pts',(-0.172119872295267,2.45423957863982,
9.28647540982104));
#26749=CARTESIAN_POINT('Ctrl Pts',(-0.153296260927022,2.46277751960126,
9.28543138216845));
#26750=CARTESIAN_POINT('Ctrl Pts',(-0.133973446854709,2.46977831945352,
9.28438735451586));
#26751=CARTESIAN_POINT('Ctrl Pts',(-0.127139220795381,2.47225441059674,
9.28401809561996));
#26752=CARTESIAN_POINT('Ctrl Pts',(-0.120242686105858,2.47453867052581,
9.28364883672406));
#26753=CARTESIAN_POINT('Ctrl Pts',(-0.113295596369067,2.47662846127633,
9.28327957782816));
#26754=CARTESIAN_POINT('Ctrl Pts',(-0.093654899083327,2.48253668314717,
9.28223561518061));
#26755=CARTESIAN_POINT('Ctrl Pts',(-0.0734922774274372,2.48692201627976,
9.28119165253306));
#26756=CARTESIAN_POINT('Ctrl Pts',(-0.053068366142764,2.48970326982839,
9.2801476898855));
#26757=CARTESIAN_POINT('Ctrl Pts',(-0.0326820268436989,2.49247940696142,
9.27910564771974));
#26758=CARTESIAN_POINT('Ctrl Pts',(-0.0120360648190486,2.49365716480032,
9.27806360555397));
#26759=CARTESIAN_POINT('Ctrl Pts',(0.00859732378919101,2.49320602236444,
9.2770215633882));
#26760=CARTESIAN_POINT('Ctrl Pts',(0.0292085524622095,2.49275536444845,
9.27598064035934));
#26761=CARTESIAN_POINT('Ctrl Pts',(0.0498065020218985,2.49067926634919,
9.27493971733049));
#26762=CARTESIAN_POINT('Ctrl Pts',(0.0701176836042718,2.48699922538162,
9.27389879430164));
#26763=CARTESIAN_POINT('Ctrl Pts',(0.0904392964801287,2.48331729444092,
9.27285733668184));
#26764=CARTESIAN_POINT('Ctrl Pts',(0.110473120288156,2.47802989028964,9.27181587906205));
#26765=CARTESIAN_POINT('Ctrl Pts',(0.129954054479622,2.47120995908557,9.27077442144226));
#26766=CARTESIAN_POINT('Ctrl Pts',(0.149440940945777,2.46438794409518,9.26973264561176));
#26767=CARTESIAN_POINT('Ctrl Pts',(0.168373919579263,2.45603274692879,9.26869086978126));
#26768=CARTESIAN_POINT('Ctrl Pts',(0.186507053839617,2.4462658066689,9.26764909395076));
#26769=CARTESIAN_POINT('Ctrl Pts',(0.20467938328117,2.436477754946,9.26660506629817));
#26770=CARTESIAN_POINT('Ctrl Pts',(0.222047797862864,2.4252722671955,9.26556103864557));
#26771=CARTESIAN_POINT('Ctrl Pts',(0.238393984122121,2.41281495861672,9.26451701099297));
#26772=CARTESIAN_POINT('Ctrl Pts',(0.24417541594022,2.40840897185975,9.26414775209711));
#26773=CARTESIAN_POINT('Ctrl Pts',(0.249829281426239,2.40384675318856,9.26377849320124));
#26774=CARTESIAN_POINT('Ctrl Pts',(0.255347000105666,2.39913675724831,9.26340923430538));
#26775=CARTESIAN_POINT('Ctrl Pts',(0.270946603163401,2.38582073456935,9.26236527165782));
#26776=CARTESIAN_POINT('Ctrl Pts',(0.285548261195769,2.37124150134435,9.26132130901027));
#26777=CARTESIAN_POINT('Ctrl Pts',(0.298942621191147,2.35557425385857,9.26027734636271));
#26778=CARTESIAN_POINT('Ctrl Pts',(0.31231234081799,2.33993582796278,9.25923530419694));
#26779=CARTESIAN_POINT('Ctrl Pts',(0.324478652988779,2.32321387503814,9.25819326203117));
#26780=CARTESIAN_POINT('Ctrl Pts',(0.335268550426577,2.30562074091604,9.2571512198654));
#26781=CARTESIAN_POINT('Ctrl Pts',(0.346046859684032,2.2880465015436,9.25611029683655));
#26782=CARTESIAN_POINT('Ctrl Pts',(0.355451281508906,2.26960354734637,9.25506937380769));
#26783=CARTESIAN_POINT('Ctrl Pts',(0.363351846764805,2.25053346954284,9.25402845077883));
#26784=CARTESIAN_POINT('Ctrl Pts',(0.371256469545107,2.23145359784438,9.25298699315904));
#26785=CARTESIAN_POINT('Ctrl Pts',(0.377655396282505,2.21174663268889,9.25194553553925));
#26786=CARTESIAN_POINT('Ctrl Pts',(0.38246645769543,2.19167496243746,9.25090407791946));
#26787=CARTESIAN_POINT('Ctrl Pts',(0.387278989097361,2.17159715941572,9.24986230208896));
#26788=CARTESIAN_POINT('Ctrl Pts',(0.390502553156715,2.15115515280235,9.24882052625846));
#26789=CARTESIAN_POINT('Ctrl Pts',(0.392106128135219,2.13062146761354,9.24777875042796));
#26790=CARTESIAN_POINT('Ctrl Pts',(0.393713169277429,2.11004339839823,9.24673472277536));
#26791=CARTESIAN_POINT('Ctrl Pts',(0.39369323118985,2.0893739914575,9.24569069512276));
#26792=CARTESIAN_POINT('Ctrl Pts',(0.392067389075343,2.06888645915934,9.24464666747017));
#26793=CARTESIAN_POINT('Ctrl Pts',(0.391492350030588,2.06164028753111,9.24427740857431));
#26794=CARTESIAN_POINT('Ctrl Pts',(0.390716894434591,2.05441680480078,9.24390814967844));
#26795=CARTESIAN_POINT('Ctrl Pts',(0.389743486338488,2.04722780223716,9.24353889078258));
#26796=CARTESIAN_POINT('Ctrl Pts',(0.386991483056925,2.02690317300357,9.24249492813503));
#26797=CARTESIAN_POINT('Ctrl Pts',(0.382637144057309,2.00673383512157,9.24145096548748));
#26798=CARTESIAN_POINT('Ctrl Pts',(0.376714450945086,1.98699065326646,9.24040700283993));
#26799=CARTESIAN_POINT('Ctrl Pts',(0.370802653265048,1.96728379112182,9.23936496067416));
#26800=CARTESIAN_POINT('Ctrl Pts',(0.363328380459119,1.94800224275369,9.23832291850839));
#26801=CARTESIAN_POINT('Ctrl Pts',(0.354376524739197,1.92940642241348,9.23728087634262));
#26802=CARTESIAN_POINT('Ctrl Pts',(0.345434283171689,1.91083057369218,9.23623995331377));
#26803=CARTESIAN_POINT('Ctrl Pts',(0.335017900533861,1.89293966309146,9.23519903028492));
#26804=CARTESIAN_POINT('Ctrl Pts',(0.323260156405853,1.87597374868006,9.23415810725606));
#26805=CARTESIAN_POINT('Ctrl Pts',(0.311496373806907,1.85899912101721,9.23311664963627));
#26806=CARTESIAN_POINT('Ctrl Pts',(0.298390259327344,1.84295105252664,9.23207519201648));
#26807=CARTESIAN_POINT('Ctrl Pts',(0.284117954082259,1.82804066817241,9.23103373439669));
#26808=CARTESIAN_POINT('Ctrl Pts',(0.269841288025699,1.81312572804571,9.2299919585662));
#26809=CARTESIAN_POINT('Ctrl Pts',(0.254398256335101,1.79934967012524,9.2289501827357));
#26810=CARTESIAN_POINT('Ctrl Pts',(0.238001210296019,1.78688610075944,9.2279084069052));
#26811=CARTESIAN_POINT('Ctrl Pts',(0.221568721669827,1.77439559110562,9.22686437925261));
#26812=CARTESIAN_POINT('Ctrl Pts',(0.20417872139403,1.76322363195713,9.22582035160001));
#26813=CARTESIAN_POINT('Ctrl Pts',(0.186072339707431,1.75350039769748,9.22477632394741));
#26814=CARTESIAN_POINT('Ctrl Pts',(0.179668349838829,1.75006141718958,9.22440706505155));
#26815=CARTESIAN_POINT('Ctrl Pts',(0.173174948101331,1.74680323241671,9.22403780615568));
#26816=CARTESIAN_POINT('Ctrl Pts',(0.166603382640256,1.7437301543874,9.22366854725981));
#26817=CARTESIAN_POINT('Ctrl Pts',(0.148024361378827,1.73504199897257,9.22262458461226));
#26818=CARTESIAN_POINT('Ctrl Pts',(0.128708538589659,1.72778517813287,9.2215806219647));
#26819=CARTESIAN_POINT('Ctrl Pts',(0.108902056998447,1.72207774346897,9.22053665931715));
#26820=CARTESIAN_POINT('Ctrl Pts',(0.089132011564391,1.71638080824614,9.21949461715138));
#26821=CARTESIAN_POINT('Ctrl Pts',(0.0688737815508266,1.71222786011648,
9.21845257498561));
#26822=CARTESIAN_POINT('Ctrl Pts',(0.0483922816111024,1.70968848712795,
9.21741053281984));
#26823=CARTESIAN_POINT('Ctrl Pts',(0.0279327784805518,1.70715184138611,
9.21636960979098));
#26824=CARTESIAN_POINT('Ctrl Pts',(0.00725120438777207,1.7062254492305,
9.21532868676212));
#26825=CARTESIAN_POINT('Ctrl Pts',(-0.0133787195590345,1.70692761498299,
9.21428776373327));
#26826=CARTESIAN_POINT('Ctrl Pts',(-0.0340192384970955,1.70763014134951,
9.21324630611348));
#26827=CARTESIAN_POINT('Ctrl Pts',(-0.0546073183950077,1.7099628876167,
9.21220484849368));
#26828=CARTESIAN_POINT('Ctrl Pts',(-0.0748700932346642,1.71389203693911,
9.21116339087389));
#26829=CARTESIAN_POINT('Ctrl Pts',(-0.0951390592354162,1.71782238678793,
9.21012161504339));
#26830=CARTESIAN_POINT('Ctrl Pts',(-0.115081807478783,1.72334993526144,
9.20907983921289));
#26831=CARTESIAN_POINT('Ctrl Pts',(-0.134437417050862,1.73039010985,9.20803806338239));
#26832=CARTESIAN_POINT('Ctrl Pts',(-0.153834864212262,1.7374455019357,9.20699403572979));
#26833=CARTESIAN_POINT('Ctrl Pts',(-0.172641968858013,1.74601974217327,
9.2059500080772));
#26834=CARTESIAN_POINT('Ctrl Pts',(-0.190618749880555,1.75598054968654,
9.2049059804246));
#26835=CARTESIAN_POINT('Ctrl Pts',(-0.196976901693017,1.75950355674018,
9.20453672152873));
#26836=CARTESIAN_POINT('Ctrl Pts',(-0.203231437474636,1.76319961089218,
9.20416746263287));
#26837=CARTESIAN_POINT('Ctrl Pts',(-0.209372643627946,1.76706158812741,
9.203798203737));
#26838=CARTESIAN_POINT('Ctrl Pts',(-0.226734960167222,1.77798010633889,
9.20275424108945));
#26839=CARTESIAN_POINT('Ctrl Pts',(-0.243292628948694,1.79029294773496,
9.2017102784419));
#26840=CARTESIAN_POINT('Ctrl Pts',(-0.258813148567935,1.80385705456933,
9.20066631579434));
#26841=CARTESIAN_POINT('Ctrl Pts',(-0.274305116518906,1.81739620876756,
9.19962427362858));
#26842=CARTESIAN_POINT('Ctrl Pts',(-0.288763135611631,1.83218162541249,
9.19858223146281));
#26843=CARTESIAN_POINT('Ctrl Pts',(-0.301985291880888,1.84802822878819,
9.19754018929704));
#26844=CARTESIAN_POINT('Ctrl Pts',(-0.315193247762026,1.86385781316081,
9.19649926626819));
#26845=CARTESIAN_POINT('Ctrl Pts',(-0.327167484621689,1.88074577813618,
9.19545834323933));
#26846=CARTESIAN_POINT('Ctrl Pts',(-0.337744441676624,1.89847188256587,
9.19441742021048));
#26847=CARTESIAN_POINT('Ctrl Pts',(-0.348326830781034,1.9162070906608,9.19337596259069));
#26848=CARTESIAN_POINT('Ctrl Pts',(-0.357510115604936,1.93478067456031,
9.1923345049709));
#26849=CARTESIAN_POINT('Ctrl Pts',(-0.365175022651471,1.95394489796143,
9.19129304735111));
#26850=CARTESIAN_POINT('Ctrl Pts',(-0.37284227166127,1.97311497686828,9.19025127152062));
#26851=CARTESIAN_POINT('Ctrl Pts',(-0.378989979904125,1.99287535851908,
9.18920949569012));
#26852=CARTESIAN_POINT('Ctrl Pts',(-0.383548016255117,2.01296087531021,
9.18816771985962));
#26853=CARTESIAN_POINT('Ctrl Pts',(-0.388115904905117,2.03308980740168,
9.18712369220703));
#26854=CARTESIAN_POINT('Ctrl Pts',(-0.391087155764448,2.05354454888473,
9.18607966455443));
#26855=CARTESIAN_POINT('Ctrl Pts',(-0.3924430868525,2.07405171331897,9.18503563690184));
#26856=CARTESIAN_POINT('Ctrl Pts',(-0.392922661905138,2.08130482857657,
9.18466637800597));
#26857=CARTESIAN_POINT('Ctrl Pts',(-0.393200646629442,2.08856449514136,
9.1842971191101));
#26858=CARTESIAN_POINT('Ctrl Pts',(-0.393277772879087,2.09581868928856,
9.18392786021423));
#26859=CARTESIAN_POINT('Ctrl Pts',(-0.393292498608396,2.09720373393763,
9.18385735754398));
#26860=CARTESIAN_POINT('Ctrl Pts',(-0.393299907597943,2.0985888565162,9.18378685487374));
#26861=CARTESIAN_POINT('Ctrl Pts',(-0.393299999141082,2.09997400722057,
9.1837163522035));
#26862=CARTESIAN_POINT('',(-0.393244728382793,2.09966251899669,9.05871635508085));
#26863=CARTESIAN_POINT('Ctrl Pts',(-0.393299999141086,2.09997400728267,
9.18371635220034));
#26864=CARTESIAN_POINT('Ctrl Pts',(-0.393301352116386,2.12044609480224,
9.18267434512414));
#26865=CARTESIAN_POINT('Ctrl Pts',(-0.391699967753018,2.14098035704797,
9.18163233804793));
#26866=CARTESIAN_POINT('Ctrl Pts',(-0.388492761615384,2.16130468312007,
9.18059033097173));
#26867=CARTESIAN_POINT('Ctrl Pts',(-0.385291446452698,2.18159167760493,
9.1795502378472));
#26868=CARTESIAN_POINT('Ctrl Pts',(-0.380490218272511,2.2016687703632,9.17851014472268));
#26869=CARTESIAN_POINT('Ctrl Pts',(-0.374137850478265,2.22126730325815,
9.17747005159816));
#26870=CARTESIAN_POINT('Ctrl Pts',(-0.367792238111552,2.24084499408711,
9.176431064561));
#26871=CARTESIAN_POINT('Ctrl Pts',(-0.359898959910504,2.25994442708309,
9.17539207752384));
#26872=CARTESIAN_POINT('Ctrl Pts',(-0.350556982617022,2.2783106613146,9.17435309048668));
#26873=CARTESIAN_POINT('Ctrl Pts',(-0.341210125737006,2.29668648876459,
9.17331356075636));
#26874=CARTESIAN_POINT('Ctrl Pts',(-0.330413379812743,2.31432768705437,
9.17227403102604));
#26875=CARTESIAN_POINT('Ctrl Pts',(-0.318312550590783,2.33100218643206,
9.17123450129572));
#26876=CARTESIAN_POINT('Ctrl Pts',(-0.306207738221479,2.34768217444087,
9.17019462939049));
#26877=CARTESIAN_POINT('Ctrl Pts',(-0.292798452407534,2.36339425514184,
9.16915475748527));
#26878=CARTESIAN_POINT('Ctrl Pts',(-0.278271375868845,2.37793871873501,
9.16811488558005));
#26879=CARTESIAN_POINT('Ctrl Pts',(-0.263713205734665,2.39251431313873,
9.16707278794439));
#26880=CARTESIAN_POINT('Ctrl Pts',(-0.248033032995366,2.40591682380063,
9.16603069030873));
#26881=CARTESIAN_POINT('Ctrl Pts',(-0.231451767951575,2.41798580017367,
9.16498859267307));
#26882=CARTESIAN_POINT('Ctrl Pts',(-0.226513517414322,2.42158019595113,
9.16467823401253));
#26883=CARTESIAN_POINT('Ctrl Pts',(-0.221495531294459,2.42505660773875,
9.16436787535198));
#26884=CARTESIAN_POINT('Ctrl Pts',(-0.216404085447837,2.42841157379344,
9.16405751669143));
#26885=CARTESIAN_POINT('Ctrl Pts',(-0.199277837781505,2.43969677279108,
9.16301355404388));
#26886=CARTESIAN_POINT('Ctrl Pts',(-0.181215421465795,2.44967232167622,
9.16196959139633));
#26887=CARTESIAN_POINT('Ctrl Pts',(-0.162443305784822,2.45818579313772,
9.16092562874878));
#26888=CARTESIAN_POINT('Ctrl Pts',(-0.14370572343345,2.46668360315109,9.15988358658301));
#26889=CARTESIAN_POINT('Ctrl Pts',(-0.124261671175083,2.4737243199629,9.15884154441724));
#26890=CARTESIAN_POINT('Ctrl Pts',(-0.104363205590169,2.47920075332064,
9.15779950225147));
#26891=CARTESIAN_POINT('Ctrl Pts',(-0.0844861106446941,2.484671305075,9.15675857922261));
#26892=CARTESIAN_POINT('Ctrl Pts',(-0.0641562693648319,2.4885806864732,
9.15571765619376));
#26893=CARTESIAN_POINT('Ctrl Pts',(-0.0436418731385263,2.49087117687156,
9.15467673316491));
#26894=CARTESIAN_POINT('Ctrl Pts',(-0.0231169412529887,2.4931628436061,
9.15363527554512));
#26895=CARTESIAN_POINT('Ctrl Pts',(-0.00240799451223308,2.4938338606837,
9.15259381792533));
#26896=CARTESIAN_POINT('Ctrl Pts',(0.0182100795606655,2.49287820377618,
9.15155236030553));
#26897=CARTESIAN_POINT('Ctrl Pts',(0.0388344533540614,2.4919222548738,9.15051058447504));
#26898=CARTESIAN_POINT('Ctrl Pts',(0.0593671665102165,2.48933871271772,
9.14946880864454));
#26899=CARTESIAN_POINT('Ctrl Pts',(0.0795378062558533,2.4851735029516,9.14842703281404));
#26900=CARTESIAN_POINT('Ctrl Pts',(0.0997520452970297,2.48099928999005,
9.14738300516144));
#26901=CARTESIAN_POINT('Ctrl Pts',(0.119601941168201,2.47523678925586,9.14633897750885));
#26902=CARTESIAN_POINT('Ctrl Pts',(0.138830896837623,2.46798216272431,9.14529494985625));
#26903=CARTESIAN_POINT('Ctrl Pts',(0.1456319264095,2.46541629641195,9.14492569096038));
#26904=CARTESIAN_POINT('Ctrl Pts',(0.152355471420382,2.46266421054394,9.14455643206452));
#26905=CARTESIAN_POINT('Ctrl Pts',(0.15899088962587,2.45973154854137,9.14418717316865));
#26906=CARTESIAN_POINT('Ctrl Pts',(0.177750434311075,2.45144037499663,9.1431432105211));
#26907=CARTESIAN_POINT('Ctrl Pts',(0.195915566738622,2.44165311682019,9.14209924787354));
#26908=CARTESIAN_POINT('Ctrl Pts',(0.21323553138064,2.43047768178323,9.14105528522599));
#26909=CARTESIAN_POINT('Ctrl Pts',(0.230523634081362,2.41932280516324,9.14001324306022));
#26910=CARTESIAN_POINT('Ctrl Pts',(0.246969011655613,2.40678516511853,9.13897120089445));
#26911=CARTESIAN_POINT('Ctrl Pts',(0.262345093838543,2.39301867131438,9.13792915872867));
#26912=CARTESIAN_POINT('Ctrl Pts',(0.277704662350762,2.37926696250831,9.13688823569982));
#26913=CARTESIAN_POINT('Ctrl Pts',(0.291996650647147,2.3642894867558,9.13584731267097));
#26914=CARTESIAN_POINT('Ctrl Pts',(0.305027349332828,2.34828049895026,9.13480638964211));
#26915=CARTESIAN_POINT('Ctrl Pts',(0.318064740245736,2.33226328934582,9.13376493202232));
#26916=CARTESIAN_POINT('Ctrl Pts',(0.329839070476426,2.31521406981387,9.13272347440253));
#26917=CARTESIAN_POINT('Ctrl Pts',(0.340196473078747,2.29736070962778,9.13168201678273));
#26918=CARTESIAN_POINT('Ctrl Pts',(0.35055704031911,2.27950189446181,9.13064024095223));
#26919=CARTESIAN_POINT('Ctrl Pts',(0.359499480451559,2.26083910356379,9.12959846512173));
#26920=CARTESIAN_POINT('Ctrl Pts',(0.366916029259334,2.2416245652158,9.12855668929124));
#26921=CARTESIAN_POINT('Ctrl Pts',(0.37434860910566,2.22236849420713,9.12751266163864));
#26922=CARTESIAN_POINT('Ctrl Pts',(0.380248502614248,2.20255900058928,9.12646863398604));
#26923=CARTESIAN_POINT('Ctrl Pts',(0.384557663885936,2.18246388995549,9.12542460633344));
#26924=CARTESIAN_POINT('Ctrl Pts',(0.386081757744297,2.17535651272613,9.12505534743758));
#26925=CARTESIAN_POINT('Ctrl Pts',(0.387407331073193,2.16821348189271,9.12468608854171));
#26926=CARTESIAN_POINT('Ctrl Pts',(0.388533368122952,2.16104680053069,9.12431682964585));
#26927=CARTESIAN_POINT('Ctrl Pts',(0.391716881459736,2.14078527742953,9.1232728669983));
#26928=CARTESIAN_POINT('Ctrl Pts',(0.393320693956306,2.12021368915352,9.12222890435075));
#26929=CARTESIAN_POINT('Ctrl Pts',(0.393299797900577,2.09960128786642,9.12118494170319));
#26930=CARTESIAN_POINT('Ctrl Pts',(0.393278940285393,2.0790268053126,9.12014289953742));
#26931=CARTESIAN_POINT('Ctrl Pts',(0.391639248087145,2.05841238630684,9.11910085737166));
#26932=CARTESIAN_POINT('Ctrl Pts',(0.388387484729823,2.03803184926721,9.11805881520589));
#26933=CARTESIAN_POINT('Ctrl Pts',(0.385139213715263,2.0176732006042,9.11701789217703));
#26934=CARTESIAN_POINT('Ctrl Pts',(0.380282395444754,1.9975486627047,9.11597696914818));
#26935=CARTESIAN_POINT('Ctrl Pts',(0.37387550451514,1.97792626357996,9.11493604611933));
#26936=CARTESIAN_POINT('Ctrl Pts',(0.367465323173333,1.95829378690246,9.11389458849954));
#26937=CARTESIAN_POINT('Ctrl Pts',(0.359503691837624,1.93916466863988,9.11285313087975));
#26938=CARTESIAN_POINT('Ctrl Pts',(0.350098916114789,1.92079163263048,9.11181167325996));
#26939=CARTESIAN_POINT('Ctrl Pts',(0.340691266822953,1.90241298285757,9.11076989742946));
#26940=CARTESIAN_POINT('Ctrl Pts',(0.329839962513473,1.884791513157,9.10972812159896));
#26941=CARTESIAN_POINT('Ctrl Pts',(0.317698746524207,1.86815436933824,9.10868634576847));
#26942=CARTESIAN_POINT('Ctrl Pts',(0.305531287021062,1.85148126395558,9.10764231811587));
#26943=CARTESIAN_POINT('Ctrl Pts',(0.292068829070921,1.83579729102943,9.10659829046327));
#26944=CARTESIAN_POINT('Ctrl Pts',(0.277505127117448,1.82129622459764,9.10555426281068));
#26945=CARTESIAN_POINT('Ctrl Pts',(0.272354136633885,1.81616738747709,9.10518500391481));
#26946=CARTESIAN_POINT('Ctrl Pts',(0.267065705212036,1.81118617003201,9.10481574501894));
#26947=CARTESIAN_POINT('Ctrl Pts',(0.261649375409,1.80635992380453,9.10444648612307));
#26948=CARTESIAN_POINT('Ctrl Pts',(0.246336417307073,1.79271524023496,9.10340252347552));
#26949=CARTESIAN_POINT('Ctrl Pts',(0.229907630246419,1.78023095353374,9.10235856082796));
#26950=CARTESIAN_POINT('Ctrl Pts',(0.21256504277933,1.76909065805236,9.10131459818041));
#26951=CARTESIAN_POINT('Ctrl Pts',(0.195254358870659,1.75797085634495,9.10027255601464));
#26952=CARTESIAN_POINT('Ctrl Pts',(0.177033791267862,1.74819058141618,9.09923051384887));
#26953=CARTESIAN_POINT('Ctrl Pts',(0.158137232563017,1.73989236931535,9.0981884716831));
#26954=CARTESIAN_POINT('Ctrl Pts',(0.139260968465368,1.73160306936396,9.09714754865424));
#26955=CARTESIAN_POINT('Ctrl Pts',(0.119710813195054,1.72479299313183,9.09610662562539));
#26956=CARTESIAN_POINT('Ctrl Pts',(0.0997437828586238,1.71955806253641,
9.09506570259653));
#26957=CARTESIAN_POINT('Ctrl Pts',(0.0797664979758132,1.71432044341707,
9.09402424497674));
#26958=CARTESIAN_POINT('Ctrl Pts',(0.0593726179459746,1.71065978823548,
9.09298278735695));
#26959=CARTESIAN_POINT('Ctrl Pts',(0.0388332652790696,1.70862183567837,
9.09194132973715));
#26960=CARTESIAN_POINT('Ctrl Pts',(0.0182876369444851,1.70658326043792,
9.09089955390665));
#26961=CARTESIAN_POINT('Ctrl Pts',(-0.00240281737467288,1.70616841143858,
9.08985777807616));
#26962=CARTESIAN_POINT('Ctrl Pts',(-0.0229638853681445,1.70737097666016,
9.08881600224566));
#26963=CARTESIAN_POINT('Ctrl Pts',(-0.0435693965766733,1.70857614125375,
9.08777197459306));
#26964=CARTESIAN_POINT('Ctrl Pts',(-0.0640442335644598,1.71140559899892,
9.08672794694046));
#26965=CARTESIAN_POINT('Ctrl Pts',(-0.084120584869788,1.71580133107835,
9.08568391928786));
#26966=CARTESIAN_POINT('Ctrl Pts',(-0.0912213271705936,1.71735604389667,
9.085314660392));
#26967=CARTESIAN_POINT('Ctrl Pts',(-0.098272347468519,1.71910622871434,
9.08494540149614));
#26968=CARTESIAN_POINT('Ctrl Pts',(-0.10526229889673,1.7210478415011,9.08457614260027));
#26969=CARTESIAN_POINT('Ctrl Pts',(-0.125024174049869,1.72653713708229,
9.08353217995272));
#26970=CARTESIAN_POINT('Ctrl Pts',(-0.144414385117009,1.73359278542209,
9.08248821730516));
#26971=CARTESIAN_POINT('Ctrl Pts',(-0.163169200974503,1.74214430023634,
9.08144425465761));
#26972=CARTESIAN_POINT('Ctrl Pts',(-0.181889515327279,1.7506800836176,9.08040221249184));
#26973=CARTESIAN_POINT('Ctrl Pts',(-0.199976068065358,1.76070602354879,
9.07936017032607));
#26974=CARTESIAN_POINT('Ctrl Pts',(-0.217182402040207,1.77210261628972,
9.0783181281603));
#26975=CARTESIAN_POINT('Ctrl Pts',(-0.234370256682658,1.78348696926908,
9.07727720513144));
#26976=CARTESIAN_POINT('Ctrl Pts',(-0.25067914300557,1.79623867253913,9.07623628210259));
#26977=CARTESIAN_POINT('Ctrl Pts',(-0.265889280680861,1.8101935466229,9.07519535907374));
#26978=CARTESIAN_POINT('Ctrl Pts',(-0.281107229886447,1.82415558756629,
9.07415390145395));
#26979=CARTESIAN_POINT('Ctrl Pts',(-0.295224750059093,1.83932154824162,
9.07311244383415));
#26980=CARTESIAN_POINT('Ctrl Pts',(-0.308056619778545,1.8554882231658,9.07207098621436));
#26981=CARTESIAN_POINT('Ctrl Pts',(-0.320892410193626,1.87165983771399,
9.07102921038386));
#26982=CARTESIAN_POINT('Ctrl Pts',(-0.332441339435636,1.88883217689623,
9.06998743455336));
#26983=CARTESIAN_POINT('Ctrl Pts',(-0.342560278685943,1.90677126128184,
9.06894565872286));
#26984=CARTESIAN_POINT('Ctrl Pts',(-0.352701090253059,1.92474912140544,
9.06790163107027));
#26985=CARTESIAN_POINT('Ctrl Pts',(-0.361405430739534,1.94349636753665,
9.06685760341767));
#26986=CARTESIAN_POINT('Ctrl Pts',(-0.368577112222484,1.96275641236934,
9.06581357576507));
#26987=CARTESIAN_POINT('Ctrl Pts',(-0.37111364195833,1.96956843777063,9.06544431686921));
#26988=CARTESIAN_POINT('Ctrl Pts',(-0.373458899918739,1.97644446854687,
9.06507505797335));
#26989=CARTESIAN_POINT('Ctrl Pts',(-0.375610144132728,1.98337277494259,
9.06470579907749));
#26990=CARTESIAN_POINT('Ctrl Pts',(-0.382959707516277,2.00704281048059,
9.0634442539482));
#26991=CARTESIAN_POINT('Ctrl Pts',(-0.388076627771857,2.03143715382748,
9.06218270881891));
#26992=CARTESIAN_POINT('Ctrl Pts',(-0.390850208804052,2.05617073719729,
9.06092116368962));
#26993=CARTESIAN_POINT('Ctrl Pts',(-0.392466008626093,2.07057973377733,
9.06018622774517));
#26994=CARTESIAN_POINT('Ctrl Pts',(-0.393287360126491,2.08510347310958,
9.05945129180072));
#26995=CARTESIAN_POINT('Ctrl Pts',(-0.393299855154148,2.09966245633422,
9.05871635585627));
#26996=CARTESIAN_POINT('',(-0.393095239940488,2.10019047587301,8.93371634952743));
#26997=CARTESIAN_POINT('Ctrl Pts',(-0.393040168128258,2.09966275151986,
9.0587163522035));
#26998=CARTESIAN_POINT('Ctrl Pts',(-0.392294723781914,2.19126251015094,
9.0540893866539));
#26999=CARTESIAN_POINT('Ctrl Pts',(-0.314706016092101,2.41512451888509,
9.04283897326335));
#27000=CARTESIAN_POINT('Ctrl Pts',(0.0583154564568577,2.56138306321075,
9.02496511203192));
#27001=CARTESIAN_POINT('Ctrl Pts',(0.419506350600682,2.30072230888762,9.0050947685091));
#27002=CARTESIAN_POINT('Ctrl Pts',(0.395857278700936,1.85592616203501,8.98522442498634));
#27003=CARTESIAN_POINT('Ctrl Pts',(0.00906304469525043,1.63503453386264,
8.96535408146352));
#27004=CARTESIAN_POINT('Ctrl Pts',(-0.332338020341264,1.81273119149951,
8.94818472386927));
#27005=CARTESIAN_POINT('Ctrl Pts',(-0.392402917414063,2.02238938101501,
8.93763881411591));
#27006=CARTESIAN_POINT('Ctrl Pts',(-0.392742359999847,2.10019025177715,
8.93371635220349));
#27007=CARTESIAN_POINT('',(-0.393444746249714,2.10025436408896,8.8087163522035));
#27008=CARTESIAN_POINT('Ctrl Pts',(-0.393299953813117,2.10019060587623,
8.93371634797498));
#27009=CARTESIAN_POINT('Ctrl Pts',(-0.393288928936479,2.12293955548056,
8.9325710447093));
#27010=CARTESIAN_POINT('Ctrl Pts',(-0.391299996201274,2.14562110664529,
8.93142574144361));
#27011=CARTESIAN_POINT('Ctrl Pts',(-0.387392643545173,2.16791045373933,
8.93028043817793));
#27012=CARTESIAN_POINT('Ctrl Pts',(-0.383457008456061,2.19036113691475,
8.92912684490985));
#27013=CARTESIAN_POINT('Ctrl Pts',(-0.377575283507818,2.21241347444076,
8.92797325164176));
#27014=CARTESIAN_POINT('Ctrl Pts',(-0.369857635818388,2.23375432414256,
8.92681965837368));
#27015=CARTESIAN_POINT('Ctrl Pts',(-0.3671676293004,2.24119273376002,8.92641757038844));
#27016=CARTESIAN_POINT('Ctrl Pts',(-0.364255000440692,2.24854490221534,
8.9260154824032));
#27017=CARTESIAN_POINT('Ctrl Pts',(-0.361125734524206,2.25579824730835,
8.92561339441796));
#27018=CARTESIAN_POINT('Ctrl Pts',(-0.353001053233094,2.27463049702693,
8.9245694317704));
#27019=CARTESIAN_POINT('Ctrl Pts',(-0.343375080858931,2.29288160972106,
8.92352546912285));
#27020=CARTESIAN_POINT('Ctrl Pts',(-0.332353499814773,2.31029988388221,
8.9224815064753));
#27021=CARTESIAN_POINT('Ctrl Pts',(-0.321352194156588,2.32768611525112,
8.92143946430953));
#27022=CARTESIAN_POINT('Ctrl Pts',(-0.308960714688259,2.34424190269951,
8.92039742214376));
#27023=CARTESIAN_POINT('Ctrl Pts',(-0.295330958138818,2.35973932156069,
8.91935537997799));
#27024=CARTESIAN_POINT('Ctrl Pts',(-0.281715839733789,2.37522009643748,
8.91831445694914));
#27025=CARTESIAN_POINT('Ctrl Pts',(-0.266865546132116,2.3896441904931,8.91727353392028));
#27026=CARTESIAN_POINT('Ctrl Pts',(-0.250972608780928,2.40281618127454,
8.91623261089143));
#27027=CARTESIAN_POINT('Ctrl Pts',(-0.235071509231343,2.41599493684714,
8.91519115327164));
#27028=CARTESIAN_POINT('Ctrl Pts',(-0.21812725238961,2.42791982255356,8.91414969565184));
#27029=CARTESIAN_POINT('Ctrl Pts',(-0.200366335677794,2.43843495907937,
8.91310823803205));
#27030=CARTESIAN_POINT('Ctrl Pts',(-0.182599992231609,2.44895330843781,
8.91206646220155));
#27031=CARTESIAN_POINT('Ctrl Pts',(-0.164017143206278,2.4580607077223,8.91102468637106));
#27032=CARTESIAN_POINT('Ctrl Pts',(-0.144869052442489,2.46564716277364,
8.90998291054056));
#27033=CARTESIAN_POINT('Ctrl Pts',(-0.125679572645992,2.47325001611974,
8.90893888288796));
#27034=CARTESIAN_POINT('Ctrl Pts',(-0.105923115829145,2.47932514532429,
8.90789485523536));
#27035=CARTESIAN_POINT('Ctrl Pts',(-0.0858669629241464,2.4838121346156,
8.90685082758277));
#27036=CARTESIAN_POINT('Ctrl Pts',(-0.0787733645327732,2.48539912391358,
8.9064815686869));
#27037=CARTESIAN_POINT('Ctrl Pts',(-0.0716423554947472,2.48678791628016,
8.90611230979103));
#27038=CARTESIAN_POINT('Ctrl Pts',(-0.0644859294174,2.4879773896855,8.90574305089517));
#27039=CARTESIAN_POINT('Ctrl Pts',(-0.0442533998876345,2.49134024923835,
8.90469908824761));
#27040=CARTESIAN_POINT('Ctrl Pts',(-0.0236968247830544,2.49312621639706,
8.90365512560006));
#27041=CARTESIAN_POINT('Ctrl Pts',(-0.00308504703835625,2.49328790025218,
8.90261116295251));
#27042=CARTESIAN_POINT('Ctrl Pts',(0.0174888131201405,2.49344928667243,
8.90156912078674));
#27043=CARTESIAN_POINT('Ctrl Pts',(0.03811694736396,2.49199225576357,8.90052707862097));
#27044=CARTESIAN_POINT('Ctrl Pts',(0.0585254881084704,2.48892114527455,
8.89948503645519));
#27045=CARTESIAN_POINT('Ctrl Pts',(0.0789121104008293,2.48585333310995,
8.89844411342634));
#27046=CARTESIAN_POINT('Ctrl Pts',(0.0990788791916744,2.48117496310345,
8.89740319039749));
#27047=CARTESIAN_POINT('Ctrl Pts',(0.118757259032441,2.47494213343808,8.89636226736863));
#27048=CARTESIAN_POINT('Ctrl Pts',(0.13844574517621,2.46870610275385,8.89532080974884));
#27049=CARTESIAN_POINT('Ctrl Pts',(0.157644634977628,2.46091422432674,8.89427935212905));
#27050=CARTESIAN_POINT('Ctrl Pts',(0.176100255171075,2.45167256095505,8.89323789450926));
#27051=CARTESIAN_POINT('Ctrl Pts',(0.194561514361092,2.44242807385229,8.89219611867876));
#27052=CARTESIAN_POINT('Ctrl Pts',(0.212278410690057,2.43173328147029,8.89115434284826));
#27053=CARTESIAN_POINT('Ctrl Pts',(0.229022445442515,2.41973990911916,8.89011256701776));
#27054=CARTESIAN_POINT('Ctrl Pts',(0.24580267280606,2.40772061282153,8.88906853936516));
#27055=CARTESIAN_POINT('Ctrl Pts',(0.261605277264181,2.39439760741178,8.88802451171256));
#27056=CARTESIAN_POINT('Ctrl Pts',(0.276234776156258,2.37996292333433,8.88698048405997));
#27057=CARTESIAN_POINT('Ctrl Pts',(0.281409038154505,2.37485756478243,8.8866112251641));
#27058=CARTESIAN_POINT('Ctrl Pts',(0.286436903683232,2.36961346310885,8.88624196626824));
#27059=CARTESIAN_POINT('Ctrl Pts',(0.291310936963311,2.36424009537835,8.88587270737237));
#27060=CARTESIAN_POINT('Ctrl Pts',(0.305090723298343,2.34904859893771,8.88482874472482));
#27061=CARTESIAN_POINT('Ctrl Pts',(0.317720041999881,2.33273103883036,8.88378478207726));
#27062=CARTESIAN_POINT('Ctrl Pts',(0.329013516404515,2.31548780945366,8.88274081942971));
#27063=CARTESIAN_POINT('Ctrl Pts',(0.34028621524604,2.29827630085546,8.88169877726394));
#27064=CARTESIAN_POINT('Ctrl Pts',(0.350227499363535,2.28014307909137,8.88065673509817));
#27065=CARTESIAN_POINT('Ctrl Pts',(0.35869276654196,2.26132076503189,8.8796146929324));
#27066=CARTESIAN_POINT('Ctrl Pts',(0.36714894215642,2.24251866584202,8.87857376990355));
#27067=CARTESIAN_POINT('Ctrl Pts',(0.374131921228497,2.22302959935182,8.8775328468747));
#27068=CARTESIAN_POINT('Ctrl Pts',(0.37954350902445,2.20310972193449,8.87649192384585));
#27069=CARTESIAN_POINT('Ctrl Pts',(0.384957876070851,2.18317961418729,8.87545046622605));
#27070=CARTESIAN_POINT('Ctrl Pts',(0.388799031131988,2.16281895931506,8.87440900860626));
#27071=CARTESIAN_POINT('Ctrl Pts',(0.391018835785393,2.14229846405055,8.87336755098647));
#27072=CARTESIAN_POINT('Ctrl Pts',(0.393239318685896,2.12177169888011,8.87232577515597));
#27073=CARTESIAN_POINT('Ctrl Pts',(0.393837421874313,2.1010857308776,8.87128399932548));
#27074=CARTESIAN_POINT('Ctrl Pts',(0.392817028224559,2.08051481750595,8.87024222349498));
#27075=CARTESIAN_POINT('Ctrl Pts',(0.391794428970775,2.05989943963825,8.86919819584238));
#27076=CARTESIAN_POINT('Ctrl Pts',(0.389146442810179,2.03940034331423,8.86815416818979));
#27077=CARTESIAN_POINT('Ctrl Pts',(0.384928714082289,2.0192858434043,8.86711014053719));
#27078=CARTESIAN_POINT('Ctrl Pts',(0.383436958716179,2.01217160844204,8.86674088164133));
#27079=CARTESIAN_POINT('Ctrl Pts',(0.38174929859508,2.00510536209381,8.86637162274546));
#27080=CARTESIAN_POINT('Ctrl Pts',(0.379869677083126,1.9980984866022,8.86600236384959));
#27081=CARTESIAN_POINT('Ctrl Pts',(0.374555642209548,1.97828876401688,8.86495840120204));
#27082=CARTESIAN_POINT('Ctrl Pts',(0.367672023925872,1.95883681660674,8.86391443855449));
#27083=CARTESIAN_POINT('Ctrl Pts',(0.359286969691899,1.94000698949763,8.86287047590693));
#27084=CARTESIAN_POINT('Ctrl Pts',(0.350917340668729,1.92121180188451,8.86182843374116));
#27085=CARTESIAN_POINT('Ctrl Pts',(0.341051999865725,1.90303715161852,8.86078639157539));
#27086=CARTESIAN_POINT('Ctrl Pts',(0.329808263283925,1.88573054471147,8.85974434940962));
#27087=CARTESIAN_POINT('Ctrl Pts',(0.31857660229858,1.86844252482837,8.85870342638077));
#27088=CARTESIAN_POINT('Ctrl Pts',(0.30596985900002,1.85202132716239,8.85766250335192));
#27089=CARTESIAN_POINT('Ctrl Pts',(0.292150259669528,1.83668817767706,8.85662158032306));
#27090=CARTESIAN_POINT('Ctrl Pts',(0.278323562953001,1.82134715348578,8.85558012270327));
#27091=CARTESIAN_POINT('Ctrl Pts',(0.263283246431304,1.80709585116084,8.85453866508348));
#27092=CARTESIAN_POINT('Ctrl Pts',(0.247230866974281,1.79412128479552,8.85349720746368));
#27093=CARTESIAN_POINT('Ctrl Pts',(0.231173582815509,1.78114275413453,8.85245543163319));
#27094=CARTESIAN_POINT('Ctrl Pts',(0.214104214612402,1.76944217001355,8.85141365580269));
#27095=CARTESIAN_POINT('Ctrl Pts',(0.196255464820033,1.7591647281629,8.85037187997219));
#27096=CARTESIAN_POINT('Ctrl Pts',(0.178368134549949,1.74886507138846,8.84932785231959));
#27097=CARTESIAN_POINT('Ctrl Pts',(0.159698724582217,1.73999501432749,8.84828382466699));
#27098=CARTESIAN_POINT('Ctrl Pts',(0.140502960150279,1.73265301391054,8.8472397970144));
#27099=CARTESIAN_POINT('Ctrl Pts',(0.133713669884053,1.7300562446002,8.84687053811853));
#27100=CARTESIAN_POINT('Ctrl Pts',(0.126858682520048,1.72765017261927,8.84650127922266));
#27101=CARTESIAN_POINT('Ctrl Pts',(0.119949703065909,1.72543764373018,8.8461320203268));
#27102=CARTESIAN_POINT('Ctrl Pts',(0.100416750539694,1.71918241862199,8.84508805767924));
#27103=CARTESIAN_POINT('Ctrl Pts',(0.0803349779260562,1.71444059751436,
8.84404409503169));
#27104=CARTESIAN_POINT('Ctrl Pts',(0.0599635407910791,1.71129797559596,
8.84300013238414));
#27105=CARTESIAN_POINT('Ctrl Pts',(0.0396295791098609,1.70816113486923,
8.84195809021837));
#27106=CARTESIAN_POINT('Ctrl Pts',(0.0190077205282317,1.70661782346517,
8.8409160480526));
#27107=CARTESIAN_POINT('Ctrl Pts',(-0.00163042219651427,1.70670337946601,
8.83987400588683));
#27108=CARTESIAN_POINT('Ctrl Pts',(-0.022246399880189,1.70678884358104,
8.83883308285797));
#27109=CARTESIAN_POINT('Ctrl Pts',(-0.0428778948260887,1.70849972805363,
8.83779215982912));
#27110=CARTESIAN_POINT('Ctrl Pts',(-0.0632510802658689,1.71181938373329,
8.83675123680026));
#27111=CARTESIAN_POINT('Ctrl Pts',(-0.0836347288427016,1.71514074430159,
8.83570977918047));
#27112=CARTESIAN_POINT('Ctrl Pts',(-0.103759074092783,1.72007242426745,
8.83466832156068));
#27113=CARTESIAN_POINT('Ctrl Pts',(-0.12335776484255,1.72654618511381,8.83362686394089));
#27114=CARTESIAN_POINT('Ctrl Pts',(-0.142962443846772,1.73302192397633,
8.83258508811039));
#27115=CARTESIAN_POINT('Ctrl Pts',(-0.162040461899702,1.74104041677721,
8.83154331227989));
#27116=CARTESIAN_POINT('Ctrl Pts',(-0.180343769788057,1.75048460019817,
8.83050153644939));
#27117=CARTESIAN_POINT('Ctrl Pts',(-0.198686640691771,1.75994919743591,
8.8294575087968));
#27118=CARTESIAN_POINT('Ctrl Pts',(-0.216250832431912,1.77084524944222,
8.8284134811442));
#27119=CARTESIAN_POINT('Ctrl Pts',(-0.232815131968949,1.78301103437772,
8.8273694534916));
#27120=CARTESIAN_POINT('Ctrl Pts',(-0.238673707594395,1.78731391304327,
8.82700019459574));
#27121=CARTESIAN_POINT('Ctrl Pts',(-0.244407504517051,1.79177525891498,
8.82663093569987));
#27122=CARTESIAN_POINT('Ctrl Pts',(-0.250007793836785,1.79638677067548,
8.82626167680401));
#27123=CARTESIAN_POINT('Ctrl Pts',(-0.265626250513275,1.80924765919971,
8.82523186321079));
#27124=CARTESIAN_POINT('Ctrl Pts',(-0.280302271003942,1.82336043277438,
8.82420204961756));
#27125=CARTESIAN_POINT('Ctrl Pts',(-0.293826368015407,1.8385598434462,8.82317223602434));
#27126=CARTESIAN_POINT('Ctrl Pts',(-0.307325503409736,1.85373120035077,
8.82214432317263));
#27127=CARTESIAN_POINT('Ctrl Pts',(-0.319676387843176,1.86998469896286,
8.82111641032092));
#27128=CARTESIAN_POINT('Ctrl Pts',(-0.330704857821977,1.88711696400853,
8.82008849746921));
#27129=CARTESIAN_POINT('Ctrl Pts',(-0.341729443646336,1.90424319518336,
8.81906094664163));
#27130=CARTESIAN_POINT('Ctrl Pts',(-0.35143208895433,1.92224697056919,8.81803339581405));
#27131=CARTESIAN_POINT('Ctrl Pts',(-0.359680771461609,1.94089427213082,
8.81700584498647));
#27132=CARTESIAN_POINT('Ctrl Pts',(-0.367927090802008,1.9595362314229,8.81597858854216));
#27133=CARTESIAN_POINT('Ctrl Pts',(-0.374719976175961,1.97882065423493,
8.81495133209784));
#27134=CARTESIAN_POINT('Ctrl Pts',(-0.379975191608948,1.99849264183448,
8.81392407565353));
#27135=CARTESIAN_POINT('Ctrl Pts',(-0.385240027035102,2.01820064021013,
8.81289493875349));
#27136=CARTESIAN_POINT('Ctrl Pts',(-0.388961406089882,2.03829687848715,
8.81186580185344));
#27137=CARTESIAN_POINT('Ctrl Pts',(-0.391105947897405,2.05851473129806,
8.8108366649534));
#27138=CARTESIAN_POINT('Ctrl Pts',(-0.392578735219475,2.07239956077302,
8.81012989403676));
#27139=CARTESIAN_POINT('Ctrl Pts',(-0.393308912464174,2.0863415328013,8.80942312312013));
#27140=CARTESIAN_POINT('Ctrl Pts',(-0.393299917806418,2.10025427045661,
8.8087163522035));
#27141=CARTESIAN_POINT('',(-0.393343477685089,2.09967036236989,8.6837163522035));
#27142=CARTESIAN_POINT('Ctrl Pts',(-0.393737740759854,2.10025455351144,
8.8087163522035));
#27143=CARTESIAN_POINT('Ctrl Pts',(-0.393852405531071,2.11552756370832,
8.80794134589607));
#27144=CARTESIAN_POINT('Ctrl Pts',(-0.386105851649887,2.26121113565208,
8.80054289174776));
#27145=CARTESIAN_POINT('Ctrl Pts',(-0.204430308564429,2.51771194909898,
8.78652098975839));
#27146=CARTESIAN_POINT('Ctrl Pts',(0.240557865830071,2.49800368926257,8.76665064623566));
#27147=CARTESIAN_POINT('Ctrl Pts',(0.464866947321644,2.11318122783806,8.74678030271284));
#27148=CARTESIAN_POINT('Ctrl Pts',(0.26272389056588,1.71626678433389,8.72690995919007));
#27149=CARTESIAN_POINT('Ctrl Pts',(-0.180432569156138,1.67137532564354,
8.70703961566727));
#27150=CARTESIAN_POINT('Ctrl Pts',(-0.381603726014139,1.92375997419914,
8.69264174667176));
#27151=CARTESIAN_POINT('Ctrl Pts',(-0.393739127627545,2.07695764050864,
8.68486732551716));
#27152=CARTESIAN_POINT('Ctrl Pts',(-0.393535259525408,2.09967020164901,
8.6837163522035));
#27153=CARTESIAN_POINT('',(-0.39305712210104,2.09992355731599,8.55871635455519));
#27154=CARTESIAN_POINT('Ctrl Pts',(-0.393299861890554,2.09967039892168,
8.6837163522035));
#27155=CARTESIAN_POINT('Ctrl Pts',(-0.393316836847012,2.1199259395421,8.68268926714426));
#27156=CARTESIAN_POINT('Ctrl Pts',(-0.391764737712971,2.14023690090369,
8.68166218208501));
#27157=CARTESIAN_POINT('Ctrl Pts',(-0.388644317798756,2.16033642550516,
8.68063509702577));
#27158=CARTESIAN_POINT('Ctrl Pts',(-0.38552796621335,2.18040974482746,8.67960935105544));
#27159=CARTESIAN_POINT('Ctrl Pts',(-0.380847424894488,2.20027142239561,
8.67858360508512));
#27160=CARTESIAN_POINT('Ctrl Pts',(-0.374655259657195,2.2196592094709,8.6775578591148));
#27161=CARTESIAN_POINT('Ctrl Pts',(-0.368461202685,2.23905291960412,8.67653179977437));
#27162=CARTESIAN_POINT('Ctrl Pts',(-0.360754805832814,2.2579717188872,8.67550574043395));
#27163=CARTESIAN_POINT('Ctrl Pts',(-0.351638689139405,2.27616788101218,
8.67447968109352));
#27164=CARTESIAN_POINT('Ctrl Pts',(-0.342520791281123,2.29436759841907,
8.6734534212751));
#27165=CARTESIAN_POINT('Ctrl Pts',(-0.331992997204494,2.31184373491231,
8.67242716145667));
#27166=CARTESIAN_POINT('Ctrl Pts',(-0.320203617888944,2.32837366987206,
8.67140090163825));
#27167=CARTESIAN_POINT('Ctrl Pts',(-0.308389629667196,2.34493810907567,
8.67037249962633));
#27168=CARTESIAN_POINT('Ctrl Pts',(-0.295309292191493,2.36055182540162,
8.66934409761441));
#27169=CARTESIAN_POINT('Ctrl Pts',(-0.281151028374483,2.37502543381289,
8.6683156956025));
#27170=CARTESIAN_POINT('Ctrl Pts',(-0.276485001215232,2.37979538659893,
8.66797677327556));
#27171=CARTESIAN_POINT('Ctrl Pts',(-0.271702180537641,2.38444182541632,
8.66763785094863));
#27172=CARTESIAN_POINT('Ctrl Pts',(-0.266810082825443,2.38895894120563,
8.66729892862169));
#27173=CARTESIAN_POINT('Ctrl Pts',(-0.251741239984959,2.40287274913135,
8.66625496597414));
#27174=CARTESIAN_POINT('Ctrl Pts',(-0.235536187121755,2.41564610892519,
8.66521100332659));
#27175=CARTESIAN_POINT('Ctrl Pts',(-0.218393668755151,2.42709187615663,
8.66416704067903));
#27176=CARTESIAN_POINT('Ctrl Pts',(-0.201282685898296,2.4385165876659,8.66312499851326));
#27177=CARTESIAN_POINT('Ctrl Pts',(-0.183238232722274,2.44861810096978,
8.6620829563475));
#27178=CARTESIAN_POINT('Ctrl Pts',(-0.164491640124325,2.4572497590331,8.66104091418173));
#27179=CARTESIAN_POINT('Ctrl Pts',(-0.145765181072325,2.46587214683127,
8.65999999115287));
#27180=CARTESIAN_POINT('Ctrl Pts',(-0.126338732492407,2.47302748085229,
8.65895906812402));
#27181=CARTESIAN_POINT('Ctrl Pts',(-0.106467570926185,2.47861530125059,
8.65791814509517));
#27182=CARTESIAN_POINT('Ctrl Pts',(-0.0865862040492851,2.48420599140782,
8.65687668747538));
#27183=CARTESIAN_POINT('Ctrl Pts',(-0.066260371850469,2.48822734496792,
8.65583522985559));
#27184=CARTESIAN_POINT('Ctrl Pts',(-0.0457603440453731,2.49062882754969,
8.6547937722358));
#27185=CARTESIAN_POINT('Ctrl Pts',(-0.0252540525880575,2.4930310438891,
8.6537519964053));
#27186=CARTESIAN_POINT('Ctrl Pts',(-0.00457419394235422,2.49381235433887,
8.6527102205748));
#27187=CARTESIAN_POINT('Ctrl Pts',(0.0160049507945768,2.49297421232196,
8.6516684447443));
#27188=CARTESIAN_POINT('Ctrl Pts',(0.0366285778198562,2.49213425864206,
8.6506244170917));
#27189=CARTESIAN_POINT('Ctrl Pts',(0.0571503251020473,2.48966795182948,
8.64958038943911));
#27190=CARTESIAN_POINT('Ctrl Pts',(0.077301395414331,2.48562855738002,8.64853636178651));
#27191=CARTESIAN_POINT('Ctrl Pts',(0.0844285648485482,2.48419987651063,
8.64816710289064));
#27192=CARTESIAN_POINT('Ctrl Pts',(0.0915094828228455,2.48257487350149,
8.64779784399478));
#27193=CARTESIAN_POINT('Ctrl Pts',(0.0985327326118787,2.48075739074119,
8.64742858509891));
#27194=CARTESIAN_POINT('Ctrl Pts',(0.118388748340246,2.4756190335193,8.64638462245135));
#27195=CARTESIAN_POINT('Ctrl Pts',(0.137900905875624,2.4689079853868,8.6453406598038));
#27196=CARTESIAN_POINT('Ctrl Pts',(0.156804266830728,2.4606900496322,8.64429669715625));
#27197=CARTESIAN_POINT('Ctrl Pts',(0.175672853016393,2.45248723165595,8.64325465499048));
#27198=CARTESIAN_POINT('Ctrl Pts',(0.193934174810419,2.44278326402489,8.64221261282471));
#27199=CARTESIAN_POINT('Ctrl Pts',(0.211339696757282,2.43169326579619,8.64117057065894));
#27200=CARTESIAN_POINT('Ctrl Pts',(0.228726525447013,2.42061517805136,8.64012964763008));
#27201=CARTESIAN_POINT('Ctrl Pts',(0.245258746033701,2.40815438386103,8.63908872460123));
#27202=CARTESIAN_POINT('Ctrl Pts',(0.260713704275977,2.39447114358235,8.63804780157238));
#27203=CARTESIAN_POINT('Ctrl Pts',(0.276176599782002,2.3807808759481,8.63700634395259));
#27204=CARTESIAN_POINT('Ctrl Pts',(0.290560566088892,2.36586738365716,8.63596488633279));
#27205=CARTESIAN_POINT('Ctrl Pts',(0.303676811103612,2.34993055915182,8.634923428713));
#27206=CARTESIAN_POINT('Ctrl Pts',(0.31679706370301,2.3339888652518,8.6338816528825));
#27207=CARTESIAN_POINT('Ctrl Pts',(0.328648384664318,2.3170238073062,8.632839877052));
#27208=CARTESIAN_POINT('Ctrl Pts',(0.339083522737738,2.29926679253645,8.6317981012215));
#27209=CARTESIAN_POINT('Ctrl Pts',(0.349541216598902,2.28147139557633,8.63075407356891));
#27210=CARTESIAN_POINT('Ctrl Pts',(0.358576294281472,2.26288128659123,8.62971004591631));
#27211=CARTESIAN_POINT('Ctrl Pts',(0.366088037572277,2.24375130867745,8.62866601826371));
#27212=CARTESIAN_POINT('Ctrl Pts',(0.368744842712165,2.23698528624035,8.62829675936785));
#27213=CARTESIAN_POINT('Ctrl Pts',(0.371211539930955,2.23015188013729,8.62792750047198));
#27214=CARTESIAN_POINT('Ctrl Pts',(0.37348517989806,2.22326276970973,8.62755824157611));
#27215=CARTESIAN_POINT('Ctrl Pts',(0.379913177235985,2.20378599056715,8.62651427892856));
#27216=CARTESIAN_POINT('Ctrl Pts',(0.384832691245211,2.18374700754316,8.625470316281));
#27217=CARTESIAN_POINT('Ctrl Pts',(0.388155634572719,2.16340420608642,8.62442635363345));
#27218=CARTESIAN_POINT('Ctrl Pts',(0.391472464987909,2.14309882740503,8.62338431146768));
#27219=CARTESIAN_POINT('Ctrl Pts',(0.393198378708398,2.12249144806461,8.62234226930191));
#27220=CARTESIAN_POINT('Ctrl Pts',(0.393295633165775,2.10185335715177,8.62130022713614));
#27221=CARTESIAN_POINT('Ctrl Pts',(0.393392783173393,2.08123743122437,8.62025930410728));
#27222=CARTESIAN_POINT('Ctrl Pts',(0.39186471403716,2.06059159110837,8.61921838107843));
#27223=CARTESIAN_POINT('Ctrl Pts',(0.388725648770774,2.04018980030345,8.61817745804958));
#27224=CARTESIAN_POINT('Ctrl Pts',(0.385584971362279,2.01977753167049,8.61713600042979));
#27225=CARTESIAN_POINT('Ctrl Pts',(0.380831740890856,1.9996102924168,8.61609454280999));
#27226=CARTESIAN_POINT('Ctrl Pts',(0.374531833929707,1.97995502770524,8.6150530851902));
#27227=CARTESIAN_POINT('Ctrl Pts',(0.368230002072328,1.96029375745341,8.6140113093597));
#27228=CARTESIAN_POINT('Ctrl Pts',(0.360380811778884,1.94114546219344,8.6129695335292));
#27229=CARTESIAN_POINT('Ctrl Pts',(0.351099124622182,1.92275921832282,8.61192775769871));
#27230=CARTESIAN_POINT('Ctrl Pts',(0.341797374888068,1.90433323216885,8.61088373004611));
#27231=CARTESIAN_POINT('Ctrl Pts',(0.331057329212009,1.88667321519026,8.60983970239351));
#27232=CARTESIAN_POINT('Ctrl Pts',(0.31903874364352,1.87000180423672,8.60879567474092));
#27233=CARTESIAN_POINT('Ctrl Pts',(0.314787927464619,1.86410534470722,8.60842641584505));
#27234=CARTESIAN_POINT('Ctrl Pts',(0.310377545040194,1.85833225532561,8.60805715694919));
#27235=CARTESIAN_POINT('Ctrl Pts',(0.305815820043715,1.85269133818042,8.60768789805332));
#27236=CARTESIAN_POINT('Ctrl Pts',(0.292918986526465,1.83674343045642,8.60664393540577));
#27237=CARTESIAN_POINT('Ctrl Pts',(0.278732872637427,1.82175955140427,8.60559997275822));
#27238=CARTESIAN_POINT('Ctrl Pts',(0.263427050212234,1.80795363515962,8.60455601011067));
#27239=CARTESIAN_POINT('Ctrl Pts',(0.248149384496693,1.79417311638558,8.6035139679449));
#27240=CARTESIAN_POINT('Ctrl Pts',(0.231756599267029,1.78156679043929,8.60247192577913));
#27241=CARTESIAN_POINT('Ctrl Pts',(0.214456368510273,1.77031324563249,8.60142988361336));
#27242=CARTESIAN_POINT('Ctrl Pts',(0.197174717929564,1.75907178695601,8.6003889605845));
#27243=CARTESIAN_POINT('Ctrl Pts',(0.17898815447507,1.74918064854344,8.59934803755565));
#27244=CARTESIAN_POINT('Ctrl Pts',(0.160134730736778,1.74077617282277,8.5983071145268));
#27245=CARTESIAN_POINT('Ctrl Pts',(0.141271624371436,1.73236738078241,8.59726565690701));
#27246=CARTESIAN_POINT('Ctrl Pts',(0.121741638985336,1.72544709105953,8.59622419928722));
#27247=CARTESIAN_POINT('Ctrl Pts',(0.101804887030289,1.72010441569196,8.59518274166742));
#27248=CARTESIAN_POINT('Ctrl Pts',(0.0818620435283626,1.71476010790414,
8.59414096583693));
#27249=CARTESIAN_POINT('Ctrl Pts',(0.0615129055036579,1.71099452942582,
8.59309919000643));
#27250=CARTESIAN_POINT('Ctrl Pts',(0.041029077495528,1.70884593214455,8.59205741417593));
#27251=CARTESIAN_POINT('Ctrl Pts',(0.0205009732283072,1.7066926906215,8.59101338652333));
#27252=CARTESIAN_POINT('Ctrl Pts',(-0.000161666023785048,1.70616342703306,
8.58996935887074));
#27253=CARTESIAN_POINT('Ctrl Pts',(-0.020685164375156,1.70724433298198,
8.58892533121814));
#27254=CARTESIAN_POINT('Ctrl Pts',(-0.0279440567250865,1.70762663524786,
8.58855607232227));
#27255=CARTESIAN_POINT('Ctrl Pts',(-0.0351855933376826,1.70820988616013,
8.58818681342641));
#27256=CARTESIAN_POINT('Ctrl Pts',(-0.0423979216362757,1.70899193583645,
8.58781755453054));
#27257=CARTESIAN_POINT('Ctrl Pts',(-0.0627884970019345,1.71120293375621,
8.58677359188299));
#27258=CARTESIAN_POINT('Ctrl Pts',(-0.0830664105610273,1.71501982783529,
8.58572962923543));
#27259=CARTESIAN_POINT('Ctrl Pts',(-0.102959990363347,1.72041584545139,
8.58468566658788));
#27260=CARTESIAN_POINT('Ctrl Pts',(-0.122816973781957,1.72580193651164,
8.58364362442211));
#27261=CARTESIAN_POINT('Ctrl Pts',(-0.14229030918972,1.73276125181886,8.58260158225634));
#27262=CARTESIAN_POINT('Ctrl Pts',(-0.161117418655004,1.74121584844652,
8.58155954009058));
#27263=CARTESIAN_POINT('Ctrl Pts',(-0.179924308100493,1.74966136497023,
8.58051861706172));
#27264=CARTESIAN_POINT('Ctrl Pts',(-0.198085669780768,1.75959870119769,
8.57947769403287));
#27265=CARTESIAN_POINT('Ctrl Pts',(-0.215358002372933,1.77090150286891,
8.57843677100402));
#27266=CARTESIAN_POINT('Ctrl Pts',(-0.232639205584959,1.7822101093645,8.57739531338423));
#27267=CARTESIAN_POINT('Ctrl Pts',(-0.249029843061413,1.79488519288077,
8.57635385576444));
#27268=CARTESIAN_POINT('Ctrl Pts',(-0.264314184235297,1.80875628416732,
8.57531239814465));
#27269=CARTESIAN_POINT('Ctrl Pts',(-0.279603195441744,1.82263161367698,
8.57427062231415));
#27270=CARTESIAN_POINT('Ctrl Pts',(-0.293784717345044,1.8377031575969,8.57322884648365));
#27271=CARTESIAN_POINT('Ctrl Pts',(-0.306679562628534,1.85376325240539,
8.57218707065316));
#27272=CARTESIAN_POINT('Ctrl Pts',(-0.319602280412728,1.86985806147326,
8.57114304300056));
#27273=CARTESIAN_POINT('Ctrl Pts',(-0.331232354691389,1.8869450785646,8.57009901534796));
#27274=CARTESIAN_POINT('Ctrl Pts',(-0.341433250110269,1.90478671735986,
8.56905498769537));
#27275=CARTESIAN_POINT('Ctrl Pts',(-0.345041173109191,1.9110970711381,8.56868572879949));
#27276=CARTESIAN_POINT('Ctrl Pts',(-0.348470739914145,1.91750160903484,
8.56831646990362));
#27277=CARTESIAN_POINT('Ctrl Pts',(-0.351717342170775,1.92398920142126,
8.56794721100774));
#27278=CARTESIAN_POINT('Ctrl Pts',(-0.361527929255108,1.94359341685747,
8.56683138397743));
#27279=CARTESIAN_POINT('Ctrl Pts',(-0.36971644841328,1.96406147404622,8.56571555694711));
#27280=CARTESIAN_POINT('Ctrl Pts',(-0.376146989037825,1.98511600356108,
8.56459972991679));
#27281=CARTESIAN_POINT('Ctrl Pts',(-0.382546775609156,2.00606983981251,
8.56348923932797));
#27282=CARTESIAN_POINT('Ctrl Pts',(-0.387205093490701,2.02760403730076,
8.56237874873916));
#27283=CARTESIAN_POINT('Ctrl Pts',(-0.390034423487106,2.04942294497422,
8.56126825815034));
#27284=CARTESIAN_POINT('Ctrl Pts',(-0.392201685815372,2.06613619394294,
8.5604176241055));
#27285=CARTESIAN_POINT('Ctrl Pts',(-0.393296703097738,2.08301597580068,
8.55956699006066));
#27286=CARTESIAN_POINT('Ctrl Pts',(-0.393299992556388,2.09992348107888,
8.55871635601582));
#27287=CARTESIAN_POINT('',(-0.393299833419068,2.10036198416185,8.43371635078876));
#27288=CARTESIAN_POINT('Ctrl Pts',(-0.392666085555113,2.09992368006247,
8.55871635220349));
#27289=CARTESIAN_POINT('Ctrl Pts',(-0.392544325623193,2.17030148723538,
8.55516985729731));
#27290=CARTESIAN_POINT('Ctrl Pts',(-0.340838535780804,2.37228409448114,
8.54499991455022));
#27291=CARTESIAN_POINT('Ctrl Pts',(-0.0172983767692793,2.56473195461531,
8.52820652396216));
#27292=CARTESIAN_POINT('Ctrl Pts',(0.381391024272932,2.36611258911132,8.50833618043939));
#27293=CARTESIAN_POINT('Ctrl Pts',(0.430206082244237,1.92337115105522,8.48846583691659));
#27294=CARTESIAN_POINT('Ctrl Pts',(0.0843656270259472,1.64266263605957,
8.46859549339382));
#27295=CARTESIAN_POINT('Ctrl Pts',(-0.304352146860463,1.77017617472703,
8.45034566515609));
#27296=CARTESIAN_POINT('Ctrl Pts',(-0.392351384769331,2.00145617334239,
8.43871928475933));
#27297=CARTESIAN_POINT('Ctrl Pts',(-0.393254489865089,2.10036191446037,
8.43371635220349));
#27298=CARTESIAN_POINT('',(-0.393299984454947,2.09988942089621,8.30871635220045));
#27299=CARTESIAN_POINT('Ctrl Pts',(-0.393299833419068,2.10036198416185,
8.43371635078876));
#27300=CARTESIAN_POINT('Ctrl Pts',(-0.393274985171444,2.12735988263749,
8.43235086541525));
#27301=CARTESIAN_POINT('Ctrl Pts',(-0.390466436935829,2.1542324317043,8.43098538004175));
#27302=CARTESIAN_POINT('Ctrl Pts',(-0.384972992563196,2.18050270179899,
8.42961989466824));
#27303=CARTESIAN_POINT('Ctrl Pts',(-0.383946991062761,2.18540915660324,
8.42936486522824));
#27304=CARTESIAN_POINT('Ctrl Pts',(-0.382827463398736,2.19029467012745,
8.42910983578824));
#27305=CARTESIAN_POINT('Ctrl Pts',(-0.381615229822244,2.19515622085663,
8.42885480634824));
#27306=CARTESIAN_POINT('Ctrl Pts',(-0.376652953412313,2.2150569718067,8.42781084370069));
#27307=CARTESIAN_POINT('Ctrl Pts',(-0.370115001986025,2.23462780852539,
8.42676688105314));
#27308=CARTESIAN_POINT('Ctrl Pts',(-0.362064829497629,2.25360322015131,
8.42572291840558));
#27309=CARTESIAN_POINT('Ctrl Pts',(-0.354029466168979,2.27254372446283,
8.42468087623981));
#27310=CARTESIAN_POINT('Ctrl Pts',(-0.344487633092111,2.29089028498473,
8.42363883407404));
#27311=CARTESIAN_POINT('Ctrl Pts',(-0.333552243348001,2.30839335631808,
8.42259679190827));
#27312=CARTESIAN_POINT('Ctrl Pts',(-0.322628598040686,2.32587762962779,
8.42155586887942));
#27313=CARTESIAN_POINT('Ctrl Pts',(-0.310314730644007,2.34251957600188,
8.42051494585056));
#27314=CARTESIAN_POINT('Ctrl Pts',(-0.296768923016812,2.3580951303908,8.4194740228217));
#27315=CARTESIAN_POINT('Ctrl Pts',(-0.283216158615866,2.3736786839785,8.41843256520191));
#27316=CARTESIAN_POINT('Ctrl Pts',(-0.268430660682067,2.38819418568803,
8.41739110758212));
#27317=CARTESIAN_POINT('Ctrl Pts',(-0.252610641546382,2.40145108023944,
8.41634964996232));
#27318=CARTESIAN_POINT('Ctrl Pts',(-0.236785788705156,2.41471202535008,
8.41530787413182));
#27319=CARTESIAN_POINT('Ctrl Pts',(-0.219926372111198,2.42671315328611,
8.41426609830132));
#27320=CARTESIAN_POINT('Ctrl Pts',(-0.202262485595872,2.4373051688317,8.41322432247082));
#27321=CARTESIAN_POINT('Ctrl Pts',(-0.184560418189,2.44792007925925,8.41218029481822));
#27322=CARTESIAN_POINT('Ctrl Pts',(-0.166051068783666,2.45711946866287,
8.41113626716562));
#27323=CARTESIAN_POINT('Ctrl Pts',(-0.146988378343778,2.4648003654492,8.41009223951302));
#27324=CARTESIAN_POINT('Ctrl Pts',(-0.140246154604264,2.46751699796321,
8.40972298061715));
#27325=CARTESIAN_POINT('Ctrl Pts',(-0.133434865917593,2.47004412688048,
8.40935372172129));
#27326=CARTESIAN_POINT('Ctrl Pts',(-0.126566165042659,2.47237869953368,
8.40898446282542));
#27327=CARTESIAN_POINT('Ctrl Pts',(-0.107147087449817,2.47897896475473,
8.40794050017787));
#27328=CARTESIAN_POINT('Ctrl Pts',(-0.0871524662926278,2.48407578567592,
8.40689653753031));
#27329=CARTESIAN_POINT('Ctrl Pts',(-0.0668398966291456,2.48757878969134,
8.40585257488276));
#27330=CARTESIAN_POINT('Ctrl Pts',(-0.0465646941263617,2.4910753495534,
8.40481053271699));
#27331=CARTESIAN_POINT('Ctrl Pts',(-0.0259734109011967,2.49298373017354,
8.40376849055122));
#27332=CARTESIAN_POINT('Ctrl Pts',(-0.00533699108396289,2.49326378745846,
8.40272644838545));
#27333=CARTESIAN_POINT('Ctrl Pts',(0.0152772655425789,2.49354354396624,
8.4016855253566));
#27334=CARTESIAN_POINT('Ctrl Pts',(0.0359358309370009,2.49219841006009,
8.40064460232775));
#27335=CARTESIAN_POINT('Ctrl Pts',(0.0563646263637204,2.48924018150093,
8.3996036792989));
#27336=CARTESIAN_POINT('Ctrl Pts',(0.0768039134873284,2.48628043367269,
8.39856222167911));
#27337=CARTESIAN_POINT('Ctrl Pts',(0.0970124644043837,2.48170602563857,
8.39752076405932));
#27338=CARTESIAN_POINT('Ctrl Pts',(0.116722760907488,2.47558046685915,8.39647930643953));
#27339=CARTESIAN_POINT('Ctrl Pts',(0.136439079765469,2.46945303645447,8.39543753060903));
#27340=CARTESIAN_POINT('Ctrl Pts',(0.155656149839517,2.46177376452319,8.39439575477853));
#27341=CARTESIAN_POINT('Ctrl Pts',(0.174123887090683,2.45265530188051,8.39335397894804));
#27342=CARTESIAN_POINT('Ctrl Pts',(0.192631542775007,2.44351712947389,8.39230995129544));
#27343=CARTESIAN_POINT('Ctrl Pts',(0.210385999370801,2.43293393280199,8.39126592364285));
#27344=CARTESIAN_POINT('Ctrl Pts',(0.22716321368654,2.42106348958984,8.39022189599025));
#27345=CARTESIAN_POINT('Ctrl Pts',(0.233097094478416,2.41686506942055,8.38985263709439));
#27346=CARTESIAN_POINT('Ctrl Pts',(0.238909023357031,2.4125059964861,8.38948337819852));
#27347=CARTESIAN_POINT('Ctrl Pts',(0.24459012573609,2.40799441617082,8.38911411930265));
#27348=CARTESIAN_POINT('Ctrl Pts',(0.260651644489097,2.39523935086752,8.3880701566551));
#27349=CARTESIAN_POINT('Ctrl Pts',(0.275760592487338,2.38118651666554,8.38702619400755));
#27350=CARTESIAN_POINT('Ctrl Pts',(0.289701541966313,2.36600358377725,8.38598223136));
#27351=CARTESIAN_POINT('Ctrl Pts',(0.303616845566501,2.35084858153006,8.38494018919423));
#27352=CARTESIAN_POINT('Ctrl Pts',(0.316367879830953,2.33456810283204,8.38389814702846));
#27353=CARTESIAN_POINT('Ctrl Pts',(0.327774223933871,2.31736823163597,8.38285610486268));
#27354=CARTESIAN_POINT('Ctrl Pts',(0.339168317802411,2.30018683283136,8.38181518183383));
#27355=CARTESIAN_POINT('Ctrl Pts',(0.349220159854912,2.28208859588042,8.38077425880498));
#27356=CARTESIAN_POINT('Ctrl Pts',(0.357791304406505,2.26331035634978,8.37973333577612));
#27357=CARTESIAN_POINT('Ctrl Pts',(0.366366850874548,2.24452247280473,8.37869187815633));
#27358=CARTESIAN_POINT('Ctrl Pts',(0.373459860454248,2.22505455164884,8.37765042053654));
#27359=CARTESIAN_POINT('Ctrl Pts',(0.378978920597747,2.2051659057992,8.37660896291674));
#27360=CARTESIAN_POINT('Ctrl Pts',(0.384499667054731,2.18527118310118,8.37556718708624));
#27361=CARTESIAN_POINT('Ctrl Pts',(0.38844534498379,2.16495619786109,8.37452541125574));
#27362=CARTESIAN_POINT('Ctrl Pts',(0.390775298198262,2.1444922051382,8.37348363542524));
#27363=CARTESIAN_POINT('Ctrl Pts',(0.39311028765948,2.12398397903066,8.37243960777265));
#27364=CARTESIAN_POINT('Ctrl Pts',(0.393822554570108,2.10332683845759,8.37139558012005));
#27365=CARTESIAN_POINT('Ctrl Pts',(0.392923482638502,2.0827945708792,8.37035155246745));
#27366=CARTESIAN_POINT('Ctrl Pts',(0.392605492681104,2.07553257696858,8.36998229357158));
#27367=CARTESIAN_POINT('Ctrl Pts',(0.392086408228187,2.06828615816552,8.36961303467572));
#27368=CARTESIAN_POINT('Ctrl Pts',(0.391368274090816,2.06106718562477,8.36924377577985));
#27369=CARTESIAN_POINT('Ctrl Pts',(0.389337977126443,2.04065782576755,8.36819981313229));
#27370=CARTESIAN_POINT('Ctrl Pts',(0.385700849074887,2.02034689870207,8.36715585048474));
#27371=CARTESIAN_POINT('Ctrl Pts',(0.380481255111292,2.00040630286541,8.36611188783718));
#27372=CARTESIAN_POINT('Ctrl Pts',(0.375271263153236,1.98050238990351,8.36506984567141));
#27373=CARTESIAN_POINT('Ctrl Pts',(0.368484710415906,1.96096817470571,8.36402780350564));
#27374=CARTESIAN_POINT('Ctrl Pts',(0.360197210923611,1.94206691530002,8.36298576133987));
#27375=CARTESIAN_POINT('Ctrl Pts',(0.351918612075579,1.92318595555,8.36194483831102));
#27376=CARTESIAN_POINT('Ctrl Pts',(0.342142534137718,1.90493728410428,8.36090391528217));
#27377=CARTESIAN_POINT('Ctrl Pts',(0.330993169544062,1.88756551194503,8.35986299225331));
#27378=CARTESIAN_POINT('Ctrl Pts',(0.319838078927337,1.87018481809637,8.35882153463352));
#27379=CARTESIAN_POINT('Ctrl Pts',(0.307308676506359,1.85368255116109,8.35778007701373));
#27380=CARTESIAN_POINT('Ctrl Pts',(0.293573513960775,1.83827594321362,8.35673861939394));
#27381=CARTESIAN_POINT('Ctrl Pts',(0.279834154724232,1.82286462787575,8.35569684356344));
#27382=CARTESIAN_POINT('Ctrl Pts',(0.264888818163925,1.8085501626491,8.35465506773294));
#27383=CARTESIAN_POINT('Ctrl Pts',(0.248943572461899,1.79551356724821,8.35361329190245));
#27384=CARTESIAN_POINT('Ctrl Pts',(0.232963860749445,1.78244879295053,8.35256926424985));
#27385=CARTESIAN_POINT('Ctrl Pts',(0.215980530050778,1.77066782273632,8.35152523659725));
#27386=CARTESIAN_POINT('Ctrl Pts',(0.19822994797147,1.76030929107903,8.35048120894466));
#27387=CARTESIAN_POINT('Ctrl Pts',(0.191951799760306,1.75664561420895,8.35011195004879));
#27388=CARTESIAN_POINT('Ctrl Pts',(0.185577891294464,1.75315945227831,8.34974269115293));
#27389=CARTESIAN_POINT('Ctrl Pts',(0.179119310946591,1.74985551204393,8.34937343225707));
#27390=CARTESIAN_POINT('Ctrl Pts',(0.160859719329671,1.74051466681835,8.34832946960951));
#27391=CARTESIAN_POINT('Ctrl Pts',(0.141813085065345,1.73257815738893,8.34728550696196));
#27392=CARTESIAN_POINT('Ctrl Pts',(0.122221214537222,1.72617268061704,8.34624154431441));
#27393=CARTESIAN_POINT('Ctrl Pts',(0.102665385366083,1.71977898740991,8.34519950214864));
#27394=CARTESIAN_POINT('Ctrl Pts',(0.0825669838577476,1.71491101881307,
8.34415745998287));
#27395=CARTESIAN_POINT('Ctrl Pts',(0.0621882933132476,1.71164770352837,
8.3431154178171));
#27396=CARTESIAN_POINT('Ctrl Pts',(0.0418314891622494,1.70838789299303,
8.34207449478825));
#27397=CARTESIAN_POINT('Ctrl Pts',(0.0211957118491833,1.7067294587717,8.34103357175939));
#27398=CARTESIAN_POINT('Ctrl Pts',(0.000553862276033012,1.70670038998674,
8.33999264873054));
#27399=CARTESIAN_POINT('Ctrl Pts',(-0.0200985884130663,1.70667130627282,
8.33895119111075));
#27400=CARTESIAN_POINT('Ctrl Pts',(-0.0407563818375821,1.7082732768905,
8.33790973349095));
#27401=CARTESIAN_POINT('Ctrl Pts',(-0.0611456253101985,1.71148217221674,
8.33686827587116));
#27402=CARTESIAN_POINT('Ctrl Pts',(-0.0815410985855914,1.7146920480004,
8.33582650004067));
#27403=CARTESIAN_POINT('Ctrl Pts',(-0.101667137965019,1.71950967589419,
8.33478472421017));
#27404=CARTESIAN_POINT('Ctrl Pts',(-0.121259990401106,1.72585977932342,
8.33374294837967));
#27405=CARTESIAN_POINT('Ctrl Pts',(-0.140895193232352,1.73222360864531,
8.33269892072707));
#27406=CARTESIAN_POINT('Ctrl Pts',(-0.159994227695969,1.74012624512724,
8.33165489307448));
#27407=CARTESIAN_POINT('Ctrl Pts',(-0.178312577388737,1.74944399199987,
8.33061086542188));
#27408=CARTESIAN_POINT('Ctrl Pts',(-0.184791537562655,1.75273955693399,
8.33024160652601));
#27409=CARTESIAN_POINT('Ctrl Pts',(-0.191173076753329,1.75621173084899,
8.32987234763015));
#27410=CARTESIAN_POINT('Ctrl Pts',(-0.197447235098884,1.75985373829512,
8.32950308873428));
#27411=CARTESIAN_POINT('Ctrl Pts',(-0.215185431878719,1.77015036155437,
8.32845912608673));
#27412=CARTESIAN_POINT('Ctrl Pts',(-0.232168878383375,1.78186893670427,
8.32741516343918));
#27413=CARTESIAN_POINT('Ctrl Pts',(-0.24816015145877,1.79487473190842,8.32637120079163));
#27414=CARTESIAN_POINT('Ctrl Pts',(-0.264122006864192,1.80785660155083,
8.32532915862586));
#27415=CARTESIAN_POINT('Ctrl Pts',(-0.279094709909914,1.82212057802843,
8.32428711646009));
#27416=CARTESIAN_POINT('Ctrl Pts',(-0.29286991724023,1.83748885437814,8.32324507429432));
#27417=CARTESIAN_POINT('Ctrl Pts',(-0.306630330214274,1.85284062544048,
8.32220415126547));
#27418=CARTESIAN_POINT('Ctrl Pts',(-0.319195290525201,1.86929381606614,
8.32116322823662));
#27419=CARTESIAN_POINT('Ctrl Pts',(-0.330393538228543,1.88663411730826,
8.32012230520777));
#27420=CARTESIAN_POINT('Ctrl Pts',(-0.341597537060042,1.90398332407716,
8.31908084758798));
#27421=CARTESIAN_POINT('Ctrl Pts',(-0.351433008325731,1.92221994229463,
8.31803938996819));
#27422=CARTESIAN_POINT('Ctrl Pts',(-0.359771977584116,1.94110061628435,
8.3169979323484));
#27423=CARTESIAN_POINT('Ctrl Pts',(-0.36811349476116,1.9599870591431,8.3159561565179));
#27424=CARTESIAN_POINT('Ctrl Pts',(-0.374957335741952,1.97951726242553,
8.31491438068741));
#27425=CARTESIAN_POINT('Ctrl Pts',(-0.38022402012802,1.99942870927702,8.31387260485691));
#27426=CARTESIAN_POINT('Ctrl Pts',(-0.385502088571906,2.01938319517272,
8.31282857720431));
#27427=CARTESIAN_POINT('Ctrl Pts',(-0.389196062778896,2.03971984522538,
8.31178454955172));
#27428=CARTESIAN_POINT('Ctrl Pts',(-0.391277588060175,2.06016610636892,
8.31074052189913));
#27429=CARTESIAN_POINT('Ctrl Pts',(-0.392013796268067,2.06739768093108,
8.31037126300325));
#27430=CARTESIAN_POINT('Ctrl Pts',(-0.392548772744236,2.07464294381873,
8.31000200410737));
#27431=CARTESIAN_POINT('Ctrl Pts',(-0.392882822954939,2.08188985292832,
8.30963274521149));
#27432=CARTESIAN_POINT('Ctrl Pts',(-0.393159161391042,2.08788475868127,
8.30932728087549));
#27433=CARTESIAN_POINT('Ctrl Pts',(-0.393298296559854,2.09388603750217,
8.30902181653949));
#27434=CARTESIAN_POINT('Ctrl Pts',(-0.393299984454931,2.09988942083648,
8.30871635220349));
#27435=CARTESIAN_POINT('',(-0.393299884528478,2.09969862003011,8.1837163522079));
#27436=CARTESIAN_POINT('Ctrl Pts',(-0.393299984454947,2.09988942089621,
8.30871635220045));
#27437=CARTESIAN_POINT('Ctrl Pts',(-0.393305711143422,2.12025770397181,
8.30767997259272));
#27438=CARTESIAN_POINT('Ctrl Pts',(-0.39172488296096,2.14069019931158,8.306643592985));
#27439=CARTESIAN_POINT('Ctrl Pts',(-0.388553715200407,2.16091716017643,
8.30560721337727));
#27440=CARTESIAN_POINT('Ctrl Pts',(-0.385388227722587,2.18110788995381,
8.30457269016115));
#27441=CARTESIAN_POINT('Ctrl Pts',(-0.380638108234441,2.20109307632513,
8.30353816694502));
#27442=CARTESIAN_POINT('Ctrl Pts',(-0.374351441161159,2.22060633690052,
8.30250364372889));
#27443=CARTESIAN_POINT('Ctrl Pts',(-0.367899197786451,2.24063353172393,
8.30144187355888));
#27444=CARTESIAN_POINT('Ctrl Pts',(-0.359828357115801,2.26016275633634,
8.30038010338886));
#27445=CARTESIAN_POINT('Ctrl Pts',(-0.350246196936911,2.27892034968452,
8.29931833321885));
#27446=CARTESIAN_POINT('Ctrl Pts',(-0.340913850098907,2.29718891999679,
8.2982842441091));
#27447=CARTESIAN_POINT('Ctrl Pts',(-0.33014852181264,2.31472498149889,8.29725015499935));
#27448=CARTESIAN_POINT('Ctrl Pts',(-0.318096431087108,2.33129969850747,
8.29621606588961));
#27449=CARTESIAN_POINT('Ctrl Pts',(-0.305560414972645,2.34853993708881,
8.29514045518945));
#27450=CARTESIAN_POINT('Ctrl Pts',(-0.291632488933008,2.36473918448366,
8.2940648444893));
#27451=CARTESIAN_POINT('Ctrl Pts',(-0.276523297341258,2.37967795055656,
8.29298923378915));
#27452=CARTESIAN_POINT('Ctrl Pts',(-0.261414105749512,2.39461671662945,
8.291913623089));
#27453=CARTESIAN_POINT('Ctrl Pts',(-0.245124381763525,2.40829447491523,
8.29083801238885));
#27454=CARTESIAN_POINT('Ctrl Pts',(-0.227901906916449,2.42053956202604,
8.2897624016887));
#27455=CARTESIAN_POINT('Ctrl Pts',(-0.211186174694493,2.43242435785221,
8.28871843904114));
#27456=CARTESIAN_POINT('Ctrl Pts',(-0.193488468378395,2.44303348834778,
8.28767447639359));
#27457=CARTESIAN_POINT('Ctrl Pts',(-0.175029715533555,2.45220659942744,
8.28663051374603));
#27458=CARTESIAN_POINT('Ctrl Pts',(-0.15660491955362,2.46136283558081,8.28558847158026));
#27459=CARTESIAN_POINT('Ctrl Pts',(-0.137422481037262,2.46908791901188,
8.28454642941449));
#27460=CARTESIAN_POINT('Ctrl Pts',(-0.117730501263245,2.47526579789838,
8.28350438724872));
#27461=CARTESIAN_POINT('Ctrl Pts',(-0.0980596703661509,2.48143704184,8.28246346421987));
#27462=CARTESIAN_POINT('Ctrl Pts',(-0.0778810744356029,2.48606413332962,
8.28142254119101));
#27463=CARTESIAN_POINT('Ctrl Pts',(-0.0574606918412579,2.48907988754641,
8.28038161816215));
#27464=CARTESIAN_POINT('Ctrl Pts',(-0.037029821870632,2.49209719057596,
8.27934016054236));
#27465=CARTESIAN_POINT('Ctrl Pts',(-0.0163576426898396,2.49350137964718,
8.27829870292257));
#27466=CARTESIAN_POINT('Ctrl Pts',(0.00428134411018631,2.49327669660509,
8.27725724530278));
#27467=CARTESIAN_POINT('Ctrl Pts',(0.0249266370204593,2.49305194491253,
8.27621546947228));
#27468=CARTESIAN_POINT('Ctrl Pts',(0.0455379826392764,2.49119737450204,
8.27517369364178));
#27469=CARTESIAN_POINT('Ctrl Pts',(0.0658435110427064,2.48774930309875,
8.27413191781128));
#27470=CARTESIAN_POINT('Ctrl Pts',(0.0861929303065745,2.48429377861088,
8.27308789015868));
#27471=CARTESIAN_POINT('Ctrl Pts',(0.10623449853258,2.47923805671871,8.27204386250608));
#27472=CARTESIAN_POINT('Ctrl Pts',(0.125708373296824,2.4726691493578,8.27099983485349));
#27473=CARTESIAN_POINT('Ctrl Pts',(0.132596027542103,2.47034581292789,8.27063057595762));
#27474=CARTESIAN_POINT('Ctrl Pts',(0.139412842493954,2.46783362900765,8.27026131706176));
#27475=CARTESIAN_POINT('Ctrl Pts',(0.146147982674934,2.46513786048566,8.2698920581659));
#27476=CARTESIAN_POINT('Ctrl Pts',(0.165189459681377,2.45751642827389,8.26884809551835));
#27477=CARTESIAN_POINT('Ctrl Pts',(0.183689894758163,2.44837879396887,8.26780413287079));
#27478=CARTESIAN_POINT('Ctrl Pts',(0.201394867236247,2.43782391485935,8.26676017022324));
#27479=CARTESIAN_POINT('Ctrl Pts',(0.219067269509644,2.4272884525873,8.26571812805747));
#27480=CARTESIAN_POINT('Ctrl Pts',(0.235946458544924,2.41534124207763,8.2646760858917));
#27481=CARTESIAN_POINT('Ctrl Pts',(0.251800554186977,2.40212807037932,8.26363404372593));
#27482=CARTESIAN_POINT('Ctrl Pts',(0.267637622779372,2.38892908941984,8.26259312069708));
#27483=CARTESIAN_POINT('Ctrl Pts',(0.282451202730362,2.37446729290567,8.26155219766822));
#27484=CARTESIAN_POINT('Ctrl Pts',(0.296040824942273,2.35892995185474,8.26051127463937));
#27485=CARTESIAN_POINT('Ctrl Pts',(0.309637426429964,2.3433846312304,8.25946981701958));
#27486=CARTESIAN_POINT('Ctrl Pts',(0.322008317855323,2.32676320576889,8.25842835939978));
#27487=CARTESIAN_POINT('Ctrl Pts',(0.332991656808402,2.30928795114864,8.25738690177999));
#27488=CARTESIAN_POINT('Ctrl Pts',(0.343978351650364,2.29180735707624,8.2563451259495));
#27489=CARTESIAN_POINT('Ctrl Pts',(0.35357628945113,2.27347305617333,8.255303350119));
#27490=CARTESIAN_POINT('Ctrl Pts',(0.361668838702044,2.25453330098045,8.2542615742885));
#27491=CARTESIAN_POINT('Ctrl Pts',(0.369778880181808,2.23555260707692,8.2532175466359));
#27492=CARTESIAN_POINT('Ctrl Pts',(0.376376801704175,2.21596454406923,8.2521735189833));
#27493=CARTESIAN_POINT('Ctrl Pts',(0.381395107063358,2.19603469325264,8.25112949133071));
#27494=CARTESIAN_POINT('Ctrl Pts',(0.383170015890168,2.18898576625448,8.25076023243484));
#27495=CARTESIAN_POINT('Ctrl Pts',(0.384747791776386,2.18189417564379,8.25039097353898));
#27496=CARTESIAN_POINT('Ctrl Pts',(0.386126994413248,2.1747718809807,8.25002171464312));
#27497=CARTESIAN_POINT('Ctrl Pts',(0.390026253313782,2.15463584722102,8.24897775199557));
#27498=CARTESIAN_POINT('Ctrl Pts',(0.392357786575117,2.1341339836137,8.24793378934802));
#27499=CARTESIAN_POINT('Ctrl Pts',(0.393067076752167,2.11353377898098,8.24688982670046));
#27500=CARTESIAN_POINT('Ctrl Pts',(0.393775062113507,2.09297147064448,8.24584778453469));
#27501=CARTESIAN_POINT('Ctrl Pts',(0.392866643621935,2.07231190537088,8.24480574236892));
#27502=CARTESIAN_POINT('Ctrl Pts',(0.390338880720678,2.05182896931009,8.24376370020315));
#27503=CARTESIAN_POINT('Ctrl Pts',(0.387813832597066,2.03136803160085,8.2427227771743));
#27504=CARTESIAN_POINT('Ctrl Pts',(0.383672953650289,2.01108407658885,8.24168185414545));
#27505=CARTESIAN_POINT('Ctrl Pts',(0.377965187160364,1.99124703546647,8.24064093111659));
#27506=CARTESIAN_POINT('Ctrl Pts',(0.372254489310332,1.97139980655679,8.2395994734968));
#27507=CARTESIAN_POINT('Ctrl Pts',(0.364975484242306,1.95200066162075,8.23855801587701));
#27508=CARTESIAN_POINT('Ctrl Pts',(0.356227457105592,1.93330600249534,8.23751655825721));
#27509=CARTESIAN_POINT('Ctrl Pts',(0.347476757065207,1.91460563133655,8.23647478242671));
#27510=CARTESIAN_POINT('Ctrl Pts',(0.337256485756988,1.89661082502997,8.23543300659622));
#27511=CARTESIAN_POINT('Ctrl Pts',(0.325712243618799,1.87955403302213,8.23439123076572));
#27512=CARTESIAN_POINT('Ctrl Pts',(0.314143048339255,1.8624603723713,8.23334720311312));
#27513=CARTESIAN_POINT('Ctrl Pts',(0.30124462838715,1.84630934938367,8.23230317546053));
#27514=CARTESIAN_POINT('Ctrl Pts',(0.287203752354838,1.83130148003143,8.23125914780793));
#27515=CARTESIAN_POINT('Ctrl Pts',(0.282237678546511,1.82599339336095,8.23088988891206));
#27516=CARTESIAN_POINT('Ctrl Pts',(0.277129020786189,1.82082796501212,8.23052063001619));
#27517=CARTESIAN_POINT('Ctrl Pts',(0.271887055220996,1.81581287994834,8.23015137112032));
#27518=CARTESIAN_POINT('Ctrl Pts',(0.257067056810563,1.80163431434178,8.22910740847277));
#27519=CARTESIAN_POINT('Ctrl Pts',(0.241090823898778,1.78857589021517,8.22806344582521));
#27520=CARTESIAN_POINT('Ctrl Pts',(0.224153754598498,1.77682824334513,8.22701948317766));
#27521=CARTESIAN_POINT('Ctrl Pts',(0.207247842862268,1.76510220753738,8.22597744101189));
#27522=CARTESIAN_POINT('Ctrl Pts',(0.189385167139861,1.75468262609251,8.22493539884612));
#27523=CARTESIAN_POINT('Ctrl Pts',(0.170794424033357,1.74572023100505,8.22389335668035));
#27524=CARTESIAN_POINT('Ctrl Pts',(0.152223647092894,1.73676746138912,8.2228524336515));
#27525=CARTESIAN_POINT('Ctrl Pts',(0.132927001952251,1.72926911519165,8.22181151062265));
#27526=CARTESIAN_POINT('Ctrl Pts',(0.11315794547275,1.72333015865829,8.22077058759379));
#27527=CARTESIAN_POINT('Ctrl Pts',(0.0933787361210852,1.71738815203165,
8.219729129974));
#27528=CARTESIAN_POINT('Ctrl Pts',(0.0731273307625204,1.71300736214477,
8.21868767235421));
#27529=CARTESIAN_POINT('Ctrl Pts',(0.0526730614975844,1.71024310321372,
8.21764621473442));
#27530=CARTESIAN_POINT('Ctrl Pts',(0.0322125425616538,1.70747799968105,
8.21660443890393));
#27531=CARTESIAN_POINT('Ctrl Pts',(0.0115497697054225,1.7063304729854,8.21556266307343));
#27532=CARTESIAN_POINT('Ctrl Pts',(-0.00904099326675641,1.70680392875723,
8.21452088724293));
#27533=CARTESIAN_POINT('Ctrl Pts',(-0.0296762636403592,1.70727840791445,
8.21347685959033));
#27534=CARTESIAN_POINT('Ctrl Pts',(-0.0502384807222144,1.70938078977478,
8.21243283193774));
#27535=CARTESIAN_POINT('Ctrl Pts',(-0.0704579458790627,1.71306257888064,
8.21138880428514));
#27536=CARTESIAN_POINT('Ctrl Pts',(-0.0776093056732729,1.71436477942739,
8.21101954538928));
#27537=CARTESIAN_POINT('Ctrl Pts',(-0.0847178990659698,1.71586409064105,
8.21065028649341));
#27538=CARTESIAN_POINT('Ctrl Pts',(-0.0917722430562946,1.71755687298055,
8.21028102759754));
#27539=CARTESIAN_POINT('Ctrl Pts',(-0.111716167796723,1.72234267923373,
8.20923706494999));
#27540=CARTESIAN_POINT('Ctrl Pts',(-0.131344148152779,1.72870702098008,
8.20819310230244));
#27541=CARTESIAN_POINT('Ctrl Pts',(-0.150390121621155,1.73658879857829,
8.20714913965488));
#27542=CARTESIAN_POINT('Ctrl Pts',(-0.169401057969011,1.74445607679729,
8.20610709748911));
#27543=CARTESIAN_POINT('Ctrl Pts',(-0.187831417730646,1.75383502665889,
8.20506505532335));
#27544=CARTESIAN_POINT('Ctrl Pts',(-0.205430665143305,1.76461494991759,
8.20402301315758));
#27545=CARTESIAN_POINT('Ctrl Pts',(-0.223011011240724,1.77538329570806,
8.20298209012872));
#27546=CARTESIAN_POINT('Ctrl Pts',(-0.239761377659703,1.78754927015365,
8.20194116709987));
#27547=CARTESIAN_POINT('Ctrl Pts',(-0.255456306122845,1.80095658231275,
8.20090024407101));
#27548=CARTESIAN_POINT('Ctrl Pts',(-0.271159295092185,1.81437078011793,
8.19985878645122));
#27549=CARTESIAN_POINT('Ctrl Pts',(-0.285805193304681,1.82902712361073,
8.19881732883143));
#27550=CARTESIAN_POINT('Ctrl Pts',(-0.299201697244564,1.84472909612341,
8.19777587121164));
#27551=CARTESIAN_POINT('Ctrl Pts',(-0.312602294400451,1.86043586627325,
8.19673409538114));
#27552=CARTESIAN_POINT('Ctrl Pts',(-0.324752287691612,1.87718831871015,
8.19569231955064));
#27553=CARTESIAN_POINT('Ctrl Pts',(-0.335500349650052,1.89475769104619,
8.19465054372014));
#27554=CARTESIAN_POINT('Ctrl Pts',(-0.346271643788316,1.91236503997922,
8.19360651606754));
#27555=CARTESIAN_POINT('Ctrl Pts',(-0.355634623120393,1.93079217754411,
8.19256248841494));
#27556=CARTESIAN_POINT('Ctrl Pts',(-0.363484070751981,1.94978608483376,
8.19151846076234));
#27557=CARTESIAN_POINT('Ctrl Pts',(-0.366260317490647,1.95650398087466,
8.19114920186648));
#27558=CARTESIAN_POINT('Ctrl Pts',(-0.368847679825564,1.96329261772501,
8.19077994297061));
#27559=CARTESIAN_POINT('Ctrl Pts',(-0.371243001992155,1.97014037012276,
8.19041068407475));
#27560=CARTESIAN_POINT('Ctrl Pts',(-0.379130780091446,1.99268996789535,
8.18919471727395));
#27561=CARTESIAN_POINT('Ctrl Pts',(-0.384971037397137,2.01599100857184,
8.18797875047315));
#27562=CARTESIAN_POINT('Ctrl Pts',(-0.388648914697292,2.03969319188833,
8.18676278367236));
#27563=CARTESIAN_POINT('Ctrl Pts',(-0.391720380442988,2.05948733895021,
8.18574730651754));
#27564=CARTESIAN_POINT('Ctrl Pts',(-0.393284453216479,2.07956080785454,
8.18473182936272));
#27565=CARTESIAN_POINT('Ctrl Pts',(-0.393299884528477,2.09969862003011,
8.1837163522079));
#27566=CARTESIAN_POINT('',(-0.393134897346159,2.1002525601452,8.058716300174));
#27567=CARTESIAN_POINT('Ctrl Pts',(-0.393299884528545,2.09969862011757,
8.18371635220349));
#27568=CARTESIAN_POINT('Ctrl Pts',(-0.393315697990375,2.12033514257448,
8.18267572688992));
#27569=CARTESIAN_POINT('Ctrl Pts',(-0.391702978785827,2.14098969196552,
8.18163510157636));
#27570=CARTESIAN_POINT('Ctrl Pts',(-0.388479577251369,2.1613881752343,8.18059447626279));
#27571=CARTESIAN_POINT('Ctrl Pts',(-0.385253698249265,2.18180233653196,
8.17955305113713));
#27572=CARTESIAN_POINT('Ctrl Pts',(-0.380414773381228,2.2019593117515,8.17851162601146));
#27573=CARTESIAN_POINT('Ctrl Pts',(-0.374032193501926,2.2215927967609,8.17747020088579));
#27574=CARTESIAN_POINT('Ctrl Pts',(-0.367646440359054,2.24123604306181,
8.17642825798887));
#27575=CARTESIAN_POINT('Ctrl Pts',(-0.359715774467009,2.2603545976506,8.17538631509195));
#27576=CARTESIAN_POINT('Ctrl Pts',(-0.35035827337408,2.27870078421298,8.17434437219502));
#27577=CARTESIAN_POINT('Ctrl Pts',(-0.34097968932248,2.29708830573105,8.17330008174411));
#27578=CARTESIAN_POINT('Ctrl Pts',(-0.330168246545375,2.3146993652735,8.17225579129319));
#27579=CARTESIAN_POINT('Ctrl Pts',(-0.318086425579717,2.33131345802162,
8.17121150084228));
#27580=CARTESIAN_POINT('Ctrl Pts',(-0.31549811678757,2.33487272300789,8.17098778074551));
#27581=CARTESIAN_POINT('Ctrl Pts',(-0.312851648599206,2.33838635565434,
8.17076406064873));
#27582=CARTESIAN_POINT('Ctrl Pts',(-0.310148846771198,2.34185239888514,
8.17054034055196));
#27583=CARTESIAN_POINT('Ctrl Pts',(-0.297536550456057,2.35802626846555,
8.1694963779044));
#27584=CARTESIAN_POINT('Ctrl Pts',(-0.283618098539485,2.37325909994786,
8.16845241525685));
#27585=CARTESIAN_POINT('Ctrl Pts',(-0.268559246455048,2.38733398884138,
8.1674084526093));
#27586=CARTESIAN_POINT('Ctrl Pts',(-0.253528096751699,2.40138298546013,
8.16636641044353));
#27587=CARTESIAN_POINT('Ctrl Pts',(-0.237361201966722,2.41427772758481,
8.16532436827776));
#27588=CARTESIAN_POINT('Ctrl Pts',(-0.22026303984912,2.42583597603154,8.16428232611199));
#27589=CARTESIAN_POINT('Ctrl Pts',(-0.203183240889036,2.43738181110101,
8.16324140308313));
#27590=CARTESIAN_POINT('Ctrl Pts',(-0.185174750446051,2.44759356811661,
8.16220048005428));
#27591=CARTESIAN_POINT('Ctrl Pts',(-0.16647316848108,2.4563307089992,8.16115955702543));
#27592=CARTESIAN_POINT('Ctrl Pts',(-0.14776198187103,2.46507233704962,8.16011809940564));
#27593=CARTESIAN_POINT('Ctrl Pts',(-0.128357652416436,2.47233750996205,
8.15907664178584));
#27594=CARTESIAN_POINT('Ctrl Pts',(-0.108518673153725,2.4780325218509,8.15803518416605));
#27595=CARTESIAN_POINT('Ctrl Pts',(-0.0886736322179369,2.48372927381417,
8.15699340833556));
#27596=CARTESIAN_POINT('Ctrl Pts',(-0.0683943936949748,2.48785474161243,
8.15595163250506));
#27597=CARTESIAN_POINT('Ctrl Pts',(-0.0479518418811187,2.49036586794981,
8.15490985667456));
#27598=CARTESIAN_POINT('Ctrl Pts',(-0.0274651030276245,2.49288242214376,
8.15386582902196));
#27599=CARTESIAN_POINT('Ctrl Pts',(-0.00681508191190315,2.49377763649144,
8.15282180136937));
#27600=CARTESIAN_POINT('Ctrl Pts',(0.0137243439128156,2.49306046911915,
8.15177777371677));
#27601=CARTESIAN_POINT('Ctrl Pts',(0.0209888696012749,2.49280681642002,
8.1514085148209));
#27602=CARTESIAN_POINT('Ctrl Pts',(0.028239602034006,2.49235193915431,8.15103925592504));
#27603=CARTESIAN_POINT('Ctrl Pts',(0.0354646524095694,2.49169777690136,
8.15066999702917));
#27604=CARTESIAN_POINT('Ctrl Pts',(0.0558911954210694,2.48984834019135,
8.14962603438162));
#27605=CARTESIAN_POINT('Ctrl Pts',(0.0762335423787659,2.48639126353976,
8.14858207173407));
#27606=CARTESIAN_POINT('Ctrl Pts',(0.0962195896921495,2.48134850276286,
8.14753810908651));
#27607=CARTESIAN_POINT('Ctrl Pts',(0.116168870517875,2.4763150186878,8.14649606692074));
#27608=CARTESIAN_POINT('Ctrl Pts',(0.135762432833069,2.4697017609996,8.14545402475497));
#27609=CARTESIAN_POINT('Ctrl Pts',(0.154736359168832,2.46158200888758,8.1444119825892));
#27610=CARTESIAN_POINT('Ctrl Pts',(0.173689907805802,2.45347097726176,8.14337105956035));
#27611=CARTESIAN_POINT('Ctrl Pts',(0.192024457209319,2.44385692465364,8.14233013653149));
#27612=CARTESIAN_POINT('Ctrl Pts',(0.209494305930319,2.43286187192704,8.14128921350264));
#27613=CARTESIAN_POINT('Ctrl Pts',(0.226973126710294,2.42186117242793,8.14024775588285));
#27614=CARTESIAN_POINT('Ctrl Pts',(0.243585728321268,2.40947843417078,8.13920629826305));
#27615=CARTESIAN_POINT('Ctrl Pts',(0.259113394225609,2.39588027803976,8.13816484064326));
#27616=CARTESIAN_POINT('Ctrl Pts',(0.274645804508845,2.3822779670792,8.13712306481276));
#27617=CARTESIAN_POINT('Ctrl Pts',(0.289092089932649,2.36746001050347,8.13608128898226));
#27618=CARTESIAN_POINT('Ctrl Pts',(0.302269412587609,2.35163086498667,8.13503951315176));
#27619=CARTESIAN_POINT('Ctrl Pts',(0.315475218324509,2.33576750441264,8.13399548549917));
#27620=CARTESIAN_POINT('Ctrl Pts',(0.327406160128445,2.31888919263453,8.13295145784657));
#27621=CARTESIAN_POINT('Ctrl Pts',(0.337921515284175,2.30123105999832,8.13190743019397));
#27622=CARTESIAN_POINT('Ctrl Pts',(0.341640658570052,2.29498560994338,8.13153817129811));
#27623=CARTESIAN_POINT('Ctrl Pts',(0.345183142098988,2.28864283101102,8.13116891240224));
#27624=CARTESIAN_POINT('Ctrl Pts',(0.348544161080997,2.28221376944771,8.13079965350638));
#27625=CARTESIAN_POINT('Ctrl Pts',(0.358046378398528,2.26403763285064,8.12975569085883));
#27626=CARTESIAN_POINT('Ctrl Pts',(0.366151286424129,2.24506204525451,8.12871172821127));
#27627=CARTESIAN_POINT('Ctrl Pts',(0.37273005141108,2.22552768131011,8.12766776556372));
#27628=CARTESIAN_POINT('Ctrl Pts',(0.379296714050938,2.20602925293313,8.12662572339795));
#27629=CARTESIAN_POINT('Ctrl Pts',(0.384342517894813,2.18597475904724,8.12558368123218));
#27630=CARTESIAN_POINT('Ctrl Pts',(0.38778621410251,2.16562577353481,8.12454163906641));
#27631=CARTESIAN_POINT('Ctrl Pts',(0.391226211834579,2.14529864251315,8.12350071603756));
#27632=CARTESIAN_POINT('Ctrl Pts',(0.393067367144397,2.12467836471419,8.1224597930087));
#27633=CARTESIAN_POINT('Ctrl Pts',(0.393279274725038,2.1040375824138,8.12141886997985));
#27634=CARTESIAN_POINT('Ctrl Pts',(0.393491291135889,2.08338619954558,8.12037741236005));
#27635=CARTESIAN_POINT('Ctrl Pts',(0.392072364526663,2.0627150267122,8.11933595474027));
#27636=CARTESIAN_POINT('Ctrl Pts',(0.389044197506231,2.04229815958973,8.11829449712047));
#27637=CARTESIAN_POINT('Ctrl Pts',(0.386015105248758,2.02187505422425,8.11725272128998));
#27638=CARTESIAN_POINT('Ctrl Pts',(0.381375937381233,2.00170713115017,8.11621094545948));
#27639=CARTESIAN_POINT('Ctrl Pts',(0.375199631271861,1.9820587998473,8.11516916962898));
#27640=CARTESIAN_POINT('Ctrl Pts',(0.369009974936675,1.96236799823044,8.11412514197638));
#27641=CARTESIAN_POINT('Ctrl Pts',(0.361276822574777,1.94319971360829,8.11308111432379));
#27642=CARTESIAN_POINT('Ctrl Pts',(0.352121700242478,1.9247995484642,8.11203708667119));
#27643=CARTESIAN_POINT('Ctrl Pts',(0.34888365347663,1.91829165123757,8.11166782777532));
#27644=CARTESIAN_POINT('Ctrl Pts',(0.345468141729564,1.91187960681759,8.11129856887946));
#27645=CARTESIAN_POINT('Ctrl Pts',(0.341881851963449,1.90557343469052,8.11092930998359));
#27646=CARTESIAN_POINT('Ctrl Pts',(0.331742752808256,1.88774472907665,8.10988534733604));
#27647=CARTESIAN_POINT('Ctrl Pts',(0.32017507217187,1.87065814886244,8.10884138468849));
#27648=CARTESIAN_POINT('Ctrl Pts',(0.307311433574845,1.85455230130601,8.10779742204093));
#27649=CARTESIAN_POINT('Ctrl Pts',(0.294471459027154,1.83847608219167,8.10675537987516));
#27650=CARTESIAN_POINT('Ctrl Pts',(0.280340666297115,1.82337762007559,8.10571333770939));
#27651=CARTESIAN_POINT('Ctrl Pts',(0.265095009923085,1.80946682510619,8.10467129554362));
#27652=CARTESIAN_POINT('Ctrl Pts',(0.249865727144491,1.79557097011204,8.10363037251477));
#27653=CARTESIAN_POINT('Ctrl Pts',(0.233524479014521,1.78286076480544,8.10258944948591));
#27654=CARTESIAN_POINT('Ctrl Pts',(0.216284049098182,1.77150936070309,8.10154852645706));
#27655=CARTESIAN_POINT('Ctrl Pts',(0.199034764946384,1.76015212681544,8.10050706883727));
#27656=CARTESIAN_POINT('Ctrl Pts',(0.180885982111509,1.75015550635439,8.09946561121748));
#27657=CARTESIAN_POINT('Ctrl Pts',(0.162079913159837,1.74164962431986,8.09842415359768));
#27658=CARTESIAN_POINT('Ctrl Pts',(0.143268098134222,1.73314114336754,8.09738237776718));
#27659=CARTESIAN_POINT('Ctrl Pts',(0.123799281928152,1.72612457760075,8.09634060193669));
#27660=CARTESIAN_POINT('Ctrl Pts',(0.103935267081649,1.7206817296034,8.09529882610619));
#27661=CARTESIAN_POINT('Ctrl Pts',(0.0840283157162946,1.7152271167666,8.09425479845359));
#27662=CARTESIAN_POINT('Ctrl Pts',(0.0637251837069782,1.71135315091492,
8.093210770801));
#27663=CARTESIAN_POINT('Ctrl Pts',(0.0432981622691779,1.70909059982636,
8.0921667431484));
#27664=CARTESIAN_POINT('Ctrl Pts',(0.036073392538989,1.7082903651633,8.09179748425253));
#27665=CARTESIAN_POINT('Ctrl Pts',(0.0288331525638997,1.70769123309004,
8.09142822535667));
#27666=CARTESIAN_POINT('Ctrl Pts',(0.0215894866807903,1.70729300481802,
8.0910589664608));
#27667=CARTESIAN_POINT('Ctrl Pts',(0.00111031421407299,1.70616714042898,
8.09001500381325));
#27668=CARTESIAN_POINT('Ctrl Pts',(-0.0195181828979126,1.70664417881538,
8.0889710411657));
#27669=CARTESIAN_POINT('Ctrl Pts',(-0.0400235878923866,1.70874177016679,
8.08792707851814));
#27670=CARTESIAN_POINT('Ctrl Pts',(-0.0604912709847918,1.71083550277287,
8.08688503635237));
#27671=CARTESIAN_POINT('Ctrl Pts',(-0.0808355816926341,1.71454385594809,
8.08584299418661));
#27672=CARTESIAN_POINT('Ctrl Pts',(-0.100784776433899,1.7198325121224,8.08480095202084));
#27673=CARTESIAN_POINT('Ctrl Pts',(-0.120712546053408,1.72511548836305,
8.08376002899198));
#27674=CARTESIAN_POINT('Ctrl Pts',(-0.140245327123944,1.7319752385794,8.08271910596313));
#27675=CARTESIAN_POINT('Ctrl Pts',(-0.159122347161594,1.74032658058485,
8.08167818293428));
#27676=CARTESIAN_POINT('Ctrl Pts',(-0.178009061944737,1.7486822116219,8.08063672531449));
#27677=CARTESIAN_POINT('Ctrl Pts',(-0.196238663487924,1.75853068188917,
8.0795952676947));
#27678=CARTESIAN_POINT('Ctrl Pts',(-0.213570626322764,1.76973877373797,
8.07855381007491));
#27679=CARTESIAN_POINT('Ctrl Pts',(-0.230907884827876,1.78095029014746,
8.07751203424441));
#27680=CARTESIAN_POINT('Ctrl Pts',(-0.247346360943412,1.7935218255598,8.07647025841391));
#27681=CARTESIAN_POINT('Ctrl Pts',(-0.262675555146807,1.80727753292869,
8.07542848258342));
#27682=CARTESIAN_POINT('Ctrl Pts',(-0.278037883751325,1.82106297357119,
8.07438445493082));
#27683=CARTESIAN_POINT('Ctrl Pts',(-0.292285635811347,1.83603716276604,
8.07334042727823));
#27684=CARTESIAN_POINT('Ctrl Pts',(-0.305245545073329,1.85198780833821,
8.07229639962563));
#27685=CARTESIAN_POINT('Ctrl Pts',(-0.309829295104064,1.85762934260004,
8.07192714072976));
#27686=CARTESIAN_POINT('Ctrl Pts',(-0.314252328799765,1.86339274498632,
8.07155788183389));
#27687=CARTESIAN_POINT('Ctrl Pts',(-0.318508293488239,1.86926778079512,
8.07118862293802));
#27688=CARTESIAN_POINT('Ctrl Pts',(-0.330631578193252,1.88600305398831,
8.07013677428508));
#27689=CARTESIAN_POINT('Ctrl Pts',(-0.341468108319497,1.90374564296446,
8.06908492563215));
#27690=CARTESIAN_POINT('Ctrl Pts',(-0.350853335476031,1.92227316751446,
8.06803307697922));
#27691=CARTESIAN_POINT('Ctrl Pts',(-0.360219866270163,1.94076378328137,
8.06698332371974));
#27692=CARTESIAN_POINT('Ctrl Pts',(-0.368140456170937,1.96003562340037,
8.06593357046027));
#27693=CARTESIAN_POINT('Ctrl Pts',(-0.374494500045934,1.97983861087959,
8.06488381720079));
#27694=CARTESIAN_POINT('Ctrl Pts',(-0.380843023719858,1.99962439412244,
8.06383497593519));
#27695=CARTESIAN_POINT('Ctrl Pts',(-0.38562743929961,2.01993973991456,8.06278613466959));
#27696=CARTESIAN_POINT('Ctrl Pts',(-0.38877563735936,2.04051560039957,8.06173729340398));
#27697=CARTESIAN_POINT('Ctrl Pts',(-0.39179818600039,2.06027024669775,8.06073031300382));
#27698=CARTESIAN_POINT('Ctrl Pts',(-0.393312707412277,2.08026435563854,
8.05972333260365));
#27699=CARTESIAN_POINT('Ctrl Pts',(-0.393299919501896,2.10025163426288,
8.05871635220349));
#27700=CARTESIAN_POINT('',(-0.393495572071111,2.10018686531557,7.93371641359789));
#27701=CARTESIAN_POINT('Ctrl Pts',(-0.39282171143197,2.10025431732318,8.05871620143025));
#27702=CARTESIAN_POINT('Ctrl Pts',(-0.393106694558029,2.14914144428112,
8.05625022742525));
#27703=CARTESIAN_POINT('Ctrl Pts',(-0.361959072798305,2.32898542981025,
8.04716080557931));
#27704=CARTESIAN_POINT('Ctrl Pts',(-0.0924540126689525,2.55577108181745,
8.03144793589244));
#27705=CARTESIAN_POINT('Ctrl Pts',(0.333173458296833,2.42445411103268,8.01157759236963));
#27706=CARTESIAN_POINT('Ctrl Pts',(0.453159638745708,1.9954946638146,7.99170724884688));
#27707=CARTESIAN_POINT('Ctrl Pts',(0.157433542759797,1.66240463542945,7.97183690532405));
#27708=CARTESIAN_POINT('Ctrl Pts',(-0.270752563968054,1.72889110048612,
7.95250666287296));
#27709=CARTESIAN_POINT('Ctrl Pts',(-0.39313119258737,1.9803820937068,7.93979986826274));
#27710=CARTESIAN_POINT('Ctrl Pts',(-0.39383935274689,2.1001849047854,7.93371652149347));
#27711=CARTESIAN_POINT('',(-0.393299840076811,2.09964532330949,7.8087163522035));
#27712=CARTESIAN_POINT('Ctrl Pts',(-0.39329995507651,2.10018798089025,7.93371635220349));
#27713=CARTESIAN_POINT('Ctrl Pts',(-0.393294878776239,2.11080878742979,
7.93317630756182));
#27714=CARTESIAN_POINT('Ctrl Pts',(-0.392859630695457,2.12141894325366,
7.93263626292015));
#27715=CARTESIAN_POINT('Ctrl Pts',(-0.391996546742083,2.13199370785455,
7.93209621827848));
#27716=CARTESIAN_POINT('Ctrl Pts',(-0.390328115394942,2.15243583133485,
7.93105225563092));
#27717=CARTESIAN_POINT('Ctrl Pts',(-0.387051361388753,2.17280800210539,
7.93000829298337));
#27718=CARTESIAN_POINT('Ctrl Pts',(-0.382185829458229,2.19283793277171,
7.92896433033582));
#27719=CARTESIAN_POINT('Ctrl Pts',(-0.377329248197983,2.21283101622223,
7.92792228817005));
#27720=CARTESIAN_POINT('Ctrl Pts',(-0.370889804441221,2.2324823883258,7.92688024600428));
#27721=CARTESIAN_POINT('Ctrl Pts',(-0.362938436792736,2.25152749287982,
7.92583820383852));
#27722=CARTESIAN_POINT('Ctrl Pts',(-0.354995608788193,2.27055214329075,
7.92479728080966));
#27723=CARTESIAN_POINT('Ctrl Pts',(-0.345544335837312,2.28897113210632,
7.92375635778081));
#27724=CARTESIAN_POINT('Ctrl Pts',(-0.334704457659796,2.30653768668856,
7.92271543475196));
#27725=CARTESIAN_POINT('Ctrl Pts',(-0.32385901240337,2.32411326299539,7.92167397713217));
#27726=CARTESIAN_POINT('Ctrl Pts',(-0.311623909871164,2.34083489584196,
7.92063251951238));
#27727=CARTESIAN_POINT('Ctrl Pts',(-0.298163827078626,2.35648240138814,
7.91959106189259));
#27728=CARTESIAN_POINT('Ctrl Pts',(-0.284699631643985,2.37213468792944,
7.91854928606209));
#27729=CARTESIAN_POINT('Ctrl Pts',(-0.270010217683464,2.38671166008147,
7.9175075102316));
#27730=CARTESIAN_POINT('Ctrl Pts',(-0.254298414321334,2.40002867608556,
7.9164657344011));
#27731=CARTESIAN_POINT('Ctrl Pts',(-0.23855264953969,2.41337447712195,7.9154217067485));
#27732=CARTESIAN_POINT('Ctrl Pts',(-0.221780680970103,2.4254544544029,7.91437767909591));
#27733=CARTESIAN_POINT('Ctrl Pts',(-0.204216383250429,2.43612580801259,
7.91333365144331));
#27734=CARTESIAN_POINT('Ctrl Pts',(-0.198004121375393,2.43990012590691,
7.91296439254744));
#27735=CARTESIAN_POINT('Ctrl Pts',(-0.191692969636716,2.44349865308767,
7.91259513365157));
#27736=CARTESIAN_POINT('Ctrl Pts',(-0.185293931287982,2.44691648710871,
7.9122258747557));
#27737=CARTESIAN_POINT('Ctrl Pts',(-0.16720267582725,2.45657933096543,7.91118191210815));
#27738=CARTESIAN_POINT('Ctrl Pts',(-0.148299623741452,2.46485200166864,
7.9101379494606));
#27739=CARTESIAN_POINT('Ctrl Pts',(-0.128824299065037,2.47160353869467,
7.90909398681304));
#27740=CARTESIAN_POINT('Ctrl Pts',(-0.109384801346949,2.47834265554083,
7.90805194464727));
#27741=CARTESIAN_POINT('Ctrl Pts',(-0.0893757885776367,2.4835658987333,
7.9070099024815));
#27742=CARTESIAN_POINT('Ctrl Pts',(-0.0690581046975076,2.48718970566841,
7.90596786031573));
#27743=CARTESIAN_POINT('Ctrl Pts',(-0.048762241690685,2.4908096206918,7.90492693728688));
#27744=CARTESIAN_POINT('Ctrl Pts',(-0.028159081291911,2.49283335263135,
7.90388601425803));
#27745=CARTESIAN_POINT('Ctrl Pts',(-0.00752098575915269,2.49322808238122,
7.90284509122917));
#27746=CARTESIAN_POINT('Ctrl Pts',(0.0131277089615774,2.49362301485399,
7.90180363360938));
#27747=CARTESIAN_POINT('Ctrl Pts',(0.0338106393244828,2.49238724358352,
7.90076217598959));
#27748=CARTESIAN_POINT('Ctrl Pts',(0.0542535281705359,2.48954004246168,
7.8997207183698));
#27749=CARTESIAN_POINT('Ctrl Pts',(0.0747026632103695,2.48669197139578,
7.8986789425393));
#27750=CARTESIAN_POINT('Ctrl Pts',(0.0949108875852173,2.48223162754792,
7.8976371667088));
#27751=CARTESIAN_POINT('Ctrl Pts',(0.114613156128634,2.47622960335709,7.8965953908783));
#27752=CARTESIAN_POINT('Ctrl Pts',(0.134358011572604,2.47021460565477,7.8955513632257));
#27753=CARTESIAN_POINT('Ctrl Pts',(0.153594042391942,2.4626515441632,7.89450733557311));
#27754=CARTESIAN_POINT('Ctrl Pts',(0.172074579293369,2.4536597646906,7.89346330792051));
#27755=CARTESIAN_POINT('Ctrl Pts',(0.178610902957094,2.45047949015316,7.89309404902464));
#27756=CARTESIAN_POINT('Ctrl Pts',(0.185052949511451,2.44712090855824,7.89272479012878));
#27757=CARTESIAN_POINT('Ctrl Pts',(0.191390640631951,2.44359061785574,7.89235553123291));
#27758=CARTESIAN_POINT('Ctrl Pts',(0.209308456223094,2.43360983832772,7.89131156858535));
#27759=CARTESIAN_POINT('Ctrl Pts',(0.226496829517949,2.4221939598158,7.8902676059378));
#27760=CARTESIAN_POINT('Ctrl Pts',(0.242715987875687,2.4094734871189,7.88922364329025));
#27761=CARTESIAN_POINT('Ctrl Pts',(0.258905309343913,2.39677641510223,7.88818160112448));
#27762=CARTESIAN_POINT('Ctrl Pts',(0.274128345891043,2.38277991483484,7.88713955895871));
#27763=CARTESIAN_POINT('Ctrl Pts',(0.288173637045684,2.36765807462481,7.88609751679294));
#27764=CARTESIAN_POINT('Ctrl Pts',(0.30220384377827,2.35255247503362,7.88505659376408));
#27765=CARTESIAN_POINT('Ctrl Pts',(0.315058296826067,2.33632445154883,7.88401567073523));
#27766=CARTESIAN_POINT('Ctrl Pts',(0.326561966685752,2.3191852456584,7.88297474770638));
#27767=CARTESIAN_POINT('Ctrl Pts',(0.338071544530455,2.30203723751854,7.88193329008658));
#27768=CARTESIAN_POINT('Ctrl Pts',(0.348228529842791,2.28397771403659,7.88089183246679));
#27769=CARTESIAN_POINT('Ctrl Pts',(0.3569006572741,2.26524772566458,7.879850374847));
#27770=CARTESIAN_POINT('Ctrl Pts',(0.365575434418412,2.24651201446456,7.8788085990165));
#27771=CARTESIAN_POINT('Ctrl Pts',(0.37276417444497,2.22710611287623,7.877766823186));
#27772=CARTESIAN_POINT('Ctrl Pts',(0.378382759002726,2.20729108858375,7.87672504735551));
#27773=CARTESIAN_POINT('Ctrl Pts',(0.384013488258505,2.1874332336666,7.87568101970291));
#27774=CARTESIAN_POINT('Ctrl Pts',(0.388067141799957,2.16716521270317,7.87463699205031));
#27775=CARTESIAN_POINT('Ctrl Pts',(0.390510541173974,2.14675903369415,7.87359296439771));
#27776=CARTESIAN_POINT('Ctrl Pts',(0.391374739505084,2.13954163565784,7.87322370550185));
#27777=CARTESIAN_POINT('Ctrl Pts',(0.392037980166997,2.13230698667105,7.87285444660598));
#27778=CARTESIAN_POINT('Ctrl Pts',(0.392500355254997,2.12506713235895,7.87248518771012));
#27779=CARTESIAN_POINT('Ctrl Pts',(0.393807574461998,2.10459873590271,7.87144122506257));
#27780=CARTESIAN_POINT('Ctrl Pts',(0.393513276453599,2.08396682257882,7.87039726241501));
#27781=CARTESIAN_POINT('Ctrl Pts',(0.391597398738457,2.06344364212242,7.86935329976746));
#27782=CARTESIAN_POINT('Ctrl Pts',(0.389685045486819,2.04295821626795,7.86831125760169));
#27783=CARTESIAN_POINT('Ctrl Pts',(0.386157042209058,2.02258185608459,7.86726921543592));
#27784=CARTESIAN_POINT('Ctrl Pts',(0.381045298097555,2.00258659846948,7.86622717327015));
#27785=CARTESIAN_POINT('Ctrl Pts',(0.375939043918924,1.98261281544694,7.8651862502413));
#27786=CARTESIAN_POINT('Ctrl Pts',(0.369252578920146,1.96302003883919,7.86414532721244));
#27787=CARTESIAN_POINT('Ctrl Pts',(0.361068772093729,1.94406978542076,7.86310440418359));
#27788=CARTESIAN_POINT('Ctrl Pts',(0.352880762277423,1.92510979964608,7.8620629465638));
#27789=CARTESIAN_POINT('Ctrl Pts',(0.34319415126381,1.90679367816525,7.86102148894401));
#27790=CARTESIAN_POINT('Ctrl Pts',(0.332140020965691,1.88936311701672,7.85998003132421));
#27791=CARTESIAN_POINT('Ctrl Pts',(0.321082513148847,1.87192723007186,7.85893825549372));
#27792=CARTESIAN_POINT('Ctrl Pts',(0.308657078511336,1.85537804357542,7.85789647966322));
#27793=CARTESIAN_POINT('Ctrl Pts',(0.295037692652914,1.83992760639767,7.85685470383272));
#27794=CARTESIAN_POINT('Ctrl Pts',(0.281388868182896,1.82444377274935,7.85581067618012));
#27795=CARTESIAN_POINT('Ctrl Pts',(0.266541469177281,1.81006394230613,7.85476664852753));
#27796=CARTESIAN_POINT('Ctrl Pts',(0.25070624473702,1.79696325495105,7.85372262087493));
#27797=CARTESIAN_POINT('Ctrl Pts',(0.245105533416708,1.79232971355413,7.85335336197906));
#27798=CARTESIAN_POINT('Ctrl Pts',(0.23938153517094,1.78785580271229,7.8529841030832));
#27799=CARTESIAN_POINT('Ctrl Pts',(0.233544428029886,1.78354796550473,7.85261484418733));
#27800=CARTESIAN_POINT('Ctrl Pts',(0.217041855192152,1.77136891934832,7.85157088153978));
#27801=CARTESIAN_POINT('Ctrl Pts',(0.199534864238156,1.76044794290577,7.85052691889222));
#27802=CARTESIAN_POINT('Ctrl Pts',(0.181241507430582,1.75094927877987,7.84948295624467));
#27803=CARTESIAN_POINT('Ctrl Pts',(0.162981803224076,1.74146808847018,7.8484409140789));
#27804=CARTESIAN_POINT('Ctrl Pts',(0.143939222834498,1.73340440484813,7.84739887191313));
#27805=CARTESIAN_POINT('Ctrl Pts',(0.124359772778037,1.72687865658127,7.84635682974736));
#27806=CARTESIAN_POINT('Ctrl Pts',(0.104801350743349,1.72035991686554,7.84531590671851));
#27807=CARTESIAN_POINT('Ctrl Pts',(0.0847078890543636,1.71537609235677,
7.84427498368965));
#27808=CARTESIAN_POINT('Ctrl Pts',(0.064344134180387,1.71199906907769,7.8432340606608));
#27809=CARTESIAN_POINT('Ctrl Pts',(0.0439699210126507,1.70862031144748,
7.84219260304101));
#27810=CARTESIAN_POINT('Ctrl Pts',(0.023325860565065,1.70685013991164,7.84115114542122));
#27811=CARTESIAN_POINT('Ctrl Pts',(0.00268613220208843,1.70670917288374,
7.84010968780142));
#27812=CARTESIAN_POINT('Ctrl Pts',(-0.0179599024977188,1.70656816278427,
7.83906791197093));
#27813=CARTESIAN_POINT('Ctrl Pts',(-0.0386008670895658,1.70805731702189,
7.83802613614043));
#27814=CARTESIAN_POINT('Ctrl Pts',(-0.0589642909510291,1.71114513968237,
7.83698436030993));
#27815=CARTESIAN_POINT('Ctrl Pts',(-0.0793717308152733,1.7142396367416,
7.83594033265733));
#27816=CARTESIAN_POINT('Ctrl Pts',(-0.0994997150711637,1.71893953361309,
7.83489630500474));
#27817=CARTESIAN_POINT('Ctrl Pts',(-0.119086900672914,1.72516243506271,
7.83385227735214));
#27818=CARTESIAN_POINT('Ctrl Pts',(-0.126014631476254,1.72736339373718,
7.83348301845627));
#27819=CARTESIAN_POINT('Ctrl Pts',(-0.132874879491201,1.72975442516975,
7.83311375956041));
#27820=CARTESIAN_POINT('Ctrl Pts',(-0.139656717709764,1.73233045924562,
7.83274450066454));
#27821=CARTESIAN_POINT('Ctrl Pts',(-0.158830218636052,1.73961338021013,
7.83170053801699));
#27822=CARTESIAN_POINT('Ctrl Pts',(-0.177489621696974,1.74842184977827,
7.83065657536943));
#27823=CARTESIAN_POINT('Ctrl Pts',(-0.195378793141691,1.75866143319206,
7.82961261272188));
#27824=CARTESIAN_POINT('Ctrl Pts',(-0.213235055527869,1.76888217978879,
7.82857057055611));
#27825=CARTESIAN_POINT('Ctrl Pts',(-0.230323237935067,1.7805285046799,7.82752852839034));
#27826=CARTESIAN_POINT('Ctrl Pts',(-0.246408914011127,1.79345875139574,
7.82648648622457));
#27827=CARTESIAN_POINT('Ctrl Pts',(-0.262477314323779,1.80637511122974,
7.82544556319571));
#27828=CARTESIAN_POINT('Ctrl Pts',(-0.277544757081132,1.82057221932032,
7.82440464016686));
#27829=CARTESIAN_POINT('Ctrl Pts',(-0.291407487180691,1.83586638529896,
7.823363717138));
#27830=CARTESIAN_POINT('Ctrl Pts',(-0.30527733681712,1.85116840596264,7.82232225951821));
#27831=CARTESIAN_POINT('Ctrl Pts',(-0.317940731673067,1.86756807576885,
7.82128080189842));
#27832=CARTESIAN_POINT('Ctrl Pts',(-0.329231917173156,1.88484602091877,
7.82023934427863));
#27833=CARTESIAN_POINT('Ctrl Pts',(-0.340526552622667,1.90212924523418,
7.81919756844813));
#27834=CARTESIAN_POINT('Ctrl Pts',(-0.350447772169409,1.92029064392291,
7.81815579261763));
#27835=CARTESIAN_POINT('Ctrl Pts',(-0.35887456487084,1.93908406949974,7.81711401678713));
#27836=CARTESIAN_POINT('Ctrl Pts',(-0.367319572275924,1.95791811749243,
7.81606998913453));
#27837=CARTESIAN_POINT('Ctrl Pts',(-0.37426345640492,1.97738622613225,7.81502596148194));
#27838=CARTESIAN_POINT('Ctrl Pts',(-0.379634026933072,1.99722405147808,
7.81398193382934));
#27839=CARTESIAN_POINT('Ctrl Pts',(-0.381533527332743,2.0042404302735,7.81361267493348));
#27840=CARTESIAN_POINT('Ctrl Pts',(-0.383236681501575,2.01130295815055,
7.81324341603761));
#27841=CARTESIAN_POINT('Ctrl Pts',(-0.384741837496011,2.01839970294053,
7.81287415714175));
#27842=CARTESIAN_POINT('Ctrl Pts',(-0.390391121414536,2.04503582993608,
7.81148822216234));
#27843=CARTESIAN_POINT('Ctrl Pts',(-0.393275160366044,2.07227807150579,
7.81010228718292));
#27844=CARTESIAN_POINT('Ctrl Pts',(-0.393299840076811,2.09964532330949,
7.8087163522035));
#27845=CARTESIAN_POINT('',(-0.392652606621955,2.10000006244036,7.6837163522035));
#27846=CARTESIAN_POINT('Ctrl Pts',(-0.39339560660603,2.09964617938564,7.80871630448812));
#27847=CARTESIAN_POINT('Ctrl Pts',(-0.392436633507189,2.20309412285361,
7.80347880753172));
#27848=CARTESIAN_POINT('Ctrl Pts',(-0.297548046247412,2.43892015636596,
7.79161786273442));
#27849=CARTESIAN_POINT('Ctrl Pts',(0.100487270537579,2.55406754116476,7.77313347009617));
#27850=CARTESIAN_POINT('Ctrl Pts',(0.436183693642714,2.26130346828162,7.75326312657338));
#27851=CARTESIAN_POINT('Ctrl Pts',(0.371740958878468,1.82056542273442,7.73339278305059));
#27852=CARTESIAN_POINT('Ctrl Pts',(-0.0337234976950709,1.63617056024581,
7.7135224395278));
#27853=CARTESIAN_POINT('Ctrl Pts',(-0.345833540474424,1.83709412712005,
7.69696362924544));
#27854=CARTESIAN_POINT('Ctrl Pts',(-0.392652513771598,2.03427171757279,
7.687028266804));
#27855=CARTESIAN_POINT('Ctrl Pts',(-0.392652606621955,2.10000006244036,
7.6837163522035));
#27856=CARTESIAN_POINT('',(-0.393299840100549,2.10035465036696,7.5587163522035));
#27857=CARTESIAN_POINT('Ctrl Pts',(-0.392652606621955,2.10000006244036,
7.6837163522035));
#27858=CARTESIAN_POINT('Ctrl Pts',(-0.392652699461621,2.16572083882566,
7.68040481896307));
#27859=CARTESIAN_POINT('Ctrl Pts',(-0.345841471197197,2.36289061215051,
7.67046983788174));
#27860=CARTESIAN_POINT('Ctrl Pts',(-0.0337501714246444,2.56382749962499,
7.65391140895943));
#27861=CARTESIAN_POINT('Ctrl Pts',(0.371724888611281,2.37945595478788,7.63404106543665));
#27862=CARTESIAN_POINT('Ctrl Pts',(0.436192969120214,1.93872161592588,7.61417072191384));
#27863=CARTESIAN_POINT('Ctrl Pts',(0.100513382771949,1.64593823838246,7.59430037839108));
#27864=CARTESIAN_POINT('Ctrl Pts',(-0.297536766592373,1.76106510782775,
7.57581560443067));
#27865=CARTESIAN_POINT('Ctrl Pts',(-0.392436806074336,1.99689847231397,
7.56395427831121));
#27866=CARTESIAN_POINT('Ctrl Pts',(-0.393395836408773,2.10035379224535,
7.55871640003268));
#27867=CARTESIAN_POINT('',(-0.393495500114951,2.09981301717212,7.43371629079915));
#27868=CARTESIAN_POINT('Ctrl Pts',(-0.393299840100549,2.10035465036696,
7.5587163522035));
#27869=CARTESIAN_POINT('Ctrl Pts',(-0.393275169063348,2.12771431467307,
7.55733079858416));
#27870=CARTESIAN_POINT('Ctrl Pts',(-0.390392727573699,2.15494904886535,
7.55594524496482));
#27871=CARTESIAN_POINT('Ctrl Pts',(-0.384746529508904,2.18157817128898,
7.55455969134548));
#27872=CARTESIAN_POINT('Ctrl Pts',(-0.380492331188422,2.20164221555212,
7.55351572869793));
#27873=CARTESIAN_POINT('Ctrl Pts',(-0.37465175991358,2.22143236931363,7.55247176605038));
#27874=CARTESIAN_POINT('Ctrl Pts',(-0.36727882436407,2.2406810405625,7.55142780340283));
#27875=CARTESIAN_POINT('Ctrl Pts',(-0.359919452123981,2.25989430180644,
7.55038576123706));
#27876=CARTESIAN_POINT('Ctrl Pts',(-0.351033515787082,2.27856735717682,
7.54934371907129));
#27877=CARTESIAN_POINT('Ctrl Pts',(-0.340725017678054,2.29644681806609,
7.54830167690552));
#27878=CARTESIAN_POINT('Ctrl Pts',(-0.330427590734058,2.31430707669522,
7.54726075387667));
#27879=CARTESIAN_POINT('Ctrl Pts',(-0.318710975674559,2.33137478424272,
7.54621983084782));
#27880=CARTESIAN_POINT('Ctrl Pts',(-0.305725417742669,2.34742040931595,
7.54517890781897));
#27881=CARTESIAN_POINT('Ctrl Pts',(-0.292733190766667,2.36347427500402,
7.54413745019918));
#27882=CARTESIAN_POINT('Ctrl Pts',(-0.27847116931383,2.37850442746855,7.54309599257939));
#27883=CARTESIAN_POINT('Ctrl Pts',(-0.263130691087117,2.39231340955901,
7.5420545349596));
#27884=CARTESIAN_POINT('Ctrl Pts',(-0.247785525675512,2.40612661089553,
7.54101275912911));
#27885=CARTESIAN_POINT('Ctrl Pts',(-0.2313618181023,2.41871743410824,7.53997098329861));
#27886=CARTESIAN_POINT('Ctrl Pts',(-0.214084229156525,2.42992852684552,
7.53892920746812));
#27887=CARTESIAN_POINT('Ctrl Pts',(-0.19676929431017,2.44116385261416,7.53788517981552));
#27888=CARTESIAN_POINT('Ctrl Pts',(-0.17859744075984,2.45101314291104,7.53684115216293));
#27889=CARTESIAN_POINT('Ctrl Pts',(-0.159818802426733,2.45936449517292,
7.53579712451033));
#27890=CARTESIAN_POINT('Ctrl Pts',(-0.153177044193876,2.46231825900057,
7.53542786561446));
#27891=CARTESIAN_POINT('Ctrl Pts',(-0.146459551390773,2.46508508472355,
7.53505860671858));
#27892=CARTESIAN_POINT('Ctrl Pts',(-0.139677861325145,2.46766150880346,
7.5346893478227));
#27893=CARTESIAN_POINT('Ctrl Pts',(-0.120504779254941,2.47494553238072,
7.53364538517515));
#27894=CARTESIAN_POINT('Ctrl Pts',(-0.100703256878215,2.4807474432975,7.5326014225276));
#27895=CARTESIAN_POINT('Ctrl Pts',(-0.080527526223084,2.48496780062804,
7.53155745988004));
#27896=CARTESIAN_POINT('Ctrl Pts',(-0.0603889109985461,2.4891803941565,
7.53051541771427));
#27897=CARTESIAN_POINT('Ctrl Pts',(-0.0398781538156886,2.4918170020599,
7.5294733755485));
#27898=CARTESIAN_POINT('Ctrl Pts',(-0.0192646066900649,2.49282790752323,
7.52843133338273));
#27899=CARTESIAN_POINT('Ctrl Pts',(0.00132680180977449,2.49383772728997,
7.52739041035388));
#27900=CARTESIAN_POINT('Ctrl Pts',(0.0220200513400488,2.49322524605851,
7.52634948732502));
#27901=CARTESIAN_POINT('Ctrl Pts',(0.0425408173313714,2.49099254322912,
7.52530856429617));
#27902=CARTESIAN_POINT('Ctrl Pts',(0.0630721222532712,2.48875869374176,
7.52426710667638));
#27903=CARTESIAN_POINT('Ctrl Pts',(0.0834300334619058,2.48490302385815,
7.52322564905659));
#27904=CARTESIAN_POINT('Ctrl Pts',(0.103344950893888,2.47947952662132,7.52218419143679));
#27905=CARTESIAN_POINT('Ctrl Pts',(0.123265953201359,2.47405437226964,7.5211424156063));
#27906=CARTESIAN_POINT('Ctrl Pts',(0.142742992456503,2.46706066499246,7.5201006397758));
#27907=CARTESIAN_POINT('Ctrl Pts',(0.161522151040302,2.45860212593251,7.5190588639453));
#27908=CARTESIAN_POINT('Ctrl Pts',(0.180341901201536,2.45012530354843,7.5180148362927));
#27909=CARTESIAN_POINT('Ctrl Pts',(0.19846011349999,2.4401776825305,7.5169708086401));
#27910=CARTESIAN_POINT('Ctrl Pts',(0.215647296245783,2.42890900507874,7.51592678098751));
#27911=CARTESIAN_POINT('Ctrl Pts',(0.221726177497598,2.4249234215711,7.51555752209164));
#27912=CARTESIAN_POINT('Ctrl Pts',(0.227688874335315,2.42077296610703,7.51518826319577));
#27913=CARTESIAN_POINT('Ctrl Pts',(0.233526229200695,2.41646546458548,7.51481900429991));
#27914=CARTESIAN_POINT('Ctrl Pts',(0.250029502400629,2.40428736747496,7.51377504165236));
#27915=CARTESIAN_POINT('Ctrl Pts',(0.265626774832429,2.39077857213967,7.5127310790048));
#27916=CARTESIAN_POINT('Ctrl Pts',(0.280096814394786,2.37609901225085,7.51168711635725));
#27917=CARTESIAN_POINT('Ctrl Pts',(0.294540234760133,2.36144645699424,7.51064507419148));
#27918=CARTESIAN_POINT('Ctrl Pts',(0.307859985361099,2.34562788862102,7.50960303202571));
#27919=CARTESIAN_POINT('Ctrl Pts',(0.319868458296564,2.32884287051813,7.50856098985994));
#27920=CARTESIAN_POINT('Ctrl Pts',(0.331864034320745,2.312075879261,7.50752006683109));
#27921=CARTESIAN_POINT('Ctrl Pts',(0.342550679009269,2.29434507739864,7.50647914380223));
#27922=CARTESIAN_POINT('Ctrl Pts',(0.351781643912968,2.27588224755754,7.50543822077338));
#27923=CARTESIAN_POINT('Ctrl Pts',(0.361017349599651,2.25740993568823,7.50439676315359));
#27924=CARTESIAN_POINT('Ctrl Pts',(0.368795538509466,2.23820549567262,7.50335530553379));
#27925=CARTESIAN_POINT('Ctrl Pts',(0.375015669574018,2.21852483948081,7.502313847914));
#27926=CARTESIAN_POINT('Ctrl Pts',(0.381237701159786,2.19883816999052,7.5012720720835));
#27927=CARTESIAN_POINT('Ctrl Pts',(0.38590054013969,2.17867570654299,7.50023029625301));
#27928=CARTESIAN_POINT('Ctrl Pts',(0.388953946912425,2.15830709374721,7.49918852042251));
#27929=CARTESIAN_POINT('Ctrl Pts',(0.39201395369319,2.13789445373265,7.49814449276991));
#27930=CARTESIAN_POINT('Ctrl Pts',(0.393457531527764,2.11727550943757,7.49710046511731));
#27931=CARTESIAN_POINT('Ctrl Pts',(0.393286358340577,2.09672427974226,7.49605643746472));
#27932=CARTESIAN_POINT('Ctrl Pts',(0.393225816627965,2.08945557917951,7.49568717856885));
#27933=CARTESIAN_POINT('Ctrl Pts',(0.392963754899772,2.08219532038326,7.49531791967299));
#27934=CARTESIAN_POINT('Ctrl Pts',(0.392501796160234,2.07495543949297,7.49494866077712));
#27935=CARTESIAN_POINT('Ctrl Pts',(0.391195754046726,2.05448696789535,7.49390469812957));
#27936=CARTESIAN_POINT('Ctrl Pts',(0.388280402454325,2.03405994697172,7.49286073548201));
#27937=CARTESIAN_POINT('Ctrl Pts',(0.38377045954345,2.01394696761991,7.49181677283446));
#27938=CARTESIAN_POINT('Ctrl Pts',(0.379268813158532,1.99387098826091,7.49077473066869));
#27939=CARTESIAN_POINT('Ctrl Pts',(0.373178499321527,1.97410862658987,7.48973268850292));
#27940=CARTESIAN_POINT('Ctrl Pts',(0.365565758954518,1.9549256539563,7.48869064633715));
#27941=CARTESIAN_POINT('Ctrl Pts',(0.357961194551069,1.93576328353398,7.4876497233083));
#27942=CARTESIAN_POINT('Ctrl Pts',(0.348837692751426,1.91717975791872,7.48660880027944));
#27943=CARTESIAN_POINT('Ctrl Pts',(0.338310702950755,1.8994239339578,7.48556787725059));
#27944=CARTESIAN_POINT('Ctrl Pts',(0.327778306762491,1.88165899106846,7.4845264196308));
#27945=CARTESIAN_POINT('Ctrl Pts',(0.31584134395354,1.86472324018675,7.48348496201101));
#27946=CARTESIAN_POINT('Ctrl Pts',(0.302660565193323,1.84883974781654,7.48244350439121));
#27947=CARTESIAN_POINT('Ctrl Pts',(0.289475759130561,1.83295140234695,7.48140172856072));
#27948=CARTESIAN_POINT('Ctrl Pts',(0.275046877859373,1.81811649807065,7.48035995273022));
#27949=CARTESIAN_POINT('Ctrl Pts',(0.259573447790861,1.80452324084293,7.47931817689972));
#27950=CARTESIAN_POINT('Ctrl Pts',(0.244066571552117,1.79090060148124,7.47827414924712));
#27951=CARTESIAN_POINT('Ctrl Pts',(0.227511228784971,1.77852540828395,7.47723012159453));
#27952=CARTESIAN_POINT('Ctrl Pts',(0.210138727760929,1.76754458179326,7.47618609394193));
#27953=CARTESIAN_POINT('Ctrl Pts',(0.203994301863178,1.76366080739747,7.47581683504606));
#27954=CARTESIAN_POINT('Ctrl Pts',(0.197747887528184,1.75995104431961,7.4754475761502));
#27955=CARTESIAN_POINT('Ctrl Pts',(0.191410399437225,1.75642038915663,7.47507831725433));
#27956=CARTESIAN_POINT('Ctrl Pts',(0.173493157847841,1.74643857923194,7.47403435460678));
#27957=CARTESIAN_POINT('Ctrl Pts',(0.154739620427987,1.73783234352959,7.47299039195922));
#27958=CARTESIAN_POINT('Ctrl Pts',(0.135386953691321,1.73073686513519,7.47194642931167));
#27959=CARTESIAN_POINT('Ctrl Pts',(0.116069888270487,1.72365443963789,7.4709043871459));
#27960=CARTESIAN_POINT('Ctrl Pts',(0.0961565438196057,1.71807756109961,
7.46986234498013));
#27961=CARTESIAN_POINT('Ctrl Pts',(0.0759062430558385,1.71409439980074,
7.46882030281436));
#27962=CARTESIAN_POINT('Ctrl Pts',(0.0556776907969656,1.71011551635454,
7.46777937978551));
#27963=CARTESIAN_POINT('Ctrl Pts',(0.0351136133577157,1.70772712181982,
7.46673845675665));
#27964=CARTESIAN_POINT('Ctrl Pts',(0.014485748874539,1.70696685498607,7.4656975337278));
#27965=CARTESIAN_POINT('Ctrl Pts',(-0.00615270954220543,1.70620619769908,
7.46465607610801));
#27966=CARTESIAN_POINT('Ctrl Pts',(-0.0268542857634539,1.70707538179094,
7.46361461848822));
#27967=CARTESIAN_POINT('Ctrl Pts',(-0.0473444042369372,1.70955999514977,
7.46257316086843));
#27968=CARTESIAN_POINT('Ctrl Pts',(-0.0678407833349112,1.7120453676663,
7.46153138503793));
#27969=CARTESIAN_POINT('Ctrl Pts',(-0.0881248506056897,1.71614702764487,
7.46048960920743));
#27970=CARTESIAN_POINT('Ctrl Pts',(-0.107930351944881,1.72179908893677,
7.45944783337693));
#27971=CARTESIAN_POINT('Ctrl Pts',(-0.127778663324661,1.72746336728742,
7.45840380572433));
#27972=CARTESIAN_POINT('Ctrl Pts',(-0.147145653511074,1.73468448021601,
7.45735977807174));
#27973=CARTESIAN_POINT('Ctrl Pts',(-0.165782577734869,1.7433474703306,7.45631575041914));
#27974=CARTESIAN_POINT('Ctrl Pts',(-0.172374213544621,1.74641145638179,
7.45594649152327));
#27975=CARTESIAN_POINT('Ctrl Pts',(-0.178874745706579,1.74965539160765,
7.45557723262741));
#27976=CARTESIAN_POINT('Ctrl Pts',(-0.185273980596595,1.75307285762873,
7.45520797373154));
#27977=CARTESIAN_POINT('Ctrl Pts',(-0.203365791715768,1.76273466108216,
7.45416401108399));
#27978=CARTESIAN_POINT('Ctrl Pts',(-0.220753697443928,1.77384426022481,
7.45312004843643));
#27979=CARTESIAN_POINT('Ctrl Pts',(-0.237195650903155,1.78627541825252,
7.45207608578888));
#27980=CARTESIAN_POINT('Ctrl Pts',(-0.253607357617271,1.79868370782551,
7.45103404362311));
#27981=CARTESIAN_POINT('Ctrl Pts',(-0.269075950105387,1.8124083392554,7.44999200145734));
#27982=CARTESIAN_POINT('Ctrl Pts',(-0.283386917144658,1.82727899752449,
7.44894995929157));
#27983=CARTESIAN_POINT('Ctrl Pts',(-0.29768251443015,1.84213368494022,7.44790903626272));
#27984=CARTESIAN_POINT('Ctrl Pts',(-0.310822426004836,1.85813144832107,
7.44686811323387));
#27985=CARTESIAN_POINT('Ctrl Pts',(-0.322627907737369,1.87506417993346,
7.44582719020501));
#27986=CARTESIAN_POINT('Ctrl Pts',(-0.334439452457633,1.89200560775548,
7.44478573258522));
#27987=CARTESIAN_POINT('Ctrl Pts',(-0.3449147641733,1.90988236874536,7.44374427496543));
#27988=CARTESIAN_POINT('Ctrl Pts',(-0.353917328138373,1.92845579332605,
7.44270281734564));
#27989=CARTESIAN_POINT('Ctrl Pts',(-0.362922642779217,1.94703489289769,
7.44166104151514));
#27990=CARTESIAN_POINT('Ctrl Pts',(-0.370454025755053,1.96631040249137,
7.44061926568465));
#27991=CARTESIAN_POINT('Ctrl Pts',(-0.376422747161753,1.98602278552623,
7.43957748985415));
#27992=CARTESIAN_POINT('Ctrl Pts',(-0.38240437009522,2.00577777732435,7.43853346220155));
#27993=CARTESIAN_POINT('Ctrl Pts',(-0.386816430782504,2.02597080833257,
7.43748943454896));
#27994=CARTESIAN_POINT('Ctrl Pts',(-0.389620937418854,2.0463305009819,7.43644540689636));
#27995=CARTESIAN_POINT('Ctrl Pts',(-0.390612854655356,2.05353145740219,
7.43607614800049));
#27996=CARTESIAN_POINT('Ctrl Pts',(-0.391404151353232,2.06075322198397,
7.43570688910462));
#27997=CARTESIAN_POINT('Ctrl Pts',(-0.391994706207888,2.0679837493608,7.43533763020876));
#27998=CARTESIAN_POINT('Ctrl Pts',(-0.392859008198951,2.07856593179309,
7.434797204207));
#27999=CARTESIAN_POINT('Ctrl Pts',(-0.393294871948269,2.08918358074563,
7.43425677820525));
#28000=CARTESIAN_POINT('Ctrl Pts',(-0.393299955020244,2.09981190142455,
7.4337163522035));
#28001=CARTESIAN_POINT('',(-0.393134823968354,2.09974753055899,7.30871640423617));
#28002=CARTESIAN_POINT('Ctrl Pts',(-0.393839208888362,2.09981497831685,
7.433716182869));
#28003=CARTESIAN_POINT('Ctrl Pts',(-0.393130725605086,2.21961039447394,
7.42763321747465));
#28004=CARTESIAN_POINT('Ctrl Pts',(-0.270765457358387,2.47109464075752,
7.41492680423937));
#28005=CARTESIAN_POINT('Ctrl Pts',(0.157408377376609,2.537604417495,7.39559694316317));
#28006=CARTESIAN_POINT('Ctrl Pts',(0.453153628130196,2.20453139620186,7.3757265996404));
#28007=CARTESIAN_POINT('Ctrl Pts',(0.333192116370157,1.77556504955804,7.35585625611758));
#28008=CARTESIAN_POINT('Ctrl Pts',(-0.0924278021488653,1.64422360211459,
7.33598591259482));
#28009=CARTESIAN_POINT('Ctrl Pts',(-0.361952445184268,1.87099925901134,
7.32027266154399));
#28010=CARTESIAN_POINT('Ctrl Pts',(-0.393106482257739,2.05085104044711,
7.3111828583341));
#28011=CARTESIAN_POINT('Ctrl Pts',(-0.39282156461649,2.09974577364633,7.30871650296516));
#28012=CARTESIAN_POINT('',(-0.393299884474588,2.10030145028756,7.18371635219909));
#28013=CARTESIAN_POINT('Ctrl Pts',(-0.393299919559953,2.09974845649634,
7.3087163522035));
#28014=CARTESIAN_POINT('Ctrl Pts',(-0.393313234865234,2.12056755307232,
7.30766746530676));
#28015=CARTESIAN_POINT('Ctrl Pts',(-0.391669130710796,2.14139400732832,
7.30661857841001));
#28016=CARTESIAN_POINT('Ctrl Pts',(-0.388390445533041,2.16194959094817,
7.30556969151327));
#28017=CARTESIAN_POINT('Ctrl Pts',(-0.385111255528112,2.1825083395615,7.30452064311685));
#28018=CARTESIAN_POINT('Ctrl Pts',(-0.380197122193991,2.2027954253499,7.30347159472042));
#28019=CARTESIAN_POINT('Ctrl Pts',(-0.37372220884026,2.22254224014419,7.302422546324));
#28020=CARTESIAN_POINT('Ctrl Pts',(-0.367229923374881,2.24234203539592,
7.30137068334383));
#28021=CARTESIAN_POINT('Ctrl Pts',(-0.359168748379053,2.26159798513236,
7.30031882036367));
#28022=CARTESIAN_POINT('Ctrl Pts',(-0.349661914960496,2.28005953245013,
7.2992669573835));
#28023=CARTESIAN_POINT('Ctrl Pts',(-0.340558352447886,2.29773795834521,
7.29825971343874));
#28024=CARTESIAN_POINT('Ctrl Pts',(-0.330129824766302,2.3146876375657,7.29725246949399));
#28025=CARTESIAN_POINT('Ctrl Pts',(-0.318521561851313,2.33071390212946,
7.29624522554923));
#28026=CARTESIAN_POINT('Ctrl Pts',(-0.306490124035975,2.34732439819791,
7.29520126290168));
#28027=CARTESIAN_POINT('Ctrl Pts',(-0.293120015089348,2.36304071600702,
7.29415730025412));
#28028=CARTESIAN_POINT('Ctrl Pts',(-0.278569202794085,2.3776402154852,7.29311333760657));
#28029=CARTESIAN_POINT('Ctrl Pts',(-0.264045158285981,2.3922128576109,7.2920712954408));
#28030=CARTESIAN_POINT('Ctrl Pts',(-0.248345193240788,2.405672202284,7.29102925327503));
#28031=CARTESIAN_POINT('Ctrl Pts',(-0.231667201436317,2.41782888128467,
7.28998721110927));
#28032=CARTESIAN_POINT('Ctrl Pts',(-0.215007121533044,2.42997250420307,
7.28894628808041));
#28033=CARTESIAN_POINT('Ctrl Pts',(-0.197371674674546,2.44081578431017,
7.28790536505156));
#28034=CARTESIAN_POINT('Ctrl Pts',(-0.178991334536187,2.45020992584585,
7.28686444202271));
#28035=CARTESIAN_POINT('Ctrl Pts',(-0.16060155473418,2.45960889196778,7.28582298440292));
#28036=CARTESIAN_POINT('Ctrl Pts',(-0.141466765217106,2.46755688348555,
7.28478152678312));
#28037=CARTESIAN_POINT('Ctrl Pts',(-0.121841977349854,2.47395109647583,
7.28374006916333));
#28038=CARTESIAN_POINT('Ctrl Pts',(-0.102211193254336,2.48034726317695,
7.28269829333283));
#28039=CARTESIAN_POINT('Ctrl Pts',(-0.0820908229596269,2.4851885128946,
7.28165651750234));
#28040=CARTESIAN_POINT('Ctrl Pts',(-0.0617500554875966,2.48842221955918,
7.28061474167184));
#28041=CARTESIAN_POINT('Ctrl Pts',(-0.0413653209850891,2.49166291595409,
7.27957071401924));
#28042=CARTESIAN_POINT('Ctrl Pts',(-0.020759972403847,2.49328907420375,
7.27852668636665));
#28043=CARTESIAN_POINT('Ctrl Pts',(-0.000208032736881453,2.49329994498141,
7.27748265871405));
#28044=CARTESIAN_POINT('Ctrl Pts',(0.00706091893365014,2.49330378983298,
7.27711339981818));
#28045=CARTESIAN_POINT('Ctrl Pts',(0.01432321417879,2.49310604779979,7.27674414092231));
#28046=CARTESIAN_POINT('Ctrl Pts',(0.0215669029512129,2.49270823609531,
7.27637488202644));
#28047=CARTESIAN_POINT('Ctrl Pts',(0.0420461401300037,2.49158354941917,
7.27533091937888));
#28048=CARTESIAN_POINT('Ctrl Pts',(0.0624981830902488,2.48884924923919,
7.27428695673133));
#28049=CARTESIAN_POINT('Ctrl Pts',(0.082650321258473,2.48451763860176,7.27324299408378));
#28050=CARTESIAN_POINT('Ctrl Pts',(0.102765387397025,2.48019399642885,7.27220095191801));
#28051=CARTESIAN_POINT('Ctrl Pts',(0.122580920138787,2.47427897118711,7.27115890975224));
#28052=CARTESIAN_POINT('Ctrl Pts',(0.141830571816359,2.46683644706905,7.27011686758647));
#28053=CARTESIAN_POINT('Ctrl Pts',(0.161059549670436,2.45940191610497,7.26907594455761));
#28054=CARTESIAN_POINT('Ctrl Pts',(0.17972315976357,2.45044338008214,7.26803502152876));
#28055=CARTESIAN_POINT('Ctrl Pts',(0.197571532391663,2.44007407955975,7.2669940984999));
#28056=CARTESIAN_POINT('Ctrl Pts',(0.215429071478752,2.42969945363487,7.26595264088011));
#28057=CARTESIAN_POINT('Ctrl Pts',(0.232469892360094,2.41791297143194,7.26491118326032));
#28058=CARTESIAN_POINT('Ctrl Pts',(0.248469513396737,2.40487340145114,7.26386972564053));
#28059=CARTESIAN_POINT('Ctrl Pts',(0.264474023015123,2.39182984731324,7.26282794981003));
#28060=CARTESIAN_POINT('Ctrl Pts',(0.279436152449859,2.3775329356746,7.26178617397953));
#28061=CARTESIAN_POINT('Ctrl Pts',(0.293165935877912,2.36218051804211,7.26074439814903));
#28062=CARTESIAN_POINT('Ctrl Pts',(0.306925396544414,2.34679491581051,7.25970037049644));
#28063=CARTESIAN_POINT('Ctrl Pts',(0.319446747018133,2.33034983864067,7.25865634284384));
#28064=CARTESIAN_POINT('Ctrl Pts',(0.330581023654338,2.31307528434722,7.25761231519124));
#28065=CARTESIAN_POINT('Ctrl Pts',(0.334519071355225,2.30696550092421,7.25724305629538));
#28066=CARTESIAN_POINT('Ctrl Pts',(0.338284017950784,2.30075219171968,7.25687379739951));
#28067=CARTESIAN_POINT('Ctrl Pts',(0.341870670364721,2.29444622584246,7.25650453850364));
#28068=CARTESIAN_POINT('Ctrl Pts',(0.352010794791812,2.2766181033348,7.25546057585609));
#28069=CARTESIAN_POINT('Ctrl Pts',(0.360782806643879,2.2579415333395,7.25441661320854));
#28070=CARTESIAN_POINT('Ctrl Pts',(0.368049427381595,2.23865247565074,7.25337265056098));
#28071=CARTESIAN_POINT('Ctrl Pts',(0.375302680387439,2.21939890226213,7.25233060839521));
#28072=CARTESIAN_POINT('Ctrl Pts',(0.381055727176377,2.19953573750688,7.25128856622944));
#28073=CARTESIAN_POINT('Ctrl Pts',(0.385218103916303,2.17932151294024,7.25024652406368));
#28074=CARTESIAN_POINT('Ctrl Pts',(0.389376010329001,2.15912899813322,7.24920560103482));
#28075=CARTESIAN_POINT('Ctrl Pts',(0.39194646221738,2.13858688318684,7.24816467800597));
#28076=CARTESIAN_POINT('Ctrl Pts',(0.392889415285432,2.11796656218288,7.24712375497712));
#28077=CARTESIAN_POINT('Ctrl Pts',(0.393832852629604,2.09733565111948,7.24608229735732));
#28078=CARTESIAN_POINT('Ctrl Pts',(0.393147071614843,2.07662718803238,7.24504083973753));
#28079=CARTESIAN_POINT('Ctrl Pts',(0.390844051671458,2.05611586536072,7.24399938211774));
#28080=CARTESIAN_POINT('Ctrl Pts',(0.388540328055078,2.03559827558577,7.24295760628724));
#28081=CARTESIAN_POINT('Ctrl Pts',(0.384618499783456,2.01527867267053,7.24191583045675));
#28082=CARTESIAN_POINT('Ctrl Pts',(0.379142092013518,1.99542388387584,7.24087405462625));
#28083=CARTESIAN_POINT('Ctrl Pts',(0.37365384686391,1.97552617850462,7.23983002697365));
#28084=CARTESIAN_POINT('Ctrl Pts',(0.366604564798395,1.95609598542352,7.23878599932106));
#28085=CARTESIAN_POINT('Ctrl Pts',(0.358106995384997,1.937383057905,7.23774197166846));
#28086=CARTESIAN_POINT('Ctrl Pts',(0.355101516467524,1.93076454072614,7.23737271277259));
#28087=CARTESIAN_POINT('Ctrl Pts',(0.35191528846334,1.92423552967978,7.23700345387673));
#28088=CARTESIAN_POINT('Ctrl Pts',(0.348554639207707,1.91780627484245,7.23663419498086));
#28089=CARTESIAN_POINT('Ctrl Pts',(0.33905346717452,1.89962959182434,7.23559023233331));
#28090=CARTESIAN_POINT('Ctrl Pts',(0.328098321245705,1.88214396239898,7.23454626968575));
#28091=CARTESIAN_POINT('Ctrl Pts',(0.315813289287133,1.86559254212026,7.2335023070382));
#28092=CARTESIAN_POINT('Ctrl Pts',(0.303550856968644,1.84907156996267,7.23246026487243));
#28093=CARTESIAN_POINT('Ctrl Pts',(0.289963780582512,1.83348201523114,7.23141822270666));
#28094=CARTESIAN_POINT('Ctrl Pts',(0.275220468382341,1.81903988933764,7.23037618054089));
#28095=CARTESIAN_POINT('Ctrl Pts',(0.260492990267855,1.80461327406046,7.22933525751203));
#28096=CARTESIAN_POINT('Ctrl Pts',(0.244612244279319,1.79133217409741,7.22829433448318));
#28097=CARTESIAN_POINT('Ctrl Pts',(0.227784746718862,1.7793771699298,7.22725341145432));
#28098=CARTESIAN_POINT('Ctrl Pts',(0.210948606994239,1.76741602598364,7.22621195383453));
#28099=CARTESIAN_POINT('Ctrl Pts',(0.193165334803768,1.7567827776921,7.22517049621474));
#28100=CARTESIAN_POINT('Ctrl Pts',(0.174672381150562,1.7476160485164,7.22412903859495));
#28101=CARTESIAN_POINT('Ctrl Pts',(0.156173777093783,1.7384465185053,7.22308726276445));
#28102=CARTESIAN_POINT('Ctrl Pts',(0.1369657346463,1.73074469372405,7.22204548693395));
#28103=CARTESIAN_POINT('Ctrl Pts',(0.117306994261685,1.72460159950089,7.22100371110345));
#28104=CARTESIAN_POINT('Ctrl Pts',(0.0976057610636193,1.71844522684016,
7.21995968345085));
#28105=CARTESIAN_POINT('Ctrl Pts',(0.0774526030808848,1.71385447481779,
7.21891565579826));
#28106=CARTESIAN_POINT('Ctrl Pts',(0.057118550715062,1.7108697375374,7.21787162814566));
#28107=CARTESIAN_POINT('Ctrl Pts',(0.049926662927011,1.70981407508453,7.21750236924979));
#28108=CARTESIAN_POINT('Ctrl Pts',(0.0427121907511549,1.70895884098676,
7.21713311035393));
#28109=CARTESIAN_POINT('Ctrl Pts',(0.0354871780069168,1.70830426323854,
7.21676385145806));
#28110=CARTESIAN_POINT('Ctrl Pts',(0.0150607413861408,1.70645365184715,
7.21571988881051));
#28111=CARTESIAN_POINT('Ctrl Pts',(-0.00557170734229821,1.70619964753602,
7.21467592616295));
#28112=CARTESIAN_POINT('Ctrl Pts',(-0.026138547631234,1.70756953950065,
7.2136319635154));
#28113=CARTESIAN_POINT('Ctrl Pts',(-0.046667553001253,1.70893691140141,
7.21258992134963));
#28114=CARTESIAN_POINT('Ctrl Pts',(-0.0671304596915965,1.71192226083354,
7.21154787918387));
#28115=CARTESIAN_POINT('Ctrl Pts',(-0.0872544790089182,1.71650091800256,
7.2105058370181));
#28116=CARTESIAN_POINT('Ctrl Pts',(-0.10735688544565,1.7210746577657,7.20946491398924));
#28117=CARTESIAN_POINT('Ctrl Pts',(-0.127120406834966,1.72723817394359,
7.20842399096039));
#28118=CARTESIAN_POINT('Ctrl Pts',(-0.146281416869147,1.73491557540926,
7.20738306793154));
#28119=CARTESIAN_POINT('Ctrl Pts',(-0.165452267498667,1.74259691978821,
7.20634161031175));
#28120=CARTESIAN_POINT('Ctrl Pts',(-0.184019299603978,1.75179344401367,
7.20530015269196));
#28121=CARTESIAN_POINT('Ctrl Pts',(-0.201737419578486,1.76238053441513,
7.20425869507217));
#28122=CARTESIAN_POINT('Ctrl Pts',(-0.2194609532111,1.77297085963427,7.20321691924167));
#28123=CARTESIAN_POINT('Ctrl Pts',(-0.236334445827727,1.78495218871504,
7.20217514341117));
#28124=CARTESIAN_POINT('Ctrl Pts',(-0.252141300819966,1.79815624170638,
7.20113336758068));
#28125=CARTESIAN_POINT('Ctrl Pts',(-0.26798232268797,1.8113888355579,7.20008933992808));
#28126=CARTESIAN_POINT('Ctrl Pts',(-0.282751577743477,1.82584891460032,
7.19904531227548));
#28127=CARTESIAN_POINT('Ctrl Pts',(-0.296268388247341,1.84133045767752,
7.19800128462289));
#28128=CARTESIAN_POINT('Ctrl Pts',(-0.301049106947568,1.84680607653571,
7.19763202572702));
#28129=CARTESIAN_POINT('Ctrl Pts',(-0.305673527235467,1.85240918024165,
7.19726276683115));
#28130=CARTESIAN_POINT('Ctrl Pts',(-0.310134937872157,1.85812976555385,
7.19689350793528));
#28131=CARTESIAN_POINT('Ctrl Pts',(-0.323402210825469,1.87514155240117,
7.1957954116243));
#28132=CARTESIAN_POINT('Ctrl Pts',(-0.335308646127504,1.89330340472553,
7.19469731531332));
#28133=CARTESIAN_POINT('Ctrl Pts',(-0.345656671368315,1.91236643280432,
7.19359921900234));
#28134=CARTESIAN_POINT('Ctrl Pts',(-0.355476559111868,1.93045653129457,
7.1925571667987));
#28135=CARTESIAN_POINT('Ctrl Pts',(-0.363892952591292,1.94935726435661,
7.19151511459507));
#28136=CARTESIAN_POINT('Ctrl Pts',(-0.37078024567161,1.96882492836022,7.19047306239144));
#28137=CARTESIAN_POINT('Ctrl Pts',(-0.377659400926478,1.98826958993752,
7.18943224144642));
#28138=CARTESIAN_POINT('Ctrl Pts',(-0.383012770788352,2.00827917357428,
7.1883914205014));
#28139=CARTESIAN_POINT('Ctrl Pts',(-0.386762892875489,2.02859023389911,
7.18735059955638));
#28140=CARTESIAN_POINT('Ctrl Pts',(-0.390512479918614,2.04889839636864,
7.18630992710919));
#28141=CARTESIAN_POINT('Ctrl Pts',(-0.392659131186697,2.06950723080602,
7.18526925466201));
#28142=CARTESIAN_POINT('Ctrl Pts',(-0.393176466959007,2.0901432343219,7.18422858221483));
#28143=CARTESIAN_POINT('Ctrl Pts',(-0.393261346342918,2.09352898755716,
7.18405783887772));
#28144=CARTESIAN_POINT('Ctrl Pts',(-0.393302479711247,2.09691546388672,
7.18388709554061));
#28145=CARTESIAN_POINT('Ctrl Pts',(-0.393299884474655,2.10030145020012,
7.1837163522035));
#28146=CARTESIAN_POINT('',(-0.393299984492277,2.10011044625411,7.0587163522066));
#28147=CARTESIAN_POINT('Ctrl Pts',(-0.393299884474588,2.10030145028756,
7.18371635219909));
#28148=CARTESIAN_POINT('Ctrl Pts',(-0.39328140121979,2.12441641144914,7.18250031983454));
#28149=CARTESIAN_POINT('Ctrl Pts',(-0.391040925770389,2.1484385973344,7.18128428747));
#28150=CARTESIAN_POINT('Ctrl Pts',(-0.386653358989397,2.17200048598598,
7.18006825510545));
#28151=CARTESIAN_POINT('Ctrl Pts',(-0.382991028073696,2.19166774976753,
7.17905322487446));
#28152=CARTESIAN_POINT('Ctrl Pts',(-0.377833722194587,2.21101458890354,
7.17803819464347));
#28153=CARTESIAN_POINT('Ctrl Pts',(-0.371250469312817,2.22983828031445,
7.17702316441248));
#28154=CARTESIAN_POINT('Ctrl Pts',(-0.364479567424196,2.24919852213014,
7.17597920176493));
#28155=CARTESIAN_POINT('Ctrl Pts',(-0.356169995743994,2.26808538203898,
7.17493523911737));
#28156=CARTESIAN_POINT('Ctrl Pts',(-0.346409350110455,2.28624030754929,
7.17389127646981));
#28157=CARTESIAN_POINT('Ctrl Pts',(-0.336666660236327,2.30436183511781,
7.17284923430404));
#28158=CARTESIAN_POINT('Ctrl Pts',(-0.325478487175651,2.32175343208349,
7.17180719213827));
#28159=CARTESIAN_POINT('Ctrl Pts',(-0.312980208580934,2.33817699098913,
7.17076514997249));
#28160=CARTESIAN_POINT('Ctrl Pts',(-0.30049535294108,2.35458291125051,7.16972422694364));
#28161=CARTESIAN_POINT('Ctrl Pts',(-0.286703605366512,2.37002225735787,
7.16868330391478));
#28162=CARTESIAN_POINT('Ctrl Pts',(-0.271783177515999,2.38428646541703,
7.16764238088593));
#28163=CARTESIAN_POINT('Ctrl Pts',(-0.256855086922622,2.39855799920167,
7.16660092326613));
#28164=CARTESIAN_POINT('Ctrl Pts',(-0.240797678718658,2.41165266914036,
7.16555946564634));
#28165=CARTESIAN_POINT('Ctrl Pts',(-0.223825845084588,2.42339895032633,
7.16451800802655));
#28166=CARTESIAN_POINT('Ctrl Pts',(-0.20684882581543,2.4351488205133,7.16347623219605));
#28167=CARTESIAN_POINT('Ctrl Pts',(-0.188957449992455,2.44554909314379,
7.16243445636555));
#28168=CARTESIAN_POINT('Ctrl Pts',(-0.170394562886644,2.45447225975902,
7.16139268053505));
#28169=CARTESIAN_POINT('Ctrl Pts',(-0.151791551679105,2.46341471400139,
7.16034865288245));
#28170=CARTESIAN_POINT('Ctrl Pts',(-0.132514818220812,2.47087342219975,
7.15930462522985));
#28171=CARTESIAN_POINT('Ctrl Pts',(-0.112826694998145,2.47676919578941,
7.15826059757725));
#28172=CARTESIAN_POINT('Ctrl Pts',(-0.105863263881689,2.47885445362762,
7.1578913386814));
#28173=CARTESIAN_POINT('Ctrl Pts',(-0.0988484829767498,2.48074466075623,
7.15752207978556));
#28174=CARTESIAN_POINT('Ctrl Pts',(-0.0917942363465021,2.48243784877227,
7.15715282088971));
#28175=CARTESIAN_POINT('Ctrl Pts',(-0.0718505868599785,2.48722480194768,
7.15610885824215));
#28176=CARTESIAN_POINT('Ctrl Pts',(-0.0514720555961654,2.49046176383376,
7.1550648955946));
#28177=CARTESIAN_POINT('Ctrl Pts',(-0.0309234553292937,2.49208242744415,
7.15402093294705));
#28178=CARTESIAN_POINT('Ctrl Pts',(-0.0104126564268489,2.49370010966919,
7.15297889078128));
#28179=CARTESIAN_POINT('Ctrl Pts',(0.0102668699228779,2.49370727912618,
7.15193684861551));
#28180=CARTESIAN_POINT('Ctrl Pts',(0.0308416363372745,2.49208887190029,
7.15089480644974));
#28181=CARTESIAN_POINT('Ctrl Pts',(0.0513943057757651,2.49047220281833,
7.14985388342088));
#28182=CARTESIAN_POINT('Ctrl Pts',(0.0718417065779379,2.48723345154411,
7.14881296039203));
#28183=CARTESIAN_POINT('Ctrl Pts',(0.0919120052963912,2.48240956222667,
7.14777203736317));
#28184=CARTESIAN_POINT('Ctrl Pts',(0.111992611597167,2.47758319548541,7.14673057974338));
#28185=CARTESIAN_POINT('Ctrl Pts',(0.131695009733336,2.47117022061305,7.14568912212359));
#28186=CARTESIAN_POINT('Ctrl Pts',(0.15075865347209,2.46325847327114,7.1446476645038));
#28187=CARTESIAN_POINT('Ctrl Pts',(0.169828121985114,2.4553443085455,7.1436058886733));
#28188=CARTESIAN_POINT('Ctrl Pts',(0.188257782432902,2.44593077491543,7.1425641128428));
#28189=CARTESIAN_POINT('Ctrl Pts',(0.205808966887233,2.43515303840009,7.1415223370123));
#28190=CARTESIAN_POINT('Ctrl Pts',(0.223398088625048,2.42435200556269,7.1404783093597));
#28191=CARTESIAN_POINT('Ctrl Pts',(0.240104348151232,2.41218131645107,7.13943428170711));
#28192=CARTESIAN_POINT('Ctrl Pts',(0.255719156987838,2.39881867871575,7.13839025405451));
#28193=CARTESIAN_POINT('Ctrl Pts',(0.261241910198285,2.39409248890293,7.13802099515864));
#28194=CARTESIAN_POINT('Ctrl Pts',(0.266628457848157,2.3892175387951,7.13765173626277));
#28195=CARTESIAN_POINT('Ctrl Pts',(0.271870711810878,2.38420275519327,7.13728247736691));
#28196=CARTESIAN_POINT('Ctrl Pts',(0.286691525574139,2.37002504187486,7.13623851471935));
#28197=CARTESIAN_POINT('Ctrl Pts',(0.300444488273553,2.35464263388032,7.1351945520718));
#28198=CARTESIAN_POINT('Ctrl Pts',(0.312930499868253,2.33824229736175,7.13415058942425));
#28199=CARTESIAN_POINT('Ctrl Pts',(0.325393542099181,2.32187213102944,7.13310854725848));
#28200=CARTESIAN_POINT('Ctrl Pts',(0.336593771575419,2.30448829597703,7.13206650509271));
#28201=CARTESIAN_POINT('Ctrl Pts',(0.346370478625851,2.28631259092315,7.13102446292694));
#28202=CARTESIAN_POINT('Ctrl Pts',(0.356136685646498,2.26815640629097,7.12998353989809));
#28203=CARTESIAN_POINT('Ctrl Pts',(0.364482033102595,2.24921067101315,7.12894261686923));
#28204=CARTESIAN_POINT('Ctrl Pts',(0.371290435939313,2.22972394605467,7.12790169384038));
#28205=CARTESIAN_POINT('Ctrl Pts',(0.37810233539428,2.21022721322214,7.12686023622059));
#28206=CARTESIAN_POINT('Ctrl Pts',(0.383375455412086,2.19018962493644,7.1258187786008));
#28207=CARTESIAN_POINT('Ctrl Pts',(0.38704261140603,2.16987780016573,7.12477732098101));
#28208=CARTESIAN_POINT('Ctrl Pts',(0.390710887876003,2.14955976924703,7.12373554515051));
#28209=CARTESIAN_POINT('Ctrl Pts',(0.392772128459542,2.1289680649251,7.12269376932001));
#28210=CARTESIAN_POINT('Ctrl Pts',(0.393210787903623,2.10837653127566,7.12165199348952));
#28211=CARTESIAN_POINT('Ctrl Pts',(0.393650395520046,2.08774048855896,7.12060796583692));
#28212=CARTESIAN_POINT('Ctrl Pts',(0.39246046235079,2.06710535250755,7.11956393818433));
#28213=CARTESIAN_POINT('Ctrl Pts',(0.389677495458099,2.04674270441054,7.11851991053173));
#28214=CARTESIAN_POINT('Ctrl Pts',(0.388693196546589,2.03954070268713,7.11815065163586));
#28215=CARTESIAN_POINT('Ctrl Pts',(0.387510086784553,2.03237269840211,7.11778139273999));
#28216=CARTESIAN_POINT('Ctrl Pts',(0.38613129373705,2.02525032443581,7.11741213384412));
#28217=CARTESIAN_POINT('Ctrl Pts',(0.382233192820861,2.00511406647181,7.11636817119657));
#28218=CARTESIAN_POINT('Ctrl Pts',(0.37674411597597,1.98522355380588,7.11532420854901));
#28219=CARTESIAN_POINT('Ctrl Pts',(0.369713323077346,1.96584729320992,7.11428024590146));
#28220=CARTESIAN_POINT('Ctrl Pts',(0.362695464079869,1.94650667733323,7.11323820373569));
#28221=CARTESIAN_POINT('Ctrl Pts',(0.354141710911723,1.92767913983654,7.11219616156992));
#28222=CARTESIAN_POINT('Ctrl Pts',(0.344151560857891,1.9096198719428,7.11115411940415));
#28223=CARTESIAN_POINT('Ctrl Pts',(0.334172140068277,1.89157999941907,7.1101131963753));
#28224=CARTESIAN_POINT('Ctrl Pts',(0.32275971400379,1.87430741302607,7.10907227334644));
#28225=CARTESIAN_POINT('Ctrl Pts',(0.310060438236427,1.85803426969789,7.10803135031759));
#28226=CARTESIAN_POINT('Ctrl Pts',(0.297354640452012,1.84175276890742,7.1069898926978));
#28227=CARTESIAN_POINT('Ctrl Pts',(0.283361112605571,1.82647232658918,7.105948435078));
#28228=CARTESIAN_POINT('Ctrl Pts',(0.26826766446845,1.81239375841153,7.10490697745821));
#28229=CARTESIAN_POINT('Ctrl Pts',(0.253169604624906,1.79831088861753,7.10386520162771));
#28230=CARTESIAN_POINT('Ctrl Pts',(0.23697151772135,1.7854310990117,7.10282342579721));
#28231=CARTESIAN_POINT('Ctrl Pts',(0.219895241833309,1.77391569706735,7.10178164996671));
#28232=CARTESIAN_POINT('Ctrl Pts',(0.202782055187426,1.76237540432038,7.10073762231412));
#28233=CARTESIAN_POINT('Ctrl Pts',(0.184787531010729,1.75220574943624,7.09969359466152));
#28234=CARTESIAN_POINT('Ctrl Pts',(0.166159781646032,1.74352304848231,7.09864956700892));
#28235=CARTESIAN_POINT('Ctrl Pts',(0.15957139086373,1.74045209096563,7.09828030811306));
#28236=CARTESIAN_POINT('Ctrl Pts',(0.15290396583066,1.73756670059935,7.0979110492172));
#28237=CARTESIAN_POINT('Ctrl Pts',(0.146168980688353,1.73487054475908,7.09754179032133));
#28238=CARTESIAN_POINT('Ctrl Pts',(0.127127942004791,1.72724801752751,7.09649782767378));
#28239=CARTESIAN_POINT('Ctrl Pts',(0.107432306350444,1.72109623771241,7.09545386502623));
#28240=CARTESIAN_POINT('Ctrl Pts',(0.0873345042869595,1.71651913429618,
7.09440990237867));
#28241=CARTESIAN_POINT('Ctrl Pts',(0.0672736742960345,1.7119504509549,7.0933678602129));
#28242=CARTESIAN_POINT('Ctrl Pts',(0.0468128425269421,1.70895091352938,
7.09232581804714));
#28243=CARTESIAN_POINT('Ctrl Pts',(0.0262204380071245,1.70757500254098,
7.09128377588137));
#28244=CARTESIAN_POINT('Ctrl Pts',(0.00565014940626087,1.70620056925936,
7.09024285285251));
#28245=CARTESIAN_POINT('Ctrl Pts',(-0.0150507029261533,1.70644637831647,
7.08920192982366));
#28246=CARTESIAN_POINT('Ctrl Pts',(-0.0356078006313174,1.70831521023379,
7.08816100679481));
#28247=CARTESIAN_POINT('Ctrl Pts',(-0.0561754559260802,1.71018500193448,
7.08711954917501));
#28248=CARTESIAN_POINT('Ctrl Pts',(-0.0765984748844406,1.71367943116632,
7.08607809155522));
#28249=CARTESIAN_POINT('Ctrl Pts',(-0.0966063432742216,1.71874928926075,
7.08503663393543));
#28250=CARTESIAN_POINT('Ctrl Pts',(-0.116620324940065,1.72382069641786,
7.08399485810493));
#28251=CARTESIAN_POINT('Ctrl Pts',(-0.136218199767095,1.73046827506646,
7.08295308227444));
#28252=CARTESIAN_POINT('Ctrl Pts',(-0.155144252585005,1.73859281843073,
7.08191130644394));
#28253=CARTESIAN_POINT('Ctrl Pts',(-0.174111214495567,1.74673492317986,
7.08086727879134));
#28254=CARTESIAN_POINT('Ctrl Pts',(-0.192402803480825,1.7563600233457,7.07982325113874));
#28255=CARTESIAN_POINT('Ctrl Pts',(-0.209786911214481,1.7673224656171,7.07877922348615));
#28256=CARTESIAN_POINT('Ctrl Pts',(-0.215935442253274,1.7711997377555,7.07840996459028));
#28257=CARTESIAN_POINT('Ctrl Pts',(-0.221970727777545,1.7752439141585,7.07804070569442));
#28258=CARTESIAN_POINT('Ctrl Pts',(-0.227883473032081,1.77944733237916,
7.07767144679855));
#28259=CARTESIAN_POINT('Ctrl Pts',(-0.244480686196773,1.79124642488616,
7.07663492850733));
#28260=CARTESIAN_POINT('Ctrl Pts',(-0.26021196929393,1.80437570726496,7.07559841021611));
#28261=CARTESIAN_POINT('Ctrl Pts',(-0.27485505209332,1.81868240307656,7.07456189192489));
#28262=CARTESIAN_POINT('Ctrl Pts',(-0.289471198982429,1.83296278176081,
7.07352728030619));
#28263=CARTESIAN_POINT('Ctrl Pts',(-0.303002545897912,1.84841580435665,
7.0724926686875));
#28264=CARTESIAN_POINT('Ctrl Pts',(-0.315259522961878,1.86484829751446,
7.07145805706881));
#28265=CARTESIAN_POINT('Ctrl Pts',(-0.327838702548867,1.88171275613384,
7.07039624833029));
#28266=CARTESIAN_POINT('Ctrl Pts',(-0.339074904738169,1.89960839978937,
7.06933443959177));
#28267=CARTESIAN_POINT('Ctrl Pts',(-0.348806813328766,1.91828952431015,
7.06827263085326));
#28268=CARTESIAN_POINT('Ctrl Pts',(-0.358284341061996,1.93648234579891,
7.06723857656956));
#28269=CARTESIAN_POINT('Ctrl Pts',(-0.366335033678184,1.9554193233398,7.06620452228586));
#28270=CARTESIAN_POINT('Ctrl Pts',(-0.372856655426999,1.9748488733419,7.06517046800216));
#28271=CARTESIAN_POINT('Ctrl Pts',(-0.379640841809533,1.99506066936748,
7.06409478203623));
#28272=CARTESIAN_POINT('Ctrl Pts',(-0.384769773501248,2.01580476897136,
7.0630190960703));
#28273=CARTESIAN_POINT('Ctrl Pts',(-0.388186045340862,2.03678224772564,
7.06194341010438));
#28274=CARTESIAN_POINT('Ctrl Pts',(-0.391602317180476,2.05775972647993,
7.06086772413845));
#28275=CARTESIAN_POINT('Ctrl Pts',(-0.393305921228637,2.07896968111761,
7.05979203817253));
#28276=CARTESIAN_POINT('Ctrl Pts',(-0.393299984492276,2.10011044625411,
7.0587163522066));
#28277=CARTESIAN_POINT('',(-0.393299833421324,2.09963801828994,6.93371635362524));
#28278=CARTESIAN_POINT('Ctrl Pts',(-0.393299984492259,2.10011044631513,
7.0587163522035));
#28279=CARTESIAN_POINT('Ctrl Pts',(-0.393298300731149,2.10610632963539,
7.05841126922758));
#28280=CARTESIAN_POINT('Ctrl Pts',(-0.393159512893997,2.11210011602306,
7.05810618625166));
#28281=CARTESIAN_POINT('Ctrl Pts',(-0.392883863779012,2.11808755323626,
7.05780110327574));
#28282=CARTESIAN_POINT('Ctrl Pts',(-0.391940620784181,2.13857594917634,
7.05675714062819));
#28283=CARTESIAN_POINT('Ctrl Pts',(-0.389387586552351,2.15905140948699,
7.05571317798064));
#28284=CARTESIAN_POINT('Ctrl Pts',(-0.38523464805053,2.17924112531624,7.05466921533309));
#28285=CARTESIAN_POINT('Ctrl Pts',(-0.381089349326588,2.19939369998765,
7.05362717316732));
#28286=CARTESIAN_POINT('Ctrl Pts',(-0.375350076778481,2.2192608490551,7.05258513100155));
#28287=CARTESIAN_POINT('Ctrl Pts',(-0.368078352856691,2.2385756694312,7.05154308883578));
#28288=CARTESIAN_POINT('Ctrl Pts',(-0.36081443865216,2.25786974599363,7.05050216580693));
#28289=CARTESIAN_POINT('Ctrl Pts',(-0.352021571301162,2.27661197620053,
7.04946124277807));
#28290=CARTESIAN_POINT('Ctrl Pts',(-0.341810773641972,2.29455149709595,
7.04842031974922));
#28291=CARTESIAN_POINT('Ctrl Pts',(-0.331594731983229,2.31250023126175,
7.04737886212943));
#28292=CARTESIAN_POINT('Ctrl Pts',(-0.31995965516463,2.32964478510415,7.04633740450964));
#28293=CARTESIAN_POINT('Ctrl Pts',(-0.307062317059976,2.34575927946216,
7.04529594688985));
#28294=CARTESIAN_POINT('Ctrl Pts',(-0.294161038256251,2.36187869750073,
7.04425417105935));
#28295=CARTESIAN_POINT('Ctrl Pts',(-0.279997217999062,2.3769668781514,7.04321239522885));
#28296=CARTESIAN_POINT('Ctrl Pts',(-0.264767017367462,2.39083211052829,
7.04217061939835));
#28297=CARTESIAN_POINT('Ctrl Pts',(-0.24950389631158,2.4047273129196,7.04112659174576));
#28298=CARTESIAN_POINT('Ctrl Pts',(-0.233170375035,2.41739383823302,7.04008256409316));
#28299=CARTESIAN_POINT('Ctrl Pts',(-0.21599512284965,2.4286806914091,7.03903853644056));
#28300=CARTESIAN_POINT('Ctrl Pts',(-0.209920461280633,2.43267270343221,
7.0386692775447));
#28301=CARTESIAN_POINT('Ctrl Pts',(-0.203740744708566,2.43649253814428,
7.03830001864883));
#28302=CARTESIAN_POINT('Ctrl Pts',(-0.197466795816991,2.44013490639711,
7.03793075975296));
#28303=CARTESIAN_POINT('Ctrl Pts',(-0.179729191202037,2.45043254972306,
7.03688679710541));
#28304=CARTESIAN_POINT('Ctrl Pts',(-0.16113105401224,2.45936964946468,7.03584283445785));
#28305=CARTESIAN_POINT('Ctrl Pts',(-0.141907118808706,2.46680684239994,
7.0347988718103));
#28306=CARTESIAN_POINT('Ctrl Pts',(-0.122718548105475,2.47423035381738,
7.03375682964453));
#28307=CARTESIAN_POINT('Ctrl Pts',(-0.102907121528119,2.48015911746761,
7.03271478747876));
#28308=CARTESIAN_POINT('Ctrl Pts',(-0.0827305591853479,2.48450038306467,
7.03167274531299));
#28309=CARTESIAN_POINT('Ctrl Pts',(-0.0625756661535695,2.48883698621068,
7.03063182228414));
#28310=CARTESIAN_POINT('Ctrl Pts',(-0.0420571254533872,2.49158929377269,
7.02959089925528));
#28311=CARTESIAN_POINT('Ctrl Pts',(-0.0214459658181039,2.49271485909006,
7.02854997622643));
#28312=CARTESIAN_POINT('Ctrl Pts',(-0.000824220828423809,2.49384100246845,
7.02750851860664));
#28313=CARTESIAN_POINT('Ctrl Pts',(0.0198895043193526,2.4933386783378,7.02646706098685));
#28314=CARTESIAN_POINT('Ctrl Pts',(0.0404204218518309,2.49121743250694,
7.02542560336705));
#28315=CARTESIAN_POINT('Ctrl Pts',(0.0609576124746873,2.48909553854299,
7.02438382753656));
#28316=CARTESIAN_POINT('Ctrl Pts',(0.0813111567395613,2.48535384968859,
7.02334205170606));
#28317=CARTESIAN_POINT('Ctrl Pts',(0.101213675164648,2.48005352512464,7.02230027587556));
#28318=CARTESIAN_POINT('Ctrl Pts',(0.12115921333496,2.47474174378886,7.02125624822296));
#28319=CARTESIAN_POINT('Ctrl Pts',(0.140651084799832,2.46786484567961,7.02021222057036));
#28320=CARTESIAN_POINT('Ctrl Pts',(0.159438547379486,2.45953336369455,7.01916819291777));
#28321=CARTESIAN_POINT('Ctrl Pts',(0.166083426632471,2.45658662772346,7.0187989340219));
#28322=CARTESIAN_POINT('Ctrl Pts',(0.17264040429098,2.45345835693534,7.01842967512604));
#28323=CARTESIAN_POINT('Ctrl Pts',(0.179099174630351,2.45015478812481,7.01806041623017));
#28324=CARTESIAN_POINT('Ctrl Pts',(0.197359303388023,2.44081499298261,7.01701645358262));
#28325=CARTESIAN_POINT('Ctrl Pts',(0.214941284571895,2.43001515981853,7.01597249093506));
#28326=CARTESIAN_POINT('Ctrl Pts',(0.231600873030352,2.41787721782408,7.01492852828751));
#28327=CARTESIAN_POINT('Ctrl Pts',(0.24822981438067,2.40576160488187,7.01388648612174));
#28328=CARTESIAN_POINT('Ctrl Pts',(0.263939108184732,2.39231314959407,7.01284444395597));
#28329=CARTESIAN_POINT('Ctrl Pts',(0.278511259789918,2.37769834023673,7.0118024017902));
#28330=CARTESIAN_POINT('Ctrl Pts',(0.293067761133201,2.36309922695504,7.01076147876135));
#28331=CARTESIAN_POINT('Ctrl Pts',(0.306489007437223,2.34733674437685,7.00972055573249));
#28332=CARTESIAN_POINT('Ctrl Pts',(0.318592596039228,2.33061580116936,7.00867963270364));
#28333=CARTESIAN_POINT('Ctrl Pts',(0.330702400728881,2.31388627052123,7.00763817508385));
#28334=CARTESIAN_POINT('Ctrl Pts',(0.341492751301786,2.29619788242215,7.00659671746406));
#28335=CARTESIAN_POINT('Ctrl Pts',(0.350822926458063,2.27778685067068,7.00555525984426));
#28336=CARTESIAN_POINT('Ctrl Pts',(0.36015595238961,2.25937019354637,7.00451348401377));
#28337=CARTESIAN_POINT('Ctrl Pts',(0.368027614683983,2.24023112532588,7.00347170818327));
#28338=CARTESIAN_POINT('Ctrl Pts',(0.374344599730752,2.22062757003448,7.00242993235277));
#28339=CARTESIAN_POINT('Ctrl Pts',(0.380675239084051,2.20098164121345,7.00138590470017));
#28340=CARTESIAN_POINT('Ctrl Pts',(0.385444322246868,2.18086993749164,7.00034187704758));
#28341=CARTESIAN_POINT('Ctrl Pts',(0.388609055986058,2.16056312083789,6.99929784939498));
#28342=CARTESIAN_POINT('Ctrl Pts',(0.389728380827061,2.1533808659642,6.99892859049911));
#28343=CARTESIAN_POINT('Ctrl Pts',(0.390647485222271,2.1461742522484,6.99855933160325));
#28344=CARTESIAN_POINT('Ctrl Pts',(0.391366034505286,2.13895532101789,6.99819007270738));
#28345=CARTESIAN_POINT('Ctrl Pts',(0.39339750516257,2.11854607795223,6.99714611005983));
#28346=CARTESIAN_POINT('Ctrl Pts',(0.393834256174918,2.09791668854596,6.99610214741227));
#28347=CARTESIAN_POINT('Ctrl Pts',(0.392646593475837,2.07733852097014,6.99505818476472));
#28348=CARTESIAN_POINT('Ctrl Pts',(0.391461115610268,2.05679820915098,6.99401614259895));
#28349=CARTESIAN_POINT('Ctrl Pts',(0.388657138203044,2.03630966180985,6.99297410043318));
#28350=CARTESIAN_POINT('Ctrl Pts',(0.384256913792191,2.01614587545684,6.99193205826741));
#28351=CARTESIAN_POINT('Ctrl Pts',(0.37986141515323,1.9960037446936,6.99089113523856));
#28352=CARTESIAN_POINT('Ctrl Pts',(0.373873200714846,1.97618640387247,6.9898502122097));
#28353=CARTESIAN_POINT('Ctrl Pts',(0.36636582349603,1.95695814118212,6.98880928918085));
#28354=CARTESIAN_POINT('Ctrl Pts',(0.358854590683942,1.9377200033572,6.98776783156106));
#28355=CARTESIAN_POINT('Ctrl Pts',(0.34982288900492,1.919072239314,6.98672637394127));
#28356=CARTESIAN_POINT('Ctrl Pts',(0.339393156267765,1.90126103683826,6.98568491632147));
#28357=CARTESIAN_POINT('Ctrl Pts',(0.328960236792561,1.88344439226366,6.98464314049098));
#28358=CARTESIAN_POINT('Ctrl Pts',(0.317128838591403,1.86646543422052,6.98360136466048));
#28359=CARTESIAN_POINT('Ctrl Pts',(0.304065316459306,1.85054224139846,6.98255958882998));
#28360=CARTESIAN_POINT('Ctrl Pts',(0.29097355722767,1.83458463023378,6.98151556117738));
#28361=CARTESIAN_POINT('Ctrl Pts',(0.276644867538597,1.81968787110294,6.98047153352479));
#28362=CARTESIAN_POINT('Ctrl Pts',(0.261283660071214,1.80603445953685,6.97942750587219));
#28363=CARTESIAN_POINT('Ctrl Pts',(0.255850602340914,1.80120542683147,6.97905824697632));
#28364=CARTESIAN_POINT('Ctrl Pts',(0.25028868031497,1.79653155718037,6.97868898808046));
#28365=CARTESIAN_POINT('Ctrl Pts',(0.2446078373961,1.79201965016514,6.97831972918459));
#28366=CARTESIAN_POINT('Ctrl Pts',(0.228547052184692,1.77926366122119,6.97727576653704));
#28367=CARTESIAN_POINT('Ctrl Pts',(0.211437913429965,1.76772937191523,6.97623180388948));
#28368=CARTESIAN_POINT('Ctrl Pts',(0.193492518414073,1.75758864604429,6.97518784124193));
#28369=CARTESIAN_POINT('Ctrl Pts',(0.175580135886038,1.74746657513132,6.97414579907616));
#28370=CARTESIAN_POINT('Ctrl Pts',(0.156835154811601,1.73873338865849,6.97310375691039));
#28371=CARTESIAN_POINT('Ctrl Pts',(0.137499161245205,1.73151815423706,6.97206171474462));
#28372=CARTESIAN_POINT('Ctrl Pts',(0.118183934232137,1.72431066886404,6.97102079171577));
#28373=CARTESIAN_POINT('Ctrl Pts',(0.0982796305767786,1.71861818211602,
6.96997986868691));
#28374=CARTESIAN_POINT('Ctrl Pts',(0.0780482840982825,1.71452191326962,
6.96893894565806));
#28375=CARTESIAN_POINT('Ctrl Pts',(0.0578065473275278,1.7104235406863,6.96789748803827));
#28376=CARTESIAN_POINT('Ctrl Pts',(0.0372381501319202,1.70792318554478,
6.96685603041847));
#28377=CARTESIAN_POINT('Ctrl Pts',(0.016616369407768,1.70705116584,6.96581457279868));
#28378=CARTESIAN_POINT('Ctrl Pts',(-0.00401171216942507,1.70617887969518,
6.96477279696818));
#28379=CARTESIAN_POINT('Ctrl Pts',(-0.0246924737159749,1.70693591435756,
6.96373102113769));
#28380=CARTESIAN_POINT('Ctrl Pts',(-0.0451524999086895,1.70930044567213,
6.96268924530719));
#28381=CARTESIAN_POINT('Ctrl Pts',(-0.0656567509123161,1.7116700879748,
6.96164521765459));
#28382=CARTESIAN_POINT('Ctrl Pts',(-0.0859385913385113,1.71565402192686,
6.960601190002));
#28383=CARTESIAN_POINT('Ctrl Pts',(-0.105733923400703,1.72117916181618,
6.9595571623494));
#28384=CARTESIAN_POINT('Ctrl Pts',(-0.112735272878758,1.72313333137286,
6.95918790345353));
#28385=CARTESIAN_POINT('Ctrl Pts',(-0.119675915054347,1.72527984490144,
6.95881864455767));
#28386=CARTESIAN_POINT('Ctrl Pts',(-0.126544750173951,1.72761402254729,
6.9584493856618));
#28387=CARTESIAN_POINT('Ctrl Pts',(-0.145964207301035,1.73421317101005,
6.95740542301425));
#28388=CARTESIAN_POINT('Ctrl Pts',(-0.164923930214275,1.7423551219909,6.9563614603667));
#28389=CARTESIAN_POINT('Ctrl Pts',(-0.183164600664807,1.75195457327627,
6.95531749771915));
#28390=CARTESIAN_POINT('Ctrl Pts',(-0.201371715436502,1.7615363653366,6.95427545555338));
#28391=CARTESIAN_POINT('Ctrl Pts',(-0.218861731941079,1.7725700494049,6.95323341338761));
#28392=CARTESIAN_POINT('Ctrl Pts',(-0.23539535292366,1.78492236223123,6.95219137122184));
#28393=CARTESIAN_POINT('Ctrl Pts',(-0.251911217057038,1.79726140886763,
6.95115044819299));
#28394=CARTESIAN_POINT('Ctrl Pts',(-0.267472121051817,1.81091585782192,
6.95010952516414));
#28395=CARTESIAN_POINT('Ctrl Pts',(-0.281867930645074,1.82570935182937,
6.94906860213528));
#28396=CARTESIAN_POINT('Ctrl Pts',(-0.296271133550944,1.84051044338978,
6.94802714451549));
#28397=CARTESIAN_POINT('Ctrl Pts',(-0.309507521970585,1.85645123259965,
6.9469856868957));
#28398=CARTESIAN_POINT('Ctrl Pts',(-0.321403674269256,1.87331835503018,
6.94594422927591));
#28399=CARTESIAN_POINT('Ctrl Pts',(-0.333303461361082,1.89019063110196,
6.94490245344542));
#28400=CARTESIAN_POINT('Ctrl Pts',(-0.343861802965516,1.90798918222806,
6.94386067761492));
#28401=CARTESIAN_POINT('Ctrl Pts',(-0.352949044568082,1.92647230209999,
6.94281890178442));
#28402=CARTESIAN_POINT('Ctrl Pts',(-0.362055928449588,1.94499537365495,
6.94177487413183));
#28403=CARTESIAN_POINT('Ctrl Pts',(-0.369685092145126,1.9642052836525,6.94073084647923));
#28404=CARTESIAN_POINT('Ctrl Pts',(-0.375755026526189,1.98384041132862,
6.93968681882663));
#28405=CARTESIAN_POINT('Ctrl Pts',(-0.377901882753596,1.99078509861535,
6.93931755993076));
#28406=CARTESIAN_POINT('Ctrl Pts',(-0.379854150765881,1.99778286138267,
6.93894830103489));
#28407=CARTESIAN_POINT('Ctrl Pts',(-0.381609756971484,2.0048218334692,6.93857904213902));
#28408=CARTESIAN_POINT('Ctrl Pts',(-0.388101192253086,2.03084875887132,
6.93721369026395));
#28409=CARTESIAN_POINT('Ctrl Pts',(-0.391931856124105,2.05756443576007,
6.93584833838888));
#28410=CARTESIAN_POINT('Ctrl Pts',(-0.392994316331167,2.08449653808342,
6.93448298651381));
#28411=CARTESIAN_POINT('Ctrl Pts',(-0.393193170304858,2.08953724975551,
6.93422744221762));
#28412=CARTESIAN_POINT('Ctrl Pts',(-0.393295183208218,2.09458547560849,
6.93397189792143));
#28413=CARTESIAN_POINT('Ctrl Pts',(-0.393299833421324,2.09963801828994,
6.93371635362524));
#28414=CARTESIAN_POINT('',(-0.393057143940665,2.10007656503152,6.80871634984815));
#28415=CARTESIAN_POINT('Ctrl Pts',(-0.393254262534486,2.09963808833903,
6.9337163522035));
#28416=CARTESIAN_POINT('Ctrl Pts',(-0.392351278880494,2.19853643597861,
6.92871380100774));
#28417=CARTESIAN_POINT('Ctrl Pts',(-0.30436299103977,2.42980898719343,6.91708780197104));
#28418=CARTESIAN_POINT('Ctrl Pts',(0.0843393264457993,2.55734221486119,
6.89883835509345));
#28419=CARTESIAN_POINT('Ctrl Pts',(0.430195924005982,2.27665358883452,6.87896801157065));
#28420=CARTESIAN_POINT('Ctrl Pts',(0.381406327177297,1.83390934426664,6.85909766804786));
#28421=CARTESIAN_POINT('Ctrl Pts',(-0.0172716510538061,1.63526705136245,
6.83922732452507));
#28422=CARTESIAN_POINT('Ctrl Pts',(-0.340830224277894,1.8277006749777,6.82243355257695));
#28423=CARTESIAN_POINT('Ctrl Pts',(-0.392544160566776,2.02969108662713,
6.81226322846976));
#28424=CARTESIAN_POINT('Ctrl Pts',(-0.392666129258272,2.10007644209519,
6.8087163522035));
#28425=CARTESIAN_POINT('',(-0.393343588509023,2.1003295827536,6.6837163522035));
#28426=CARTESIAN_POINT('Ctrl Pts',(-0.393299992532543,2.10007664138394,
6.80871634838531));
#28427=CARTESIAN_POINT('Ctrl Pts',(-0.393295695528997,2.12212754098503,
6.80760694442949));
#28428=CARTESIAN_POINT('Ctrl Pts',(-0.39143267046183,2.1441308409618,6.80649754047367));
#28429=CARTESIAN_POINT('Ctrl Pts',(-0.38776007247249,2.16578005925909,6.80538813651785));
#28430=CARTESIAN_POINT('Ctrl Pts',(-0.384068304695278,2.18754227955757,
6.80427294182791));
#28431=CARTESIAN_POINT('Ctrl Pts',(-0.378548221487941,2.20894615427118,
6.80315774713797));
#28432=CARTESIAN_POINT('Ctrl Pts',(-0.371299894246872,2.22969687171348,
6.80204255244803));
#28433=CARTESIAN_POINT('Ctrl Pts',(-0.365762413285198,2.24554972975315,
6.80119058079185));
#28434=CARTESIAN_POINT('Ctrl Pts',(-0.359217317625601,2.26102165989602,
6.80033860913567));
#28435=CARTESIAN_POINT('Ctrl Pts',(-0.351727463573401,2.27599057181628,
6.79948663747949));
#28436=CARTESIAN_POINT('Ctrl Pts',(-0.342549778131173,2.29433271360692,
6.79844267483194));
#28437=CARTESIAN_POINT('Ctrl Pts',(-0.33190610509672,2.3120096670508,6.79739871218439));
#28438=CARTESIAN_POINT('Ctrl Pts',(-0.319916205420557,2.32877611656227,
6.79635474953683));
#28439=CARTESIAN_POINT('Ctrl Pts',(-0.307948362456833,2.34551172238317,
6.79531270737106));
#28440=CARTESIAN_POINT('Ctrl Pts',(-0.294639583445627,2.36133952269403,
6.79427066520529));
#28441=CARTESIAN_POINT('Ctrl Pts',(-0.280154423622598,2.37604055666639,
6.79322862303952));
#28442=CARTESIAN_POINT('Ctrl Pts',(-0.265684820633667,2.39072580195921,
6.79218770001067));
#28443=CARTESIAN_POINT('Ctrl Pts',(-0.250041838204806,2.40428614156079,
6.79114677698182));
#28444=CARTESIAN_POINT('Ctrl Pts',(-0.233428761290965,2.41653736493843,
6.79010585395297));
#28445=CARTESIAN_POINT('Ctrl Pts',(-0.216807152333808,2.42879488022509,
6.78906439633318));
#28446=CARTESIAN_POINT('Ctrl Pts',(-0.19921503617343,2.43974148645848,6.78802293871339));
#28447=CARTESIAN_POINT('Ctrl Pts',(-0.180887370870302,2.44923437554117,
6.7869814810936));
#28448=CARTESIAN_POINT('Ctrl Pts',(-0.162554105666405,2.45873016511533,
6.7859397052631));
#28449=CARTESIAN_POINT('Ctrl Pts',(-0.143485513341916,2.46677104730492,
6.7848979294326));
#28450=CARTESIAN_POINT('Ctrl Pts',(-0.123938681256822,2.47326142753882,
6.7838561536021));
#28451=CARTESIAN_POINT('Ctrl Pts',(-0.104349598250602,2.47976583687688,
6.78281212594951));
#28452=CARTESIAN_POINT('Ctrl Pts',(-0.084280926772598,2.48471287699348,
6.78176809829691));
#28453=CARTESIAN_POINT('Ctrl Pts',(-0.064002939122556,2.48805735888355,
6.78072407064432));
#28454=CARTESIAN_POINT('Ctrl Pts',(-0.0568308806894853,2.48924025828944,
6.78035481174844));
#28455=CARTESIAN_POINT('Ctrl Pts',(-0.0496326908711968,2.49022316086833,
6.77998555285257));
#28456=CARTESIAN_POINT('Ctrl Pts',(-0.0424204075583441,2.49100562530811,
6.7796162939567));
#28457=CARTESIAN_POINT('Ctrl Pts',(-0.0220299593758823,2.49321779584022,
6.77857233130915));
#28458=CARTESIAN_POINT('Ctrl Pts',(-0.00140524789277181,2.4938372592859,
6.77752836866159));
#28459=CARTESIAN_POINT('Ctrl Pts',(0.0191826323878835,2.49283191903748,
6.77648440601404));
#28460=CARTESIAN_POINT('Ctrl Pts',(0.0397326390442958,2.49182842822079,
6.77544236384827));
#28461=CARTESIAN_POINT('Ctrl Pts',(0.0602452194858398,2.48920604284114,
6.7744003216825));
#28462=CARTESIAN_POINT('Ctrl Pts',(0.0804471908052092,2.48498459643413,
6.77335827951673));
#28463=CARTESIAN_POINT('Ctrl Pts',(0.100627465524746,2.48076768379425,6.77231735648788));
#28464=CARTESIAN_POINT('Ctrl Pts',(0.120497070890807,2.47495524093621,6.77127643345902));
#28465=CARTESIAN_POINT('Ctrl Pts',(0.139791077570064,2.467618477,6.77023551043017));
#28466=CARTESIAN_POINT('Ctrl Pts',(0.159094993148286,2.46027794509306,6.76919405281038));
#28467=CARTESIAN_POINT('Ctrl Pts',(0.177822026008554,2.45141177459615,6.76815259519059));
#28468=CARTESIAN_POINT('Ctrl Pts',(0.195724913502099,2.44114021784978,6.76711113757079));
#28469=CARTESIAN_POINT('Ctrl Pts',(0.213633271108271,2.43086552269503,6.7660693617403));
#28470=CARTESIAN_POINT('Ctrl Pts',(0.230716362393179,2.41918498367593,6.7650275859098));
#28471=CARTESIAN_POINT('Ctrl Pts',(0.24675464369661,2.40626301737911,6.7639858100793));
#28472=CARTESIAN_POINT('Ctrl Pts',(0.262827592109034,2.39331311995891,6.7629417824267));
#28473=CARTESIAN_POINT('Ctrl Pts',(0.277850686501704,2.37911694386544,6.76189775477411));
#28474=CARTESIAN_POINT('Ctrl Pts',(0.291639627870715,2.36387727726243,6.76085372712151));
#28475=CARTESIAN_POINT('Ctrl Pts',(0.296516595690895,2.35848720694273,6.76048446822564));
#28476=CARTESIAN_POINT('Ctrl Pts',(0.301239547989098,2.35296690299031,6.76011520932978));
#28477=CARTESIAN_POINT('Ctrl Pts',(0.305801597374482,2.34732624818894,6.75974595043391));
#28478=CARTESIAN_POINT('Ctrl Pts',(0.318699347998627,2.33137908215912,6.75870198778636));
#28479=CARTESIAN_POINT('Ctrl Pts',(0.330384732945562,2.31437278222749,6.7576580251388));
#28480=CARTESIAN_POINT('Ctrl Pts',(0.340684016460012,2.29651791503238,6.75661406249125));
#28481=CARTESIAN_POINT('Ctrl Pts',(0.350964353332628,2.27869589378945,6.75557202032548));
#28482=CARTESIAN_POINT('Ctrl Pts',(0.359863235185042,2.26002900429957,6.75452997815971));
#28483=CARTESIAN_POINT('Ctrl Pts',(0.367249459565265,2.24075767989357,6.75348793599394));
#28484=CARTESIAN_POINT('Ctrl Pts',(0.374627751256537,2.22150705258724,6.75244701296508));
#28485=CARTESIAN_POINT('Ctrl Pts',(0.380496321638926,2.20165395229917,6.75140608993623));
#28486=CARTESIAN_POINT('Ctrl Pts',(0.384771633597181,2.18145968315036,6.75036516690738));
#28487=CARTESIAN_POINT('Ctrl Pts',(0.389049141244229,2.16125504275124,6.74932370928758));
#28488=CARTESIAN_POINT('Ctrl Pts',(0.391731587610378,2.14070959993482,6.74828225166779));
#28489=CARTESIAN_POINT('Ctrl Pts',(0.392786235277038,2.12009635232801,6.747240794048));
#28490=CARTESIAN_POINT('Ctrl Pts',(0.393841205184539,2.09947680647539,6.7461990182175));
#28491=CARTESIAN_POINT('Ctrl Pts',(0.393267384828812,2.07879015063581,6.745157242387));
#28492=CARTESIAN_POINT('Ctrl Pts',(0.391084175669496,2.05830998271875,6.7441154665565));
#28493=CARTESIAN_POINT('Ctrl Pts',(0.388896247454038,2.03778554645398,6.74307143890391));
#28494=CARTESIAN_POINT('Ctrl Pts',(0.385092120865691,2.01746921308134,6.74202741125131));
#28495=CARTESIAN_POINT('Ctrl Pts',(0.379742539442433,1.99762571740026,6.74098338359871));
#28496=CARTESIAN_POINT('Ctrl Pts',(0.377850462614033,1.99060733308155,6.74061412470285));
#28497=CARTESIAN_POINT('Ctrl Pts',(0.375765511630558,1.98364794995271,6.74024486580698));
#28498=CARTESIAN_POINT('Ctrl Pts',(0.373492267844443,1.9767587087847,6.73987560691112));
#28499=CARTESIAN_POINT('Ctrl Pts',(0.367065390582806,1.9572815600147,6.73883164426357));
#28500=CARTESIAN_POINT('Ctrl Pts',(0.35909169912626,1.93825046169438,6.73778768161601));
#28501=CARTESIAN_POINT('Ctrl Pts',(0.349654195370835,1.91992547748342,6.73674371896846));
#28502=CARTESIAN_POINT('Ctrl Pts',(0.340234052920517,1.90163420405555,6.73570167680269));
#28503=CARTESIAN_POINT('Ctrl Pts',(0.329355723557583,1.88404714029489,6.73465963463692));
#28504=CARTESIAN_POINT('Ctrl Pts',(0.317150345673459,1.8674047544785,6.73361759247115));
#28505=CARTESIAN_POINT('Ctrl Pts',(0.304958076173439,1.85078024232304,6.7325766694423));
#28506=CARTESIAN_POINT('Ctrl Pts',(0.291441997180033,1.8350990013637,6.73153574641345));
#28507=CARTESIAN_POINT('Ctrl Pts',(0.27677659772676,1.82057271974483,6.73049482338459));
#28508=CARTESIAN_POINT('Ctrl Pts',(0.262103666506556,1.80603897780633,6.7294533657648));
#28509=CARTESIAN_POINT('Ctrl Pts',(0.24628074701975,1.792661909445,6.72841190814501));
#28510=CARTESIAN_POINT('Ctrl Pts',(0.229519659202689,1.78061681941674,6.72737045052522));
#28511=CARTESIAN_POINT('Ctrl Pts',(0.212753450142578,1.76856804908835,6.72632867469472));
#28512=CARTESIAN_POINT('Ctrl Pts',(0.195049120204018,1.75785246692723,6.72528689886422));
#28513=CARTESIAN_POINT('Ctrl Pts',(0.176647217768549,1.74860186333074,6.72424512303372));
#28514=CARTESIAN_POINT('Ctrl Pts',(0.158205539203375,1.73933126434465,6.72320109538113));
#28515=CARTESIAN_POINT('Ctrl Pts',(0.139063959893764,1.73153224374321,6.72215706772853));
#28516=CARTESIAN_POINT('Ctrl Pts',(0.119483368354343,1.72528862482345,6.72111304007593));
#28517=CARTESIAN_POINT('Ctrl Pts',(0.112557969784387,1.72308033865134,6.72074378118007));
#28518=CARTESIAN_POINT('Ctrl Pts',(0.105577774206092,1.72106616293227,6.7203745222842));
#28519=CARTESIAN_POINT('Ctrl Pts',(0.0985546289480032,1.71924827628372,
6.72000526338833));
#28520=CARTESIAN_POINT('Ctrl Pts',(0.0786989087478119,1.71410877719563,
6.71896130074078));
#28521=CARTESIAN_POINT('Ctrl Pts',(0.0583809172791021,1.71051132234542,
6.71791733809322));
#28522=CARTESIAN_POINT('Ctrl Pts',(0.03786425114929,1.70852689941082,6.71687337544567));
#28523=CARTESIAN_POINT('Ctrl Pts',(0.0173853276376203,1.70654612703605,
6.7158313332799));
#28524=CARTESIAN_POINT('Ctrl Pts',(-0.003290826700979,1.70617262574247,
6.71478929111413));
#28525=CARTESIAN_POINT('Ctrl Pts',(-0.0238910342529198,1.70742630184598,
6.71374724894836));
#28526=CARTESIAN_POINT('Ctrl Pts',(-0.0444691175055708,1.70867863152104,
6.71270632591951));
#28527=CARTESIAN_POINT('Ctrl Pts',(-0.0649706834463184,1.71155465366243,
6.71166540289066));
#28528=CARTESIAN_POINT('Ctrl Pts',(-0.0851232868265916,1.71602224538414,
6.7106244798618));
#28529=CARTESIAN_POINT('Ctrl Pts',(-0.105286240058719,1.72049213154452,
6.70958302224201));
#28530=CARTESIAN_POINT('Ctrl Pts',(-0.125099150865311,1.72655507673637,
6.70854156462222));
#28531=CARTESIAN_POINT('Ctrl Pts',(-0.144299957910001,1.73412787459664,
6.70750010700243));
#28532=CARTESIAN_POINT('Ctrl Pts',(-0.163506631638328,1.7417029862768,6.70645833117193));
#28533=CARTESIAN_POINT('Ctrl Pts',(-0.182100158667977,1.75078856563216,
6.70541655534143));
#28534=CARTESIAN_POINT('Ctrl Pts',(-0.199839514087861,1.76125369580005,
6.70437477951094));
#28535=CARTESIAN_POINT('Ctrl Pts',(-0.217617213527045,1.77174144658427,
6.70333075185834));
#28536=CARTESIAN_POINT('Ctrl Pts',(-0.234536452432076,1.78361427841506,
6.70228672420575));
#28537=CARTESIAN_POINT('Ctrl Pts',(-0.250385527007085,1.79669820662353,
6.70124269655315));
#28538=CARTESIAN_POINT('Ctrl Pts',(-0.255991136938539,1.80132582052999,
6.70087343765728));
#28539=CARTESIAN_POINT('Ctrl Pts',(-0.26146319793638,1.80610458423775,6.70050417876141));
#28540=CARTESIAN_POINT('Ctrl Pts',(-0.266793465007023,1.81102571562586,
6.70013491986554));
#28541=CARTESIAN_POINT('Ctrl Pts',(-0.281638481231432,1.82473127190113,
6.69910651843133));
#28542=CARTESIAN_POINT('Ctrl Pts',(-0.295475092709904,1.8396306599348,6.69807811699712));
#28543=CARTESIAN_POINT('Ctrl Pts',(-0.308103769275524,1.85554763785511,
6.69704971556291));
#28544=CARTESIAN_POINT('Ctrl Pts',(-0.320708900013305,1.87143493899814,
6.69602323155552));
#28545=CARTESIAN_POINT('Ctrl Pts',(-0.332110047029178,1.88833551806399,
6.69499674754813));
#28546=CARTESIAN_POINT('Ctrl Pts',(-0.342145090725859,1.90603704762972,
6.69397026354073));
#28547=CARTESIAN_POINT('Ctrl Pts',(-0.352174893520385,1.92372933239421,
6.6929443156249));
#28548=CARTESIAN_POINT('Ctrl Pts',(-0.360839597491012,1.94222110075685,
6.69191836770907));
#28549=CARTESIAN_POINT('Ctrl Pts',(-0.368020943743174,1.96127193879253,
6.69089241979324));
#28550=CARTESIAN_POINT('Ctrl Pts',(-0.375200246816398,1.98031735663683,
6.68986676377187));
#28551=CARTESIAN_POINT('Ctrl Pts',(-0.380896771828865,1.99992081446266,
6.6888411077505));
#28552=CARTESIAN_POINT('Ctrl Pts',(-0.385041122121011,2.01982379233343,
6.68781545172912));
#28553=CARTESIAN_POINT('Ctrl Pts',(-0.389191248184781,2.03975450797894,
6.68678836630277));
#28554=CARTESIAN_POINT('Ctrl Pts',(-0.391784765705901,2.05998482575166,
6.68576128087642));
#28555=CARTESIAN_POINT('Ctrl Pts',(-0.392803692771429,2.08024781163697,
6.68473419545006));
#28556=CARTESIAN_POINT('Ctrl Pts',(-0.393140278870883,2.08694136175765,
6.68439491436787));
#28557=CARTESIAN_POINT('Ctrl Pts',(-0.393305468394936,2.09363846652409,
6.68405563328569));
#28558=CARTESIAN_POINT('Ctrl Pts',(-0.393299861936612,2.10032954611508,
6.6837163522035));
#28559=CARTESIAN_POINT('',(-0.393444654250221,2.09974553930462,6.5587163522035));
#28560=CARTESIAN_POINT('Ctrl Pts',(-0.393535481127247,2.1003297435405,6.6837163522035));
#28561=CARTESIAN_POINT('Ctrl Pts',(-0.393739262162669,2.123034746097,6.68256576024992));
#28562=CARTESIAN_POINT('Ctrl Pts',(-0.38160853246158,2.27622476562375,6.67479172045541));
#28563=CARTESIAN_POINT('Ctrl Pts',(-0.180457218096371,2.52861429737727,
6.66039423281995));
#28564=CARTESIAN_POINT('Ctrl Pts',(0.262701822499401,2.48374832369023,6.64052388929717));
#28565=CARTESIAN_POINT('Ctrl Pts',(0.464867704575669,2.08684550563379,6.62065354577438));
#28566=CARTESIAN_POINT('Ctrl Pts',(0.240580753727069,1.70201014533589,6.60078320225161));
#28567=CARTESIAN_POINT('Ctrl Pts',(-0.204406286553996,1.68227629526599,
6.58091285872879));
#28568=CARTESIAN_POINT('Ctrl Pts',(-0.386101521636573,1.9387736364229,6.56689057537943));
#28569=CARTESIAN_POINT('Ctrl Pts',(-0.393852311160616,2.08446480552085,
6.559491739871));
#28570=CARTESIAN_POINT('Ctrl Pts',(-0.39373755682333,2.09974534986961,6.5587163522035));
#28571=CARTESIAN_POINT('',(-0.393095185008428,2.09980963099506,6.43371635487844));
#28572=CARTESIAN_POINT('Ctrl Pts',(-0.393299917743934,2.09974563291309,
6.5587163522035));
#28573=CARTESIAN_POINT('Ctrl Pts',(-0.393313019800725,2.12000390579344,
6.55768722808122));
#28574=CARTESIAN_POINT('Ctrl Pts',(-0.39175662785168,2.14032428942168,6.55665810395893));
#28575=CARTESIAN_POINT('Ctrl Pts',(-0.388628280275941,2.16043963740597,
6.55562897983665));
#28576=CARTESIAN_POINT('Ctrl Pts',(-0.385504851375482,2.18052335819331,
6.55460147379779));
#28577=CARTESIAN_POINT('Ctrl Pts',(-0.380814432876337,2.20040193311181,
6.55357396775894));
#28578=CARTESIAN_POINT('Ctrl Pts',(-0.374606423218514,2.21981200976293,
6.55254646172009));
#28579=CARTESIAN_POINT('Ctrl Pts',(-0.368398006858026,2.23922335801804,
6.55151888836667));
#28580=CARTESIAN_POINT('Ctrl Pts',(-0.360671990179837,2.25816541306581,
6.55049131501326));
#28581=CARTESIAN_POINT('Ctrl Pts',(-0.351528071102636,2.27638850650442,
6.54946374165984));
#28582=CARTESIAN_POINT('Ctrl Pts',(-0.342384631981106,2.29461064343008,
6.54843622224278));
#28583=CARTESIAN_POINT('Ctrl Pts',(-0.331823796686522,2.31211322546783,
6.54740870282572));
#28584=CARTESIAN_POINT('Ctrl Pts',(-0.319991410043564,2.3286709152873,6.54638118340866));
#28585=CARTESIAN_POINT('Ctrl Pts',(-0.308133033489064,2.3452649741764,6.54535140703875));
#28586=CARTESIAN_POINT('Ctrl Pts',(-0.294998004680345,2.36090940404951,
6.54432163066884));
#28587=CARTESIAN_POINT('Ctrl Pts',(-0.280773126646011,2.37541122227212,
6.54329185429893));
#28588=CARTESIAN_POINT('Ctrl Pts',(-0.271013005399951,2.38536136060015,
6.54258529342703));
#28589=CARTESIAN_POINT('Ctrl Pts',(-0.26074065664211,2.3947743075843,6.54187873255513));
#28590=CARTESIAN_POINT('Ctrl Pts',(-0.250025253535614,2.40359885143797,
6.54117217168322));
#28591=CARTESIAN_POINT('Ctrl Pts',(-0.234192957916791,2.41663735177286,
6.54012820903567));
#28592=CARTESIAN_POINT('Ctrl Pts',(-0.217290831138302,2.42847291551465,
6.53908424638812));
#28593=CARTESIAN_POINT('Ctrl Pts',(-0.19952789267338,2.4389299485813,6.53804028374056));
#28594=CARTESIAN_POINT('Ctrl Pts',(-0.181797631047831,2.44936774480881,
6.53699824157479));
#28595=CARTESIAN_POINT('Ctrl Pts',(-0.163210297763946,2.4584316238263,6.53595619940902));
#28596=CARTESIAN_POINT('Ctrl Pts',(-0.144005154564302,2.46598825863532,
6.53491415724325));
#28597=CARTESIAN_POINT('Ctrl Pts',(-0.124820637386743,2.47353677773726,
6.5338732342144));
#28598=CARTESIAN_POINT('Ctrl Pts',(-0.10502029815858,2.47958097130056,6.53283231118554));
#28599=CARTESIAN_POINT('Ctrl Pts',(-0.0848646908004932,2.48403499092574,
6.53179138815669));
#28600=CARTESIAN_POINT('Ctrl Pts',(-0.0646987320477896,2.48849129801932,
6.5307499305369));
#28601=CARTESIAN_POINT('Ctrl Pts',(-0.0441778556250099,2.49135562514288,
6.52970847291711));
#28602=CARTESIAN_POINT('Ctrl Pts',(-0.0235747584700142,2.4925928180228,
6.52866701529732));
#28603=CARTESIAN_POINT('Ctrl Pts',(-0.00296536617062622,2.49383038891907,
6.52762523946682));
#28604=CARTESIAN_POINT('Ctrl Pts',(0.0177255608677979,2.49343982789248,
6.52658346363632));
#28605=CARTESIAN_POINT('Ctrl Pts',(0.0382242636162741,2.49143811218505,
6.52554168780582));
#28606=CARTESIAN_POINT('Ctrl Pts',(0.0587672747759153,2.48943206972369,
6.52449766015323));
#28607=CARTESIAN_POINT('Ctrl Pts',(0.0791165070566686,2.48580804897436,
6.52345363250063));
#28608=CARTESIAN_POINT('Ctrl Pts',(0.0990066094176043,2.48063444575029,
6.52240960484803));
#28609=CARTESIAN_POINT('Ctrl Pts',(0.106041477908135,2.47880461010425,6.52204034595217));
#28610=CARTESIAN_POINT('Ctrl Pts',(0.113019055950688,2.47678138525304,6.5216710870563));
#28611=CARTESIAN_POINT('Ctrl Pts',(0.119928162630974,2.47456925368743,6.52130182816043));
#28612=CARTESIAN_POINT('Ctrl Pts',(0.139461474848773,2.46831515188565,6.52025786551288));
#28613=CARTESIAN_POINT('Ctrl Pts',(0.1585624553786,2.46051034557662,6.51921390286533));
#28614=CARTESIAN_POINT('Ctrl Pts',(0.176970315554775,2.45123552982642,6.51816994021777));
#28615=CARTESIAN_POINT('Ctrl Pts',(0.195344312488598,2.4419777760992,6.517127898052));
#28616=CARTESIAN_POINT('Ctrl Pts',(0.213027043608052,2.43125565496542,6.51608585588624));
#28617=CARTESIAN_POINT('Ctrl Pts',(0.229776888481254,2.41919816966874,6.51504381372047));
#28618=CARTESIAN_POINT('Ctrl Pts',(0.246508744284196,2.40715363392185,6.51400289069161));
#28619=CARTESIAN_POINT('Ctrl Pts',(0.262309091843415,2.39377698537339,6.51296196766276));
#28620=CARTESIAN_POINT('Ctrl Pts',(0.276964705742394,2.37924083113511,6.51192104463391));
#28621=CARTESIAN_POINT('Ctrl Pts',(0.291627846382698,2.36469721150688,6.51087958701412));
#28622=CARTESIAN_POINT('Ctrl Pts',(0.305144545108561,2.34899340322404,6.50983812939432));
#28623=CARTESIAN_POINT('Ctrl Pts',(0.31733762779751,2.33233966511091,6.50879667177453));
#28624=CARTESIAN_POINT('Ctrl Pts',(0.329534436004794,2.31568083855474,6.50775489594403));
#28625=CARTESIAN_POINT('Ctrl Pts',(0.340406417968111,2.29807211890184,6.50671312011354));
#28626=CARTESIAN_POINT('Ctrl Pts',(0.349819657747619,2.27975287773312,6.50567134428304));
#28627=CARTESIAN_POINT('Ctrl Pts',(0.359253244458523,2.26139403910891,6.50462731663044));
#28628=CARTESIAN_POINT('Ctrl Pts',(0.367221510047495,2.24232229235326,6.50358328897785));
#28629=CARTESIAN_POINT('Ctrl Pts',(0.373638323625835,2.22279777326188,6.50253926132525));
#28630=CARTESIAN_POINT('Ctrl Pts',(0.375907866478482,2.21589220678185,6.50217000242938));
#28631=CARTESIAN_POINT('Ctrl Pts',(0.377983791870252,2.20893012606515,6.50180074353352));
#28632=CARTESIAN_POINT('Ctrl Pts',(0.379863816328703,2.20192335867795,6.50143148463765));
#28633=CARTESIAN_POINT('Ctrl Pts',(0.385178990405976,2.18211394172355,6.5003875219901));
#28634=CARTESIAN_POINT('Ctrl Pts',(0.388956275414707,2.1618286126238,6.49934355934255));
#28635=CARTESIAN_POINT('Ctrl Pts',(0.391122351594362,2.1413303288554,6.49829959669499));
#28636=CARTESIAN_POINT('Ctrl Pts',(0.393284443043476,2.12086975388883,6.49725755452922));
#28637=CARTESIAN_POINT('Ctrl Pts',(0.393841073482857,2.10019771905904,6.49621551236345));
#28638=CARTESIAN_POINT('Ctrl Pts',(0.39276991764392,2.07958721493799,6.49517347019768));
#28639=CARTESIAN_POINT('Ctrl Pts',(0.391699912209527,2.05899884617456,6.49413254716883));
#28640=CARTESIAN_POINT('Ctrl Pts',(0.389005600237303,2.03847260949129,6.49309162413998));
#28641=CARTESIAN_POINT('Ctrl Pts',(0.38471669010653,2.01828122398447,6.49205070111112));
#28642=CARTESIAN_POINT('Ctrl Pts',(0.380425577303298,1.99807946870831,6.49100924349133));
#28643=CARTESIAN_POINT('Ctrl Pts',(0.374538367383634,1.97821363123813,6.48996778587154));
#28644=CARTESIAN_POINT('Ctrl Pts',(0.367135942177745,1.95894649964903,6.48892632825175));
#28645=CARTESIAN_POINT('Ctrl Pts',(0.359731255208238,1.93967348111127,6.48788455242125));
#28646=CARTESIAN_POINT('Ctrl Pts',(0.350810728731795,1.92100020590288,6.48684277659075));
#28647=CARTESIAN_POINT('Ctrl Pts',(0.340503139541513,1.9031688491057,6.48580100076025));
#28648=CARTESIAN_POINT('Ctrl Pts',(0.330173270263286,1.88529894942616,6.48475697310766));
#28649=CARTESIAN_POINT('Ctrl Pts',(0.318450770263997,1.86827520792864,6.48371294545506));
#28650=CARTESIAN_POINT('Ctrl Pts',(0.305507742171899,1.85231086121303,6.48266891780246));
#28651=CARTESIAN_POINT('Ctrl Pts',(0.300929962789732,1.84666448103643,6.48229965890659));
#28652=CARTESIAN_POINT('Ctrl Pts',(0.296199856595505,1.84115030571008,6.48193040001073));
#28653=CARTESIAN_POINT('Ctrl Pts',(0.291326132333721,1.83577665769377,6.48156114111486));
#28654=CARTESIAN_POINT('Ctrl Pts',(0.277547219650182,1.82058436883381,6.48051717846731));
#28655=CARTESIAN_POINT('Ctrl Pts',(0.262535664373227,1.80642754479418,6.47947321581975));
#28656=CARTESIAN_POINT('Ctrl Pts',(0.246472876546173,1.79351017777575,6.4784292531722));
#28657=CARTESIAN_POINT('Ctrl Pts',(0.230439637948193,1.78061657364587,6.47738721100643));
#28658=CARTESIAN_POINT('Ctrl Pts',(0.213359535057764,1.76895840283298,6.47634516884066));
#28659=CARTESIAN_POINT('Ctrl Pts',(0.195450018164215,1.75870221155184,6.47530312667489));
#28660=CARTESIAN_POINT('Ctrl Pts',(0.177559735810453,1.748457035259,6.47426220364604));
#28661=CARTESIAN_POINT('Ctrl Pts',(0.158842428743844,1.73961123820303,6.47322128061718));
#28662=CARTESIAN_POINT('Ctrl Pts',(0.139543485745911,1.73228746882125,6.47218035758833));
#28663=CARTESIAN_POINT('Ctrl Pts',(0.12023463131385,1.7249599381424,6.47113889996854));
#28664=CARTESIAN_POINT('Ctrl Pts',(0.100344226378691,1.71915627287421,6.47009744234875));
#28665=CARTESIAN_POINT('Ctrl Pts',(0.0801370106551709,1.71495071805903,
6.46905598472895));
#28666=CARTESIAN_POINT('Ctrl Pts',(0.0599236207462894,1.71074387826352,
6.46801420889846));
#28667=CARTESIAN_POINT('Ctrl Pts',(0.0393939544522009,1.70813623536647,
6.46697243306796));
#28668=CARTESIAN_POINT('Ctrl Pts',(0.0188213461226517,1.70715060528221,
6.46593065723746));
#28669=CARTESIAN_POINT('Ctrl Pts',(-0.00179573036665489,1.70616284473616,
6.46488662958486));
#28670=CARTESIAN_POINT('Ctrl Pts',(-0.0224551980791312,1.70680407374761,
6.46384260193227));
#28671=CARTESIAN_POINT('Ctrl Pts',(-0.0428846016013375,1.7090450141698,
6.46279857427967));
#28672=CARTESIAN_POINT('Ctrl Pts',(-0.0501102138435607,1.70983760542343,
6.4624293153838));
#28673=CARTESIAN_POINT('Ctrl Pts',(-0.057307123136383,1.71082984066219,
6.46206005648794));
#28674=CARTESIAN_POINT('Ctrl Pts',(-0.0644636176058504,1.71201890251564,
6.46169079759207));
#28675=CARTESIAN_POINT('Ctrl Pts',(-0.0846963404926527,1.71538059853578,
6.46064683494451));
#28676=CARTESIAN_POINT('Ctrl Pts',(-0.10472567772742,1.72033923833506,6.45960287229696));
#28677=CARTESIAN_POINT('Ctrl Pts',(-0.124281908480982,1.7268527137653,6.45855890964941));
#28678=CARTESIAN_POINT('Ctrl Pts',(-0.143802163440763,1.7333542069556,6.45751686748364));
#28679=CARTESIAN_POINT('Ctrl Pts',(-0.16285033050509,1.74140468476381,6.45647482531786));
#28680=CARTESIAN_POINT('Ctrl Pts',(-0.181168664863993,1.75091146556869,
6.45543278315209));
#28681=CARTESIAN_POINT('Ctrl Pts',(-0.199467325619588,1.76040803624034,
6.45439186012324));
#28682=CARTESIAN_POINT('Ctrl Pts',(-0.217037046678252,1.77135749336402,
6.45335093709438));
#28683=CARTESIAN_POINT('Ctrl Pts',(-0.233641869656607,1.78361990147393,
6.45231001406553));
#28684=CARTESIAN_POINT('Ctrl Pts',(-0.250255220439252,1.79588860723704,
6.45126855644573));
#28685=CARTESIAN_POINT('Ctrl Pts',(-0.265902081696018,1.80947118695674,
6.45022709882594));
#28686=CARTESIAN_POINT('Ctrl Pts',(-0.280376718474852,1.82418523292385,
6.44918564120615));
#28687=CARTESIAN_POINT('Ctrl Pts',(-0.294855777886267,1.83890377467348,
6.44814386537565));
#28688=CARTESIAN_POINT('Ctrl Pts',(-0.308161410034871,1.85475392144732,
6.44710208954515));
#28689=CARTESIAN_POINT('Ctrl Pts',(-0.320126470069047,1.87151819949692,
6.44606031371465));
#28690=CARTESIAN_POINT('Ctrl Pts',(-0.33211739285201,1.88831871391394,6.44501628606205));
#28691=CARTESIAN_POINT('Ctrl Pts',(-0.342761579184032,1.90603667311185,
6.44397225840945));
#28692=CARTESIAN_POINT('Ctrl Pts',(-0.35193616161686,1.92442714291101,6.44292823075685));
#28693=CARTESIAN_POINT('Ctrl Pts',(-0.355181091165119,1.93093161102109,
6.44255897186099));
#28694=CARTESIAN_POINT('Ctrl Pts',(-0.358242619051046,1.93752001607389,
6.44218971296513));
#28695=CARTESIAN_POINT('Ctrl Pts',(-0.36111677432116,1.94418098542257,6.44182045406927));
#28696=CARTESIAN_POINT('Ctrl Pts',(-0.370099885543174,1.96499970357876,
6.44066634323688));
#28697=CARTESIAN_POINT('Ctrl Pts',(-0.377294905324939,1.98663448604179,
6.43951223240448));
#28698=CARTESIAN_POINT('Ctrl Pts',(-0.382575171450579,2.00877978190357,
6.43835812157209));
#28699=CARTESIAN_POINT('Ctrl Pts',(-0.387818378277732,2.03076965205197,
6.43721211081208));
#28700=CARTESIAN_POINT('Ctrl Pts',(-0.391173400330171,2.05326247125569,
6.43606610005207));
#28701=CARTESIAN_POINT('Ctrl Pts',(-0.392563289122906,2.07593853634947,
6.43492008929206));
#28702=CARTESIAN_POINT('Ctrl Pts',(-0.393049920625344,2.08387793961947,
6.43451884500484));
#28703=CARTESIAN_POINT('Ctrl Pts',(-0.393296093584315,2.09183965120009,
6.43411760071762));
#28704=CARTESIAN_POINT('Ctrl Pts',(-0.393299953864913,2.09980950103034,
6.4337163564304));
#28705=CARTESIAN_POINT('',(-0.39324503037053,2.10033752756207,6.30871634932427));
#28706=CARTESIAN_POINT('Ctrl Pts',(-0.392742250083973,2.0998098549993,6.4337163522035));
#28707=CARTESIAN_POINT('Ctrl Pts',(-0.392403036532226,2.17760321604289,
6.42979427165116));
#28708=CARTESIAN_POINT('Ctrl Pts',(-0.332346957112888,2.38725364339046,
6.41924874325792));
#28709=CARTESIAN_POINT('Ctrl Pts',(0.0090363055646272,2.56496598656384,
6.40207976702369));
#28710=CARTESIAN_POINT('Ctrl Pts',(0.395843241910259,2.34409660242095,6.38220942350092));
#28711=CARTESIAN_POINT('Ctrl Pts',(0.419517892994406,1.89930181630866,6.36233907997812));
#28712=CARTESIAN_POINT('Ctrl Pts',(0.0583419894601582,1.63862029114263,
6.34246873645533));
#28713=CARTESIAN_POINT('Ctrl Pts',(-0.314695852507185,1.78486050374472,
6.32459449386379));
#28714=CARTESIAN_POINT('Ctrl Pts',(-0.392294735639502,2.00873010655664,
6.31334369911318));
#28715=CARTESIAN_POINT('Ctrl Pts',(-0.393040371861386,2.10033729489334,
6.3087163522035));
#28716=CARTESIAN_POINT('',(-0.393299999150334,2.10002585241028,6.18371635220694));
#28717=CARTESIAN_POINT('Ctrl Pts',(-0.393299855114474,2.10033758989031,
6.30871634855296));
#28718=CARTESIAN_POINT('Ctrl Pts',(-0.393278402612745,2.12533023944529,
6.30745471991717));
#28719=CARTESIAN_POINT('Ctrl Pts',(-0.39087066562027,2.15021782623328,6.30619309128138));
#28720=CARTESIAN_POINT('Ctrl Pts',(-0.386159708715007,2.17460274368373,
6.30493146264559));
#28721=CARTESIAN_POINT('Ctrl Pts',(-0.383417172994628,2.18879869335834,
6.30419699156698));
#28722=CARTESIAN_POINT('Ctrl Pts',(-0.379894970891419,2.20282469293395,
6.30346252048836));
#28723=CARTESIAN_POINT('Ctrl Pts',(-0.375616850480374,2.21660562437209,
6.30272804940975));
#28724=CARTESIAN_POINT('Ctrl Pts',(-0.369536014841058,2.23619356743597,
6.3016840867622));
#28725=CARTESIAN_POINT('Ctrl Pts',(-0.361900706051859,2.25536293149472,
6.30064012411464));
#28726=CARTESIAN_POINT('Ctrl Pts',(-0.352789306017484,2.27385222333839,
6.29959616146709));
#28727=CARTESIAN_POINT('Ctrl Pts',(-0.343694667385279,2.29230750213739,
6.29855411930131));
#28728=CARTESIAN_POINT('Ctrl Pts',(-0.333129595748178,2.31008451321221,
6.29751207713554));
#28729=CARTESIAN_POINT('Ctrl Pts',(-0.321220949080374,2.32694050293393,
6.29647003496977));
#28730=CARTESIAN_POINT('Ctrl Pts',(-0.309325092112015,2.34377838958748,
6.29542911194092));
#28731=CARTESIAN_POINT('Ctrl Pts',(-0.296088923552708,2.3596966040367,6.29438818891206));
#28732=CARTESIAN_POINT('Ctrl Pts',(-0.281683155049516,2.37448040032277,
6.29334726588321));
#28733=CARTESIAN_POINT('Ctrl Pts',(-0.267269988119078,2.38927178918131,
6.29230580826341));
#28734=CARTESIAN_POINT('Ctrl Pts',(-0.251686523175508,2.40292705773903,
6.29126435064362));
#28735=CARTESIAN_POINT('Ctrl Pts',(-0.235141441433974,2.41526717640813,
6.29022289302383));
#28736=CARTESIAN_POINT('Ctrl Pts',(-0.218591304448665,2.42761106552146,
6.28918111719333));
#28737=CARTESIAN_POINT('Ctrl Pts',(-0.201079576677824,2.43863859426122,
6.28813934136283));
#28738=CARTESIAN_POINT('Ctrl Pts',(-0.182844434120438,2.44821373165224,
6.28709756553233));
#28739=CARTESIAN_POINT('Ctrl Pts',(-0.164569875888608,2.45780956592002,
6.28605353787973));
#28740=CARTESIAN_POINT('Ctrl Pts',(-0.145569458073787,2.46594645129903,
6.28500951022713));
#28741=CARTESIAN_POINT('Ctrl Pts',(-0.126102543342242,2.47253595606682,
6.28396548257454));
#28742=CARTESIAN_POINT('Ctrl Pts',(-0.119217350769364,2.47486657752953,
6.28359622367868));
#28743=CARTESIAN_POINT('Ctrl Pts',(-0.112273931165657,2.47700408971494,
6.28322696478282));
#28744=CARTESIAN_POINT('Ctrl Pts',(-0.105284091406899,2.4789461044748,6.28285770588696));
#28745=CARTESIAN_POINT('Ctrl Pts',(-0.0855225319634753,2.48443653650778,
6.28181374323941));
#28746=CARTESIAN_POINT('Ctrl Pts',(-0.0652714568383826,2.48839335530575,
6.28076978059186));
#28747=CARTESIAN_POINT('Ctrl Pts',(-0.0447931637457112,2.49074091477813,
6.2797258179443));
#28748=CARTESIAN_POINT('Ctrl Pts',(-0.0243525426798438,2.49308415566189,
6.27868377577853));
#28749=CARTESIAN_POINT('Ctrl Pts',(-0.00368624930583731,2.49382387157334,
6.27764173361276));
#28750=CARTESIAN_POINT('Ctrl Pts',(0.0169329342651354,2.49293532004284,
6.27659969144699));
#28751=CARTESIAN_POINT('Ctrl Pts',(0.0375299731568701,2.49204772280274,
6.27555876841814));
#28752=CARTESIAN_POINT('Ctrl Pts',(0.0580792700751206,2.48953533239789,
6.27451784538928));
#28753=CARTESIAN_POINT('Ctrl Pts',(0.0783078534736942,2.48542544036991,
6.27347692236043));
#28754=CARTESIAN_POINT('Ctrl Pts',(0.0985468257454806,2.48131343760851,
6.27243546474064));
#28755=CARTESIAN_POINT('Ctrl Pts',(0.118464031187259,2.47560242487698,6.27139400712085));
#28756=CARTESIAN_POINT('Ctrl Pts',(0.137795975603788,2.4683709531266,6.27035254950106));
#28757=CARTESIAN_POINT('Ctrl Pts',(0.157133826772139,2.46113727184634,6.26931077367056));
#28758=CARTESIAN_POINT('Ctrl Pts',(0.175885385036822,2.45238249816158,6.26826899784006));
#28759=CARTESIAN_POINT('Ctrl Pts',(0.193807344146551,2.44223325869188,6.26722722200956));
#28760=CARTESIAN_POINT('Ctrl Pts',(0.211768041977596,2.43206208141075,6.26618319435697));
#28761=CARTESIAN_POINT('Ctrl Pts',(0.228894950369111,2.42049083300115,6.26513916670437));
#28762=CARTESIAN_POINT('Ctrl Pts',(0.244973316647901,2.40768972054738,6.26409513905177));
#28763=CARTESIAN_POINT('Ctrl Pts',(0.250660024049458,2.4031621348663,6.26372588015591));
#28764=CARTESIAN_POINT('Ctrl Pts',(0.256215881057035,2.39848105731411,6.26335662126004));
#28765=CARTESIAN_POINT('Ctrl Pts',(0.261632488397629,2.39365512257556,6.26298736236417));
#28766=CARTESIAN_POINT('Ctrl Pts',(0.276946231149214,2.38001131964224,6.26194339971662));
#28767=CARTESIAN_POINT('Ctrl Pts',(0.291235468117868,2.36512575060456,6.26089943706907));
#28768=CARTESIAN_POINT('Ctrl Pts',(0.304294608224188,2.34917801148113,6.25985547442151));
#28769=CARTESIAN_POINT('Ctrl Pts',(0.31732972463508,2.33325960994227,6.25881343225574));
#28770=CARTESIAN_POINT('Ctrl Pts',(0.329138729037153,2.31628344204484,6.25777139008998));
#28771=CARTESIAN_POINT('Ctrl Pts',(0.339553155633321,2.29846547432602,6.25672934792421));
#28772=CARTESIAN_POINT('Ctrl Pts',(0.349956397298931,2.28066664282463,6.25568842489535));
#28773=CARTESIAN_POINT('Ctrl Pts',(0.358967640187817,2.2620284237311,6.2546475018665));
#28774=CARTESIAN_POINT('Ctrl Pts',(0.366462067086566,2.24279510981347,6.25360657883765));
#28775=CARTESIAN_POINT('Ctrl Pts',(0.37396034292764,2.2235519181671,6.25256512121786));
#28776=CARTESIAN_POINT('Ctrl Pts',(0.379939964357503,2.20371370084333,6.25152366359807));
#28777=CARTESIAN_POINT('Ctrl Pts',(0.384324344253478,2.18354452952847,6.25048220597828));
#28778=CARTESIAN_POINT('Ctrl Pts',(0.388710063768655,2.16336919565248,6.24944043014778));
#28779=CARTESIAN_POINT('Ctrl Pts',(0.391499450613506,2.14286343254415,6.24839865431728));
#28780=CARTESIAN_POINT('Ctrl Pts',(0.392667268646851,2.12230036173298,6.24735687848678));
#28781=CARTESIAN_POINT('Ctrl Pts',(0.393837610945376,2.10169284337762,6.24631285083419));
#28782=CARTESIAN_POINT('Ctrl Pts',(0.393379403082437,2.08102850631199,6.24526882318159));
#28783=CARTESIAN_POINT('Ctrl Pts',(0.391319508719631,2.06058005459889,6.24422479552899));
#28784=CARTESIAN_POINT('Ctrl Pts',(0.390590951084092,2.05334770526121,6.24385553663313));
#28785=CARTESIAN_POINT('Ctrl Pts',(0.389662503052564,2.04614228935432,6.24348627773726));
#28786=CARTESIAN_POINT('Ctrl Pts',(0.388536878144342,2.03897554324823,6.24311701884139));
#28787=CARTESIAN_POINT('Ctrl Pts',(0.385354530007331,2.01871383710388,6.24207305619384));
#28788=CARTESIAN_POINT('Ctrl Pts',(0.38057349920476,1.99864136333538,6.24102909354628));
#28789=CARTESIAN_POINT('Ctrl Pts',(0.374233503118566,1.97902820517325,6.23998513089873));
#28790=CARTESIAN_POINT('Ctrl Pts',(0.367905170138346,1.95945112752899,6.23894308873296));
#28791=CARTESIAN_POINT('Ctrl Pts',(0.360023731680361,1.940332398772,6.23790104656719));
#28792=CARTESIAN_POINT('Ctrl Pts',(0.350679582695893,1.9219305745496,6.23685900440142));
#28793=CARTESIAN_POINT('Ctrl Pts',(0.341345469180641,1.90354851359733,6.23581808137257));
#28794=CARTESIAN_POINT('Ctrl Pts',(0.330552069459546,1.88588249446903,6.23477715834371));
#28795=CARTESIAN_POINT('Ctrl Pts',(0.318437223452953,1.86916970580192,6.23373623531486));
#28796=CARTESIAN_POINT('Ctrl Pts',(0.306316155577203,1.85244833388214,6.23269477769507));
#28797=CARTESIAN_POINT('Ctrl Pts',(0.292872704385196,1.83668177563127,6.23165332007528));
#28798=CARTESIAN_POINT('Ctrl Pts',(0.278287448085478,1.82207737364858,6.23061186245548));
#28799=CARTESIAN_POINT('Ctrl Pts',(0.263697735354096,1.80746850938438,6.22957008662498));
#28800=CARTESIAN_POINT('Ctrl Pts',(0.247966068089686,1.79402300289681,6.22852831079448));
#28801=CARTESIAN_POINT('Ctrl Pts',(0.231308430985115,1.78190991880412,6.22748653496399));
#28802=CARTESIAN_POINT('Ctrl Pts',(0.214614788019932,1.76977065200527,6.22644250731139));
#28803=CARTESIAN_POINT('Ctrl Pts',(0.19699180723741,1.75896994234586,6.22539847965879));
#28804=CARTESIAN_POINT('Ctrl Pts',(0.178683324881579,1.74963282201487,6.22435445200619));
#28805=CARTESIAN_POINT('Ctrl Pts',(0.172207854655414,1.74633040494248,6.22398519311033));
#28806=CARTESIAN_POINT('Ctrl Pts',(0.165646826256953,1.7432106388467,6.22361593421446));
#28807=CARTESIAN_POINT('Ctrl Pts',(0.159011576713248,1.74027759526106,6.2232466753186));
#28808=CARTESIAN_POINT('Ctrl Pts',(0.140252508865768,1.73198534291091,6.22220271267104));
#28809=CARTESIAN_POINT('Ctrl Pts',(0.120787155174758,1.72513972647364,6.22115875002349));
#28810=CARTESIAN_POINT('Ctrl Pts',(0.100864106192603,1.7198535517962,6.22011478737594));
#28811=CARTESIAN_POINT('Ctrl Pts',(0.0809777078058816,1.71457710160669,
6.21907274521017));
#28812=CARTESIAN_POINT('Ctrl Pts',(0.0606359733120824,1.71085464284479,
6.2180307030444));
#28813=CARTESIAN_POINT('Ctrl Pts',(0.0401052333492136,1.70875013066072,
6.21698866087863));
#28814=CARTESIAN_POINT('Ctrl Pts',(0.0195965430785354,1.70664787868967,
6.21594773784977));
#28815=CARTESIAN_POINT('Ctrl Pts',(-0.00110002439711979,1.70616022706547,
6.21490681482092));
#28816=CARTESIAN_POINT('Ctrl Pts',(-0.0217104213853552,1.70729967201023,
6.21386589179207));
#28817=CARTESIAN_POINT('Ctrl Pts',(-0.0423314033363119,1.70843970214422,
6.21282443417228));
#28818=CARTESIAN_POINT('Ctrl Pts',(-0.0628653908421377,1.71120847373835,
6.21178297655248));
#28819=CARTESIAN_POINT('Ctrl Pts',(-0.0830402962858998,1.71556639169715,
6.21074151893269));
#28820=CARTESIAN_POINT('Ctrl Pts',(-0.103221366042826,1.71992564118988,
6.20969974310219));
#28821=CARTESIAN_POINT('Ctrl Pts',(-0.123042424374501,1.72587481308499,
6.2086579672717));
#28822=CARTESIAN_POINT('Ctrl Pts',(-0.142244402306054,1.73332382131833,
6.2076161914412));
#28823=CARTESIAN_POINT('Ctrl Pts',(-0.161487885748656,1.740788930752,6.2065721637886));
#28824=CARTESIAN_POINT('Ctrl Pts',(-0.180108953734982,1.74976002922748,
6.205528136136));
#28825=CARTESIAN_POINT('Ctrl Pts',(-0.197870483997161,1.76009977704813,
6.20448410848341));
#28826=CARTESIAN_POINT('Ctrl Pts',(-0.204152504437129,1.76375681032143,
6.20411484958754));
#28827=CARTESIAN_POINT('Ctrl Pts',(-0.210327262850315,1.76758465471179,
6.20374559069167));
#28828=CARTESIAN_POINT('Ctrl Pts',(-0.216385198880832,1.77157598183857,
6.20337633179581));
#28829=CARTESIAN_POINT('Ctrl Pts',(-0.2334803086943,1.78283925289159,6.2023343066997));
#28830=CARTESIAN_POINT('Ctrl Pts',(-0.249745511449496,1.79547506393309,
6.20129228160359));
#28831=CARTESIAN_POINT('Ctrl Pts',(-0.264951878099973,1.80933629003383,
6.20025025650748));
#28832=CARTESIAN_POINT('Ctrl Pts',(-0.280130271322575,1.82317201720919,
6.19921014830674));
#28833=CARTESIAN_POINT('Ctrl Pts',(-0.294253114086703,1.83822823763965,
6.198170040106));
#28834=CARTESIAN_POINT('Ctrl Pts',(-0.307122888588786,1.85431642035968,
6.19712993190526));
#28835=CARTESIAN_POINT('Ctrl Pts',(-0.319978940282616,1.87038744854088,
6.19609093275313));
#28836=CARTESIAN_POINT('Ctrl Pts',(-0.331584094239873,1.88748769870106,
6.19505193360099));
#28837=CARTESIAN_POINT('Ctrl Pts',(-0.341779899852588,1.90539427023658,
6.19401293444885));
#28838=CARTESIAN_POINT('Ctrl Pts',(-0.351980988928091,1.923310120951,6.19297339688773));
#28839=CARTESIAN_POINT('Ctrl Pts',(-0.360770892043115,1.9420324931187,6.19193385932661));
#28840=CARTESIAN_POINT('Ctrl Pts',(-0.368036025297585,1.96131195407262,
6.19089432176548));
#28841=CARTESIAN_POINT('Ctrl Pts',(-0.375303531796892,1.9805977128988,6.18985444462667));
#28842=CARTESIAN_POINT('Ctrl Pts',(-0.381045052205479,2.00044021872025,
6.18881456748786));
#28843=CARTESIAN_POINT('Ctrl Pts',(-0.385196512858386,2.02057370409153,
6.18777469034905));
#28844=CARTESIAN_POINT('Ctrl Pts',(-0.389356845623493,2.04075021685875,
6.18673259088238));
#28845=CARTESIAN_POINT('Ctrl Pts',(-0.391920246540558,2.06121821665557,
6.18569049141572));
#28846=CARTESIAN_POINT('Ctrl Pts',(-0.392874256139133,2.0817049497644,6.18464839194905));
#28847=CARTESIAN_POINT('Ctrl Pts',(-0.39315867392223,2.08781263591602,6.18433771203501));
#28848=CARTESIAN_POINT('Ctrl Pts',(-0.393300400369471,2.09392199268277,
6.18402703212098));
#28849=CARTESIAN_POINT('Ctrl Pts',(-0.393299999150334,2.10002585241028,
6.18371635220694));
#28850=CARTESIAN_POINT('',(-0.393299842784111,2.09964833823957,6.05871635220607));
#28851=CARTESIAN_POINT('Ctrl Pts',(-0.39329999915033,2.10002585247783,6.1837163522035));
#28852=CARTESIAN_POINT('Ctrl Pts',(-0.393299908593832,2.10140351038807,
6.18364623089334));
#28853=CARTESIAN_POINT('Ctrl Pts',(-0.393292579542064,2.10278114062278,
6.18357610958318));
#28854=CARTESIAN_POINT('Ctrl Pts',(-0.393278012686526,2.10415869418649,
6.18350598827302));
#28855=CARTESIAN_POINT('Ctrl Pts',(-0.393061142051354,2.12466764449294,
6.18246202562547));
#28856=CARTESIAN_POINT('Ctrl Pts',(-0.39123503229439,2.14522069248777,6.18141806297791));
#28857=CARTESIAN_POINT('Ctrl Pts',(-0.3877999002043,2.16554485030523,6.18037410033036));
#28858=CARTESIAN_POINT('Ctrl Pts',(-0.384371087409844,2.18583161964435,
6.17933205816459));
#28859=CARTESIAN_POINT('Ctrl Pts',(-0.379339190301892,2.20588960740347,
6.17829001599882));
#28860=CARTESIAN_POINT('Ctrl Pts',(-0.372756237950457,2.22544989864094,
6.17724797383305));
#28861=CARTESIAN_POINT('Ctrl Pts',(-0.366180355586435,2.2449891824329,6.17620705080419));
#28862=CARTESIAN_POINT('Ctrl Pts',(-0.358056931096819,2.26403112781519,
6.17516612777534));
#28863=CARTESIAN_POINT('Ctrl Pts',(-0.348488031076856,2.28232109641009,
6.17412520474649));
#28864=CARTESIAN_POINT('Ctrl Pts',(-0.338914216719235,2.30062045825617,
6.17308374712669));
#28865=CARTESIAN_POINT('Ctrl Pts',(-0.32789377056395,2.31816641236441,6.1720422895069));
#28866=CARTESIAN_POINT('Ctrl Pts',(-0.315575366552483,2.33472766778815,
6.17100083188711));
#28867=CARTESIAN_POINT('Ctrl Pts',(-0.303253198731549,2.35129398339745,
6.16995905605661));
#28868=CARTESIAN_POINT('Ctrl Pts',(-0.289632751336844,2.36687443308267,
6.16891728022611));
#28869=CARTESIAN_POINT('Ctrl Pts',(-0.274903271170681,2.38127047747615,
6.16787550439561));
#28870=CARTESIAN_POINT('Ctrl Pts',(-0.260141952898891,2.39569763924626,
6.16683147674301));
#28871=CARTESIAN_POINT('Ctrl Pts',(-0.244267381595321,2.40893481291498,
6.16578744909042));
#28872=CARTESIAN_POINT('Ctrl Pts',(-0.227502734208435,2.42082299781606,
6.16474342143782));
#28873=CARTESIAN_POINT('Ctrl Pts',(-0.221573298174556,2.42502769298818,
6.16437416254195));
#28874=CARTESIAN_POINT('Ctrl Pts',(-0.215532773868685,2.42906404037763,
6.16400490364609));
#28875=CARTESIAN_POINT('Ctrl Pts',(-0.209391789819131,2.43292637077339,
6.16363564475022));
#28876=CARTESIAN_POINT('Ctrl Pts',(-0.192030101207922,2.4438458874345,6.16259168210267));
#28877=CARTESIAN_POINT('Ctrl Pts',(-0.173760224257052,2.45343619790509,
6.16154771945511));
#28878=CARTESIAN_POINT('Ctrl Pts',(-0.154811809403332,2.46154971120064,
6.16050375680756));
#28879=CARTESIAN_POINT('Ctrl Pts',(-0.13589825220054,2.46964829881421,6.15946171464179));
#28880=CARTESIAN_POINT('Ctrl Pts',(-0.116309280141604,2.47627514083168,
6.15841967247602));
#28881=CARTESIAN_POINT('Ctrl Pts',(-0.0962991659999387,2.48132841570976,
6.15737763031025));
#28882=CARTESIAN_POINT('Ctrl Pts',(-0.0763105424065161,2.48637626345001,
6.1563367072814));
#28883=CARTESIAN_POINT('Ctrl Pts',(-0.0559023773375834,2.48985369179578,
6.15529578425255));
#28884=CARTESIAN_POINT('Ctrl Pts',(-0.0353440257925067,2.49170867981292,
6.15425486122369));
#28885=CARTESIAN_POINT('Ctrl Pts',(-0.0147751160138901,2.49356462050355,
6.1532134036039));
#28886=CARTESIAN_POINT('Ctrl Pts',(0.00594340298049596,2.49379637405595,
6.15217194598411));
#28887=CARTESIAN_POINT('Ctrl Pts',(0.0265365777307039,2.49240374621344,
6.15113048836432));
#28888=CARTESIAN_POINT('Ctrl Pts',(0.0471360445935823,2.49101069286241,
6.15008871253382));
#28889=CARTESIAN_POINT('Ctrl Pts',(0.0676093599278807,2.4879923557627,6.14904693670333));
#28890=CARTESIAN_POINT('Ctrl Pts',(0.087687145564979,2.48340038406693,6.14800516087283));
#28891=CARTESIAN_POINT('Ctrl Pts',(0.107808329791356,2.47879848672013,6.14696113322023));
#28892=CARTESIAN_POINT('Ctrl Pts',(0.12753157469738,2.4726163842311,6.14591710556764));
#28893=CARTESIAN_POINT('Ctrl Pts',(0.146602379961316,2.46495565784034,6.14487307791504));
#28894=CARTESIAN_POINT('Ctrl Pts',(0.153347473807763,2.46224615933084,6.14450381901917));
#28895=CARTESIAN_POINT('Ctrl Pts',(0.160011151913248,2.45935212611668,6.14413456012331));
#28896=CARTESIAN_POINT('Ctrl Pts',(0.166582894089214,2.45627942600838,6.14376530122744));
#28897=CARTESIAN_POINT('Ctrl Pts',(0.185162414956153,2.44759233904554,6.14272133857989));
#28898=CARTESIAN_POINT('Ctrl Pts',(0.20311593421766,2.437422107738,6.14167737593233));
#28899=CARTESIAN_POINT('Ctrl Pts',(0.220195040800469,2.42588193261806,6.14063341328478));
#28900=CARTESIAN_POINT('Ctrl Pts',(0.237242728526341,2.41436298689377,6.13959137111901));
#28901=CARTESIAN_POINT('Ctrl Pts',(0.253418560469922,2.40147945778163,6.13854932895324));
#28902=CARTESIAN_POINT('Ctrl Pts',(0.268499280807892,2.38739002454094,6.13750728678747));
#28903=CARTESIAN_POINT('Ctrl Pts',(0.283563804689129,2.37331572313022,6.13646636375861));
#28904=CARTESIAN_POINT('Ctrl Pts',(0.297534997207425,2.35803856734134,6.13542544072976));
#28905=CARTESIAN_POINT('Ctrl Pts',(0.310223311501841,2.3417568758088,6.13438451770091));
#28906=CARTESIAN_POINT('Ctrl Pts',(0.322918142183783,2.32546682242384,6.13334306008111));
#28907=CARTESIAN_POINT('Ctrl Pts',(0.334328313411587,2.30817177308647,6.13230160246132));
#28908=CARTESIAN_POINT('Ctrl Pts',(0.344304824574808,2.29010280843404,6.13126014484153));
#28909=CARTESIAN_POINT('Ctrl Pts',(0.354284383997128,2.27202832292518,6.13021836901103));
#28910=CARTESIAN_POINT('Ctrl Pts',(0.362829087642008,2.25318011242003,6.12917659318053));
#28911=CARTESIAN_POINT('Ctrl Pts',(0.369836543771707,2.23381263352538,6.12813481735003));
#28912=CARTESIAN_POINT('Ctrl Pts',(0.376859146676849,2.2144032913856,6.12709078969743));
#28913=CARTESIAN_POINT('Ctrl Pts',(0.382337673061383,2.19447315015525,6.12604676204484));
#28914=CARTESIAN_POINT('Ctrl Pts',(0.386219768628404,2.17429118602245,6.12500273439224));
#28915=CARTESIAN_POINT('Ctrl Pts',(0.387592814944907,2.16715308984889,6.12463347549637));
#28916=CARTESIAN_POINT('Ctrl Pts',(0.388766629366076,2.15998355751807,6.12426421660051));
#28917=CARTESIAN_POINT('Ctrl Pts',(0.38974045088391,2.15279461094474,6.12389495770464));
#28918=CARTESIAN_POINT('Ctrl Pts',(0.392493622984526,2.13247014000626,6.12285099505709));
#28919=CARTESIAN_POINT('Ctrl Pts',(0.393660874785178,2.11186916959329,6.12180703240953));
#28920=CARTESIAN_POINT('Ctrl Pts',(0.393202917917753,2.09126184567742,6.12076306976198));
#28921=CARTESIAN_POINT('Ctrl Pts',(0.392745803511332,2.07069243115447,6.11972102759621));
#28922=CARTESIAN_POINT('Ctrl Pts',(0.390669371671991,2.050117414939,6.11867898543044));
#28923=CARTESIAN_POINT('Ctrl Pts',(0.386986190350865,2.02981041047474,6.11763694326467));
#28924=CARTESIAN_POINT('Ctrl Pts',(0.383306964708616,2.00952521541426,6.11659602023582));
#28925=CARTESIAN_POINT('Ctrl Pts',(0.378024517546849,1.98950818613007,6.11555509720697));
#28926=CARTESIAN_POINT('Ctrl Pts',(0.371202993583489,1.97002605047681,6.11451417417811));
#28927=CARTESIAN_POINT('Ctrl Pts',(0.364377966263212,1.95053390930645,6.11347271655832));
#28928=CARTESIAN_POINT('Ctrl Pts',(0.35601251097747,1.93157791033799,6.11243125893853));
#28929=CARTESIAN_POINT('Ctrl Pts',(0.346220267740802,1.91340842407684,6.11138980131874));
#28930=CARTESIAN_POINT('Ctrl Pts',(0.336425032546919,1.89523338624552,6.11034802548825));
#28931=CARTESIAN_POINT('Ctrl Pts',(0.325202522164563,1.87784596952126,6.10930624965775));
#28932=CARTESIAN_POINT('Ctrl Pts',(0.312711261766873,1.86147000866941,6.10826447382725));
#28933=CARTESIAN_POINT('Ctrl Pts',(0.300193001226371,1.84505865080657,6.10722044617466));
#28934=CARTESIAN_POINT('Ctrl Pts',(0.286401006965626,1.82966366217002,6.10617641852206));
#28935=CARTESIAN_POINT('Ctrl Pts',(0.271533098652582,1.81547466486071,6.10513239086946));
#28936=CARTESIAN_POINT('Ctrl Pts',(0.266274514367124,1.81045620249827,6.1047631319736));
#28937=CARTESIAN_POINT('Ctrl Pts',(0.260881650172954,1.80558824092061,6.10439387307773));
#28938=CARTESIAN_POINT('Ctrl Pts',(0.255364202363869,1.80087792767657,6.10402461418186));
#28939=CARTESIAN_POINT('Ctrl Pts',(0.239765365106384,1.78756100792163,6.10298065153431));
#28940=CARTESIAN_POINT('Ctrl Pts',(0.223075554826068,1.77542788418826,6.10193668888676));
#28941=CARTESIAN_POINT('Ctrl Pts',(0.205500647589076,1.76465782573546,6.1008927262392));
#28942=CARTESIAN_POINT('Ctrl Pts',(0.187958071287748,1.75390757996572,6.09985068407343));
#28943=CARTESIAN_POINT('Ctrl Pts',(0.169534219197412,1.74451585298908,6.09880864190766));
#28944=CARTESIAN_POINT('Ctrl Pts',(0.150465953659464,1.73662018934819,6.09776659974189));
#28945=CARTESIAN_POINT('Ctrl Pts',(0.131418167139149,1.728733005526,6.09672567671304));
#28946=CARTESIAN_POINT('Ctrl Pts',(0.111728006427996,1.72233900204228,6.09568475368418));
#28947=CARTESIAN_POINT('Ctrl Pts',(0.0916544637766103,1.7175286294769,6.09464383065533));
#28948=CARTESIAN_POINT('Ctrl Pts',(0.0715706118769009,1.71271578642953,
6.09360237303554));
#28949=CARTESIAN_POINT('Ctrl Pts',(0.0511036964483818,1.70948838625732,
6.09256091541575));
#28950=CARTESIAN_POINT('Ctrl Pts',(0.030525748887928,1.70788640847985,6.09151945779596));
#28951=CARTESIAN_POINT('Ctrl Pts',(0.00994151386737211,1.70628394122833,
6.09047768196546));
#28952=CARTESIAN_POINT('Ctrl Pts',(-0.0107530850732378,1.70630790604642,
6.08943590613496));
#28953=CARTESIAN_POINT('Ctrl Pts',(-0.0312840311149845,1.70794617793319,
6.08839413030446));
#28954=CARTESIAN_POINT('Ctrl Pts',(-0.051859355262508,1.70958799098181,
6.08735010265186));
#28955=CARTESIAN_POINT('Ctrl Pts',(-0.0722695930447734,1.71285096117465,
6.08630607499927));
#28956=CARTESIAN_POINT('Ctrl Pts',(-0.0922482234436121,1.71767140406256,
6.08526204734667));
#28957=CARTESIAN_POINT('Ctrl Pts',(-0.0993144031407224,1.71937633152683,
6.0848927884508));
#28958=CARTESIAN_POINT('Ctrl Pts',(-0.106326727224237,1.72127563273673,
6.08452352955494));
#28959=CARTESIAN_POINT('Ctrl Pts',(-0.11327393712809,1.72336502397215,6.08415427065907));
#28960=CARTESIAN_POINT('Ctrl Pts',(-0.13291497414987,1.729272116341,6.08311030801152));
#28961=CARTESIAN_POINT('Ctrl Pts',(-0.152151217691466,1.73673732853695,
6.08206634536396));
#28962=CARTESIAN_POINT('Ctrl Pts',(-0.170720490515658,1.7456845979666,6.08102238271641));
#28963=CARTESIAN_POINT('Ctrl Pts',(-0.189255603161535,1.75461540793,6.07998034055064));
#28964=CARTESIAN_POINT('Ctrl Pts',(-0.207125499390956,1.76502260112509,
6.07893829838487));
#28965=CARTESIAN_POINT('Ctrl Pts',(-0.224086311424601,1.77678147480054,
6.0778962562191));
#28966=CARTESIAN_POINT('Ctrl Pts',(-0.241028907812571,1.78852771963039,
6.07685533319025));
#28967=CARTESIAN_POINT('Ctrl Pts',(-0.257063740193955,1.80162236967847,
6.07581441016139));
#28968=CARTESIAN_POINT('Ctrl Pts',(-0.271974558916785,1.81589662215662,
6.07477348713254));
#28969=CARTESIAN_POINT('Ctrl Pts',(-0.286893035447487,1.8301782055188,6.07373202951275));
#28970=CARTESIAN_POINT('Ctrl Pts',(-0.300685802432052,1.84564010442998,
6.07269057189296));
#28971=CARTESIAN_POINT('Ctrl Pts',(-0.313171988864168,1.86207523165744,
6.07164911427316));
#28972=CARTESIAN_POINT('Ctrl Pts',(-0.325661990370595,1.87851538053279,
6.07060733844267));
#28973=CARTESIAN_POINT('Ctrl Pts',(-0.336844200656697,1.89592874243516,
6.06956556261217));
#28974=CARTESIAN_POINT('Ctrl Pts',(-0.346580484385113,1.91407835563501,
6.06852378678167));
#28975=CARTESIAN_POINT('Ctrl Pts',(-0.35633781331175,1.93226719963566,6.06747975912907));
#28976=CARTESIAN_POINT('Ctrl Pts',(-0.364642680053273,1.95119479771925,
6.06643573147648));
#28977=CARTESIAN_POINT('Ctrl Pts',(-0.371404358991896,1.97060258069877,
6.06539170382388));
#28978=CARTESIAN_POINT('Ctrl Pts',(-0.373795876202062,1.97746685914618,
6.06502244492801));
#28979=CARTESIAN_POINT('Ctrl Pts',(-0.375994807470021,1.98439107285004,
6.06465318603215));
#28980=CARTESIAN_POINT('Ctrl Pts',(-0.377998660159086,1.99136343655134,
6.06428392713628));
#28981=CARTESIAN_POINT('Ctrl Pts',(-0.385025732525039,2.01581398850962,
6.06298901708767));
#28982=CARTESIAN_POINT('Ctrl Pts',(-0.389684076670332,2.04097403727138,
6.06169410703905));
#28983=CARTESIAN_POINT('Ctrl Pts',(-0.391864857411872,2.06643180782983,
6.06039919699043));
#28984=CARTESIAN_POINT('Ctrl Pts',(-0.39280956022492,2.07745998090674,6.05983824872898));
#28985=CARTESIAN_POINT('Ctrl Pts',(-0.393289913826653,2.08854375466981,
6.05927730046753));
#28986=CARTESIAN_POINT('Ctrl Pts',(-0.393299842784111,2.09964833823957,
6.05871635220607));
#28987=CARTESIAN_POINT('',(-0.393077172497714,2.10015043742846,5.93371631113999));
#28988=CARTESIAN_POINT('Ctrl Pts',(-0.393299842784156,2.0996483382905,6.0587163522035));
#28989=CARTESIAN_POINT('Ctrl Pts',(-0.393318117775776,2.12008716099077,
6.05768388466541));
#28990=CARTESIAN_POINT('Ctrl Pts',(-0.391738844875401,2.14055949436901,
6.05665141712732));
#28991=CARTESIAN_POINT('Ctrl Pts',(-0.388572825286167,2.16079514330213,
6.05561894958924));
#28992=CARTESIAN_POINT('Ctrl Pts',(-0.385406021092393,2.18103580704376,
6.05458622618453));
#28993=CARTESIAN_POINT('Ctrl Pts',(-0.380651767631321,2.20103892416321,
6.05355350277983));
#28994=CARTESIAN_POINT('Ctrl Pts',(-0.374372619051574,2.22054058281121,
6.05252077937513));
#28995=CARTESIAN_POINT('Ctrl Pts',(-0.368092998734516,2.24004370657184,
6.0514879783844));
#28996=CARTESIAN_POINT('Ctrl Pts',(-0.360288510019637,2.25904459142575,
6.05045517739367));
#28997=CARTESIAN_POINT('Ctrl Pts',(-0.351070906641866,2.27729666807264,
6.04942237640295));
#28998=CARTESIAN_POINT('Ctrl Pts',(-0.341832636631956,2.29558966739089,
6.04838725978664));
#28999=CARTESIAN_POINT('Ctrl Pts',(-0.331175306035825,2.3131298581053,6.04735214317034));
#29000=CARTESIAN_POINT('Ctrl Pts',(-0.319255925186921,2.3296966352236,6.04631702655404));
#29001=CARTESIAN_POINT('Ctrl Pts',(-0.311949868724265,2.33985134129138,
6.04568254557386));
#29002=CARTESIAN_POINT('Ctrl Pts',(-0.304170494125852,2.34964090855378,
6.04504806459368));
#29003=CARTESIAN_POINT('Ctrl Pts',(-0.2959610723649,2.35902110656203,6.0444135836135));
#29004=CARTESIAN_POINT('Ctrl Pts',(-0.282453449687211,2.37445510167483,
6.04336962096594));
#29005=CARTESIAN_POINT('Ctrl Pts',(-0.267695034824309,2.38887563042575,
6.04232565831839));
#29006=CARTESIAN_POINT('Ctrl Pts',(-0.251863595678851,2.40207551898775,
6.04128169567084));
#29007=CARTESIAN_POINT('Ctrl Pts',(-0.236061280171633,2.41525112493237,
6.04023965350507));
#29008=CARTESIAN_POINT('Ctrl Pts',(-0.219190379233024,2.42721003637822,
6.0391976113393));
#29009=CARTESIAN_POINT('Ctrl Pts',(-0.201465358703167,2.43778188116387,
6.03815556917353));
#29010=CARTESIAN_POINT('Ctrl Pts',(-0.183759374566912,2.4483423719543,6.03711464614467));
#29011=CARTESIAN_POINT('Ctrl Pts',(-0.165201705818374,2.45751835364565,
6.03607372311582));
#29012=CARTESIAN_POINT('Ctrl Pts',(-0.14603553004465,2.4651828500417,6.03503280008697));
#29013=CARTESIAN_POINT('Ctrl Pts',(-0.126859511022575,2.47285128272334,
6.03399134246717));
#29014=CARTESIAN_POINT('Ctrl Pts',(-0.107075037835066,2.47900639114825,
6.03294988484738));
#29015=CARTESIAN_POINT('Ctrl Pts',(-0.086945493420707,2.48356925212252,
6.03190842722759));
#29016=CARTESIAN_POINT('Ctrl Pts',(-0.0668097985529559,2.48813350724974,
6.03086665139709));
#29017=CARTESIAN_POINT('Ctrl Pts',(-0.0463295475315251,2.49110441918453,
6.02982487556659));
#29018=CARTESIAN_POINT('Ctrl Pts',(-0.0257776276362968,2.49245433353888,
6.02878309973609));
#29019=CARTESIAN_POINT('Ctrl Pts',(-0.00518128429983682,2.49380716576374,
6.0277390720835));
#29020=CARTESIAN_POINT('Ctrl Pts',(0.015486300775959,2.49353201500072,6.0266950444309));
#29021=CARTESIAN_POINT('Ctrl Pts',(0.0359521962755143,2.49165332831851,
6.0256510167783));
#29022=CARTESIAN_POINT('Ctrl Pts',(0.0431907152518356,2.49098886146437,
6.02528175788244));
#29023=CARTESIAN_POINT('Ctrl Pts',(0.0504040724291839,2.49012427348697,
6.02491249898657));
#29024=CARTESIAN_POINT('Ctrl Pts',(0.0575805078623604,2.48906217384155,
6.0245432400907));
#29025=CARTESIAN_POINT('Ctrl Pts',(0.0778696075120675,2.48605942327764,
6.02349927744315));
#29026=CARTESIAN_POINT('Ctrl Pts',(0.0979836429094615,2.48145637659588,
6.02245531479559));
#29027=CARTESIAN_POINT('Ctrl Pts',(0.117652189613658,2.47529035729567,6.02141135214804));
#29028=CARTESIAN_POINT('Ctrl Pts',(0.137284553906781,2.46913568105239,6.02036930998227));
#29029=CARTESIAN_POINT('Ctrl Pts',(0.156472344283298,2.46142390032958,6.0193272678165));
#29030=CARTESIAN_POINT('Ctrl Pts',(0.174956214545047,2.45224311631609,6.01828522565073));
#29031=CARTESIAN_POINT('Ctrl Pts',(0.193420233420518,2.44307219232039,6.01724430262188));
#29032=CARTESIAN_POINT('Ctrl Pts',(0.211181164526297,2.43243569686198,6.01620337959302));
#29033=CARTESIAN_POINT('Ctrl Pts',(0.228000607581332,2.4204693635007,6.01516245656417));
#29034=CARTESIAN_POINT('Ctrl Pts',(0.244828688663949,2.40849688454248,6.01412099894438));
#29035=CARTESIAN_POINT('Ctrl Pts',(0.260713706850183,2.39519361666377,6.01307954132459));
#29036=CARTESIAN_POINT('Ctrl Pts',(0.275446728161847,2.38073829440412,6.0120380837048));
#29037=CARTESIAN_POINT('Ctrl Pts',(0.290184251053825,2.36627855541332,6.0109963078743));
#29038=CARTESIAN_POINT('Ctrl Pts',(0.303768576933495,2.35066660197949,6.0099545320438));
#29039=CARTESIAN_POINT('Ctrl Pts',(0.31602873468093,2.33411691279352,6.0089127562133));
#29040=CARTESIAN_POINT('Ctrl Pts',(0.328315393037552,2.31753145107883,6.00786872856071));
#29041=CARTESIAN_POINT('Ctrl Pts',(0.339271778590694,2.30000483142703,6.00682470090811));
#29042=CARTESIAN_POINT('Ctrl Pts',(0.34877070422074,2.28177977301496,6.00578067325552));
#29043=CARTESIAN_POINT('Ctrl Pts',(0.352130349706522,2.27533380874416,6.00541141435965));
#29044=CARTESIAN_POINT('Ctrl Pts',(0.355308109232392,2.26880067178446,6.00504215546378));
#29045=CARTESIAN_POINT('Ctrl Pts',(0.358299811004213,2.26219166265362,6.00467289656791));
#29046=CARTESIAN_POINT('Ctrl Pts',(0.366757900808832,2.2435067812678,6.00362893392036));
#29047=CARTESIAN_POINT('Ctrl Pts',(0.373775667542263,2.22410282783564,6.00258497127281));
#29048=CARTESIAN_POINT('Ctrl Pts',(0.37923810783494,2.20422738395342,6.00154100862525));
#29049=CARTESIAN_POINT('Ctrl Pts',(0.384690499380086,2.18438850309194,6.00049896645949));
#29050=CARTESIAN_POINT('Ctrl Pts',(0.38859299370584,2.16408053914949,5.99945692429372));
#29051=CARTESIAN_POINT('Ctrl Pts',(0.390879279086038,2.14356924581834,5.99841488212795));
#29052=CARTESIAN_POINT('Ctrl Pts',(0.393163109031653,2.12307998129402,5.99737395909909));
#29053=CARTESIAN_POINT('Ctrl Pts',(0.393834066137538,2.10238854524085,5.99633303607024));
#29054=CARTESIAN_POINT('Ctrl Pts',(0.392877227231284,2.08176886391203,5.99529211304139));
#29055=CARTESIAN_POINT('Ctrl Pts',(0.391919896917505,2.06113859285228,5.9942506554216));
#29056=CARTESIAN_POINT('Ctrl Pts',(0.389333118466535,2.04058088587227,5.9932091978018));
#29057=CARTESIAN_POINT('Ctrl Pts',(0.38515407534178,2.0203681706375,5.99216774018201));
#29058=CARTESIAN_POINT('Ctrl Pts',(0.380973755337161,2.00014927953703,5.99112596435151));
#29059=CARTESIAN_POINT('Ctrl Pts',(0.375200386419442,1.98027630263458,5.99008418852102));
#29060=CARTESIAN_POINT('Ctrl Pts',(0.367921756355568,1.9610090966997,5.98904241269052));
#29061=CARTESIAN_POINT('Ctrl Pts',(0.36062739336764,1.94170024426196,5.98799838503792));
#29062=CARTESIAN_POINT('Ctrl Pts',(0.35182158723032,1.92300044321811,5.98695435738532));
#29063=CARTESIAN_POINT('Ctrl Pts',(0.341639571887238,1.90514802305159,5.98591032973273));
#29064=CARTESIAN_POINT('Ctrl Pts',(0.338038326523736,1.89883385604381,5.98554107083686));
#29065=CARTESIAN_POINT('Ctrl Pts',(0.334265326646065,1.89262543385607,5.98517181194099));
#29066=CARTESIAN_POINT('Ctrl Pts',(0.330327815664333,1.88653238138202,5.98480255304513));
#29067=CARTESIAN_POINT('Ctrl Pts',(0.319195749693074,1.86930620412889,5.98375859039757));
#29068=CARTESIAN_POINT('Ctrl Pts',(0.306679402167288,1.85290182961062,5.98271462775002));
#29069=CARTESIAN_POINT('Ctrl Pts',(0.29292469072401,1.83754997511099,5.98167066510247));
#29070=CARTESIAN_POINT('Ctrl Pts',(0.279195282554585,1.82222636200197,5.9806286229367));
#29071=CARTESIAN_POINT('Ctrl Pts',(0.264232473562321,1.80795200707744,5.97958658077093));
#29072=CARTESIAN_POINT('Ctrl Pts',(0.248223818474283,1.79492652369954,5.97854453860516));
#29073=CARTESIAN_POINT('Ctrl Pts',(0.232232356430318,1.78191502948616,5.9775036155763));
#29074=CARTESIAN_POINT('Ctrl Pts',(0.215197827734225,1.77015022853234,5.97646269254745));
#29075=CARTESIAN_POINT('Ctrl Pts',(0.197342476301318,1.75979294973904,5.97542176951859));
#29076=CARTESIAN_POINT('Ctrl Pts',(0.179477954825285,1.74943035171729,5.9743803118988));
#29077=CARTESIAN_POINT('Ctrl Pts',(0.160792396807795,1.74047710311107,5.97333885427901));
#29078=CARTESIAN_POINT('Ctrl Pts',(0.141534992388243,1.73304940941639,5.97229739665922));
#29079=CARTESIAN_POINT('Ctrl Pts',(0.122271703992083,1.72561944623746,5.97125562082872));
#29080=CARTESIAN_POINT('Ctrl Pts',(0.102436920285775,1.71971619671289,5.97021384499822));
#29081=CARTESIAN_POINT('Ctrl Pts',(0.0822966545981881,1.7154065124811,5.96917206916772));
#29082=CARTESIAN_POINT('Ctrl Pts',(0.0621128552692868,1.71108751276906,
5.96812804151513));
#29083=CARTESIAN_POINT('Ctrl Pts',(0.0416229857702449,1.70836905204285,
5.96708401386253));
#29084=CARTESIAN_POINT('Ctrl Pts',(0.0211006423750957,1.70726643523712,
5.96603998620993));
#29085=CARTESIAN_POINT('Ctrl Pts',(0.0138421585180325,1.70687645412576,
5.96567072731406));
#29086=CARTESIAN_POINT('Ctrl Pts',(0.00657961297702736,1.70668812886686,
5.9653014684182));
#29087=CARTESIAN_POINT('Ctrl Pts',(-0.000674980476240858,1.70670057920033,
5.96493220952233));
#29088=CARTESIAN_POINT('Ctrl Pts',(-0.0211850471886834,1.70673577857736,
5.96388824687478));
#29089=CARTESIAN_POINT('Ctrl Pts',(-0.041753464065631,1.70837976333955,
5.96284428422722));
#29090=CARTESIAN_POINT('Ctrl Pts',(-0.0621072520305343,1.71163473475964,
5.96180032157967));
#29091=CARTESIAN_POINT('Ctrl Pts',(-0.0824235970092251,1.71488371830906,
5.9607582794139));
#29092=CARTESIAN_POINT('Ctrl Pts',(-0.102525369071605,1.71973774976776,
5.95971623724813));
#29093=CARTESIAN_POINT('Ctrl Pts',(-0.122143202966196,1.72614718408288,
5.95867419508236));
#29094=CARTESIAN_POINT('Ctrl Pts',(-0.141739967615372,1.73254973476624,
5.95763327205351));
#29095=CARTESIAN_POINT('Ctrl Pts',(-0.160853121076448,1.74050417215389,
5.95659234902466));
#29096=CARTESIAN_POINT('Ctrl Pts',(-0.17922713088291,1.74991068917278,5.95555142599581));
#29097=CARTESIAN_POINT('Ctrl Pts',(-0.197610577101928,1.75932203713364,
5.95450996837601));
#29098=CARTESIAN_POINT('Ctrl Pts',(-0.215253459013915,1.77018663362267,
5.95346851075622));
#29099=CARTESIAN_POINT('Ctrl Pts',(-0.231923177832209,1.78235785924376,
5.95242705313643));
#29100=CARTESIAN_POINT('Ctrl Pts',(-0.248597989976352,1.7945328037049,5.95138527730593));
#29101=CARTESIAN_POINT('Ctrl Pts',(-0.26429847468269,1.80801470934215,5.95034350147543));
#29102=CARTESIAN_POINT('Ctrl Pts',(-0.278824424075222,1.82261609538562,
5.94930172564494));
#29103=CARTESIAN_POINT('Ctrl Pts',(-0.293381771636991,1.83724904265635,
5.94825769799234));
#29104=CARTESIAN_POINT('Ctrl Pts',(-0.306759038676237,1.85300573987908,
5.94721367033974));
#29105=CARTESIAN_POINT('Ctrl Pts',(-0.318795253923177,1.86966442724569,
5.94616964268715));
#29106=CARTESIAN_POINT('Ctrl Pts',(-0.323052305488274,1.87555638660928,
5.94580038379128));
#29107=CARTESIAN_POINT('Ctrl Pts',(-0.327141999865019,1.88156092106608,
5.94543112489541));
#29108=CARTESIAN_POINT('Ctrl Pts',(-0.331058573920149,1.88766745272107,
5.94506186599955));
#29109=CARTESIAN_POINT('Ctrl Pts',(-0.342388352507316,1.9053322920967,5.94399368205291));
#29110=CARTESIAN_POINT('Ctrl Pts',(-0.352331112848581,1.92395378138503,
5.94292549810627));
#29111=CARTESIAN_POINT('Ctrl Pts',(-0.360732399787938,1.94329318539631,
5.94185731415963));
#29112=CARTESIAN_POINT('Ctrl Pts',(-0.369114934475254,1.96258942252364,
5.94079151447326));
#29113=CARTESIAN_POINT('Ctrl Pts',(-0.37596250182271,1.9825997914935,5.93972571478688));
#29114=CARTESIAN_POINT('Ctrl Pts',(-0.381166155586733,2.00306057646535,
5.9386599151005));
#29115=CARTESIAN_POINT('Ctrl Pts',(-0.386360756782567,2.02348576670712,
5.93759596953909));
#29116=CARTESIAN_POINT('Ctrl Pts',(-0.389916919389646,2.04435916204525,
5.93653202397768));
#29117=CARTESIAN_POINT('Ctrl Pts',(-0.39177519953194,2.06540111227642,5.93546807841626));
#29118=CARTESIAN_POINT('Ctrl Pts',(-0.392795050595118,2.07694923940009,
5.93488416967867));
#29119=CARTESIAN_POINT('Ctrl Pts',(-0.393304387679479,2.0885478865703,5.93430026094109));
#29120=CARTESIAN_POINT('Ctrl Pts',(-0.393299971507302,2.10014970756677,
5.9337163522035));
#29121=CARTESIAN_POINT('',(-0.393409105398565,2.10028637322991,5.80871640015418));
#29122=CARTESIAN_POINT('Ctrl Pts',(-0.392706208187778,2.10015165266115,
5.93371624276851));
#29123=CARTESIAN_POINT('Ctrl Pts',(-0.392898096062828,2.15652638923434,
5.93087466933792));
#29124=CARTESIAN_POINT('Ctrl Pts',(-0.355155351020755,2.3440598714961,5.92140964806639));
#29125=CARTESIAN_POINT('Ctrl Pts',(-0.0665060678930708,2.56027379505342,
5.90532117895399));
#29126=CARTESIAN_POINT('Ctrl Pts',(0.351005511560806,2.40507401451683,5.88545083543116));
#29127=CARTESIAN_POINT('Ctrl Pts',(0.44651731924308,1.97001035773783,5.8655804919084));
#29128=CARTESIAN_POINT('Ctrl Pts',(0.132410274363759,1.65419450124252,5.84571014838559));
#29129=CARTESIAN_POINT('Ctrl Pts',(-0.283092572096759,1.74305187273891,
5.82675548880205));
#29130=CARTESIAN_POINT('Ctrl Pts',(-0.392741683210659,1.98774849000428,
5.81442427705941));
#29131=CARTESIAN_POINT('Ctrl Pts',(-0.393666477116067,2.10028433320096,
5.80871651315772));
#29132=CARTESIAN_POINT('',(-0.393383440529804,2.09969440306954,5.68371631382268));
#29133=CARTESIAN_POINT('Ctrl Pts',(-0.393299895110372,2.10028723887339,
5.8087163522035));
#29134=CARTESIAN_POINT('Ctrl Pts',(-0.393286722953847,2.11832312558545,
5.80780072191567));
#29135=CARTESIAN_POINT('Ctrl Pts',(-0.392032844841001,2.13631441240402,
5.80688509162785));
#29136=CARTESIAN_POINT('Ctrl Pts',(-0.389556943360793,2.15413204115306,
5.80596946134003));
#29137=CARTESIAN_POINT('Ctrl Pts',(-0.386734025968569,2.17444694240656,
5.80492549869248));
#29138=CARTESIAN_POINT('Ctrl Pts',(-0.382309324566935,2.19460096126699,
5.80388153604494));
#29139=CARTESIAN_POINT('Ctrl Pts',(-0.376317765844307,2.21432335330084,
5.80283757339739));
#29140=CARTESIAN_POINT('Ctrl Pts',(-0.370337229239578,2.23400946386934,
5.80179553123162));
#29141=CARTESIAN_POINT('Ctrl Pts',(-0.362795711325402,2.25326481037358,
5.80075348906585));
#29142=CARTESIAN_POINT('Ctrl Pts',(-0.353779012615713,2.2718292764131,5.79971144690009));
#29143=CARTESIAN_POINT('Ctrl Pts',(-0.34477199769879,2.29037380450774,5.79867052387123));
#29144=CARTESIAN_POINT('Ctrl Pts',(-0.33429324105237,2.30822825405188,5.79762960084238));
#29145=CARTESIAN_POINT('Ctrl Pts',(-0.32247635922602,2.32515303182576,5.79658867781353));
#29146=CARTESIAN_POINT('Ctrl Pts',(-0.31065340855715,2.34208650172438,5.79554722019374));
#29147=CARTESIAN_POINT('Ctrl Pts',(-0.297491367778473,2.35808873349275,
5.79450576257394));
#29148=CARTESIAN_POINT('Ctrl Pts',(-0.283167113736886,2.3729492181669,5.79346430495415));
#29149=CARTESIAN_POINT('Ctrl Pts',(-0.268838483011204,2.38781424336698,
5.79242252912365));
#29150=CARTESIAN_POINT('Ctrl Pts',(-0.2533474683363,2.40153632279997,5.79138075329315));
#29151=CARTESIAN_POINT('Ctrl Pts',(-0.236907025572907,2.41394259225884,
5.79033897746265));
#29152=CARTESIAN_POINT('Ctrl Pts',(-0.220431046419399,2.42637567815067,
5.78929494981006));
#29153=CARTESIAN_POINT('Ctrl Pts',(-0.203002163053162,2.43748687994941,
5.78825092215746));
#29154=CARTESIAN_POINT('Ctrl Pts',(-0.184861958539821,2.44714686558404,
5.78720689450486));
#29155=CARTESIAN_POINT('Ctrl Pts',(-0.178446005980517,2.45056347588244,
5.78683763560898));
#29156=CARTESIAN_POINT('Ctrl Pts',(-0.171941273055359,2.45379897950855,
5.7864683767131));
#29157=CARTESIAN_POINT('Ctrl Pts',(-0.165359022886146,2.45684910473496,
5.78609911781722));
#29158=CARTESIAN_POINT('Ctrl Pts',(-0.146749793995061,2.46547236836449,
5.78505515516966));
#29159=CARTESIAN_POINT('Ctrl Pts',(-0.127408763273877,2.47266173477362,
5.78401119252211));
#29160=CARTESIAN_POINT('Ctrl Pts',(-0.107582483937317,2.47830001209341,
5.78296722987455));
#29161=CARTESIAN_POINT('Ctrl Pts',(-0.087792677178002,2.48392791719451,
5.78192518770878));
#29162=CARTESIAN_POINT('Ctrl Pts',(-0.0675200771685368,2.48801014089082,
5.78088314554301));
#29163=CARTESIAN_POINT('Ctrl Pts',(-0.0470298398041594,2.49047802008307,
5.77984110337724));
#29164=CARTESIAN_POINT('Ctrl Pts',(-0.0265616086328142,2.49294324881184,
5.77880018034838));
#29165=CARTESIAN_POINT('Ctrl Pts',(-0.00587692747130106,2.4937974587555,
5.77775925731953));
#29166=CARTESIAN_POINT('Ctrl Pts',(0.014750420358856,2.49302330096222,5.77671833429068));
#29167=CARTESIAN_POINT('Ctrl Pts',(0.0353883618572411,2.49224874558166,
5.77567687667089));
#29168=CARTESIAN_POINT('Ctrl Pts',(0.055968175334715,2.48984416323488,5.7746354190511));
#29169=CARTESIAN_POINT('Ctrl Pts',(0.0762171144521648,2.48584432283576,
5.77359396143131));
#29170=CARTESIAN_POINT('Ctrl Pts',(0.0964722405032938,2.48184326031102,
5.77255218560081));
#29171=CARTESIAN_POINT('Ctrl Pts',(0.116395576724372,2.47624614735455,5.77151040977031));
#29172=CARTESIAN_POINT('Ctrl Pts',(0.135726498939805,2.46913846654818,5.77046863393982));
#29173=CARTESIAN_POINT('Ctrl Pts',(0.155099205382283,2.46201542232845,5.76942460628722));
#29174=CARTESIAN_POINT('Ctrl Pts',(0.173876272279996,2.45337559944097,5.76838057863463));
#29175=CARTESIAN_POINT('Ctrl Pts',(0.191818181633477,2.44335211546578,5.76733655098203));
#29176=CARTESIAN_POINT('Ctrl Pts',(0.198163999793638,2.43980694056914,5.76696729208617));
#29177=CARTESIAN_POINT('Ctrl Pts',(0.204405598637342,2.43608908123724,5.7665980331903));
#29178=CARTESIAN_POINT('Ctrl Pts',(0.210533289488355,2.43220569534132,5.76622877429444));
#29179=CARTESIAN_POINT('Ctrl Pts',(0.227857395788466,2.42122665091808,5.76518481164689));
#29180=CARTESIAN_POINT('Ctrl Pts',(0.244371993186064,2.40885609993933,5.76414084899933));
#29181=CARTESIAN_POINT('Ctrl Pts',(0.259845080949438,2.39523791068625,5.76309688635178));
#29182=CARTESIAN_POINT('Ctrl Pts',(0.275289704300553,2.38164477355973,5.76205484418601));
#29183=CARTESIAN_POINT('Ctrl Pts',(0.289696035761867,2.36680898995127,5.76101280202024));
#29184=CARTESIAN_POINT('Ctrl Pts',(0.302862808493005,2.35091633910873,5.75997075985447));
#29185=CARTESIAN_POINT('Ctrl Pts',(0.316015440317073,2.33504075672354,5.75892983682562));
#29186=CARTESIAN_POINT('Ctrl Pts',(0.327930666993002,2.31811110573357,5.75788891379676));
#29187=CARTESIAN_POINT('Ctrl Pts',(0.338445697352575,2.30034819675637,5.75684799076791));
#29188=CARTESIAN_POINT('Ctrl Pts',(0.348966127957685,2.28257616521208,5.75580653314812));
#29189=CARTESIAN_POINT('Ctrl Pts',(0.358084536956932,2.26397064569898,5.75476507552832));
#29190=CARTESIAN_POINT('Ctrl Pts',(0.365682516154062,2.24477978926367,5.75372361790853));
#29191=CARTESIAN_POINT('Ctrl Pts',(0.373282816865082,2.22558306918508,5.75268184207803));
#29192=CARTESIAN_POINT('Ctrl Pts',(0.379361525966739,2.20580135299859,5.75164006624753));
#29193=CARTESIAN_POINT('Ctrl Pts',(0.38384943816891,2.18570005144346,5.75059829041703));
#29194=CARTESIAN_POINT('Ctrl Pts',(0.388347051095149,2.16555530046887,5.74955426276444));
#29195=CARTESIAN_POINT('Ctrl Pts',(0.391246898912448,2.14509031418877,5.74851023511184));
#29196=CARTESIAN_POINT('Ctrl Pts',(0.392531253844577,2.1245785425769,5.74746620745924));
#29197=CARTESIAN_POINT('Ctrl Pts',(0.392985513349061,2.11732379782107,5.74709694856338));
#29198=CARTESIAN_POINT('Ctrl Pts',(0.393238160889453,2.11006320532748,5.74672768966751));
#29199=CARTESIAN_POINT('Ctrl Pts',(0.393289970276536,2.10280878619362,5.74635843077165));
#29200=CARTESIAN_POINT('Ctrl Pts',(0.39343644491943,2.08229921231399,5.74531446812409));
#29201=CARTESIAN_POINT('Ctrl Pts',(0.391974714140571,2.06171704037194,5.74427050547654));
#29202=CARTESIAN_POINT('Ctrl Pts',(0.388900158778556,2.04133521923663,5.74322654282899));
#29203=CARTESIAN_POINT('Ctrl Pts',(0.385831259392432,2.02099089265757,5.74218450066321));
#29204=CARTESIAN_POINT('Ctrl Pts',(0.381155474434773,2.00084691349555,5.74114245849745));
#29205=CARTESIAN_POINT('Ctrl Pts',(0.374920061046105,1.98117307617722,5.74010041633167));
#29206=CARTESIAN_POINT('Ctrl Pts',(0.36869134439346,1.9615203682511,5.73905949330282));
#29207=CARTESIAN_POINT('Ctrl Pts',(0.360906518220287,1.94233750634693,5.73801857027397));
#29208=CARTESIAN_POINT('Ctrl Pts',(0.3516631222465,1.92388089697071,5.73697764724511));
#29209=CARTESIAN_POINT('Ctrl Pts',(0.342414979105453,1.90541480876094,5.73593618962532));
#29210=CARTESIAN_POINT('Ctrl Pts',(0.331707084728963,1.88767638332203,5.73489473200553));
#29211=CARTESIAN_POINT('Ctrl Pts',(0.31968399246388,1.87089950903074,5.73385327438574));
#29212=CARTESIAN_POINT('Ctrl Pts',(0.307657226619948,1.85411750867295,5.73281149855524));
#29213=CARTESIAN_POINT('Ctrl Pts',(0.29431492054294,1.83829822082006,5.73176972272474));
#29214=CARTESIAN_POINT('Ctrl Pts',(0.27984277426044,1.82364350614791,5.73072794689424));
#29215=CARTESIAN_POINT('Ctrl Pts',(0.265339346105336,1.80895711497744,5.72968391924164));
#29216=CARTESIAN_POINT('Ctrl Pts',(0.24970175924849,1.79544080416041,5.72863989158905));
#29217=CARTESIAN_POINT('Ctrl Pts',(0.233150338958184,1.78325750294019,5.72759586393645));
#29218=CARTESIAN_POINT('Ctrl Pts',(0.227296318553429,1.7789484289943,5.72722660504058));
#29219=CARTESIAN_POINT('Ctrl Pts',(0.221328245067012,1.77480570851145,5.72685734614472));
#29220=CARTESIAN_POINT('Ctrl Pts',(0.215256644930681,1.77083519809496,5.72648808724885));
#29221=CARTESIAN_POINT('Ctrl Pts',(0.198091117372228,1.75960983666715,5.7254441246013));
#29222=CARTESIAN_POINT('Ctrl Pts',(0.17999399740984,1.74969738450892,5.72440016195374));
#29223=CARTESIAN_POINT('Ctrl Pts',(0.161192284904169,1.74124947764864,5.72335619930619));
#29224=CARTESIAN_POINT('Ctrl Pts',(0.142425160174654,1.73281711162335,5.72231415714042));
#29225=CARTESIAN_POINT('Ctrl Pts',(0.122956654946036,1.72584429543379,5.72127211497465));
#29226=CARTESIAN_POINT('Ctrl Pts',(0.103039198346786,1.72043733902812,5.72023007280888));
#29227=CARTESIAN_POINT('Ctrl Pts',(0.0831431327830263,1.7150361896087,5.71918914978003));
#29228=CARTESIAN_POINT('Ctrl Pts',(0.0627997719662527,1.71119778107657,
5.71814822675118));
#29229=CARTESIAN_POINT('Ctrl Pts',(0.0422775070903213,1.70897889776353,
5.71710730372232));
#29230=CARTESIAN_POINT('Ctrl Pts',(0.0217447025140247,1.70675887488984,
5.71606584610253));
#29231=CARTESIAN_POINT('Ctrl Pts',(0.00103354010403899,1.70616013399676,
5.71502438848274));
#29232=CARTESIAN_POINT('Ctrl Pts',(-0.0195810732662579,1.70718774004654,
5.71398293086295));
#29233=CARTESIAN_POINT('Ctrl Pts',(-0.040201985299664,1.70821566007478,
5.71294115503245));
#29234=CARTESIAN_POINT('Ctrl Pts',(-0.0607255571206432,1.71087084355894,
5.71189937920196));
#29235=CARTESIAN_POINT('Ctrl Pts',(-0.0808815378784357,1.71510642142221,
5.71085760337146));
#29236=CARTESIAN_POINT('Ctrl Pts',(-0.101081086246029,1.71935115458314,
5.70981357571886));
#29237=CARTESIAN_POINT('Ctrl Pts',(-0.120910750701084,1.72518289432425,
5.70876954806626));
#29238=CARTESIAN_POINT('Ctrl Pts',(-0.140114271369878,1.73250458375853,
5.70772552041367));
#29239=CARTESIAN_POINT('Ctrl Pts',(-0.14690630491541,1.73509416934054,5.7073562615178));
#29240=CARTESIAN_POINT('Ctrl Pts',(-0.153620204484674,1.73786970293102,
5.70698700262194));
#29241=CARTESIAN_POINT('Ctrl Pts',(-0.160245347593037,1.74082550400288,
5.70661774372607));
#29242=CARTESIAN_POINT('Ctrl Pts',(-0.17897584269351,1.74918209594194,5.70557378107852));
#29243=CARTESIAN_POINT('Ctrl Pts',(-0.197106707974342,1.7590326889642,5.70452981843097));
#29244=CARTESIAN_POINT('Ctrl Pts',(-0.214387566021736,1.77026850084459,
5.70348585578341));
#29245=CARTESIAN_POINT('Ctrl Pts',(-0.231636634068633,1.78148364323829,
5.70244381361764));
#29246=CARTESIAN_POINT('Ctrl Pts',(-0.248038156418609,1.79407859961191,
5.70140177145187));
#29247=CARTESIAN_POINT('Ctrl Pts',(-0.263366101315495,1.80789867053045,
5.7003597292861));
#29248=CARTESIAN_POINT('Ctrl Pts',(-0.27867758424036,1.82170389890995,5.69931880625725));
#29249=CARTESIAN_POINT('Ctrl Pts',(-0.292917215649837,1.83673116102595,
5.6982778832284));
#29250=CARTESIAN_POINT('Ctrl Pts',(-0.305891965258325,1.85278552714212,
5.69723696019954));
#29251=CARTESIAN_POINT('Ctrl Pts',(-0.318873378360047,1.86884813836229,
5.69619550257975));
#29252=CARTESIAN_POINT('Ctrl Pts',(-0.330588136862522,1.88593834527322,
5.69515404495996));
#29253=CARTESIAN_POINT('Ctrl Pts',(-0.340883169996976,1.90382774300933,
5.69411258734017));
#29254=CARTESIAN_POINT('Ctrl Pts',(-0.351181348712877,1.92172260673636,
5.69307081150967));
#29255=CARTESIAN_POINT('Ctrl Pts',(-0.360058603164078,1.94041649218144,
5.69202903567917));
#29256=CARTESIAN_POINT('Ctrl Pts',(-0.367408050040885,1.95965679651243,
5.69098725984867));
#29257=CARTESIAN_POINT('Ctrl Pts',(-0.374773382913896,1.97893868919784,
5.68994323219608));
#29258=CARTESIAN_POINT('Ctrl Pts',(-0.380604107394695,1.99876865220429,
5.68889920454348));
#29259=CARTESIAN_POINT('Ctrl Pts',(-0.384843112551628,2.01887867899513,
5.68785517689088));
#29260=CARTESIAN_POINT('Ctrl Pts',(-0.386342393111804,2.0259913318738,5.68748591799502));
#29261=CARTESIAN_POINT('Ctrl Pts',(-0.387643029924026,2.03313894532313,
5.68711665909915));
#29262=CARTESIAN_POINT('Ctrl Pts',(-0.388744049134309,2.04030951279591,
5.68674740020328));
#29263=CARTESIAN_POINT('Ctrl Pts',(-0.391756607633146,2.05992929216021,
5.68573705087002));
#29264=CARTESIAN_POINT('Ctrl Pts',(-0.393284374731537,2.07978273465513,
5.68472670153676));
#29265=CARTESIAN_POINT('Ctrl Pts',(-0.393299880736251,2.09969371116471,
5.6837163522035));
#29266=CARTESIAN_POINT('',(-0.393067535617534,2.0998785711675,5.55871638557015));
#29267=CARTESIAN_POINT('Ctrl Pts',(-0.393615161326375,2.0996963218002,5.68371620738833));
#29268=CARTESIAN_POINT('Ctrl Pts',(-0.392664726535533,2.2104023257077,5.67810315715238));
#29269=CARTESIAN_POINT('Ctrl Pts',(-0.28609226402674,2.45334197563328,5.66586665907551));
#29270=CARTESIAN_POINT('Ctrl Pts',(0.126029412727711,2.54765121535297,5.6470067131577));
#29271=CARTESIAN_POINT('Ctrl Pts',(0.444615155104554,2.23635390471428,5.62713636963491));
#29272=CARTESIAN_POINT('Ctrl Pts',(0.355327021560618,1.79997044940816,5.60726602611212));
#29273=CARTESIAN_POINT('Ctrl Pts',(-0.0599252808592673,1.63882326143504,
5.58739568258933));
#29274=CARTESIAN_POINT('Ctrl Pts',(-0.35335079016512,1.85214103468178,5.57121248728709));
#29275=CARTESIAN_POINT('Ctrl Pts',(-0.392846519052558,2.04161642652764,
5.56165273982576));
#29276=CARTESIAN_POINT('Ctrl Pts',(-0.392686924180345,2.09987760405252,
5.55871644020536));
#29277=CARTESIAN_POINT('',(-0.39329983717694,2.10035787790198,5.43371635219978));
#29278=CARTESIAN_POINT('Ctrl Pts',(-0.393299981436727,2.09987916180092,
5.5587163522035));
#29279=CARTESIAN_POINT('Ctrl Pts',(-0.393306508722677,2.12112394583906,
5.55764730633775));
#29280=CARTESIAN_POINT('Ctrl Pts',(-0.391587338751787,2.14235300093295,
5.556578260472));
#29281=CARTESIAN_POINT('Ctrl Pts',(-0.388176079816389,2.16327891480091,
5.55550921460626));
#29282=CARTESIAN_POINT('Ctrl Pts',(-0.384761280410992,2.1842265472108,5.55443905920151));
#29283=CARTESIAN_POINT('Ctrl Pts',(-0.379651056279692,2.20486974989942,
5.55336890379676));
#29284=CARTESIAN_POINT('Ctrl Pts',(-0.372929877145995,2.22493276884738,
5.55229874839202));
#29285=CARTESIAN_POINT('Ctrl Pts',(-0.366188560547455,2.24505589902444,
5.55122538667237));
#29286=CARTESIAN_POINT('Ctrl Pts',(-0.357826919027129,2.26459474733118,
5.55015202495272));
#29287=CARTESIAN_POINT('Ctrl Pts',(-0.347977653231523,2.28329332462335,
5.54907866323307));
#29288=CARTESIAN_POINT('Ctrl Pts',(-0.34362308470784,2.29156036074603,5.54860410733663));
#29289=CARTESIAN_POINT('Ctrl Pts',(-0.338978322112813,2.29966349503001,
5.54812955144019));
#29290=CARTESIAN_POINT('Ctrl Pts',(-0.334057509852243,2.30758244172212,
5.54765499554374));
#29291=CARTESIAN_POINT('Ctrl Pts',(-0.323232348402992,2.3250031178038,5.54661103289619));
#29292=CARTESIAN_POINT('Ctrl Pts',(-0.311008564576172,2.34162664233014,
5.54556707024864));
#29293=CARTESIAN_POINT('Ctrl Pts',(-0.297527966009004,2.35721974932447,
5.54452310760108));
#29294=CARTESIAN_POINT('Ctrl Pts',(-0.284072166455519,2.37278417111824,
5.54348106543531));
#29295=CARTESIAN_POINT('Ctrl Pts',(-0.269364572260165,2.38732134878226,
5.54243902326954));
#29296=CARTESIAN_POINT('Ctrl Pts',(-0.253589172615231,2.40062837778946,
5.54139698110377));
#29297=CARTESIAN_POINT('Ctrl Pts',(-0.237830715501688,2.41392111525656,
5.54035605807492));
#29298=CARTESIAN_POINT('Ctrl Pts',(-0.22100727053391,2.4259858327749,5.53931513504607));
#29299=CARTESIAN_POINT('Ctrl Pts',(-0.203338197706689,2.43665778968174,
5.53827421201721));
#29300=CARTESIAN_POINT('Ctrl Pts',(-0.185660050504178,2.4473352274275,5.53723275439742));
#29301=CARTESIAN_POINT('Ctrl Pts',(-0.167136029301738,2.45661808138098,
5.53619129677763));
#29302=CARTESIAN_POINT('Ctrl Pts',(-0.148013226583032,2.46438574993608,
5.53514983915784));
#29303=CARTESIAN_POINT('Ctrl Pts',(-0.128884581014407,2.47215579185257,
5.53410806332734));
#29304=CARTESIAN_POINT('Ctrl Pts',(-0.109157484439478,2.47840948359018,
5.53306628749684));
#29305=CARTESIAN_POINT('Ctrl Pts',(-0.0890967241835292,2.483075271637,5.53202451166634));
#29306=CARTESIAN_POINT('Ctrl Pts',(-0.0689926021390549,2.48775114489057,
5.53098048401375));
#29307=CARTESIAN_POINT('Ctrl Pts',(-0.048554104779658,2.49083215227422,
5.52993645636115));
#29308=CARTESIAN_POINT('Ctrl Pts',(-0.0280545143236507,2.49229814456108,
5.52889242870856));
#29309=CARTESIAN_POINT('Ctrl Pts',(-0.0208040778829734,2.49281664681707,
5.52852316981269));
#29310=CARTESIAN_POINT('Ctrl Pts',(-0.0135460081095542,2.49313359681599,
5.52815391091683));
#29311=CARTESIAN_POINT('Ctrl Pts',(-0.00629233248348705,2.49324966185862,
5.52778465202096));
#29312=CARTESIAN_POINT('Ctrl Pts',(0.0142151393631943,2.4935777990289,5.52674068937341));
#29313=CARTESIAN_POINT('Ctrl Pts',(0.0348094514741135,2.49229843692212,
5.52569672672586));
#29314=CARTESIAN_POINT('Ctrl Pts',(0.055217706603292,2.48940453885063,5.5246527640783));
#29315=CARTESIAN_POINT('Ctrl Pts',(0.0755884185480483,2.48651596441648,
5.52361072191253));
#29316=CARTESIAN_POINT('Ctrl Pts',(0.0957730242944711,2.48201879282628,
5.52256867974676));
#29317=CARTESIAN_POINT('Ctrl Pts',(0.115501321409074,2.47595788960036,5.52152663758099));
#29318=CARTESIAN_POINT('Ctrl Pts',(0.135208430642493,2.4699034956893,5.52048571455214));
#29319=CARTESIAN_POINT('Ctrl Pts',(0.15445949588466,2.46228889153527,5.51944479152329));
#29320=CARTESIAN_POINT('Ctrl Pts',(0.172997256708,2.45320934185198,5.51840386849443));
#29321=CARTESIAN_POINT('Ctrl Pts',(0.191544538042147,2.44412512914861,5.51736241087464));
#29322=CARTESIAN_POINT('Ctrl Pts',(0.209377115234713,2.43357477703596,5.51632095325485));
#29323=CARTESIAN_POINT('Ctrl Pts',(0.226259828669919,2.42170076146982,5.51527949563506));
#29324=CARTESIAN_POINT('Ctrl Pts',(0.243147700510096,2.40982311787426,5.51423771980456));
#29325=CARTESIAN_POINT('Ctrl Pts',(0.259084550313592,2.39662145820717,5.51319594397406));
#29326=CARTESIAN_POINT('Ctrl Pts',(0.273866880442892,2.38227968718361,5.51215416814356));
#29327=CARTESIAN_POINT('Ctrl Pts',(0.288681162914224,2.36790691609653,5.51111014049097));
#29328=CARTESIAN_POINT('Ctrl Pts',(0.30233545700679,2.35238966654509,5.51006611283837));
#29329=CARTESIAN_POINT('Ctrl Pts',(0.314664888287206,2.33594681197083,5.50902208518577));
#29330=CARTESIAN_POINT('Ctrl Pts',(0.319025646519955,2.33013118983679,5.5086528262899));
#29331=CARTESIAN_POINT('Ctrl Pts',(0.323221068067221,2.32420004558132,5.50828356739404));
#29332=CARTESIAN_POINT('Ctrl Pts',(0.327245203315154,2.31816385334703,5.50791430849817));
#29333=CARTESIAN_POINT('Ctrl Pts',(0.338622171980128,2.30109843042402,5.50687034585062));
#29334=CARTESIAN_POINT('Ctrl Pts',(0.348694534675806,2.28308982224769,5.50582638320307));
#29335=CARTESIAN_POINT('Ctrl Pts',(0.357308650619032,2.26436367662232,5.50478242055551));
#29336=CARTESIAN_POINT('Ctrl Pts',(0.365906919967752,2.2456719797597,5.50374037838974));
#29337=CARTESIAN_POINT('Ctrl Pts',(0.37305190937884,2.22626600161468,5.50269833622397));
#29338=CARTESIAN_POINT('Ctrl Pts',(0.378635077125592,2.20639721974796,5.50165629405821));
#29339=CARTESIAN_POINT('Ctrl Pts',(0.3842122486379,2.18654977664083,5.50061537102935));
#29340=CARTESIAN_POINT('Ctrl Pts',(0.388230702590658,2.16624121349099,5.4995744480005));
#29341=CARTESIAN_POINT('Ctrl Pts',(0.390631279542963,2.14573940798291,5.49853352497165));
#29342=CARTESIAN_POINT('Ctrl Pts',(0.393033089369024,2.12522707328187,5.49749206735186));
#29343=CARTESIAN_POINT('Ctrl Pts',(0.39381526066371,2.10452202686571,5.49645060973206));
#29344=CARTESIAN_POINT('Ctrl Pts',(0.392970293612514,2.08389911995901,5.49540915211227));
#29345=CARTESIAN_POINT('Ctrl Pts',(0.392125068387046,2.06326991185515,5.49436737628178));
#29346=CARTESIAN_POINT('Ctrl Pts',(0.389651781330608,2.04272362628423,5.49332560045128));
#29347=CARTESIAN_POINT('Ctrl Pts',(0.385594905872169,2.02253091864858,5.49228382462078));
#29348=CARTESIAN_POINT('Ctrl Pts',(0.381529261385364,2.00229456401714,5.49123979696818));
#29349=CARTESIAN_POINT('Ctrl Pts',(0.375873396245463,1.98241402151128,5.49019576931559));
#29350=CARTESIAN_POINT('Ctrl Pts',(0.368722093651012,1.96314640065525,5.48915174166299));
#29351=CARTESIAN_POINT('Ctrl Pts',(0.366192771660865,1.95633169571369,5.48878248276712));
#29352=CARTESIAN_POINT('Ctrl Pts',(0.363476816867384,1.94959347460586,5.48841322387126));
#29353=CARTESIAN_POINT('Ctrl Pts',(0.360579815483704,1.94294240971625,5.48804396497539));
#29354=CARTESIAN_POINT('Ctrl Pts',(0.352389461051284,1.92413862898428,5.48700000232784));
#29355=CARTESIAN_POINT('Ctrl Pts',(0.342699852786798,1.90592122108955,5.48595603968028));
#29356=CARTESIAN_POINT('Ctrl Pts',(0.331617550872154,1.88854151718705,5.48491207703273));
#29357=CARTESIAN_POINT('Ctrl Pts',(0.320555636046073,1.87119378512266,5.48387003486696));
#29358=CARTESIAN_POINT('Ctrl Pts',(0.308106454039638,1.85468134348551,5.48282799270119));
#29359=CARTESIAN_POINT('Ctrl Pts',(0.294422696090562,1.8392315854503,5.48178595053542));
#29360=CARTESIAN_POINT('Ctrl Pts',(0.280753634282543,1.8237984202125,5.48074502750656));
#29361=CARTESIAN_POINT('Ctrl Pts',(0.26585309250733,1.80942623999562,5.47970410447771));
#29362=CARTESIAN_POINT('Ctrl Pts',(0.24991428304389,1.79630979414762,5.47866318144886));
#29363=CARTESIAN_POINT('Ctrl Pts',(0.233967287823335,1.78318661203491,5.47762172382906));
#29364=CARTESIAN_POINT('Ctrl Pts',(0.216981517540274,1.77132093266452,5.47658026620927));
#29365=CARTESIAN_POINT('Ctrl Pts',(0.199184012240271,1.7608678439489,5.47553880858948));
#29366=CARTESIAN_POINT('Ctrl Pts',(0.181381069026487,1.75041156135896,5.47449703275898));
#29367=CARTESIAN_POINT('Ctrl Pts',(0.162766549276754,1.74136906977133,5.47345525692848));
#29368=CARTESIAN_POINT('Ctrl Pts',(0.14359209916996,1.73384948579039,5.47241348109798));
#29369=CARTESIAN_POINT('Ctrl Pts',(0.12437620305414,1.72631364805803,5.47136945344538));
#29370=CARTESIAN_POINT('Ctrl Pts',(0.104598664971117,1.72030750385541,5.47032542579279));
#29371=CARTESIAN_POINT('Ctrl Pts',(0.0845269750702698,1.71589053580331,
5.46928139814019));
#29372=CARTESIAN_POINT('Ctrl Pts',(0.0774278814471054,1.71432831209981,
5.46891213924432));
#29373=CARTESIAN_POINT('Ctrl Pts',(0.0702920690920527,1.71296441468007,
5.46854288034846));
#29374=CARTESIAN_POINT('Ctrl Pts',(0.0631315354551739,1.71179992371063,
5.46817362145259));
#29375=CARTESIAN_POINT('Ctrl Pts',(0.042887393101039,1.70850769408768,5.46712965880504));
#29376=CARTESIAN_POINT('Ctrl Pts',(0.0223247103380108,1.70679347814184,
5.46608569615748));
#29377=CARTESIAN_POINT('Ctrl Pts',(0.00171249385301841,1.70670372825972,
5.46504173350993));
#29378=CARTESIAN_POINT('Ctrl Pts',(-0.0188618042386542,1.70661414348218,
5.46399969134416));
#29379=CARTESIAN_POINT('Ctrl Pts',(-0.039484727974799,1.70814315558904,
5.46295764917839));
#29380=CARTESIAN_POINT('Ctrl Pts',(-0.0598824265768568,1.71128547108801,
5.46191560701263));
#29381=CARTESIAN_POINT('Ctrl Pts',(-0.0802582183710648,1.7144244117895,
5.46087468398377));
#29382=CARTESIAN_POINT('Ctrl Pts',(-0.10040853732107,1.71917313325891,5.45983376095492));
#29383=CARTESIAN_POINT('Ctrl Pts',(-0.12006504539051,1.72547460049367,5.45879283792607));
#29384=CARTESIAN_POINT('Ctrl Pts',(-0.139731648530185,1.73177930399777,
5.45775138030628));
#29385=CARTESIAN_POINT('Ctrl Pts',(-0.158903228560105,1.73963813712911,
5.45670992268648));
#29386=CARTESIAN_POINT('Ctrl Pts',(-0.177326483907724,1.74894415244163,
5.45566846506669));
#29387=CARTESIAN_POINT('Ctrl Pts',(-0.195755368363045,1.75825301114754,
5.45462668923619));
#29388=CARTESIAN_POINT('Ctrl Pts',(-0.213434833073728,1.76900956855079,
5.4535849134057));
#29389=CARTESIAN_POINT('Ctrl Pts',(-0.230136910221563,1.78106130282816,
5.4525431375752));
#29390=CARTESIAN_POINT('Ctrl Pts',(-0.246875089288167,1.79313908720265,
5.4514991099226));
#29391=CARTESIAN_POINT('Ctrl Pts',(-0.26263110159182,1.80651716094648,5.45045508227001));
#29392=CARTESIAN_POINT('Ctrl Pts',(-0.277210135828873,1.8210028125702,5.44941105461741));
#29393=CARTESIAN_POINT('Ctrl Pts',(-0.282366549140134,1.82612619767517,
5.44904179572154));
#29394=CARTESIAN_POINT('Ctrl Pts',(-0.287376082674135,1.83138781414826,
5.44867253682567));
#29395=CARTESIAN_POINT('Ctrl Pts',(-0.292231333771012,1.83677815903232,
5.44830327792981));
#29396=CARTESIAN_POINT('Ctrl Pts',(-0.30582172046043,1.85186633262047,5.44726968129738));
#29397=CARTESIAN_POINT('Ctrl Pts',(-0.318285162804529,1.86805964649283,
5.44623608466495));
#29398=CARTESIAN_POINT('Ctrl Pts',(-0.329438218792112,1.88516203780737,
5.44520248803252));
#29399=CARTESIAN_POINT('Ctrl Pts',(-0.340571639718522,1.9022343201993,5.44417071105679));
#29400=CARTESIAN_POINT('Ctrl Pts',(-0.350398789634137,1.92021191835659,
5.44313893408107));
#29401=CARTESIAN_POINT('Ctrl Pts',(-0.358776823701344,1.93886626431819,
5.44210715710534));
#29402=CARTESIAN_POINT('Ctrl Pts',(-0.367145819706796,1.95750048633074,
5.44107649319074));
#29403=CARTESIAN_POINT('Ctrl Pts',(-0.374068469320275,1.97680933592006,
5.44004582927614));
#29404=CARTESIAN_POINT('Ctrl Pts',(-0.379448363355163,1.99654068651355,
5.43901516536154));
#29405=CARTESIAN_POINT('Ctrl Pts',(-0.384831406635258,2.01628358730874,
5.43798389812402));
#29406=CARTESIAN_POINT('Ctrl Pts',(-0.388669681058896,2.03644876007996,
5.43695263088649));
#29407=CARTESIAN_POINT('Ctrl Pts',(-0.390916911969147,2.05676971042768,
5.43592136364897));
#29408=CARTESIAN_POINT('Ctrl Pts',(-0.392518556268971,2.07125283903853,
5.43518635983381));
#29409=CARTESIAN_POINT('Ctrl Pts',(-0.393313070471383,2.08581477928863,
5.43445135601866));
#29410=CARTESIAN_POINT('Ctrl Pts',(-0.393299837177007,2.10035787782838,
5.4337163522035));
#29411=CARTESIAN_POINT('',(-0.393299995348526,2.09993951157533,5.3087163521999));
#29412=CARTESIAN_POINT('Ctrl Pts',(-0.39329983717694,2.10035787790198,5.43371635219978));
#29413=CARTESIAN_POINT('Ctrl Pts',(-0.393276057989764,2.12649067457004,
5.43239560853574));
#29414=CARTESIAN_POINT('Ctrl Pts',(-0.390643793227004,2.15250592406765,
5.43107486487169));
#29415=CARTESIAN_POINT('Ctrl Pts',(-0.385495397888704,2.17796273601298,
5.42975412120765));
#29416=CARTESIAN_POINT('Ctrl Pts',(-0.38377869031185,2.18645118708899,5.42931372560744));
#29417=CARTESIAN_POINT('Ctrl Pts',(-0.381782613840906,2.19487774264244,
5.42887333000723));
#29418=CARTESIAN_POINT('Ctrl Pts',(-0.379511737965943,2.20322659902404,
5.42843293440702));
#29419=CARTESIAN_POINT('Ctrl Pts',(-0.374128601555078,2.22301765553767,
5.42738897175947));
#29420=CARTESIAN_POINT('Ctrl Pts',(-0.36717713989106,2.24244546136991,5.42634500911192));
#29421=CARTESIAN_POINT('Ctrl Pts',(-0.358726422556043,2.26124591083232,
5.42530104646436));
#29422=CARTESIAN_POINT('Ctrl Pts',(-0.350291251226182,2.28001177484207,
5.4242590042986));
#29423=CARTESIAN_POINT('Ctrl Pts',(-0.34036254283658,2.29815188540302,5.42321696213283));
#29424=CARTESIAN_POINT('Ctrl Pts',(-0.329058476444429,2.3154191474314,5.42217491996706));
#29425=CARTESIAN_POINT('Ctrl Pts',(-0.317766550442001,2.33266786469162,
5.42113399693821));
#29426=CARTESIAN_POINT('Ctrl Pts',(-0.305102575620766,2.3490449661173,5.42009307390936));
#29427=CARTESIAN_POINT('Ctrl Pts',(-0.291229549329997,2.36432979324519,
5.4190521508805));
#29428=CARTESIAN_POINT('Ctrl Pts',(-0.277349398214499,2.37962247026193,
5.41801069326071));
#29429=CARTESIAN_POINT('Ctrl Pts',(-0.26225943770187,2.39382119663989,5.41696923564092));
#29430=CARTESIAN_POINT('Ctrl Pts',(-0.246161876094521,2.40673966283744,
5.41592777802113));
#29431=CARTESIAN_POINT('Ctrl Pts',(-0.230059395980306,2.41966207618961,
5.41488600219063));
#29432=CARTESIAN_POINT('Ctrl Pts',(-0.212949297887291,2.43130301871467,
5.41384422636013));
#29433=CARTESIAN_POINT('Ctrl Pts',(-0.195064789571651,2.4415181076742,5.41280245052964));
#29434=CARTESIAN_POINT('Ctrl Pts',(-0.177141623485433,2.45175527678033,
5.41175842287704));
#29435=CARTESIAN_POINT('Ctrl Pts',(-0.158441371620449,2.46056012550098,
5.41071439522444));
#29436=CARTESIAN_POINT('Ctrl Pts',(-0.139220101257428,2.46783508995999,
5.40967036757185));
#29437=CARTESIAN_POINT('Ctrl Pts',(-0.132421789877577,2.47040814953075,
5.40930110867597));
#29438=CARTESIAN_POINT('Ctrl Pts',(-0.125558447314126,2.47279028365725,
5.4089318497801));
#29439=CARTESIAN_POINT('Ctrl Pts',(-0.118641788434857,2.47497868744367,
5.40856259088423));
#29440=CARTESIAN_POINT('Ctrl Pts',(-0.099087124765188,2.48116570646021,
5.40751862823667));
#29441=CARTESIAN_POINT('Ctrl Pts',(-0.0789889259748524,2.48583741536663,
5.40647466558912));
#29442=CARTESIAN_POINT('Ctrl Pts',(-0.0586066454681531,2.48890892392303,
5.40543070294157));
#29443=CARTESIAN_POINT('Ctrl Pts',(-0.038261860362759,2.49197478210847,
5.4043886607758));
#29444=CARTESIAN_POINT('Ctrl Pts',(-0.0176347413639124,2.49344611594472,
5.40334661861003));
#29445=CARTESIAN_POINT('Ctrl Pts',(0.00300297709885603,2.49328853546543,
5.40230457644426));
#29446=CARTESIAN_POINT('Ctrl Pts',(0.0236185309762048,2.4931311242251,5.4012636534154));
#29447=CARTESIAN_POINT('Ctrl Pts',(0.0442439294710951,2.4913482483719,5.40022273038655));
#29448=CARTESIAN_POINT('Ctrl Pts',(0.0646054055865343,2.48795751258224,
5.3991818073577));
#29449=CARTESIAN_POINT('Ctrl Pts',(0.0849773388254204,2.48456503539906,
5.39814034973791));
#29450=CARTESIAN_POINT('Ctrl Pts',(0.10508435046725,2.47956315356667,5.39709889211811));
#29451=CARTESIAN_POINT('Ctrl Pts',(0.124660329105881,2.47302103472487,5.39605743449832));
#29452=CARTESIAN_POINT('Ctrl Pts',(0.144242289059426,2.46647691698055,5.39501565866782));
#29453=CARTESIAN_POINT('Ctrl Pts',(0.163292207216022,2.45839189268546,5.39397388283733));
#29454=CARTESIAN_POINT('Ctrl Pts',(0.181562444411897,2.44888389011128,5.39293210700683));
#29455=CARTESIAN_POINT('Ctrl Pts',(0.199872173140076,2.43935533577377,5.39188807935423));
#29456=CARTESIAN_POINT('Ctrl Pts',(0.217398231816419,2.42839805289518,5.39084405170164));
#29457=CARTESIAN_POINT('Ctrl Pts',(0.233919973141138,2.41617453434084,5.38980002404904));
#29458=CARTESIAN_POINT('Ctrl Pts',(0.239763496484775,2.41185123605105,5.38943076515317));
#29459=CARTESIAN_POINT('Ctrl Pts',(0.245481688851205,2.40736990698496,5.38906150625731));
#29460=CARTESIAN_POINT('Ctrl Pts',(0.251065850364198,2.40273887887237,5.38869224736144));
#29461=CARTESIAN_POINT('Ctrl Pts',(0.266853299502816,2.3896461127307,5.38764828471389));
#29462=CARTESIAN_POINT('Ctrl Pts',(0.281660874152024,2.37527606778538,5.38660432206633));
#29463=CARTESIAN_POINT('Ctrl Pts',(0.295276750262427,2.35980094448339,5.38556035941878));
#29464=CARTESIAN_POINT('Ctrl Pts',(0.308867578501532,2.34435428933824,5.38451831725301));
#29465=CARTESIAN_POINT('Ctrl Pts',(0.321270534556845,2.32780709795903,5.38347627508724));
#29466=CARTESIAN_POINT('Ctrl Pts',(0.332309607972287,2.31036923360916,5.38243423292147));
#29467=CARTESIAN_POINT('Ctrl Pts',(0.343336825596299,2.29295009725166,5.38139330989262));
#29468=CARTESIAN_POINT('Ctrl Pts',(0.353002652540214,2.27464278999824,5.38035238686376));
#29469=CARTESIAN_POINT('Ctrl Pts',(0.361173696109049,2.25568702977104,5.37931146383491));
#29470=CARTESIAN_POINT('Ctrl Pts',(0.369348936112899,2.23672153435943,5.37827000621512));
#29471=CARTESIAN_POINT('Ctrl Pts',(0.376027553024985,2.21710758995318,5.37722854859533));
#29472=CARTESIAN_POINT('Ctrl Pts',(0.381123653322771,2.19710638948032,5.37618709097553));
#29473=CARTESIAN_POINT('Ctrl Pts',(0.386221310701368,2.17709907776875,5.37514531514504));
#29474=CARTESIAN_POINT('Ctrl Pts',(0.389735342425015,2.15670499576757,5.37410353931454));
#29475=CARTESIAN_POINT('Ctrl Pts',(0.391630853142078,2.13619619962383,5.37306176348404));
#29476=CARTESIAN_POINT('Ctrl Pts',(0.393530461048571,2.11564307325181,5.37201773583144));
#29477=CARTESIAN_POINT('Ctrl Pts',(0.393804553658141,2.09497547411574,5.37097370817884));
#29478=CARTESIAN_POINT('Ctrl Pts',(0.392470317511078,2.07446688673988,5.36992968052625));
#29479=CARTESIAN_POINT('Ctrl Pts',(0.391998415674701,2.06721326820657,5.36956042163038));
#29480=CARTESIAN_POINT('Ctrl Pts',(0.391325794809628,2.05997948528822,5.36919116273452));
#29481=CARTESIAN_POINT('Ctrl Pts',(0.39045475098324,2.05277736311242,5.36882190383865));
#29482=CARTESIAN_POINT('Ctrl Pts',(0.387992150273246,2.03241564232837,5.3677779411911));
#29483=CARTESIAN_POINT('Ctrl Pts',(0.383925166909935,2.01218640346367,5.36673397854354));
#29484=CARTESIAN_POINT('Ctrl Pts',(0.378283925926897,1.99236096718507,5.36569001589599));
#29485=CARTESIAN_POINT('Ctrl Pts',(0.372653062614526,1.97257200193281,5.36464797373022));
#29486=CARTESIAN_POINT('Ctrl Pts',(0.365453832055553,1.95318608073188,5.36360593156445));
#29487=CARTESIAN_POINT('Ctrl Pts',(0.356767413399143,1.93446479910157,5.36256388939868));
#29488=CARTESIAN_POINT('Ctrl Pts',(0.348090323819911,1.91576362383363,5.36152296636983));
#29489=CARTESIAN_POINT('Ctrl Pts',(0.337929498875328,1.89772634727018,5.36048204334097));
#29490=CARTESIAN_POINT('Ctrl Pts',(0.326414289810293,1.88059489202017,5.35944112031212));
#29491=CARTESIAN_POINT('Ctrl Pts',(0.314893166834003,1.86345463850124,5.35839966269233));
#29492=CARTESIAN_POINT('Ctrl Pts',(0.3020166672111,1.84722175531644,5.35735820507254));
#29493=CARTESIAN_POINT('Ctrl Pts',(0.287957910916233,1.83210985172881,5.35631674745275));
#29494=CARTESIAN_POINT('Ctrl Pts',(0.273894859058409,1.81699333079581,5.35527497162225));
#29495=CARTESIAN_POINT('Ctrl Pts',(0.258649358634886,1.80299898492108,5.35423319579175));
#29496=CARTESIAN_POINT('Ctrl Pts',(0.242431269840718,1.79030342364918,5.35319141996125));
#29497=CARTESIAN_POINT('Ctrl Pts',(0.226178125279587,1.7775804206335,5.35214739230865));
#29498=CARTESIAN_POINT('Ctrl Pts',(0.208948809167448,1.76616221380773,5.35110336465606));
#29499=CARTESIAN_POINT('Ctrl Pts',(0.190982575573689,1.75618239453565,5.35005933700346));
#29500=CARTESIAN_POINT('Ctrl Pts',(0.184628154248526,1.75265266327212,5.34969007810759));
#29501=CARTESIAN_POINT('Ctrl Pts',(0.178181758226575,1.74930243753846,5.34932081921173));
#29502=CARTESIAN_POINT('Ctrl Pts',(0.171654573189592,1.74613618791532,5.34895156031586));
#29503=CARTESIAN_POINT('Ctrl Pts',(0.153201023529593,1.73718461931027,5.34790759766831));
#29504=CARTESIAN_POINT('Ctrl Pts',(0.13399038571981,1.72965375922237,5.34686363502075));
#29505=CARTESIAN_POINT('Ctrl Pts',(0.114267098259657,1.72366514876334,5.3458196723732));
#29506=CARTESIAN_POINT('Ctrl Pts',(0.0945800939120914,1.71768755499856,
5.34477763020743));
#29507=CARTESIAN_POINT('Ctrl Pts',(0.0743829906899506,1.7132468475229,5.34373558804166));
#29508=CARTESIAN_POINT('Ctrl Pts',(0.0539396865298279,1.71041637583561,
5.34269354587589));
#29509=CARTESIAN_POINT('Ctrl Pts',(0.033518338157218,1.70758894403044,5.34165262284704));
#29510=CARTESIAN_POINT('Ctrl Pts',(0.0128520349393816,1.70636844385046,
5.34061169981818));
#29511=CARTESIAN_POINT('Ctrl Pts',(-0.00778579009651449,1.70677707153248,
5.33957077678933));
#29512=CARTESIAN_POINT('Ctrl Pts',(-0.0284342141814631,1.70718590907503,
5.33852931916954));
#29513=CARTESIAN_POINT('Ctrl Pts',(-0.0490533949124762,1.70922554752625,
5.33748786154975));
#29514=CARTESIAN_POINT('Ctrl Pts',(-0.069370012826302,1.71286605506559,
5.33644640392995));
#29515=CARTESIAN_POINT('Ctrl Pts',(-0.0896928383526334,1.7165076749387,
5.33540462809946));
#29516=CARTESIAN_POINT('Ctrl Pts',(-0.10971219977222,1.72175097237232,5.33436285226896));
#29517=CARTESIAN_POINT('Ctrl Pts',(-0.129165999502396,1.72851509509464,
5.33332107643846));
#29518=CARTESIAN_POINT('Ctrl Pts',(-0.148661849062148,1.73529383862171,
5.33227704878586));
#29519=CARTESIAN_POINT('Ctrl Pts',(-0.1675890219227,1.7435996744204,5.33123302113327));
#29520=CARTESIAN_POINT('Ctrl Pts',(-0.185705679522728,1.75330374880452,
5.33018899348067));
#29521=CARTESIAN_POINT('Ctrl Pts',(-0.19211330384717,1.75673595271556,5.3298197345848));
#29522=CARTESIAN_POINT('Ctrl Pts',(-0.19841978427341,1.76034266018519,5.32945047568894));
#29523=CARTESIAN_POINT('Ctrl Pts',(-0.204615306845539,1.764116886098,5.32908121679307));
#29524=CARTESIAN_POINT('Ctrl Pts',(-0.222131185866424,1.77478731522107,
5.32803725414552));
#29525=CARTESIAN_POINT('Ctrl Pts',(-0.238862333224376,1.78686337280658,
5.32699329149796));
#29526=CARTESIAN_POINT('Ctrl Pts',(-0.254574236000076,1.80020532298759,
5.32594932885041));
#29527=CARTESIAN_POINT('Ctrl Pts',(-0.270257235037567,1.81352272921356,
5.32490728668464));
#29528=CARTESIAN_POINT('Ctrl Pts',(-0.284924118303874,1.82810098002436,
5.32386524451887));
#29529=CARTESIAN_POINT('Ctrl Pts',(-0.298370359505342,1.84375789071924,
5.3228232023531));
#29530=CARTESIAN_POINT('Ctrl Pts',(-0.311802159654996,1.859397986138,5.32178227932425));
#29531=CARTESIAN_POINT('Ctrl Pts',(-0.324015421406848,1.87611390510052,
5.3207413562954));
#29532=CARTESIAN_POINT('Ctrl Pts',(-0.334843467529343,1.89368775544596,
5.31970043326654));
#29533=CARTESIAN_POINT('Ctrl Pts',(-0.345677074654112,1.9112706312629,5.31865897564675));
#29534=CARTESIAN_POINT('Ctrl Pts',(-0.355123645220509,1.92971170074283,
5.31761751802696));
#29535=CARTESIAN_POINT('Ctrl Pts',(-0.36306039367513,1.94876494935214,5.31657606040717));
#29536=CARTESIAN_POINT('Ctrl Pts',(-0.370999567152417,1.96782401955956,
5.31553428457667));
#29537=CARTESIAN_POINT('Ctrl Pts',(-0.377427750855548,1.98749494871666,
5.31449250874617));
#29538=CARTESIAN_POINT('Ctrl Pts',(-0.382271048664976,2.00751359368761,
5.31345073291567));
#29539=CARTESIAN_POINT('Ctrl Pts',(-0.387124815372529,2.02757550941396,
5.31240670526308));
#29540=CARTESIAN_POINT('Ctrl Pts',(-0.390386740583849,2.04798591422924,
5.31136267761048));
#29541=CARTESIAN_POINT('Ctrl Pts',(-0.392034255202344,2.06847171511256,
5.31031864995788));
#29542=CARTESIAN_POINT('Ctrl Pts',(-0.392616959527691,2.07571727436218,
5.30994939106201));
#29543=CARTESIAN_POINT('Ctrl Pts',(-0.39299818711695,2.08297225194062,5.30958013216615));
#29544=CARTESIAN_POINT('Ctrl Pts',(-0.393178498708552,2.09022461492885,
5.30921087327028));
#29545=CARTESIAN_POINT('Ctrl Pts',(-0.393258991358046,2.09346213231099,
5.30904603291468));
#29546=CARTESIAN_POINT('Ctrl Pts',(-0.393299497219904,2.09670064799264,
5.30888119255909));
#29547=CARTESIAN_POINT('Ctrl Pts',(-0.393299995348515,2.09993951150465,
5.3087163522035));
#29548=CARTESIAN_POINT('',(-0.393222743871143,2.09967523239219,5.18371635531477));
#29549=CARTESIAN_POINT('Ctrl Pts',(-0.393299995348526,2.09993951157533,
5.3087163521999));
#29550=CARTESIAN_POINT('Ctrl Pts',(-0.393303136849036,2.12036576904277,
5.30767676793465));
#29551=CARTESIAN_POINT('Ctrl Pts',(-0.391710695555704,2.14085529073421,
5.30663718366939));
#29552=CARTESIAN_POINT('Ctrl Pts',(-0.38851918392407,2.16113700780194,5.30559759940414));
#29553=CARTESIAN_POINT('Ctrl Pts',(-0.3853334959826,2.18138171593791,5.30455991211354));
#29554=CARTESIAN_POINT('Ctrl Pts',(-0.380554582847914,2.20141863733601,
5.30352222482293));
#29555=CARTESIAN_POINT('Ctrl Pts',(-0.374230820545827,2.22098009321205,
5.30248453753233));
#29556=CARTESIAN_POINT('Ctrl Pts',(-0.367913650014553,2.24052115859463,
5.30144793190743));
#29557=CARTESIAN_POINT('Ctrl Pts',(-0.360055026981877,2.25958703034488,
5.30041132628253));
#29558=CARTESIAN_POINT('Ctrl Pts',(-0.350753523762467,2.27792373525815,
5.29937472065763));
#29559=CARTESIAN_POINT('Ctrl Pts',(-0.341446999305944,2.29627033888791,
5.29833755544117));
#29560=CARTESIAN_POINT('Ctrl Pts',(-0.330696363142974,2.31388632122879,
5.29730039022472));
#29561=CARTESIAN_POINT('Ctrl Pts',(-0.318646999340026,2.33054062507853,
5.29626322500827));
#29562=CARTESIAN_POINT('Ctrl Pts',(-0.306593243899986,2.34720099892994,
5.29522568177574));
#29563=CARTESIAN_POINT('Ctrl Pts',(-0.293240286425889,2.36289841977707,
5.29418813854321));
#29564=CARTESIAN_POINT('Ctrl Pts',(-0.27877432215448,2.37743425763108,5.29315059531067));
#29565=CARTESIAN_POINT('Ctrl Pts',(-0.264277792181525,2.39200080882526,
5.29211085981248));
#29566=CARTESIAN_POINT('Ctrl Pts',(-0.248664130199837,2.40540040086757,
5.29107112431428));
#29567=CARTESIAN_POINT('Ctrl Pts',(-0.232153588232405,2.41747378076121,
5.29003138881609));
#29568=CARTESIAN_POINT('Ctrl Pts',(-0.228496742279588,2.42014785957025,
5.28980110245989));
#29569=CARTESIAN_POINT('Ctrl Pts',(-0.224796006455495,2.42275705217892,
5.28957081610369));
#29570=CARTESIAN_POINT('Ctrl Pts',(-0.221053944425669,2.42529992876398,
5.28934052974749));
#29571=CARTESIAN_POINT('Ctrl Pts',(-0.204089965106973,2.43682761201864,
5.28829656709993));
#29572=CARTESIAN_POINT('Ctrl Pts',(-0.186171281688737,2.44705909496488,
5.28725260445238));
#29573=CARTESIAN_POINT('Ctrl Pts',(-0.167522172214379,2.45583874411955,
5.28620864180483));
#29574=CARTESIAN_POINT('Ctrl Pts',(-0.148907369786457,2.46460224216353,
5.28516659963906));
#29575=CARTESIAN_POINT('Ctrl Pts',(-0.129565441336004,2.47191884419368,
5.28412455747329));
#29576=CARTESIAN_POINT('Ctrl Pts',(-0.109746893124813,2.47767778522101,
5.28308251530752));
#29577=CARTESIAN_POINT('Ctrl Pts',(-0.0899496297230533,2.48343054123616,
5.28204159227866));
#29578=CARTESIAN_POINT('Ctrl Pts',(-0.0696774576688189,2.48762872531793,
5.28100066924981));
#29579=CARTESIAN_POINT('Ctrl Pts',(-0.0491977201192234,2.49021080755801,
5.27995974622096));
#29580=CARTESIAN_POINT('Ctrl Pts',(-0.0287074647101889,2.49279421588822,
5.27891828860117));
#29581=CARTESIAN_POINT('Ctrl Pts',(-0.00801015882493114,2.49375975621462,
5.27787683098138));
#29582=CARTESIAN_POINT('Ctrl Pts',(0.0126194235258416,2.49309749445891,
5.27683537336158));
#29583=CARTESIAN_POINT('Ctrl Pts',(0.0332553091133903,2.49243503035337,
5.27579359753109));
#29584=CARTESIAN_POINT('Ctrl Pts',(0.0538226963536793,2.49014383378103,
5.27475182170059));
#29585=CARTESIAN_POINT('Ctrl Pts',(0.0740505465286713,2.48626597903363,
5.27371004587009));
#29586=CARTESIAN_POINT('Ctrl Pts',(0.0943221196608452,2.48237974221518,
5.2726660182175));
#29587=CARTESIAN_POINT('Ctrl Pts',(0.114251980371752,2.47690019544089,5.2716219905649));
#29588=CARTESIAN_POINT('Ctrl Pts',(0.133582189659656,2.4699198407841,5.2705779629123));
#29589=CARTESIAN_POINT('Ctrl Pts',(0.140419031309186,2.46745098083875,5.27020870401643));
#29590=CARTESIAN_POINT('Ctrl Pts',(0.147181045268516,2.46479481793859,5.26983944512057));
#29591=CARTESIAN_POINT('Ctrl Pts',(0.153857510090674,2.4619568435445,5.2694701862247));
#29592=CARTESIAN_POINT('Ctrl Pts',(0.17273310109213,2.4539333692415,5.26842622357715));
#29593=CARTESIAN_POINT('Ctrl Pts',(0.191035622246087,2.44440550599042,5.26738226092959));
#29594=CARTESIAN_POINT('Ctrl Pts',(0.208512808376046,2.43347758356917,5.26633829828204));
#29595=CARTESIAN_POINT('Ctrl Pts',(0.225957843338845,2.42256976423877,5.26529625611627));
#29596=CARTESIAN_POINT('Ctrl Pts',(0.242579908681752,2.41026733337383,5.2642542139505));
#29597=CARTESIAN_POINT('Ctrl Pts',(0.258150267652994,2.39672096203451,5.26321217178473));
#29598=CARTESIAN_POINT('Ctrl Pts',(0.273703904303309,2.3831891392852,5.26217124875588));
#29599=CARTESIAN_POINT('Ctrl Pts',(0.28820750567303,2.36841648696108,5.26113032572702));
#29600=CARTESIAN_POINT('Ctrl Pts',(0.30146461863205,2.3525944847241,5.26008940269817));
#29601=CARTESIAN_POINT('Ctrl Pts',(0.314728540098761,2.33676435671915,5.25904794507838));
#29602=CARTESIAN_POINT('Ctrl Pts',(0.326744209344882,2.31988435578319,5.25800648745858));
#29603=CARTESIAN_POINT('Ctrl Pts',(0.337354533482663,2.30218013932801,5.25696502983879));
#29604=CARTESIAN_POINT('Ctrl Pts',(0.347968099537041,2.28447051346287,5.25592325400829));
#29605=CARTESIAN_POINT('Ctrl Pts',(0.357175118778837,2.26593681992092,5.25488147817779));
#29606=CARTESIAN_POINT('Ctrl Pts',(0.364864249870397,2.24682972848341,5.2538397023473));
#29607=CARTESIAN_POINT('Ctrl Pts',(0.3725700011933,2.22768133663417,5.2527956746947));
#29608=CARTESIAN_POINT('Ctrl Pts',(0.378751093870111,2.20795777523849,5.2517516470421));
#29609=CARTESIAN_POINT('Ctrl Pts',(0.383345678257984,2.18792599707098,5.25070761938951));
#29610=CARTESIAN_POINT('Ctrl Pts',(0.384970722531286,2.18084101970479,5.25033836049364));
#29611=CARTESIAN_POINT('Ctrl Pts',(0.386397773545883,2.17371756832646,5.24996910159778));
#29612=CARTESIAN_POINT('Ctrl Pts',(0.387625644907437,2.16656763034759,5.24959984270191));
#29613=CARTESIAN_POINT('Ctrl Pts',(0.391097062527484,2.14635344386255,5.24855588005436));
#29614=CARTESIAN_POINT('Ctrl Pts',(0.392993349921659,2.12580675184556,5.24751191740681));
#29615=CARTESIAN_POINT('Ctrl Pts',(0.393265673737016,2.1051961389676,5.24646795475925));
#29616=CARTESIAN_POINT('Ctrl Pts',(0.393537496583371,2.08462344153295,5.24542591259349));
#29617=CARTESIAN_POINT('Ctrl Pts',(0.392191216756465,2.0639877832668,5.24438387042772));
#29618=CARTESIAN_POINT('Ctrl Pts',(0.389229701844604,2.04356305109274,5.24334182826195));
#29619=CARTESIAN_POINT('Ctrl Pts',(0.386271367553231,2.02316025476014,5.24230090523309));
#29620=CARTESIAN_POINT('Ctrl Pts',(0.381701318468743,2.00296866342249,5.24125998220424));
#29621=CARTESIAN_POINT('Ctrl Pts',(0.375574210490237,1.98325710978978,5.24021905917539));
#29622=CARTESIAN_POINT('Ctrl Pts',(0.369443955788769,1.96353543281689,5.23917760155559));
#29623=CARTESIAN_POINT('Ctrl Pts',(0.361755247648095,1.9442949934727,5.2381361439358));
#29624=CARTESIAN_POINT('Ctrl Pts',(0.35261278564167,1.92579003070426,5.23709468631601));
#29625=CARTESIAN_POINT('Ctrl Pts',(0.343467530214528,1.90727941386296,5.23605291048551));
#29626=CARTESIAN_POINT('Ctrl Pts',(0.332867994725971,1.88950536404161,5.23501113465502));
#29627=CARTESIAN_POINT('Ctrl Pts',(0.32096467573827,1.87269719111232,5.23396935882452));
#29628=CARTESIAN_POINT('Ctrl Pts',(0.309035627456456,1.85585268693583,5.23292533117192));
#29629=CARTESIAN_POINT('Ctrl Pts',(0.295797641047986,1.83997879337889,5.23188130351933));
#29630=CARTESIAN_POINT('Ctrl Pts',(0.281441694856146,1.82527202108904,5.23083727586673));
#29631=CARTESIAN_POINT('Ctrl Pts',(0.276364184862279,1.82007042850285,5.23046801697086));
#29632=CARTESIAN_POINT('Ctrl Pts',(0.271147147901713,1.81501448551558,5.230098758075));
#29633=CARTESIAN_POINT('Ctrl Pts',(0.265800020988035,1.81011167867132,5.22972949917913));
#29634=CARTESIAN_POINT('Ctrl Pts',(0.250682712151121,1.79625054419126,5.22868553653158));
#29635=CARTESIAN_POINT('Ctrl Pts',(0.234433180257581,1.78353381615442,5.22764157388402));
#29636=CARTESIAN_POINT('Ctrl Pts',(0.217250821731293,1.7721479442537,5.22659761123647));
#29637=CARTESIAN_POINT('Ctrl Pts',(0.20010007200502,1.76078301789123,5.2255555690707));
#29638=CARTESIAN_POINT('Ctrl Pts',(0.182020475470047,1.75074453939185,5.22451352690493));
#29639=CARTESIAN_POINT('Ctrl Pts',(0.16324387343287,1.74217835757653,5.22347148473916));
#29640=CARTESIAN_POINT('Ctrl Pts',(0.144487437171302,1.7336213757059,5.2224305617103));
#29641=CARTESIAN_POINT('Ctrl Pts',(0.125036135511626,1.72653388157008,5.22138963868145));
#29642=CARTESIAN_POINT('Ctrl Pts',(0.105145594035449,1.72101544351394,5.22034871565259));
#29643=CARTESIAN_POINT('Ctrl Pts',(0.085244837295583,1.71549417133185,5.2193072580328));
#29644=CARTESIAN_POINT('Ctrl Pts',(0.0649050947640875,1.71154377732843,
5.21826580041301));
#29645=CARTESIAN_POINT('Ctrl Pts',(0.0443968108705369,1.70921385236356,
5.21722434279322));
#29646=CARTESIAN_POINT('Ctrl Pts',(0.0238822608021649,1.70688321550505,
5.21618256696272));
#29647=CARTESIAN_POINT('Ctrl Pts',(0.00319980139753719,1.70617408039698,
5.21514079113222));
#29648=CARTESIAN_POINT('Ctrl Pts',(-0.0173762929887746,1.70708403641241,
5.21409901530172));
#29649=CARTESIAN_POINT('Ctrl Pts',(-0.0379968630700355,1.7079959593184,
5.21305498764912));
#29650=CARTESIAN_POINT('Ctrl Pts',(-0.0585098782231471,1.71053386990322,
5.21201095999652));
#29651=CARTESIAN_POINT('Ctrl Pts',(-0.0786467287493022,1.71464356492069,
5.21096693234393));
#29652=CARTESIAN_POINT('Ctrl Pts',(-0.0857688688315183,1.7160971101795,
5.21059767344806));
#29653=CARTESIAN_POINT('Ctrl Pts',(-0.0928440725913599,1.71774681496967,
5.21022841455219));
#29654=CARTESIAN_POINT('Ctrl Pts',(-0.0998609367825471,1.7195887970828,
5.20985915565633));
#29655=CARTESIAN_POINT('Ctrl Pts',(-0.119698899254308,1.72479641847012,
5.20881519300878));
#29656=CARTESIAN_POINT('Ctrl Pts',(-0.139187517097244,1.73157552116103,
5.20777123036122));
#29657=CARTESIAN_POINT('Ctrl Pts',(-0.158062083184193,1.73985937765996,
5.20672726771367));
#29658=CARTESIAN_POINT('Ctrl Pts',(-0.176901927472966,1.74812799511222,
5.2056852255479));
#29659=CARTESIAN_POINT('Ctrl Pts',(-0.195129272209971,1.75789563378735,
5.20464318338213));
#29660=CARTESIAN_POINT('Ctrl Pts',(-0.212495985206887,1.76904630796597,
5.20360114121636));
#29661=CARTESIAN_POINT('Ctrl Pts',(-0.229844046626877,1.78018500649571,
5.20256021818751));
#29662=CARTESIAN_POINT('Ctrl Pts',(-0.246332679644588,1.79270342055612,
5.20151929515866));
#29663=CARTESIAN_POINT('Ctrl Pts',(-0.261739790666748,1.80644051372554,
5.2004783721298));
#29664=CARTESIAN_POINT('Ctrl Pts',(-0.277154814379576,1.82018466190798,
5.19943691451001));
#29665=CARTESIAN_POINT('Ctrl Pts',(-0.291486646535155,1.83514826194588,
5.19839545689022));
#29666=CARTESIAN_POINT('Ctrl Pts',(-0.304547193794242,1.85113076374921,
5.19735399927043));
#29667=CARTESIAN_POINT('Ctrl Pts',(-0.31761173161991,1.86711814890362,5.19631222343993));
#29668=CARTESIAN_POINT('Ctrl Pts',(-0.329403774099449,1.88412446343047,
5.19527044760943));
#29669=CARTESIAN_POINT('Ctrl Pts',(-0.339776878467228,1.90191778762578,
5.19422867177894));
#29670=CARTESIAN_POINT('Ctrl Pts',(-0.35017240453549,1.91974957249511,5.19318464412634));
#29671=CARTESIAN_POINT('Ctrl Pts',(-0.359142549625092,1.93837109976543,
5.19214061647374));
#29672=CARTESIAN_POINT('Ctrl Pts',(-0.366587485512455,1.95752717639614,
5.19109658882115));
#29673=CARTESIAN_POINT('Ctrl Pts',(-0.369220661749444,1.96430242960733,
5.19072732992528));
#29674=CARTESIAN_POINT('Ctrl Pts',(-0.37166349606096,1.97114440261701,5.19035807102941));
#29675=CARTESIAN_POINT('Ctrl Pts',(-0.373913079894079,1.97804140586197,
5.18998881213354));
#29676=CARTESIAN_POINT('Ctrl Pts',(-0.381478973819856,2.00123769407711,
5.18874690525452));
#29677=CARTESIAN_POINT('Ctrl Pts',(-0.386891989129394,2.02516888945576,
5.1875049983755));
#29678=CARTESIAN_POINT('Ctrl Pts',(-0.390039890821214,2.04946512522846,
5.18626309149648));
#29679=CARTESIAN_POINT('Ctrl Pts',(-0.392191654911472,2.06607293982444,
5.18541417978088));
#29680=CARTESIAN_POINT('Ctrl Pts',(-0.393285969585091,2.08285087349683,
5.18456526806529));
#29681=CARTESIAN_POINT('Ctrl Pts',(-0.393299865841963,2.09967514819741,
5.1837163563497));
#29682=CARTESIAN_POINT('',(-0.393112574114025,2.1002161969804,5.05871634925479));
#29683=CARTESIAN_POINT('Ctrl Pts',(-0.392990894347882,2.09967548550446,
5.1837163522035));
#29684=CARTESIAN_POINT('Ctrl Pts',(-0.392294416640166,2.1894360675245,5.17918372433925));
#29685=CARTESIAN_POINT('Ctrl Pts',(-0.317199300604699,2.41141571974295,
5.16802764863407));
#29686=CARTESIAN_POINT('Ctrl Pts',(0.0517462396427426,2.56216593358049,
5.15024812508798));
#29687=CARTESIAN_POINT('Ctrl Pts',(0.416608566264656,2.30666960587948,5.13037778156518));
#29688=CARTESIAN_POINT('Ctrl Pts',(0.399289249473655,1.86158205031028,5.11050743804239));
#29689=CARTESIAN_POINT('Ctrl Pts',(0.015676404613339,1.63521050590846,5.0906370945196));
#29690=CARTESIAN_POINT('Ctrl Pts',(-0.330107445811104,1.80898222584714,
5.07337339923997));
#29691=CARTESIAN_POINT('Ctrl Pts',(-0.39237518151986,2.02055869281699,5.06273315180127));
#29692=CARTESIAN_POINT('Ctrl Pts',(-0.392771469173745,2.100215950882,5.0587163522035));
#29693=CARTESIAN_POINT('',(-0.393299933199252,2.10022922797308,4.93371635220805));
#29694=CARTESIAN_POINT('Ctrl Pts',(-0.393299940503932,2.1002163321604,5.05871634763509));
#29695=CARTESIAN_POINT('Ctrl Pts',(-0.393287312904279,2.12317377955501,
5.05756024661416));
#29696=CARTESIAN_POINT('Ctrl Pts',(-0.391260460548536,2.14605889974054,
5.05640414559323));
#29697=CARTESIAN_POINT('Ctrl Pts',(-0.387281563959997,2.16854108415176,
5.0552480445723));
#29698=CARTESIAN_POINT('Ctrl Pts',(-0.383271022275013,2.19120207464103,
5.05408274880919));
#29699=CARTESIAN_POINT('Ctrl Pts',(-0.377277462436426,2.2134532889445,5.05291745304608));
#29700=CARTESIAN_POINT('Ctrl Pts',(-0.369413741228829,2.23497547107278,
5.05175215728296));
#29701=CARTESIAN_POINT('Ctrl Pts',(-0.367488799900917,2.24024383407191,
5.05146690734665));
#29702=CARTESIAN_POINT('Ctrl Pts',(-0.365452017723983,2.2454686187123,5.05118165741033));
#29703=CARTESIAN_POINT('Ctrl Pts',(-0.363305472136611,2.25064535809508,
5.05089640747402));
#29704=CARTESIAN_POINT('Ctrl Pts',(-0.355449507492256,2.26959127836966,
5.04985244482647));
#29705=CARTESIAN_POINT('Ctrl Pts',(-0.346084136819551,2.28797747675009,
5.04880848217892));
#29706=CARTESIAN_POINT('Ctrl Pts',(-0.335311451306619,2.30555077383131,
5.04776451953136));
#29707=CARTESIAN_POINT('Ctrl Pts',(-0.32455858330951,2.32309174293891,5.04672247736559));
#29708=CARTESIAN_POINT('Ctrl Pts',(-0.312403868846199,2.33982212780493,
5.04568043519982));
#29709=CARTESIAN_POINT('Ctrl Pts',(-0.298995946977492,2.35551186604742,
5.04463839303406));
#29710=CARTESIAN_POINT('Ctrl Pts',(-0.285602425006236,2.37118475375752,
5.0435974700052));
#29711=CARTESIAN_POINT('Ctrl Pts',(-0.270958821209181,2.3858186383141,5.04255654697635));
#29712=CARTESIAN_POINT('Ctrl Pts',(-0.255254867607614,2.3992153782188,5.0415156239475));
#29713=CARTESIAN_POINT('Ctrl Pts',(-0.239542848864775,2.41261899833995,
5.04047416632771));
#29714=CARTESIAN_POINT('Ctrl Pts',(-0.222769941696439,2.42478371470128,
5.03943270870791));
#29715=CARTESIAN_POINT('Ctrl Pts',(-0.205160403175313,2.43555044176538,
5.03839125108812));
#29716=CARTESIAN_POINT('Ctrl Pts',(-0.187545484172456,2.44632045853399,
5.03734947525763));
#29717=CARTESIAN_POINT('Ctrl Pts',(-0.169094071009059,2.45569128303871,
5.03630769942713));
#29718=CARTESIAN_POINT('Ctrl Pts',(-0.150055837400931,2.46354935794457,
5.03526592359663));
#29719=CARTESIAN_POINT('Ctrl Pts',(-0.130976452218827,2.47142441825765,
5.03422189594403));
#29720=CARTESIAN_POINT('Ctrl Pts',(-0.111308415039399,2.47777997443441,
5.03317786829144));
#29721=CARTESIAN_POINT('Ctrl Pts',(-0.091318120317115,2.48255181466273,
5.03213384063884));
#29722=CARTESIAN_POINT('Ctrl Pts',(-0.0842478151016081,2.4842395520034,
5.03176458174297));
#29723=CARTESIAN_POINT('Ctrl Pts',(-0.0771372836124449,2.48572964464515,
5.0313953228471));
#29724=CARTESIAN_POINT('Ctrl Pts',(-0.0699985022821658,2.48702080005893,
5.03102606395123));
#29725=CARTESIAN_POINT('Ctrl Pts',(-0.049815857689946,2.49067113330545,
5.02998210130367));
#29726=CARTESIAN_POINT('Ctrl Pts',(-0.0292867685314287,2.49274934336349,
5.02893813865612));
#29727=CARTESIAN_POINT('Ctrl Pts',(-0.00867937638820636,2.4932042197453,
5.02789417600856));
#29728=CARTESIAN_POINT('Ctrl Pts',(0.0118901062365955,2.49365825933299,
5.02685213384279));
#29729=CARTESIAN_POINT('Ctrl Pts',(0.0325368799399694,2.49249481741639,
5.02581009167702));
#29730=CARTESIAN_POINT('Ctrl Pts',(0.0529870431427076,2.48971433545482,
5.02476804951125));
#29731=CARTESIAN_POINT('Ctrl Pts',(0.0734152431914291,2.48693683968719,
5.02372712648239));
#29732=CARTESIAN_POINT('Ctrl Pts',(0.0936465226658073,2.48254582155789,
5.02268620345354));
#29733=CARTESIAN_POINT('Ctrl Pts',(0.113411575275055,2.47659355357418,5.02164528042468));
#29734=CARTESIAN_POINT('Ctrl Pts',(0.133186778700184,2.47063822866078,5.02060382280489));
#29735=CARTESIAN_POINT('Ctrl Pts',(0.152494567736001,2.46312024877389,5.01956236518509));
#29736=CARTESIAN_POINT('Ctrl Pts',(0.171079786008797,2.45414205739955,5.0185209075653));
#29737=CARTESIAN_POINT('Ctrl Pts',(0.189670682876021,2.44516112279632,5.0174791317348));
#29738=CARTESIAN_POINT('Ctrl Pts',(0.207537923239685,2.43471944087176,5.0164373559043));
#29739=CARTESIAN_POINT('Ctrl Pts',(0.224450873165666,2.42296547111908,5.0153955800738));
#29740=CARTESIAN_POINT('Ctrl Pts',(0.241400380816714,2.41118609489405,5.0143515524212));
#29741=CARTESIAN_POINT('Ctrl Pts',(0.257390910146576,2.39808923448553,5.0133075247686));
#29742=CARTESIAN_POINT('Ctrl Pts',(0.27222426658229,2.38386412010632,5.01226349711601));
#29743=CARTESIAN_POINT('Ctrl Pts',(0.27747063032145,2.37883288360985,5.01189423822015));
#29744=CARTESIAN_POINT('Ctrl Pts',(0.282572586067836,2.37366083549554,5.0115249793243));
#29745=CARTESIAN_POINT('Ctrl Pts',(0.287522563980542,2.36835734609296,5.01115572042844));
#29746=CARTESIAN_POINT('Ctrl Pts',(0.301517059726161,2.35336340850572,5.01011175778089));
#29747=CARTESIAN_POINT('Ctrl Pts',(0.314377222850617,2.33722715543588,5.00906779513334));
#29748=CARTESIAN_POINT('Ctrl Pts',(0.325914844775779,2.32014632396381,5.00802383248578));
#29749=CARTESIAN_POINT('Ctrl Pts',(0.33743124200216,2.3030969145218,5.00698179032001));
#29750=CARTESIAN_POINT('Ctrl Pts',(0.347629470877126,2.28510694539278,5.00593974815425));
#29751=CARTESIAN_POINT('Ctrl Pts',(0.356361634713657,2.26640695689847,5.00489770598848));
#29752=CARTESIAN_POINT('Ctrl Pts',(0.365084420343407,2.24772705189804,5.00385678295962));
#29753=CARTESIAN_POINT('Ctrl Pts',(0.372343930817319,2.22833929243338,5.00281585993077));
#29754=CARTESIAN_POINT('Ctrl Pts',(0.378038337434165,2.20849841210825,5.00177493690192));
#29755=CARTESIAN_POINT('Ctrl Pts',(0.383735668549835,2.18864734202411,5.00073347928213));
#29756=CARTESIAN_POINT('Ctrl Pts',(0.38786607153086,2.16834338895473,4.99969202166234));
#29757=CARTESIAN_POINT('Ctrl Pts',(0.390377561939004,2.14785654745758,4.99865056404255));
#29758=CARTESIAN_POINT('Ctrl Pts',(0.392889819716959,2.1273634463372,4.99760878821205));
#29759=CARTESIAN_POINT('Ctrl Pts',(0.393782126652338,2.10668807964256,4.99656701238155));
#29760=CARTESIAN_POINT('Ctrl Pts',(0.393054463829288,2.08610473232102,4.99552523655106));
#29761=CARTESIAN_POINT('Ctrl Pts',(0.392325228146534,2.06547689362714,4.99448120889846));
#29762=CARTESIAN_POINT('Ctrl Pts',(0.389969115880667,2.04494220308168,4.99343718124586));
#29763=CARTESIAN_POINT('Ctrl Pts',(0.386037948879175,2.0247697399635,4.99239315359327));
#29764=CARTESIAN_POINT('Ctrl Pts',(0.384647546639489,2.01763500417414,4.99202389469739));
#29765=CARTESIAN_POINT('Ctrl Pts',(0.383060576814579,2.0105454653376,4.99165463580152));
#29766=CARTESIAN_POINT('Ctrl Pts',(0.381280820453666,2.00351256064037,4.99128537690565));
#29767=CARTESIAN_POINT('Ctrl Pts',(0.376249122684712,1.98362924871547,4.9902414142581));
#29768=CARTESIAN_POINT('Ctrl Pts',(0.369642910861621,1.96408134795691,4.98919745161055));
#29769=CARTESIAN_POINT('Ctrl Pts',(0.361526565157871,1.94513414616142,4.988153488963));
#29770=CARTESIAN_POINT('Ctrl Pts',(0.35342515034663,1.92622179978531,4.98711144679724));
#29771=CARTESIAN_POINT('Ctrl Pts',(0.343819347764002,1.90790865100664,4.98606940463148));
#29772=CARTESIAN_POINT('Ctrl Pts',(0.332822940691177,1.8904438496496,4.98502736246571));
#29773=CARTESIAN_POINT('Ctrl Pts',(0.3218383435868,1.87299780521486,4.98398643943686));
#29774=CARTESIAN_POINT('Ctrl Pts',(0.309466472493654,1.85639893431858,4.98294551640801));
#29775=CARTESIAN_POINT('Ctrl Pts',(0.295866390270717,1.84087074825837,4.98190459337916));
#29776=CARTESIAN_POINT('Ctrl Pts',(0.282259323400011,1.82533458732652,4.98086313575938));
#29777=CARTESIAN_POINT('Ctrl Pts',(0.267423257894862,1.81087077388217,4.97982167813959));
#29778=CARTESIAN_POINT('Ctrl Pts',(0.251557069897546,1.79766917030418,4.9787802205198));
#29779=CARTESIAN_POINT('Ctrl Pts',(0.235686034088089,1.78446353306076,4.97773844468931));
#29780=CARTESIAN_POINT('Ctrl Pts',(0.218784837458711,1.77252131584131,4.97669666885882));
#29781=CARTESIAN_POINT('Ctrl Pts',(0.201084093464547,1.76199100994864,4.97565489302832));
#29782=CARTESIAN_POINT('Ctrl Pts',(0.183345088910557,1.75143794256081,4.97461086537573));
#29783=CARTESIAN_POINT('Ctrl Pts',(0.164803747297285,1.7423032049081,4.97356683772314));
#29784=CARTESIAN_POINT('Ctrl Pts',(0.145714367402498,1.73468888172889,4.97252281007055));
#29785=CARTESIAN_POINT('Ctrl Pts',(0.138962703952014,1.73199579542684,4.97215355117465));
#29786=CARTESIAN_POINT('Ctrl Pts',(0.132142637323045,1.72949245259711,4.97178429227876));
#29787=CARTESIAN_POINT('Ctrl Pts',(0.125265830857022,1.72718186522153,4.97141503338286));
#29788=CARTESIAN_POINT('Ctrl Pts',(0.105823837272394,1.72064941078139,4.97037107073529));
#29789=CARTESIAN_POINT('Ctrl Pts',(0.0858115504945747,1.71562240007358,
4.96932710808772));
#29790=CARTESIAN_POINT('Ctrl Pts',(0.065486879404064,1.71219030617335,4.96828314544015));
#29791=CARTESIAN_POINT('Ctrl Pts',(0.0451995977361308,1.70876452597968,
4.96724110327437));
#29792=CARTESIAN_POINT('Ctrl Pts',(0.0246017798531759,1.7069280184457,4.96619906110858));
#29793=CARTESIAN_POINT('Ctrl Pts',(0.0039645083343114,1.70671998185305,
4.9651570189428));
#29794=CARTESIAN_POINT('Ctrl Pts',(-0.0166505990791454,1.70651216868843,
4.96411609591393));
#29795=CARTESIAN_POINT('Ctrl Pts',(-0.0373043442899069,1.70792939067573,
4.96307517288506));
#29796=CARTESIAN_POINT('Ctrl Pts',(-0.0577226913974393,1.7109588956192,
4.96203424985619));
#29797=CARTESIAN_POINT('Ctrl Pts',(-0.0781515248358711,1.71398995643744,
4.96099279223638));
#29798=CARTESIAN_POINT('Ctrl Pts',(-0.098343988474489,1.71863486238312,
4.95995133461658));
#29799=CARTESIAN_POINT('Ctrl Pts',(-0.118032787376494,1.72482917077132,
4.95890987699677));
#29800=CARTESIAN_POINT('Ctrl Pts',(-0.137727602064921,1.73102537179078,
4.95786810116626));
#29801=CARTESIAN_POINT('Ctrl Pts',(-0.156917755242051,1.73877166255961,
4.95682632533574));
#29802=CARTESIAN_POINT('Ctrl Pts',(-0.175353557531653,1.747954520181,4.95578454950523));
#29803=CARTESIAN_POINT('Ctrl Pts',(-0.193829209226259,1.75715722675752,
4.95474052185262));
#29804=CARTESIAN_POINT('Ctrl Pts',(-0.211546623432728,1.76780232021209,
4.95369649420001));
#29805=CARTESIAN_POINT('Ctrl Pts',(-0.22828230895195,1.77973124189274,4.95265246654739));
#29806=CARTESIAN_POINT('Ctrl Pts',(-0.234201501551311,1.78395034512872,
4.95228320765162));
#29807=CARTESIAN_POINT('Ctrl Pts',(-0.239998182318464,1.78832967455179,
4.95191394875585));
#29808=CARTESIAN_POINT('Ctrl Pts',(-0.245663505147719,1.79286105385585,
4.95154468986007));
#29809=CARTESIAN_POINT('Ctrl Pts',(-0.261477141913282,1.8055095098258,4.95051397612562));
#29810=CARTESIAN_POINT('Ctrl Pts',(-0.276364208224235,1.81942499701367,
4.94948326239116));
#29811=CARTESIAN_POINT('Ctrl Pts',(-0.290112689812862,1.83444488856445,
4.9484525486567));
#29812=CARTESIAN_POINT('Ctrl Pts',(-0.303835828818759,1.84943709394192,
4.94742373483737));
#29813=CARTESIAN_POINT('Ctrl Pts',(-0.31642399524006,1.86552915697693,4.94639492101804));
#29814=CARTESIAN_POINT('Ctrl Pts',(-0.327699970669064,1.88251984177058,
4.94536610719871));
#29815=CARTESIAN_POINT('Ctrl Pts',(-0.338972373206054,1.89950514291628,
4.94433761936808));
#29816=CARTESIAN_POINT('Ctrl Pts',(-0.348932950714574,1.91738790085643,
4.94330913153746));
#29817=CARTESIAN_POINT('Ctrl Pts',(-0.357446176121318,1.93593561880698,
4.94228064370684));
#29818=CARTESIAN_POINT('Ctrl Pts',(-0.365956920978892,1.95447793239853,
4.94125245555284));
#29819=CARTESIAN_POINT('Ctrl Pts',(-0.373020843267589,1.97368413017175,
4.94022426739884));
#29820=CARTESIAN_POINT('Ctrl Pts',(-0.378549904924822,1.9933001430113,4.93919607924483));
#29821=CARTESIAN_POINT('Ctrl Pts',(-0.384089670934554,2.01295413276793,
4.93816590050199));
#29822=CARTESIAN_POINT('Ctrl Pts',(-0.388088463864271,2.0330187842476,4.93713572175915));
#29823=CARTESIAN_POINT('Ctrl Pts',(-0.390508923268107,2.05322745625922,
4.93610554301631));
#29824=CARTESIAN_POINT('Ctrl Pts',(-0.392380099961015,2.06885010872049,
4.93530914608023));
#29825=CARTESIAN_POINT('Ctrl Pts',(-0.393309066605004,2.08455850583689,
4.93451274914414));
#29826=CARTESIAN_POINT('Ctrl Pts',(-0.393299933199252,2.10022922797308,
4.93371635220805));
#29827=CARTESIAN_POINT('',(-0.393315750863,2.09965835142492,4.80871634439493));
#29828=CARTESIAN_POINT('Ctrl Pts',(-0.3932999331992,2.10022922806266,4.9337163522035));
#29829=CARTESIAN_POINT('Ctrl Pts',(-0.39329212701003,2.11362276131211,4.93303568358143));
#29830=CARTESIAN_POINT('Ctrl Pts',(-0.39260021454605,2.12699611331515,4.93235501495935));
#29831=CARTESIAN_POINT('Ctrl Pts',(-0.391230019245934,2.14029841238592,
4.93167434633727));
#29832=CARTESIAN_POINT('Ctrl Pts',(-0.389128508074786,2.16070056242748,
4.93063038368973));
#29833=CARTESIAN_POINT('Ctrl Pts',(-0.385420519122019,2.1809986726012,4.9295864210422));
#29834=CARTESIAN_POINT('Ctrl Pts',(-0.380131366312023,2.20092093115779,
4.92854245839467));
#29835=CARTESIAN_POINT('Ctrl Pts',(-0.374851943468561,2.22080654057301,
4.92750041622893));
#29836=CARTESIAN_POINT('Ctrl Pts',(-0.367997259653949,2.24031695244025,
4.92645837406319));
#29837=CARTESIAN_POINT('Ctrl Pts',(-0.359643847175506,2.25918917421986,
4.92541633189744));
#29838=CARTESIAN_POINT('Ctrl Pts',(-0.351299406130838,2.27804112752976,
4.92437540886862));
#29839=CARTESIAN_POINT('Ctrl Pts',(-0.341459701736896,2.29625557033757,
4.9233344858398));
#29840=CARTESIAN_POINT('Ctrl Pts',(-0.330249779338624,2.31358832656957,
4.92229356281097));
#29841=CARTESIAN_POINT('Ctrl Pts',(-0.319034099816375,2.33092998445343,
4.92125210519121));
#29842=CARTESIAN_POINT('Ctrl Pts',(-0.306447182478844,2.34738842456622,
4.92021064757146));
#29843=CARTESIAN_POINT('Ctrl Pts',(-0.292658336096874,2.36274700438446,
4.9191691899517));
#29844=CARTESIAN_POINT('Ctrl Pts',(-0.278865276621196,2.37811027691841,
4.91812741412124));
#29845=CARTESIAN_POINT('Ctrl Pts',(-0.263870075060144,2.39237249728365,
4.91708563829077));
#29846=CARTESIAN_POINT('Ctrl Pts',(-0.247879430081077,2.40535336602481,
4.91604386246031));
#29847=CARTESIAN_POINT('Ctrl Pts',(-0.231854220960001,2.41836229320834,
4.91499983480774));
#29848=CARTESIAN_POINT('Ctrl Pts',(-0.214829879308957,2.43008392159923,
4.91395580715518));
#29849=CARTESIAN_POINT('Ctrl Pts',(-0.197043255114176,2.44038044246697,
4.91291177950261));
#29850=CARTESIAN_POINT('Ctrl Pts',(-0.190752359276096,2.44402218693541,
4.91254252060658));
#29851=CARTESIAN_POINT('Ctrl Pts',(-0.184366323275313,2.4474860833518,4.91217326171054));
#29852=CARTESIAN_POINT('Ctrl Pts',(-0.177896251843067,2.45076746368526,
4.91180400281451));
#29853=CARTESIAN_POINT('Ctrl Pts',(-0.159604172828913,2.46004452792847,
4.91076004016685));
#29854=CARTESIAN_POINT('Ctrl Pts',(-0.14052995694789,2.46791451822913,4.90971607751919));
#29855=CARTESIAN_POINT('Ctrl Pts',(-0.120915851270176,2.47425158237689,
4.90867211487152));
#29856=CARTESIAN_POINT('Ctrl Pts',(-0.101337827853386,2.4805769888123,4.90763007270564));
#29857=CARTESIAN_POINT('Ctrl Pts',(-0.0812225600257416,2.48537478640656,
4.90658803053976));
#29858=CARTESIAN_POINT('Ctrl Pts',(-0.0608326049441621,2.48856696228026,
4.90554598837388));
#29859=CARTESIAN_POINT('Ctrl Pts',(-0.0404645483540277,2.49175570980721,
4.90450506534491));
#29860=CARTESIAN_POINT('Ctrl Pts',(-0.0198231089396549,2.49334211718406,
4.90346414231595));
#29861=CARTESIAN_POINT('Ctrl Pts',(0.000818716379649284,2.49329914785503,
4.90242321928698));
#29862=CARTESIAN_POINT('Ctrl Pts',(0.0214711428024116,2.49325615645806,
4.90138176166708));
#29863=CARTESIAN_POINT('Ctrl Pts',(0.0421232197158089,2.49158210201624,
4.90034030404717));
#29864=CARTESIAN_POINT('Ctrl Pts',(0.0625011403103141,2.48830206986303,
4.89929884642727));
#29865=CARTESIAN_POINT('Ctrl Pts',(0.0828852872479474,2.485021035517,4.89825707059666));
#29866=CARTESIAN_POINT('Ctrl Pts',(0.10299439104046,2.48013319914792,4.89721529476605));
#29867=CARTESIAN_POINT('Ctrl Pts',(0.122564962954127,2.47371475734316,4.89617351893544));
#29868=CARTESIAN_POINT('Ctrl Pts',(0.142177837103041,2.46728244193079,4.89512949128274));
#29869=CARTESIAN_POINT('Ctrl Pts',(0.161249175870259,2.45931319990156,4.89408546363003));
#29870=CARTESIAN_POINT('Ctrl Pts',(0.179534896030575,2.44993158060868,4.89304143597733));
#29871=CARTESIAN_POINT('Ctrl Pts',(0.186002315554453,2.44661342484296,4.89267217708212));
#29872=CARTESIAN_POINT('Ctrl Pts',(0.19237169834148,2.44311900116171,4.8923029181869));
#29873=CARTESIAN_POINT('Ctrl Pts',(0.198633108236113,2.43945511973229,4.89193365929169));
#29874=CARTESIAN_POINT('Ctrl Pts',(0.216335262835472,2.42909665469184,4.89088969664426));
#29875=CARTESIAN_POINT('Ctrl Pts',(0.233277709289957,2.41731888042127,4.88984573399683));
#29876=CARTESIAN_POINT('Ctrl Pts',(0.249223496091635,2.40425735651889,4.88880177134941));
#29877=CARTESIAN_POINT('Ctrl Pts',(0.265139948900249,2.39121986069718,4.88775972918376));
#29878=CARTESIAN_POINT('Ctrl Pts',(0.280062780951827,2.37690371788836,4.88671768701811));
#29879=CARTESIAN_POINT('Ctrl Pts',(0.293784270687491,2.36148746106959,4.88567564485247));
#29880=CARTESIAN_POINT('Ctrl Pts',(0.307491023758754,2.34608776106844,4.88463472182374));
#29881=CARTESIAN_POINT('Ctrl Pts',(0.319998487605928,2.32959082021855,4.88359379879501));
#29882=CARTESIAN_POINT('Ctrl Pts',(0.331136151243724,2.31221154384127,4.88255287576628));
#29883=CARTESIAN_POINT('Ctrl Pts',(0.342279534895317,2.29482334192054,4.88151141814661));
#29884=CARTESIAN_POINT('Ctrl Pts',(0.352051302340476,2.27655250997617,4.88046996052694));
#29885=CARTESIAN_POINT('Ctrl Pts',(0.360324329203391,2.25764284882013,4.87942850290727));
#29886=CARTESIAN_POINT('Ctrl Pts',(0.368599883836701,2.23872740993818,4.87838672707689));
#29887=CARTESIAN_POINT('Ctrl Pts',(0.375375524736701,2.21917344128914,4.87734495124651));
#29888=CARTESIAN_POINT('Ctrl Pts',(0.380572688145833,2.19924373550736,4.87630317541613));
#29889=CARTESIAN_POINT('Ctrl Pts',(0.385781085341637,2.17927095121417,4.87525914776365));
#29890=CARTESIAN_POINT('Ctrl Pts',(0.389404064233882,2.15892153341763,4.87421512011117));
#29891=CARTESIAN_POINT('Ctrl Pts',(0.391414221488676,2.1384681324789,4.87317109245868));
#29892=CARTESIAN_POINT('Ctrl Pts',(0.392125187762522,2.13123403265003,4.87280183356209));
#29893=CARTESIAN_POINT('Ctrl Pts',(0.392634875758463,2.12398694685707,4.87243257466551));
#29894=CARTESIAN_POINT('Ctrl Pts',(0.392943632966605,2.11673891606425,4.87206331576891));
#29895=CARTESIAN_POINT('Ctrl Pts',(0.393816546240716,2.09624740324003,4.87101935312151));
#29896=CARTESIAN_POINT('Ctrl Pts',(0.393084835156576,2.07562636889449,4.86997539047411));
#29897=CARTESIAN_POINT('Ctrl Pts',(0.390734214518835,2.05514842695792,4.8689314278267));
#29898=CARTESIAN_POINT('Ctrl Pts',(0.388387918101057,2.03470815640222,4.86788938566109));
#29899=CARTESIAN_POINT('Ctrl Pts',(0.384428647533905,2.01441118525129,4.86684734349547));
#29900=CARTESIAN_POINT('Ctrl Pts',(0.378894073107929,1.99452881263737,4.86580530132985));
#29901=CARTESIAN_POINT('Ctrl Pts',(0.373365442727952,1.97466779337933,4.86476437830115));
#29902=CARTESIAN_POINT('Ctrl Pts',(0.36626503567026,1.955221201676,4.86372345527245));
#29903=CARTESIAN_POINT('Ctrl Pts',(0.357681247499471,1.93644873835026,4.86268253224375));
#29904=CARTESIAN_POINT('Ctrl Pts',(0.349093050918806,1.91766663397664,4.86164107462411));
#29905=CARTESIAN_POINT('Ctrl Pts',(0.339020242575313,1.89956002548728,4.86059961700448));
#29906=CARTESIAN_POINT('Ctrl Pts',(0.32759899983515,1.88236777511818,4.85955815938484));
#29907=CARTESIAN_POINT('Ctrl Pts',(0.316174267407413,1.86517027176709,4.8585163835545));
#29908=CARTESIAN_POINT('Ctrl Pts',(0.303400717313503,1.84888827503743,4.85747460772415));
#29909=CARTESIAN_POINT('Ctrl Pts',(0.289456782323964,1.83373009714454,4.85643283189381));
#29910=CARTESIAN_POINT('Ctrl Pts',(0.275482707202496,1.81853915450612,4.85538880424137));
#29911=CARTESIAN_POINT('Ctrl Pts',(0.260333736313617,1.80447738144244,4.85434477658892));
#29912=CARTESIAN_POINT('Ctrl Pts',(0.244224285042832,1.79171540973426,4.85330074893648));
#29913=CARTESIAN_POINT('Ctrl Pts',(0.238526583272011,1.78720166760992,4.85293149003969));
#29914=CARTESIAN_POINT('Ctrl Pts',(0.232709007101227,1.78285013432857,4.8525622311429));
#29915=CARTESIAN_POINT('Ctrl Pts',(0.2267818688915,1.77866703570583,4.85219297224612));
#29916=CARTESIAN_POINT('Ctrl Pts',(0.210024761733678,1.7668406484355,4.85114900959779));
#29917=CARTESIAN_POINT('Ctrl Pts',(0.192290138401755,1.75629334571834,4.85010504694946));
#29918=CARTESIAN_POINT('Ctrl Pts',(0.173799484735446,1.74718470964867,4.84906108430113));
#29919=CARTESIAN_POINT('Ctrl Pts',(0.155342846618986,1.73809282989653,4.84801904213458));
#29920=CARTESIAN_POINT('Ctrl Pts',(0.136133565155466,1.73043473824831,4.84697699996803));
#29921=CARTESIAN_POINT('Ctrl Pts',(0.116420145122099,1.72432561997156,4.84593495780148));
#29922=CARTESIAN_POINT('Ctrl Pts',(0.0967278969921625,1.71822306279188,
4.84489403477185));
#29923=CARTESIAN_POINT('Ctrl Pts',(0.0765332758542779,1.71366642071083,
4.84385311174222));
#29924=CARTESIAN_POINT('Ctrl Pts',(0.0561024929268396,1.71072194990291,
4.84281218871259));
#29925=CARTESIAN_POINT('Ctrl Pts',(0.0356612172819931,1.70777596689155,
4.84177073109203));
#29926=CARTESIAN_POINT('Ctrl Pts',(0.0149842634987702,1.70644393016169,
4.84072927347147));
#29927=CARTESIAN_POINT('Ctrl Pts',(-0.005653813508861,1.70674063978996,
4.83968781585091));
#29928=CARTESIAN_POINT('Ctrl Pts',(-0.0262981963486536,1.70703744007596,
4.83864604001965));
#29929=CARTESIAN_POINT('Ctrl Pts',(-0.0469029442032106,1.70896393068438,
4.83760426418839));
#29930=CARTESIAN_POINT('Ctrl Pts',(-0.0671963155490089,1.71248284531309,
4.83656248835713));
#29931=CARTESIAN_POINT('Ctrl Pts',(-0.087533551477086,1.71600936615556,
4.83551846070379));
#29932=CARTESIAN_POINT('Ctrl Pts',(-0.107557353716536,1.72113500029117,
4.83447443305045));
#29933=CARTESIAN_POINT('Ctrl Pts',(-0.127008185088199,1.72777182949083,
4.83343040539711));
#29934=CARTESIAN_POINT('Ctrl Pts',(-0.133887689096931,1.73011918895388,
4.83306114650585));
#29935=CARTESIAN_POINT('Ctrl Pts',(-0.140695695187009,1.73265514753066,
4.83269188761459));
#29936=CARTESIAN_POINT('Ctrl Pts',(-0.147421386314326,1.73537440455014,
4.83232262872333));
#29937=CARTESIAN_POINT('Ctrl Pts',(-0.166436149329981,1.7430622431418,4.83127866607684));
#29938=CARTESIAN_POINT('Ctrl Pts',(-0.184904582322735,1.75226438641009,
4.83023470343036));
#29939=CARTESIAN_POINT('Ctrl Pts',(-0.202572611524001,1.76288098976719,
4.82919074078387));
#29940=CARTESIAN_POINT('Ctrl Pts',(-0.220208138481783,1.77347806273847,
4.82814869861916));
#29941=CARTESIAN_POINT('Ctrl Pts',(-0.237045530177403,1.78548410711521,
4.82710665645445));
#29942=CARTESIAN_POINT('Ctrl Pts',(-0.252853416649968,1.79875252749867,
4.82606461428974));
#29943=CARTESIAN_POINT('Ctrl Pts',(-0.268644325700925,1.81200669780719,
4.82502369126194));
#29944=CARTESIAN_POINT('Ctrl Pts',(-0.283407345248792,1.82652010410806,
4.82398276823414));
#29945=CARTESIAN_POINT('Ctrl Pts',(-0.296942660973606,1.84210477690753,
4.82294184520633));
#29946=CARTESIAN_POINT('Ctrl Pts',(-0.310484928084148,1.85769745358917,
4.82190038758757));
#29947=CARTESIAN_POINT('Ctrl Pts',(-0.322797737103604,1.87436195095103,
4.8208589299688));
#29948=CARTESIAN_POINT('Ctrl Pts',(-0.333720022327178,1.89187542985522,
4.81981747235003));
#29949=CARTESIAN_POINT('Ctrl Pts',(-0.344645644785207,1.90939425989098,
4.81877569652054));
#29950=CARTESIAN_POINT('Ctrl Pts',(-0.354179539312652,1.92776194493778,
4.81773392069106));
#29951=CARTESIAN_POINT('Ctrl Pts',(-0.362205941487288,1.94672982693522,
4.81669214486157));
#29952=CARTESIAN_POINT('Ctrl Pts',(-0.370249692912656,1.96573870844072,
4.81564811720995));
#29953=CARTESIAN_POINT('Ctrl Pts',(-0.376779213936063,1.9853496782075,4.81460408955833));
#29954=CARTESIAN_POINT('Ctrl Pts',(-0.38172793561452,2.00529692100319,4.81356006190671));
#29955=CARTESIAN_POINT('Ctrl Pts',(-0.383478233636536,2.01235199944131,
4.81319080300465));
#29956=CARTESIAN_POINT('Ctrl Pts',(-0.385031251020226,2.01944905325987,
4.8128215441026));
#29957=CARTESIAN_POINT('Ctrl Pts',(-0.38638558920318,2.02657611794442,4.81245228520054));
#29958=CARTESIAN_POINT('Ctrl Pts',(-0.39095304099983,2.05061186086891,4.81120697420153));
#29959=CARTESIAN_POINT('Ctrl Pts',(-0.393278498021054,2.07508656686066,
4.80996166320251));
#29960=CARTESIAN_POINT('Ctrl Pts',(-0.393299851487826,2.09965821109775,
4.8087163522035));
#29961=CARTESIAN_POINT('',(-0.39305280653286,2.09995383756141,4.68371636473574));
#29962=CARTESIAN_POINT('Ctrl Pts',(-0.393479809868051,2.09965979940225,
4.80871626382152));
#29963=CARTESIAN_POINT('Ctrl Pts',(-0.392508166945697,2.20582651071962,
4.80333815644026));
#29964=CARTESIAN_POINT('Ctrl Pts',(-0.293340422281615,2.44434164323185,
4.79133660121808));
#29965=CARTESIAN_POINT('Ctrl Pts',(0.110092729177043,2.55183472037241,4.77271159815497));
#29966=CARTESIAN_POINT('Ctrl Pts',(0.4395059068619,2.25201835981764,4.75284125463216));
#29967=CARTESIAN_POINT('Ctrl Pts',(0.36573224633123,1.81274585059014,4.7329709111094));
#29968=CARTESIAN_POINT('Ctrl Pts',(-0.0435509564148769,1.63698991534316,
4.71310056758659));
#29969=CARTESIAN_POINT('Ctrl Pts',(-0.348716460461016,1.84272401725045,
4.69668239214361));
#29970=CARTESIAN_POINT('Ctrl Pts',(-0.392722693669812,2.03701811531716,
4.68688766454154));
#29971=CARTESIAN_POINT('Ctrl Pts',(-0.392657437396775,2.09995348595077,
4.68371638478041));
#29972=CARTESIAN_POINT('',(-0.393299834232345,2.10036109944607,4.55871635220349));
#29973=CARTESIAN_POINT('Ctrl Pts',(-0.39329999731665,2.09995405739372,4.6837163522035));
#29974=CARTESIAN_POINT('Ctrl Pts',(-0.393302510661517,2.12147000107707,
4.68263394642612));
#29975=CARTESIAN_POINT('Ctrl Pts',(-0.391535126025817,2.14295809897274,
4.68155154064874));
#29976=CARTESIAN_POINT('Ctrl Pts',(-0.388037245285784,2.16412477111866,
4.68046913487136));
#29977=CARTESIAN_POINT('Ctrl Pts',(-0.38453365162738,2.18532601376001,4.6793849612533));
#29978=CARTESIAN_POINT('Ctrl Pts',(-0.379294099505847,2.20620415606676,
4.67830078763524));
#29979=CARTESIAN_POINT('Ctrl Pts',(-0.372408589511198,2.2264781896545,4.67721661401719));
#29980=CARTESIAN_POINT('Ctrl Pts',(-0.365500533233302,2.24681860962527,
4.67612889032288));
#29981=CARTESIAN_POINT('Ctrl Pts',(-0.356936024386469,2.26655037781274,
4.67504116662858));
#29982=CARTESIAN_POINT('Ctrl Pts',(-0.346852916917358,2.28541290145489,
4.67395344293428));
#29983=CARTESIAN_POINT('Ctrl Pts',(-0.34501882570705,2.28884394579536,4.67375558880319));
#29984=CARTESIAN_POINT('Ctrl Pts',(-0.343134606349185,2.29224630457451,
4.6735577346721));
#29985=CARTESIAN_POINT('Ctrl Pts',(-0.341201241198039,2.29561851396255,
4.67335988054101));
#29986=CARTESIAN_POINT('Ctrl Pts',(-0.330999981106641,2.31341173063956,
4.67231591766096));
#29987=CARTESIAN_POINT('Ctrl Pts',(-0.319372737625787,2.33045784032205,
4.67127195478091));
#29988=CARTESIAN_POINT('Ctrl Pts',(-0.306452966299499,2.346518699993,4.67022799190086));
#29989=CARTESIAN_POINT('Ctrl Pts',(-0.293556962264146,2.36255001400754,
4.66918594950135));
#29990=CARTESIAN_POINT('Ctrl Pts',(-0.279373559743091,2.37759907158861,
4.66814390710184));
#29991=CARTESIAN_POINT('Ctrl Pts',(-0.264079444876189,2.39145657788749,
4.66710186470234));
#29992=CARTESIAN_POINT('Ctrl Pts',(-0.248801755638117,2.4052992014516,4.6660609414393));
#29993=CARTESIAN_POINT('Ctrl Pts',(-0.232416245287508,2.41795230129518,
4.66502001817626));
#29994=CARTESIAN_POINT('Ctrl Pts',(-0.215136300475679,2.42924346951403,
4.66397909491322));
#29995=CARTESIAN_POINT('Ctrl Pts',(-0.197847481170762,2.44054043655894,
4.66293763706131));
#29996=CARTESIAN_POINT('Ctrl Pts',(-0.17966391683757,2.45047365866721,4.66189617920939));
#29997=CARTESIAN_POINT('Ctrl Pts',(-0.160828272786028,2.45891385689698,
4.66085472135748));
#29998=CARTESIAN_POINT('Ctrl Pts',(-0.141986873641556,2.46735663396743,
4.65981294529575));
#29999=CARTESIAN_POINT('Ctrl Pts',(-0.122493683820887,2.47430521140443,
4.65877116923402));
#30000=CARTESIAN_POINT('Ctrl Pts',(-0.102610789848103,2.47967870075466,
4.6577293931723));
#30001=CARTESIAN_POINT('Ctrl Pts',(-0.0826849186502222,2.48506380499665,
4.65668536529329));
#30002=CARTESIAN_POINT('Ctrl Pts',(-0.0623683854883882,2.48886688856434,
4.65564133741428));
#30003=CARTESIAN_POINT('Ctrl Pts',(-0.0419335873946778,2.49105813410312,
4.65459730953527));
#30004=CARTESIAN_POINT('Ctrl Pts',(-0.0347060959408396,2.49183314584202,
4.65422805202959));
#30005=CARTESIAN_POINT('Ctrl Pts',(-0.0274638362901075,2.49240700373886,
4.65385879452391));
#30006=CARTESIAN_POINT('Ctrl Pts',(-0.0202188518732227,2.49277994860854,
4.65348953701823));
#30007=CARTESIAN_POINT('Ctrl Pts',(0.000264115230046272,2.4938343356241,
4.6524455748913));
#30008=CARTESIAN_POINT('Ctrl Pts',(0.0208908123270126,2.49328531004609,
4.65140161276437));
#30009=CARTESIAN_POINT('Ctrl Pts',(0.0413887629450701,2.491116172386,4.65035765063744));
#30010=CARTESIAN_POINT('Ctrl Pts',(0.0618490053731108,2.4889510250885,4.64931560899139));
#30011=CARTESIAN_POINT('Ctrl Pts',(0.0821802417579286,2.48517169904134,
4.64827356734533));
#30012=CARTESIAN_POINT('Ctrl Pts',(0.102110850141772,2.47981345985013,4.64723152569928));
#30013=CARTESIAN_POINT('Ctrl Pts',(0.122020053404073,2.47446097531322,4.64619060318756));
#30014=CARTESIAN_POINT('Ctrl Pts',(0.141528768394392,2.46753310618056,4.64514968067584));
#30015=CARTESIAN_POINT('Ctrl Pts',(0.160376521685547,2.45911594407941,4.64410875816412));
#30016=CARTESIAN_POINT('Ctrl Pts',(0.179233954872339,2.45069445906245,4.64306730105174));
#30017=CARTESIAN_POINT('Ctrl Pts',(0.19742906979512,2.44078243833551,4.64202584393937));
#30018=CARTESIAN_POINT('Ctrl Pts',(0.214721807551827,2.42951393803855,4.64098438682699));
#30019=CARTESIAN_POINT('Ctrl Pts',(0.232019829078899,2.41824199466805,4.63994261149894));
#30020=CARTESIAN_POINT('Ctrl Pts',(0.24841432836989,2.4056131782879,4.63890083617089));
#30021=CARTESIAN_POINT('Ctrl Pts',(0.263695421065623,2.39180406938393,4.63785906084284));
#30022=CARTESIAN_POINT('Ctrl Pts',(0.279009544424255,2.377965111566,4.6368150336778));
#30023=CARTESIAN_POINT('Ctrl Pts',(0.293204950586356,2.36294130310269,4.63577100651276));
#30024=CARTESIAN_POINT('Ctrl Pts',(0.306109115434745,2.34694553943685,4.63472697934773));
#30025=CARTESIAN_POINT('Ctrl Pts',(0.31067318928691,2.34128799804999,4.63435771739697));
#30026=CARTESIAN_POINT('Ctrl Pts',(0.315076119829795,2.33550914814184,4.6339884554462));
#30027=CARTESIAN_POINT('Ctrl Pts',(0.319311589995046,2.32961924678658,4.63361919349544));
#30028=CARTESIAN_POINT('Ctrl Pts',(0.331285944740875,2.31296754921957,4.63257523062472));
#30029=CARTESIAN_POINT('Ctrl Pts',(0.341989923292617,2.2953270437564,4.63153126775399));
#30030=CARTESIAN_POINT('Ctrl Pts',(0.351261987899915,2.27691779406436,4.63048730488327));
#30031=CARTESIAN_POINT('Ctrl Pts',(0.360516995491423,2.2585424102777,4.6294452625008));
#30032=CARTESIAN_POINT('Ctrl Pts',(0.368344937507908,2.23940171233885,4.62840322011833));
#30033=CARTESIAN_POINT('Ctrl Pts',(0.374628431954159,2.21974317505214,4.62736117773587));
#30034=CARTESIAN_POINT('Ctrl Pts',(0.38090517798497,2.20010575085429,4.62632025449737));
#30035=CARTESIAN_POINT('Ctrl Pts',(0.385640518980635,2.17995227989731,4.62527933125887));
#30036=CARTESIAN_POINT('Ctrl Pts',(0.388765843277035,2.15954837614155,4.62423840802036));
#30037=CARTESIAN_POINT('Ctrl Pts',(0.391892772620308,2.1391339937222,4.62319695020355));
#30038=CARTESIAN_POINT('Ctrl Pts',(0.393407906080117,2.11846964641939,4.62215549238674));
#30039=CARTESIAN_POINT('Ctrl Pts',(0.393294012163239,2.09782974735531,4.62111403456992));
#30040=CARTESIAN_POINT('Ctrl Pts',(0.39318008344758,2.07718354204287,4.62007225854944));
#30041=CARTESIAN_POINT('Ctrl Pts',(0.39143617673339,2.05656253478705,4.61903048252895));
#30042=CARTESIAN_POINT('Ctrl Pts',(0.388097149784235,2.03623878663833,4.61798870650847));
#30043=CARTESIAN_POINT('Ctrl Pts',(0.384750905496115,2.01587110851189,4.61694467867907));
#30044=CARTESIAN_POINT('Ctrl Pts',(0.379802833779225,1.99580268733233,4.61590065084966));
#30045=CARTESIAN_POINT('Ctrl Pts',(0.373338550443823,1.97629382896353,4.61485662302026));
#30046=CARTESIAN_POINT('Ctrl Pts',(0.371052226060063,1.96939382531678,4.61448736533772));
#30047=CARTESIAN_POINT('Ctrl Pts',(0.368576677877943,1.96256364576548,4.61411810765519));
#30048=CARTESIAN_POINT('Ctrl Pts',(0.3659171104889,1.95581415377557,4.61374884997265));
#30049=CARTESIAN_POINT('Ctrl Pts',(0.358397990258774,1.93673201208086,4.61270488585942));
#30050=CARTESIAN_POINT('Ctrl Pts',(0.349359781576677,1.91818276843518,4.61166092174618));
#30051=CARTESIAN_POINT('Ctrl Pts',(0.338900075299647,1.90042137148008,4.61061695763295));
#30052=CARTESIAN_POINT('Ctrl Pts',(0.328459610650787,1.88269264831016,4.60957491399135));
#30053=CARTESIAN_POINT('Ctrl Pts',(0.316603156946611,1.8657495520126,4.60853287034976));
#30054=CARTESIAN_POINT('Ctrl Pts',(0.303475255083612,1.84982474232663,4.60749082670817));
#30055=CARTESIAN_POINT('Ctrl Pts',(0.290361452296511,1.83391703553363,4.60644990219837));
#30056=CARTESIAN_POINT('Ctrl Pts',(0.275979355542149,1.81902602751197,4.60540897768858));
#30057=CARTESIAN_POINT('Ctrl Pts',(0.260515157659317,1.8053531900228,4.60436805317878));
#30058=CARTESIAN_POINT('Ctrl Pts',(0.245043017923279,1.79167333065839,4.60332659408777));
#30059=CARTESIAN_POINT('Ctrl Pts',(0.228488207378558,1.7792133910942,4.60228513499677));
#30060=CARTESIAN_POINT('Ctrl Pts',(0.211072130331362,1.76813640483268,4.60124367590576));
#30061=CARTESIAN_POINT('Ctrl Pts',(0.193650731983767,1.75705603411373,4.6002018986078));
#30062=CARTESIAN_POINT('Ctrl Pts',(0.175368182998202,1.74735982189582,4.59916012130985));
#30063=CARTESIAN_POINT('Ctrl Pts',(0.156472106851897,1.73916573087174,4.5981183440119));
#30064=CARTESIAN_POINT('Ctrl Pts',(0.137535186968691,1.73095392837701,4.59707431491957));
#30065=CARTESIAN_POINT('Ctrl Pts',(0.11798278903514,1.72425096803732,4.59603028582725));
#30066=CARTESIAN_POINT('Ctrl Pts',(0.0980801287989144,1.71912577097579,
4.59498625673493));
#30067=CARTESIAN_POINT('Ctrl Pts',(0.0910409962331123,1.71731310165853,
4.5946170066399));
#30068=CARTESIAN_POINT('Ctrl Pts',(0.0839581446602437,1.71569732406559,
4.59424775654488));
#30069=CARTESIAN_POINT('Ctrl Pts',(0.0768435248601465,1.71427994259169,
4.59387850644986));
#30070=CARTESIAN_POINT('Ctrl Pts',(0.056728784763575,1.71027266451274,4.59283454768598));
#30071=CARTESIAN_POINT('Ctrl Pts',(0.0362398046289374,1.70783111395,4.5917905889221));
#30072=CARTESIAN_POINT('Ctrl Pts',(0.0156437749488127,1.70701124404717,
4.59074663015821));
#30073=CARTESIAN_POINT('Ctrl Pts',(-0.00491436603069629,1.70619288238675,
4.58970459187326));
#30074=CARTESIAN_POINT('Ctrl Pts',(-0.0255784411254026,1.70699036808954,
4.58866255358831));
#30075=CARTESIAN_POINT('Ctrl Pts',(-0.0460745855597139,1.7094081125196,
4.58762051530336));
#30076=CARTESIAN_POINT('Ctrl Pts',(-0.0665487176794167,1.71182326035638,
4.58657959613984));
#30077=CARTESIAN_POINT('Ctrl Pts',(-0.0868545467815963,1.71585515534059,
4.58553867697633));
#30078=CARTESIAN_POINT('Ctrl Pts',(-0.106721884374345,1.72145630450952,
4.58449775781281));
#30079=CARTESIAN_POINT('Ctrl Pts',(-0.126599426632449,1.72706033065442,
4.58345630399125));
#30080=CARTESIAN_POINT('Ctrl Pts',(-0.146037314875636,1.73423503711632,
4.5824148501697));
#30081=CARTESIAN_POINT('Ctrl Pts',(-0.164778619486665,1.74288251714587,
4.58137339634815));
#30082=CARTESIAN_POINT('Ctrl Pts',(-0.183525651014859,1.75153263964898,
4.58033162428195));
#30083=CARTESIAN_POINT('Ctrl Pts',(-0.201575022785195,1.76165609079279,
4.57928985221576));
#30084=CARTESIAN_POINT('Ctrl Pts',(-0.218693508662671,1.77310852065432,
4.57824808014956));
#30085=CARTESIAN_POINT('Ctrl Pts',(-0.235848998422755,1.78458570646524,
4.57720405615457));
#30086=CARTESIAN_POINT('Ctrl Pts',(-0.252069007019751,1.79739714983084,
4.57616003215958));
#30087=CARTESIAN_POINT('Ctrl Pts',(-0.267152020423162,1.8113571619045,4.57511600816459));
#30088=CARTESIAN_POINT('Ctrl Pts',(-0.272487033362416,1.81629495802344,
4.57474672641875));
#30089=CARTESIAN_POINT('Ctrl Pts',(-0.277680138024386,1.82137611966157,
4.57437744467291));
#30090=CARTESIAN_POINT('Ctrl Pts',(-0.282723598343368,1.82659141026702,
4.57400816292707));
#30091=CARTESIAN_POINT('Ctrl Pts',(-0.296797343894201,1.84114464719416,
4.57297768444626));
#30092=CARTESIAN_POINT('Ctrl Pts',(-0.309791624911384,1.85683650285156,
4.57194720596545));
#30093=CARTESIAN_POINT('Ctrl Pts',(-0.321516802775297,1.87347884087099,
4.57091672748464));
#30094=CARTESIAN_POINT('Ctrl Pts',(-0.333223256999998,1.89009460316284,
4.56988789454878));
#30095=CARTESIAN_POINT('Ctrl Pts',(-0.34366413939655,1.90765726636389,4.56885906161293));
#30096=CARTESIAN_POINT('Ctrl Pts',(-0.352689122616453,1.92594462723594,
4.56783022867707));
#30097=CARTESIAN_POINT('Ctrl Pts',(-0.361704682477759,1.94421289351744,
4.56680246998828));
#30098=CARTESIAN_POINT('Ctrl Pts',(-0.369306917863024,1.96320369221295,
4.56577471129948));
#30099=CARTESIAN_POINT('Ctrl Pts',(-0.375391091138084,1.98266961734419,
4.56474695261069));
#30100=CARTESIAN_POINT('Ctrl Pts',(-0.381481113779663,2.00215425715129,
4.56371820582754));
#30101=CARTESIAN_POINT('Ctrl Pts',(-0.386049919062549,2.02211421592566,
4.56268945904439));
#30102=CARTESIAN_POINT('Ctrl Pts',(-0.389042356387749,2.04228574754649,
4.56166071226124));
#30103=CARTESIAN_POINT('Ctrl Pts',(-0.391897225723248,2.06152995580087,
4.56067925890865));
#30104=CARTESIAN_POINT('Ctrl Pts',(-0.393317641356229,2.08096605758746,
4.55969780555607));
#30105=CARTESIAN_POINT('Ctrl Pts',(-0.393299834232345,2.10036109944607,
4.55871635220349));
#30106=CARTESIAN_POINT('',(-0.393445918996423,2.09985495139376,4.4337163522035));
#30107=CARTESIAN_POINT('Ctrl Pts',(-0.393310908181485,2.10036110961337,
4.55871635220349));
#30108=CARTESIAN_POINT('Ctrl Pts',(-0.39358942096467,2.13052187855199,4.55719017460375));
#30109=CARTESIAN_POINT('Ctrl Pts',(-0.376632741138322,2.29126728843717,
4.54904054916312));
#30110=CARTESIAN_POINT('Ctrl Pts',(-0.155906186004341,2.5381425209697,4.53426747588148));
#30111=CARTESIAN_POINT('Ctrl Pts',(0.284004796300236,2.46826155993621,4.5143971323587));
#30112=CARTESIAN_POINT('Ctrl Pts',(0.463374845213788,2.06055343100496,4.49452678883592));
#30113=CARTESIAN_POINT('Ctrl Pts',(0.217671564353364,1.6890269994191,4.47465644531311));
#30114=CARTESIAN_POINT('Ctrl Pts',(-0.227735017592104,1.69452228360619,
4.45478610179035));
#30115=CARTESIAN_POINT('Ctrl Pts',(-0.390128315479153,1.95374788316366,
4.44113940408713));
#30116=CARTESIAN_POINT('Ctrl Pts',(-0.393918994188849,2.09198357827423,
4.43411615422485));
#30117=CARTESIAN_POINT('Ctrl Pts',(-0.393882594814329,2.09985479040793,
4.4337163522035));
#30118=CARTESIAN_POINT('',(0.293078184270657,1.8377213925906,4.35670005929419));
#30119=CARTESIAN_POINT('Ctrl Pts',(-0.393299973272956,2.09985500519842,
4.4337163522035));
#30120=CARTESIAN_POINT('Ctrl Pts',(-0.393307473039213,2.12019820258479,
4.43268152877099));
#30121=CARTESIAN_POINT('Ctrl Pts',(-0.39173231746941,2.14060550769227,4.43164670533848));
#30122=CARTESIAN_POINT('Ctrl Pts',(-0.388570851337203,2.16080775847769,
4.43061188190596));
#30123=CARTESIAN_POINT('Ctrl Pts',(-0.38541493166847,2.18097456651554,4.42957887396352));
#30124=CARTESIAN_POINT('Ctrl Pts',(-0.380678279633258,2.2009362922915,4.42854586602108));
#30125=CARTESIAN_POINT('Ctrl Pts',(-0.374409109528847,2.22042719253481,
4.42751285807864));
#30126=CARTESIAN_POINT('Ctrl Pts',(-0.368103856053702,2.24003027626775,
4.42647390446748));
#30127=CARTESIAN_POINT('Ctrl Pts',(-0.360248522858196,2.25915634225469,
4.42543495085633));
#30128=CARTESIAN_POINT('Ctrl Pts',(-0.350943650004022,2.27754842866625,
4.42439599724517));
#30129=CARTESIAN_POINT('Ctrl Pts',(-0.341695228996082,2.29582893190518,
4.42336334687431));
#30130=CARTESIAN_POINT('Ctrl Pts',(-0.331015194686975,2.3133836840058,4.42233069650344));
#30131=CARTESIAN_POINT('Ctrl Pts',(-0.319048907629175,2.32998409627761,
4.42129804613258));
#30132=CARTESIAN_POINT('Ctrl Pts',(-0.306973058247754,2.34673650053598,
4.42025594090128));
#30133=CARTESIAN_POINT('Ctrl Pts',(-0.29358773345619,2.36251636979888,4.41921383566997));
#30134=CARTESIAN_POINT('Ctrl Pts',(-0.279083872946256,2.37712286419803,
4.41817173043867));
#30135=CARTESIAN_POINT('Ctrl Pts',(-0.264580012436322,2.39172935859718,
4.41712962520737));
#30136=CARTESIAN_POINT('Ctrl Pts',(-0.248958245337701,2.40516202011686,
4.41608751997606));
#30137=CARTESIAN_POINT('Ctrl Pts',(-0.232442705828144,2.41726216053493,
4.41504541474476));
#30138=CARTESIAN_POINT('Ctrl Pts',(-0.215920112107219,2.42936746923394,
4.41400286440353));
#30139=CARTESIAN_POINT('Ctrl Pts',(-0.19839928804482,2.44021524029002,4.4129603140623));
#30140=CARTESIAN_POINT('Ctrl Pts',(-0.180098122380582,2.44964204025687,
4.41191776372107));
#30141=CARTESIAN_POINT('Ctrl Pts',(-0.161830718147231,2.45905144995136,
4.41087713664484));
#30142=CARTESIAN_POINT('Ctrl Pts',(-0.142786450456267,2.46704470382945,
4.4098365095686));
#30143=CARTESIAN_POINT('Ctrl Pts',(-0.123211075344355,2.47350223682394,
4.40879588249237));
#30144=CARTESIAN_POINT('Ctrl Pts',(-0.103656718593553,2.47995283627261,
4.40775637275236));
#30145=CARTESIAN_POINT('Ctrl Pts',(-0.0835730745182236,2.48487073034174,
4.40671686301234));
#30146=CARTESIAN_POINT('Ctrl Pts',(-0.0632245156711306,2.48818494383238,
4.40567735327233));
#30147=CARTESIAN_POINT('Ctrl Pts',(-0.0428651243813793,2.49150092162623,
4.40463729015506));
#30148=CARTESIAN_POINT('Ctrl Pts',(-0.0222412624082241,2.49321137882844,
4.4035972270378));
#30149=CARTESIAN_POINT('Ctrl Pts',(-0.0016265849958498,2.4932966364225,
4.40255716392053));
#30150=CARTESIAN_POINT('Ctrl Pts',(0.0189945776486265,2.493381920838,4.40151677360674));
#30151=CARTESIAN_POINT('Ctrl Pts',(0.0396058124959531,2.49184102187124,
4.40047638329295));
#30152=CARTESIAN_POINT('Ctrl Pts',(0.0599353663630418,2.48870636971746,
4.39943599297916));
#30153=CARTESIAN_POINT('Ctrl Pts',(0.0803095879231295,2.48556483016808,
4.39839331674039));
#30154=CARTESIAN_POINT('Ctrl Pts',(0.100400174222778,2.48082271714529,4.39735064050161));
#30155=CARTESIAN_POINT('Ctrl Pts',(0.11994670300977,2.47456331699338,4.39630796426284));
#30156=CARTESIAN_POINT('Ctrl Pts',(0.12702596232744,2.47229632026311,4.39593033324922));
#30157=CARTESIAN_POINT('Ctrl Pts',(0.134034034163761,2.46983076463011,4.39555270223559));
#30158=CARTESIAN_POINT('Ctrl Pts',(0.1409592423106,2.4671721421993,4.39517507122197));
#30159=CARTESIAN_POINT('Ctrl Pts',(0.160140515404261,2.45980835445211,4.39412911802499));
#30160=CARTESIAN_POINT('Ctrl Pts',(0.17879941889945,2.45091589366128,4.393083164828));
#30161=CARTESIAN_POINT('Ctrl Pts',(0.196679518697313,2.44059074697501,4.39203721163102));
#30162=CARTESIAN_POINT('Ctrl Pts',(0.21452659328169,2.43028467122108,4.39099319034874));
#30163=CARTESIAN_POINT('Ctrl Pts',(0.231597062858027,2.41855147410596,4.38994916906646));
#30164=CARTESIAN_POINT('Ctrl Pts',(0.247656429732667,2.40553425800075,4.38890514778418));
#30165=CARTESIAN_POINT('Ctrl Pts',(0.263698306885079,2.39253121851257,4.38786226351074));
#30166=CARTESIAN_POINT('Ctrl Pts',(0.278730683003493,2.37824737297298,4.38681937923731));
#30167=CARTESIAN_POINT('Ctrl Pts',(0.29254990300435,2.36286773147754,4.38577649496387));
#30168=CARTESIAN_POINT('Ctrl Pts',(0.306375559559247,2.34748092663324,4.38473312494805));
#30169=CARTESIAN_POINT('Ctrl Pts',(0.318986428939915,2.33099783993888,4.38368975493222));
#30170=CARTESIAN_POINT('Ctrl Pts',(0.330216985574048,2.3136390236787,4.3826463849164));
#30171=CARTESIAN_POINT('Ctrl Pts',(0.341450687666683,2.29627534555478,4.3816027226731));
#30172=CARTESIAN_POINT('Ctrl Pts',(0.351302938472491,2.27803608295674,4.38055906042981));
#30173=CARTESIAN_POINT('Ctrl Pts',(0.359653019480331,2.25916845032443,4.37951539818652));
#30174=CARTESIAN_POINT('Ctrl Pts',(0.368020583496849,2.24026131352627,4.37846955077209));
#30175=CARTESIAN_POINT('Ctrl Pts',(0.374879453596798,2.22072387138932,4.37742370335765));
#30176=CARTESIAN_POINT('Ctrl Pts',(0.380157769311558,2.20082142843692,4.37637785594322));
#30177=CARTESIAN_POINT('Ctrl Pts',(0.381963102669721,2.19401422968023,4.37602014652854));
#30178=CARTESIAN_POINT('Ctrl Pts',(0.383583977842243,2.18716442574047,4.37566243711386));
#30179=CARTESIAN_POINT('Ctrl Pts',(0.385018902038723,2.18028284420034,4.37530472769918));
#30180=CARTESIAN_POINT('Ctrl Pts',(0.389170687082921,2.16037179427255,4.37426973741769));
#30181=CARTESIAN_POINT('Ctrl Pts',(0.391786937179193,2.14007437079021,4.37323474713619));
#30182=CARTESIAN_POINT('Ctrl Pts',(0.392808659387981,2.11965317047748,4.3721997568547));
#30183=CARTESIAN_POINT('Ctrl Pts',(0.393828534995012,2.09926887826369,4.37116663715491));
#30184=CARTESIAN_POINT('Ctrl Pts',(0.393259502817064,2.07876199016779,4.37013351745512));
#30185=CARTESIAN_POINT('Ctrl Pts',(0.391094023194851,2.05840246375967,4.36910039775533));
#30186=CARTESIAN_POINT('Ctrl Pts',(0.388928036664634,2.03803817147577,4.3680670362169));
#30187=CARTESIAN_POINT('Ctrl Pts',(0.385164873135253,2.01782206049515,4.36703367467847));
#30188=CARTESIAN_POINT('Ctrl Pts',(0.379849126078133,1.99802190716787,4.36600031314005));
#30189=CARTESIAN_POINT('Ctrl Pts',(0.374537207809709,1.978236015355,4.36496769590396));
#30190=CARTESIAN_POINT('Ctrl Pts',(0.367675141274041,1.95886620608699,4.36393507866787));
#30191=CARTESIAN_POINT('Ctrl Pts',(0.359357831763001,1.94016621524035,4.36290246143178));
#30192=CARTESIAN_POINT('Ctrl Pts',(0.351021974972372,1.92142452413498,4.36186754149906));
#30193=CARTESIAN_POINT('Ctrl Pts',(0.341224718531711,1.90335631496584,4.36083262156635));
#30194=CARTESIAN_POINT('Ctrl Pts',(0.330108221488342,1.88619295590228,4.35979770163363));
#30195=CARTESIAN_POINT('Ctrl Pts',(0.319017208287179,1.86906894271651,4.35876515418715));
#30196=CARTESIAN_POINT('Ctrl Pts',(0.306613508066773,1.85284617978107,4.35773260674067));
#30197=CARTESIAN_POINT('Ctrl Pts',(0.293078184270657,1.8377213925906,4.35670005929419));
#30198=CARTESIAN_POINT('',(0.287740166859834,1.83187598694732,4.3567));
#30199=CARTESIAN_POINT('Ctrl Pts',(0.293078184270657,1.8377213925906,4.3567));
#30200=CARTESIAN_POINT('Ctrl Pts',(0.291298845133716,1.83577292404284,4.3567));
#30201=CARTESIAN_POINT('Ctrl Pts',(0.289519505996775,1.83382445549508,4.3567));
#30202=CARTESIAN_POINT('Ctrl Pts',(0.287740166859834,1.83187598694732,4.3567));
#30203=CARTESIAN_POINT('',(0.386085631082133,2.17498516834622,4.3567));
#30204=CARTESIAN_POINT('Origin',(0.,2.1,4.3567));
#30205=CARTESIAN_POINT('',(-0.393882850542516,2.09986682733705,4.41538364779653));
#30206=CARTESIAN_POINT('Ctrl Pts',(0.386085631082133,2.17498516834622,4.3567));
#30207=CARTESIAN_POINT('Ctrl Pts',(0.36112075890231,2.30352496685583,4.36332344784093));
#30208=CARTESIAN_POINT('Ctrl Pts',(0.173109802419442,2.53147029156881,4.37657034352279));
#30209=CARTESIAN_POINT('Ctrl Pts',(-0.263054777401013,2.47987360215571,
4.39613155945497));
#30210=CARTESIAN_POINT('Ctrl Pts',(-0.393452793012018,2.22418599272304,
4.40906932754621));
#30211=CARTESIAN_POINT('Ctrl Pts',(-0.393882850542516,2.09986682733705,
4.41538364779653));
#30212=CARTESIAN_POINT('',(-0.393255881934822,2.1003613435798,4.54038364779653));
#30213=CARTESIAN_POINT('Ctrl Pts',(-0.393882850542516,2.09986682733705,
4.41538364779653));
#30214=CARTESIAN_POINT('Ctrl Pts',(-0.393903904692916,2.09378058486925,
4.41569277538714));
#30215=CARTESIAN_POINT('Ctrl Pts',(-0.390978467245773,1.95731419778572,
4.42262535081861));
#30216=CARTESIAN_POINT('Ctrl Pts',(-0.233315454838252,1.69771858502018,
4.43618137409123));
#30217=CARTESIAN_POINT('Ctrl Pts',(0.212061907806772,1.6860660404583,4.4560517176139));
#30218=CARTESIAN_POINT('Ctrl Pts',(0.4627766764693,2.05423342872913,4.47592206113677));
#30219=CARTESIAN_POINT('Ctrl Pts',(0.289021540344744,2.46433772613338,4.4957924046595));
#30220=CARTESIAN_POINT('Ctrl Pts',(-0.149905097511465,2.5402365181872,4.51566274818232));
#30221=CARTESIAN_POINT('Ctrl Pts',(-0.375357159811075,2.29490204802152,
4.53052649589464));
#30222=CARTESIAN_POINT('Ctrl Pts',(-0.393547872205643,2.13232530629972,
4.53876679576605));
#30223=CARTESIAN_POINT('Ctrl Pts',(-0.393255881934822,2.1003613435798,4.54038364779653));
#30224=CARTESIAN_POINT('',(-0.393062271237487,2.09992472497766,4.66538365014497));
#30225=CARTESIAN_POINT('Ctrl Pts',(-0.393255881934822,2.1003613435798,4.54038364779653));
#30226=CARTESIAN_POINT('Ctrl Pts',(-0.39235173162358,2.00138466617034,4.54539024360698));
#30227=CARTESIAN_POINT('Ctrl Pts',(-0.304249124076242,1.77003449934502,
4.55702028725837));
#30228=CARTESIAN_POINT('Ctrl Pts',(0.0846189449362708,1.64270878203361,
4.57527377875067));
#30229=CARTESIAN_POINT('Ctrl Pts',(0.430303245215323,1.92360908410859,4.59514412227347));
#30230=CARTESIAN_POINT('Ctrl Pts',(0.381244165381663,2.36632310413653,4.61501446579626));
#30231=CARTESIAN_POINT('Ctrl Pts',(-0.0175551922214225,2.56472241761119,
4.63488480931905));
#30232=CARTESIAN_POINT('Ctrl Pts',(-0.340918328246028,2.37213778114564,
4.65167453665247));
#30233=CARTESIAN_POINT('Ctrl Pts',(-0.392545913529889,2.1702301438735,4.66184081614497));
#30234=CARTESIAN_POINT('Ctrl Pts',(-0.392665676133501,2.09992484756078,
4.66538364779653));
#30235=CARTESIAN_POINT('',(-0.393336985380828,2.09966984214535,4.79038364779653));
#30236=CARTESIAN_POINT('Ctrl Pts',(-0.393299992782359,2.09992465150058,
4.66538365155264));
#30237=CARTESIAN_POINT('Ctrl Pts',(-0.393295769512778,2.07788025900139,
4.66649272362475));
#30238=CARTESIAN_POINT('Ctrl Pts',(-0.391433911723158,2.05588325308345,
4.66760179569686));
#30239=CARTESIAN_POINT('Ctrl Pts',(-0.387763466838727,2.03423995297134,
4.66871086776897));
#30240=CARTESIAN_POINT('Ctrl Pts',(-0.384073922335051,2.01248402923884,
4.66982571103638));
#30241=CARTESIAN_POINT('Ctrl Pts',(-0.378557116761919,1.99108606085747,
4.6709405543038));
#30242=CARTESIAN_POINT('Ctrl Pts',(-0.371313017604665,1.97034070431582,
4.67205539757122));
#30243=CARTESIAN_POINT('Ctrl Pts',(-0.365746300725396,1.95439896692102,
4.67291209716902));
#30244=CARTESIAN_POINT('Ctrl Pts',(-0.359160659068457,1.938842327753,4.67376879676682));
#30245=CARTESIAN_POINT('Ctrl Pts',(-0.351620062476746,1.92379494427273,
4.67462549636463));
#30246=CARTESIAN_POINT('Ctrl Pts',(-0.342431196821245,1.90545841299364,
4.67566945852539));
#30247=CARTESIAN_POINT('Ctrl Pts',(-0.331776750804907,1.88778796277536,
4.67671342068616));
#30248=CARTESIAN_POINT('Ctrl Pts',(-0.319776634642432,1.87102883601475,
4.67775738284692));
#30249=CARTESIAN_POINT('Ctrl Pts',(-0.307798594125831,1.85430053966798,
4.6787994245147));
#30250=CARTESIAN_POINT('Ctrl Pts',(-0.294480172437816,1.83848086511535,
4.67984146618247));
#30251=CARTESIAN_POINT('Ctrl Pts',(-0.27998605802235,1.82378867272846,4.68088350785025));
#30252=CARTESIAN_POINT('Ctrl Pts',(-0.265507510197148,1.80911225966637,
4.68192443037164));
#30253=CARTESIAN_POINT('Ctrl Pts',(-0.24985626990208,1.79556146627513,4.68296535289304));
#30254=CARTESIAN_POINT('Ctrl Pts',(-0.2332357341274,1.78332037904839,4.68400627541443));
#30255=CARTESIAN_POINT('Ctrl Pts',(-0.216606662603788,1.77107300521041,
4.68504773251867));
#30256=CARTESIAN_POINT('Ctrl Pts',(-0.199007883991114,1.76013713059733,
4.68608918962291));
#30257=CARTESIAN_POINT('Ctrl Pts',(-0.180674443153325,1.7506554199773,4.68713064672715));
#30258=CARTESIAN_POINT('Ctrl Pts',(-0.16233540074126,1.74117081232846,4.68817242203676));
#30259=CARTESIAN_POINT('Ctrl Pts',(-0.143261918860075,1.73314155875621,
4.68921419734637));
#30260=CARTESIAN_POINT('Ctrl Pts',(-0.123711142893961,1.72666309702379,
4.69025597265598));
#30261=CARTESIAN_POINT('Ctrl Pts',(-0.104118107463642,1.72017063194326,
4.69129999978754));
#30262=CARTESIAN_POINT('Ctrl Pts',(-0.084046433425361,1.71523582678645,
4.6923440269191));
#30263=CARTESIAN_POINT('Ctrl Pts',(-0.063766420372174,1.71190370572122,
4.69338805405065));
#30264=CARTESIAN_POINT('Ctrl Pts',(-0.0565935827607402,1.7107251678554,
4.69375731599624));
#30265=CARTESIAN_POINT('Ctrl Pts',(-0.0493947352562634,1.70974664603408,
4.69412657794183));
#30266=CARTESIAN_POINT('Ctrl Pts',(-0.0421819163230374,1.70896857423563,
4.69449583988742));
#30267=CARTESIAN_POINT('Ctrl Pts',(-0.0217901178502496,1.70676884019846,
4.69553980276072));
#30268=CARTESIAN_POINT('Ctrl Pts',(-0.00116502768758128,1.70616195661353,
4.69658376563402));
#30269=CARTESIAN_POINT('Ctrl Pts',(0.0194222400179982,1.70717985465014,
4.69762772850732));
#30270=CARTESIAN_POINT('Ctrl Pts',(0.039971635303871,1.70819588015747,4.69866977090236));
#30271=CARTESIAN_POINT('Ctrl Pts',(0.0604826167254509,1.71083077780269,
4.6997118132974));
#30272=CARTESIAN_POINT('Ctrl Pts',(0.0806820134259272,1.71506454734652,
4.70075385569243));
#30273=CARTESIAN_POINT('Ctrl Pts',(0.100859716349234,1.71929376990043,4.70179477895328));
#30274=CARTESIAN_POINT('Ctrl Pts',(0.120725776473047,1.72511833351522,4.70283570221412));
#30275=CARTESIAN_POINT('Ctrl Pts',(0.140015307863677,1.7324668673931,4.70387662547497));
#30276=CARTESIAN_POINT('Ctrl Pts',(0.159314745876898,1.73981917529484,4.70491808332806));
#30277=CARTESIAN_POINT('Ctrl Pts',(0.178036370321091,1.74869677019204,4.70595954118115));
#30278=CARTESIAN_POINT('Ctrl Pts',(0.195932991866882,1.75897924887466,4.70700099903424));
#30279=CARTESIAN_POINT('Ctrl Pts',(0.213835081627622,1.76926486931247,4.70804277509909));
#30280=CARTESIAN_POINT('Ctrl Pts',(0.23091104725502,1.78095583046984,4.70908455116394));
#30281=CARTESIAN_POINT('Ctrl Pts',(0.246941445344783,1.79388758180853,4.71012632722879));
#30282=CARTESIAN_POINT('Ctrl Pts',(0.263006493465729,1.80684728539049,4.71117035511377));
#30283=CARTESIAN_POINT('Ctrl Pts',(0.278020927055499,1.82105262746797,4.71221438299874));
#30284=CARTESIAN_POINT('Ctrl Pts',(0.291800570764912,1.83630070743123,4.71325841088372));
#30285=CARTESIAN_POINT('Ctrl Pts',(0.296674230733087,1.841693731988,4.71362766839255));
#30286=CARTESIAN_POINT('Ctrl Pts',(0.3013937969224,1.84721689521838,4.71399692590138));
#30287=CARTESIAN_POINT('Ctrl Pts',(0.305952388048845,1.85286031025509,4.71436618341021));
#30288=CARTESIAN_POINT('Ctrl Pts',(0.318840410004825,1.86881533997423,4.71541014606209));
#30289=CARTESIAN_POINT('Ctrl Pts',(0.330515420489601,1.88582876395813,4.71645410871397));
#30290=CARTESIAN_POINT('Ctrl Pts',(0.340803812214894,1.90368990963327,4.71749807136584));
#30291=CARTESIAN_POINT('Ctrl Pts',(0.35107327734531,1.92151819782424,4.71854011353698));
#30292=CARTESIAN_POINT('Ctrl Pts',(0.359960772381131,1.94019051152622,4.71958215570812));
#30293=CARTESIAN_POINT('Ctrl Pts',(0.367335241547277,1.95946633742265,4.72062419787925));
#30294=CARTESIAN_POINT('Ctrl Pts',(0.374701790656649,1.97872146140387,4.72166512091449));
#30295=CARTESIAN_POINT('Ctrl Pts',(0.380558251252852,1.99857813743754,4.72270604394973));
#30296=CARTESIAN_POINT('Ctrl Pts',(0.384821245619206,2.01877501049503,4.72374696698497));
#30297=CARTESIAN_POINT('Ctrl Pts',(0.389086429354271,2.03898225616813,4.7247884246126));
#30298=CARTESIAN_POINT('Ctrl Pts',(0.391756344222165,2.05952933132301,4.72582988224022));
#30299=CARTESIAN_POINT('Ctrl Pts',(0.392798419325999,2.08014321841293,4.72687133986785));
#30300=CARTESIAN_POINT('Ctrl Pts',(0.393840812830054,2.10076340396077,4.72791311570703));
#30301=CARTESIAN_POINT('Ctrl Pts',(0.39325437542767,2.12144970603567,4.72895489154621));
#30302=CARTESIAN_POINT('Ctrl Pts',(0.391058675456665,2.1419285386113,4.72999666738539));
#30303=CARTESIAN_POINT('Ctrl Pts',(0.388858229427969,2.16245163667043,4.73104069504781));
#30304=CARTESIAN_POINT('Ctrl Pts',(0.385041712244149,2.18276564610716,4.73208472271024));
#30305=CARTESIAN_POINT('Ctrl Pts',(0.379680028905663,2.20260587532006,4.73312875037266));
#30306=CARTESIAN_POINT('Ctrl Pts',(0.377783672024161,2.20962310345966,4.73349800922611));
#30307=CARTESIAN_POINT('Ctrl Pts',(0.375694477057357,2.21658121279524,4.73386726807955));
#30308=CARTESIAN_POINT('Ctrl Pts',(0.373417032150404,2.2234690653564,4.734236526933));
#30309=CARTESIAN_POINT('Ctrl Pts',(0.36697827720004,2.24294228933658,4.73528048951727));
#30310=CARTESIAN_POINT('Ctrl Pts',(0.358992980580432,2.26196851967134,4.73632445210155));
#30311=CARTESIAN_POINT('Ctrl Pts',(0.349544302746481,2.28028774339227,4.73736841468582));
#30312=CARTESIAN_POINT('Ctrl Pts',(0.340113006788501,2.29857326689818,4.73841045678677));
#30313=CARTESIAN_POINT('Ctrl Pts',(0.329223953843854,2.31615369166456,4.73945249888773));
#30314=CARTESIAN_POINT('Ctrl Pts',(0.317008428904983,2.33278862945426,4.74049454098868));
#30315=CARTESIAN_POINT('Ctrl Pts',(0.304806023264139,2.34940570156012,4.74153546395141));
#30316=CARTESIAN_POINT('Ctrl Pts',(0.291280383801512,2.36507869541469,4.74257638691414));
#30317=CARTESIAN_POINT('Ctrl Pts',(0.276606128593381,2.37959602934338,4.74361730987687));
#30318=CARTESIAN_POINT('Ctrl Pts',(0.261924337086183,2.39412081898062,4.74465876742938));
#30319=CARTESIAN_POINT('Ctrl Pts',(0.246093263074994,2.40748823405086,4.74570022498188));
#30320=CARTESIAN_POINT('Ctrl Pts',(0.229324833344335,2.41952309902665,4.74674168253438));
#30321=CARTESIAN_POINT('Ctrl Pts',(0.212551280139252,2.43156164116982,4.74778345829683));
#30322=CARTESIAN_POINT('Ctrl Pts',(0.194840419405803,2.44226642341539,4.74882523405928));
#30323=CARTESIAN_POINT('Ctrl Pts',(0.176432879831052,2.45150580210648,4.74986700982173));
#30324=CARTESIAN_POINT('Ctrl Pts',(0.157985551941207,2.46076515192457,4.75091103740617));
#30325=CARTESIAN_POINT('Ctrl Pts',(0.138839220988392,2.46855249695004,4.7519550649906));
#30326=CARTESIAN_POINT('Ctrl Pts',(0.11925482653518,2.47478417302237,4.75299909257504));
#30327=CARTESIAN_POINT('Ctrl Pts',(0.112328075011662,2.47698823768372,4.75336835186862));
#30328=CARTESIAN_POINT('Ctrl Pts',(0.105346644754062,2.47899815808783,4.75373761116221));
#30329=CARTESIAN_POINT('Ctrl Pts',(0.0983223844569184,2.48081176283658,
4.75410687045579));
#30330=CARTESIAN_POINT('Ctrl Pts',(0.0784635325716178,2.48593915085474,
4.75515083313775));
#30331=CARTESIAN_POINT('Ctrl Pts',(0.0581433500240972,2.48952421285417,
4.7561947958197));
#30332=CARTESIAN_POINT('Ctrl Pts',(0.0376254766890382,2.4914961219526,4.75723875850166));
#30333=CARTESIAN_POINT('Ctrl Pts',(0.0171453481802259,2.49346440351297,
4.75828080070242));
#30334=CARTESIAN_POINT('Ctrl Pts',(-0.00353103079621325,2.4938252938848,
4.75932284290317));
#30335=CARTESIAN_POINT('Ctrl Pts',(-0.0241304705196809,2.49255905338242,
4.76036488510393));
#30336=CARTESIAN_POINT('Ctrl Pts',(-0.0447077867783312,2.49129417280184,
4.76140580816822));
#30337=CARTESIAN_POINT('Ctrl Pts',(-0.0652075953844509,2.48840564662385,
4.76244673123252));
#30338=CARTESIAN_POINT('Ctrl Pts',(-0.085357470718213,2.48392576390832,
4.76348765429682));
#30339=CARTESIAN_POINT('Ctrl Pts',(-0.105517694507556,2.47944358044073,
4.76452911195233));
#30340=CARTESIAN_POINT('Ctrl Pts',(-0.125326904251082,2.47336855164252,
4.76557056960783));
#30341=CARTESIAN_POINT('Ctrl Pts',(-0.144523089397569,2.46578404370746,
4.76661202726333));
#30342=CARTESIAN_POINT('Ctrl Pts',(-0.163725139818961,2.4581972183732,4.76765380312974));
#30343=CARTESIAN_POINT('Ctrl Pts',(-0.182313122331425,2.44910029953093,
4.76869557899614));
#30344=CARTESIAN_POINT('Ctrl Pts',(-0.200046091905373,2.43862435103428,
4.76973735486255));
#30345=CARTESIAN_POINT('Ctrl Pts',(-0.217817391689976,2.42812575854047,
4.77078138255081));
#30346=CARTESIAN_POINT('Ctrl Pts',(-0.234729386239739,2.41624260877569,
4.77182541023907));
#30347=CARTESIAN_POINT('Ctrl Pts',(-0.250570477902909,2.40314901550806,
4.77286943792733));
#30348=CARTESIAN_POINT('Ctrl Pts',(-0.256173260973188,2.39851798601535,
4.77323869661108));
#30349=CARTESIAN_POINT('Ctrl Pts',(-0.261642403097666,2.3937358883794,4.77360795529483));
#30350=CARTESIAN_POINT('Ctrl Pts',(-0.26696966465499,2.38881150973256,4.77397721397858));
#30351=CARTESIAN_POINT('Ctrl Pts',(-0.281806371321473,2.37509685339147,
4.77500561904484));
#30352=CARTESIAN_POINT('Ctrl Pts',(-0.29563393681208,2.36018897340975,4.7760340241111));
#30353=CARTESIAN_POINT('Ctrl Pts',(-0.308252937633149,2.344264234878,4.77706242917736));
#30354=CARTESIAN_POINT('Ctrl Pts',(-0.320848406880124,2.32836919237132,
4.77808891650145));
#30355=CARTESIAN_POINT('Ctrl Pts',(-0.332239266041854,2.31146160149699,
4.77911540382553));
#30356=CARTESIAN_POINT('Ctrl Pts',(-0.342263524440448,2.29375388986444,
4.78014189114962));
#30357=CARTESIAN_POINT('Ctrl Pts',(-0.352282526817308,2.27605546292045,
4.78116784025538));
#30358=CARTESIAN_POINT('Ctrl Pts',(-0.360935939505943,2.25755838482288,
4.78219378936113));
#30359=CARTESIAN_POINT('Ctrl Pts',(-0.368105650349287,2.23850314141177,
4.78321973846688));
#30360=CARTESIAN_POINT('Ctrl Pts',(-0.375273320297017,2.21945332217515,
4.78424539553086));
#30361=CARTESIAN_POINT('Ctrl Pts',(-0.380957869115705,2.19984636711062,
4.78527105259485));
#30362=CARTESIAN_POINT('Ctrl Pts',(-0.385090057524706,2.1799408380968,4.78629670965883));
#30363=CARTESIAN_POINT('Ctrl Pts',(-0.389227985100154,2.16000766243841,
4.78732379125046));
#30364=CARTESIAN_POINT('Ctrl Pts',(-0.391809133214506,2.13977583627541,
4.78835087284208));
#30365=CARTESIAN_POINT('Ctrl Pts',(-0.392815682131082,2.11951230052794,
4.78937795443371));
#30366=CARTESIAN_POINT('Ctrl Pts',(-0.393144211553025,2.11289844642109,
4.78971318555465));
#30367=CARTESIAN_POINT('Ctrl Pts',(-0.393305410862432,2.10628122371761,
4.79004841667559));
#30368=CARTESIAN_POINT('Ctrl Pts',(-0.393299861449716,2.09966987330631,
4.79038364779653));
#30369=CARTESIAN_POINT('',(-0.393440202014609,2.10025343067764,4.91538364779653));
#30370=CARTESIAN_POINT('Ctrl Pts',(-0.393533145238993,2.09966967749336,
4.79038364779653));
#30371=CARTESIAN_POINT('Ctrl Pts',(-0.39373784894553,2.07688450824866,4.79153828436481));
#30372=CARTESIAN_POINT('Ctrl Pts',(-0.381557546592789,1.92361338030581,
4.79931636877403));
#30373=CARTESIAN_POINT('Ctrl Pts',(-0.180195773708327,1.67127570200156,
4.81371790102414));
#30374=CARTESIAN_POINT('Ctrl Pts',(0.262935837116425,1.71641195809303,4.83358824454696));
#30375=CARTESIAN_POINT('Ctrl Pts',(0.464859613354694,2.11343802147946,4.85345858806974));
#30376=CARTESIAN_POINT('Ctrl Pts',(0.240337979009523,2.49813652976592,4.87332893159252));
#30377=CARTESIAN_POINT('Ctrl Pts',(-0.204661031884562,2.51759897328978,
4.89319927511531));
#30378=CARTESIAN_POINT('Ctrl Pts',(-0.386147435745799,2.26106486793884,
4.90721751384998));
#30379=CARTESIAN_POINT('Ctrl Pts',(-0.393853325308977,2.11545426420355,
4.91461230474372));
#30380=CARTESIAN_POINT('Ctrl Pts',(-0.393739520313072,2.10025362348061,
4.91538364779653));
#30381=CARTESIAN_POINT('',(-0.39310121130446,2.10019150475592,5.0403836450683));
#30382=CARTESIAN_POINT('Ctrl Pts',(-0.393299918406659,2.10025334031532,
4.91538364779653));
#30383=CARTESIAN_POINT('Ctrl Pts',(-0.393312967850958,2.07999464058418,
4.91641281199908));
#30384=CARTESIAN_POINT('Ctrl Pts',(-0.391756457283335,2.05967378052778,
4.91744197620162));
#30385=CARTESIAN_POINT('Ctrl Pts',(-0.388627900065919,2.03955791788535,
4.91847114040417));
#30386=CARTESIAN_POINT('Ctrl Pts',(-0.385504269603249,2.0194737330787,4.9194986839109));
#30387=CARTESIAN_POINT('Ctrl Pts',(-0.380813566429206,1.99959465497,4.92052622741762));
#30388=CARTESIAN_POINT('Ctrl Pts',(-0.374605164255451,1.98018405401139,
4.92155377092434));
#30389=CARTESIAN_POINT('Ctrl Pts',(-0.368396369260136,1.96077222489417,
4.92258137944639));
#30390=CARTESIAN_POINT('Ctrl Pts',(-0.360669872719226,1.94182966575812,
4.92360898796843));
#30391=CARTESIAN_POINT('Ctrl Pts',(-0.351525349917601,1.92360607049757,
4.92463659649047));
#30392=CARTESIAN_POINT('Ctrl Pts',(-0.342381329015625,1.90538347544406,
4.92566414861194));
#30393=CARTESIAN_POINT('Ctrl Pts',(-0.331819794710035,1.88788043413982,
4.9266917007334));
#30394=CARTESIAN_POINT('Ctrl Pts',(-0.319986573370135,1.87132231664887,
4.92771925285487));
#30395=CARTESIAN_POINT('Ctrl Pts',(-0.308127343858601,1.85472780616322,
4.92874906342745));
#30396=CARTESIAN_POINT('Ctrl Pts',(-0.294991322080486,1.83908295917413,
4.92977887400003));
#30397=CARTESIAN_POINT('Ctrl Pts',(-0.280765301029734,1.82458079998358,
4.93080868457261));
#30398=CARTESIAN_POINT('Ctrl Pts',(-0.270951327909145,1.81457633000714,
4.93151911043537));
#30399=CARTESIAN_POINT('Ctrl Pts',(-0.260619465562916,1.80511495377878,
4.93222953629813));
#30400=CARTESIAN_POINT('Ctrl Pts',(-0.249840037995042,1.79624871125436,
4.93293996216089));
#30401=CARTESIAN_POINT('Ctrl Pts',(-0.233999792961889,1.78321986967388,
4.93398392480855));
#30402=CARTESIAN_POINT('Ctrl Pts',(-0.217090450655174,1.77139461696758,
4.93502788745621));
#30403=CARTESIAN_POINT('Ctrl Pts',(-0.199321137606527,1.76094841970101,
4.93607185010387));
#30404=CARTESIAN_POINT('Ctrl Pts',(-0.181584513123947,1.75052143933994,
4.93711389226974));
#30405=CARTESIAN_POINT('Ctrl Pts',(-0.162991655113017,1.74146889867327,
4.93815593443562));
#30406=CARTESIAN_POINT('Ctrl Pts',(-0.143781906589812,1.73392397874567,
4.9391979766015));
#30407=CARTESIAN_POINT('Ctrl Pts',(-0.124592789034708,1.72638716194354,
4.94023889963046));
#30408=CARTESIAN_POINT('Ctrl Pts',(-0.104788767051975,1.72035504599876,
4.94127982265942));
#30409=CARTESIAN_POINT('Ctrl Pts',(-0.0846304468739844,1.71591332037949,
4.94232074568838));
#30410=CARTESIAN_POINT('Ctrl Pts',(-0.0644617739081169,1.7114693136057,
4.94336220330829));
#30411=CARTESIAN_POINT('Ctrl Pts',(-0.0439391543082961,1.70861750297522,
4.94440366092819));
#30412=CARTESIAN_POINT('Ctrl Pts',(-0.023335306402776,1.70739287643359,
4.94544511854809));
#30413=CARTESIAN_POINT('Ctrl Pts',(-0.00272516312345551,1.70616787571517,
4.9464868943787));
#30414=CARTESIAN_POINT('Ctrl Pts',(0.0179655218600142,1.70657105634623,
4.94752867020931));
#30415=CARTESIAN_POINT('Ctrl Pts',(0.0384629999241706,1.70858527411857,
4.94857044603992));
#30416=CARTESIAN_POINT('Ctrl Pts',(0.0590047837522991,1.71060384566834,
4.94961447369263));
#30417=CARTESIAN_POINT('Ctrl Pts',(0.0793518019106534,1.71424027701707,
4.95065850134533));
#30418=CARTESIAN_POINT('Ctrl Pts',(0.0992387451231446,1.71942601052307,
4.95170252899804));
#30419=CARTESIAN_POINT('Ctrl Pts',(0.106272496251066,1.72126013648739,4.95207178789325));
#30420=CARTESIAN_POINT('Ctrl Pts',(0.113248838991173,1.72328761667799,4.95244104678847));
#30421=CARTESIAN_POINT('Ctrl Pts',(0.120156595165249,1.72550396178558,4.95281030568368));
#30422=CARTESIAN_POINT('Ctrl Pts',(0.139686089288282,1.73176997605455,4.95385426833121));
#30423=CARTESIAN_POINT('Ctrl Pts',(0.158782306008209,1.73958643085733,4.95489823097873));
#30424=CARTESIAN_POINT('Ctrl Pts',(0.177184505924877,1.74887247208435,4.95594219362625));
#30425=CARTESIAN_POINT('Ctrl Pts',(0.19555285301185,1.7581414306379,4.956984235792));
#30426=CARTESIAN_POINT('Ctrl Pts',(0.213229041275652,1.76887433471324,4.95802627795774));
#30427=CARTESIAN_POINT('Ctrl Pts',(0.22997152901017,1.78094203372314,4.95906832012348));
#30428=CARTESIAN_POINT('Ctrl Pts',(0.246696035575856,1.79299677221387,4.9601092431523));
#30429=CARTESIAN_POINT('Ctrl Pts',(0.262488221597581,1.8063830551189,4.96115016618113));
#30430=CARTESIAN_POINT('Ctrl Pts',(0.277134966973898,1.82092814530953,4.96219108920995));
#30431=CARTESIAN_POINT('Ctrl Pts',(0.291789234536915,1.83548070547942,4.96323254682972));
#30432=CARTESIAN_POINT('Ctrl Pts',(0.305296352784089,1.85119275485768,4.96427400444948));
#30433=CARTESIAN_POINT('Ctrl Pts',(0.317479275865602,1.86785392659825,4.96531546206924));
#30434=CARTESIAN_POINT('Ctrl Pts',(0.329665921361247,1.88452018905314,4.96635723789971));
#30435=CARTESIAN_POINT('Ctrl Pts',(0.340527161506805,1.90213553639867,4.96739901373018));
#30436=CARTESIAN_POINT('Ctrl Pts',(0.349929226383304,1.92046051542131,4.96844078956065));
#30437=CARTESIAN_POINT('Ctrl Pts',(0.359351614036396,1.93882510430195,4.96948481721322));
#30438=CARTESIAN_POINT('Ctrl Pts',(0.367308246027899,1.95790170746229,4.97052884486579));
#30439=CARTESIAN_POINT('Ctrl Pts',(0.373713150145471,1.97743013662262,4.97157287251835));
#30440=CARTESIAN_POINT('Ctrl Pts',(0.375978480779071,1.98433708604621,4.97194213141439));
#30441=CARTESIAN_POINT('Ctrl Pts',(0.37805015951883,1.99130043160611,4.97231139031043));
#30442=CARTESIAN_POINT('Ctrl Pts',(0.379925910106522,1.99830834434561,4.97268064920647));
#30443=CARTESIAN_POINT('Ctrl Pts',(0.385229001164475,2.01812099941161,4.97372461185401));
#30444=CARTESIAN_POINT('Ctrl Pts',(0.38899391317474,2.03840862855515,4.97476857450155));
#30445=CARTESIAN_POINT('Ctrl Pts',(0.391147486771727,2.05890822962974,4.97581253714909));
#30446=CARTESIAN_POINT('Ctrl Pts',(0.39329709863802,2.0793701194792,4.97685457931485));
#30447=CARTESIAN_POINT('Ctrl Pts',(0.39384112082101,2.10004248996021,4.97789662148061));
#30448=CARTESIAN_POINT('Ctrl Pts',(0.392757394556891,2.12065233693515,4.97893866364636));
#30449=CARTESIAN_POINT('Ctrl Pts',(0.391674832197754,2.14124004925822,4.97997958667521));
#30450=CARTESIAN_POINT('Ctrl Pts',(0.388968001498133,2.16176463882623,4.98102050970405));
#30451=CARTESIAN_POINT('Ctrl Pts',(0.384666777166834,2.18195340471317,4.98206143273289));
#30452=CARTESIAN_POINT('Ctrl Pts',(0.380363343838828,2.20215253902407,4.98310289035267));
#30453=CARTESIAN_POINT('Ctrl Pts',(0.374464018572094,2.22201478211032,4.98414434797245));
#30454=CARTESIAN_POINT('Ctrl Pts',(0.36704984345978,2.24127739527664,4.98518580559222));
#30455=CARTESIAN_POINT('Ctrl Pts',(0.359633402993741,2.26054589401105,4.98622758142271));
#30456=CARTESIAN_POINT('Ctrl Pts',(0.350701489094281,2.27921372499669,4.98726935725319));
#30457=CARTESIAN_POINT('Ctrl Pts',(0.34038302623639,2.29703879173949,4.98831113308368));
#30458=CARTESIAN_POINT('Ctrl Pts',(0.330042259786875,2.31490238776855,4.98935516073626));
#30459=CARTESIAN_POINT('Ctrl Pts',(0.318309378958636,2.33191897638875,4.99039918838884));
#30460=CARTESIAN_POINT('Ctrl Pts',(0.305356616403787,2.34787542600756,4.99144321604143));
#30461=CARTESIAN_POINT('Ctrl Pts',(0.300775394068722,2.3535190130858,4.99181247493737));
#30462=CARTESIAN_POINT('Ctrl Pts',(0.296041925583385,2.35903030243214,4.99218173383332));
#30463=CARTESIAN_POINT('Ctrl Pts',(0.291164924766646,2.36440097689992,4.99255099272926));
#30464=CARTESIAN_POINT('Ctrl Pts',(0.277376748663788,2.37958485898965,4.99359495537683));
#30465=CARTESIAN_POINT('Ctrl Pts',(0.262356561740721,2.39373252464626,4.9946389180244));
#30466=CARTESIAN_POINT('Ctrl Pts',(0.246285898424623,2.40664009235124,4.99568288067196));
#30467=CARTESIAN_POINT('Ctrl Pts',(0.230244798825399,2.41952391519456,4.99672492283775));
#30468=CARTESIAN_POINT('Ctrl Pts',(0.213157588635871,2.43117166645398,4.99776696500354));
#30469=CARTESIAN_POINT('Ctrl Pts',(0.195241819683713,2.44141693257159,4.99880900716932));
#30470=CARTESIAN_POINT('Ctrl Pts',(0.177345291985949,2.45165119543434,4.99984993019819));
#30471=CARTESIAN_POINT('Ctrl Pts',(0.15862259322943,2.46048557490693,5.00089085322706));
#30472=CARTESIAN_POINT('Ctrl Pts',(0.13931918695498,2.46779757224077,5.00193177625593));
#30473=CARTESIAN_POINT('Ctrl Pts',(0.120005866954183,2.47511332482586,5.00297323387574));
#30474=CARTESIAN_POINT('Ctrl Pts',(0.100111925984529,2.48090485758819,5.00401469149554));
#30475=CARTESIAN_POINT('Ctrl Pts',(0.0799021489945708,2.48509808696753,
5.00505614911535));
#30476=CARTESIAN_POINT('Ctrl Pts',(0.0596861970366758,2.48929259756125,
5.00609792494586));
#30477=CARTESIAN_POINT('Ctrl Pts',(0.0391549441241704,2.49188771865266,
5.00713970077638));
#30478=CARTESIAN_POINT('Ctrl Pts',(0.0185817384717031,2.49286080104201,
5.00818147660689));
#30479=CARTESIAN_POINT('Ctrl Pts',(-0.00203593663165084,2.49383598677102,
5.0092255042595));
#30480=CARTESIAN_POINT('Ctrl Pts',(-0.0226950094075678,2.4931821573905,
5.01026953191211));
#30481=CARTESIAN_POINT('Ctrl Pts',(-0.0431230423504149,2.490928757216,5.01131355956473));
#30482=CARTESIAN_POINT('Ctrl Pts',(-0.050348169834772,2.4901317591115,5.0116828184605));
#30483=CARTESIAN_POINT('Ctrl Pts',(-0.0575444726095197,2.48913513456542,
5.01205207735628));
#30484=CARTESIAN_POINT('Ctrl Pts',(-0.0647002405212437,2.48794170809091,
5.01242133625205));
#30485=CARTESIAN_POINT('Ctrl Pts',(-0.0849309093009322,2.48456767248543,
5.0134652988996));
#30486=CARTESIAN_POINT('Ctrl Pts',(-0.104957218468869,2.47959681744548,
5.01450926154715));
#30487=CARTESIAN_POINT('Ctrl Pts',(-0.124509472928379,2.47307141561784,
5.01555322419469));
#30488=CARTESIAN_POINT('Ctrl Pts',(-0.144025758908919,2.46655801797001,
5.01659526636046));
#30489=CARTESIAN_POINT('Ctrl Pts',(-0.163069012335207,2.45849592392518,
5.01763730852622));
#30490=CARTESIAN_POINT('Ctrl Pts',(-0.181381544972989,2.44897797228939,
5.01867935069199));
#30491=CARTESIAN_POINT('Ctrl Pts',(-0.199674410238418,2.43947024278411,
5.01972027372083));
#30492=CARTESIAN_POINT('Ctrl Pts',(-0.217237449807466,2.42851007168722,
5.02076119674968));
#30493=CARTESIAN_POINT('Ctrl Pts',(-0.233834790689169,2.41623753835266,
5.02180211977853));
#30494=CARTESIAN_POINT('Ctrl Pts',(-0.25044065553257,2.40395870216485,5.02284357739832));
#30495=CARTESIAN_POINT('Ctrl Pts',(-0.266079229680419,2.39036658173983,
5.02388503501811));
#30496=CARTESIAN_POINT('Ctrl Pts',(-0.280544889471852,2.37564371023338,
5.02492649263789));
#30497=CARTESIAN_POINT('Ctrl Pts',(-0.295014969153004,2.36091634024783,
5.02596826846839));
#30498=CARTESIAN_POINT('Ctrl Pts',(-0.308310931608444,2.34505808113766,
5.02701004429888));
#30499=CARTESIAN_POINT('Ctrl Pts',(-0.320265764657819,2.3282865085548,5.02805182012937));
#30500=CARTESIAN_POINT('Ctrl Pts',(-0.332246438350117,2.31147868383721,
5.02909584778196));
#30501=CARTESIAN_POINT('Ctrl Pts',(-0.342879816280033,2.29375423590212,
5.03013987543456));
#30502=CARTESIAN_POINT('Ctrl Pts',(-0.35204318041083,2.27535817382212,5.03118390308715));
#30503=CARTESIAN_POINT('Ctrl Pts',(-0.355284142193057,2.2688517277949,5.03155316198304));
#30504=CARTESIAN_POINT('Ctrl Pts',(-0.358341651152754,2.2622614566997,5.03192242087894));
#30505=CARTESIAN_POINT('Ctrl Pts',(-0.361211743273508,2.2555987356032,5.03229167977484));
#30506=CARTESIAN_POINT('Ctrl Pts',(-0.37018587552907,2.23476590592863,5.03344626925451));
#30507=CARTESIAN_POINT('Ctrl Pts',(-0.377369900235882,2.21311751646781,
5.03460085873419));
#30508=CARTESIAN_POINT('Ctrl Pts',(-0.38263725037188,2.19095946695011,5.03575544821386));
#30509=CARTESIAN_POINT('Ctrl Pts',(-0.38786747216244,2.16895760445159,5.03690189925658));
#30510=CARTESIAN_POINT('Ctrl Pts',(-0.391207731046514,2.14645366367599,
5.03804835029929));
#30511=CARTESIAN_POINT('Ctrl Pts',(-0.392581187677273,2.12376764779909,
5.039194801342));
#30512=CARTESIAN_POINT('Ctrl Pts',(-0.393055934862718,2.11592602983656,
5.03959108207893));
#30513=CARTESIAN_POINT('Ctrl Pts',(-0.393296118158558,2.10806280903969,
5.03998736281586));
#30514=CARTESIAN_POINT('Ctrl Pts',(-0.393299953314656,2.10019163165046,
5.04038364355279));
#30515=CARTESIAN_POINT('',(-0.39324855931036,2.09966296070036,5.1653836507501));
#30516=CARTESIAN_POINT('Ctrl Pts',(-0.392743434489697,2.10019127631944,
5.04038364779653));
#30517=CARTESIAN_POINT('Ctrl Pts',(-0.392401791420311,2.02231826806415,
5.04430977296356));
#30518=CARTESIAN_POINT('Ctrl Pts',(-0.332252156026397,1.8125855117155,5.05485934597154));
#30519=CARTESIAN_POINT('Ctrl Pts',(0.00931989327823174,1.63503959300418,
5.07203236682041));
#30520=CARTESIAN_POINT('Ctrl Pts',(0.395992061663179,1.85614486352699,5.09190271034321));
#30521=CARTESIAN_POINT('Ctrl Pts',(0.419395422923265,2.30095402388483,5.111773053866));
#30522=CARTESIAN_POINT('Ctrl Pts',(0.0580605791824544,2.56141522474824,
5.13164339738879));
#30523=CARTESIAN_POINT('Ctrl Pts',(-0.314803622727929,2.41498065574447,
5.14951359536563));
#30524=CARTESIAN_POINT('Ctrl Pts',(-0.392294629728231,2.19119159158929,
5.16076034550154));
#30525=CARTESIAN_POINT('Ctrl Pts',(-0.393038228349958,2.09966319944716,
5.16538364779653));
#30526=CARTESIAN_POINT('',(-0.393299999049727,2.09997265983606,5.29038364779291));
#30527=CARTESIAN_POINT('Ctrl Pts',(-0.393299855536788,2.09966290247398,
5.16538365147043));
#30528=CARTESIAN_POINT('Ctrl Pts',(-0.393278448914784,2.0746872776426,5.16664439623088));
#30529=CARTESIAN_POINT('Ctrl Pts',(-0.390874000548172,2.04981650347134,
5.16790514099134));
#30530=CARTESIAN_POINT('Ctrl Pts',(-0.386169426696434,2.02544757626376,
5.16916588575179));
#30531=CARTESIAN_POINT('Ctrl Pts',(-0.383410295784998,2.01115572700049,
5.16990528531265));
#30532=CARTESIAN_POINT('Ctrl Pts',(-0.379860949704092,1.99703607904903,
5.17064468487351));
#30533=CARTESIAN_POINT('Ctrl Pts',(-0.375545661273262,1.98316530353175,
5.17138408443437));
#30534=CARTESIAN_POINT('Ctrl Pts',(-0.369452879814242,1.9635810728949,5.17242804708192));
#30535=CARTESIAN_POINT('Ctrl Pts',(-0.361805880791454,1.94441636927946,
5.17347200972948));
#30536=CARTESIAN_POINT('Ctrl Pts',(-0.35268320558326,1.92593263804057,5.17451597237703));
#30537=CARTESIAN_POINT('Ctrl Pts',(-0.343577312519135,1.90748290961703,
5.1755580145428));
#30538=CARTESIAN_POINT('Ctrl Pts',(-0.33300140040825,1.88971234562842,5.17660005670857));
#30539=CARTESIAN_POINT('Ctrl Pts',(-0.321082475259915,1.87286362228616,
5.17764209887434));
#30540=CARTESIAN_POINT('Ctrl Pts',(-0.309176350849944,1.85603299420807,
5.17868302190319));
#30541=CARTESIAN_POINT('Ctrl Pts',(-0.295930476018805,1.84012285563736,
5.17972394493204));
#30542=CARTESIAN_POINT('Ctrl Pts',(-0.281515693358266,1.82534784837359,
5.1807648679609));
#30543=CARTESIAN_POINT('Ctrl Pts',(-0.267093507641053,1.81056525305118,
5.18180632558069));
#30544=CARTESIAN_POINT('Ctrl Pts',(-0.251501717063482,1.79691949159882,
5.18284778320048));
#30545=CARTESIAN_POINT('Ctrl Pts',(-0.234949111994465,1.78458946629351,
5.18388924082027));
#30546=CARTESIAN_POINT('Ctrl Pts',(-0.218391449382962,1.77225567362793,
5.18493101665077));
#30547=CARTESIAN_POINT('Ctrl Pts',(-0.20087299903073,1.76123882757827,5.18597279248126));
#30548=CARTESIAN_POINT('Ctrl Pts',(-0.182632019859586,1.75167481382764,
5.18701456831176));
#30549=CARTESIAN_POINT('Ctrl Pts',(-0.164351612398027,1.74209012724426,
5.18805859596436));
#30550=CARTESIAN_POINT('Ctrl Pts',(-0.145346235321096,1.73396483198983,
5.18910262361695));
#30551=CARTESIAN_POINT('Ctrl Pts',(-0.125875305182518,1.72738720158158,
5.19014665126955));
#30552=CARTESIAN_POINT('Ctrl Pts',(-0.118988692412658,1.72506077992414,
5.19051591016542));
#30553=CARTESIAN_POINT('Ctrl Pts',(-0.112043970402749,1.72292750302154,
5.19088516906128));
#30554=CARTESIAN_POINT('Ctrl Pts',(-0.105052947482939,1.72098975182042,
5.19125442795715));
#30555=CARTESIAN_POINT('Ctrl Pts',(-0.0852880430265416,1.71551137365034,
5.1922983906047));
#30556=CARTESIAN_POINT('Ctrl Pts',(-0.0650345583509261,1.71156690699225,
5.19334235325226));
#30557=CARTESIAN_POINT('Ctrl Pts',(-0.0445548372589666,1.70923183794374,
5.19438631589981));
#30558=CARTESIAN_POINT('Ctrl Pts',(-0.0241127908207696,1.70690106450636,
5.19542835806558));
#30559=CARTESIAN_POINT('Ctrl Pts',(-0.00344605012792134,1.70617395338364,
5.19647040023135));
#30560=CARTESIAN_POINT('Ctrl Pts',(0.0171725876683758,1.70707508066709,
5.19751244239712));
#30561=CARTESIAN_POINT('Ctrl Pts',(0.0377690813715958,1.707975240154,5.19855336542598));
#30562=CARTESIAN_POINT('Ctrl Pts',(0.0583168421269406,1.71050016338497,
5.19959428845483));
#30563=CARTESIAN_POINT('Ctrl Pts',(0.0785429150844682,1.71462239233444,
5.20063521148369));
#30564=CARTESIAN_POINT('Ctrl Pts',(0.098779375625906,1.71874673835325,5.20167666910348));
#30565=CARTESIAN_POINT('Ctrl Pts',(0.11869309413943,1.72446989779485,5.20271812672327));
#30566=CARTESIAN_POINT('Ctrl Pts',(0.138020624388094,1.7317131590139,5.20375958434306));
#30567=CARTESIAN_POINT('Ctrl Pts',(0.157354060039858,1.73895863336503,5.20480136017356));
#30568=CARTESIAN_POINT('Ctrl Pts',(0.176100275162223,1.74772484224979,5.20584313600406));
#30569=CARTESIAN_POINT('Ctrl Pts',(0.194016040780442,1.75788501067641,5.20688491183456));
#30570=CARTESIAN_POINT('Ctrl Pts',(0.211970531732606,1.76806714053764,5.20792893948716));
#30571=CARTESIAN_POINT('Ctrl Pts',(0.229090379478053,1.7796488327275,5.20897296713976));
#30572=CARTESIAN_POINT('Ctrl Pts',(0.245160935195129,1.79245974921281,5.21001699479235));
#30573=CARTESIAN_POINT('Ctrl Pts',(0.25084488010337,1.79699080245132,5.21038625368822));
#30574=CARTESIAN_POINT('Ctrl Pts',(0.256397881025208,1.80167526772497,5.21075551258409));
#30575=CARTESIAN_POINT('Ctrl Pts',(0.26181154395561,1.8065045052278,5.21112477147995));
#30576=CARTESIAN_POINT('Ctrl Pts',(0.277116962319406,1.8201576456817,5.2121687341275));
#30577=CARTESIAN_POINT('Ctrl Pts',(0.291397117720928,1.83505192714911,5.21321269677506));
#30578=CARTESIAN_POINT('Ctrl Pts',(0.304446528657043,1.85100762825204,5.21425665942261));
#30579=CARTESIAN_POINT('Ctrl Pts',(0.317471933795589,1.86693397712346,5.21529870158838));
#30580=CARTESIAN_POINT('Ctrl Pts',(0.329270582007397,1.88391734433447,5.21634074375415));
#30581=CARTESIAN_POINT('Ctrl Pts',(0.33967413924762,1.90174166063848,5.21738278591992));
#30582=CARTESIAN_POINT('Ctrl Pts',(0.350066523230802,1.91954683390678,5.21842370894877));
#30583=CARTESIAN_POINT('Ctrl Pts',(0.359066396742351,1.93819054561226,5.21946463197762));
#30584=CARTESIAN_POINT('Ctrl Pts',(0.366549091589525,1.95742842690461,5.22050555500647));
#30585=CARTESIAN_POINT('Ctrl Pts',(0.37403562935375,1.9766761882714,5.22154701262627));
#30586=CARTESIAN_POINT('Ctrl Pts',(0.380003150075041,1.9965180489571,5.22258847024606));
#30587=CARTESIAN_POINT('Ctrl Pts',(0.38437522770585,2.01668989061299,5.22362992786585));
#30588=CARTESIAN_POINT('Ctrl Pts',(0.388748641196982,2.03686789564592,5.22467170369634));
#30589=CARTESIAN_POINT('Ctrl Pts',(0.391525520781456,2.05737535622491,5.22571347952684));
#30590=CARTESIAN_POINT('Ctrl Pts',(0.392680796903289,2.07793913547937,5.22675525535734));
#30591=CARTESIAN_POINT('Ctrl Pts',(0.393838570180677,2.09854736380935,5.22779928300993));
#30592=CARTESIAN_POINT('Ctrl Pts',(0.393367758945009,2.11921141756431,5.22884331066253));
#30593=CARTESIAN_POINT('Ctrl Pts',(0.391295393178771,2.1396586091167,5.22988733831512));
#30594=CARTESIAN_POINT('Ctrl Pts',(0.39056242457131,2.14689051275205,5.23025659721099));
#30595=CARTESIAN_POINT('Ctrl Pts',(0.389629582032103,2.15409536104576,5.23062585610686));
#30596=CARTESIAN_POINT('Ctrl Pts',(0.38849958623811,2.16126141928504,5.23099511500273));
#30597=CARTESIAN_POINT('Ctrl Pts',(0.385304880805083,2.1815211807037,5.23203907765028));
#30598=CARTESIAN_POINT('Ctrl Pts',(0.380511608419225,2.2015907347236,5.23308304029783));
#30599=CARTESIAN_POINT('Ctrl Pts',(0.374159651182492,2.22120002238859,5.23412700294539));
#30600=CARTESIAN_POINT('Ctrl Pts',(0.367819379055558,2.24077323665591,5.23516904511116));
#30601=CARTESIAN_POINT('Ctrl Pts',(0.359926281292902,2.25988715486123,5.23621108727693));
#30602=CARTESIAN_POINT('Ctrl Pts',(0.35057091052557,2.27828327653842,5.2372531294427));
#30603=CARTESIAN_POINT('Ctrl Pts',(0.341225587279472,2.29665964106992,5.23829405247155));
#30604=CARTESIAN_POINT('Ctrl Pts',(0.330421414822523,2.31431907387229,5.23933497550041));
#30605=CARTESIAN_POINT('Ctrl Pts',(0.318296377713979,2.33102447042285,5.24037589852926));
#30606=CARTESIAN_POINT('Ctrl Pts',(0.306165113502394,2.34773844642969,5.24141735614905));
#30607=CARTESIAN_POINT('Ctrl Pts',(0.292712048574248,2.36349680240577,5.24245881376884));
#30608=CARTESIAN_POINT('Ctrl Pts',(0.27811788756555,2.3780923059275,5.24350027138864));
#30609=CARTESIAN_POINT('Ctrl Pts',(0.263519267404413,2.39269226901187,5.24454204721914));
#30610=CARTESIAN_POINT('Ctrl Pts',(0.24777940247025,2.40612817804252,5.24558382304964));
#30611=CARTESIAN_POINT('Ctrl Pts',(0.231114380530547,2.41823110016462,5.24662559888013));
#30612=CARTESIAN_POINT('Ctrl Pts',(0.214413336767746,2.43036018302753,5.24766962653273));
#30613=CARTESIAN_POINT('Ctrl Pts',(0.196783771764517,2.44115014218432,5.24871365418533));
#30614=CARTESIAN_POINT('Ctrl Pts',(0.178469597978355,2.45047609418824,5.24975768183793));
#30615=CARTESIAN_POINT('Ctrl Pts',(0.17199211476789,2.45377456116974,5.25012694073379));
#30616=CARTESIAN_POINT('Ctrl Pts',(0.165429184802336,2.45689032502551,5.25049619962966));
#30617=CARTESIAN_POINT('Ctrl Pts',(0.158792147589922,2.4598193211374,5.25086545852552));
#30618=CARTESIAN_POINT('Ctrl Pts',(0.140028025675,2.46810013053666,5.25190942117308));
#30619=CARTESIAN_POINT('Ctrl Pts',(0.120558500370676,2.47493387351884,5.25295338382063));
#30620=CARTESIAN_POINT('Ctrl Pts',(0.100632230984904,2.48020789587672,5.25399734646818));
#30621=CARTESIAN_POINT('Ctrl Pts',(0.0807426181188446,2.48547221610216,
5.25503938863395));
#30622=CARTESIAN_POINT('Ctrl Pts',(0.0603986170307354,2.48918226747339,
5.25608143079972));
#30623=CARTESIAN_POINT('Ctrl Pts',(0.0398665973161565,2.49127425729075,
5.25712347296549));
#30624=CARTESIAN_POINT('Ctrl Pts',(0.0193566286682032,2.49336400034392,
5.25816439599434));
#30625=CARTESIAN_POINT('Ctrl Pts',(-0.00134023238324855,2.49383902876169,
5.2592053190232));
#30626=CARTESIAN_POINT('Ctrl Pts',(-0.0219499305751598,2.49268701346969,
5.26024624205205));
#30627=CARTESIAN_POINT('Ctrl Pts',(-0.0425702133709115,2.49153440653266,
5.26128769967184));
#30628=CARTESIAN_POINT('Ctrl Pts',(-0.0631025083463235,2.48875311149752,
5.26232915729163));
#30629=CARTESIAN_POINT('Ctrl Pts',(-0.0832747520846534,2.48438288940227,
5.26337061491142));
#30630=CARTESIAN_POINT('Ctrl Pts',(-0.10345315932288,2.48001133201365,5.26441239074192));
#30631=CARTESIAN_POINT('Ctrl Pts',(-0.123270585487693,2.47405007209419,
5.26545416657242));
#30632=CARTESIAN_POINT('Ctrl Pts',(-0.142468016597115,2.46658935370096,
5.26649594240292));
#30633=CARTESIAN_POINT('Ctrl Pts',(-0.161706943389524,2.45911250879561,
5.26753997005552));
#30634=CARTESIAN_POINT('Ctrl Pts',(-0.180322536318393,2.45013005474816,
5.26858399770811));
#30635=CARTESIAN_POINT('Ctrl Pts',(-0.198077756925285,2.43977947585375,
5.26962802536071));
#30636=CARTESIAN_POINT('Ctrl Pts',(-0.204357545722892,2.43611861177163,
5.26999728425658));
#30637=CARTESIAN_POINT('Ctrl Pts',(-0.210529968333663,2.43228700202477,
5.27036654315244));
#30638=CARTESIAN_POINT('Ctrl Pts',(-0.216585468873167,2.42829198082346,
5.27073580204831));
#30639=CARTESIAN_POINT('Ctrl Pts',(-0.233671942193388,2.41701944889573,
5.27177771959605));
#30640=CARTESIAN_POINT('Ctrl Pts',(-0.249927900178604,2.40437512782881,
5.27281963714379));
#30641=CARTESIAN_POINT('Ctrl Pts',(-0.265124530554396,2.39050623624685,
5.27386155469154));
#30642=CARTESIAN_POINT('Ctrl Pts',(-0.280293205464843,2.37666285764431,
5.27490155554531));
#30643=CARTESIAN_POINT('Ctrl Pts',(-0.294405840299752,2.36159982764347,
5.27594155639907));
#30644=CARTESIAN_POINT('Ctrl Pts',(-0.307265055974466,2.34550575426455,
5.27698155725284));
#30645=CARTESIAN_POINT('Ctrl Pts',(-0.320110565501371,2.32942883494497,
5.27802044960934));
#30646=CARTESIAN_POINT('Ctrl Pts',(-0.331704826296372,2.31232361015645,
5.27905934196584));
#30647=CARTESIAN_POINT('Ctrl Pts',(-0.34188954617818,2.29441303509302,5.28009823432234));
#30648=CARTESIAN_POINT('Ctrl Pts',(-0.352079545237533,2.27649317620963,
5.28113766518135));
#30649=CARTESIAN_POINT('Ctrl Pts',(-0.360858165496563,2.25776776814142,
5.28217709604036));
#30650=CARTESIAN_POINT('Ctrl Pts',(-0.368111998054116,2.2384862696754,5.28321652689937));
#30651=CARTESIAN_POINT('Ctrl Pts',(-0.375368208515285,2.21919845047554,
5.28425629849776));
#30652=CARTESIAN_POINT('Ctrl Pts',(-0.381098411966207,2.19935488235279,
5.28529607009615));
#30653=CARTESIAN_POINT('Ctrl Pts',(-0.385238720190411,2.17922132582868,
5.28633584169454));
#30654=CARTESIAN_POINT('Ctrl Pts',(-0.389387870101292,2.15904477381032,
5.28737783373985));
#30655=CARTESIAN_POINT('Ctrl Pts',(-0.391940259039512,2.13857773128581,
5.28841982578517));
#30656=CARTESIAN_POINT('Ctrl Pts',(-0.392883617329559,2.11809290562736,
5.28946181783049));
#30657=CARTESIAN_POINT('Ctrl Pts',(-0.393161807532951,2.11205206422437,
5.28976909448463));
#30658=CARTESIAN_POINT('Ctrl Pts',(-0.393300418711213,2.10600967052975,
5.29007637113877));
#30659=CARTESIAN_POINT('Ctrl Pts',(-0.393299999049727,2.09997265983607,
5.29038364779291));
#30660=CARTESIAN_POINT('',(-0.393299842496665,2.10035198309414,5.41538364779399));
#30661=CARTESIAN_POINT('Ctrl Pts',(-0.393299999049722,2.09997265976493,
5.29038364779653));
#30662=CARTESIAN_POINT('Ctrl Pts',(-0.393299897757734,2.09851553480785,
5.29045781372138));
#30663=CARTESIAN_POINT('Ctrl Pts',(-0.393291698817535,2.09705844255106,
5.29053197964624));
#30664=CARTESIAN_POINT('Ctrl Pts',(-0.393275403094208,2.09560144102145,
5.2906061455711));
#30665=CARTESIAN_POINT('Ctrl Pts',(-0.3930460238139,2.07509262680193,5.29165010821865));
#30666=CARTESIAN_POINT('Ctrl Pts',(-0.391207378815338,2.05454069639888,
5.29269407086621));
#30667=CARTESIAN_POINT('Ctrl Pts',(-0.387759851386128,2.03421863749505,
5.29373803351376));
#30668=CARTESIAN_POINT('Ctrl Pts',(-0.384318666055116,2.01393396320839,
5.29478007567953));
#30669=CARTESIAN_POINT('Ctrl Pts',(-0.379274536245748,1.99387904820193,
5.2958221178453));
#30670=CARTESIAN_POINT('Ctrl Pts',(-0.372679655033211,1.97432277563406,
5.29686416001107));
#30671=CARTESIAN_POINT('Ctrl Pts',(-0.366091856619499,1.95478750619573,
5.29790508303992));
#30672=CARTESIAN_POINT('Ctrl Pts',(-0.357956819701436,1.93575051894137,
5.29894600606878));
#30673=CARTESIAN_POINT('Ctrl Pts',(-0.348376766162668,1.91746638994957,
5.29998692909763));
#30674=CARTESIAN_POINT('Ctrl Pts',(-0.338791792558084,1.89917287070565,
5.30102838671742));
#30675=CARTESIAN_POINT('Ctrl Pts',(-0.327760646938449,1.8816336413797,5.30206984433721));
#30676=CARTESIAN_POINT('Ctrl Pts',(-0.31543214428506,1.86507990219709,5.30311130195701));
#30677=CARTESIAN_POINT('Ctrl Pts',(-0.303099874736633,1.84852110512548,
5.3041530777875));
#30678=CARTESIAN_POINT('Ctrl Pts',(-0.289469927148838,1.8329489656328,5.305194853618));
#30679=CARTESIAN_POINT('Ctrl Pts',(-0.27473166938063,1.81856190762562,5.3062366294485));
#30680=CARTESIAN_POINT('Ctrl Pts',(-0.259961554533801,1.80414375166606,
5.3072806571011));
#30681=CARTESIAN_POINT('Ctrl Pts',(-0.24407891265205,1.79091626257462,5.3083246847537));
#30682=CARTESIAN_POINT('Ctrl Pts',(-0.227307017618983,1.77903830486931,
5.30936871240629));
#30683=CARTESIAN_POINT('Ctrl Pts',(-0.221375018187665,1.7748372269223,5.30973797130216));
#30684=CARTESIAN_POINT('Ctrl Pts',(-0.215332033182601,1.77080456448087,
5.31010723019802));
#30685=CARTESIAN_POINT('Ctrl Pts',(-0.209188694587853,1.76694598027252,
5.31047648909389));
#30686=CARTESIAN_POINT('Ctrl Pts',(-0.191820349245343,1.75603705477052,
5.31152045174144));
#30687=CARTESIAN_POINT('Ctrl Pts',(-0.173544626432881,1.74645788912813,
5.312564414389));
#30688=CARTESIAN_POINT('Ctrl Pts',(-0.154591266562296,1.73835593423552,
5.31360837703655));
#30689=CARTESIAN_POINT('Ctrl Pts',(-0.135672773439533,1.73026888376197,
5.31465041920232));
#30690=CARTESIAN_POINT('Ctrl Pts',(-0.116079763223746,1.7236539905554,5.31569246136809));
#30691=CARTESIAN_POINT('Ctrl Pts',(-0.0960665707433878,1.71861292105578,
5.31673450353386));
#30692=CARTESIAN_POINT('Ctrl Pts',(-0.0760748721173508,1.71357726558561,
5.31777542656271));
#30693=CARTESIAN_POINT('Ctrl Pts',(-0.0556645899138119,1.71011228510182,
5.31881634959157));
#30694=CARTESIAN_POINT('Ctrl Pts',(-0.0351051108103078,1.70826983624567,
5.31985727262042));
#30695=CARTESIAN_POINT('Ctrl Pts',(-0.0145350728941838,1.7064264411558,
5.32089873024021));
#30696=CARTESIAN_POINT('Ctrl Pts',(0.00618358359623564,1.70620732415075,
5.32194018786001));
#30697=CARTESIAN_POINT('Ctrl Pts',(0.0267759051336634,1.70761251178934,
5.3229816454798));
#30698=CARTESIAN_POINT('Ctrl Pts',(0.047374518523068,1.709018128774,5.3240234213103));
#30699=CARTESIAN_POINT('Ctrl Pts',(0.0678459891248714,1.71204895226355,
5.32506519714079));
#30700=CARTESIAN_POINT('Ctrl Pts',(0.0879209703220723,1.71665316881755,
5.32610697297129));
#30701=CARTESIAN_POINT('Ctrl Pts',(0.108039344046691,1.72126733749012,5.32715100062389));
#30702=CARTESIAN_POINT('Ctrl Pts',(0.127758814736537,1.72746146830245,5.32819502827648));
#30703=CARTESIAN_POINT('Ctrl Pts',(0.146824944072981,1.73513382480974,5.32923905592908));
#30704=CARTESIAN_POINT('Ctrl Pts',(0.153568384105152,1.73784743673901,5.32960831482495));
#30705=CARTESIAN_POINT('Ctrl Pts',(0.160230295861298,1.74074553368207,5.32997757372081));
#30706=CARTESIAN_POINT('Ctrl Pts',(0.166800162733676,1.74382224141306,5.33034683261668));
#30707=CARTESIAN_POINT('Ctrl Pts',(0.185374381773336,1.75252065866055,5.33139079526423));
#30708=CARTESIAN_POINT('Ctrl Pts',(0.203321694734255,1.76270183817006,5.33243475791179));
#30709=CARTESIAN_POINT('Ctrl Pts',(0.220393759631902,1.77425242792107,5.33347872055934));
#30710=CARTESIAN_POINT('Ctrl Pts',(0.237434418626551,1.78578176911759,5.33452076272511));
#30711=CARTESIAN_POINT('Ctrl Pts',(0.253602389723254,1.79867516169156,5.33556280489088));
#30712=CARTESIAN_POINT('Ctrl Pts',(0.268674513920839,1.81277379024643,5.33660484705665));
#30713=CARTESIAN_POINT('Ctrl Pts',(0.283730450893813,1.82685727709572,5.3376457700855));
#30714=CARTESIAN_POINT('Ctrl Pts',(0.297692323070091,1.84214295126189,5.33868669311436));
#30715=CARTESIAN_POINT('Ctrl Pts',(0.310370704581198,1.85843237854015,5.33972761614321));
#30716=CARTESIAN_POINT('Ctrl Pts',(0.323055597378609,1.8747301716437,5.340769073763));
#30717=CARTESIAN_POINT('Ctrl Pts',(0.334455218000237,1.8920321769816,5.34181053138279));
#30718=CARTESIAN_POINT('Ctrl Pts',(0.344420706802546,1.91010722308199,5.34285198900258));
#30719=CARTESIAN_POINT('Ctrl Pts',(0.354389240496144,1.92818779189697,5.34389376483308));
#30720=CARTESIAN_POINT('Ctrl Pts',(0.362922446773869,1.94704121042643,5.34493554066358));
#30721=CARTESIAN_POINT('Ctrl Pts',(0.36991808911354,1.9664129596608,5.34597731649408));
#30722=CARTESIAN_POINT('Ctrl Pts',(0.37692885269288,1.98582658137074,5.34702134414668));
#30723=CARTESIAN_POINT('Ctrl Pts',(0.382395222396415,2.0057600603213,5.34806537179927));
#30724=CARTESIAN_POINT('Ctrl Pts',(0.386265007989182,2.02594438844276,5.34910939945187));
#30725=CARTESIAN_POINT('Ctrl Pts',(0.387633700429152,2.03308332072814,5.34947865834774));
#30726=CARTESIAN_POINT('Ctrl Pts',(0.388803141837507,2.04025356765072,5.3498479172436));
#30727=CARTESIAN_POINT('Ctrl Pts',(0.389772578538716,2.04744310683383,5.35021717613947));
#30728=CARTESIAN_POINT('Ctrl Pts',(0.39251335395823,2.06776925318883,5.35126113878702));
#30729=CARTESIAN_POINT('Ctrl Pts',(0.393668040731998,2.0883709316927,5.35230510143458));
#30730=CARTESIAN_POINT('Ctrl Pts',(0.393197515264884,2.10897797246158,5.35334906408213));
#30731=CARTESIAN_POINT('Ctrl Pts',(0.39272785538007,2.12954710435845,5.3543911062479));
#30732=CARTESIAN_POINT('Ctrl Pts',(0.390638874946974,2.15012085030323,5.35543314841367));
#30733=CARTESIAN_POINT('Ctrl Pts',(0.386943308794926,2.17042560456847,5.35647519057944));
#30734=CARTESIAN_POINT('Ctrl Pts',(0.38325171162287,2.19070855184661,5.35751611360829));
#30735=CARTESIAN_POINT('Ctrl Pts',(0.377957056787415,2.2107223555719,5.35855703663715));
#30736=CARTESIAN_POINT('Ctrl Pts',(0.371123651675472,2.23020032706204,5.359597959666));
#30737=CARTESIAN_POINT('Ctrl Pts',(0.364286737104763,2.24968830193069,5.36063941728579));
#30738=CARTESIAN_POINT('Ctrl Pts',(0.355909721855467,2.26863919516935,5.36168087490559));
#30739=CARTESIAN_POINT('Ctrl Pts',(0.346106398625333,2.28680270562977,5.36272233252538));
#30740=CARTESIAN_POINT('Ctrl Pts',(0.336300080052563,2.3049717658345,5.36376410835588));
#30741=CARTESIAN_POINT('Ctrl Pts',(0.325066966937527,2.32235233456427,5.36480588418637));
#30742=CARTESIAN_POINT('Ctrl Pts',(0.312565720943722,2.338720673782,5.36584766001687));
#30743=CARTESIAN_POINT('Ctrl Pts',(0.300037453223013,2.35512439353639,5.36689168766947));
#30744=CARTESIAN_POINT('Ctrl Pts',(0.286236071916274,2.37051096738615,5.36793571532207));
#30745=CARTESIAN_POINT('Ctrl Pts',(0.271359512307732,2.38469089391849,5.36897974297466));
#30746=CARTESIAN_POINT('Ctrl Pts',(0.266097868172478,2.38970614806599,5.36934900187053));
#30747=CARTESIAN_POINT('Ctrl Pts',(0.260702035945947,2.39457081955757,5.36971826076639));
#30748=CARTESIAN_POINT('Ctrl Pts',(0.255181716279521,2.39927776675964,5.37008751966226));
#30749=CARTESIAN_POINT('Ctrl Pts',(0.239574759754362,2.41258517009638,5.37113148230981));
#30750=CARTESIAN_POINT('Ctrl Pts',(0.222877552422454,2.42470811223257,5.37217544495737));
#30751=CARTESIAN_POINT('Ctrl Pts',(0.205296079650398,2.43546744950915,5.37321940760492));
#30752=CARTESIAN_POINT('Ctrl Pts',(0.187746949892017,2.44620699382543,5.37426144977069));
#30753=CARTESIAN_POINT('Ctrl Pts',(0.169317373087481,2.45558748209929,5.37530349193646));
#30754=CARTESIAN_POINT('Ctrl Pts',(0.150244295424405,2.46347151427921,5.37634553410223));
#30755=CARTESIAN_POINT('Ctrl Pts',(0.131191701947108,2.47134707913243,5.37738645713108));
#30756=CARTESIAN_POINT('Ctrl Pts',(0.111497645109286,2.47772907213223,5.37842738015994));
#30757=CARTESIAN_POINT('Ctrl Pts',(0.091421172280401,2.48252720067843,5.37946830318879));
#30758=CARTESIAN_POINT('Ctrl Pts',(0.0713343886983286,2.4873277934184,5.38050976080858));
#30759=CARTESIAN_POINT('Ctrl Pts',(0.0508655086416936,2.49054270994249,
5.38155121842837));
#30760=CARTESIAN_POINT('Ctrl Pts',(0.0302865878408223,2.49213213665416,
5.38259267604817));
#30761=CARTESIAN_POINT('Ctrl Pts',(0.00970137928248253,2.49372204900499,
5.38363445187866));
#30762=CARTESIAN_POINT('Ctrl Pts',(-0.0109932011925229,2.49368546227628,
5.38467622770916));
#30763=CARTESIAN_POINT('Ctrl Pts',(-0.0315231442114445,2.49203466859326,
5.38571800353966));
#30764=CARTESIAN_POINT('Ctrl Pts',(-0.0520974631680873,2.49038030668223,
5.38676203119226));
#30765=CARTESIAN_POINT('Ctrl Pts',(-0.0725057070245646,2.48710488861692,
5.38780605884485));
#30766=CARTESIAN_POINT('Ctrl Pts',(-0.0924813936542848,2.48227226138939,
5.38885008649745));
#30767=CARTESIAN_POINT('Ctrl Pts',(-0.099546532178845,2.4805630244839,5.38921934539332));
#30768=CARTESIAN_POINT('Ctrl Pts',(-0.106557696548657,2.47865944671621,
5.38958860428918));
#30769=CARTESIAN_POINT('Ctrl Pts',(-0.113503630812447,2.47656581867237,
5.38995786318505));
#30770=CARTESIAN_POINT('Ctrl Pts',(-0.133141061365718,2.47064674806877,
5.3910018258326));
#30771=CARTESIAN_POINT('Ctrl Pts',(-0.152372748195794,2.46316980481688,
5.39204578848016));
#30772=CARTESIAN_POINT('Ctrl Pts',(-0.170936560505818,2.45421121140139,
5.39308975112771));
#30773=CARTESIAN_POINT('Ctrl Pts',(-0.189466222682733,2.44526909828384,
5.39413179329348));
#30774=CARTESIAN_POINT('Ctrl Pts',(-0.20732976810087,2.43485100793367,5.39517383545925));
#30775=CARTESIAN_POINT('Ctrl Pts',(-0.224283405084158,2.42308179181727,
5.39621587762502));
#30776=CARTESIAN_POINT('Ctrl Pts',(-0.241218834127655,2.41132521565409,
5.39725680065387));
#30777=CARTESIAN_POINT('Ctrl Pts',(-0.257245676922874,2.39822078818098,
5.39829772368273));
#30778=CARTESIAN_POINT('Ctrl Pts',(-0.272147786813168,2.38393744404832,
5.39933864671158));
#30779=CARTESIAN_POINT('Ctrl Pts',(-0.287057550038711,2.36964676436238,
5.40038010433137));
#30780=CARTESIAN_POINT('Ctrl Pts',(-0.300840884037119,2.35417645593242,
5.40142156195116));
#30781=CARTESIAN_POINT('Ctrl Pts',(-0.31331704414102,2.3377337162683,5.40246301957095));
#30782=CARTESIAN_POINT('Ctrl Pts',(-0.325797016255748,2.32128595263036,
5.40350479540145));
#30783=CARTESIAN_POINT('Ctrl Pts',(-0.336968603817644,2.30386577378592,
5.40454657123195));
#30784=CARTESIAN_POINT('Ctrl Pts',(-0.346693816041194,2.28571022567106,
5.40558834706245));
#30785=CARTESIAN_POINT('Ctrl Pts',(-0.356440049531657,2.26751543392694,
5.40663237471505));
#30786=CARTESIAN_POINT('Ctrl Pts',(-0.364733370531078,2.24858277411358,
5.40767640236764));
#30787=CARTESIAN_POINT('Ctrl Pts',(-0.371483211143384,2.22917087070466,
5.40872043002024));
#30788=CARTESIAN_POINT('Ctrl Pts',(-0.373870541292716,2.22230513491535,
5.40908968891611));
#30789=CARTESIAN_POINT('Ctrl Pts',(-0.376065248980338,2.2153795813415,5.40945894781197));
#30790=CARTESIAN_POINT('Ctrl Pts',(-0.378064848758017,2.20840599676022,
5.40982820670784));
#30791=CARTESIAN_POINT('Ctrl Pts',(-0.385082654093672,2.18393146959264,
5.4111241595673));
#30792=CARTESIAN_POINT('Ctrl Pts',(-0.389727460306299,2.15874785035819,
5.41242011242676));
#30793=CARTESIAN_POINT('Ctrl Pts',(-0.391890476555899,2.13326776795625,
5.41371606528622));
#30794=CARTESIAN_POINT('Ctrl Pts',(-0.392818238713173,2.12233883655264,
5.41427192612214));
#30795=CARTESIAN_POINT('Ctrl Pts',(-0.393289994800293,2.11135562928169,
5.41482778695806));
#30796=CARTESIAN_POINT('Ctrl Pts',(-0.393299842496665,2.10035198309414,
5.41538364779398));
#30797=CARTESIAN_POINT('',(-0.393082160614917,2.09985082257753,5.54038368632201));
#30798=CARTESIAN_POINT('Ctrl Pts',(-0.39329984249671,2.10035198304379,5.41538364779653));
#30799=CARTESIAN_POINT('Ctrl Pts',(-0.39331813262776,2.07991490293939,5.41641604853325));
#30800=CARTESIAN_POINT('Ctrl Pts',(-0.391739146712473,2.05944415779562,
5.41744844926996));
#30801=CARTESIAN_POINT('Ctrl Pts',(-0.38857361574904,2.03920990916509,5.41848085000668));
#30802=CARTESIAN_POINT('Ctrl Pts',(-0.385407316009461,2.01897074647499,
5.41951350147071));
#30803=CARTESIAN_POINT('Ctrl Pts',(-0.380653784186541,1.99896894018719,
5.42054615293473));
#30804=CARTESIAN_POINT('Ctrl Pts',(-0.374375506108631,1.97946838412306,
5.42157880439876));
#30805=CARTESIAN_POINT('Ctrl Pts',(-0.368096782342726,1.95996644373609,
5.42261152916957));
#30806=CARTESIAN_POINT('Ctrl Pts',(-0.36029335144596,1.94096653004302,5.42364425394037));
#30807=CARTESIAN_POINT('Ctrl Pts',(-0.351076903972026,1.92271520793532,
5.42467697871118));
#30808=CARTESIAN_POINT('Ctrl Pts',(-0.341839789496302,1.90442295898376,
5.4257120192685));
#30809=CARTESIAN_POINT('Ctrl Pts',(-0.331183711860069,1.88688330180213,
5.42674705982581));
#30810=CARTESIAN_POINT('Ctrl Pts',(-0.319265627307391,1.87031685037857,
5.42778210038312));
#30811=CARTESIAN_POINT('Ctrl Pts',(-0.311909905459202,1.86009220327655,
5.42842091699896));
#30812=CARTESIAN_POINT('Ctrl Pts',(-0.304074315194476,1.85023768421479,
5.4290597336148));
#30813=CARTESIAN_POINT('Ctrl Pts',(-0.295803036849655,1.84079843096439,
5.42969855023063));
#30814=CARTESIAN_POINT('Ctrl Pts',(-0.282286003282509,1.82537267720357,
5.43074251287818));
#30815=CARTESIAN_POINT('Ctrl Pts',(-0.267518795889601,1.81096115249115,
5.43178647552574));
#30816=CARTESIAN_POINT('Ctrl Pts',(-0.251679308898635,1.79777092219261,
5.43283043817329));
#30817=CARTESIAN_POINT('Ctrl Pts',(-0.235868960350793,1.78460495674403,
5.43387248033906));
#30818=CARTESIAN_POINT('Ctrl Pts',(-0.218990768648704,1.7726563373126,5.43491452250483));
#30819=CARTESIAN_POINT('Ctrl Pts',(-0.2012593035049,1.76209530522243,5.4359565646706));
#30820=CARTESIAN_POINT('Ctrl Pts',(-0.183546881676084,1.75154561551481,
5.43699748769945));
#30821=CARTESIAN_POINT('Ctrl Pts',(-0.164983619824173,1.74238095410268,
5.43803841072831));
#30822=CARTESIAN_POINT('Ctrl Pts',(-0.145812772935528,1.73472814884137,
5.43907933375716));
#30823=CARTESIAN_POINT('Ctrl Pts',(-0.126632080399596,1.72707141329874,
5.44012079137695));
#30824=CARTESIAN_POINT('Ctrl Pts',(-0.106843856808282,1.72092837283578,
5.44116224899674));
#30825=CARTESIAN_POINT('Ctrl Pts',(-0.086711533187502,1.71637778999089,
5.44220370661654));
#30826=CARTESIAN_POINT('Ctrl Pts',(-0.0665730582641609,1.71182581674456,
5.44324548244703));
#30827=CARTESIAN_POINT('Ctrl Pts',(-0.0460909990527346,1.70886739654375,
5.44428725827753));
#30828=CARTESIAN_POINT('Ctrl Pts',(-0.0255382596491352,1.70753001733369,
5.44532903410803));
#30829=CARTESIAN_POINT('Ctrl Pts',(-0.00494109503290615,1.70618974734812,
5.44637306176062));
#30830=CARTESIAN_POINT('Ctrl Pts',(0.0157263183806198,1.70647750349892,
5.44741708941322));
#30831=CARTESIAN_POINT('Ctrl Pts',(0.036191064237229,1.70836867225747,5.44846111706582));
#30832=CARTESIAN_POINT('Ctrl Pts',(0.0434291765998863,1.7090375538584,5.44883037596169));
#30833=CARTESIAN_POINT('Ctrl Pts',(0.0506420051116785,1.70990654119884,
5.44919963485755));
#30834=CARTESIAN_POINT('Ctrl Pts',(0.0578177914211348,1.7109730176515,5.44956889375342));
#30835=CARTESIAN_POINT('Ctrl Pts',(0.0781050558790529,1.7139881422525,5.45061285640097));
#30836=CARTESIAN_POINT('Ctrl Pts',(0.0982162800750279,1.71860345589965,
5.45165681904853));
#30837=CARTESIAN_POINT('Ctrl Pts',(0.117881062382578,1.72478147016498,5.45270078169608));
#30838=CARTESIAN_POINT('Ctrl Pts',(0.137509669204067,1.73094811930735,5.45374282386185));
#30839=CARTESIAN_POINT('Ctrl Pts',(0.156692752492609,1.738671601488,5.45478486602762));
#30840=CARTESIAN_POINT('Ctrl Pts',(0.175171019832387,1.74786365735573,5.45582690819339));
#30841=CARTESIAN_POINT('Ctrl Pts',(0.193629441803336,1.75704584109987,5.45686783122224));
#30842=CARTESIAN_POINT('Ctrl Pts',(0.211383882263559,1.76769316721141,5.4579087542511));
#30843=CARTESIAN_POINT('Ctrl Pts',(0.228196023762074,1.77966975675222,5.45894967727995));
#30844=CARTESIAN_POINT('Ctrl Pts',(0.245016799538276,1.79165249715727,5.45999113489974));
#30845=CARTESIAN_POINT('Ctrl Pts',(0.260893700927387,1.80496545104851,5.46103259251953));
#30846=CARTESIAN_POINT('Ctrl Pts',(0.275617903002686,1.81942975648797,5.46207405013933));
#30847=CARTESIAN_POINT('Ctrl Pts',(0.290346603963644,1.83389848140333,5.46311582596982));
#30848=CARTESIAN_POINT('Ctrl Pts',(0.303921405375651,1.84951871719701,5.46415760180032));
#30849=CARTESIAN_POINT('Ctrl Pts',(0.316171466964028,1.86607588094039,5.46519937763082));
#30850=CARTESIAN_POINT('Ctrl Pts',(0.328448007338517,1.88266883336893,5.46624340528342));
#30851=CARTESIAN_POINT('Ctrl Pts',(0.339393701132029,1.90020213220819,5.46728743293601));
#30852=CARTESIAN_POINT('Ctrl Pts',(0.348881509286305,1.91843298075336,5.46833146058861));
#30853=CARTESIAN_POINT('Ctrl Pts',(0.352237222666619,1.92488099291831,5.46870071948448));
#30854=CARTESIAN_POINT('Ctrl Pts',(0.355410996953054,1.93141606682124,5.46906997838034));
#30855=CARTESIAN_POINT('Ctrl Pts',(0.358398667244586,1.93802689940208,5.46943923727621));
#30856=CARTESIAN_POINT('Ctrl Pts',(0.36684535931479,1.95671693601564,5.47048319992376));
#30857=CARTESIAN_POINT('Ctrl Pts',(0.373851290009961,1.97612516606932,5.47152716257132));
#30858=CARTESIAN_POINT('Ctrl Pts',(0.379301606985278,1.99600393787077,5.47257112521887));
#30859=CARTESIAN_POINT('Ctrl Pts',(0.384741897515215,2.01584614052945,5.47361316738464));
#30860=CARTESIAN_POINT('Ctrl Pts',(0.388632005013936,2.0361564808786,5.47465520955041));
#30861=CARTESIAN_POINT('Ctrl Pts',(0.390905779854375,2.056669164831,5.47569725171618));
#30862=CARTESIAN_POINT('Ctrl Pts',(0.393177112696356,2.07715981848309,5.47673817474503));
#30863=CARTESIAN_POINT('Ctrl Pts',(0.393835449691452,2.09785165991352,5.47777909777389));
#30864=CARTESIAN_POINT('Ctrl Pts',(0.392866034741345,2.11847075381819,5.47882002080274));
#30865=CARTESIAN_POINT('Ctrl Pts',(0.391896121924987,2.13910043715209,5.47986147842253));
#30866=CARTESIAN_POINT('Ctrl Pts',(0.389296805532323,2.15965656259733,5.48090293604233));
#30867=CARTESIAN_POINT('Ctrl Pts',(0.38510543517715,2.17986672521781,5.48194439366212));
#30868=CARTESIAN_POINT('Ctrl Pts',(0.380912784175606,2.20008306292406,5.48298616949262));
#30869=CARTESIAN_POINT('Ctrl Pts',(0.375127295534998,2.2199525148746,5.48402794532312));
#30870=CARTESIAN_POINT('Ctrl Pts',(0.367836915496096,2.23921527789118,5.48506972115361));
#30871=CARTESIAN_POINT('Ctrl Pts',(0.3605307771353,2.25851967780714,5.48611374880621));
#30872=CARTESIAN_POINT('Ctrl Pts',(0.351713567374897,2.27721410459293,5.48715777645881));
#30873=CARTESIAN_POINT('Ctrl Pts',(0.34152066549373,2.29506031129043,5.4882018041114));
#30874=CARTESIAN_POINT('Ctrl Pts',(0.337915569704419,2.30137228067564,5.48857106300727));
#30875=CARTESIAN_POINT('Ctrl Pts',(0.334138783928079,2.30757840050508,5.48894032190313));
#30876=CARTESIAN_POINT('Ctrl Pts',(0.330197557443822,2.31366905030475,5.489309580799));
#30877=CARTESIAN_POINT('Ctrl Pts',(0.319054987065194,2.33088843475665,5.49035354344655));
#30878=CARTESIAN_POINT('Ctrl Pts',(0.306528636618086,2.34728517233454,5.49139750609411));
#30879=CARTESIAN_POINT('Ctrl Pts',(0.292764564429977,2.3626286347947,5.49244146874166));
#30880=CARTESIAN_POINT('Ctrl Pts',(0.279025812735833,2.37794387130229,5.49348351090743));
#30881=CARTESIAN_POINT('Ctrl Pts',(0.264054300404986,2.39220909755274,5.4945255530732));
#30882=CARTESIAN_POINT('Ctrl Pts',(0.248037703876494,2.40522481461322,5.49556759523897));
#30883=CARTESIAN_POINT('Ctrl Pts',(0.232038308921056,2.41822655299806,5.49660851826782));
#30884=CARTESIAN_POINT('Ctrl Pts',(0.214996607882537,2.42998096217478,5.49764944129667));
#30885=CARTESIAN_POINT('Ctrl Pts',(0.19713494272663,2.44032734882194,5.49869036432552));
#30886=CARTESIAN_POINT('Ctrl Pts',(0.179264104285027,2.45067904910361,5.49973182194532));
#30887=CARTESIAN_POINT('Ctrl Pts',(0.1605730890359,2.45962089947064,5.50077327956511));
#30888=CARTESIAN_POINT('Ctrl Pts',(0.141311157947594,2.46703684643304,5.5018147371849));
#30889=CARTESIAN_POINT('Ctrl Pts',(0.122043341499598,2.47445505929055,5.5028565130154));
#30890=CARTESIAN_POINT('Ctrl Pts',(0.102204961011002,2.48034621021496,5.50389828884589));
#30891=CARTESIAN_POINT('Ctrl Pts',(0.0820620705349193,2.48464360982541,
5.50494006467639));
#30892=CARTESIAN_POINT('Ctrl Pts',(0.0618756407439544,2.48895029836264,
5.50598409232899));
#30893=CARTESIAN_POINT('Ctrl Pts',(0.0413841170300968,2.4916562615354,5.50702811998158));
#30894=CARTESIAN_POINT('Ctrl Pts',(0.0208611049511767,2.49274636128195,
5.50807214763418));
#30895=CARTESIAN_POINT('Ctrl Pts',(0.0136023845893694,2.49313191527356,
5.50844140653005));
#30896=CARTESIAN_POINT('Ctrl Pts',(0.00633972553699942,2.49331581097294,
5.50881066542592));
#30897=CARTESIAN_POINT('Ctrl Pts',(-0.000914858973369157,2.49329893596736,
5.50917992432179));
#30898=CARTESIAN_POINT('Ctrl Pts',(-0.0214249004024134,2.4932512272305,
5.51022388696934));
#30899=CARTESIAN_POINT('Ctrl Pts',(-0.0419923107651998,2.49159469781914,
5.5112678496169));
#30900=CARTESIAN_POINT('Ctrl Pts',(-0.0623441096933663,2.4883273129546,
5.51231181226445));
#30901=CARTESIAN_POINT('Ctrl Pts',(-0.0826584692943649,2.4850659387966,
5.51335385443022));
#30902=CARTESIAN_POINT('Ctrl Pts',(-0.10275727707859,2.48019964789877,5.51439589659599));
#30903=CARTESIAN_POINT('Ctrl Pts',(-0.122371198123852,2.47377824959424,
5.51543793876176));
#30904=CARTESIAN_POINT('Ctrl Pts',(-0.141964054126048,2.46736374777061,
5.51647886179061));
#30905=CARTESIAN_POINT('Ctrl Pts',(-0.161072352513457,2.45939765449231,
5.51751978481946));
#30906=CARTESIAN_POINT('Ctrl Pts',(-0.179440621740774,2.44997993266655,
5.51856070784832));
#30907=CARTESIAN_POINT('Ctrl Pts',(-0.197818324432443,2.44055737414431,
5.51960216546811));
#30908=CARTESIAN_POINT('Ctrl Pts',(-0.215454576598941,2.42968201904437,
5.5206436230879));
#30909=CARTESIAN_POINT('Ctrl Pts',(-0.232116868922016,2.4175006286007,5.52168508070769));
#30910=CARTESIAN_POINT('Ctrl Pts',(-0.248784252301796,2.4053155162112,5.52272685653819));
#30911=CARTESIAN_POINT('Ctrl Pts',(-0.264476511291741,2.39182403714412,
5.52376863236869));
#30912=CARTESIAN_POINT('Ctrl Pts',(-0.27899355240014,2.37721379424399,5.52481040819919));
#30913=CARTESIAN_POINT('Ctrl Pts',(-0.293541972422333,2.36257197097228,
5.52585443585178));
#30914=CARTESIAN_POINT('Ctrl Pts',(-0.306909626751238,2.34680711770463,
5.52689846350438));
#30915=CARTESIAN_POINT('Ctrl Pts',(-0.318935679401313,2.33014109238644,
5.52794249115697));
#30916=CARTESIAN_POINT('Ctrl Pts',(-0.323189136589131,2.32424653768552,
5.52831175005284));
#30917=CARTESIAN_POINT('Ctrl Pts',(-0.327275167958654,2.31823950998575,
5.52868100894871));
#30918=CARTESIAN_POINT('Ctrl Pts',(-0.331188016829293,2.31213059069517,
5.52905026784458));
#30919=CARTESIAN_POINT('Ctrl Pts',(-0.342509195383825,2.29445544699543,
5.53011865715149));
#30920=CARTESIAN_POINT('Ctrl Pts',(-0.35244220085537,2.27582419445772,5.53118704645841));
#30921=CARTESIAN_POINT('Ctrl Pts',(-0.360832686475196,2.25647575649631,
5.53225543576533));
#30922=CARTESIAN_POINT('Ctrl Pts',(-0.36920441509842,2.23717057212016,5.53332143667954));
#30923=CARTESIAN_POINT('Ctrl Pts',(-0.376040145698522,2.21715198672075,
5.53438743759376));
#30924=CARTESIAN_POINT('Ctrl Pts',(-0.381231056446065,2.1966838745656,5.53545343850798));
#30925=CARTESIAN_POINT('Ctrl Pts',(-0.386412884918501,2.17625157443546,
5.53651757429408));
#30926=CARTESIAN_POINT('Ctrl Pts',(-0.389955404934743,2.15537196405331,
5.53758171008019));
#30927=CARTESIAN_POINT('Ctrl Pts',(-0.391799306690207,2.1343248201317,5.53864584586629));
#30928=CARTESIAN_POINT('Ctrl Pts',(-0.392803043265827,2.12286770854543,
5.53922511317637));
#30929=CARTESIAN_POINT('Ctrl Pts',(-0.393304317595768,2.11136119740429,
5.53980438048645));
#30930=CARTESIAN_POINT('Ctrl Pts',(-0.393299971966862,2.0998515046609,5.54038364779653));
#30931=CARTESIAN_POINT('',(-0.393402607802015,2.09971271023449,5.66538360260035));
#30932=CARTESIAN_POINT('Ctrl Pts',(-0.392705315208772,2.09984964247381,
5.54038375297671));
#30933=CARTESIAN_POINT('Ctrl Pts',(-0.392895903822687,2.04339430721444,
5.54322937244026));
#30934=CARTESIAN_POINT('Ctrl Pts',(-0.355079068065668,1.855777880858,5.55269843974473));
#30935=CARTESIAN_POINT('Ctrl Pts',(-0.0662253309296011,1.63968570951168,
5.56879095489017));
#30936=CARTESIAN_POINT('Ctrl Pts',(0.351191528838419,1.79514011323788,5.58866129841293));
#30937=CARTESIAN_POINT('Ctrl Pts',(0.446437971306593,2.2302619601424,5.60853164193575));
#30938=CARTESIAN_POINT('Ctrl Pts',(0.132138352142635,2.54588619218082,5.62840198545851));
#30939=CARTESIAN_POINT('Ctrl Pts',(-0.283221592391678,2.45679442678442,
5.64735260062244));
#30940=CARTESIAN_POINT('Ctrl Pts',(-0.392738243985543,2.21217249115798,
5.65967976794542));
#30941=CARTESIAN_POINT('Ctrl Pts',(-0.393664350931912,2.0997147892973,5.66538348742747));
#30942=CARTESIAN_POINT('',(-0.393379133237835,2.10030487424134,5.79038368413719));
#30943=CARTESIAN_POINT('Ctrl Pts',(-0.393299894476397,2.09971189436798,
5.66538364779653));
#30944=CARTESIAN_POINT('Ctrl Pts',(-0.393286623951248,2.08159598283861,
5.66630332269905));
#30945=CARTESIAN_POINT('Ctrl Pts',(-0.392021608078033,2.06352518737575,
5.66722299760158));
#30946=CARTESIAN_POINT('Ctrl Pts',(-0.389523855042085,2.04563037288014,
5.66814267250411));
#30947=CARTESIAN_POINT('Ctrl Pts',(-0.386688547842559,2.02531719714043,
5.66918663515167));
#30948=CARTESIAN_POINT('Ctrl Pts',(-0.382251555055874,2.00516588071356,
5.67023059779923));
#30949=CARTESIAN_POINT('Ctrl Pts',(-0.376247968494637,1.98544714668041,
5.67127456044679));
#30950=CARTESIAN_POINT('Ctrl Pts',(-0.370255426177802,1.96576468738333,
5.67231660261256));
#30951=CARTESIAN_POINT('Ctrl Pts',(-0.362702165570659,1.94651394413396,
5.67335864477834));
#30952=CARTESIAN_POINT('Ctrl Pts',(-0.353674145819687,1.92795498095349,
5.67440068694411));
#30953=CARTESIAN_POINT('Ctrl Pts',(-0.3446558220201,1.90941594980791,5.67544160997296));
#30954=CARTESIAN_POINT('Ctrl Pts',(-0.334166177652963,1.89156789471963,
5.67648253300182));
#30955=CARTESIAN_POINT('Ctrl Pts',(-0.322338975374128,1.87465032736931,
5.67752345603067));
#30956=CARTESIAN_POINT('Ctrl Pts',(-0.310505698952456,1.85772407159733,
5.67856491365047));
#30957=CARTESIAN_POINT('Ctrl Pts',(-0.297333900644732,1.84172987051153,
5.67960637127026));
#30958=CARTESIAN_POINT('Ctrl Pts',(-0.283000585657215,1.82687812515715,
5.68064782889005));
#30959=CARTESIAN_POINT('Ctrl Pts',(-0.268662891217087,1.81202184194708,
5.68168960472055));
#30960=CARTESIAN_POINT('Ctrl Pts',(-0.253163510141973,1.79830921324518,
5.68273138055105));
#30961=CARTESIAN_POINT('Ctrl Pts',(-0.236715503685208,1.78591297334169,
5.68377315638155));
#30962=CARTESIAN_POINT('Ctrl Pts',(-0.220231944489237,1.77348993868434,
5.68481718403414));
#30963=CARTESIAN_POINT('Ctrl Pts',(-0.202796287492711,1.76238936906338,
5.68586121168674));
#30964=CARTESIAN_POINT('Ctrl Pts',(-0.184650194597699,1.75274044918097,
5.68690523933934));
#30965=CARTESIAN_POINT('Ctrl Pts',(-0.178232159395585,1.74932775269441,
5.68727449823519));
#30966=CARTESIAN_POINT('Ctrl Pts',(-0.171725454303548,1.74609621699476,
5.68764375713103));
#30967=CARTESIAN_POINT('Ctrl Pts',(-0.165141345046674,1.74305010693912,
5.68801301602688));
#30968=CARTESIAN_POINT('Ctrl Pts',(-0.14652686017205,1.73443819493324,5.68905697867443));
#30969=CARTESIAN_POINT('Ctrl Pts',(-0.127181448156699,1.72726062621688,
5.69010094132198));
#30970=CARTESIAN_POINT('Ctrl Pts',(-0.107351733646389,1.72163444226104,
5.69114490396954));
#30971=CARTESIAN_POINT('Ctrl Pts',(-0.0875584980326944,1.71601860827684,
5.6921869461353));
#30972=CARTESIAN_POINT('Ctrl Pts',(-0.0672834119905888,1.71194874987206,
5.69322898830107));
#30973=CARTESIAN_POINT('Ctrl Pts',(-0.0467916732445428,1.70949336841101,
5.69427103046684));
#30974=CARTESIAN_POINT('Ctrl Pts',(-0.0263219423039875,1.70704062399109,
5.6953119534957));
#30975=CARTESIAN_POINT('Ctrl Pts',(-0.0056367439956138,1.7061990300724,
5.69635287652455));
#30976=CARTESIAN_POINT('Ctrl Pts',(0.0149901278286173,1.7069857686194,5.69739379955341));
#30977=CARTESIAN_POINT('Ctrl Pts',(0.0356275930766123,1.70777291121482,
5.6984352571732));
#30978=CARTESIAN_POINT('Ctrl Pts',(0.0562059361390714,1.71019004502023,
5.69947671479299));
#30979=CARTESIAN_POINT('Ctrl Pts',(0.0764524319336417,1.71420223477652,
5.70051817241279));
#30980=CARTESIAN_POINT('Ctrl Pts',(0.0967051139153531,1.7182156504317,5.70155994824329));
#30981=CARTESIAN_POINT('Ctrl Pts',(0.116625032676036,1.72382491385864,5.70260172407379));
#30982=CARTESIAN_POINT('Ctrl Pts',(0.135951616225552,1.73094438353324,5.70364349990428));
#30983=CARTESIAN_POINT('Ctrl Pts',(0.155319974623986,1.7380792421031,5.70468752755688));
#30984=CARTESIAN_POINT('Ctrl Pts',(0.174091768484672,1.74673051577,5.70573155520948));
#30985=CARTESIAN_POINT('Ctrl Pts',(0.1920275610429,1.75676494089339,5.70677558286208));
#30986=CARTESIAN_POINT('Ctrl Pts',(0.198371215772838,1.76031398553079,5.70714484175795));
#30987=CARTESIAN_POINT('Ctrl Pts',(0.204610545883134,1.76403565100655,5.70751410065382));
#30988=CARTESIAN_POINT('Ctrl Pts',(0.210735867065037,1.76792277354153,5.70788335954968));
#30989=CARTESIAN_POINT('Ctrl Pts',(0.228053273875588,1.77891238212885,5.70892732219724));
#30990=CARTESIAN_POINT('Ctrl Pts',(0.244560323235575,1.79129300328244,5.70997128484479));
#30991=CARTESIAN_POINT('Ctrl Pts',(0.260025102203642,1.80492062724754,5.71101524749234));
#30992=CARTESIAN_POINT('Ctrl Pts',(0.275461432044374,1.8185231817299,5.71205728965811));
#30993=CARTESIAN_POINT('Ctrl Pts',(0.289858712281573,1.83336774919484,5.71309933182388));
#30994=CARTESIAN_POINT('Ctrl Pts',(0.30301578942157,1.84926842767369,5.71414137398965));
#30995=CARTESIAN_POINT('Ctrl Pts',(0.316158736067408,1.86515202907364,5.71518229701851));
#30996=CARTESIAN_POINT('Ctrl Pts',(0.328063634904601,1.88208894417223,5.71622322004736));
#30997=CARTESIAN_POINT('Ctrl Pts',(0.338567829470585,1.89985826310443,5.71726414307621));
#30998=CARTESIAN_POINT('Ctrl Pts',(0.349077418717127,1.91763670789571,5.718305600696));
#30999=CARTESIAN_POINT('Ctrl Pts',(0.358184478263024,1.93624778538888,5.71934705831579));
#31000=CARTESIAN_POINT('Ctrl Pts',(0.365770751284716,1.95544327236474,5.72038851593558));
#31001=CARTESIAN_POINT('Ctrl Pts',(0.373359342243549,1.97464462439872,5.72143029176608));
#31002=CARTESIAN_POINT('Ctrl Pts',(0.379425985079017,1.99443004439254,5.72247206759658));
#31003=CARTESIAN_POINT('Ctrl Pts',(0.383901636391456,2.01453407944705,5.72351384342707));
#31004=CARTESIAN_POINT('Ctrl Pts',(0.388386961925772,2.03468156982956,5.72455787107967));
#31005=CARTESIAN_POINT('Ctrl Pts',(0.391274327332497,2.05514832095952,5.72560189873226));
#31006=CARTESIAN_POINT('Ctrl Pts',(0.392546171619527,2.07566087210164,5.72664592638486));
#31007=CARTESIAN_POINT('Ctrl Pts',(0.392996006272832,2.08291589256721,5.72701518528073));
#31008=CARTESIAN_POINT('Ctrl Pts',(0.393244225432926,2.09017663780359,5.7273844441766));
#31009=CARTESIAN_POINT('Ctrl Pts',(0.393291610242275,2.09743108718749,5.72775370307247));
#31010=CARTESIAN_POINT('Ctrl Pts',(0.393425575792125,2.11794074658926,5.72879766572002));
#31011=CARTESIAN_POINT('Ctrl Pts',(0.391951291940804,2.13852202317378,5.72984162836757));
#31012=CARTESIAN_POINT('Ctrl Pts',(0.388864306002967,2.15890196530534,5.73088559101513));
#31013=CARTESIAN_POINT('Ctrl Pts',(0.385782998908404,2.17924441633728,5.7319276331809));
#31014=CARTESIAN_POINT('Ctrl Pts',(0.381094928735773,2.19938553992826,5.73296967534667));
#31015=CARTESIAN_POINT('Ctrl Pts',(0.374847517168071,2.21905557052458,5.73401171751244));
#31016=CARTESIAN_POINT('Ctrl Pts',(0.368606815222249,2.23870447581704,5.73505264054129));
#31017=CARTESIAN_POINT('Ctrl Pts',(0.360810290610757,2.25788258608275,5.73609356357015));
#31018=CARTESIAN_POINT('Ctrl Pts',(0.351555639421154,2.27633355435419,5.737134486599));
#31019=CARTESIAN_POINT('Ctrl Pts',(0.342296235283906,2.29479399856205,5.73817594421879));
#31020=CARTESIAN_POINT('Ctrl Pts',(0.331577523994065,2.31252588981243,5.73921740183859));
#31021=CARTESIAN_POINT('Ctrl Pts',(0.31954420152327,2.3292954279371,5.74025885945838));
#31022=CARTESIAN_POINT('Ctrl Pts',(0.307507202347852,2.34607008988675,5.74130063528888));
#31023=CARTESIAN_POINT('Ctrl Pts',(0.294155250355389,2.36188123714482,5.74234241111938));
#31024=CARTESIAN_POINT('Ctrl Pts',(0.279674168656474,2.37652712233398,5.74338418694988));
#31025=CARTESIAN_POINT('Ctrl Pts',(0.265161785770851,2.39120466493632,5.74442821460247));
#31026=CARTESIAN_POINT('Ctrl Pts',(0.249515958042227,2.40471143566417,5.74547224225507));
#31027=CARTESIAN_POINT('Ctrl Pts',(0.23295711007065,2.4168846396838,5.74651626990767));
#31028=CARTESIAN_POINT('Ctrl Pts',(0.22710046259244,2.42119014238216,5.74688552880353));
#31029=CARTESIAN_POINT('Ctrl Pts',(0.221129863515003,2.4253292220859,5.7472547876994));
#31030=CARTESIAN_POINT('Ctrl Pts',(0.215055842840153,2.42929602861303,5.74762404659526));
#31031=CARTESIAN_POINT('Ctrl Pts',(0.197883471975067,2.44051091846612,5.74866800924282));
#31032=CARTESIAN_POINT('Ctrl Pts',(0.179780309640395,2.45041233110304,5.74971197189037));
#31033=CARTESIAN_POINT('Ctrl Pts',(0.160973448139428,2.45884876897393,5.75075593453792));
#31034=CARTESIAN_POINT('Ctrl Pts',(0.142201183886746,2.46726968710827,5.75179797670369));
#31035=CARTESIAN_POINT('Ctrl Pts',(0.122728429464549,2.47423062789692,5.75284001886946));
#31036=CARTESIAN_POINT('Ctrl Pts',(0.102807678794231,2.47962543537142,5.75388206103523));
#31037=CARTESIAN_POINT('Ctrl Pts',(0.082908322697187,2.48501444890745,5.75492298406409));
#31038=CARTESIAN_POINT('Ctrl Pts',(0.0625626245670739,2.48884044903543,
5.75596390709294));
#31039=CARTESIAN_POINT('Ctrl Pts',(0.0420390101813584,2.49104681512956,
5.75700483012179));
#31040=CARTESIAN_POINT('Ctrl Pts',(0.0215048554022065,2.49325431435581,
5.75804628774159));
#31041=CARTESIAN_POINT('Ctrl Pts',(0.000793331664292161,2.49384042312017,
5.75908774536138));
#31042=CARTESIAN_POINT('Ctrl Pts',(-0.0198206511209501,2.49280024413071,
5.76012920298117));
#31043=CARTESIAN_POINT('Ctrl Pts',(-0.0404409323766265,2.49175974732122,
5.76117097881167));
#31044=CARTESIAN_POINT('Ctrl Pts',(-0.0609628809480463,2.48909204672758,
5.76221275464216));
#31045=CARTESIAN_POINT('Ctrl Pts',(-0.0811162746207978,2.48484417624753,
5.76325453047266));
#31046=CARTESIAN_POINT('Ctrl Pts',(-0.101313230311313,2.48058712389905,
5.76429855812526));
#31047=CARTESIAN_POINT('Ctrl Pts',(-0.121139334221363,2.47474329086276,
5.76534258577786));
#31048=CARTESIAN_POINT('Ctrl Pts',(-0.140338385721195,2.46740989030396,
5.76638661343045));
#31049=CARTESIAN_POINT('Ctrl Pts',(-0.147128838580244,2.46481616265072,
5.76675587232632));
#31050=CARTESIAN_POINT('Ctrl Pts',(-0.153841044065357,2.46203653467856,
5.76712513122218));
#31051=CARTESIAN_POINT('Ctrl Pts',(-0.160464383158511,2.45907669339232,
5.76749439011805));
#31052=CARTESIAN_POINT('Ctrl Pts',(-0.179189777977002,2.45070867902591,
5.7685383527656));
#31053=CARTESIAN_POINT('Ctrl Pts',(-0.197314631875966,2.44084702957649,
5.76958231541316));
#31054=CARTESIAN_POINT('Ctrl Pts',(-0.214588633835922,2.42960067995748,
5.77062627806071));
#31055=CARTESIAN_POINT('Ctrl Pts',(-0.231830858407894,2.41837501921045,
5.77166832022648));
#31056=CARTESIAN_POINT('Ctrl Pts',(-0.248224695873425,2.40577006166971,
5.77271036239225));
#31057=CARTESIAN_POINT('Ctrl Pts',(-0.263544208871659,2.39194064460128,
5.77375240455802));
#31058=CARTESIAN_POINT('Ctrl Pts',(-0.2788472689536,2.37812608010952,5.77479332758687));
#31059=CARTESIAN_POINT('Ctrl Pts',(-0.29307773238465,2.36309013584524,5.77583425061573));
#31060=CARTESIAN_POINT('Ctrl Pts',(-0.306042687805391,2.34702785924031,
5.77687517364458));
#31061=CARTESIAN_POINT('Ctrl Pts',(-0.319014301689326,2.33095733346876,
5.77791663126437));
#31062=CARTESIAN_POINT('Ctrl Pts',(-0.330718634465133,2.31385998474731,
5.77895808888416));
#31063=CARTESIAN_POINT('Ctrl Pts',(-0.341002754699717,2.29596431125897,
5.77999954650396));
#31064=CARTESIAN_POINT('Ctrl Pts',(-0.351290017181381,2.27806316986221,
5.78104132233445));
#31065=CARTESIAN_POINT('Ctrl Pts',(-0.360155868328508,2.25936387353689,
5.78208309816495));
#31066=CARTESIAN_POINT('Ctrl Pts',(-0.367493578917158,2.24011909025775,
5.78312487399545));
#31067=CARTESIAN_POINT('Ctrl Pts',(-0.37484715013376,2.22083270894282,5.78416890164805));
#31068=CARTESIAN_POINT('Ctrl Pts',(-0.380665778968099,2.20099919338717,
5.78521292930064));
#31069=CARTESIAN_POINT('Ctrl Pts',(-0.384892517959947,2.18088658491031,
5.78625695695324));
#31070=CARTESIAN_POINT('Ctrl Pts',(-0.386387460138313,2.17377301892314,
5.78662621584911));
#31071=CARTESIAN_POINT('Ctrl Pts',(-0.387683737282749,2.16662461352731,
5.78699547474497));
#31072=CARTESIAN_POINT('Ctrl Pts',(-0.388780382862406,2.15945337586177,
5.78736473364084));
#31073=CARTESIAN_POINT('Ctrl Pts',(-0.391768962511404,2.13991031168231,
5.78837103835941));
#31074=CARTESIAN_POINT('Ctrl Pts',(-0.393284476002902,2.12013639346441,
5.78937734307797));
#31075=CARTESIAN_POINT('Ctrl Pts',(-0.393299881326936,2.10030552940591,
5.79038364779653));
#31076=CARTESIAN_POINT('',(-0.393073346508676,2.10012267207431,5.91538361492347));
#31077=CARTESIAN_POINT('Ctrl Pts',(-0.393617414534465,2.10030290440287,
5.79038379340017));
#31078=CARTESIAN_POINT('Ctrl Pts',(-0.392667861142396,1.98951876646131,
5.79600088798799));
#31079=CARTESIAN_POINT('Ctrl Pts',(-0.285965102257327,1.74650375455207,
5.80824143041673));
#31080=CARTESIAN_POINT('Ctrl Pts',(0.126302422767384,1.65242571735234,5.82710542068643));
#31081=CARTESIAN_POINT('Ctrl Pts',(0.444698253975958,1.96391729207861,5.84697576420921));
#31082=CARTESIAN_POINT('Ctrl Pts',(0.355143977362131,2.40024622533497,5.866846107732));
#31083=CARTESIAN_POINT('Ctrl Pts',(-0.0602065499947629,2.56114012167909,
5.88671645125477));
#31084=CARTESIAN_POINT('Ctrl Pts',(-0.353428603581954,2.34769677766452,
5.90289560167169));
#31085=CARTESIAN_POINT('Ctrl Pts',(-0.392848721613529,2.15830431178998,
5.91245130424765));
#31086=CARTESIAN_POINT('Ctrl Pts',(-0.392687677656695,2.10012366230725,
5.91538355898269));
#31087=CARTESIAN_POINT('',(-0.393299837367108,2.09964233114976,6.04038364780031));
#31088=CARTESIAN_POINT('Ctrl Pts',(-0.393299981050075,2.10012209017358,
5.91538364779653));
#31089=CARTESIAN_POINT('Ctrl Pts',(-0.393306574629672,2.07888160328984,
5.9164524844718));
#31090=CARTESIAN_POINT('Ctrl Pts',(-0.391588166963785,2.05765663935881,
5.91752132114708));
#31091=CARTESIAN_POINT('Ctrl Pts',(-0.388178268836697,2.03673451491576,
5.91859015782235));
#31092=CARTESIAN_POINT('Ctrl Pts',(-0.384764862865103,2.01579086737831,
5.9196600940357));
#31093=CARTESIAN_POINT('Ctrl Pts',(-0.379656662610636,1.99515134218412,
5.92073003024906));
#31094=CARTESIAN_POINT('Ctrl Pts',(-0.3729380446889,1.97509161427822,5.92179996646242));
#31095=CARTESIAN_POINT('Ctrl Pts',(-0.366199323910776,1.95497186542248,
5.92287310404461));
#31096=CARTESIAN_POINT('Ctrl Pts',(-0.357840831602137,1.93543600556655,
5.92394624162681));
#31097=CARTESIAN_POINT('Ctrl Pts',(-0.347995182185459,1.9167399575038,5.925019379209));
#31098=CARTESIAN_POINT('Ctrl Pts',(-0.343598208863494,1.90839048038156,
5.92549863223945));
#31099=CARTESIAN_POINT('Ctrl Pts',(-0.338905235391115,1.90020814633051,
5.9259778852699));
#31100=CARTESIAN_POINT('Ctrl Pts',(-0.333930840386804,1.89221385070568,
5.92645713830036));
#31101=CARTESIAN_POINT('Ctrl Pts',(-0.323095055845649,1.87479978027621,
5.92750110094791));
#31102=CARTESIAN_POINT('Ctrl Pts',(-0.310861135380553,1.85818371429248,
5.92854506359546));
#31103=CARTESIAN_POINT('Ctrl Pts',(-0.29737102887443,1.84259883219736,5.92958902624301));
#31104=CARTESIAN_POINT('Ctrl Pts',(-0.283905738872863,1.82704262017221,
5.93063106840878));
#31105=CARTESIAN_POINT('Ctrl Pts',(-0.269189280992312,1.81251441557219,
5.93167311057455));
#31106=CARTESIAN_POINT('Ctrl Pts',(-0.253405768145051,1.79921701066913,
5.93271515274032));
#31107=CARTESIAN_POINT('Ctrl Pts',(-0.23763920654264,1.78593388697003,5.93375607576918));
#31108=CARTESIAN_POINT('Ctrl Pts',(-0.220808406270014,1.77387943254175,
5.93479699879803));
#31109=CARTESIAN_POINT('Ctrl Pts',(-0.203132827758717,1.76321825422576,
5.93583792182689));
#31110=CARTESIAN_POINT('Ctrl Pts',(-0.185448171530978,1.75255160060644,
5.93687937944668));
#31111=CARTESIAN_POINT('Ctrl Pts',(-0.166918492036109,1.74328004642999,
5.93792083706647));
#31112=CARTESIAN_POINT('Ctrl Pts',(-0.147790955268361,1.73552404257501,
5.93896229468627));
#31113=CARTESIAN_POINT('Ctrl Pts',(-0.128657574204237,1.72776566892271,
5.94000407051677));
#31114=CARTESIAN_POINT('Ctrl Pts',(-0.108926667087551,1.7215240101706,5.94104584634727));
#31115=CARTESIAN_POINT('Ctrl Pts',(-0.0888630648357885,1.71687045831992,
5.94208762217777));
#31116=CARTESIAN_POINT('Ctrl Pts',(-0.0687560946524599,1.7122068477113,
5.94313164983036));
#31117=CARTESIAN_POINT('Ctrl Pts',(-0.0483157219466113,1.70913830661598,
5.94417567748296));
#31118=CARTESIAN_POINT('Ctrl Pts',(-0.0278152411750107,1.70768481757855,
5.94521970513556));
#31119=CARTESIAN_POINT('Ctrl Pts',(-0.0205644898413008,1.70717073755798,
5.94558896403142));
#31120=CARTESIAN_POINT('Ctrl Pts',(-0.0133062281057095,1.70685821441269,
5.94595822292729));
#31121=CARTESIAN_POINT('Ctrl Pts',(-0.00605248303909771,1.70674657350627,
5.94632748182316));
#31122=CARTESIAN_POINT('Ctrl Pts',(0.0144551851285342,1.70643094418076,
5.94737144447072));
#31123=CARTESIAN_POINT('Ctrl Pts',(0.0350487131087565,1.70772286679837,
5.94841540711827));
#31124=CARTESIAN_POINT('Ctrl Pts',(0.055455199414578,1.71062921160173,5.94945936976582));
#31125=CARTESIAN_POINT('Ctrl Pts',(0.0758241457899177,1.71353020987065,
5.95050141193159));
#31126=CARTESIAN_POINT('Ctrl Pts',(0.096006004896433,1.71803969148774,5.95154345409736));
#31127=CARTESIAN_POINT('Ctrl Pts',(0.115730601714979,1.7241126261409,5.95258549626313));
#31128=CARTESIAN_POINT('Ctrl Pts',(0.135434014626404,1.73017903855765,5.95362641929198));
#31129=CARTESIAN_POINT('Ctrl Pts',(0.154680432038124,1.73780538277979,5.95466734232083));
#31130=CARTESIAN_POINT('Ctrl Pts',(0.173212651673648,1.74689623720472,5.95570826534969));
#31131=CARTESIAN_POINT('Ctrl Pts',(0.191754388974173,1.75599176045555,5.95674972296948));
#31132=CARTESIAN_POINT('Ctrl Pts',(0.209580528047845,1.76655298693527,5.95779118058927));
#31133=CARTESIAN_POINT('Ctrl Pts',(0.226455996220631,1.77843729728757,5.95883263820906));
#31134=CARTESIAN_POINT('Ctrl Pts',(0.24333662058465,1.79032523881479,5.95987441403956));
#31135=CARTESIAN_POINT('Ctrl Pts',(0.259265415553611,1.80353661612611,5.96091618987005));
#31136=CARTESIAN_POINT('Ctrl Pts',(0.274038995693815,1.81788740042471,5.96195796570055));
#31137=CARTESIAN_POINT('Ctrl Pts',(0.288844509262749,1.83226920426924,5.96300199335315));
#31138=CARTESIAN_POINT('Ctrl Pts',(0.302489336635816,1.84779477887269,5.96404602100574));
#31139=CARTESIAN_POINT('Ctrl Pts',(0.314808736904162,1.86424515027511,5.96509004865834));
#31140=CARTESIAN_POINT('Ctrl Pts',(0.319165947299418,1.87006343101273,5.9654593075542));
#31141=CARTESIAN_POINT('Ctrl Pts',(0.323357750581443,1.87599713300921,5.96582856645007));
#31142=CARTESIAN_POINT('Ctrl Pts',(0.327378203525815,1.88203577849516,5.96619782534594));
#31143=CARTESIAN_POINT('Ctrl Pts',(0.338744761643042,1.89910813721073,5.96724178799349));
#31144=CARTESIAN_POINT('Ctrl Pts',(0.348806138772213,1.91712288530741,5.96828575064105));
#31145=CARTESIAN_POINT('Ctrl Pts',(0.357408831784391,1.9358542813153,5.9693297132886));
#31146=CARTESIAN_POINT('Ctrl Pts',(0.365995699215781,1.95455121890181,5.97037175545437));
#31147=CARTESIAN_POINT('Ctrl Pts',(0.373128851330051,1.97396155126283,5.97141379762014));
#31148=CARTESIAN_POINT('Ctrl Pts',(0.378699899800244,1.99383373468335,5.97245583978591));
#31149=CARTESIAN_POINT('Ctrl Pts',(0.384264965051899,2.01368457569106,5.97349676281477));
#31150=CARTESIAN_POINT('Ctrl Pts',(0.388271031790586,2.03399558597284,5.97453768584362));
#31151=CARTESIAN_POINT('Ctrl Pts',(0.39065910396862,2.05449885181191,5.97557860887248));
#31152=CARTESIAN_POINT('Ctrl Pts',(0.393048402598285,2.07501264759393,5.97662006649227));
#31153=CARTESIAN_POINT('Ctrl Pts',(0.393817945460347,2.09571816721585,5.97766152411206));
#31154=CARTESIAN_POINT('Ctrl Pts',(0.392960400377164,2.11634055492995,5.97870298173186));
#31155=CARTESIAN_POINT('Ctrl Pts',(0.392102593276572,2.13696924368257,5.97974475756236));
#31156=CARTESIAN_POINT('Ctrl Pts',(0.389616775223395,2.15751401694081,5.98078653339286));
#31157=CARTESIAN_POINT('Ctrl Pts',(0.385547584714711,2.17770424647761,5.98182830922336));
#31158=CARTESIAN_POINT('Ctrl Pts',(0.381469598558404,2.19793811765371,5.98287233687595));
#31159=CARTESIAN_POINT('Ctrl Pts',(0.375801609059394,2.21781520687339,5.98391636452855));
#31160=CARTESIAN_POINT('Ctrl Pts',(0.368638556213166,2.23707846246976,5.98496039218115));
#31161=CARTESIAN_POINT('Ctrl Pts',(0.366105078313,2.24389162347615,5.98532965107701));
#31162=CARTESIAN_POINT('Ctrl Pts',(0.363385014292737,2.25062818683317,5.98569890997288));
#31163=CARTESIAN_POINT('Ctrl Pts',(0.360483956873705,2.25727748356544,5.98606816886874));
#31164=CARTESIAN_POINT('Ctrl Pts',(0.352282135285122,2.2760762653923,5.98711213151629));
#31165=CARTESIAN_POINT('Ctrl Pts',(0.342581417780033,2.29428776007584,5.98815609416385));
#31166=CARTESIAN_POINT('Ctrl Pts',(0.331488517810789,2.31166070150032,5.9892000568114));
#31167=CARTESIAN_POINT('Ctrl Pts',(0.320416024426366,2.329001683527,5.99024209897717));
#31168=CARTESIAN_POINT('Ctrl Pts',(0.307956773574515,2.34550652916884,5.99128414114294));
#31169=CARTESIAN_POINT('Ctrl Pts',(0.294263595154714,2.36094793842187,5.99232618330871));
#31170=CARTESIAN_POINT('Ctrl Pts',(0.280585122993427,2.37637276384393,5.99336710633756));
#31171=CARTESIAN_POINT('Ctrl Pts',(0.265675818203077,2.39073585334616,5.99440802936641));
#31172=CARTESIAN_POINT('Ctrl Pts',(0.24972901180695,2.4038425754596,5.99544895239527));
#31173=CARTESIAN_POINT('Ctrl Pts',(0.233774015546679,2.41695602884392,5.99649041001506));
#31174=CARTESIAN_POINT('Ctrl Pts',(0.216781011384998,2.42881134615688,5.99753186763485));
#31175=CARTESIAN_POINT('Ctrl Pts',(0.198977133915454,2.43925357798967,5.99857332525464));
#31176=CARTESIAN_POINT('Ctrl Pts',(0.181167816585161,2.44969900037953,5.99961510108513));
#31177=CARTESIAN_POINT('Ctrl Pts',(0.162547785160077,2.45873013703855,6.00065687691563));
#31178=CARTESIAN_POINT('Ctrl Pts',(0.143368752323972,2.46623802486507,6.00169865274613));
#31179=CARTESIAN_POINT('Ctrl Pts',(0.124148263573157,2.4737621411615,6.00274268039872));
#31180=CARTESIAN_POINT('Ctrl Pts',(0.104367065940325,2.47975622165971,6.00378670805132));
#31181=CARTESIAN_POINT('Ctrl Pts',(0.0842926858043522,2.48416094689581,
6.00483073570392));
#31182=CARTESIAN_POINT('Ctrl Pts',(0.0771926406802738,2.48571884047578,
6.00519999459978));
#31183=CARTESIAN_POINT('Ctrl Pts',(0.0700559977930121,2.48707838541361,
6.00556925349565));
#31184=CARTESIAN_POINT('Ctrl Pts',(0.0628947552492071,2.48823850886039,
6.00593851239152));
#31185=CARTESIAN_POINT('Ctrl Pts',(0.0426486086851545,2.49151839069546,
6.00698247503907));
#31186=CARTESIAN_POINT('Ctrl Pts',(0.0220848842232862,2.49322006486484,
6.00802643768662));
#31187=CARTESIAN_POINT('Ctrl Pts',(0.00147261683243485,2.49329724306136,
6.00907040033418));
#31188=CARTESIAN_POINT('Ctrl Pts',(-0.0191017320714582,2.49337427928027,
6.01011244249995));
#31189=CARTESIAN_POINT('Ctrl Pts',(-0.0397237194067034,2.49183268925838,
6.01115448466572));
#31190=CARTESIAN_POINT('Ctrl Pts',(-0.0601194976742482,2.48867793351231,
6.01219652683149));
#31191=CARTESIAN_POINT('Ctrl Pts',(-0.0804933711963228,2.48552656592435,
6.01323744986034));
#31192=CARTESIAN_POINT('Ctrl Pts',(-0.100640790089124,2.48076555538682,
6.0142783728892));
#31193=CARTESIAN_POINT('Ctrl Pts',(-0.120293451152618,2.47445210055465,
6.01531929591805));
#31194=CARTESIAN_POINT('Ctrl Pts',(-0.139956205310639,2.46813540329663,
6.01636075353784));
#31195=CARTESIAN_POINT('Ctrl Pts',(-0.159122988566352,2.46026487862171,
6.01740221115763));
#31196=CARTESIAN_POINT('Ctrl Pts',(-0.177540564623014,2.45094762844809,
6.01844366877743));
#31197=CARTESIAN_POINT('Ctrl Pts',(-0.195963768052096,2.44162753144836,
6.01948544460792));
#31198=CARTESIAN_POINT('Ctrl Pts',(-0.213636668904965,2.43086019310176,
6.02052722043842));
#31199=CARTESIAN_POINT('Ctrl Pts',(-0.230331392430929,2.41879827424381,
6.02156899626892));
#31200=CARTESIAN_POINT('Ctrl Pts',(-0.247062201980651,2.40671028327452,
6.02261302392152));
#31201=CARTESIAN_POINT('Ctrl Pts',(-0.262810051886074,2.3933226022145,6.02365705157412));
#31202=CARTESIAN_POINT('Ctrl Pts',(-0.27738024841712,2.3788280613354,6.02470107922672));
#31203=CARTESIAN_POINT('Ctrl Pts',(-0.28253353594759,2.37370153221734,6.02507033812258));
#31204=CARTESIAN_POINT('Ctrl Pts',(-0.287539859418942,2.36843686134083,
6.02543959701845));
#31205=CARTESIAN_POINT('Ctrl Pts',(-0.292391821968674,2.36304355617623,
6.02580885591431));
#31206=CARTESIAN_POINT('Ctrl Pts',(-0.305973877518868,2.34794612506585,
6.02684251905261));
#31207=CARTESIAN_POINT('Ctrl Pts',(-0.318428148253966,2.33174412380622,
6.0278761821909));
#31208=CARTESIAN_POINT('Ctrl Pts',(-0.329571298961343,2.31463375526914,
6.0289098453292));
#31209=CARTESIAN_POINT('Ctrl Pts',(-0.340694798819114,2.29755356071854,
6.02994168561152));
#31210=CARTESIAN_POINT('Ctrl Pts',(-0.350511304813724,2.27956876371628,
6.03097352589383));
#31211=CARTESIAN_POINT('Ctrl Pts',(-0.358878100659044,2.26090804475649,
6.03200536617615));
#31212=CARTESIAN_POINT('Ctrl Pts',(-0.36723586424299,2.24226747072365,6.03303609254924));
#31213=CARTESIAN_POINT('Ctrl Pts',(-0.37414669104312,2.22295309431302,6.03406681892232));
#31214=CARTESIAN_POINT('Ctrl Pts',(-0.379514314441636,2.20321712616565,
6.03509754529541));
#31215=CARTESIAN_POINT('Ctrl Pts',(-0.384885045315495,2.18346973228479,
6.03612886838636));
#31216=CARTESIAN_POINT('Ctrl Pts',(-0.388710579364642,2.16330098220474,
6.03716019147732));
#31217=CARTESIAN_POINT('Ctrl Pts',(-0.390944793159439,2.14297742083377,
6.03819151456827));
#31218=CARTESIAN_POINT('Ctrl Pts',(-0.392527774070581,2.12857780976183,
6.03892222564436));
#31219=CARTESIAN_POINT('Ctrl Pts',(-0.393312985966233,2.11410079734308,
6.03965293672044));
#31220=CARTESIAN_POINT('Ctrl Pts',(-0.393299837367176,2.09964233122461,
6.04038364779653));
#31221=CARTESIAN_POINT('',(-0.393299995571548,2.10005902050583,6.16538364780005));
#31222=CARTESIAN_POINT('Ctrl Pts',(-0.393299837367108,2.09964233114976,
6.04038364780031));
#31223=CARTESIAN_POINT('Ctrl Pts',(-0.393276092566639,2.07353207257771,
6.04170322450934));
#31224=CARTESIAN_POINT('Ctrl Pts',(-0.390648350684809,2.04753914190753,
6.04302280121837));
#31225=CARTESIAN_POINT('Ctrl Pts',(-0.385508793148372,2.02210352764544,
6.0443423779274));
#31226=CARTESIAN_POINT('Ctrl Pts',(-0.383773218647329,2.01351418834557,
6.0447879850973));
#31227=CARTESIAN_POINT('Ctrl Pts',(-0.381751609043668,2.00498820323357,
6.0452335922672));
#31228=CARTESIAN_POINT('Ctrl Pts',(-0.379448708082446,1.99654195084691,
6.0456791994371));
#31229=CARTESIAN_POINT('Ctrl Pts',(-0.374053501840455,1.97675418126185,
6.04672316208466));
#31230=CARTESIAN_POINT('Ctrl Pts',(-0.367090192188503,1.95733061883335,
6.04776712473221));
#31231=CARTESIAN_POINT('Ctrl Pts',(-0.358628009777519,1.93853532707426,
6.04881108737976));
#31232=CARTESIAN_POINT('Ctrl Pts',(-0.350181394462932,1.91977461127967,
6.04985312954553));
#31233=CARTESIAN_POINT('Ctrl Pts',(-0.340241624021866,1.9016405597459,6.0508951717113));
#31234=CARTESIAN_POINT('Ctrl Pts',(-0.328927028196155,1.88438019543176,
6.05193721387707));
#31235=CARTESIAN_POINT('Ctrl Pts',(-0.317624584068612,1.86713836847774,
6.05297813690593));
#31236=CARTESIAN_POINT('Ctrl Pts',(-0.304950622987712,1.85076899402723,
6.05401905993478));
#31237=CARTESIAN_POINT('Ctrl Pts',(-0.291068276854987,1.83549263108815,
6.05505998296363));
#31238=CARTESIAN_POINT('Ctrl Pts',(-0.277178801111106,1.82020842260722,
6.05610144058343));
#31239=CARTESIAN_POINT('Ctrl Pts',(-0.262080183410367,1.80601890244067,
6.05714289820322));
#31240=CARTESIAN_POINT('Ctrl Pts',(-0.245974745650272,1.79311025676591,
6.05818435582301));
#31241=CARTESIAN_POINT('Ctrl Pts',(-0.229864386976807,1.78019766693714,
6.05922613165351));
#31242=CARTESIAN_POINT('Ctrl Pts',(-0.2127471920983,1.76856716225692,6.06026790748401));
#31243=CARTESIAN_POINT('Ctrl Pts',(-0.194856456788532,1.75836298320027,
6.06130968331451));
#31244=CARTESIAN_POINT('Ctrl Pts',(-0.176927050248394,1.74813674757903,
6.0623537109671));
#31245=CARTESIAN_POINT('Ctrl Pts',(-0.158221431665553,1.73934330603197,
6.0633977386197));
#31246=CARTESIAN_POINT('Ctrl Pts',(-0.138995727778631,1.7320800662382,6.0644417662723));
#31247=CARTESIAN_POINT('Ctrl Pts',(-0.132195848319658,1.72951115352792,
6.06481102516816));
#31248=CARTESIAN_POINT('Ctrl Pts',(-0.125331054137186,1.72713320588977,
6.06518028406403));
#31249=CARTESIAN_POINT('Ctrl Pts',(-0.118413061807564,1.72494902107399,
6.06554954295989));
#31250=CARTESIAN_POINT('Ctrl Pts',(-0.098854628228644,1.7187739298614,6.06659350560744));
#31251=CARTESIAN_POINT('Ctrl Pts',(-0.0787535838382332,1.71411447998649,
6.067637468255));
#31252=CARTESIAN_POINT('Ctrl Pts',(-0.058369433768079,1.71105540342924,
6.06868143090255));
#31253=CARTESIAN_POINT('Ctrl Pts',(-0.0380227825384923,1.70800195437295,
6.06972347306832));
#31254=CARTESIAN_POINT('Ctrl Pts',(-0.0173947699898787,1.70654320156851,
6.07076551523409));
#31255=CARTESIAN_POINT('Ctrl Pts',(0.00324284852386898,1.7067133692414,
6.07180755739986));
#31256=CARTESIAN_POINT('Ctrl Pts',(0.0238583025595397,1.70688335415688,
6.07284848042871));
#31257=CARTESIAN_POINT('Ctrl Pts',(0.0444826098181244,1.70867880938727,
6.07388940345757));
#31258=CARTESIAN_POINT('Ctrl Pts',(0.0648420140908806,1.71208196328523,
6.07493032648642));
#31259=CARTESIAN_POINT('Ctrl Pts',(0.0852118744230393,1.71548686495434,
6.07597178410621));
#31260=CARTESIAN_POINT('Ctrl Pts',(0.105315831609809,1.72050100939405,6.077013241726));
#31261=CARTESIAN_POINT('Ctrl Pts',(0.124887816480819,1.7270550666725,6.0780546993458));
#31262=CARTESIAN_POINT('Ctrl Pts',(0.144465781446479,1.73361112650118,6.07909647517629));
#31263=CARTESIAN_POINT('Ctrl Pts',(0.163510764894453,1.74170776809457,6.08013825100679));
#31264=CARTESIAN_POINT('Ctrl Pts',(0.181775199633076,1.75122691216443,6.08118002683729));
#31265=CARTESIAN_POINT('Ctrl Pts',(0.200079113361855,1.76076663208022,6.08222405448989));
#31266=CARTESIAN_POINT('Ctrl Pts',(0.217598485783747,1.77173460230041,6.08326808214248));
#31267=CARTESIAN_POINT('Ctrl Pts',(0.234112768746594,1.78396819541413,6.08431210979508));
#31268=CARTESIAN_POINT('Ctrl Pts',(0.239953654165408,1.78829505694353,6.08468136869095));
#31269=CARTESIAN_POINT('Ctrl Pts',(0.245669112245223,1.79277987277877,6.08505062758681));
#31270=CARTESIAN_POINT('Ctrl Pts',(0.251250448193061,1.79741430588545,6.08541988648268));
#31271=CARTESIAN_POINT('Ctrl Pts',(0.267029908940553,1.81051669857012,6.08646384913023));
#31272=CARTESIAN_POINT('Ctrl Pts',(0.281828716351315,1.82489577218219,6.08750781177779));
#31273=CARTESIAN_POINT('Ctrl Pts',(0.295435151442728,1.84037919711238,6.08855177442534));
#31274=CARTESIAN_POINT('Ctrl Pts',(0.309016556030614,1.85583413861398,6.08959381659111));
#31275=CARTESIAN_POINT('Ctrl Pts',(0.321409417423752,1.87238889164568,6.09063585875688));
#31276=CARTESIAN_POINT('Ctrl Pts',(0.332437853197238,1.88983348563196,6.09167790092265));
#31277=CARTESIAN_POINT('Ctrl Pts',(0.343454444603954,1.90725934439834,6.0927188239515));
#31278=CARTESIAN_POINT('Ctrl Pts',(0.353109103876376,1.9255725435649,6.09375974698036));
#31279=CARTESIAN_POINT('Ctrl Pts',(0.361268584551529,1.94453328389609,6.09480067000921));
#31280=CARTESIAN_POINT('Ctrl Pts',(0.369432255723295,1.96350376196933,6.095842127629));
#31281=CARTESIAN_POINT('Ctrl Pts',(0.376098908583875,1.98312177610599,6.09688358524879));
#31282=CARTESIAN_POINT('Ctrl Pts',(0.3811828089318,2.003126081039,6.09792504286859));
#31283=CARTESIAN_POINT('Ctrl Pts',(0.38626826263292,2.02313649815927,6.09896681869908));
#31284=CARTESIAN_POINT('Ctrl Pts',(0.389769855077223,2.04353271962256,6.10000859452958));
#31285=CARTESIAN_POINT('Ctrl Pts',(0.391652856850279,2.06404266804928,6.10105037036008));
#31286=CARTESIAN_POINT('Ctrl Pts',(0.3935399287744,2.08459694919495,6.10209439801268));
#31287=CARTESIAN_POINT('Ctrl Pts',(0.393801415885455,2.10526471165969,6.10313842566527));
#31288=CARTESIAN_POINT('Ctrl Pts',(0.392454671522441,2.12577248145237,6.10418245331787));
#31289=CARTESIAN_POINT('Ctrl Pts',(0.391978345694036,2.13302581081726,6.10455171221374));
#31290=CARTESIAN_POINT('Ctrl Pts',(0.391301312972275,2.14025918214962,6.1049209711096));
#31291=CARTESIAN_POINT('Ctrl Pts',(0.390425876636419,2.14746077172448,6.10529023000547));
#31292=CARTESIAN_POINT('Ctrl Pts',(0.387950857496259,2.16782098674792,6.10633419265302));
#31293=CARTESIAN_POINT('Ctrl Pts',(0.383871536803702,2.18804774134201,6.10737815530058));
#31294=CARTESIAN_POINT('Ctrl Pts',(0.378218205068872,2.20786973326416,6.10842211794813));
#31295=CARTESIAN_POINT('Ctrl Pts',(0.372575273246948,2.22765526049623,6.1094641601139));
#31296=CARTESIAN_POINT('Ctrl Pts',(0.365364220292138,2.24703678718359,6.11050620227967));
#31297=CARTESIAN_POINT('Ctrl Pts',(0.356666384889145,2.26575276736787,6.11154824444544));
#31298=CARTESIAN_POINT('Ctrl Pts',(0.347977890824735,2.28444864688345,6.11258916747429));
#31299=CARTESIAN_POINT('Ctrl Pts',(0.33780606659172,2.30247972286781,6.11363009050315));
#31300=CARTESIAN_POINT('Ctrl Pts',(0.326280410962804,2.31960415165006,6.114671013532));
#31301=CARTESIAN_POINT('Ctrl Pts',(0.314748836057552,2.33673737509262,6.11571247115179));
#31302=CARTESIAN_POINT('Ctrl Pts',(0.30186243817519,2.35296240170731,6.11675392877158));
#31303=CARTESIAN_POINT('Ctrl Pts',(0.28779446754134,2.36806572785904,6.11779538639138));
#31304=CARTESIAN_POINT('Ctrl Pts',(0.27372219852915,2.38317366873536,6.11883716222187));
#31305=CARTESIAN_POINT('Ctrl Pts',(0.258468165600901,2.39715871357079,6.11987893805237));
#31306=CARTESIAN_POINT('Ctrl Pts',(0.242242336629156,2.4098443808502,6.12092071388287));
#31307=CARTESIAN_POINT('Ctrl Pts',(0.225981435159879,2.42255746848731,6.12196474153547));
#31308=CARTESIAN_POINT('Ctrl Pts',(0.208745158133959,2.43396516479699,6.12300876918806));
#31309=CARTESIAN_POINT('Ctrl Pts',(0.190772841055458,2.4439340243646,6.12405279684066));
#31310=CARTESIAN_POINT('Ctrl Pts',(0.184416268081496,2.44745987932431,6.12442205573653));
#31311=CARTESIAN_POINT('Ctrl Pts',(0.177967829910699,2.45080617269093,6.12479131463239));
#31312=CARTESIAN_POINT('Ctrl Pts',(0.171438714949408,2.45396844070693,6.12516057352826));
#31313=CARTESIAN_POINT('Ctrl Pts',(0.152979709039263,2.46290875257812,6.12620453617581));
#31314=CARTESIAN_POINT('Ctrl Pts',(0.133764481629443,2.47042789443814,6.12724849882337));
#31315=CARTESIAN_POINT('Ctrl Pts',(0.114037545303458,2.4764044742842,6.12829246147092));
#31316=CARTESIAN_POINT('Ctrl Pts',(0.0943468988025437,2.48237005956761,
6.12933450363669));
#31317=CARTESIAN_POINT('Ctrl Pts',(0.0741470908896119,2.48679844773158,
6.13037654580246));
#31318=CARTESIAN_POINT('Ctrl Pts',(0.0537020641890218,2.48961645024542,
6.13141858796823));
#31319=CARTESIAN_POINT('Ctrl Pts',(0.0332789951259194,2.49243142626882,
6.13245951099708));
#31320=CARTESIAN_POINT('Ctrl Pts',(0.0126119513524283,2.49363932156465,
6.13350043402594));
#31321=CARTESIAN_POINT('Ctrl Pts',(-0.00802562061735804,2.49321810667072,
6.13454135705479));
#31322=CARTESIAN_POINT('Ctrl Pts',(-0.0286737915062241,2.4927966754518,
6.13558281467458));
#31323=CARTESIAN_POINT('Ctrl Pts',(-0.0492917243991184,2.49074446146345,
6.13662427229437));
#31324=CARTESIAN_POINT('Ctrl Pts',(-0.0696061181394477,2.48709156322188,
6.13766572991417));
#31325=CARTESIAN_POINT('Ctrl Pts',(-0.0899267188126951,2.48343754886064,
6.13870750574466));
#31326=CARTESIAN_POINT('Ctrl Pts',(-0.109942878550889,2.47818204232365,
6.13974928157516));
#31327=CARTESIAN_POINT('Ctrl Pts',(-0.129392549133005,2.47140605572454,
6.14079105740566));
#31328=CARTESIAN_POINT('Ctrl Pts',(-0.148884260619454,2.46461542267663,
6.14183508505826));
#31329=CARTESIAN_POINT('Ctrl Pts',(-0.167806364118297,2.45629804448474,
6.14287911271085));
#31330=CARTESIAN_POINT('Ctrl Pts',(-0.185917099702794,2.44658292231168,
6.14392314036345));
#31331=CARTESIAN_POINT('Ctrl Pts',(-0.192322629487972,2.44314681094249,
6.14429239925932));
#31332=CARTESIAN_POINT('Ctrl Pts',(-0.198626908961687,2.43953625773621,
6.14466165815518));
#31333=CARTESIAN_POINT('Ctrl Pts',(-0.20482012843017,2.43575825379259,6.14503091705105));
#31334=CARTESIAN_POINT('Ctrl Pts',(-0.222329496154477,2.42507714348327,
6.1460748796986));
#31335=CARTESIAN_POINT('Ctrl Pts',(-0.239053275050047,2.41299088359138,
6.14711884234616));
#31336=CARTESIAN_POINT('Ctrl Pts',(-0.25475703746797,2.39963935299046,6.14816280499371));
#31337=CARTESIAN_POINT('Ctrl Pts',(-0.270431911122744,2.3863123839688,6.14920484715948));
#31338=CARTESIAN_POINT('Ctrl Pts',(-0.285089900189208,2.37172519033955,
6.15024688932525));
#31339=CARTESIAN_POINT('Ctrl Pts',(-0.298526589528653,2.3560600815129,6.15128893149102));
#31340=CARTESIAN_POINT('Ctrl Pts',(-0.311948848074838,2.34041179676703,
6.15232985451987));
#31341=CARTESIAN_POINT('Ctrl Pts',(-0.324151912290571,2.32368843188051,
6.15337077754873));
#31342=CARTESIAN_POINT('Ctrl Pts',(-0.334969237870668,2.30610798063235,
6.15441170057758));
#31343=CARTESIAN_POINT('Ctrl Pts',(-0.345792118947249,2.28851850052263,
6.15545315819737));
#31344=CARTESIAN_POINT('Ctrl Pts',(-0.35522744029955,2.27007167288185,6.15649461581716));
#31345=CARTESIAN_POINT('Ctrl Pts',(-0.363152566444587,2.25101358708643,
6.15753607343695));
#31346=CARTESIAN_POINT('Ctrl Pts',(-0.371080114061167,2.23194967821494,
6.15857784926745));
#31347=CARTESIAN_POINT('Ctrl Pts',(-0.377496299003602,2.2122748320806,6.15961962509795));
#31348=CARTESIAN_POINT('Ctrl Pts',(-0.382327386270553,2.19225323684038,
6.16066140092845));
#31349=CARTESIAN_POINT('Ctrl Pts',(-0.387168916042263,2.1721883644677,6.16170542858104));
#31350=CARTESIAN_POINT('Ctrl Pts',(-0.39041839206562,2.1517759739565,6.16274945623364));
#31351=CARTESIAN_POINT('Ctrl Pts',(-0.39205341181135,2.1312891720421,6.16379348388624));
#31352=CARTESIAN_POINT('Ctrl Pts',(-0.392631696863979,2.12404325874091,
6.1641627427821));
#31353=CARTESIAN_POINT('Ctrl Pts',(-0.393008499473629,2.11678804999605,
6.16453200167797));
#31354=CARTESIAN_POINT('Ctrl Pts',(-0.393184387717665,2.10953557838228,
6.16490126057383));
#31355=CARTESIAN_POINT('Ctrl Pts',(-0.393260979184605,2.10637745122671,
6.16506205631473));
#31356=CARTESIAN_POINT('Ctrl Pts',(-0.393299521459542,2.10321839755623,
6.16522285205563));
#31357=CARTESIAN_POINT('Ctrl Pts',(-0.393299995571538,2.10005902057492,
6.16538364779653));
#31358=CARTESIAN_POINT('',(-0.393227355315136,2.10032536725365,6.2903836446444));
#31359=CARTESIAN_POINT('Ctrl Pts',(-0.393299995571548,2.10005902050583,
6.16538364780004));
#31360=CARTESIAN_POINT('Ctrl Pts',(-0.393303061112308,2.07963091419915,
6.16642333141745));
#31361=CARTESIAN_POINT('Ctrl Pts',(-0.391710255539657,2.05913958273797,
6.16746301503486));
#31362=CARTESIAN_POINT('Ctrl Pts',(-0.388518105140135,2.0388561370347,6.16850269865227));
#31363=CARTESIAN_POINT('Ctrl Pts',(-0.385331781825707,2.01860971758312,
6.16954048438763));
#31364=CARTESIAN_POINT('Ctrl Pts',(-0.380551962062052,1.9985711652666,6.170578270123));
#31365=CARTESIAN_POINT('Ctrl Pts',(-0.374227035493721,1.97900819901505,
6.17161605585837));
#31366=CARTESIAN_POINT('Ctrl Pts',(-0.367908708593547,1.95946564550412,
6.17265275872876));
#31367=CARTESIAN_POINT('Ctrl Pts',(-0.360048675288858,1.94039840477248,
6.17368946159915));
#31368=CARTESIAN_POINT('Ctrl Pts',(-0.350745521553215,1.92206049030538,
6.17472616446954));
#31369=CARTESIAN_POINT('Ctrl Pts',(-0.341437353842434,1.90371269253958,
6.17576342607544));
#31370=CARTESIAN_POINT('Ctrl Pts',(-0.330684836323542,1.88609567427874,
6.17680068768135));
#31371=CARTESIAN_POINT('Ctrl Pts',(-0.318633368128757,1.86944053540372,
6.17783794928726));
#31372=CARTESIAN_POINT('Ctrl Pts',(-0.306577526772869,1.85277935281649,
6.17887558728814));
#31373=CARTESIAN_POINT('Ctrl Pts',(-0.293222264163319,1.83708132115032,
6.17991322528903));
#31374=CARTESIAN_POINT('Ctrl Pts',(-0.278753793705845,1.82254511628988,
6.18095086328991));
#31375=CARTESIAN_POINT('Ctrl Pts',(-0.264254735541846,1.80797818052601,
6.18199069495507));
#31376=CARTESIAN_POINT('Ctrl Pts',(-0.248638340683192,1.79457845148889,
6.18303052662022));
#31377=CARTESIAN_POINT('Ctrl Pts',(-0.232124886913118,1.78250523330995,
6.18407035828537));
#31378=CARTESIAN_POINT('Ctrl Pts',(-0.228412750717217,1.77979123835607,
6.18430410688912));
#31379=CARTESIAN_POINT('Ctrl Pts',(-0.224655394221444,1.77714409837398,
6.18453785549287));
#31380=CARTESIAN_POINT('Ctrl Pts',(-0.22085549849512,1.774565307958,6.18477160409662));
#31381=CARTESIAN_POINT('Ctrl Pts',(-0.203884491442143,1.76304797340731,
6.18581556674418));
#31382=CARTESIAN_POINT('Ctrl Pts',(-0.185959571037253,1.75282742121085,
6.18685952939173));
#31383=CARTESIAN_POINT('Ctrl Pts',(-0.167305110205114,1.74405914803263,
6.18790349203929));
#31384=CARTESIAN_POINT('Ctrl Pts',(-0.148684966263819,1.73530700503777,
6.18894553420505));
#31385=CARTESIAN_POINT('Ctrl Pts',(-0.129338578916634,1.72800220127159,
6.18998757637082));
#31386=CARTESIAN_POINT('Ctrl Pts',(-0.109516521935822,1.72225534891533,
6.19102961853659));
#31387=CARTESIAN_POINT('Ctrl Pts',(-0.0897157535328079,1.71651466858821,
6.19207054156545));
#31388=CARTESIAN_POINT('Ctrl Pts',(-0.0694410247200447,1.71232884955851,
6.1931114645943));
#31389=CARTESIAN_POINT('Ctrl Pts',(-0.0489597161328431,1.70975925866692,
6.19415238762315));
#31390=CARTESIAN_POINT('Ctrl Pts',(-0.028467888879353,1.70718834810042,
6.19519384524295));
#31391=CARTESIAN_POINT('Ctrl Pts',(-0.00776999794767176,1.70623543151968,
6.19623530286274));
#31392=CARTESIAN_POINT('Ctrl Pts',(0.0128591766436706,1.70691027541279,
6.19727676048253));
#31393=CARTESIAN_POINT('Ctrl Pts',(0.0334946543472138,1.70758532550014,
6.19831853631303));
#31394=CARTESIAN_POINT('Ctrl Pts',(0.0540606403303332,1.70988906597326,
6.19936031214353));
#31395=CARTESIAN_POINT('Ctrl Pts',(0.0742861215870826,1.71377925723811,
6.20040208797403));
#31396=CARTESIAN_POINT('Ctrl Pts',(0.0945553206805387,1.71767785723965,
6.20144611562662));
#31397=CARTESIAN_POINT('Ctrl Pts',(0.114481835635049,1.72316955848568,6.20249014327922));
#31398=CARTESIAN_POINT('Ctrl Pts',(0.133807783915114,1.73016170159957,6.20353417093182));
#31399=CARTESIAN_POINT('Ctrl Pts',(0.140643118502037,1.73263473096767,6.20390342982768));
#31400=CARTESIAN_POINT('Ctrl Pts',(0.147403511174077,1.73529501761734,6.20427268872355));
#31401=CARTESIAN_POINT('Ctrl Pts',(0.154078243835575,1.73813706354955,6.20464194761942));
#31402=CARTESIAN_POINT('Ctrl Pts',(0.172948937701002,1.7461720488378,6.20568591026697));
#31403=CARTESIAN_POINT('Ctrl Pts',(0.191245644278404,1.75571107327129,6.20672987291453));
#31404=CARTESIAN_POINT('Ctrl Pts',(0.208716162070342,1.76664965323158,6.20777383556208));
#31405=CARTESIAN_POINT('Ctrl Pts',(0.226154540962252,1.77756811049533,6.20881587772785));
#31406=CARTESIAN_POINT('Ctrl Pts',(0.242769099794949,1.78988067709395,6.20985791989362));
#31407=CARTESIAN_POINT('Ctrl Pts',(0.258331193755519,1.80343654248568,6.21089996205939));
#31408=CARTESIAN_POINT('Ctrl Pts',(0.273876574271647,1.81697784909093,6.21194088508825));
#31409=CARTESIAN_POINT('Ctrl Pts',(0.288371162903788,1.83175934460952,6.2129818081171));
#31410=CARTESIAN_POINT('Ctrl Pts',(0.301618623344404,1.8475894295957,6.21402273114595));
#31411=CARTESIAN_POINT('Ctrl Pts',(0.314872887335429,1.86342764450093,6.21506418876575));
#31412=CARTESIAN_POINT('Ctrl Pts',(0.326878259006371,1.88031497081602,6.21610564638554));
#31413=CARTESIAN_POINT('Ctrl Pts',(0.3374777831302,1.8980256553581,6.21714710400533));
#31414=CARTESIAN_POINT('Ctrl Pts',(0.348080545870744,1.91574175128641,6.21818887983583));
#31415=CARTESIAN_POINT('Ctrl Pts',(0.357276259450329,1.93428105686638,6.21923065566632));
#31416=CARTESIAN_POINT('Ctrl Pts',(0.36495373543889,1.95339283445479,6.22027243149682));
#31417=CARTESIAN_POINT('Ctrl Pts',(0.37264780646603,1.97254592258418,6.22131645914942));
#31418=CARTESIAN_POINT('Ctrl Pts',(0.378816868326995,1.99227325024314,6.22236048680201));
#31419=CARTESIAN_POINT('Ctrl Pts',(0.38339923420854,2.01230782698379,6.22340451445461));
#31420=CARTESIAN_POINT('Ctrl Pts',(0.385019956956315,2.01939379416864,6.22377377335048));
#31421=CARTESIAN_POINT('Ctrl Pts',(0.386442663016391,2.0265181145997,6.22414303224634));
#31422=CARTESIAN_POINT('Ctrl Pts',(0.387666173305935,2.03366880014403,6.22451229114221));
#31423=CARTESIAN_POINT('Ctrl Pts',(0.391125261375264,2.05388510013373,6.22555625378976));
#31424=CARTESIAN_POINT('Ctrl Pts',(0.393009016712081,2.07443294490035,6.22660021643731));
#31425=CARTESIAN_POINT('Ctrl Pts',(0.393268769785939,2.09504372003876,6.22764417908486));
#31426=CARTESIAN_POINT('Ctrl Pts',(0.393528045016027,2.11561657943536,6.22868622125063));
#31427=CARTESIAN_POINT('Ctrl Pts',(0.392169179473157,2.13625141274911,6.2297282634164));
#31428=CARTESIAN_POINT('Ctrl Pts',(0.389195207792429,2.15667433485633,6.23077030558217));
#31429=CARTESIAN_POINT('Ctrl Pts',(0.386224430110566,2.17707532306606,6.23181122861102));
#31430=CARTESIAN_POINT('Ctrl Pts',(0.381642066752141,2.19726412331353,6.23285215163988));
#31431=CARTESIAN_POINT('Ctrl Pts',(0.37550293757078,2.21697193627411,6.23389307466873));
#31432=CARTESIAN_POINT('Ctrl Pts',(0.369360655492676,2.23668987065379,6.23493453228852));
#31433=CARTESIAN_POINT('Ctrl Pts',(0.361660213778556,2.25592561697248,6.23597598990831));
#31434=CARTESIAN_POINT('Ctrl Pts',(0.352506467046164,2.27442500018814,6.23701744752811));
#31435=CARTESIAN_POINT('Ctrl Pts',(0.343349923445087,2.29293003577185,6.2380592233586));
#31436=CARTESIAN_POINT('Ctrl Pts',(0.33273954929525,2.31069761748757,6.2391009991891));
#31437=CARTESIAN_POINT('Ctrl Pts',(0.320825980990119,2.32749852729573,6.2401427750196));
#31438=CARTESIAN_POINT('Ctrl Pts',(0.308886661236732,2.34433575265173,6.24118680267219));
#31439=CARTESIAN_POINT('Ctrl Pts',(0.295638995588657,2.36020156922966,6.24223083032479));
#31440=CARTESIAN_POINT('Ctrl Pts',(0.281274082208155,2.37489958289885,6.24327485797739));
#31441=CARTESIAN_POINT('Ctrl Pts',(0.276193400637187,2.38009807767573,6.24364411687325));
#31442=CARTESIAN_POINT('Ctrl Pts',(0.270973280959128,2.38515083778139,6.24401337576912));
#31443=CARTESIAN_POINT('Ctrl Pts',(0.265623164751951,2.39005038242891,6.24438263466499));
#31444=CARTESIAN_POINT('Ctrl Pts',(0.250497404633898,2.40390229408023,6.24542659731255));
#31445=CARTESIAN_POINT('Ctrl Pts',(0.23424011965874,2.41660910894307,6.2464705599601));
#31446=CARTESIAN_POINT('Ctrl Pts',(0.217050819931449,2.42798449897379,6.24751452260765));
#31447=CARTESIAN_POINT('Ctrl Pts',(0.19989314177325,2.43933896274878,6.24855656477342));
#31448=CARTESIAN_POINT('Ctrl Pts',(0.18180742599756,2.4493664123912,6.24959860693919));
#31449=CARTESIAN_POINT('Ctrl Pts',(0.163025602822916,2.45792114051034,6.25064064910496));
#31450=CARTESIAN_POINT('Ctrl Pts',(0.144263951031311,2.46646668098588,6.25168157213382));
#31451=CARTESIAN_POINT('Ctrl Pts',(0.124808330231236,2.47354231019215,6.25272249516267));
#31452=CARTESIAN_POINT('Ctrl Pts',(0.104914426684827,2.47904861571228,6.25376341819153));
#31453=CARTESIAN_POINT('Ctrl Pts',(0.0850103061480592,2.48455774912741,
6.25480487581132));
#31454=CARTESIAN_POINT('Ctrl Pts',(0.0646681580011058,2.4884957369127,6.25584633343111));
#31455=CARTESIAN_POINT('Ctrl Pts',(0.0441584568693738,2.49081315316519,
6.2568877910509));
#31456=CARTESIAN_POINT('Ctrl Pts',(0.0236424891298007,2.49313127748937,
6.2579295668814));
#31457=CARTESIAN_POINT('Ctrl Pts',(0.00295960106099637,2.49382779795452,
6.2589713427119));
#31458=CARTESIAN_POINT('Ctrl Pts',(-0.0176159345037573,2.49290529247079,
6.2600131185424));
#31459=CARTESIAN_POINT('Ctrl Pts',(-0.0382359445555444,2.49198079297053,
6.261057146195));
#31460=CARTESIAN_POINT('Ctrl Pts',(-0.0587474079873671,2.48943037169309,
6.26210117384759));
#31461=CARTESIAN_POINT('Ctrl Pts',(-0.0788817482096687,2.48530839570322,
6.26314520150019));
#31462=CARTESIAN_POINT('Ctrl Pts',(-0.0860030004303546,2.48385050682544,
6.26351446039606));
#31463=CARTESIAN_POINT('Ctrl Pts',(-0.0930771966970507,2.48219648707988,
6.26388371929192));
#31464=CARTESIAN_POINT('Ctrl Pts',(-0.10009293613341,2.48035022562921,6.26425297818779));
#31465=CARTESIAN_POINT('Ctrl Pts',(-0.119927718716834,2.47513050576955,
6.26529694083534));
#31466=CARTESIAN_POINT('Ctrl Pts',(-0.139412198268763,2.4683395179686,6.2663409034829));
#31467=CARTESIAN_POINT('Ctrl Pts',(-0.158281708409268,2.46004415115794,
6.26738486613045));
#31468=CARTESIAN_POINT('Ctrl Pts',(-0.177116506052565,2.45176404456841,
6.26842690829622));
#31469=CARTESIAN_POINT('Ctrl Pts',(-0.19533788998475,2.44198529060657,6.26946895046199));
#31470=CARTESIAN_POINT('Ctrl Pts',(-0.212697798804906,2.43082402630938,
6.27051099262776));
#31471=CARTESIAN_POINT('Ctrl Pts',(-0.230039063355709,2.4196747490347,6.27155191565661));
#31472=CARTESIAN_POINT('Ctrl Pts',(-0.246520058156968,2.40714628066294,
6.27259283868546));
#31473=CARTESIAN_POINT('Ctrl Pts',(-0.261918787875003,2.3933997930437,6.27363376171432));
#31474=CARTESIAN_POINT('Ctrl Pts',(-0.277325425979278,2.37964624558671,
6.27467521933411));
#31475=CARTESIAN_POINT('Ctrl Pts',(-0.291648128967637,2.36467390715421,
6.2757166769539));
#31476=CARTESIAN_POINT('Ctrl Pts',(-0.304698925854026,2.34868344251961,
6.27675813457369));
#31477=CARTESIAN_POINT('Ctrl Pts',(-0.317753710327837,2.33268809210092,
6.27779991040419));
#31478=CARTESIAN_POINT('Ctrl Pts',(-0.329535378233429,2.3156745886114,6.27884168623469));
#31479=CARTESIAN_POINT('Ctrl Pts',(-0.339897628283363,2.29787494102929,
6.27988346206518));
#31480=CARTESIAN_POINT('Ctrl Pts',(-0.350282276571922,2.28003681910502,
6.28092748971778));
#31481=CARTESIAN_POINT('Ctrl Pts',(-0.359241062472394,2.26140982428574,
6.28197151737038));
#31482=CARTESIAN_POINT('Ctrl Pts',(-0.366674313425443,2.24224921045117,
6.28301554502297));
#31483=CARTESIAN_POINT('Ctrl Pts',(-0.369303356854312,2.23547235249049,
6.28338480391884));
#31484=CARTESIAN_POINT('Ctrl Pts',(-0.371742017699808,2.22862889083584,
6.2837540628147));
#31485=CARTESIAN_POINT('Ctrl Pts',(-0.373987394539171,2.22173051682221,
6.28412332171057));
#31486=CARTESIAN_POINT('Ctrl Pts',(-0.381544018087779,2.19851462958019,
6.28536603091604));
#31487=CARTESIAN_POINT('Ctrl Pts',(-0.386944506159296,2.17456429864603,
6.28660874012152));
#31488=CARTESIAN_POINT('Ctrl Pts',(-0.390076693750689,2.15025000490081,
6.28785144932699));
#31489=CARTESIAN_POINT('Ctrl Pts',(-0.39220411762502,2.13373541007154,6.28869551410774));
#31490=CARTESIAN_POINT('Ctrl Pts',(-0.393286023394877,2.11705335145469,
6.28953957888848));
#31491=CARTESIAN_POINT('Ctrl Pts',(-0.393299865350261,2.10032544656516,
6.29038364366923));
#31492=CARTESIAN_POINT('',(-0.393115187231275,2.09978487279504,6.41538365076377));
#31493=CARTESIAN_POINT('Ctrl Pts',(-0.392992974431572,2.10032511088776,
6.29038364779653));
#31494=CARTESIAN_POINT('Ctrl Pts',(-0.392294339636222,2.01048562007843,
6.29492032027548));
#31495=CARTESIAN_POINT('Ctrl Pts',(-0.317093268726177,1.7884251043508,6.30608044059534));
#31496=CARTESIAN_POINT('Ctrl Pts',(0.0520281133013657,1.63786569494271,
6.32386400875615));
#31497=CARTESIAN_POINT('Ctrl Pts',(0.416734555740583,1.89358451963055,6.34373435227894));
#31498=CARTESIAN_POINT('Ctrl Pts',(0.399143776574688,2.33866144662726,6.36360469580175));
#31499=CARTESIAN_POINT('Ctrl Pts',(0.0153929209198437,2.56479898716546,
6.38347503932451));
#31500=CARTESIAN_POINT('Ctrl Pts',(-0.330203906139794,2.39085715588212,
6.40073468998947));
#31501=CARTESIAN_POINT('Ctrl Pts',(-0.392376313660633,2.17936284500731,
6.41137089281346));
#31502=CARTESIAN_POINT('Ctrl Pts',(-0.392770159222556,2.09978512047867,
6.41538364779653));
#31503=CARTESIAN_POINT('',(-0.393299932545456,2.09976965300128,6.54038364779198));
#31504=CARTESIAN_POINT('Ctrl Pts',(-0.393299941092297,2.09978474016666,
6.41538365235266));
#31505=CARTESIAN_POINT('Ctrl Pts',(-0.393287381153227,2.07683655136687,
6.41653927342683));
#31506=CARTESIAN_POINT('Ctrl Pts',(-0.391262216182739,2.05396047902279,
6.41769489450101));
#31507=CARTESIAN_POINT('Ctrl Pts',(-0.38728651038287,2.03148687078042,6.41885051557518));
#31508=CARTESIAN_POINT('Ctrl Pts',(-0.383279315437034,2.00883526276493,
6.42001528962056));
#31509=CARTESIAN_POINT('Ctrl Pts',(-0.377290759060769,1.98659292679144,
6.42118006366594));
#31510=CARTESIAN_POINT('Ctrl Pts',(-0.369433581160785,1.96507884113039,
6.42234483771131));
#31511=CARTESIAN_POINT('Ctrl Pts',(-0.36747533951717,1.95971689323994,6.42263513393091));
#31512=CARTESIAN_POINT('Ctrl Pts',(-0.365401256312991,1.95440007141614,
6.4229254301505));
#31513=CARTESIAN_POINT('Ctrl Pts',(-0.363213523926563,1.94913308501581,
6.4232157263701));
#31514=CARTESIAN_POINT('Ctrl Pts',(-0.355346005371014,1.9301919597239,6.42425968901765));
#31515=CARTESIAN_POINT('Ctrl Pts',(-0.345969422449791,1.91181147682915,
6.42530365166521));
#31516=CARTESIAN_POINT('Ctrl Pts',(-0.335186020749563,1.89424475342273,
6.42634761431276));
#31517=CARTESIAN_POINT('Ctrl Pts',(-0.324422456278741,1.87671034589693,
6.42738965647853));
#31518=CARTESIAN_POINT('Ctrl Pts',(-0.312257539988718,1.85998737746704,
6.4284316986443));
#31519=CARTESIAN_POINT('Ctrl Pts',(-0.298840051230804,1.84430581981521,
6.42947374081007));
#31520=CARTESIAN_POINT('Ctrl Pts',(-0.285436972645028,1.82864110390995,
6.43051466383893));
#31521=CARTESIAN_POINT('Ctrl Pts',(-0.270784446168001,1.81401615340673,
6.43155558686778));
#31522=CARTESIAN_POINT('Ctrl Pts',(-0.255072324634896,1.80062899404694,
6.43259650989664));
#31523=CARTESIAN_POINT('Ctrl Pts',(-0.239352133765684,1.78723495939101,
6.43363796751643));
#31524=CARTESIAN_POINT('Ctrl Pts',(-0.222571810292413,1.77508047531464,
6.43467942513622));
#31525=CARTESIAN_POINT('Ctrl Pts',(-0.204955708274494,1.76432449054824,
6.43572088275601));
#31526=CARTESIAN_POINT('Ctrl Pts',(-0.187334223769412,1.75356521935957,
6.43676265858651));
#31527=CARTESIAN_POINT('Ctrl Pts',(-0.168877098645611,1.74420565036361,
6.43780443441701));
#31528=CARTESIAN_POINT('Ctrl Pts',(-0.149834075832615,1.73635918859486,
6.43884621024751));
#31529=CARTESIAN_POINT('Ctrl Pts',(-0.130749891093668,1.72849576652095,
6.43989023790011));
#31530=CARTESIAN_POINT('Ctrl Pts',(-0.111077981232955,1.72215220732753,
6.4409342655527));
#31531=CARTESIAN_POINT('Ctrl Pts',(-0.0910847798190486,1.71739256033721,
6.4419782932053));
#31532=CARTESIAN_POINT('Ctrl Pts',(-0.0840134465449763,1.71570913558503,
6.44234755210116));
#31533=CARTESIAN_POINT('Ctrl Pts',(-0.0769020075508997,1.71422338002955,
6.44271681099702));
#31534=CARTESIAN_POINT('Ctrl Pts',(-0.069762440055462,1.712936578895,6.44308606989289));
#31535=CARTESIAN_POINT('Ctrl Pts',(-0.0495775728297026,1.70929855599466,
6.44413003254044));
#31536=CARTESIAN_POINT('Ctrl Pts',(-0.0290472199612253,1.70723286729158,
6.44517399518799));
#31537=CARTESIAN_POINT('Ctrl Pts',(-0.00843955421571544,1.70679055972085,
6.44621795783555));
#31538=CARTESIAN_POINT('Ctrl Pts',(0.012130201508055,1.70634906582256,6.44726000000132));
#31539=CARTESIAN_POINT('Ctrl Pts',(0.0327762617722319,1.70752510026857,
6.44830204216709));
#31540=CARTESIAN_POINT('Ctrl Pts',(0.0532247253178052,1.7103180545434,6.44934408433286));
#31541=CARTESIAN_POINT('Ctrl Pts',(0.0736512275347659,1.7131080092292,6.45038500736171));
#31542=CARTESIAN_POINT('Ctrl Pts',(0.0938798251049557,1.71751136587206,
6.45142593039057));
#31543=CARTESIAN_POINT('Ctrl Pts',(0.113641243669386,1.72347568772087,6.45246685341942));
#31544=CARTESIAN_POINT('Ctrl Pts',(0.133412811183346,1.72944307268992,6.45350831103921));
#31545=CARTESIAN_POINT('Ctrl Pts',(0.152716011310585,1.73697282725947,6.454549768659));
#31546=CARTESIAN_POINT('Ctrl Pts',(0.171295750206517,1.74596235233921,6.45559122627879));
#31547=CARTESIAN_POINT('Ctrl Pts',(0.189881166022688,1.75495462411077,6.45663300210929));
#31548=CARTESIAN_POINT('Ctrl Pts',(0.207742034540402,1.76540720156411,6.45767477793979));
#31549=CARTESIAN_POINT('Ctrl Pts',(0.224647812415882,1.77717148456687,6.45871655377029));
#31550=CARTESIAN_POINT('Ctrl Pts',(0.241590132513881,1.7889611963343,6.45976058142289));
#31551=CARTESIAN_POINT('Ctrl Pts',(0.257572670917688,1.80206780714636,6.46080460907548));
#31552=CARTESIAN_POINT('Ctrl Pts',(0.272397348505266,1.81630196594389,6.46184863672808));
#31553=CARTESIAN_POINT('Ctrl Pts',(0.277640642649778,1.82133640133274,6.46221789562395));
#31554=CARTESIAN_POINT('Ctrl Pts',(0.28273944294546,1.82651156023687,6.46258715451981));
#31555=CARTESIAN_POINT('Ctrl Pts',(0.287686185267906,1.83181806771149,6.46295641341568));
#31556=CARTESIAN_POINT('Ctrl Pts',(0.301671533405767,1.84682053794165,6.46400037606323));
#31557=CARTESIAN_POINT('Ctrl Pts',(0.314521852419824,1.86296463159717,6.46504433871078));
#31558=CARTESIAN_POINT('Ctrl Pts',(0.326049054369466,1.8800524968435,6.46608830135834));
#31559=CARTESIAN_POINT('Ctrl Pts',(0.337555050788995,1.8971089271204,6.46713034352411));
#31560=CARTESIAN_POINT('Ctrl Pts',(0.347742305442243,1.91510511294071,6.46817238568987));
#31561=CARTESIAN_POINT('Ctrl Pts',(0.356463062279352,1.93381042382139,6.46921442785564));
#31562=CARTESIAN_POINT('Ctrl Pts',(0.365174453160618,1.95249564549204,6.4702553508845));
#31563=CARTESIAN_POINT('Ctrl Pts',(0.372422137428226,1.97188782902399,6.47129627391335));
#31564=CARTESIAN_POINT('Ctrl Pts',(0.378104441765347,1.99173217875419,6.4723371969422));
#31565=CARTESIAN_POINT('Ctrl Pts',(0.383789664385877,2.01158672002519,6.47337865456199));
#31566=CARTESIAN_POINT('Ctrl Pts',(0.387907682943764,2.03189318850659,6.47442011218178));
#31567=CARTESIAN_POINT('Ctrl Pts',(0.390406677683765,2.05238155798512,6.47546156980157));
#31568=CARTESIAN_POINT('Ctrl Pts',(0.392906435975606,2.07287618755374,6.47650334563207));
#31569=CARTESIAN_POINT('Ctrl Pts',(0.393786132559946,2.09355209463284,6.47754512146257));
#31570=CARTESIAN_POINT('Ctrl Pts',(0.393045915811025,2.11413499431456,6.47858689729306));
#31571=CARTESIAN_POINT('Ctrl Pts',(0.392304099066804,2.13476238440103,6.47963092494566));
#31572=CARTESIAN_POINT('Ctrl Pts',(0.389935462854378,2.15529563410243,6.48067495259825));
#31573=CARTESIAN_POINT('Ctrl Pts',(0.385991993126678,2.17546569579679,6.48171898025085));
#31574=CARTESIAN_POINT('Ctrl Pts',(0.384597239573994,2.18259958223403,6.48208823914672));
#31575=CARTESIAN_POINT('Ctrl Pts',(0.383005946038878,2.18968815183762,6.48245749804259));
#31576=CARTESIAN_POINT('Ctrl Pts',(0.381221900545541,2.19671996972935,6.48282675693847));
#31577=CARTESIAN_POINT('Ctrl Pts',(0.376178076612252,2.21660020905579,6.48387071958602));
#31578=CARTESIAN_POINT('Ctrl Pts',(0.369559943489457,2.2361440769609,6.48491468223358));
#31579=CARTESIAN_POINT('Ctrl Pts',(0.361432043141268,2.25508632496364,6.48595864488113));
#31580=CARTESIAN_POINT('Ctrl Pts',(0.3533190949416,2.27399372666004,6.4870006870469));
#31581=CARTESIAN_POINT('Ctrl Pts',(0.343702124709039,2.29230101332403,6.48804272921268));
#31582=CARTESIAN_POINT('Ctrl Pts',(0.332695067663452,2.30975910457573,6.48908477137845));
#31583=CARTESIAN_POINT('Ctrl Pts',(0.321699832024213,2.32719844611168,6.4901256944073));
#31584=CARTESIAN_POINT('Ctrl Pts',(0.309317839356789,2.34378976814962,6.49116661743616));
#31585=CARTESIAN_POINT('Ctrl Pts',(0.295708288813132,2.35930965644806,6.49220754046502));
#31586=CARTESIAN_POINT('Ctrl Pts',(0.282091748759025,2.37483751535663,6.49324899808481));
#31587=CARTESIAN_POINT('Ctrl Pts',(0.267246864338255,2.38929227739429,6.4942904557046));
#31588=CARTESIAN_POINT('Ctrl Pts',(0.251372627455732,2.40248420151473,6.4953319133244));
#31589=CARTESIAN_POINT('Ctrl Pts',(0.235493540301784,2.41568015634311,6.4963736891549));
#31590=CARTESIAN_POINT('Ctrl Pts',(0.218585063096429,2.4276120630735,6.4974154649854));
#31591=CARTESIAN_POINT('Ctrl Pts',(0.200877899818762,2.43813157108499,6.4984572408159));
#31592=CARTESIAN_POINT('Ctrl Pts',(0.183132462105845,2.44867381725176,6.49950126846849));
#31593=CARTESIAN_POINT('Ctrl Pts',(0.164585552541311,2.45779724459101,6.50054529612109));
#31594=CARTESIAN_POINT('Ctrl Pts',(0.145491532118493,2.46539992348359,6.50158932377369));
#31595=CARTESIAN_POINT('Ctrl Pts',(0.138738227374833,2.46808889135378,6.50195858266955));
#31596=CARTESIAN_POINT('Ctrl Pts',(0.131916635192529,2.47058807406696,6.50232784156541));
#31597=CARTESIAN_POINT('Ctrl Pts',(0.125038420747888,2.47289446675551,6.50269710046126));
#31598=CARTESIAN_POINT('Ctrl Pts',(0.105592446547591,2.47941506204636,6.50374106310882));
#31599=CARTESIAN_POINT('Ctrl Pts',(0.0855770974506221,2.48442986605543,
6.50478502575637));
#31600=CARTESIAN_POINT('Ctrl Pts',(0.0652503368603409,2.4878495630262,6.50582898840393));
#31601=CARTESIAN_POINT('Ctrl Pts',(0.0449609695365006,2.4912629690959,6.5068710305697));
#31602=CARTESIAN_POINT('Ctrl Pts',(0.0243620353742315,2.49308691340133,
6.50791307273547));
#31603=CARTESIAN_POINT('Ctrl Pts',(0.00372464080977932,2.49328236300505,
6.50895511490124));
#31604=CARTESIAN_POINT('Ctrl Pts',(-0.0168905895171121,2.49347760269898,
6.50999603793009));
#31605=CARTESIAN_POINT('Ctrl Pts',(-0.0375434665032679,2.49204778397756,
6.51103696095895));
#31606=CARTESIAN_POINT('Ctrl Pts',(-0.0579599620768663,2.48900582617237,
6.5120778839878));
#31607=CARTESIAN_POINT('Ctrl Pts',(-0.0783869430304766,2.48596230609694,
6.51311934160759));
#31608=CARTESIAN_POINT('Ctrl Pts',(-0.0985765699223359,2.48130508535941,
6.51416079922739));
#31609=CARTESIAN_POINT('Ctrl Pts',(-0.11826158716983,2.4750987696595,6.51520225684718));
#31610=CARTESIAN_POINT('Ctrl Pts',(-0.137952619048288,2.46889055765958,
6.51624403267768));
#31611=CARTESIAN_POINT('Ctrl Pts',(-0.157138044088684,2.4611325639985,6.51728580850818));
#31612=CARTESIAN_POINT('Ctrl Pts',(-0.175568242200381,2.45193846384087,
6.51832758433868));
#31613=CARTESIAN_POINT('Ctrl Pts',(-0.19403827760353,2.4427244904271,6.51937161199128));
#31614=CARTESIAN_POINT('Ctrl Pts',(-0.211749195928382,2.43206859286288,
6.52041563964387));
#31615=CARTESIAN_POINT('Ctrl Pts',(-0.228477602724462,2.42012946608096,
6.52145966729647));
#31616=CARTESIAN_POINT('Ctrl Pts',(-0.234394220936296,2.41590675343341,
6.52182892619233));
#31617=CARTESIAN_POINT('Ctrl Pts',(-0.24018822961454,2.4115238893501,6.52219818508819));
#31618=CARTESIAN_POINT('Ctrl Pts',(-0.245850787641983,2.406989055531,6.52256744398405));
#31619=CARTESIAN_POINT('Ctrl Pts',(-0.261656045743758,2.39433148652912,
6.52359811459743));
#31620=CARTESIAN_POINT('Ctrl Pts',(-0.276534058619568,2.38040754097505,
6.52462878521081));
#31621=CARTESIAN_POINT('Ctrl Pts',(-0.290272920650004,2.36537995692463,
6.52565945582419));
#31622=CARTESIAN_POINT('Ctrl Pts',(-0.30398645661347,2.35038007455716,6.52668822651071));
#31623=CARTESIAN_POINT('Ctrl Pts',(-0.316564456390915,2.33428109815806,
6.52771699719724));
#31624=CARTESIAN_POINT('Ctrl Pts',(-0.327829832865636,2.31728435443743,
6.52874576788376));
#31625=CARTESIAN_POINT('Ctrl Pts',(-0.339091623489328,2.30029302090358,
6.52977421110511));
#31626=CARTESIAN_POINT('Ctrl Pts',(-0.349041161188116,2.28240508741081,
6.53080265432646));
#31627=CARTESIAN_POINT('Ctrl Pts',(-0.35754306959627,2.26385311526998,6.53183109754781));
#31628=CARTESIAN_POINT('Ctrl Pts',(-0.366042502827262,2.24530654420094,
6.53285924135648));
#31629=CARTESIAN_POINT('Ctrl Pts',(-0.373094836165821,2.22609700970157,
6.53388738516516));
#31630=CARTESIAN_POINT('Ctrl Pts',(-0.378612195223621,2.20647861582473,
6.53491552897383));
#31631=CARTESIAN_POINT('Ctrl Pts',(-0.384140211372701,2.1868223279098,6.53594565870046));
#31632=CARTESIAN_POINT('Ctrl Pts',(-0.388127154582712,2.16675634147602,
6.53697578842708));
#31633=CARTESIAN_POINT('Ctrl Pts',(-0.390535836004804,2.14654729633425,
6.53800591815371));
#31634=CARTESIAN_POINT('Ctrl Pts',(-0.392389063178822,2.1309985603021,6.5387984946998));
#31635=CARTESIAN_POINT('Ctrl Pts',(-0.393309066661416,2.11536545937624,
6.53959107124589));
#31636=CARTESIAN_POINT('Ctrl Pts',(-0.393299932545456,2.09976965300128,
6.54038364779198));
#31637=CARTESIAN_POINT('',(-0.39331152360305,2.10034122134638,6.66538365352491));
#31638=CARTESIAN_POINT('Ctrl Pts',(-0.393299932545403,2.09976965291168,
6.54038364779653));
#31639=CARTESIAN_POINT('Ctrl Pts',(-0.393292041506276,2.08629631066401,
6.5410683610333));
#31640=CARTESIAN_POINT('Ctrl Pts',(-0.392591866303222,2.07284347841698,
6.54175307427007));
#31641=CARTESIAN_POINT('Ctrl Pts',(-0.391205367932869,2.05946297864287,
6.54243778750684));
#31642=CARTESIAN_POINT('Ctrl Pts',(-0.389091413606023,2.0390621141358,6.54348175015438));
#31643=CARTESIAN_POINT('Ctrl Pts',(-0.385371045251637,2.01876626928969,
6.54452571280192));
#31644=CARTESIAN_POINT('Ctrl Pts',(-0.380069742571046,1.998847240364,6.54556967544945));
#31645=CARTESIAN_POINT('Ctrl Pts',(-0.374778192207985,1.97896485463841,
6.54661171761521));
#31646=CARTESIAN_POINT('Ctrl Pts',(-0.367911610004776,1.95945862716396,
6.54765375978097));
#31647=CARTESIAN_POINT('Ctrl Pts',(-0.359546688657205,1.94059150375329,
6.54869580194672));
#31648=CARTESIAN_POINT('Ctrl Pts',(-0.351190751103754,1.92174464333676,
6.54973672497556));
#31649=CARTESIAN_POINT('Ctrl Pts',(-0.341339939305365,1.90353620528506,
6.5507776480044));
#31650=CARTESIAN_POINT('Ctrl Pts',(-0.330119447510008,1.88621028935964,
6.55181857103324));
#31651=CARTESIAN_POINT('Ctrl Pts',(-0.318893193162514,1.86887547529539,
6.55286002865302));
#31652=CARTESIAN_POINT('Ctrl Pts',(-0.306296239941186,1.85242471517439,
6.5539014862728));
#31653=CARTESIAN_POINT('Ctrl Pts',(-0.292498028718581,1.83707454821615,
6.55494294389258));
#31654=CARTESIAN_POINT('Ctrl Pts',(-0.278695601540899,1.82171969111268,
6.55598471972306));
#31655=CARTESIAN_POINT('Ctrl Pts',(-0.263691704047982,1.80746661917585,
6.55702649555355));
#31656=CARTESIAN_POINT('Ctrl Pts',(-0.24769314483582,1.79449550575918,6.55806827138403));
#31657=CARTESIAN_POINT('Ctrl Pts',(-0.231660004374866,1.7814963549865,6.55911229903662));
#31658=CARTESIAN_POINT('Ctrl Pts',(-0.214628516710658,1.76978511215146,
6.5601563266892));
#31659=CARTESIAN_POINT('Ctrl Pts',(-0.196835615836783,1.75949944150097,
6.56120035434178));
#31660=CARTESIAN_POINT('Ctrl Pts',(-0.190542500021145,1.75586153461305,
6.56156961323773));
#31661=CARTESIAN_POINT('Ctrl Pts',(-0.184154352532472,1.75240153377129,
6.56193887213368));
#31662=CARTESIAN_POINT('Ctrl Pts',(-0.177682280947023,1.74912410023277,
6.56230813102963));
#31663=CARTESIAN_POINT('Ctrl Pts',(-0.159384547130388,1.73985819430176,
6.56335209367719));
#31664=CARTESIAN_POINT('Ctrl Pts',(-0.140305534785827,1.73199983908709,
6.56439605632475));
#31665=CARTESIAN_POINT('Ctrl Pts',(-0.120687567697363,1.72567473902595,
6.5654400189723));
#31666=CARTESIAN_POINT('Ctrl Pts',(-0.101105689973313,1.71936127466793,
6.56648206113807));
#31667=CARTESIAN_POINT('Ctrl Pts',(-0.0809874996476068,1.71457574653924,
6.56752410330385));
#31668=CARTESIAN_POINT('Ctrl Pts',(-0.0605956014093857,1.71139600736761,
6.56856614546962));
#31669=CARTESIAN_POINT('Ctrl Pts',(-0.0402256037495277,1.7082196831859,
6.56960706849847));
#31670=CARTESIAN_POINT('Ctrl Pts',(-0.0195832006051351,1.70664586559583,
6.57064799152733));
#31671=CARTESIAN_POINT('Ctrl Pts',(0.00105859466534771,1.70670142464365,
6.57168891455618));
#31672=CARTESIAN_POINT('Ctrl Pts',(0.021710991023893,1.70675701222515,6.57273037217598));
#31673=CARTESIAN_POINT('Ctrl Pts',(0.0423620430658482,1.70844366233467,
6.57377182979577));
#31674=CARTESIAN_POINT('Ctrl Pts',(0.0627379593325417,1.71173612264494,
6.57481328741556));
#31675=CARTESIAN_POINT('Ctrl Pts',(0.083120101329971,1.71502958894537,6.57585506324606));
#31676=CARTESIAN_POINT('Ctrl Pts',(0.103226220223315,1.71992968921717,6.57689683907656));
#31677=CARTESIAN_POINT('Ctrl Pts',(0.122792873801231,1.72636006618185,6.57793861490706));
#31678=CARTESIAN_POINT('Ctrl Pts',(0.142401821144877,1.73280434255225,6.57898264255966));
#31679=CARTESIAN_POINT('Ctrl Pts',(0.161468295815427,1.74078521496365,6.58002667021226));
#31680=CARTESIAN_POINT('Ctrl Pts',(0.17974829059745,1.75017798521635,6.58107069786486));
#31681=CARTESIAN_POINT('Ctrl Pts',(0.186213685141952,1.75350008493649,6.58143995676071));
#31682=CARTESIAN_POINT('Ctrl Pts',(0.192580935459323,1.75699839274605,6.58180921565656));
#31683=CARTESIAN_POINT('Ctrl Pts',(0.198840109549427,1.76066609241873,6.58217847455242));
#31684=CARTESIAN_POINT('Ctrl Pts',(0.216535943090567,1.77103535231666,6.58322243719997));
#31685=CARTESIAN_POINT('Ctrl Pts',(0.233471202972059,1.78282345782475,6.58426639984752));
#31686=CARTESIAN_POINT('Ctrl Pts',(0.249409020409639,1.79589470484994,6.58531036249508));
#31687=CARTESIAN_POINT('Ctrl Pts',(0.265317518514646,1.80894190590772,6.58635240466085));
#31688=CARTESIAN_POINT('Ctrl Pts',(0.28023161618312,1.8232671476923,6.58739444682662));
#31689=CARTESIAN_POINT('Ctrl Pts',(0.293943700784461,1.83869177056752,6.58843648899239));
#31690=CARTESIAN_POINT('Ctrl Pts',(0.307641058822351,1.85409982764009,6.58947741202125));
#31691=CARTESIAN_POINT('Ctrl Pts',(0.320138458636934,1.87060439389482,6.5905183350501));
#31692=CARTESIAN_POINT('Ctrl Pts',(0.331265520348259,1.88799046005333,6.59155925807896));
#31693=CARTESIAN_POINT('Ctrl Pts',(0.342398296628475,1.9053854552423,6.59260071569875));
#31694=CARTESIAN_POINT('Ctrl Pts',(0.352158918629106,1.92366224372364,6.59364217331854));
#31695=CARTESIAN_POINT('Ctrl Pts',(0.360420410695364,1.94257694719583,6.59468363093834));
#31696=CARTESIAN_POINT('Ctrl Pts',(0.368684427007619,1.96149742993454,6.59572540676884));
#31697=CARTESIAN_POINT('Ctrl Pts',(0.375448140417293,1.98105552750404,6.59676718259934));
#31698=CARTESIAN_POINT('Ctrl Pts',(0.380633147462184,2.00098839940173,6.59780895842984));
#31699=CARTESIAN_POINT('Ctrl Pts',(0.385829362017467,2.02096435665437,6.59885298608243));
#31700=CARTESIAN_POINT('Ctrl Pts',(0.389439928849869,2.04131598037234,6.59989701373503));
#31701=CARTESIAN_POINT('Ctrl Pts',(0.391437610923698,2.06177060353148,6.60094104138763));
#31702=CARTESIAN_POINT('Ctrl Pts',(0.392144164888067,2.06900513562849,6.60131030028349));
#31703=CARTESIAN_POINT('Ctrl Pts',(0.39264943269245,2.07625253092481,6.60167955917935));
#31704=CARTESIAN_POINT('Ctrl Pts',(0.392953769170832,2.08350074867042,6.6020488180752));
#31705=CARTESIAN_POINT('Ctrl Pts',(0.393814184232686,2.10399279008812,6.60309278072275));
#31706=CARTESIAN_POINT('Ctrl Pts',(0.393069896237303,2.1246133743209,6.60413674337031));
#31707=CARTESIAN_POINT('Ctrl Pts',(0.390706786262966,2.14508987877634,6.60518070601786));
#31708=CARTESIAN_POINT('Ctrl Pts',(0.388348023484066,2.16552871449537,6.60622274818363));
#31709=CARTESIAN_POINT('Ctrl Pts',(0.384376374255578,2.18582326706139,6.6072647903494));
#31710=CARTESIAN_POINT('Ctrl Pts',(0.378829674330109,2.20570226036819,6.60830683251517));
#31711=CARTESIAN_POINT('Ctrl Pts',(0.373288931473224,2.22555990394846,6.60934775554402));
#31712=CARTESIAN_POINT('Ctrl Pts',(0.366176664995522,2.24500216140303,6.61038867857287));
#31713=CARTESIAN_POINT('Ctrl Pts',(0.357581428840274,2.26376938587095,6.61142960160173));
#31714=CARTESIAN_POINT('Ctrl Pts',(0.348981778395756,2.28254624869622,6.61247105922152));
#31715=CARTESIAN_POINT('Ctrl Pts',(0.338897928458248,2.30064671027781,6.6135125168413));
#31716=CARTESIAN_POINT('Ctrl Pts',(0.327466202053937,2.31783199148052,6.6145539744611));
#31717=CARTESIAN_POINT('Ctrl Pts',(0.316030982758827,2.33502252353586,6.61559575029159));
#31718=CARTESIAN_POINT('Ctrl Pts',(0.303247504427968,2.35129672647759,6.61663752612209));
#31719=CARTESIAN_POINT('Ctrl Pts',(0.289294326851198,2.36644639695765,6.61767930195259));
#31720=CARTESIAN_POINT('Ctrl Pts',(0.275310989164459,2.38162881379424,6.61872332960518));
#31721=CARTESIAN_POINT('Ctrl Pts',(0.260153444624358,2.39568134468094,6.61976735725778));
#31722=CARTESIAN_POINT('Ctrl Pts',(0.244036212647197,2.40843348864352,6.62081138491038));
#31723=CARTESIAN_POINT('Ctrl Pts',(0.238335758957439,2.41294375481123,6.62118064380625));
#31724=CARTESIAN_POINT('Ctrl Pts',(0.232515529823981,2.41729173905392,6.62154990270212));
#31725=CARTESIAN_POINT('Ctrl Pts',(0.226585841403053,2.42147122184679,6.621919161598));
#31726=CARTESIAN_POINT('Ctrl Pts',(0.209821524301329,2.43328738652312,6.62296312424555));
#31727=CARTESIAN_POINT('Ctrl Pts',(0.192080471339188,2.44382387068611,6.62400708689311));
#31728=CARTESIAN_POINT('Ctrl Pts',(0.17358426564602,2.45292122735836,6.62505104954066));
#31729=CARTESIAN_POINT('Ctrl Pts',(0.155122085716303,2.46200184846271,6.62609309170643));
#31730=CARTESIAN_POINT('Ctrl Pts',(0.135908137066768,2.46964822268475,6.6271351338722));
#31731=CARTESIAN_POINT('Ctrl Pts',(0.116190994681086,2.47574531634475,6.62817717603797));
#31732=CARTESIAN_POINT('Ctrl Pts',(0.0964950281965777,2.48183586182195,
6.62921809906682));
#31733=CARTESIAN_POINT('Ctrl Pts',(0.0762976316722112,2.4863801860862,6.63025902209567));
#31734=CARTESIAN_POINT('Ctrl Pts',(0.0558650566870586,2.48931219534116,
6.63129994512453));
#31735=CARTESIAN_POINT('Ctrl Pts',(0.0354219880639309,2.49224571039965,
6.63234140274432));
#31736=CARTESIAN_POINT('Ctrl Pts',(0.0147442257137023,2.49356513573576,
6.63338286036411));
#31737=CARTESIAN_POINT('Ctrl Pts',(-0.0058936664742866,2.49325583873032,
6.6344243179839));
#31738=CARTESIAN_POINT('Ctrl Pts',(-0.0265378644380765,2.49294644722117,
6.6354660938144));
#31739=CARTESIAN_POINT('Ctrl Pts',(-0.0471414334543857,2.4910073898688,
6.6365078696449));
#31740=CARTESIAN_POINT('Ctrl Pts',(-0.0674326547797886,2.4874760987072,
6.6375496454754));
#31741=CARTESIAN_POINT('Ctrl Pts',(-0.0877677360405539,2.48393717457962,
6.63859367312799));
#31742=CARTESIAN_POINT('Ctrl Pts',(-0.107788408351039,2.47879932862586,
6.63963770078059));
#31743=CARTESIAN_POINT('Ctrl Pts',(-0.12723518820322,2.47215063735387,6.64068172843319));
#31744=CARTESIAN_POINT('Ctrl Pts',(-0.134113259333297,2.46979908240039,
6.64105098732905));
#31745=CARTESIAN_POINT('Ctrl Pts',(-0.140919717527131,2.46725897197108,
6.64142024622492));
#31746=CARTESIAN_POINT('Ctrl Pts',(-0.14764374897517,2.46453561333367,6.64178950512078));
#31747=CARTESIAN_POINT('Ctrl Pts',(-0.166653819555366,2.4568361788036,6.64283346776834));
#31748=CARTESIAN_POINT('Ctrl Pts',(-0.185116636617798,2.44762277309,6.64387743041589));
#31749=CARTESIAN_POINT('Ctrl Pts',(-0.202778187337366,2.43699539572548,
6.64492139306345));
#31750=CARTESIAN_POINT('Ctrl Pts',(-0.220407247731244,2.42638756856678,
6.64596343522922));
#31751=CARTESIAN_POINT('Ctrl Pts',(-0.2372373136588,2.41437125705591,6.64700547739499));
#31752=CARTESIAN_POINT('Ctrl Pts',(-0.253037104612386,2.40109319768035,
6.64804751956077));
#31753=CARTESIAN_POINT('Ctrl Pts',(-0.268819926838699,2.38782939873197,
6.64908844258962));
#31754=CARTESIAN_POINT('Ctrl Pts',(-0.283574091725867,2.37330699094726,
6.65012936561848));
#31755=CARTESIAN_POINT('Ctrl Pts',(-0.297099899635937,2.35771406565478,
6.65117028864734));
#31756=CARTESIAN_POINT('Ctrl Pts',(-0.31063265404842,2.34211313224227,6.65221174626713));
#31757=CARTESIAN_POINT('Ctrl Pts',(-0.322935296878158,2.32544112821049,
6.65325320388693));
#31758=CARTESIAN_POINT('Ctrl Pts',(-0.333846898362626,2.30792099089235,
6.65429466150672));
#31759=CARTESIAN_POINT('Ctrl Pts',(-0.344761833817051,2.29039550040844,
6.65533643733722));
#31760=CARTESIAN_POINT('Ctrl Pts',(-0.354284523868938,2.27202200390388,
6.65637821316772));
#31761=CARTESIAN_POINT('Ctrl Pts',(-0.362299355777202,2.25304922999945,
6.65741998899822));
#31762=CARTESIAN_POINT('Ctrl Pts',(-0.370331511926516,2.23403544601368,
6.65846401665082));
#31763=CARTESIAN_POINT('Ctrl Pts',(-0.376849070730866,2.2144204974274,6.65950804430342));
#31764=CARTESIAN_POINT('Ctrl Pts',(-0.381785625383631,2.19447024002526,
6.66055207195602));
#31765=CARTESIAN_POINT('Ctrl Pts',(-0.383531620057107,2.18741409548544,
6.66092133085188));
#31766=CARTESIAN_POINT('Ctrl Pts',(-0.385080308534198,2.18031609589856,
6.66129058974773));
#31767=CARTESIAN_POINT('Ctrl Pts',(-0.386430299550126,2.17318820662921,
6.66165984864358));
#31768=CARTESIAN_POINT('Ctrl Pts',(-0.390968303877209,2.14922775654797,
6.6629011150279));
#31769=CARTESIAN_POINT('Ctrl Pts',(-0.393278597173609,2.1248326289864,6.66414238141221));
#31770=CARTESIAN_POINT('Ctrl Pts',(-0.393299851891308,2.10034132429566,
6.66538364779653));
#31771=CARTESIAN_POINT('',(-0.393058384114589,2.10004747884629,6.79038363519587));
#31772=CARTESIAN_POINT('Ctrl Pts',(-0.393482223946032,2.10033971569951,
6.66538373730318));
#31773=CARTESIAN_POINT('Ctrl Pts',(-0.392510478521912,1.99409483509794,
6.67076588892424));
#31774=CARTESIAN_POINT('Ctrl Pts',(-0.29321797659763,1.75550278257759,6.68277148838622));
#31775=CARTESIAN_POINT('Ctrl Pts',(0.110368293424312,1.64823249309944,6.70140053568915));
#31776=CARTESIAN_POINT('Ctrl Pts',(0.439598559880011,1.94824972278144,6.72127087921195));
#31777=CARTESIAN_POINT('Ctrl Pts',(0.365556993585621,2.38747717287657,6.74114122273472));
#31778=CARTESIAN_POINT('Ctrl Pts',(-0.0438333482327071,2.56298345334063,
6.76101156625752));
#31779=CARTESIAN_POINT('Ctrl Pts',(-0.348798170201786,2.35711399190874,
6.77742569677967));
#31780=CARTESIAN_POINT('Ctrl Pts',(-0.392724778002082,2.16290283319788,
6.7872163794609));
#31781=CARTESIAN_POINT('Ctrl Pts',(-0.392657736298662,2.10004784536838,
6.7903836143012));
#31782=CARTESIAN_POINT('',(-0.393299834087712,2.0996387430578,6.91538364779653));
#31783=CARTESIAN_POINT('Ctrl Pts',(-0.393299997160818,2.10004725781296,
6.79038364779653));
#31784=CARTESIAN_POINT('Ctrl Pts',(-0.393302581849858,2.07853635562221,
6.79146580267118));
#31785=CARTESIAN_POINT('Ctrl Pts',(-0.391536095407621,2.05705308860708,
6.79254795754583));
#31786=CARTESIAN_POINT('Ctrl Pts',(-0.388039837948008,2.03589091979069,
6.79363011242049));
#31787=CARTESIAN_POINT('Ctrl Pts',(-0.384537910187648,2.0146944297428,6.7947140223557));
#31788=CARTESIAN_POINT('Ctrl Pts',(-0.379300790769184,1.99382070473038,
6.79579793229092));
#31789=CARTESIAN_POINT('Ctrl Pts',(-0.372418383116233,1.97355065078423,
6.79688184222614));
#31790=CARTESIAN_POINT('Ctrl Pts',(-0.365513477736801,1.95321433657679,
6.79796929532684));
#31791=CARTESIAN_POINT('Ctrl Pts',(-0.356952812209818,1.9334862275484,6.79905674842755));
#31792=CARTESIAN_POINT('Ctrl Pts',(-0.346874149351669,1.91462682364604,
6.80014420152825));
#31793=CARTESIAN_POINT('Ctrl Pts',(-0.344995647239727,1.91111173136057,
6.8003468854532));
#31794=CARTESIAN_POINT('Ctrl Pts',(-0.343064534298844,1.90762673863315,
6.80054956937815));
#31795=CARTESIAN_POINT('Ctrl Pts',(-0.341081867415064,1.90417341926936,
6.80075225330309));
#31796=CARTESIAN_POINT('Ctrl Pts',(-0.330869759228678,1.8863864318366,6.80179621595065));
#31797=CARTESIAN_POINT('Ctrl Pts',(-0.319232124137762,1.86934742047409,
6.8028401785982));
#31798=CARTESIAN_POINT('Ctrl Pts',(-0.306302562791849,1.85329444670388,
6.80388414124575));
#31799=CARTESIAN_POINT('Ctrl Pts',(-0.293396786767268,1.83727100410872,
6.80492618341152));
#31800=CARTESIAN_POINT('Ctrl Pts',(-0.27920421202316,1.82223060239925,6.80596822557729));
#31801=CARTESIAN_POINT('Ctrl Pts',(-0.263901652210097,1.8083824285802,6.80701026774306));
#31802=CARTESIAN_POINT('Ctrl Pts',(-0.248615527105874,1.79454912748228,
6.80805119077191));
#31803=CARTESIAN_POINT('Ctrl Pts',(-0.232222306929764,1.78190602495015,
6.80909211380076));
#31804=CARTESIAN_POINT('Ctrl Pts',(-0.214935483346197,1.77062539867389,
6.81013303682962));
#31805=CARTESIAN_POINT('Ctrl Pts',(-0.197639781700593,1.75933897896198,
6.81117449444941));
#31806=CARTESIAN_POINT('Ctrl Pts',(-0.179450167183249,1.74941684901224,
6.8122159520692));
#31807=CARTESIAN_POINT('Ctrl Pts',(-0.160609383812146,1.74098813970638,
6.81325740968899));
#31808=CARTESIAN_POINT('Ctrl Pts',(-0.141762843760332,1.73255685506237,
6.81429918551949));
#31809=CARTESIAN_POINT('Ctrl Pts',(-0.122265424613192,1.72562016664315,
6.81534096134999));
#31810=CARTESIAN_POINT('Ctrl Pts',(-0.102379262085259,1.72025880300542,
6.81638273718049));
#31811=CARTESIAN_POINT('Ctrl Pts',(-0.082450115165751,1.71488585065851,
6.81742676483308));
#31812=CARTESIAN_POINT('Ctrl Pts',(-0.0621312712786171,1.71109515627656,
6.81847079248568));
#31813=CARTESIAN_POINT('Ctrl Pts',(-0.0416951454928683,1.70891637103769,
6.81951482013828));
#31814=CARTESIAN_POINT('Ctrl Pts',(-0.034467155674026,1.70814576325767,
6.81988407903415));
#31815=CARTESIAN_POINT('Ctrl Pts',(-0.0272245202219977,1.70757631980235,
6.82025333793002));
#31816=CARTESIAN_POINT('Ctrl Pts',(-0.0199792825574456,1.70720779250539,
6.82062259682589));
#31817=CARTESIAN_POINT('Ctrl Pts',(0.000504333623478286,1.70616589822218,
6.82166655947345));
#31818=CARTESIAN_POINT('Ctrl Pts',(0.0211307016035394,1.70672750544539,
6.822710522121));
#31819=CARTESIAN_POINT('Ctrl Pts',(0.0416273345470524,1.70890914736022,
6.82375448476855));
#31820=CARTESIAN_POINT('Ctrl Pts',(0.0620862617256241,1.71108677590967,
6.82479652693432));
#31821=CARTESIAN_POINT('Ctrl Pts',(0.0824151979246268,1.71487850565568,
6.82583856910009));
#31822=CARTESIAN_POINT('Ctrl Pts',(0.102342542541241,1.72024890522055,6.82688061126586));
#31823=CARTESIAN_POINT('Ctrl Pts',(0.122248485502793,1.72561353706064,6.82792153429472));
#31824=CARTESIAN_POINT('Ctrl Pts',(0.1417529787668,1.73255331024823,6.82896245732357));
#31825=CARTESIAN_POINT('Ctrl Pts',(0.160595601271428,1.74098197419591,6.83000338035242));
#31826=CARTESIAN_POINT('Ctrl Pts',(0.179447900855871,1.74941496688571,6.83104483797221));
#31827=CARTESIAN_POINT('Ctrl Pts',(0.197636972370958,1.75933809222245,6.832086295592));
#31828=CARTESIAN_POINT('Ctrl Pts',(0.214922838536312,1.77061714756913,6.83312775321179));
#31829=CARTESIAN_POINT('Ctrl Pts',(0.232213986287385,1.78189964915895,6.83416952904229));
#31830=CARTESIAN_POINT('Ctrl Pts',(0.248600783387758,1.79453847348784,6.83521130487279));
#31831=CARTESIAN_POINT('Ctrl Pts',(0.263873453022812,1.80835691198004,6.83625308070329));
#31832=CARTESIAN_POINT('Ctrl Pts',(0.279179134879864,1.82220521934062,6.83729710835588));
#31833=CARTESIAN_POINT('Ctrl Pts',(0.293365375920581,1.83723769571488,6.83834113600848));
#31834=CARTESIAN_POINT('Ctrl Pts',(0.306259781704422,1.85324134035386,6.83938516366108));
#31835=CARTESIAN_POINT('Ctrl Pts',(0.310820364013487,1.85890161969085,6.83975442255694));
#31836=CARTESIAN_POINT('Ctrl Pts',(0.315219731702494,1.86468310722222,6.84012368145281));
#31837=CARTESIAN_POINT('Ctrl Pts',(0.31945157411294,1.8705755422873,6.84049294034868));
#31838=CARTESIAN_POINT('Ctrl Pts',(0.331415769034932,1.88723453731743,6.84153690299623));
#31839=CARTESIAN_POINT('Ctrl Pts',(0.342108985308859,1.904881564955,6.84258086564378));
#31840=CARTESIAN_POINT('Ctrl Pts',(0.351369819488892,1.92329646310177,6.84362482829134));
#31841=CARTESIAN_POINT('Ctrl Pts',(0.360613617366539,1.94167748505908,6.84466687045711));
#31842=CARTESIAN_POINT('Ctrl Pts',(0.368429883592596,1.96082295041602,6.84570891262288));
#31843=CARTESIAN_POINT('Ctrl Pts',(0.374701387190005,1.98048531287793,6.84675095478865));
#31844=CARTESIAN_POINT('Ctrl Pts',(0.380966155291075,2.00012655827145,6.8477918778175));
#31845=CARTESIAN_POINT('Ctrl Pts',(0.385689204370225,2.02028291004397,6.84883280084636));
#31846=CARTESIAN_POINT('Ctrl Pts',(0.388802084839317,2.04068871250259,6.84987372387521));
#31847=CARTESIAN_POINT('Ctrl Pts',(0.391916564002687,2.06110499484952,6.850915181495));
#31848=CARTESIAN_POINT('Ctrl Pts',(0.393419095618887,2.08177025888781,6.8519566391148));
#31849=CARTESIAN_POINT('Ctrl Pts',(0.393292615629937,2.1024100811112,6.85299809673459));
#31850=CARTESIAN_POINT('Ctrl Pts',(0.393166096995836,2.1230562097001,6.85403987256509));
#31851=CARTESIAN_POINT('Ctrl Pts',(0.3914096165708,2.1436761460759,6.85508164839559));
#31852=CARTESIAN_POINT('Ctrl Pts',(0.388058198109005,2.16399785059197,6.85612342422609));
#31853=CARTESIAN_POINT('Ctrl Pts',(0.384699535480151,2.18436348093351,6.85716745187868));
#31854=CARTESIAN_POINT('Ctrl Pts',(0.379739228801881,2.20442887747746,6.85821147953128));
#31855=CARTESIAN_POINT('Ctrl Pts',(0.373263052691939,2.22393378673749,6.85925550718388));
#31856=CARTESIAN_POINT('Ctrl Pts',(0.370972514089987,2.23083241747718,6.85962476607974));
#31857=CARTESIAN_POINT('Ctrl Pts',(0.368492793081253,2.23766110826359,6.85999402497561));
#31858=CARTESIAN_POINT('Ctrl Pts',(0.365829100939446,2.24440899870104,6.86036328387147));
#31859=CARTESIAN_POINT('Ctrl Pts',(0.358298354539635,2.26348652302173,6.86140724651902));
#31860=CARTESIAN_POINT('Ctrl Pts',(0.349248848926038,2.28203022564207,6.86245120916658));
#31861=CARTESIAN_POINT('Ctrl Pts',(0.338778329731138,2.29978521793311,6.86349517181413));
#31862=CARTESIAN_POINT('Ctrl Pts',(0.328327072184561,2.31750754800262,6.8645372139799));
#31863=CARTESIAN_POINT('Ctrl Pts',(0.316460308263824,2.33444339092523,6.86557925614567));
#31864=CARTESIAN_POINT('Ctrl Pts',(0.303322720079523,2.35036017551432,6.86662129831144));
#31865=CARTESIAN_POINT('Ctrl Pts',(0.290199241458535,2.36625986572681,6.86766222134029));
#31866=CARTESIAN_POINT('Ctrl Pts',(0.275808091807768,2.38114208737248,6.86870314436915));
#31867=CARTESIAN_POINT('Ctrl Pts',(0.260335586191335,2.39480548258541,6.869744067398));
#31868=CARTESIAN_POINT('Ctrl Pts',(0.244855134299287,2.408475894962,6.87078552501779));
#31869=CARTESIAN_POINT('Ctrl Pts',(0.228292757809945,2.42092573126836,6.87182698263758));
#31870=CARTESIAN_POINT('Ctrl Pts',(0.210869959837856,2.43199209333654,6.87286844025738));
#31871=CARTESIAN_POINT('Ctrl Pts',(0.193441838441429,2.44306183666079,6.87391021608787));
#31872=CARTESIAN_POINT('Ctrl Pts',(0.175153412157756,2.45274690060954,6.87495199191837));
#31873=CARTESIAN_POINT('Ctrl Pts',(0.156252375783406,2.46092947380623,6.87599376774887));
#31874=CARTESIAN_POINT('Ctrl Pts',(0.137310484390003,2.46912973382057,6.87703779540146));
#31875=CARTESIAN_POINT('Ctrl Pts',(0.117754036085296,2.4758207808622,6.87808182305406));
#31876=CARTESIAN_POINT('Ctrl Pts',(0.0978482880106924,2.48093385585082,
6.87912585070666));
#31877=CARTESIAN_POINT('Ctrl Pts',(0.0908078858363308,2.48274228345338,
6.87949510960252));
#31878=CARTESIAN_POINT('Ctrl Pts',(0.0837238825718224,2.48435378334066,
6.87986436849839));
#31879=CARTESIAN_POINT('Ctrl Pts',(0.0766082307889138,2.48576685831651,
6.88023362739426));
#31880=CARTESIAN_POINT('Ctrl Pts',(0.0564909776705838,2.48976188053396,
6.88127759004181));
#31881=CARTESIAN_POINT('Ctrl Pts',(0.0360004395909989,2.49219093548006,
6.88232155268936));
#31882=CARTESIAN_POINT('Ctrl Pts',(0.015403842950015,2.49299823361228,6.88336551533691));
#31883=CARTESIAN_POINT('Ctrl Pts',(-0.00515486403204175,2.4938040466326,
6.88440755750268));
#31884=CARTESIAN_POINT('Ctrl Pts',(-0.0258185177163293,2.49299393684622,
6.88544959966845));
#31885=CARTESIAN_POINT('Ctrl Pts',(-0.0463132490443797,2.49056366057655,
6.88649164183422));
#31886=CARTESIAN_POINT('Ctrl Pts',(-0.0667859693529384,2.48813599438542,
6.88753256486308));
#31887=CARTESIAN_POINT('Ctrl Pts',(-0.087089397107138,2.48409167357587,
6.88857348789193));
#31888=CARTESIAN_POINT('Ctrl Pts',(-0.106953371297437,2.47847835653854,
6.88961441092078));
#31889=CARTESIAN_POINT('Ctrl Pts',(-0.126827547107173,2.47286215664788,
6.89065586854057));
#31890=CARTESIAN_POINT('Ctrl Pts',(-0.146261106037048,2.46567553530339,
6.89169732616036));
#31891=CARTESIAN_POINT('Ctrl Pts',(-0.164997176752652,2.45701655656798,
6.89273878378016));
#31892=CARTESIAN_POINT('Ctrl Pts',(-0.183738972154671,2.44835493213706,
6.89378055961065));
#31893=CARTESIAN_POINT('Ctrl Pts',(-0.201782202926135,2.43822039598821,
6.89482233544115));
#31894=CARTESIAN_POINT('Ctrl Pts',(-0.218893729483336,2.42675744091432,
6.89586411127165));
#31895=CARTESIAN_POINT('Ctrl Pts',(-0.236042242993499,2.41526970840292,
6.89690813892425));
#31896=CARTESIAN_POINT('Ctrl Pts',(-0.252254453975106,2.40244828118534,
6.89795216657684));
#31897=CARTESIAN_POINT('Ctrl Pts',(-0.267328960078824,2.38847897168281,
6.89899619422944));
#31898=CARTESIAN_POINT('Ctrl Pts',(-0.272660615294824,2.38353821001801,
6.89936545312531));
#31899=CARTESIAN_POINT('Ctrl Pts',(-0.277850292219873,2.37845418724543,
6.89973471202117));
#31900=CARTESIAN_POINT('Ctrl Pts',(-0.282890261841573,2.37323614284206,
6.90010397091704));
#31901=CARTESIAN_POINT('Ctrl Pts',(-0.296955634656005,2.35867380508913,
6.9011344858656));
#31902=CARTESIAN_POINT('Ctrl Pts',(-0.309940758242874,2.34297343956352,
6.90216500081415));
#31903=CARTESIAN_POINT('Ctrl Pts',(-0.321656101468961,2.3263233138406,6.90319551576271));
#31904=CARTESIAN_POINT('Ctrl Pts',(-0.333352706677958,2.3096998190353,6.90422438246193));
#31905=CARTESIAN_POINT('Ctrl Pts',(-0.343783071916386,2.2921301483415,6.90525324916115));
#31906=CARTESIAN_POINT('Ctrl Pts',(-0.352796999717656,2.27383661004006,
6.90628211586036));
#31907=CARTESIAN_POINT('Ctrl Pts',(-0.361801511979625,2.2555621803373,6.90730990785219));
#31908=CARTESIAN_POINT('Ctrl Pts',(-0.36939216422126,2.23656604732395,6.90833769984402));
#31909=CARTESIAN_POINT('Ctrl Pts',(-0.375464363780332,2.21709569390473,
6.90936549183584));
#31910=CARTESIAN_POINT('Ctrl Pts',(-0.381542362665326,2.19760674509447,
6.91039426543255));
#31911=CARTESIAN_POINT('Ctrl Pts',(-0.386098772648862,2.1776433911913,6.91142303902926));
#31912=CARTESIAN_POINT('Ctrl Pts',(-0.389078598302285,2.15746942093956,
6.91245181262597));
#31913=CARTESIAN_POINT('Ctrl Pts',(-0.391909268944431,2.13830525767334,
6.91342909101616));
#31914=CARTESIAN_POINT('Ctrl Pts',(-0.393317573582477,2.11895170160064,
6.91440636940634));
#31915=CARTESIAN_POINT('Ctrl Pts',(-0.393299834087712,2.0996387430578,6.91538364779653));
#31916=CARTESIAN_POINT('',(-0.393445913694928,2.10014151066963,7.04038364779653));
#31917=CARTESIAN_POINT('Ctrl Pts',(-0.393308615227651,2.09963873499208,
6.91538364779653));
#31918=CARTESIAN_POINT('Ctrl Pts',(-0.393587780238266,2.06939755311191,
6.91691387001097));
#31919=CARTESIAN_POINT('Ctrl Pts',(-0.376576601026969,1.9085705283121,6.92506754006631));
#31920=CARTESIAN_POINT('Ctrl Pts',(-0.155638169461425,1.66176284880085,
6.93984465796265));
#31921=CARTESIAN_POINT('Ctrl Pts',(0.284227889761795,1.73191095212428,6.95971500148539));
#31922=CARTESIAN_POINT('Ctrl Pts',(0.463353554261716,2.13973064607486,6.97958534500821));
#31923=CARTESIAN_POINT('Ctrl Pts',(0.217415412616838,2.51110288109078,6.999455688531));
#31924=CARTESIAN_POINT('Ctrl Pts',(-0.227971771668255,2.50534418930942,
7.01932603205377));
#31925=CARTESIAN_POINT('Ctrl Pts',(-0.390179988506806,2.24608553033568,
7.03296868514229));
#31926=CARTESIAN_POINT('Ctrl Pts',(-0.393924158185101,2.10793299234673,
7.03998789038988));
#31927=CARTESIAN_POINT('Ctrl Pts',(-0.393888044763371,2.10014166969089,
7.04038364779653));
#31928=CARTESIAN_POINT('',(-0.393238618660761,2.1002837677798,7.16538364368174));
#31929=CARTESIAN_POINT('Ctrl Pts',(-0.393299974560873,2.10014145817971,
7.04038364779653));
#31930=CARTESIAN_POINT('Ctrl Pts',(-0.393307289300358,2.07980409162154,
7.04141822341494));
#31931=CARTESIAN_POINT('Ctrl Pts',(-0.391732853256908,2.05940230957188,
7.04245279903335));
#31932=CARTESIAN_POINT('Ctrl Pts',(-0.388572870996293,2.03920514885537,
7.04348737465176));
#31933=CARTESIAN_POINT('Ctrl Pts',(-0.385418453513969,2.01904355565545,
7.04452012836629));
#31934=CARTESIAN_POINT('Ctrl Pts',(-0.380684085738039,1.99908661093811,
7.04555288208082));
#31935=CARTESIAN_POINT('Ctrl Pts',(-0.374417843067382,1.97959996348518,
7.04658563579535));
#31936=CARTESIAN_POINT('Ctrl Pts',(-0.3681070857465,1.95997488518286,7.04762572607068));
#31937=CARTESIAN_POINT('Ctrl Pts',(-0.360242731002926,1.9408275735491,7.04866581634602));
#31938=CARTESIAN_POINT('Ctrl Pts',(-0.350925623435377,1.92241594436298,
7.04970590662135));
#31939=CARTESIAN_POINT('Ctrl Pts',(-0.341677524073189,1.90414068297971,
7.05073829335105));
#31940=CARTESIAN_POINT('Ctrl Pts',(-0.330998514642647,1.8865908935706,7.05177068008075));
#31941=CARTESIAN_POINT('Ctrl Pts',(-0.319033892043583,1.86999507455812,
7.05280306681045));
#31942=CARTESIAN_POINT('Ctrl Pts',(-0.306935351581878,1.8532135015369,7.0538470088586));
#31943=CARTESIAN_POINT('Ctrl Pts',(-0.293522685922765,1.83740802937615,
7.05489095090675));
#31944=CARTESIAN_POINT('Ctrl Pts',(-0.278987967121695,1.82278058473241,
7.0559348929549));
#31945=CARTESIAN_POINT('Ctrl Pts',(-0.264453248320622,1.80815314008867,
7.05697883500306));
#31946=CARTESIAN_POINT('Ctrl Pts',(-0.248797112435385,1.7947041855536,7.05802277705121));
#31947=CARTESIAN_POINT('Ctrl Pts',(-0.232245073167206,1.78259313808684,
7.05906671909936));
#31948=CARTESIAN_POINT('Ctrl Pts',(-0.215692707288845,1.77048185164099,
7.06011068174691));
#31949=CARTESIAN_POINT('Ctrl Pts',(-0.198141089577947,1.75963274225577,
7.06115464439446));
#31950=CARTESIAN_POINT('Ctrl Pts',(-0.17980894382752,1.75020915718156,7.06219860704202));
#31951=CARTESIAN_POINT('Ctrl Pts',(-0.161510522034605,1.74080290780756,
7.06324064920779));
#31952=CARTESIAN_POINT('Ctrl Pts',(-0.142435042141189,1.73281736284896,
7.06428269137356));
#31953=CARTESIAN_POINT('Ctrl Pts',(-0.122829002330193,1.72637194138212,
7.06532473353932));
#31954=CARTESIAN_POINT('Ctrl Pts',(-0.103244019097943,1.71993344219667,
7.06636565656818));
#31955=CARTESIAN_POINT('Ctrl Pts',(-0.0831302935632959,1.71503203887742,
7.06740657959703));
#31956=CARTESIAN_POINT('Ctrl Pts',(-0.0627528646893455,1.71173853143367,
7.06844750262589));
#31957=CARTESIAN_POINT('Ctrl Pts',(-0.0423649704990329,1.70844333253034,
7.06948896024568));
#31958=CARTESIAN_POINT('Ctrl Pts',(-0.021713826188412,1.70675781252406,
7.07053041786547));
#31959=CARTESIAN_POINT('Ctrl Pts',(-0.00107369334917631,1.70670146557279,
7.07157187548526));
#31960=CARTESIAN_POINT('Ctrl Pts',(0.0195727459504677,1.70664510140506,
7.07261365131576));
#31961=CARTESIAN_POINT('Ctrl Pts',(0.0402074318264637,1.70821886708768,
7.07365542714626));
#31962=CARTESIAN_POINT('Ctrl Pts',(0.0605580250734511,1.71139014989426,
7.07469720297676));
#31963=CARTESIAN_POINT('Ctrl Pts',(0.0809526065895549,1.7145682875006,7.07574123062935));
#31964=CARTESIAN_POINT('Ctrl Pts',(0.101061153017379,1.71935066571312,7.07678525828195));
#31965=CARTESIAN_POINT('Ctrl Pts',(0.120622661312042,1.72565381853423,7.07782928593455));
#31966=CARTESIAN_POINT('Ctrl Pts',(0.127541310388466,1.7278831610669,7.07819854483041));
#31967=CARTESIAN_POINT('Ctrl Pts',(0.134391697982113,1.73030229809388,7.07856780372628));
#31968=CARTESIAN_POINT('Ctrl Pts',(0.141162917963318,1.73290611474436,7.07893706262215));
#31969=CARTESIAN_POINT('Ctrl Pts',(0.160306399184353,1.7402675821446,7.0799810252697));
#31970=CARTESIAN_POINT('Ctrl Pts',(0.178929532406589,1.74915247762564,7.08102498791726));
#31971=CARTESIAN_POINT('Ctrl Pts',(0.19677657319603,1.75946531712434,7.08206895056481));
#31972=CARTESIAN_POINT('Ctrl Pts',(0.214590782430805,1.7697591850435,7.08311099273058));
#31973=CARTESIAN_POINT('Ctrl Pts',(0.231631073546616,1.78147547029687,7.08415303489635));
#31974=CARTESIAN_POINT('Ctrl Pts',(0.247663602925591,1.79447155650265,7.08519507706212));
#31975=CARTESIAN_POINT('Ctrl Pts',(0.263678913619891,1.80745368511601,7.08623600009097));
#31976=CARTESIAN_POINT('Ctrl Pts',(0.278688024351192,1.82171244748997,7.08727692311983));
#31977=CARTESIAN_POINT('Ctrl Pts',(0.292487934824368,1.8370633194433,7.08831784614868));
#31978=CARTESIAN_POINT('Ctrl Pts',(0.306294932571885,1.85242207520437,7.08935930376847));
#31979=CARTESIAN_POINT('Ctrl Pts',(0.318890985529203,1.86887352465195,7.09040076138827));
#31980=CARTESIAN_POINT('Ctrl Pts',(0.330111239904106,1.8861976162692,7.09144221900806));
#31981=CARTESIAN_POINT('Ctrl Pts',(0.341334922555885,1.90352700115171,7.09248399483856));
#31982=CARTESIAN_POINT('Ctrl Pts',(0.351181600502437,1.92172892228774,7.09352577066905));
#31983=CARTESIAN_POINT('Ctrl Pts',(0.359531272975277,1.94055673813931,7.09456754649955));
#31984=CARTESIAN_POINT('Ctrl Pts',(0.367898993454642,1.95942525074209,7.09561157415215));
#31985=CARTESIAN_POINT('Ctrl Pts',(0.37476300374778,1.97892166434828,7.09665560180474));
#31986=CARTESIAN_POINT('Ctrl Pts',(0.380052197895641,1.99878134127201,7.09769962945734));
#31987=CARTESIAN_POINT('Ctrl Pts',(0.381922916536285,2.00580544868418,7.09806888835321));
#31988=CARTESIAN_POINT('Ctrl Pts',(0.383597101393925,2.0128748998086,7.09843814724907));
#31989=CARTESIAN_POINT('Ctrl Pts',(0.385073149458468,2.01997775580417,7.09880740614494));
#31990=CARTESIAN_POINT('Ctrl Pts',(0.389246208151508,2.04005883288409,7.09985136879249));
#31991=CARTESIAN_POINT('Ctrl Pts',(0.391856667464328,2.06052705119684,7.10089533144004));
#31992=CARTESIAN_POINT('Ctrl Pts',(0.392846373023673,2.0811156889947,7.1019392940876));
#31993=CARTESIAN_POINT('Ctrl Pts',(0.393834257912996,2.10166645177478,7.10298133625337));
#31994=CARTESIAN_POINT('Ctrl Pts',(0.393207212978599,2.12233647054837,7.10402337841914));
#31995=CARTESIAN_POINT('Ctrl Pts',(0.390958568852128,2.14285192459034,7.10506542058491));
#31996=CARTESIAN_POINT('Ctrl Pts',(0.388712339734123,2.16334534535695,7.10610634361376));
#31997=CARTESIAN_POINT('Ctrl Pts',(0.384848019872022,2.1836838001012,7.10714726664261));
#31998=CARTESIAN_POINT('Ctrl Pts',(0.379410872773451,2.20359671626692,7.10818818967147));
#31999=CARTESIAN_POINT('Ctrl Pts',(0.373970933297836,2.22351985918739,7.10922964729126));
#32000=CARTESIAN_POINT('Ctrl Pts',(0.366956731111274,2.24301631288328,7.11027110491105));
#32001=CARTESIAN_POINT('Ctrl Pts',(0.358464051132569,2.26182834747233,7.11131256253084));
#32002=CARTESIAN_POINT('Ctrl Pts',(0.349968776269881,2.28064612995809,7.11235433836134));
#32003=CARTESIAN_POINT('Ctrl Pts',(0.339994459775168,2.29877842187304,7.11339611419184));
#32004=CARTESIAN_POINT('Ctrl Pts',(0.328683523685281,2.31599081290145,7.11443789002234));
#32005=CARTESIAN_POINT('Ctrl Pts',(0.317348138750357,2.33324040890366,7.11548191767494));
#32006=CARTESIAN_POINT('Ctrl Pts',(0.304670817915465,2.34956555261688,7.11652594532753));
#32007=CARTESIAN_POINT('Ctrl Pts',(0.290835582344614,2.36476320371658,7.11756997298013));
#32008=CARTESIAN_POINT('Ctrl Pts',(0.285942240872061,2.37013841370348,7.117939231876));
#32009=CARTESIAN_POINT('Ctrl Pts',(0.280904386306522,2.37537291993756,7.11830849077186));
#32010=CARTESIAN_POINT('Ctrl Pts',(0.27573118930101,2.38045891186883,7.11867774966773));
#32011=CARTESIAN_POINT('Ctrl Pts',(0.261105612225831,2.39483794419938,7.11972171231529));
#32012=CARTESIAN_POINT('Ctrl Pts',(0.245308656591666,2.4081126815382,7.12076567496284));
#32013=CARTESIAN_POINT('Ctrl Pts',(0.228533106806461,2.42008984534563,7.12180963761039));
#32014=CARTESIAN_POINT('Ctrl Pts',(0.21178841745276,2.43204497586961,7.12285167977616));
#32015=CARTESIAN_POINT('Ctrl Pts',(0.194069264831007,2.4427067999076,7.12389372194193));
#32016=CARTESIAN_POINT('Ctrl Pts',(0.175602272059871,2.45192148562913,7.1249357641077));
#32017=CARTESIAN_POINT('Ctrl Pts',(0.157155112548858,2.46112627492295,7.12597668713655));
#32018=CARTESIAN_POINT('Ctrl Pts',(0.137962349487193,2.46888665864025,7.12701761016541));
#32019=CARTESIAN_POINT('Ctrl Pts',(0.118275987079078,2.47509422933507,7.12805853319426));
#32020=CARTESIAN_POINT('Ctrl Pts',(0.0985795142683154,2.48130498807641,
7.12909999081405));
#32021=CARTESIAN_POINT('Ctrl Pts',(0.0783896325466369,2.48596110395713,
7.13014144843385));
#32022=CARTESIAN_POINT('Ctrl Pts',(0.0579748959208028,2.48900360080978,
7.13118290605364));
#32023=CARTESIAN_POINT('Ctrl Pts',(0.0375539217029225,2.49204702727786,
7.13222468188414));
#32024=CARTESIAN_POINT('Ctrl Pts',(0.0169086882702682,2.49347578062839,
7.13326645771463));
#32025=CARTESIAN_POINT('Ctrl Pts',(-0.00368661236477904,2.49328272132052,
7.13430823354513));
#32026=CARTESIAN_POINT('Ctrl Pts',(-0.0243264302095114,2.49308924471057,
7.13535226119773));
#32027=CARTESIAN_POINT('Ctrl Pts',(-0.0449153661678067,2.49126702164157,
7.13639628885033));
#32028=CARTESIAN_POINT('Ctrl Pts',(-0.0651830863183576,2.48786087100662,
7.13744031650292));
#32029=CARTESIAN_POINT('Ctrl Pts',(-0.0723515132713222,2.48665616017402,
7.13780957539879));
#32030=CARTESIAN_POINT('Ctrl Pts',(-0.0794798615381201,2.48525377466167,
7.13817883429465));
#32031=CARTESIAN_POINT('Ctrl Pts',(-0.0865565996283024,2.48365719732697,
7.13854809319052));
#32032=CARTESIAN_POINT('Ctrl Pts',(-0.106563836597748,2.47914338027336,
7.13959205583807));
#32033=CARTESIAN_POINT('Ctrl Pts',(-0.126276650945867,2.47304687232218,
7.14063601848563));
#32034=CARTESIAN_POINT('Ctrl Pts',(-0.145428172932575,2.46542514488947,
7.14167998113318));
#32035=CARTESIAN_POINT('Ctrl Pts',(-0.164544463630889,2.45781743844567,
7.14272202329895));
#32036=CARTESIAN_POINT('Ctrl Pts',(-0.183100813654346,2.44869029566948,
7.14376406546472));
#32037=CARTESIAN_POINT('Ctrl Pts',(-0.200845203256677,2.43815099338725,
7.14480610763049));
#32038=CARTESIAN_POINT('Ctrl Pts',(-0.218570535663357,2.42762301015008,
7.14584703065934));
#32039=CARTESIAN_POINT('Ctrl Pts',(-0.235484994674274,2.41568622726063,
7.1468879536882));
#32040=CARTESIAN_POINT('Ctrl Pts',(-0.251361014938732,2.40249385145647,
7.14792887671705));
#32041=CARTESIAN_POINT('Ctrl Pts',(-0.267245188713404,2.38929470039194,
7.14897033433685));
#32042=CARTESIAN_POINT('Ctrl Pts',(-0.282089282094752,2.37483912600987,
7.15001179195664));
#32043=CARTESIAN_POINT('Ctrl Pts',(-0.295698333728938,2.35932100846235,
7.15105324957643));
#32044=CARTESIAN_POINT('Ctrl Pts',(-0.309311543521694,2.3437981494534,7.15209502540693));
#32045=CARTESIAN_POINT('Ctrl Pts',(-0.321688502812557,2.32721267754762,
7.15313680123742));
#32046=CARTESIAN_POINT('Ctrl Pts',(-0.332674783457099,2.3097912735358,7.15417857706792));
#32047=CARTESIAN_POINT('Ctrl Pts',(-0.343684811196566,2.29233221276386,
7.15522260472052));
#32048=CARTESIAN_POINT('Ctrl Pts',(-0.353297816467056,2.27403426450518,
7.15626663237312));
#32049=CARTESIAN_POINT('Ctrl Pts',(-0.36140514716012,2.25514899163763,7.15731066002571));
#32050=CARTESIAN_POINT('Ctrl Pts',(-0.36427260375736,2.24846951816788,7.15767991892158));
#32051=CARTESIAN_POINT('Ctrl Pts',(-0.366952156627619,2.24171673869915,
7.15804917781744));
#32052=CARTESIAN_POINT('Ctrl Pts',(-0.369440492015627,2.2349022344487,7.15841843671331));
#32053=CARTESIAN_POINT('Ctrl Pts',(-0.377534369956373,2.21273650634965,
7.15961953542616));
#32054=CARTESIAN_POINT('Ctrl Pts',(-0.383641314242097,2.18980835275673,
7.16082063413901));
#32055=CARTESIAN_POINT('Ctrl Pts',(-0.387644613228899,2.16645708265202,
7.16202173285185));
#32056=CARTESIAN_POINT('Ctrl Pts',(-0.391379729877021,2.14467012194525,
7.16314236956002));
#32057=CARTESIAN_POINT('Ctrl Pts',(-0.393283854254901,2.12251519922877,
7.1642630062682));
#32058=CARTESIAN_POINT('Ctrl Pts',(-0.393299897588104,2.1002838259803,7.16538364297637));
#32059=CARTESIAN_POINT('',(-0.393212132698943,2.09972772529158,7.29038365170245));
#32060=CARTESIAN_POINT('Ctrl Pts',(-0.392881147913482,2.10028342826704,
7.16538364779653));
#32061=CARTESIAN_POINT('Ctrl Pts',(-0.392314472383569,2.01503579577097,
7.16968535860972));
#32062=CARTESIAN_POINT('Ctrl Pts',(-0.323128061668355,1.79769261307425,
7.18061051726384));
#32063=CARTESIAN_POINT('Ctrl Pts',(0.0356248266137504,1.63631269996556,
7.19815912375889));
#32064=CARTESIAN_POINT('Ctrl Pts',(0.409160946250237,1.87895167825091,7.21802946728168));
#32065=CARTESIAN_POINT('Ctrl Pts',(0.407347599935112,2.32437239872943,7.23789981080447));
#32066=CARTESIAN_POINT('Ctrl Pts',(0.0318482860476476,2.56396198891753,
7.25777015432726));
#32067=CARTESIAN_POINT('Ctrl Pts',(-0.324479005289757,2.40017195559432,
7.27526476665795));
#32068=CARTESIAN_POINT('Ctrl Pts',(-0.392323111645839,2.18391812223174,
7.2861359311477));
#32069=CARTESIAN_POINT('Ctrl Pts',(-0.392858015080995,2.09972804792847,
7.29038364779653));
#32070=CARTESIAN_POINT('',(-0.393452426999084,2.09984062647883,7.41538364779653));
#32071=CARTESIAN_POINT('Ctrl Pts',(-0.39329990569911,2.09972764532152,7.29038365267059));
#32072=CARTESIAN_POINT('Ctrl Pts',(-0.393283516148222,2.07605994533971,
7.29157644434568));
#32073=CARTESIAN_POINT('Ctrl Pts',(-0.39112659367968,2.05247744071622,7.29276923602077));
#32074=CARTESIAN_POINT('Ctrl Pts',(-0.386899369366362,2.02933340262959,
7.29396202769585));
#32075=CARTESIAN_POINT('Ctrl Pts',(-0.382707066616411,2.00638055997824,
7.29514496558818));
#32076=CARTESIAN_POINT('Ctrl Pts',(-0.376478845323879,1.98385918914853,
7.2963279034805));
#32077=CARTESIAN_POINT('Ctrl Pts',(-0.368329867046097,1.96209423854746,
7.29751084137283));
#32078=CARTESIAN_POINT('Ctrl Pts',(-0.361138256232981,1.94288630244137,
7.29855480402038));
#32079=CARTESIAN_POINT('Ctrl Pts',(-0.352418668001632,1.92418519980553,
7.29959876666793));
#32080=CARTESIAN_POINT('Ctrl Pts',(-0.342264317354093,1.90624751081306,
7.30064272931548));
#32081=CARTESIAN_POINT('Ctrl Pts',(-0.332128646728762,1.88834282013237,
7.30168477148125));
#32082=CARTESIAN_POINT('Ctrl Pts',(-0.320563759413357,1.87119941782039,
7.30272681364702));
#32083=CARTESIAN_POINT('Ctrl Pts',(-0.307710194871082,1.85505240157862,
7.30376885581279));
#32084=CARTESIAN_POINT('Ctrl Pts',(-0.294870434855203,1.83892272697864,
7.30480977884164));
#32085=CARTESIAN_POINT('Ctrl Pts',(-0.280745178513786,1.82378790479044,
7.30585070187049));
#32086=CARTESIAN_POINT('Ctrl Pts',(-0.265517144667215,1.80985256181078,
7.30689162489935));
#32087=CARTESIAN_POINT('Ctrl Pts',(-0.250281290099351,1.79591006200216,
7.30793308251914));
#32088=CARTESIAN_POINT('Ctrl Pts',(-0.233942058489515,1.78316878069185,
7.30897454013893));
#32089=CARTESIAN_POINT('Ctrl Pts',(-0.2167180324914,1.77179551436177,7.31001599775872));
#32090=CARTESIAN_POINT('Ctrl Pts',(-0.199488743802439,1.76041877300299,
7.31105777358922));
#32091=CARTESIAN_POINT('Ctrl Pts',(-0.181374755953678,1.7504112536381,7.31209954941971));
#32092=CARTESIAN_POINT('Ctrl Pts',(-0.1626216378728,1.74189513701212,7.31314132525021));
#32093=CARTESIAN_POINT('Ctrl Pts',(-0.143827984501629,1.7333606126068,7.31418535290281));
#32094=CARTESIAN_POINT('Ctrl Pts',(-0.124393135300646,1.72632417761872,
7.3152293805554));
#32095=CARTESIAN_POINT('Ctrl Pts',(-0.104581087736443,1.72085927930666,
7.316273408208));
#32096=CARTESIAN_POINT('Ctrl Pts',(-0.0975738262041833,1.71892641640616,
7.31664266710387));
#32097=CARTESIAN_POINT('Ctrl Pts',(-0.0905194818952901,1.71718967793619,
7.31701192599975));
#32098=CARTESIAN_POINT('Ctrl Pts',(-0.0834299789834502,1.715650772595,7.31738118489563));
#32099=CARTESIAN_POINT('Ctrl Pts',(-0.0633866535218433,1.71130000484841,
7.31842514754318));
#32100=CARTESIAN_POINT('Ctrl Pts',(-0.0429423609312796,1.70850834598792,
7.31946911019074));
#32101=CARTESIAN_POINT('Ctrl Pts',(-0.0223632973801085,1.70733631065467,
7.32051307283829));
#32102=CARTESIAN_POINT('Ctrl Pts',(-0.00182209123385836,1.7061664314067,
7.32155511500406));
#32103=CARTESIAN_POINT('Ctrl Pts',(0.0188526708402339,1.70661036229058,
7.32259715716983));
#32104=CARTESIAN_POINT('Ctrl Pts',(0.0393872379346304,1.70867719784316,
7.3236391993356));
#32105=CARTESIAN_POINT('Ctrl Pts',(0.0598997512265555,1.71074181364682,
7.32468012236445));
#32106=CARTESIAN_POINT('Ctrl Pts',(0.0802716371868918,1.71442582936336,
7.3257210453933));
#32107=CARTESIAN_POINT('Ctrl Pts',(0.100231932942214,1.71968637991959,7.32676196842215));
#32108=CARTESIAN_POINT('Ctrl Pts',(0.120202479785208,1.72494963215747,7.32780342604194));
#32109=CARTESIAN_POINT('Ctrl Pts',(0.139760298537318,1.73179086484532,7.32884488366174));
#32110=CARTESIAN_POINT('Ctrl Pts',(0.158646820990185,1.74011657972378,7.32988634128152));
#32111=CARTESIAN_POINT('Ctrl Pts',(0.177539114099043,1.74844483847111,7.33092811711202));
#32112=CARTESIAN_POINT('Ctrl Pts',(0.195759044481055,1.75825815271757,7.33196989294252));
#32113=CARTESIAN_POINT('Ctrl Pts',(0.213070949480534,1.76941618235693,7.33301166877302));
#32114=CARTESIAN_POINT('Ctrl Pts',(0.230420274555529,1.78059833033057,7.33405569642561));
#32115=CARTESIAN_POINT('Ctrl Pts',(0.246857070114484,1.79313055010845,7.33509972407821));
#32116=CARTESIAN_POINT('Ctrl Pts',(0.262176673788396,1.80683062622222,7.3361437517308));
#32117=CARTESIAN_POINT('Ctrl Pts',(0.267595016802297,1.81167616356647,7.33651301062667));
#32118=CARTESIAN_POINT('Ctrl Pts',(0.272873941641249,1.81666745465028,7.33688226952254));
#32119=CARTESIAN_POINT('Ctrl Pts',(0.278005556830508,1.82179539836416,7.33725152841841));
#32120=CARTESIAN_POINT('Ctrl Pts',(0.292513574481946,1.83629303608107,7.33829549106596));
#32121=CARTESIAN_POINT('Ctrl Pts',(0.305927716218984,1.85197178795044,7.33933945371351));
#32122=CARTESIAN_POINT('Ctrl Pts',(0.318053003452094,1.86864058913651,7.34038341636107));
#32123=CARTESIAN_POINT('Ctrl Pts',(0.330155984912766,1.88527872626663,7.34142545852684));
#32124=CARTESIAN_POINT('Ctrl Pts',(0.340974342157243,1.90290274419619,7.34246750069261));
#32125=CARTESIAN_POINT('Ctrl Pts',(0.350352242023501,1.92128739129791,7.34350954285838));
#32126=CARTESIAN_POINT('Ctrl Pts',(0.359720070172624,1.93965229357745,7.34455046588723));
#32127=CARTESIAN_POINT('Ctrl Pts',(0.367650153765075,1.95877556431229,7.34559138891609));
#32128=CARTESIAN_POINT('Ctrl Pts',(0.374031857422495,1.97840616942838,7.34663231194494));
#32129=CARTESIAN_POINT('Ctrl Pts',(0.380416838556585,1.99804685631163,7.34767376956473));
#32130=CARTESIAN_POINT('Ctrl Pts',(0.385251608302461,2.01819470335628,7.34871522718453));
#32131=CARTESIAN_POINT('Ctrl Pts',(0.388474814027385,2.03858168948605,7.34975668480432));
#32132=CARTESIAN_POINT('Ctrl Pts',(0.391699004582178,2.05897490472888,7.35079846063482));
#32133=CARTESIAN_POINT('Ctrl Pts',(0.393310571791438,2.07960667272766,7.35184023646532));
#32134=CARTESIAN_POINT('Ctrl Pts',(0.393299947675492,2.10020287546682,7.35288201229582));
#32135=CARTESIAN_POINT('Ctrl Pts',(0.393289300595279,2.12084359736559,7.35392603994841));
#32136=CARTESIAN_POINT('Ctrl Pts',(0.391649520254463,2.14144786637088,7.35497006760101));
#32137=CARTESIAN_POINT('Ctrl Pts',(0.388423029242925,2.16174496217304,7.35601409525361));
#32138=CARTESIAN_POINT('Ctrl Pts',(0.387281861664202,2.16892377890888,7.35638335414947));
#32139=CARTESIAN_POINT('Ctrl Pts',(0.385942672154399,2.17606426947985,7.35675261304534));
#32140=CARTESIAN_POINT('Ctrl Pts',(0.384408841291466,2.18315487199769,7.3571218719412));
#32141=CARTESIAN_POINT('Ctrl Pts',(0.380072420025781,2.20320130624799,7.35816583458876));
#32142=CARTESIAN_POINT('Ctrl Pts',(0.374150762036044,2.22296734847639,7.35920979723631));
#32143=CARTESIAN_POINT('Ctrl Pts',(0.366698972623503,2.24218563034592,7.36025375988386));
#32144=CARTESIAN_POINT('Ctrl Pts',(0.359260891580563,2.26136855811507,7.36129580204963));
#32145=CARTESIAN_POINT('Ctrl Pts',(0.350298474009957,2.28000502593331,7.3623378442154));
#32146=CARTESIAN_POINT('Ctrl Pts',(0.339916760206563,2.29784207371202,7.36337988638117));
#32147=CARTESIAN_POINT('Ctrl Pts',(0.3295461962007,2.31565996478164,7.36442080941003));
#32148=CARTESIAN_POINT('Ctrl Pts',(0.317759705312583,2.33267949303378,7.36546173243888));
#32149=CARTESIAN_POINT('Ctrl Pts',(0.304708472556916,2.34867174498127,7.36650265546773));
#32150=CARTESIAN_POINT('Ctrl Pts',(0.291650537028262,2.36467221013256,7.36754411308752));
#32151=CARTESIAN_POINT('Ctrl Pts',(0.277327014720529,2.37964376475223,7.36858557070731));
#32152=CARTESIAN_POINT('Ctrl Pts',(0.26193005126473,2.39338973779677,7.36962702832711));
#32153=CARTESIAN_POINT('Ctrl Pts',(0.246528383365344,2.40713991083534,7.3706688041576));
#32154=CARTESIAN_POINT('Ctrl Pts',(0.230053193882422,2.41966329420914,7.3717105799881));
#32155=CARTESIAN_POINT('Ctrl Pts',(0.212729786831095,2.43080345795472,7.3727523558186));
#32156=CARTESIAN_POINT('Ctrl Pts',(0.195368934842308,2.44196770141703,7.3737963834712));
#32157=CARTESIAN_POINT('Ctrl Pts',(0.177156853828494,2.45174240785529,7.37484041112379));
#32158=CARTESIAN_POINT('Ctrl Pts',(0.158344134387518,2.46001670114742,7.37588443877639));
#32159=CARTESIAN_POINT('Ctrl Pts',(0.151690322113735,2.46294321022744,7.37625369767226));
#32160=CARTESIAN_POINT('Ctrl Pts',(0.144961542316253,2.4656824722768,7.37662295656812));
#32161=CARTESIAN_POINT('Ctrl Pts',(0.138169346405668,2.46823107108693,7.37699221546399));
#32162=CARTESIAN_POINT('Ctrl Pts',(0.118966562383692,2.47543642752156,7.37803617811154));
#32163=CARTESIAN_POINT('Ctrl Pts',(0.0991414197118359,2.4811571072681,7.3790801407591));
#32164=CARTESIAN_POINT('Ctrl Pts',(0.0789485559701378,2.48529471253864,
7.38012410340665));
#32165=CARTESIAN_POINT('Ctrl Pts',(0.0587928391771958,2.48942470623842,
7.38116614557242));
#32166=CARTESIAN_POINT('Ctrl Pts',(0.0382714447895694,2.49197720184811,
7.38220818773819));
#32167=CARTESIAN_POINT('Ctrl Pts',(0.0176539263884321,2.49290358726165,
7.38325022990396));
#32168=CARTESIAN_POINT('Ctrl Pts',(-0.00294144912182975,2.49382897775181,
7.38429115293281));
#32169=CARTESIAN_POINT('Ctrl Pts',(-0.0236320136864995,2.49313166334946,
7.38533207596166));
#32170=CARTESIAN_POINT('Ctrl Pts',(-0.0441434535668194,2.49081484811506,
7.38637299899052));
#32171=CARTESIAN_POINT('Ctrl Pts',(-0.0646654275880691,2.48849684302473,
7.38741445661031));
#32172=CARTESIAN_POINT('Ctrl Pts',(-0.0850073602035416,2.484557742049,7.3884559142301));
#32173=CARTESIAN_POINT('Ctrl Pts',(-0.104899874976661,2.47905264308521,
7.38949737184989));
#32174=CARTESIAN_POINT('Ctrl Pts',(-0.124798467780291,2.47354586207368,
7.39053914768039));
#32175=CARTESIAN_POINT('Ctrl Pts',(-0.144246670499333,2.46647236148174,
7.39158092351089));
#32176=CARTESIAN_POINT('Ctrl Pts',(-0.162990992885366,2.45793690259352,
7.39262269934139));
#32177=CARTESIAN_POINT('Ctrl Pts',(-0.181775831549595,2.44938299411722,
7.39366672699398));
#32178=CARTESIAN_POINT('Ctrl Pts',(-0.199853108257183,2.4393611755375,7.39471075464658));
#32179=CARTESIAN_POINT('Ctrl Pts',(-0.216993947160994,2.4280221286674,7.39575478229918));
#32180=CARTESIAN_POINT('Ctrl Pts',(-0.223056437203418,2.42401165641885,
7.39612404119505));
#32181=CARTESIAN_POINT('Ctrl Pts',(-0.229002067865071,2.41983678993309,
7.39649330009091));
#32182=CARTESIAN_POINT('Ctrl Pts',(-0.234821713749347,2.41550539258754,
7.39686255898678));
#32183=CARTESIAN_POINT('Ctrl Pts',(-0.251115636933297,2.40337828777207,
7.39789641503299));
#32184=CARTESIAN_POINT('Ctrl Pts',(-0.266520733870789,2.38994591250046,
7.39893027107921));
#32185=CARTESIAN_POINT('Ctrl Pts',(-0.280818729815168,2.37536472356676,
7.39996412712542));
#32186=CARTESIAN_POINT('Ctrl Pts',(-0.295090416083402,2.36081036541131,
7.40099608077791));
#32187=CARTESIAN_POINT('Ctrl Pts',(-0.308258478460216,2.34511187397496,
7.4020280344304));
#32188=CARTESIAN_POINT('Ctrl Pts',(-0.320138146793209,2.32846543932904,
7.40305998808288));
#32189=CARTESIAN_POINT('Ctrl Pts',(-0.332014905654445,2.31182308159251,
7.40409168899768));
#32190=CARTESIAN_POINT('Ctrl Pts',(-0.342603417874453,2.29423382004764,
7.40512338991247));
#32191=CARTESIAN_POINT('Ctrl Pts',(-0.351759479259452,2.2759265720439,7.40615509082726));
#32192=CARTESIAN_POINT('Ctrl Pts',(-0.360912697844894,2.25762500812575,
7.40718647141666));
#32193=CARTESIAN_POINT('Ctrl Pts',(-0.368634018416044,2.23860657620211,
7.40821785200607));
#32194=CARTESIAN_POINT('Ctrl Pts',(-0.374825953099693,2.21912344388451,
7.40924923259547));
#32195=CARTESIAN_POINT('Ctrl Pts',(-0.381031373848938,2.19959787720449,
7.41028285953711));
#32196=CARTESIAN_POINT('Ctrl Pts',(-0.38570054657744,2.17960631464732,7.41131648647874));
#32197=CARTESIAN_POINT('Ctrl Pts',(-0.388786161499595,2.1594155756213,7.41235011342038));
#32198=CARTESIAN_POINT('Ctrl Pts',(-0.391804761525357,2.13966334895605,
7.41336129154576));
#32199=CARTESIAN_POINT('Ctrl Pts',(-0.393308020622564,2.11972120808856,
7.41437246967114));
#32200=CARTESIAN_POINT('Ctrl Pts',(-0.393299967734249,2.09984068823463,
7.41538364779653));
#32201=CARTESIAN_POINT('',(-0.393299835621208,2.10035958355185,7.54038364779653));
#32202=CARTESIAN_POINT('Ctrl Pts',(-0.393871230970384,2.0998404568363,7.41538364779653));
#32203=CARTESIAN_POINT('Ctrl Pts',(-0.393916702120302,2.09098514042463,
7.41583339936755));
#32204=CARTESIAN_POINT('Ctrl Pts',(-0.38962793339212,1.95176327063558,7.42290659877944));
#32205=CARTESIAN_POINT('Ctrl Pts',(-0.224663887225575,1.69281309173686,
7.4366032460324));
#32206=CARTESIAN_POINT('Ctrl Pts',(0.220755421324649,1.69068095030845,7.45647358955513));
#32207=CARTESIAN_POINT('Ctrl Pts',(0.463661683946385,2.06404331321586,7.47634393307795));
#32208=CARTESIAN_POINT('Ctrl Pts',(0.281221473385678,2.47039104118654,7.49621427660072));
#32209=CARTESIAN_POINT('Ctrl Pts',(-0.159201154159844,2.53695541305568,
7.51608462012352));
#32210=CARTESIAN_POINT('Ctrl Pts',(-0.377322826346887,2.2892653798589,7.53080774385545));
#32211=CARTESIAN_POINT('Ctrl Pts',(-0.39361134344189,2.12952756160154,7.53890741974645));
#32212=CARTESIAN_POINT('Ctrl Pts',(-0.39334115544482,2.10035962132946,7.54038364779653));
#32213=CARTESIAN_POINT('',(-0.393056831489965,2.09997021398409,7.66538365574708));
#32214=CARTESIAN_POINT('Ctrl Pts',(-0.393299835621208,2.10035958355185,
7.54038364779653));
#32215=CARTESIAN_POINT('Ctrl Pts',(-0.393318404588432,2.08004950062605,
7.54141168552471));
#32216=CARTESIAN_POINT('Ctrl Pts',(-0.391759450431452,2.0596927690009,7.5424397232529));
#32217=CARTESIAN_POINT('Ctrl Pts',(-0.38862778303309,2.0395571653975,7.54346776098108));
#32218=CARTESIAN_POINT('Ctrl Pts',(-0.385490760961835,2.01938713298762,
7.54449755649675));
#32219=CARTESIAN_POINT('Ctrl Pts',(-0.380775683903768,1.99943974722539,
7.54552735201241));
#32220=CARTESIAN_POINT('Ctrl Pts',(-0.374539625500721,1.97997933957114,
7.54655714752808));
#32221=CARTESIAN_POINT('Ctrl Pts',(-0.36831701768203,1.96056090616374,7.54758472187285));
#32222=CARTESIAN_POINT('Ctrl Pts',(-0.360580232459262,1.94162807082187,
7.54861229621762));
#32223=CARTESIAN_POINT('Ctrl Pts',(-0.351435703674561,1.92342753277261,
7.54963987056239));
#32224=CARTESIAN_POINT('Ctrl Pts',(-0.342261525120969,1.9051679821969,7.55067077666351));
#32225=CARTESIAN_POINT('Ctrl Pts',(-0.331670832463183,1.88764615303161,
7.55170168276462));
#32226=CARTESIAN_POINT('Ctrl Pts',(-0.319816577306472,1.87108462943705,
7.55273258886574));
#32227=CARTESIAN_POINT('Ctrl Pts',(-0.30796232214976,1.85452310584248,7.55376349496686));
#32228=CARTESIAN_POINT('Ctrl Pts',(-0.29484504310219,1.83892242880877,7.55479440106798));
#32229=CARTESIAN_POINT('Ctrl Pts',(-0.280656185780356,1.82446961078091,
7.5558253071691));
#32230=CARTESIAN_POINT('Ctrl Pts',(-0.266287624919792,1.80983374612109,
7.55686926981665));
#32231=CARTESIAN_POINT('Ctrl Pts',(-0.250728306984616,1.79628125247181,
7.5579132324642));
#32232=CARTESIAN_POINT('Ctrl Pts',(-0.234167562247261,1.78400879317428,
7.55895719511176));
#32233=CARTESIAN_POINT('Ctrl Pts',(-0.217637282784374,1.77175891038806,
7.55999923727753));
#32234=CARTESIAN_POINT('Ctrl Pts',(-0.20010978234379,1.76078486875542,7.5610412794433));
#32235=CARTESIAN_POINT('Ctrl Pts',(-0.181808923387943,1.75124449054314,
7.56208332160907));
#32236=CARTESIAN_POINT('Ctrl Pts',(-0.163527719267103,1.74171435854717,
7.56312424463792));
#32237=CARTESIAN_POINT('Ctrl Pts',(-0.144475441288614,1.73361519728125,
7.56416516766677));
#32238=CARTESIAN_POINT('Ctrl Pts',(-0.124902133699992,1.7270598613756,7.56520609069563));
#32239=CARTESIAN_POINT('Ctrl Pts',(-0.105318773770749,1.72050115882028,
7.56624754831542));
#32240=CARTESIAN_POINT('Ctrl Pts',(-0.0852145422218727,1.71548811454974,
7.56728900593521));
#32241=CARTESIAN_POINT('Ctrl Pts',(-0.0648569061699768,1.71208445284823,
7.568330463555));
#32242=CARTESIAN_POINT('Ctrl Pts',(-0.0444930499727531,1.70867975117968,
7.5693722393855));
#32243=CARTESIAN_POINT('Ctrl Pts',(-0.0238763661954681,1.70688549655674,
7.570414015216));
#32244=CARTESIAN_POINT('Ctrl Pts',(-0.00328087734933675,1.70671368464715,
7.57145579104649));
#32245=CARTESIAN_POINT('Ctrl Pts',(0.0173591291133135,1.70654150136223,
7.57249981869909));
#32246=CARTESIAN_POINT('Ctrl Pts',(0.0379771145355644,1.70799871031615,
7.57354384635169));
#32247=CARTESIAN_POINT('Ctrl Pts',(0.0583019934603891,1.71104528855078,
7.57458787400428));
#32248=CARTESIAN_POINT('Ctrl Pts',(0.0654906367226648,1.71212282333858,
7.57495713290015));
#32249=CARTESIAN_POINT('Ctrl Pts',(0.0726427093484844,1.71339871177181,
7.57532639179602));
#32250=CARTESIAN_POINT('Ctrl Pts',(0.0797466199589037,1.71486967581722,
7.57569565069189));
#32251=CARTESIAN_POINT('Ctrl Pts',(0.0998306786282814,1.71902836105536,
7.57673961333944));
#32252=CARTESIAN_POINT('Ctrl Pts',(0.119648397875006,1.72477470446489,7.577783575987));
#32253=CARTESIAN_POINT('Ctrl Pts',(0.138931931743202,1.73205597118298,7.57882753863455));
#32254=CARTESIAN_POINT('Ctrl Pts',(0.158179991472921,1.73932384322633,7.57986958080032));
#32255=CARTESIAN_POINT('Ctrl Pts',(0.17689511485143,1.74812083239178,7.58091162296609));
#32256=CARTESIAN_POINT('Ctrl Pts',(0.194823421295257,1.75834414315746,7.58195366513186));
#32257=CARTESIAN_POINT('Ctrl Pts',(0.212732473019612,1.76855647424798,7.58299458816071));
#32258=CARTESIAN_POINT('Ctrl Pts',(0.229855735145054,1.7801917483558,7.58403551118957));
#32259=CARTESIAN_POINT('Ctrl Pts',(0.245962964008723,1.79310081405119,7.58507643421842));
#32260=CARTESIAN_POINT('Ctrl Pts',(0.262078465125334,1.80601650950627,7.58611789183821));
#32261=CARTESIAN_POINT('Ctrl Pts',(0.277176306301301,1.82020685590285,7.587159349458));
#32262=CARTESIAN_POINT('Ctrl Pts',(0.291058122234436,1.83548145720694,7.58820080707779));
#32263=CARTESIAN_POINT('Ctrl Pts',(0.304944179667533,1.85076072556764,7.58924258290829));
#32264=CARTESIAN_POINT('Ctrl Pts',(0.317613004528018,1.8671243399691,7.59028435873879));
#32265=CARTESIAN_POINT('Ctrl Pts',(0.328906177307067,1.88434839084938,7.59132613456929));
#32266=CARTESIAN_POINT('Ctrl Pts',(0.340223760535351,1.9016096719065,7.59237016222188));
#32267=CARTESIAN_POINT('Ctrl Pts',(0.350159401208883,1.91973445673872,7.59341418987448));
#32268=CARTESIAN_POINT('Ctrl Pts',(0.358600007891362,1.93847314668974,7.59445821752707));
#32269=CARTESIAN_POINT('Ctrl Pts',(0.361585339837577,1.94510077570331,7.59482747642294));
#32270=CARTESIAN_POINT('Ctrl Pts',(0.364384096141018,1.95180502788328,7.59519673531881));
#32271=CARTESIAN_POINT('Ctrl Pts',(0.366992758407857,1.95857438253204,7.59556599421468));
#32272=CARTESIAN_POINT('Ctrl Pts',(0.374367925254579,1.97771259011604,7.59660995686223));
#32273=CARTESIAN_POINT('Ctrl Pts',(0.380263986342827,1.99748628280016,7.59765391950978));
#32274=CARTESIAN_POINT('Ctrl Pts',(0.384580292233866,2.01764170457499,7.59869788215734));
#32275=CARTESIAN_POINT('Ctrl Pts',(0.388888657815109,2.03776004827958,7.59973992432311));
#32276=CARTESIAN_POINT('Ctrl Pts',(0.391622826265736,2.05825802828576,7.60078196648888));
#32277=CARTESIAN_POINT('Ctrl Pts',(0.392731799753853,2.07886653217998,7.60182400865464));
#32278=CARTESIAN_POINT('Ctrl Pts',(0.393839582221865,2.09945290286478,7.6028649316835));
#32279=CARTESIAN_POINT('Ctrl Pts',(0.39332556661581,2.12014883235194,7.60390585471235));
#32280=CARTESIAN_POINT('Ctrl Pts',(0.391190527073315,2.14067998928346,7.6049467777412));
#32281=CARTESIAN_POINT('Ctrl Pts',(0.389054391030155,2.16122169048208,7.605988235361));
#32282=CARTESIAN_POINT('Ctrl Pts',(0.385295627939723,2.18159771656814,7.60702969298079));
#32283=CARTESIAN_POINT('Ctrl Pts',(0.379966947474016,2.20153821363053,7.60807115060058));
#32284=CARTESIAN_POINT('Ctrl Pts',(0.374636638864115,2.2214848033841,7.60911292643108));
#32285=CARTESIAN_POINT('Ctrl Pts',(0.367735682703048,2.24099489830156,7.61015470226157));
#32286=CARTESIAN_POINT('Ctrl Pts',(0.35936659081686,2.25981409013184,7.61119647809207));
#32287=CARTESIAN_POINT('Ctrl Pts',(0.350979408948642,2.27867396007232,7.61224050574467));
#32288=CARTESIAN_POINT('Ctrl Pts',(0.341118107170815,2.29683929816591,7.61328453339727));
#32289=CARTESIAN_POINT('Ctrl Pts',(0.329931334064598,2.31407990284554,7.61432856104986));
#32290=CARTESIAN_POINT('Ctrl Pts',(0.325974719050399,2.32017767873512,7.61469781994573));
#32291=CARTESIAN_POINT('Ctrl Pts',(0.321852681139374,2.32616005598819,7.6150670788416));
#32292=CARTESIAN_POINT('Ctrl Pts',(0.317573002570163,2.33201783991446,7.61543633773746));
#32293=CARTESIAN_POINT('Ctrl Pts',(0.305473566050664,2.34857886981768,7.61648030038501));
#32294=CARTESIAN_POINT('Ctrl Pts',(0.292039135608204,2.36424024068389,7.61752426303257));
#32295=CARTESIAN_POINT('Ctrl Pts',(0.277428590479045,2.37877996194994,7.61856822568012));
#32296=CARTESIAN_POINT('Ctrl Pts',(0.262844923022031,2.39329293583198,7.61961026784589));
#32297=CARTESIAN_POINT('Ctrl Pts',(0.247089909214749,2.4066878005712,7.62065231001166));
#32298=CARTESIAN_POINT('Ctrl Pts',(0.230362217544916,2.41877600086548,7.62169435217743));
#32299=CARTESIAN_POINT('Ctrl Pts',(0.213652491153156,2.43085121862254,7.62273527520629));
#32300=CARTESIAN_POINT('Ctrl Pts',(0.195972737157262,2.44162210568095,7.62377619823514));
#32301=CARTESIAN_POINT('Ctrl Pts',(0.177554037329464,2.45094081242855,7.62481712126399));
#32302=CARTESIAN_POINT('Ctrl Pts',(0.15912587813748,2.46026430502106,7.62585857888378));
#32303=CARTESIAN_POINT('Ctrl Pts',(0.139958664206744,2.4681337808081,7.62690003650358));
#32304=CARTESIAN_POINT('Ctrl Pts',(0.120307826235156,2.47444748222758,7.62794149412337));
#32305=CARTESIAN_POINT('Ctrl Pts',(0.100650984075859,2.4807631127581,7.62898326995387));
#32306=CARTESIAN_POINT('Ctrl Pts',(0.0805109346906823,2.48552183216438,
7.63002504578437));
#32307=CARTESIAN_POINT('Ctrl Pts',(0.0601570805958678,2.48867211844199,
7.63106682161486));
#32308=CARTESIAN_POINT('Ctrl Pts',(0.0397592311835402,2.49182921413488,
7.63211084926746));
#32309=CARTESIAN_POINT('Ctrl Pts',(0.0191473888405084,2.49337088077645,
7.63315487692006));
#32310=CARTESIAN_POINT('Ctrl Pts',(-0.00140442267107771,2.49329749248751,
7.63419890457266));
#32311=CARTESIAN_POINT('Ctrl Pts',(-0.00867332901469911,2.49327153601166,
7.63456816346852));
#32312=CARTESIAN_POINT('Ctrl Pts',(-0.0159347525216559,2.49304402163531,
7.63493742236439));
#32313=CARTESIAN_POINT('Ctrl Pts',(-0.0231767494653366,2.49261651555203,
7.63530668126026));
#32314=CARTESIAN_POINT('Ctrl Pts',(-0.0436512035339527,2.49140787741892,
7.63635064390782));
#32315=CARTESIAN_POINT('Ctrl Pts',(-0.0640918645087113,2.48858975080059,
7.63739460655537));
#32316=CARTESIAN_POINT('Ctrl Pts',(-0.0842260745481705,2.48417555670059,
7.63843856920292));
#32317=CARTESIAN_POINT('Ctrl Pts',(-0.104323245538683,2.47976948298629,
7.63948061136869));
#32318=CARTESIAN_POINT('Ctrl Pts',(-0.124114361287151,2.4737732676065,7.64052265353446));
#32319=CARTESIAN_POINT('Ctrl Pts',(-0.143333338277454,2.46625188619069,
7.64156469570023));
#32320=CARTESIAN_POINT('Ctrl Pts',(-0.162531674388393,2.45873858262037,
7.64260561872908));
#32321=CARTESIAN_POINT('Ctrl Pts',(-0.181158399364075,2.44970360469781,
7.64364654175794));
#32322=CARTESIAN_POINT('Ctrl Pts',(-0.198964109864743,2.43926121644793,
7.64468746478679));
#32323=CARTESIAN_POINT('Ctrl Pts',(-0.216778964914245,2.42881346525962,
7.64572892240658));
#32324=CARTESIAN_POINT('Ctrl Pts',(-0.233771320284392,2.41695721804542,
7.64677038002637));
#32325=CARTESIAN_POINT('Ctrl Pts',(-0.249717347142957,2.40385216230247,
7.64781183764616));
#32326=CARTESIAN_POINT('Ctrl Pts',(-0.265668246207912,2.39074310239365,
7.64885361347666));
#32327=CARTESIAN_POINT('Ctrl Pts',(-0.280571635326441,2.37638496907464,
7.64989538930716));
#32328=CARTESIAN_POINT('Ctrl Pts',(-0.294238361424916,2.36097639101264,
7.65093716513766));
#32329=CARTESIAN_POINT('Ctrl Pts',(-0.307934628462002,2.34553450695947,
7.65198119279025));
#32330=CARTESIAN_POINT('Ctrl Pts',(-0.320388452069471,2.32903823288433,
7.65302522044285));
#32331=CARTESIAN_POINT('Ctrl Pts',(-0.33145181280105,2.31171817539101,7.65406924809545));
#32332=CARTESIAN_POINT('Ctrl Pts',(-0.335364778476012,2.30559229808265,
7.65443850699131));
#32333=CARTESIAN_POINT('Ctrl Pts',(-0.339104220064762,2.29936360554387,
7.65480776588718));
#32334=CARTESIAN_POINT('Ctrl Pts',(-0.342664989095891,2.29304298808274,
7.65517702478305));
#32335=CARTESIAN_POINT('Ctrl Pts',(-0.353181870689793,2.27437477768831,
7.6562676465143));
#32336=CARTESIAN_POINT('Ctrl Pts',(-0.362194639744218,2.25480029445585,
7.65735826824556));
#32337=CARTESIAN_POINT('Ctrl Pts',(-0.369558942677454,2.23457740481642,
7.65844888997681));
#32338=CARTESIAN_POINT('Ctrl Pts',(-0.376903549625527,2.21440860172638,
7.659536594817));
#32339=CARTESIAN_POINT('Ctrl Pts',(-0.382608177514571,2.19359541255137,
7.66062429965719));
#32340=CARTESIAN_POINT('Ctrl Pts',(-0.386575409562742,2.17241783427719,
7.66171200449738));
#32341=CARTESIAN_POINT('Ctrl Pts',(-0.390531598309264,2.15129920652121,
7.66279668157098));
#32342=CARTESIAN_POINT('Ctrl Pts',(-0.392759846853305,2.1298188234893,7.66388135864457));
#32343=CARTESIAN_POINT('Ctrl Pts',(-0.393213048917556,2.10826971347505,
7.66496603571817));
#32344=CARTESIAN_POINT('Ctrl Pts',(-0.393271211437559,2.10550416882927,
7.66510523974429));
#32345=CARTESIAN_POINT('Ctrl Pts',(-0.393300207467801,2.10273750562405,
7.66524444377041));
#32346=CARTESIAN_POINT('Ctrl Pts',(-0.393299998882636,2.09997035343927,
7.66538364779653));
#32347=CARTESIAN_POINT('',(-0.393299846840641,2.09965290472694,7.79038364779653));
#32348=CARTESIAN_POINT('Ctrl Pts',(-0.392654629287079,2.09996998332331,
7.66538366889741));
#32349=CARTESIAN_POINT('Ctrl Pts',(-0.392697384672877,2.03604211742209,
7.66860490203355));
#32350=CARTESIAN_POINT('Ctrl Pts',(-0.347701914019137,1.84072366953728,
7.67844958301063));
#32351=CARTESIAN_POINT('Ctrl Pts',(-0.0400622663258958,1.63667500034933,
7.69491771182861));
#32352=CARTESIAN_POINT('Ctrl Pts',(0.367885526613611,1.81550873512054,7.71478805535143));
#32353=CARTESIAN_POINT('Ctrl Pts',(0.438348431977121,2.2553244754303,7.73465839887419));
#32354=CARTESIAN_POINT('Ctrl Pts',(0.106686326751942,2.55265115505061,7.754528742397));
#32355=CARTESIAN_POINT('Ctrl Pts',(-0.294846097879019,2.4424188008677,7.77310380060152));
#32356=CARTESIAN_POINT('Ctrl Pts',(-0.392480938382109,2.20485551238996,
7.78505541096512));
#32357=CARTESIAN_POINT('Ctrl Pts',(-0.393450074714008,2.09965423931595,
7.79038357348779));
#32358=CARTESIAN_POINT('',(-0.393472008642783,2.10021399309012,7.91538370816546));
#32359=CARTESIAN_POINT('Ctrl Pts',(-0.393299846840641,2.09965290472694,
7.79038364779653));
#32360=CARTESIAN_POINT('Ctrl Pts',(-0.393277285971461,2.0740887813239,7.79167890834521));
#32361=CARTESIAN_POINT('Ctrl Pts',(-0.390760409603109,2.04863121630469,
7.79297416889389));
#32362=CARTESIAN_POINT('Ctrl Pts',(-0.385821589392683,2.02366788907344,
7.79426942944257));
#32363=CARTESIAN_POINT('Ctrl Pts',(-0.381840966476314,2.00354778179849,
7.79531339209014));
#32364=CARTESIAN_POINT('Ctrl Pts',(-0.376270388510308,1.98367994044972,
7.79635735473771));
#32365=CARTESIAN_POINT('Ctrl Pts',(-0.369160215781451,1.96433266758651,
7.79740131738527));
#32366=CARTESIAN_POINT('Ctrl Pts',(-0.36206312298149,1.94502098611651,7.79844335955106));
#32367=CARTESIAN_POINT('Ctrl Pts',(-0.353432252440912,1.92622867558337,
7.79948540171684));
#32368=CARTESIAN_POINT('Ctrl Pts',(-0.343368146843134,1.90821051714572,
7.80052744388263));
#32369=CARTESIAN_POINT('Ctrl Pts',(-0.333314849936666,1.89021170992718,
7.80156836691149));
#32370=CARTESIAN_POINT('Ctrl Pts',(-0.321831705523261,1.87298605743524,
7.80260928994036));
#32371=CARTESIAN_POINT('Ctrl Pts',(-0.309065819745101,1.85676511544335,
7.80365021296923));
#32372=CARTESIAN_POINT('Ctrl Pts',(-0.296293377740715,1.8405358427984,7.80469167058903));
#32373=CARTESIAN_POINT('Ctrl Pts',(-0.282237320642678,1.82531289965662,
7.80573312820884));
#32374=CARTESIAN_POINT('Ctrl Pts',(-0.26708627994932,1.81129633001496,7.80677458582865));
#32375=CARTESIAN_POINT('Ctrl Pts',(-0.251930609952505,1.7972754777002,7.80781636165916));
#32376=CARTESIAN_POINT('Ctrl Pts',(-0.235679854536496,1.78446220536074,
7.80885813748967));
#32377=CARTESIAN_POINT('Ctrl Pts',(-0.21855651124187,1.77301690962103,7.80989991332018));
#32378=CARTESIAN_POINT('Ctrl Pts',(-0.201396155452133,1.76154687461485,
7.81094394097279));
#32379=CARTESIAN_POINT('Ctrl Pts',(-0.183360088888524,1.75145107926569,
7.8119879686254));
#32380=CARTESIAN_POINT('Ctrl Pts',(-0.164696898682035,1.74284482145079,
7.81303199627801));
#32381=CARTESIAN_POINT('Ctrl Pts',(-0.158095972940099,1.7398009008711,7.81340125517379));
#32382=CARTESIAN_POINT('Ctrl Pts',(-0.15141677440106,1.73694286990731,7.81377051406958));
#32383=CARTESIAN_POINT('Ctrl Pts',(-0.144670792145537,1.73427434886245,
7.81413977296536));
#32384=CARTESIAN_POINT('Ctrl Pts',(-0.125598662601031,1.72672995026606,
7.81518373561291));
#32385=CARTESIAN_POINT('Ctrl Pts',(-0.105877971366907,1.72065897044652,
7.81622769826046));
#32386=CARTESIAN_POINT('Ctrl Pts',(-0.0857615729720408,1.71616430259633,
7.81727166090801));
#32387=CARTESIAN_POINT('Ctrl Pts',(-0.0656821808596817,1.71167790317198,
7.81831370307378));
#32388=CARTESIAN_POINT('Ctrl Pts',(-0.0452092235254467,1.70876227640579,
7.81935574523955));
#32389=CARTESIAN_POINT('Ctrl Pts',(-0.0246113511004285,1.70747080185417,
7.82039778740532));
#32390=CARTESIAN_POINT('Ctrl Pts',(-0.00403560046681622,1.70618071432592,
7.82143871043417));
#32391=CARTESIAN_POINT('Ctrl Pts',(0.0166640701210328,1.70651139080553,
7.82247963346302));
#32392=CARTESIAN_POINT('Ctrl Pts',(0.0372133332101566,1.70846448713892,
7.82352055649188));
#32393=CARTESIAN_POINT('Ctrl Pts',(0.0577731498652244,1.71041858653168,
7.82456201411167));
#32394=CARTESIAN_POINT('Ctrl Pts',(0.0781816706999862,1.71399671682075,
7.82560347173146));
#32395=CARTESIAN_POINT('Ctrl Pts',(0.098168585501751,1.71914856069514,7.82664492935125));
#32396=CARTESIAN_POINT('Ctrl Pts',(0.118161607177343,1.72430197868243,7.82768670518174));
#32397=CARTESIAN_POINT('Ctrl Pts',(0.137732063513107,1.73102984895718,7.82872848101224));
#32398=CARTESIAN_POINT('Ctrl Pts',(0.156624648216409,1.7392319171946,7.82977025684274));
#32399=CARTESIAN_POINT('Ctrl Pts',(0.175558069670281,1.74745171438864,7.83081428449533));
#32400=CARTESIAN_POINT('Ctrl Pts',(0.193810043880642,1.75715172563766,7.83185831214793));
#32401=CARTESIAN_POINT('Ctrl Pts',(0.211149061622278,1.76818534725538,7.83290233980053));
#32402=CARTESIAN_POINT('Ctrl Pts',(0.217281644922087,1.77208779459568,7.8332715986964));
#32403=CARTESIAN_POINT('Ctrl Pts',(0.223300299383926,1.77615668051319,7.83364085759228));
#32404=CARTESIAN_POINT('Ctrl Pts',(0.229195761745247,1.78038430451867,7.83401011648815));
#32405=CARTESIAN_POINT('Ctrl Pts',(0.245863315496847,1.79233657323556,7.83505407913571));
#32406=CARTESIAN_POINT('Ctrl Pts',(0.261643070521576,1.80563175244007,7.83609804178326));
#32407=CARTESIAN_POINT('Ctrl Pts',(0.276311637655667,1.82011293546138,7.83714200443081));
#32408=CARTESIAN_POINT('Ctrl Pts',(0.290953220379886,1.8345674787861,7.83818404659658));
#32409=CARTESIAN_POINT('Ctrl Pts',(0.304487113295279,1.85020322641783,7.83922608876235));
#32410=CARTESIAN_POINT('Ctrl Pts',(0.316723008744935,1.86682318783473,7.84026813092811));
#32411=CARTESIAN_POINT('Ctrl Pts',(0.328945763035101,1.88342529967417,7.84130905395697));
#32412=CARTESIAN_POINT('Ctrl Pts',(0.339872830039004,1.90100895447264,7.84234997698582));
#32413=CARTESIAN_POINT('Ctrl Pts',(0.349354319084676,1.91934438913534,7.84339090001467));
#32414=CARTESIAN_POINT('Ctrl Pts',(0.358840677576003,1.93768924039941,7.84443235763446));
#32415=CARTESIAN_POINT('Ctrl Pts',(0.36687962265116,1.95678599669745,7.84547381525425));
#32416=CARTESIAN_POINT('Ctrl Pts',(0.373367138203819,1.97638013869329,7.84651527287404));
#32417=CARTESIAN_POINT('Ctrl Pts',(0.379856635975311,1.99598026755374,7.84755704870454));
#32418=CARTESIAN_POINT('Ctrl Pts',(0.384793563820189,2.01607737538244,7.84859882453503));
#32419=CARTESIAN_POINT('Ctrl Pts',(0.388124015460432,2.03640252659995,7.84964060036553));
#32420=CARTESIAN_POINT('Ctrl Pts',(0.391461665947473,2.05677161109305,7.85068462801812));
#32421=CARTESIAN_POINT('Ctrl Pts',(0.39318584624889,2.07736898915665,7.85172865567072));
#32422=CARTESIAN_POINT('Ctrl Pts',(0.393294503242237,2.09792064446481,7.85277268332331));
#32423=CARTESIAN_POINT('Ctrl Pts',(0.393332933796537,2.10518949556152,7.85314194221919));
#32424=CARTESIAN_POINT('Ctrl Pts',(0.393169748076574,2.11245264946065,7.85351120111507));
#32425=CARTESIAN_POINT('Ctrl Pts',(0.392806406420191,2.11969814903121,7.85388046001095));
#32426=CARTESIAN_POINT('Ctrl Pts',(0.391779172894343,2.14018250566815,7.8549244226585));
#32427=CARTESIAN_POINT('Ctrl Pts',(0.389142214694143,2.16064732695185,7.85596838530606));
#32428=CARTESIAN_POINT('Ctrl Pts',(0.384906537167002,2.18081984685773,7.85701234795361));
#32429=CARTESIAN_POINT('Ctrl Pts',(0.380678651625093,2.20095525723953,7.85805439011938));
#32430=CARTESIAN_POINT('Ctrl Pts',(0.374857975844893,2.22079870943196,7.85909643228515));
#32431=CARTESIAN_POINT('Ctrl Pts',(0.367507126010841,2.24008355482087,7.86013847445092));
#32432=CARTESIAN_POINT('Ctrl Pts',(0.360164170874032,2.25934768858879,7.86117939747978));
#32433=CARTESIAN_POINT('Ctrl Pts',(0.351294537903702,2.27805371222702,7.86222032050863));
#32434=CARTESIAN_POINT('Ctrl Pts',(0.341010277494635,2.29595122006008,7.86326124353749));
#32435=CARTESIAN_POINT('Ctrl Pts',(0.330720735357464,2.31385791958669,7.86430270115728));
#32436=CARTESIAN_POINT('Ctrl Pts',(0.319015466970043,2.33095462777889,7.86534415877707));
#32437=CARTESIAN_POINT('Ctrl Pts',(0.306052170949453,2.34701611011658,7.86638561639686));
#32438=CARTESIAN_POINT('Ctrl Pts',(0.293084914076774,2.36308249993735,7.86742739222736));
#32439=CARTESIAN_POINT('Ctrl Pts',(0.278859354235047,2.37811248486136,7.86846916805786));
#32440=CARTESIAN_POINT('Ctrl Pts',(0.263572436832274,2.39191515983638,7.86951094388836));
#32441=CARTESIAN_POINT('Ctrl Pts',(0.248252476410633,2.40574766960658,7.87055497154096));
#32442=CARTESIAN_POINT('Ctrl Pts',(0.231867162102429,2.41834712419121,7.87159899919356));
#32443=CARTESIAN_POINT('Ctrl Pts',(0.214645780348323,2.42956346729979,7.87264302684616));
#32444=CARTESIAN_POINT('Ctrl Pts',(0.208554803355672,2.43353054083614,7.87301228574201));
#32445=CARTESIAN_POINT('Ctrl Pts',(0.202359478136538,2.43732500780329,7.87338154463787));
#32446=CARTESIAN_POINT('Ctrl Pts',(0.19607064896799,2.4409416234684,7.87375080353373));
#32447=CARTESIAN_POINT('Ctrl Pts',(0.178290975079414,2.45116645950429,7.87479476618128));
#32448=CARTESIAN_POINT('Ctrl Pts',(0.15965635381351,2.46002723537316,7.87583872882884));
#32449=CARTESIAN_POINT('Ctrl Pts',(0.140402089120858,2.4673855513905,7.87688269147639));
#32450=CARTESIAN_POINT('Ctrl Pts',(0.121183244722872,2.47473033099261,7.87792473364216));
#32451=CARTESIAN_POINT('Ctrl Pts',(0.101347677861961,2.4805778218012,7.87896677580793));
#32452=CARTESIAN_POINT('Ctrl Pts',(0.0811534867391165,2.48483633091236,
7.8800088179737));
#32453=CARTESIAN_POINT('Ctrl Pts',(0.0609809838603006,2.48909026645163,
7.88104974100255));
#32454=CARTESIAN_POINT('Ctrl Pts',(0.0404513316745512,2.49175842883664,
7.8820906640314));
#32455=CARTESIAN_POINT('Ctrl Pts',(0.0198357306604741,2.49279948292884,
7.88313158706026));
#32456=CARTESIAN_POINT('Ctrl Pts',(-0.000790457988976343,2.4938410716793,
7.88417304468005));
#32457=CARTESIAN_POINT('Ctrl Pts',(-0.0215019496218682,2.4932538295059,
7.88521450229984));
#32458=CARTESIAN_POINT('Ctrl Pts',(-0.0420239979101587,2.49104842871395,
7.88625595991963));
#32459=CARTESIAN_POINT('Ctrl Pts',(-0.0625523165788904,2.4888423540759,
7.88729773575013));
#32460=CARTESIAN_POINT('Ctrl Pts',(-0.0828903495874746,2.48501725107508,
7.88833951158063));
#32461=CARTESIAN_POINT('Ctrl Pts',(-0.102770970442034,2.47963537458251,
7.88938128741113));
#32462=CARTESIAN_POINT('Ctrl Pts',(-0.122694563709719,2.47424186504177,
7.89042531506373));
#32463=CARTESIAN_POINT('Ctrl Pts',(-0.142158077408814,2.46728511182687,
7.89146934271632));
#32464=CARTESIAN_POINT('Ctrl Pts',(-0.160911224630327,2.45887667490096,
7.89251337036892));
#32465=CARTESIAN_POINT('Ctrl Pts',(-0.167543966990968,2.45590272097597,
7.89288262926479));
#32466=CARTESIAN_POINT('Ctrl Pts',(-0.174088064238261,2.45274759413915,
7.89325188816065));
#32467=CARTESIAN_POINT('Ctrl Pts',(-0.180533236303805,2.44941757338416,
7.89362114705652));
#32468=CARTESIAN_POINT('Ctrl Pts',(-0.198754920246359,2.44000299374183,
7.89466510970407));
#32469=CARTESIAN_POINT('Ctrl Pts',(-0.2162924764411,2.42913116862194,7.89570907235163));
#32470=CARTESIAN_POINT('Ctrl Pts',(-0.232902161675197,2.41692502754914,
7.89675303499918));
#32471=CARTESIAN_POINT('Ctrl Pts',(-0.249481291603513,2.40474134098812,
7.89779507716495));
#32472=CARTESIAN_POINT('Ctrl Pts',(-0.26513531731884,2.39122859366002,7.89883711933072));
#32473=CARTESIAN_POINT('Ctrl Pts',(-0.279647428566151,2.37655416412764,
7.89987916149648));
#32474=CARTESIAN_POINT('Ctrl Pts',(-0.294143954033967,2.36189549470205,
7.90092008452534));
#32475=CARTESIAN_POINT('Ctrl Pts',(-0.307500464414512,2.34607812008314,
7.90196100755419));
#32476=CARTESIAN_POINT('Ctrl Pts',(-0.319535398663865,2.32930769503164,
7.90300193058304));
#32477=CARTESIAN_POINT('Ctrl Pts',(-0.331576513741777,2.31252865712693,
7.90404338820283));
#32478=CARTESIAN_POINT('Ctrl Pts',(-0.342294254661971,2.29479617933626,
7.90508484582262));
#32479=CARTESIAN_POINT('Ctrl Pts',(-0.351548869738086,2.2763470504031,7.90612630344241));
#32480=CARTESIAN_POINT('Ctrl Pts',(-0.360806312502575,2.25789228445674,
7.90716807927291));
#32481=CARTESIAN_POINT('Ctrl Pts',(-0.368599442165857,2.23872110479362,
7.90820985510341));
#32482=CARTESIAN_POINT('Ctrl Pts',(-0.374836003340324,2.21909181583909,
7.90925163093391));
#32483=CARTESIAN_POINT('Ctrl Pts',(-0.381086044983296,2.19942009773105,
7.9102956585865));
#32484=CARTESIAN_POINT('Ctrl Pts',(-0.385772633972532,2.17928901071487,
7.9113396862391));
#32485=CARTESIAN_POINT('Ctrl Pts',(-0.388854087096225,2.15896938992868,
7.91238371389169));
#32486=CARTESIAN_POINT('Ctrl Pts',(-0.389943956675164,2.15178260640108,
7.91275297278756));
#32487=CARTESIAN_POINT('Ctrl Pts',(-0.390833507624469,2.14457228510115,
7.91312223168343));
#32488=CARTESIAN_POINT('Ctrl Pts',(-0.39152245464766,2.1373504686272,7.9134914905793));
#32489=CARTESIAN_POINT('Ctrl Pts',(-0.392699222580031,2.12501511953074,
7.91412220965171));
#32490=CARTESIAN_POINT('Ctrl Pts',(-0.393293155378434,2.11262329265773,
7.91475292872412));
#32491=CARTESIAN_POINT('Ctrl Pts',(-0.393299941186222,2.10021508815424,
7.91538364779652));
#32492=CARTESIAN_POINT('',(-0.393123696123607,2.1002301365466,8.04038359743823));
#32493=CARTESIAN_POINT('Ctrl Pts',(-0.39380310770544,2.10021188592406,7.91538382432977));
#32494=CARTESIAN_POINT('Ctrl Pts',(-0.393024373222605,1.98216613471237,
7.92137649425388));
#32495=CARTESIAN_POINT('Ctrl Pts',(-0.273797281021035,1.73228844719605,
7.93399261201892));
#32496=CARTESIAN_POINT('Ctrl Pts',(0.151435609798601,1.6602929423249,7.95323217762489));
#32497=CARTESIAN_POINT('Ctrl Pts',(0.451688398629209,1.98930839675799,7.97310252114768));
#32498=CARTESIAN_POINT('Ctrl Pts',(0.337578573540234,2.41986832786486,7.99297286467047));
#32499=CARTESIAN_POINT('Ctrl Pts',(-0.0862136355990253,2.55699261429619,
8.01284320819326));
#32500=CARTESIAN_POINT('Ctrl Pts',(-0.360367354736448,2.33262573473897,
8.02864675384896));
#32501=CARTESIAN_POINT('Ctrl Pts',(-0.393056166243688,2.15092736107523,
8.03782685166375));
#32502=CARTESIAN_POINT('Ctrl Pts',(-0.392788426279983,2.10023184074339,
8.0403835016376));
#32503=CARTESIAN_POINT('',(-0.393299872203804,2.09968294405636,8.16538364780065));
#32504=CARTESIAN_POINT('Ctrl Pts',(-0.393299933191821,2.10022924072298,
8.04038364779653));
#32505=CARTESIAN_POINT('Ctrl Pts',(-0.393312109279616,2.0793391717426,8.04143579816531));
#32506=CARTESIAN_POINT('Ctrl Pts',(-0.391655576185796,2.05844602648898,
8.04248794853408));
#32507=CARTESIAN_POINT('Ctrl Pts',(-0.38835514890639,2.03782952213554,8.04354009890286));
#32508=CARTESIAN_POINT('Ctrl Pts',(-0.385053731339344,2.01720683183473,
8.04459256496758));
#32509=CARTESIAN_POINT('Ctrl Pts',(-0.380107581434242,1.99686164941892,
8.04564503103231));
#32510=CARTESIAN_POINT('Ctrl Pts',(-0.373592758590756,1.97706367205521,
8.04669749709703));
#32511=CARTESIAN_POINT('Ctrl Pts',(-0.367060207838806,1.95721182112673,
8.04775282709566));
#32512=CARTESIAN_POINT('Ctrl Pts',(-0.358950717066223,1.93791081977075,
8.04880815709429));
#32513=CARTESIAN_POINT('Ctrl Pts',(-0.349389250212133,1.91941195544499,
8.04986348709293));
#32514=CARTESIAN_POINT('Ctrl Pts',(-0.341173465465354,1.90351662372658,
8.05077028980823));
#32515=CARTESIAN_POINT('Ctrl Pts',(-0.33188659664511,1.88821339649346,8.05167709252353));
#32516=CARTESIAN_POINT('Ctrl Pts',(-0.321633311049409,1.87364429933533,
8.05258389523884));
#32517=CARTESIAN_POINT('Ctrl Pts',(-0.309829147921141,1.85687152948697,
8.05362785788639));
#32518=CARTESIAN_POINT('Ctrl Pts',(-0.296674263106577,1.84097462839784,
8.05467182053395));
#32519=CARTESIAN_POINT('Ctrl Pts',(-0.282323578400054,1.82617836630502,
8.0557157831815));
#32520=CARTESIAN_POINT('Ctrl Pts',(-0.267999293324419,1.8114093235307,8.05675782534727));
#32521=CARTESIAN_POINT('Ctrl Pts',(-0.252484038663387,1.79773746432086,
8.05779986751304));
#32522=CARTESIAN_POINT('Ctrl Pts',(-0.235973111516883,1.78535483375548,
8.05884190967881));
#32523=CARTESIAN_POINT('Ctrl Pts',(-0.219479916846765,1.77298550194081,
8.05988283270766));
#32524=CARTESIAN_POINT('Ctrl Pts',(-0.201993740875486,1.7619031123392,8.06092375573651));
#32525=CARTESIAN_POINT('Ctrl Pts',(-0.183743009992987,1.75225958492186,
8.06196467876536));
#32526=CARTESIAN_POINT('Ctrl Pts',(-0.165482906010769,1.74261110484018,
8.06300613638516));
#32527=CARTESIAN_POINT('Ctrl Pts',(-0.1464581056945,1.73440332121998,8.06404759400495));
#32528=CARTESIAN_POINT('Ctrl Pts',(-0.12692219704885,1.72774250055064,8.06508905162474));
#32529=CARTESIAN_POINT('Ctrl Pts',(-0.107380319331415,1.72107964471019,
8.06613082745523));
#32530=CARTESIAN_POINT('Ctrl Pts',(-0.0873277298967882,1.71596489578267,
8.06717260328573));
#32531=CARTESIAN_POINT('Ctrl Pts',(-0.0670328762866684,1.71245454009015,
8.06821437911623));
#32532=CARTESIAN_POINT('Ctrl Pts',(-0.0466941548899186,1.70893659668415,
8.06925840676883));
#32533=CARTESIAN_POINT('Ctrl Pts',(-0.0261128571950155,1.70703003800371,
8.07030243442142));
#32534=CARTESIAN_POINT('Ctrl Pts',(-0.00556297059209929,1.70673934425347,
8.07134646207402));
#32535=CARTESIAN_POINT('Ctrl Pts',(0.00170525493651206,1.70663652968435,
8.07171572096989));
#32536=CARTESIAN_POINT('Ctrl Pts',(0.00896956935361507,1.70673537394422,
8.07208497986575));
#32537=CARTESIAN_POINT('Ctrl Pts',(0.0162180030620408,1.70703452266557,
8.07245423876162));
#32538=CARTESIAN_POINT('Ctrl Pts',(0.0367106550456766,1.70788027098645,
8.07349820140917));
#32539=CARTESIAN_POINT('Ctrl Pts',(0.0571980309494468,1.71033585387032,
8.07454216405673));
#32540=CARTESIAN_POINT('Ctrl Pts',(0.0774072779671117,1.7143926824894,8.07558612670428));
#32541=CARTESIAN_POINT('Ctrl Pts',(0.0975793478972116,1.71844204813508,
8.07662816887005));
#32542=CARTESIAN_POINT('Ctrl Pts',(0.117473579597926,1.72408672762005,8.07767021103582));
#32543=CARTESIAN_POINT('Ctrl Pts',(0.136822780278586,1.73126646911782,8.07871225320159));
#32544=CARTESIAN_POINT('Ctrl Pts',(0.156151200221679,1.73843849968602,8.07975317623044));
#32545=CARTESIAN_POINT('Ctrl Pts',(0.174935054830473,1.74714209178445,8.0807940992593));
#32546=CARTESIAN_POINT('Ctrl Pts',(0.192922955740864,1.75726741744006,8.08183502228815));
#32547=CARTESIAN_POINT('Ctrl Pts',(0.210920094768347,1.76739794319902,8.08287647990794));
#32548=CARTESIAN_POINT('Ctrl Pts',(0.228119814359035,1.77895131435342,8.08391793752773));
#32549=CARTESIAN_POINT('Ctrl Pts',(0.244295491977069,1.79177183353937,8.08495939514752));
#32550=CARTESIAN_POINT('Ctrl Pts',(0.260476111969821,1.80459626995287,8.08600117097802));
#32551=CARTESIAN_POINT('Ctrl Pts',(0.275631513432774,1.81868814016664,8.08704294680852));
#32552=CARTESIAN_POINT('Ctrl Pts',(0.289569054313693,1.83385219748442,8.08808472263902));
#32553=CARTESIAN_POINT('Ctrl Pts',(0.303536721505506,1.8490490322562,8.08912875029162));
#32554=CARTESIAN_POINT('Ctrl Pts',(0.316280818502472,1.86532210119047,8.09017277794421));
#32555=CARTESIAN_POINT('Ctrl Pts',(0.327649263943418,1.88244345599974,8.09121680559681));
#32556=CARTESIAN_POINT('Ctrl Pts',(0.331670134081134,1.88849905477333,8.09158606449268));
#32557=CARTESIAN_POINT('Ctrl Pts',(0.335519328709527,1.89466052658222,8.09195532338855));
#32558=CARTESIAN_POINT('Ctrl Pts',(0.339191507245826,1.90091707403118,8.09232458228442));
#32559=CARTESIAN_POINT('Ctrl Pts',(0.349573429712498,1.91860548157514,8.09336854493197));
#32560=CARTESIAN_POINT('Ctrl Pts',(0.358598918418144,1.9371608854335,8.09441250757953));
#32561=CARTESIAN_POINT('Ctrl Pts',(0.366127494848793,1.95634921679383,8.09545647022708));
#32562=CARTESIAN_POINT('Ctrl Pts',(0.373642221651847,1.97550224915096,8.09649851239285));
#32563=CARTESIAN_POINT('Ctrl Pts',(0.379665181161932,1.995285242357,8.09754055455862));
#32564=CARTESIAN_POINT('Ctrl Pts',(0.384102397908064,2.01544092052727,8.09858259672439));
#32565=CARTESIAN_POINT('Ctrl Pts',(0.388534849153124,2.03557495181586,8.09962351975324));
#32566=CARTESIAN_POINT('Ctrl Pts',(0.391384752986762,2.05608016475114,8.1006644427821));
#32567=CARTESIAN_POINT('Ctrl Pts',(0.39260837367134,2.07668573562933,8.10170536581095));
#32568=CARTESIAN_POINT('Ctrl Pts',(0.393832622775608,2.09730188899165,8.10274682343074));
#32569=CARTESIAN_POINT('Ctrl Pts',(0.393428860446642,2.11801776973594,8.10378828105053));
#32570=CARTESIAN_POINT('Ctrl Pts',(0.391405324942168,2.13855854778018,8.10482973867033));
#32571=CARTESIAN_POINT('Ctrl Pts',(0.389381171159378,2.15910560192761,8.10587151450082));
#32572=CARTESIAN_POINT('Ctrl Pts',(0.38573636702999,2.17947671879645,8.10691329033132));
#32573=CARTESIAN_POINT('Ctrl Pts',(0.380530798848308,2.19940423093545,8.10795506616182));
#32574=CARTESIAN_POINT('Ctrl Pts',(0.375313978712872,2.21937481684416,8.10899909381441));
#32575=CARTESIAN_POINT('Ctrl Pts',(0.368529900969318,2.23889918802424,8.11004312146701));
#32576=CARTESIAN_POINT('Ctrl Pts',(0.360287904230309,2.25772607921752,8.11108714911961));
#32577=CARTESIAN_POINT('Ctrl Pts',(0.357372818017805,2.26438490385428,8.11145640801547));
#32578=CARTESIAN_POINT('Ctrl Pts',(0.354275780806462,2.27095669163608,8.11182566691134));
#32579=CARTESIAN_POINT('Ctrl Pts',(0.351002980285546,2.27743110728016,8.1121949258072));
#32580=CARTESIAN_POINT('Ctrl Pts',(0.341750172743193,2.29573546818485,8.11323888845475));
#32581=CARTESIAN_POINT('Ctrl Pts',(0.331034117072615,2.31336863606777,8.11428285110231));
#32582=CARTESIAN_POINT('Ctrl Pts',(0.318975578964254,2.33008578840167,8.11532681374986));
#32583=CARTESIAN_POINT('Ctrl Pts',(0.306939223836122,2.34677218773249,8.11636885591563));
#32584=CARTESIAN_POINT('Ctrl Pts',(0.29356566575696,2.36254529160438,8.1174108980814));
#32585=CARTESIAN_POINT('Ctrl Pts',(0.279020356276489,2.37718681567373,8.11845294024717));
#32586=CARTESIAN_POINT('Ctrl Pts',(0.264490668229895,2.39181261497624,8.11949386327603));
#32587=CARTESIAN_POINT('Ctrl Pts',(0.248792222500366,2.40530870741288,8.12053478630488));
#32588=CARTESIAN_POINT('Ctrl Pts',(0.23212905756193,2.41749171742805,8.12157570933374));
#32589=CARTESIAN_POINT('Ctrl Pts',(0.215457334856286,2.42968098431962,8.12261716695353));
#32590=CARTESIAN_POINT('Ctrl Pts',(0.197820487577217,2.44055537428341,8.12365862457332));
#32591=CARTESIAN_POINT('Ctrl Pts',(0.179454057296113,2.44997304370475,8.12470008219311));
#32592=CARTESIAN_POINT('Ctrl Pts',(0.161082015269849,2.45939359063467,8.12574185802361));
#32593=CARTESIAN_POINT('Ctrl Pts',(0.141980617141569,2.46735622770853,8.12678363385411));
#32594=CARTESIAN_POINT('Ctrl Pts',(0.12240734002988,2.47376641516703,8.12782540968461));
#32595=CARTESIAN_POINT('Ctrl Pts',(0.102791754835532,2.48019045839118,8.12886943733721));
#32596=CARTESIAN_POINT('Ctrl Pts',(0.0827029701123902,2.48505517926245,
8.1299134649898));
#32597=CARTESIAN_POINT('Ctrl Pts',(0.0624114411549417,2.48831649721968,
8.1309574926424));
#32598=CARTESIAN_POINT('Ctrl Pts',(0.0552345933390587,2.4894699826326,8.13132675153827));
#32599=CARTESIAN_POINT('Ctrl Pts',(0.0480324343058591,2.49042336576572,
8.13169601043413));
#32600=CARTESIAN_POINT('Ctrl Pts',(0.0408170036541203,2.49117625466367,
8.13206526933));
#32601=CARTESIAN_POINT('Ctrl Pts',(0.0204176573668355,2.49330480971277,
8.13310923197755));
#32602=CARTESIAN_POINT('Ctrl Pts',(-0.000209420461472831,2.49383971062672,
8.13415319462511));
#32603=CARTESIAN_POINT('Ctrl Pts',(-0.0207930060161651,2.49274997250262,
8.13519715727266));
#32604=CARTESIAN_POINT('Ctrl Pts',(-0.0413387258472349,2.49166223906923,
8.13623919943843));
#32605=CARTESIAN_POINT('Ctrl Pts',(-0.0618403826235695,2.48895577811871,
8.1372812416042));
#32606=CARTESIAN_POINT('Ctrl Pts',(-0.0820248770474154,2.484651543017,8.13832328376997));
#32607=CARTESIAN_POINT('Ctrl Pts',(-0.102187693641291,2.48035193059618,
8.13936420679882));
#32608=CARTESIAN_POINT('Ctrl Pts',(-0.122033302127519,2.47445807505066,
8.14040512982768));
#32609=CARTESIAN_POINT('Ctrl Pts',(-0.141297067342993,2.46704227108096,
8.14144605285653));
#32610=CARTESIAN_POINT('Ctrl Pts',(-0.160570725926243,2.45962265854761,
8.14248751047632));
#32611=CARTESIAN_POINT('Ctrl Pts',(-0.179261251816834,2.45067978535362,
8.14352896809611));
#32612=CARTESIAN_POINT('Ctrl Pts',(-0.19712187745538,2.44033491655789,8.14457042571591));
#32613=CARTESIAN_POINT('Ctrl Pts',(-0.214987960293711,2.42998688695375,
8.1456122015464));
#32614=CARTESIAN_POINT('Ctrl Pts',(-0.232023020058744,2.41823640873251,
8.1466539773769));
#32615=CARTESIAN_POINT('Ctrl Pts',(-0.248008189011547,2.40524879718553,
8.1476957532074));
#32616=CARTESIAN_POINT('Ctrl Pts',(-0.264027910269793,2.39223311262146,
8.14873978086));
#32617=CARTESIAN_POINT('Ctrl Pts',(-0.278992676830141,2.37797546405646,
8.14978380851259));
#32618=CARTESIAN_POINT('Ctrl Pts',(-0.292719022629805,2.36267939354021,
8.15082783616519));
#32619=CARTESIAN_POINT('Ctrl Pts',(-0.297573851217542,2.35726937389579,
8.15119709506105));
#32620=CARTESIAN_POINT('Ctrl Pts',(-0.302274131644997,2.35172975314699,
8.15156635395692));
#32621=CARTESIAN_POINT('Ctrl Pts',(-0.306813017096715,2.34607044223151,
8.15193561285278));
#32622=CARTESIAN_POINT('Ctrl Pts',(-0.31961886759936,2.3301034630463,8.15297742681074));
#32623=CARTESIAN_POINT('Ctrl Pts',(-0.331215043950816,2.31308411630537,
8.15401924076871));
#32624=CARTESIAN_POINT('Ctrl Pts',(-0.341428155603478,2.29522219279889,
8.15506105472667));
#32625=CARTESIAN_POINT('Ctrl Pts',(-0.351620131549464,2.27739723396966,
8.15610071268409));
#32626=CARTESIAN_POINT('Ctrl Pts',(-0.360434309648539,2.25873376402489,
8.15714037064152));
#32627=CARTESIAN_POINT('Ctrl Pts',(-0.367739873823155,2.23947141356038,
8.15818002859894));
#32628=CARTESIAN_POINT('Ctrl Pts',(-0.375036810917241,2.2202318098468,8.15921845883285));
#32629=CARTESIAN_POINT('Ctrl Pts',(-0.380828381163626,2.20039540589499,
8.16025688906676));
#32630=CARTESIAN_POINT('Ctrl Pts',(-0.385031436584233,2.18022270776957,
8.16129531930067));
#32631=CARTESIAN_POINT('Ctrl Pts',(-0.389234429074351,2.16005031168103,
8.16233373398663));
#32632=CARTESIAN_POINT('Ctrl Pts',(-0.391848790948663,2.13954235110016,
8.16337214867258));
#32633=CARTESIAN_POINT('Ctrl Pts',(-0.392842214006138,2.11897063242898,
8.16441056335854));
#32634=CARTESIAN_POINT('Ctrl Pts',(-0.393152521802127,2.11254480545373,
8.16473492483786));
#32635=CARTESIAN_POINT('Ctrl Pts',(-0.393305055583653,2.10611279720991,
8.16505928631719));
#32636=CARTESIAN_POINT('Ctrl Pts',(-0.39329987220387,2.09968294413829,8.16538364779652));
#32637=CARTESIAN_POINT('',(-0.393299992164447,2.09992149238468,8.29038364779182));
#32638=CARTESIAN_POINT('Ctrl Pts',(-0.393299872203804,2.09968294405636,
8.16538364780065));
#32639=CARTESIAN_POINT('Ctrl Pts',(-0.393280180214925,2.07525553033001,
8.16661591733532));
#32640=CARTESIAN_POINT('Ctrl Pts',(-0.390980683010069,2.05092561102102,
8.16784818686999));
#32641=CARTESIAN_POINT('Ctrl Pts',(-0.386479320274873,2.0270710962658,8.16908045640465));
#32642=CARTESIAN_POINT('Ctrl Pts',(-0.383160656714444,2.0094841756982,8.16998895639496));
#32643=CARTESIAN_POINT('Ctrl Pts',(-0.378646245086477,1.99215525616916,
8.17089745638527));
#32644=CARTESIAN_POINT('Ctrl Pts',(-0.372983863481854,1.97522849851769,
8.17180595637558));
#32645=CARTESIAN_POINT('Ctrl Pts',(-0.366477187692725,1.95577786239148,
8.17284991902312));
#32646=CARTESIAN_POINT('Ctrl Pts',(-0.358425539429026,1.93677961460506,
8.17389388167067));
#32647=CARTESIAN_POINT('Ctrl Pts',(-0.348912986099889,1.91849347634077,
8.17493784431822));
#32648=CARTESIAN_POINT('Ctrl Pts',(-0.339417932137639,1.90024097739826,
8.17597988648398));
#32649=CARTESIAN_POINT('Ctrl Pts',(-0.328467590641094,1.88269866048875,
8.17702192864974));
#32650=CARTESIAN_POINT('Ctrl Pts',(-0.316194084772954,1.8661064542263,8.17806397081551));
#32651=CARTESIAN_POINT('Ctrl Pts',(-0.303933760457306,1.84953206773273,
8.17910489384435));
#32652=CARTESIAN_POINT('Ctrl Pts',(-0.290353505003252,1.83390637187051,
8.1801458168732));
#32653=CARTESIAN_POINT('Ctrl Pts',(-0.275628673858284,1.81944033763364,
8.18118673990205));
#32654=CARTESIAN_POINT('Ctrl Pts',(-0.260896280423819,1.80496687401863,
8.18222819752183));
#32655=CARTESIAN_POINT('Ctrl Pts',(-0.245018650525355,1.79165478898914,
8.18326965514162));
#32656=CARTESIAN_POINT('Ctrl Pts',(-0.228208321034623,1.77967851740703,
8.1843111127614));
#32657=CARTESIAN_POINT('Ctrl Pts',(-0.211392855255364,1.76769858655183,
8.18535288859189));
#32658=CARTESIAN_POINT('Ctrl Pts',(-0.19364474229533,1.75705567877349,8.18639466442239));
#32659=CARTESIAN_POINT('Ctrl Pts',(-0.175205068829557,1.74788059715995,
8.18743644025288));
#32660=CARTESIAN_POINT('Ctrl Pts',(-0.156725537591138,1.73868568339931,
8.18848046790547));
#32661=CARTESIAN_POINT('Ctrl Pts',(-0.137552144677004,1.73096520511339,
8.18952449555806));
#32662=CARTESIAN_POINT('Ctrl Pts',(-0.117946120068504,1.72480191530235,
8.19056852321065));
#32663=CARTESIAN_POINT('Ctrl Pts',(-0.11101172615467,1.72262204048283,8.19093778210655));
#32664=CARTESIAN_POINT('Ctrl Pts',(-0.104023331508305,1.72063649914217,
8.19130704100246));
#32665=CARTESIAN_POINT('Ctrl Pts',(-0.0969927922902984,1.71884742130778,
8.19167629989836));
#32666=CARTESIAN_POINT('Ctrl Pts',(-0.0771161680107532,1.71378937002345,
8.19272026254591));
#32667=CARTESIAN_POINT('Ctrl Pts',(-0.0567835984306736,1.71027524524002,
8.19376422519347));
#32668=CARTESIAN_POINT('Ctrl Pts',(-0.0362589689778868,1.70837495334356,
8.19480818784102));
#32669=CARTESIAN_POINT('Ctrl Pts',(-0.0157720967926314,1.70647815723881,
8.19585023000679));
#32670=CARTESIAN_POINT('Ctrl Pts',(0.00490541506159886,1.70618942731558,
8.19689227217256));
#32671=CARTESIAN_POINT('Ctrl Pts',(0.025500309655024,1.70752754974712,8.19793431433833));
#32672=CARTESIAN_POINT('Ctrl Pts',(0.0460730856551914,1.70886423505619,
8.19897523736719));
#32673=CARTESIAN_POINT('Ctrl Pts',(0.0665626881616451,1.71182428547951,
8.20001616039604));
#32674=CARTESIAN_POINT('Ctrl Pts',(0.0866968059131255,1.71637446142825,
8.20105708342489));
#32675=CARTESIAN_POINT('Ctrl Pts',(0.106841264022724,1.72092697422877,8.20209854104468));
#32676=CARTESIAN_POINT('Ctrl Pts',(0.126629151414903,1.72707109756612,8.20313999866448));
#32677=CARTESIAN_POINT('Ctrl Pts',(0.145798750085708,1.73472255137574,8.20418145628427));
#32678=CARTESIAN_POINT('Ctrl Pts',(0.164974205904633,1.74237634303809,8.20522323211477));
#32679=CARTESIAN_POINT('Ctrl Pts',(0.183530327552762,1.7515380758985,8.20626500794527));
#32680=CARTESIAN_POINT('Ctrl Pts',(0.201226628878443,1.76207584603906,8.20730678377577));
#32681=CARTESIAN_POINT('Ctrl Pts',(0.218961181161015,1.77263639380891,8.20835081142836));
#32682=CARTESIAN_POINT('Ctrl Pts',(0.235831601559906,1.78457849146271,8.20939483908096));
#32683=CARTESIAN_POINT('Ctrl Pts',(0.251626901361927,1.79772728784921,8.21043886673356));
#32684=CARTESIAN_POINT('Ctrl Pts',(0.25721349186098,1.80237784477991,8.21080812562942));
#32685=CARTESIAN_POINT('Ctrl Pts',(0.262665914863867,1.80717900271683,8.21117738452529));
#32686=CARTESIAN_POINT('Ctrl Pts',(0.267975961451293,1.81212194580994,8.21154664342115));
#32687=CARTESIAN_POINT('Ctrl Pts',(0.28298843740279,1.82609655282952,8.2125906060687));
#32688=CARTESIAN_POINT('Ctrl Pts',(0.29694956373887,1.84129028213312,8.21363456871626));
#32689=CARTESIAN_POINT('Ctrl Pts',(0.309657715968291,1.85751909571824,8.21467853136381));
#32690=CARTESIAN_POINT('Ctrl Pts',(0.322342490182303,1.87371805465201,8.21572057352958));
#32691=CARTESIAN_POINT('Ctrl Pts',(0.333778370256915,1.89094778211271,8.21676261569535));
#32692=CARTESIAN_POINT('Ctrl Pts',(0.343801641527771,1.90898868807631,8.21780465786112));
#32693=CARTESIAN_POINT('Ctrl Pts',(0.353814147962746,1.92701021839032,8.21884558088998));
#32694=CARTESIAN_POINT('Ctrl Pts',(0.362416676629305,1.94584057181033,8.21988650391883));
#32695=CARTESIAN_POINT('Ctrl Pts',(0.369489768962802,1.96523279096229,8.22092742694769));
#32696=CARTESIAN_POINT('Ctrl Pts',(0.376566493852174,1.98463496945257,8.22196888456748));
#32697=CARTESIAN_POINT('Ctrl Pts',(0.38211194593321,2.00459890444163,8.22301034218727));
#32698=CARTESIAN_POINT('Ctrl Pts',(0.386055316708674,2.02485891642407,8.22405179980707));
#32699=CARTESIAN_POINT('Ctrl Pts',(0.389999892355826,2.04512511872342,8.22509357563757));
#32700=CARTESIAN_POINT('Ctrl Pts',(0.392341307267576,2.06568684958046,8.22613535146806));
#32701=CARTESIAN_POINT('Ctrl Pts',(0.393060289120565,2.08627050195899,8.22717712729856));
#32702=CARTESIAN_POINT('Ctrl Pts',(0.393780825069144,2.10689864636923,8.22822115495116));
#32703=CARTESIAN_POINT('Ctrl Pts',(0.392871958936984,2.12754807113513,8.22926518260376));
#32704=CARTESIAN_POINT('Ctrl Pts',(0.390366496699893,2.14794672308148,8.23030921025636));
#32705=CARTESIAN_POINT('Ctrl Pts',(0.389480347547631,2.15516145889428,8.23067846915222));
#32706=CARTESIAN_POINT('Ctrl Pts',(0.388394943082999,2.16234490731996,8.23104772804808));
#32707=CARTESIAN_POINT('Ctrl Pts',(0.387113252194205,2.16948539397331,8.23141698694394));
#32708=CARTESIAN_POINT('Ctrl Pts',(0.383489676896194,2.18967285982725,8.23246094959149));
#32709=CARTESIAN_POINT('Ctrl Pts',(0.378271927210641,2.20963626502126,8.23350491223904));
#32710=CARTESIAN_POINT('Ctrl Pts',(0.371505602604905,2.22910645697705,8.2345488748866));
#32711=CARTESIAN_POINT('Ctrl Pts',(0.364751725382394,2.2485408314167,8.23559091705236));
#32712=CARTESIAN_POINT('Ctrl Pts',(0.356455110563429,2.26748308693169,8.23663295921813));
#32713=CARTESIAN_POINT('Ctrl Pts',(0.346711771665886,2.28567670125329,8.2376750013839));
#32714=CARTESIAN_POINT('Ctrl Pts',(0.336978896961253,2.30385077591892,8.23871592441276));
#32715=CARTESIAN_POINT('Ctrl Pts',(0.32580270286489,2.32127714659387,8.23975684744161));
#32716=CARTESIAN_POINT('Ctrl Pts',(0.313326170479009,2.33772168788934,8.24079777047046));
#32717=CARTESIAN_POINT('Ctrl Pts',(0.300843230471275,2.35417467467263,8.24183922809025));
#32718=CARTESIAN_POINT('Ctrl Pts',(0.287059049901972,2.36964422880525,8.24288068571004));
#32719=CARTESIAN_POINT('Ctrl Pts',(0.27215868693709,2.38392699611815,8.24392214332984));
#32720=CARTESIAN_POINT('Ctrl Pts',(0.257253771261723,2.39821412743915,8.24496391916033));
#32721=CARTESIAN_POINT('Ctrl Pts',(0.241232550010455,2.41131326745835,8.24600569499083));
#32722=CARTESIAN_POINT('Ctrl Pts',(0.224314644421214,2.42306010322877,8.24704747082133));
#32723=CARTESIAN_POINT('Ctrl Pts',(0.207360170395124,2.43483233005128,8.24809149847393));
#32724=CARTESIAN_POINT('Ctrl Pts',(0.189505778677255,2.44524604587189,8.24913552612652));
#32725=CARTESIAN_POINT('Ctrl Pts',(0.170997974915739,2.45418156724301,8.25017955377912));
#32726=CARTESIAN_POINT('Ctrl Pts',(0.164452007320945,2.4573419440274,8.25054881267499));
#32727=CARTESIAN_POINT('Ctrl Pts',(0.157824486220507,2.46031784694963,8.25091807157086));
#32728=CARTESIAN_POINT('Ctrl Pts',(0.151126834759383,2.46310545274839,8.25128733046673));
#32729=CARTESIAN_POINT('Ctrl Pts',(0.132191345242563,2.47098652579104,8.25233129311428));
#32730=CARTESIAN_POINT('Ctrl Pts',(0.112581294539392,2.4774059003822,8.25337525576184));
#32731=CARTESIAN_POINT('Ctrl Pts',(0.0925476747723407,2.48225622021654,
8.25441921840939));
#32732=CARTESIAN_POINT('Ctrl Pts',(0.0725509090075942,2.48709761736488,
8.25546126057516));
#32733=CARTESIAN_POINT('Ctrl Pts',(0.0521328139093224,2.49037546025442,
8.25650330274093));
#32734=CARTESIAN_POINT('Ctrl Pts',(0.0315610518460417,2.49203161863091,
8.2575453449067));
#32735=CARTESIAN_POINT('Ctrl Pts',(0.0110113835320483,2.49368599831932,
8.25858626793556));
#32736=CARTESIAN_POINT('Ctrl Pts',(-0.00969089674527533,2.49372206354111,
8.25962719096441));
#32737=CARTESIAN_POINT('Ctrl Pts',(-0.0302715339130159,2.49213329906366,
8.26066811399327));
#32738=CARTESIAN_POINT('Ctrl Pts',(-0.0508627407596095,2.49054371863819,
8.26170957161306));
#32739=CARTESIAN_POINT('Ctrl Pts',(-0.0713314448536748,2.48732768198734,
8.26275102923285));
#32740=CARTESIAN_POINT('Ctrl Pts',(-0.0914064870398968,2.48253071004434,
8.26379248685264));
#32741=CARTESIAN_POINT('Ctrl Pts',(-0.111487663026712,2.47773227241727,
8.26483426268314));
#32742=CARTESIAN_POINT('Ctrl Pts',(-0.13117423103532,2.47135214391792,8.26587603851364));
#32743=CARTESIAN_POINT('Ctrl Pts',(-0.150209148853575,2.46348604044816,
8.26691781434414));
#32744=CARTESIAN_POINT('Ctrl Pts',(-0.169285211078648,2.45560293421725,
8.26796184199674));
#32745=CARTESIAN_POINT('Ctrl Pts',(-0.187706154637065,2.44622777452656,
8.26900586964933));
#32746=CARTESIAN_POINT('Ctrl Pts',(-0.205237909581819,2.43550304092584,
8.27004989730193));
#32747=CARTESIAN_POINT('Ctrl Pts',(-0.211438661503814,2.43170984322845,
8.27041915619779));
#32748=CARTESIAN_POINT('Ctrl Pts',(-0.217528450885799,2.42774821484854,
8.27078841509366));
#32749=CARTESIAN_POINT('Ctrl Pts',(-0.223497879506443,2.42362569097048,
8.27115767398952));
#32750=CARTESIAN_POINT('Ctrl Pts',(-0.24028556491258,2.41203201285784,8.27219613220238));
#32751=CARTESIAN_POINT('Ctrl Pts',(-0.256221330552324,2.39909216363466,
8.27323459041524));
#32752=CARTESIAN_POINT('Ctrl Pts',(-0.271080375257495,2.38495669872852,
8.2742730486281));
#32753=CARTESIAN_POINT('Ctrl Pts',(-0.285912087438807,2.37084723535475,
8.27530959664522));
#32754=CARTESIAN_POINT('Ctrl Pts',(-0.299670433632189,2.35554698333978,
8.27634614466234));
#32755=CARTESIAN_POINT('Ctrl Pts',(-0.312162814572205,2.33924729298021,
8.27738269267946));
#32756=CARTESIAN_POINT('Ctrl Pts',(-0.325220007064758,2.32221065315824,
8.27846610560549));
#32757=CARTESIAN_POINT('Ctrl Pts',(-0.336893256897875,2.30408251658651,
8.27954951853152));
#32758=CARTESIAN_POINT('Ctrl Pts',(-0.347008653253265,2.28512126989451,
8.28063293145755));
#32759=CARTESIAN_POINT('Ctrl Pts',(-0.356681299088095,2.26698995626181,
8.28166892344029));
#32760=CARTESIAN_POINT('Ctrl Pts',(-0.36492945832098,2.24809776107575,8.28270491542302));
#32761=CARTESIAN_POINT('Ctrl Pts',(-0.371647986438992,2.22869601460746,
8.28374090740576));
#32762=CARTESIAN_POINT('Ctrl Pts',(-0.378369177488813,2.20928657813223,
8.28477731001057));
#32763=CARTESIAN_POINT('Ctrl Pts',(-0.383559328269682,2.18936790464986,
8.28581371261539));
#32764=CARTESIAN_POINT('Ctrl Pts',(-0.387163296964183,2.16920600757033,
8.2868501152202));
#32765=CARTESIAN_POINT('Ctrl Pts',(-0.390774685009338,2.14900260397478,
8.28788865142689));
#32766=CARTESIAN_POINT('Ctrl Pts',(-0.392793313258072,2.12855571880385,
8.28892718763358));
#32767=CARTESIAN_POINT('Ctrl Pts',(-0.393215829492166,2.10813642653673,
8.28996572384026));
#32768=CARTESIAN_POINT('Ctrl Pts',(-0.393272505306007,2.10539740750289,
8.29010503182411));
#32769=CARTESIAN_POINT('Ctrl Pts',(-0.393300538581425,2.10265888024152,
8.29024433980797));
#32770=CARTESIAN_POINT('Ctrl Pts',(-0.393299992164447,2.09992149238468,
8.29038364779182));
#32771=CARTESIAN_POINT('',(-0.393299835176423,2.10036006971291,8.41538364626984));
#32772=CARTESIAN_POINT('Ctrl Pts',(-0.393299992164429,2.09992149229233,
8.29038364779652));
#32773=CARTESIAN_POINT('Ctrl Pts',(-0.393299149678696,2.09570089227957,
8.29059843770178));
#32774=CARTESIAN_POINT('Ctrl Pts',(-0.39323037085516,2.09148104825922,8.29081322760705));
#32775=CARTESIAN_POINT('Ctrl Pts',(-0.393093715813908,2.08726341538659,
8.29102801751231));
#32776=CARTESIAN_POINT('Ctrl Pts',(-0.392429519056185,2.06676407592866,
8.29207198015986));
#32777=CARTESIAN_POINT('Ctrl Pts',(-0.390155504155932,2.04625575286325,
8.29311594280742));
#32778=CARTESIAN_POINT('Ctrl Pts',(-0.386277842747431,2.02601136436999,
8.29415990545497));
#32779=CARTESIAN_POINT('Ctrl Pts',(-0.382407314714933,2.00580421761081,
8.29520194762074));
#32780=CARTESIAN_POINT('Ctrl Pts',(-0.376939074411953,1.98586076732159,
8.29624398978651));
#32781=CARTESIAN_POINT('Ctrl Pts',(-0.369931004579584,1.96644872950533,
8.29728603195228));
#32782=CARTESIAN_POINT('Ctrl Pts',(-0.362930461304121,1.94705753991273,
8.29832695498113));
#32783=CARTESIAN_POINT('Ctrl Pts',(-0.354393592969436,1.92819732813193,
8.29936787800998));
#32784=CARTESIAN_POINT('Ctrl Pts',(-0.344427996509661,1.91012044549152,
8.30040880103884));
#32785=CARTESIAN_POINT('Ctrl Pts',(-0.33445728197928,1.89203427903532,8.30145025865863));
#32786=CARTESIAN_POINT('Ctrl Pts',(-0.323056714546065,1.87473289755203,
8.30249171627842));
#32787=CARTESIAN_POINT('Ctrl Pts',(-0.310379978104497,1.85844429381227,
8.30353317389821));
#32788=CARTESIAN_POINT('Ctrl Pts',(-0.297699368367291,1.84215071319395,
8.30457494972871));
#32789=CARTESIAN_POINT('Ctrl Pts',(-0.283742293442603,1.82687108429887,
8.3056167255592));
#32790=CARTESIAN_POINT('Ctrl Pts',(-0.268702285995754,1.81279977106441,
8.3066585013897));
#32791=CARTESIAN_POINT('Ctrl Pts',(-0.253629769231506,1.79869804236707,
8.3077025290423));
#32792=CARTESIAN_POINT('Ctrl Pts',(-0.237470222471159,1.78581030287142,
8.30874655669489));
#32793=CARTESIAN_POINT('Ctrl Pts',(-0.220450237964016,1.77429064707686,
8.30979058434749));
#32794=CARTESIAN_POINT('Ctrl Pts',(-0.214430492537541,1.7702162958191,8.31015984324336));
#32795=CARTESIAN_POINT('Ctrl Pts',(-0.208303357573862,1.76631267554095,
8.31052910213923));
#32796=CARTESIAN_POINT('Ctrl Pts',(-0.202079582739162,1.7625852222561,8.3108983610351));
#32797=CARTESIAN_POINT('Ctrl Pts',(-0.184483829388642,1.75204702793388,
8.31194232368265));
#32798=CARTESIAN_POINT('Ctrl Pts',(-0.166009098811989,1.74285753453965,
8.3129862863302));
#32799=CARTESIAN_POINT('Ctrl Pts',(-0.146888206318207,1.73515928839476,
8.31403024897776));
#32800=CARTESIAN_POINT('Ctrl Pts',(-0.127802488766564,1.72747520400318,
8.31507229114353));
#32801=CARTESIAN_POINT('Ctrl Pts',(-0.108073621407342,1.72127724835857,
8.3161143333093));
#32802=CARTESIAN_POINT('Ctrl Pts',(-0.0879580376227832,1.71666167212559,
8.31715637547507));
#32803=CARTESIAN_POINT('Ctrl Pts',(-0.0678640576591956,1.71205105294898,
8.31819729850392));
#32804=CARTESIAN_POINT('Ctrl Pts',(-0.0473848928324123,1.7090196312728,
8.31923822153277));
#32805=CARTESIAN_POINT('Ctrl Pts',(-0.0267909688223041,1.70761354000225,
8.32027914456163));
#32806=CARTESIAN_POINT('Ctrl Pts',(-0.00618646830957055,1.70620672659988,
8.32132060218142));
#32807=CARTESIAN_POINT('Ctrl Pts',(0.0145321761589518,1.70642697740485,
8.32236205980121));
#32808=CARTESIAN_POINT('Ctrl Pts',(0.03509007231069,1.70826848885336,8.323403517421));
#32809=CARTESIAN_POINT('Ctrl Pts',(0.0556542497959508,1.7101105629639,8.3244452932515));
#32810=CARTESIAN_POINT('Ctrl Pts',(0.0760568521883709,1.71357478224715,
8.325487069082));
#32811=CARTESIAN_POINT('Ctrl Pts',(0.0960296920807883,1.71860363368424,
8.3265288449125));
#32812=CARTESIAN_POINT('Ctrl Pts',(0.116045703719874,1.72364335509783,8.32757287256509));
#32813=CARTESIAN_POINT('Ctrl Pts',(0.135629400480723,1.73025422508501,8.32861690021769));
#32814=CARTESIAN_POINT('Ctrl Pts',(0.154528558470463,1.73832913496241,8.32966092787029));
#32815=CARTESIAN_POINT('Ctrl Pts',(0.161212942925885,1.7411851247421,8.33003018676615));
#32816=CARTESIAN_POINT('Ctrl Pts',(0.167811905613704,1.74422382933159,8.33039944566202));
#32817=CARTESIAN_POINT('Ctrl Pts',(0.174315056847757,1.74743915283151,8.33076870455788));
#32818=CARTESIAN_POINT('Ctrl Pts',(0.192700658537479,1.75652946229004,8.33181266720544));
#32819=CARTESIAN_POINT('Ctrl Pts',(0.210428054593902,1.76708890771966,8.33285662985299));
#32820=CARTESIAN_POINT('Ctrl Pts',(0.227251362384367,1.77899889673951,8.33390059250054));
#32821=CARTESIAN_POINT('Ctrl Pts',(0.244043721887338,1.7908869760512,8.33494263466631));
#32822=CARTESIAN_POINT('Ctrl Pts',(0.259934666343468,1.80412029557966,8.33598467683208));
#32823=CARTESIAN_POINT('Ctrl Pts',(0.274704454447322,1.81853534376977,8.33702671899785));
#32824=CARTESIAN_POINT('Ctrl Pts',(0.289458380030778,1.83293491042458,8.33806764202671));
#32825=CARTESIAN_POINT('Ctrl Pts',(0.303092995607605,1.84851319555014,8.33910856505556));
#32826=CARTESIAN_POINT('Ctrl Pts',(0.315423125498342,1.86506779296815,8.34014948808442));
#32827=CARTESIAN_POINT('Ctrl Pts',(0.327759587822429,1.88163089239593,8.34119094570421));
#32828=CARTESIAN_POINT('Ctrl Pts',(0.338789773615118,1.89917072536003,8.342232403324));
#32829=CARTESIAN_POINT('Ctrl Pts',(0.348369758462629,1.91745301594195,8.34327386094379));
#32830=CARTESIAN_POINT('Ctrl Pts',(0.357952670413164,1.93574089256069,8.34431563677429));
#32831=CARTESIAN_POINT('Ctrl Pts',(0.366084190141754,1.95477101044075,8.34535741260479));
#32832=CARTESIAN_POINT('Ctrl Pts',(0.372667500935047,1.97428673997216,8.34639918843529));
#32833=CARTESIAN_POINT('Ctrl Pts',(0.379265041704014,1.99384465319582,8.34744321608789));
#32834=CARTESIAN_POINT('Ctrl Pts',(0.384307512766835,2.01388955944127,8.34848724374049));
#32835=CARTESIAN_POINT('Ctrl Pts',(0.387748439671595,2.03415140447782,8.34953127139308));
#32836=CARTESIAN_POINT('Ctrl Pts',(0.388965450414985,2.04131775347997,8.34990053028895));
#32837=CARTESIAN_POINT('Ctrl Pts',(0.389982590928619,2.04851118515848,8.35026978918482));
#32838=CARTESIAN_POINT('Ctrl Pts',(0.39079936262898,2.05571966385874,8.35063904808068));
#32839=CARTESIAN_POINT('Ctrl Pts',(0.393108526081241,2.07609935570369,8.35168301072824));
#32840=CARTESIAN_POINT('Ctrl Pts',(0.39382611510272,2.09672088631415,8.35272697337579));
#32841=CARTESIAN_POINT('Ctrl Pts',(0.392918743578669,2.11731331697162,8.35377093602334));
#32842=CARTESIAN_POINT('Ctrl Pts',(0.392013041262312,2.13786786563394,8.35481297818911));
#32843=CARTESIAN_POINT('Ctrl Pts',(0.389488284633596,2.15839269122189,8.35585502035488));
#32844=CARTESIAN_POINT('Ctrl Pts',(0.38536300719655,2.17861451955226,8.35689706252065));
#32845=CARTESIAN_POINT('Ctrl Pts',(0.381242160242664,2.19881462995668,8.3579379855495));
#32846=CARTESIAN_POINT('Ctrl Pts',(0.37552432296311,2.21871166607327,8.35897890857835));
#32847=CARTESIAN_POINT('Ctrl Pts',(0.368279443155349,2.23804036275375,8.36001983160721));
#32848=CARTESIAN_POINT('Ctrl Pts',(0.361030842566146,2.25737898614906,8.361061289227));
#32849=CARTESIAN_POINT('Ctrl Pts',(0.352253875842425,2.27614799236037,8.36210274684679));
#32850=CARTESIAN_POINT('Ctrl Pts',(0.342067617485302,2.2940995493759,8.36314420446658));
#32851=CARTESIAN_POINT('Ctrl Pts',(0.331878246782168,2.31205659137473,8.36418598029708));
#32852=CARTESIAN_POINT('Ctrl Pts',(0.320279121502411,2.32919506541326,8.36522775612758));
#32853=CARTESIAN_POINT('Ctrl Pts',(0.307433611780586,2.34529464802059,8.36626953195807));
#32854=CARTESIAN_POINT('Ctrl Pts',(0.294560336197995,2.36142903024107,8.36731355961067));
#32855=CARTESIAN_POINT('Ctrl Pts',(0.280435800833115,2.37651950013216,8.36835758726327));
#32856=CARTESIAN_POINT('Ctrl Pts',(0.265261914657696,2.39038079590795,8.36940161491586));
#32857=CARTESIAN_POINT('Ctrl Pts',(0.259895110012964,2.39528335453344,8.36977087381173));
#32858=CARTESIAN_POINT('Ctrl Pts',(0.254397340402247,2.40003251903327,8.3701401327076));
#32859=CARTESIAN_POINT('Ctrl Pts',(0.248778455727177,2.40462135507216,8.37050939160347));
#32860=CARTESIAN_POINT('Ctrl Pts',(0.232892837838741,2.41759483648032,8.37155335425102));
#32861=CARTESIAN_POINT('Ctrl Pts',(0.215942329588985,2.42936100530444,8.37259731689857));
#32862=CARTESIAN_POINT('Ctrl Pts',(0.198136668596248,2.43974512587759,8.37364127954613));
#32863=CARTESIAN_POINT('Ctrl Pts',(0.180363763035575,2.450110143742,8.3746833217119));
#32864=CARTESIAN_POINT('Ctrl Pts',(0.161739425814271,2.45909774211519,8.37572536387767));
#32865=CARTESIAN_POINT('Ctrl Pts',(0.142503463278991,2.46657557604605,8.37676740604344));
#32866=CARTESIAN_POINT('Ctrl Pts',(0.123288159865291,2.47404537890074,8.37780832907229));
#32867=CARTESIAN_POINT('Ctrl Pts',(0.103463207020081,2.48000834410828,8.37884925210114));
#32868=CARTESIAN_POINT('Ctrl Pts',(0.08328950843611,2.48437969221132,8.37989017513));
#32869=CARTESIAN_POINT('Ctrl Pts',(0.0631054491663324,2.48875328532482,
8.38093163274979));
#32870=CARTESIAN_POINT('Ctrl Pts',(0.0425730020190756,2.49153345675393,
8.38197309036958));
#32871=CARTESIAN_POINT('Ctrl Pts',(0.0219650057661074,2.49268617052513,
8.38301454798937));
#32872=CARTESIAN_POINT('Ctrl Pts',(0.00135071287185152,2.49383923650065,
8.38405632381987));
#32873=CARTESIAN_POINT('Ctrl Pts',(-0.0193384390504099,2.49336384995985,
8.38509809965037));
#32874=CARTESIAN_POINT('Ctrl Pts',(-0.0398287628758352,2.49127811036113,
8.38613987548087));
#32875=CARTESIAN_POINT('Ctrl Pts',(-0.0603633770011931,2.48918786238894,
8.38718390313347));
#32876=CARTESIAN_POINT('Ctrl Pts',(-0.0806975804783717,2.48548044418256,
8.38822793078606));
#32877=CARTESIAN_POINT('Ctrl Pts',(-0.100566304906113,2.48022533886832,
8.38927195843866));
#32878=CARTESIAN_POINT('Ctrl Pts',(-0.107593612301816,2.47836667700131,
8.38964121733452));
#32879=CARTESIAN_POINT('Ctrl Pts',(-0.114562836872709,2.47631486243418,
8.39001047623039));
#32880=CARTESIAN_POINT('Ctrl Pts',(-0.121462816175818,2.47407442345961,
8.39037973512625));
#32881=CARTESIAN_POINT('Ctrl Pts',(-0.140970323623923,2.46774029141898,
8.39142369777381));
#32882=CARTESIAN_POINT('Ctrl Pts',(-0.160039145429101,2.45985724037983,
8.39246766042136));
#32883=CARTESIAN_POINT('Ctrl Pts',(-0.178408825951557,2.45050703391314,
8.39351162306892));
#32884=CARTESIAN_POINT('Ctrl Pts',(-0.196744713467248,2.44117402815878,
8.39455366523469));
#32885=CARTESIAN_POINT('Ctrl Pts',(-0.214383337355163,2.43037950136081,
8.39559570740046));
#32886=CARTESIAN_POINT('Ctrl Pts',(-0.231083608102391,2.41825344627573,
8.39663774956623));
#32887=CARTESIAN_POINT('Ctrl Pts',(-0.247765943021182,2.40614041438332,
8.39767867259509));
#32888=CARTESIAN_POINT('Ctrl Pts',(-0.263511316120186,2.39269909988827,
8.39871959562394));
#32889=CARTESIAN_POINT('Ctrl Pts',(-0.278107211430637,2.37810298263463,
8.3997605186528));
#32890=CARTESIAN_POINT('Ctrl Pts',(-0.292710602812506,2.36349936919558,
8.40080197627259));
#32891=CARTESIAN_POINT('Ctrl Pts',(-0.306162805365953,2.34774027704241,
8.40184343389239));
#32892=CARTESIAN_POINT('Ctrl Pts',(-0.318287508478008,2.33103668961198,
8.40288489151218));
#32893=CARTESIAN_POINT('Ctrl Pts',(-0.330415916215455,2.31432799850737,
8.40392666734268));
#32894=CARTESIAN_POINT('Ctrl Pts',(-0.341215614465228,2.29667485382037,
8.40496844317318));
#32895=CARTESIAN_POINT('Ctrl Pts',(-0.350553669790102,2.27831717414958,
8.40601021900368));
#32896=CARTESIAN_POINT('Ctrl Pts',(-0.359911909533465,2.25991981393761,
8.40705424665628));
#32897=CARTESIAN_POINT('Ctrl Pts',(-0.367801917684434,2.24081555911867,
8.40809827430888));
#32898=CARTESIAN_POINT('Ctrl Pts',(-0.374138630584593,2.22126489642219,
8.40914230196147));
#32899=CARTESIAN_POINT('Ctrl Pts',(-0.376379842877265,2.21435008329185,
8.40951156085733));
#32900=CARTESIAN_POINT('Ctrl Pts',(-0.378427207638841,2.20737955019393,
8.40988081975319));
#32901=CARTESIAN_POINT('Ctrl Pts',(-0.380278489906803,2.20036513395697,
8.41025007864905));
#32902=CARTESIAN_POINT('Ctrl Pts',(-0.386974892832756,2.17499279704981,
8.41158575089821));
#32903=CARTESIAN_POINT('Ctrl Pts',(-0.391134538405294,2.14892449232814,
8.41292142314736));
#32904=CARTESIAN_POINT('Ctrl Pts',(-0.39264977411344,2.12260630196791,8.41425709539652));
#32905=CARTESIAN_POINT('Ctrl Pts',(-0.393075774356986,2.11520708649083,
8.41463261235429));
#32906=CARTESIAN_POINT('Ctrl Pts',(-0.393293034601751,2.10778825598276,
8.41500812931207));
#32907=CARTESIAN_POINT('Ctrl Pts',(-0.393299835176423,2.10036006971291,
8.41538364626984));
#32908=CARTESIAN_POINT('',(-0.393068738817681,2.09989474590746,8.54038365103395));
#32909=CARTESIAN_POINT('Ctrl Pts',(-0.393200853125335,2.10035994890194,
8.41538364779652));
#32910=CARTESIAN_POINT('Ctrl Pts',(-0.392329112146126,2.00321302993875,
8.42029590592163));
#32911=CARTESIAN_POINT('Ctrl Pts',(-0.306910870380854,1.77370848694128,
8.43183161188765));
#32912=CARTESIAN_POINT('Ctrl Pts',(0.0781045900267053,1.64155184207887,
8.44999076569464));
#32913=CARTESIAN_POINT('Ctrl Pts',(0.427750845253811,1.91750546619381,8.4698611092174));
#32914=CARTESIAN_POINT('Ctrl Pts',(0.384993932979691,2.3608729806885,8.4897314527402));
#32915=CARTESIAN_POINT('Ctrl Pts',(-0.0109425006120916,2.56492505005092,
8.509601796263));
#32916=CARTESIAN_POINT('Ctrl Pts',(-0.338844730225498,2.37590380025287,
8.52648586128176));
#32917=CARTESIAN_POINT('Ctrl Pts',(-0.392506215664613,2.17206643209509,
8.53674647845961));
#32918=CARTESIAN_POINT('Ctrl Pts',(-0.392678456924488,2.09989491469267,
8.54038364779652));
#32919=CARTESIAN_POINT('',(-0.393364049700885,2.09968468653314,8.66538364779653));
#32920=CARTESIAN_POINT('Ctrl Pts',(-0.393299985889287,2.09989464590004,
8.54038365295217));
#32921=CARTESIAN_POINT('Ctrl Pts',(-0.393294038661158,2.07769290206561,
8.5415007688402));
#32922=CARTESIAN_POINT('Ctrl Pts',(-0.391403923263078,2.05554353096737,
8.54261788472822));
#32923=CARTESIAN_POINT('Ctrl Pts',(-0.38768122540452,2.03375683077592,8.54373500061624));
#32924=CARTESIAN_POINT('Ctrl Pts',(-0.383937656161153,2.01184798298596,
8.54485837963828));
#32925=CARTESIAN_POINT('Ctrl Pts',(-0.37834109873788,1.99030641866694,8.54598175866031));
#32926=CARTESIAN_POINT('Ctrl Pts',(-0.370993975156392,1.96943062994079,
8.54710513768235));
#32927=CARTESIAN_POINT('Ctrl Pts',(-0.366116412467435,1.95557174121191,
8.54785091955775));
#32928=CARTESIAN_POINT('Ctrl Pts',(-0.360468356591718,1.94200590930795,
8.54859670143316));
#32929=CARTESIAN_POINT('Ctrl Pts',(-0.354091051801312,1.92881467050521,
8.54934248330856));
#32930=CARTESIAN_POINT('Ctrl Pts',(-0.345163953660686,1.91034927058176,
8.55038644595611));
#32931=CARTESIAN_POINT('Ctrl Pts',(-0.334761946975892,1.89252903725973,
8.55143040860367));
#32932=CARTESIAN_POINT('Ctrl Pts',(-0.32300144151329,1.87560089398499,8.55247437125122));
#32933=CARTESIAN_POINT('Ctrl Pts',(-0.311262570767752,1.85870389185391,
8.55351641341699));
#32934=CARTESIAN_POINT('Ctrl Pts',(-0.298170528088468,1.84269635363174,
8.55455845558276));
#32935=CARTESIAN_POINT('Ctrl Pts',(-0.283886872206727,1.82779946034462,
8.55560049774853));
#32936=CARTESIAN_POINT('Ctrl Pts',(-0.269618556747013,1.81291856608686,
8.55664142077739));
#32937=CARTESIAN_POINT('Ctrl Pts',(-0.25416165451208,1.79914649715438,8.55768234380624));
#32938=CARTESIAN_POINT('Ctrl Pts',(-0.23771692350351,1.78667021482147,8.55872326683509));
#32939=CARTESIAN_POINT('Ctrl Pts',(-0.221263746909695,1.77418752499511,
8.55976472445489));
#32940=CARTESIAN_POINT('Ctrl Pts',(-0.203822304452074,1.7630024088121,8.56080618207468));
#32941=CARTESIAN_POINT('Ctrl Pts',(-0.185625588014758,1.75326086019289,
8.56184763969447));
#32942=CARTESIAN_POINT('Ctrl Pts',(-0.167423311687262,1.74351633510588,
8.56288941552497));
#32943=CARTESIAN_POINT('Ctrl Pts',(-0.148465967176074,1.73521657072913,
8.56393119135547));
#32944=CARTESIAN_POINT('Ctrl Pts',(-0.129009316447134,1.72846065313369,
8.56497296718597));
#32945=CARTESIAN_POINT('Ctrl Pts',(-0.109510609726116,1.72169013246906,
8.56601699483857));
#32946=CARTESIAN_POINT('Ctrl Pts',(-0.089511154700245,1.71647030685164,
8.56706102249117));
#32947=CARTESIAN_POINT('Ctrl Pts',(-0.0692805833476899,1.71285004097765,
8.56810505014377));
#32948=CARTESIAN_POINT('Ctrl Pts',(-0.0621252954376586,1.71156960039158,
8.56847430903963));
#32949=CARTESIAN_POINT('Ctrl Pts',(-0.0549411555171371,1.71048878230323,
8.5688435679355));
#32950=CARTESIAN_POINT('Ctrl Pts',(-0.0477401943522662,1.70960819188512,
8.56921282683136));
#32951=CARTESIAN_POINT('Ctrl Pts',(-0.0273817559590799,1.70711860120878,
8.57025678947892));
#32952=CARTESIAN_POINT('Ctrl Pts',(-0.00676739055080256,1.70621838038248,
8.57130075212647));
#32953=CARTESIAN_POINT('Ctrl Pts',(0.0138322695083255,1.70694331411328,
8.57234471477402));
#32954=CARTESIAN_POINT('Ctrl Pts',(0.0343940342730368,1.70766691425037,
8.57338675693979));
#32955=CARTESIAN_POINT('Ctrl Pts',(0.0549404182758393,1.71000976846255,
8.57442879910556));
#32956=CARTESIAN_POINT('Ctrl Pts',(0.07519799388942,1.71395576456187,8.57547084127133));
#32957=CARTESIAN_POINT('Ctrl Pts',(0.095433813185032,1.71789752272338,8.57651176430019));
#32958=CARTESIAN_POINT('Ctrl Pts',(0.115380715792135,1.72343889311018,8.57755268732904));
#32959=CARTESIAN_POINT('Ctrl Pts',(0.134772827390175,1.73051228031603,8.57859361035789));
#32960=CARTESIAN_POINT('Ctrl Pts',(0.154174898271309,1.7375893002292,8.57963506797769));
#32961=CARTESIAN_POINT('Ctrl Pts',(0.173020912169774,1.74619967183376,8.58067652559748));
#32962=CARTESIAN_POINT('Ctrl Pts',(0.191061992066552,1.75622652052905,8.58171798321727));
#32963=CARTESIAN_POINT('Ctrl Pts',(0.209108584299766,1.76625643286376,8.58275975904776));
#32964=CARTESIAN_POINT('Ctrl Pts',(0.226349127911292,1.77770329512398,8.58380153487826));
#32965=CARTESIAN_POINT('Ctrl Pts',(0.242561860985024,1.79040569515012,8.58484331070876));
#32966=CARTESIAN_POINT('Ctrl Pts',(0.258809638249209,1.80313555170217,8.58588733836136));
#32967=CARTESIAN_POINT('Ctrl Pts',(0.274024627458827,1.81712586564286,8.58693136601395));
#32968=CARTESIAN_POINT('Ctrl Pts',(0.28801978564067,1.83217637692036,8.58797539366655));
#32969=CARTESIAN_POINT('Ctrl Pts',(0.292969689644507,1.83749954548083,8.58834465256242));
#32970=CARTESIAN_POINT('Ctrl Pts',(0.297767365592751,1.84295503259325,8.58871391145828));
#32971=CARTESIAN_POINT('Ctrl Pts',(0.302405792174401,1.84853305016489,8.58908317035415));
#32972=CARTESIAN_POINT('Ctrl Pts',(0.31551947514552,1.86430312925404,8.5901271330017));
#32973=CARTESIAN_POINT('Ctrl Pts',(0.327435325407625,1.88114875097759,8.59117109564925));
#32974=CARTESIAN_POINT('Ctrl Pts',(0.337976756349517,1.89886173370674,8.59221505829681));
#32975=CARTESIAN_POINT('Ctrl Pts',(0.348498795193288,1.91654213149547,8.59325710046258));
#32976=CARTESIAN_POINT('Ctrl Pts',(0.357651010334645,1.93508612835312,8.59429914262835));
#32977=CARTESIAN_POINT('Ctrl Pts',(0.365298937874502,1.95425509961662,8.59534118479412));
#32978=CARTESIAN_POINT('Ctrl Pts',(0.372938651660327,1.97340348370612,8.59638210782297));
#32979=CARTESIAN_POINT('Ctrl Pts',(0.379076987023166,1.99317484047176,8.59742303085183));
#32980=CARTESIAN_POINT('Ctrl Pts',(0.383626856817083,2.01330902740974,8.59846395388068));
#32981=CARTESIAN_POINT('Ctrl Pts',(0.38817906330554,2.03345355474136,8.59950541150047));
#32982=CARTESIAN_POINT('Ctrl Pts',(0.39114099654613,2.05396057038255,8.60054686912027));
#32983=CARTESIAN_POINT('Ctrl Pts',(0.392476205168331,2.0745575477466,8.60158832674006));
#32984=CARTESIAN_POINT('Ctrl Pts',(0.393811821754976,2.0951608183852,8.60263010257056));
#32985=CARTESIAN_POINT('Ctrl Pts',(0.393519712791342,2.11585336950821,8.60367187840105));
#32986=CARTESIAN_POINT('Ctrl Pts',(0.391615552779024,2.13636136440756,8.60471365423155));
#32987=CARTESIAN_POINT('Ctrl Pts',(0.38970727688163,2.15691368780326,8.60575768188415));
#32988=CARTESIAN_POINT('Ctrl Pts',(0.386180119008918,2.17727993287075,8.60680170953675));
#32989=CARTESIAN_POINT('Ctrl Pts',(0.381101211656955,2.19719442614472,8.60784573718934));
#32990=CARTESIAN_POINT('Ctrl Pts',(0.379304868699628,2.20423792138146,8.60821499608521));
#32991=CARTESIAN_POINT('Ctrl Pts',(0.377314866137651,2.21122504696654,8.60858425498108));
#32992=CARTESIAN_POINT('Ctrl Pts',(0.375135633212143,2.21814460078448,8.60895351387694));
#32993=CARTESIAN_POINT('Ctrl Pts',(0.36897454190192,2.23770744897722,8.6099974765245));
#32994=CARTESIAN_POINT('Ctrl Pts',(0.3612607065989,2.25684534864359,8.61104143917205));
#32995=CARTESIAN_POINT('Ctrl Pts',(0.352073580620603,2.27529713012194,8.61208540181961));
#32996=CARTESIAN_POINT('Ctrl Pts',(0.342903355350511,2.29371496755997,8.61312744398538));
#32997=CARTESIAN_POINT('Ctrl Pts',(0.332265490199807,2.3114485144834,8.61416948615115));
#32998=CARTESIAN_POINT('Ctrl Pts',(0.320287837319435,2.32825553939661,8.61521152831692));
#32999=CARTESIAN_POINT('Ctrl Pts',(0.308323048250094,2.3450445138291,8.61625245134577));
#33000=CARTESIAN_POINT('Ctrl Pts',(0.295021729332165,2.36090832876827,8.61729337437462));
#33001=CARTESIAN_POINT('Ctrl Pts',(0.280555471194879,2.37563293994481,8.61833429740348));
#33002=CARTESIAN_POINT('Ctrl Pts',(0.266081783564447,2.39036511329788,8.61937575502327));
#33003=CARTESIAN_POINT('Ctrl Pts',(0.250442465629713,2.403956377903,8.62041721264306));
#33004=CARTESIAN_POINT('Ctrl Pts',(0.2338469308387,2.41622856122956,8.62145867026286));
#33005=CARTESIAN_POINT('Ctrl Pts',(0.217246325388308,2.42850449424316,8.62250044609335));
#33006=CARTESIAN_POINT('Ctrl Pts',(0.199689534056603,2.43946013561006,8.62354222192385));
#33007=CARTESIAN_POINT('Ctrl Pts',(0.181415288541559,2.44896043197386,8.62458399775435));
#33008=CARTESIAN_POINT('Ctrl Pts',(0.163101542830138,2.45848126344384,8.62562802540695));
#33009=CARTESIAN_POINT('Ctrl Pts',(0.144067925044122,2.4665401824026,8.62667205305954));
#33010=CARTESIAN_POINT('Ctrl Pts',(0.124574158222978,2.47304982120762,8.62771608071214));
#33011=CARTESIAN_POINT('Ctrl Pts',(0.117679468417838,2.47535219512621,8.628085339608));
#33012=CARTESIAN_POINT('Ctrl Pts',(0.110727343781885,2.47746122267087,8.62845459850387));
#33013=CARTESIAN_POINT('Ctrl Pts',(0.103729600882616,2.47937456411933,8.62882385739973));
#33014=CARTESIAN_POINT('Ctrl Pts',(0.0839456978113508,2.48478393144011,
8.62986782004729));
#33015=CARTESIAN_POINT('Ctrl Pts',(0.0636785706898904,2.48865769149517,
8.63091178269484));
#33016=CARTESIAN_POINT('Ctrl Pts',(0.0431908251622427,2.49092127419956,
8.63195574534239));
#33017=CARTESIAN_POINT('Ctrl Pts',(0.0227407690501717,2.49318069279964,
8.63299778750816));
#33018=CARTESIAN_POINT('Ctrl Pts',(0.00207161666862456,2.49383567469102,
8.63403982967393));
#33019=CARTESIAN_POINT('Ctrl Pts',(-0.0185437507244163,2.49286259596591,
8.6350818718397));
#33020=CARTESIAN_POINT('Ctrl Pts',(-0.039136977536738,2.49189056231205,
8.63612279486855));
#33021=CARTESIAN_POINT('Ctrl Pts',(-0.0596758014392799,2.48929394488147,
8.6371637178974));
#33022=CARTESIAN_POINT('Ctrl Pts',(-0.079887365070007,2.4851011541169,8.63820464092625));
#33023=CARTESIAN_POINT('Ctrl Pts',(-0.100109308833038,2.48090621004428,
8.63924609854604));
#33024=CARTESIAN_POINT('Ctrl Pts',(-0.120002932838844,2.47511358862173,
8.64028755616583));
#33025=CARTESIAN_POINT('Ctrl Pts',(-0.139305067150353,2.46780292041559,
8.64132901378562));
#33026=CARTESIAN_POINT('Ctrl Pts',(-0.158613099105392,2.46049001848159,
8.64237078961612));
#33027=CARTESIAN_POINT('Ctrl Pts',(-0.177328606899627,2.45165844061416,
8.64341256544661));
#33028=CARTESIAN_POINT('Ctrl Pts',(-0.195208805471213,2.4414358098772,8.64445434127711));
#33029=CARTESIAN_POINT('Ctrl Pts',(-0.213127652497767,2.43119108269193,
8.64549836892971));
#33030=CARTESIAN_POINT('Ctrl Pts',(-0.230206977071488,2.41954971452007,
8.6465423965823));
#33031=CARTESIAN_POINT('Ctrl Pts',(-0.24623272614012,2.40668279145985,8.6475864242349));
#33032=CARTESIAN_POINT('Ctrl Pts',(-0.251900823524189,2.40213192942985,
8.64795568313077));
#33033=CARTESIAN_POINT('Ctrl Pts',(-0.257437442327009,2.39742811328002,
8.64832494202664));
#33034=CARTESIAN_POINT('Ctrl Pts',(-0.2628342187467,2.39258001205792,8.64869420092251));
#33035=CARTESIAN_POINT('Ctrl Pts',(-0.277864808745112,2.37907754019818,
8.64972262578866));
#33036=CARTESIAN_POINT('Ctrl Pts',(-0.291903284089961,2.36436757417959,
8.65075105065482));
#33037=CARTESIAN_POINT('Ctrl Pts',(-0.304747731190058,2.34862363189068,
8.65177947552097));
#33038=CARTESIAN_POINT('Ctrl Pts',(-0.317568308372067,2.33290894789603,
8.65280598917857));
#33039=CARTESIAN_POINT('Ctrl Pts',(-0.329198735141888,2.31616464048174,
8.65383250283615));
#33040=CARTESIAN_POINT('Ctrl Pts',(-0.339474010293861,2.29860082158693,
8.65485901649375));
#33041=CARTESIAN_POINT('Ctrl Pts',(-0.349744380750245,2.28104538642723,
8.65588504016572));
#33042=CARTESIAN_POINT('Ctrl Pts',(-0.358660462020373,2.26267184650269,
8.6569110638377));
#33043=CARTESIAN_POINT('Ctrl Pts',(-0.366100711712632,2.24371902756248,
8.65793708750967));
#33044=CARTESIAN_POINT('Ctrl Pts',(-0.373538861149918,2.22477155867822,
8.65896282155275));
#33045=CARTESIAN_POINT('Ctrl Pts',(-0.379501738069724,2.20524584583435,
8.65998855559583));
#33046=CARTESIAN_POINT('Ctrl Pts',(-0.383916419493351,2.18539948971396,
8.66101428963891));
#33047=CARTESIAN_POINT('Ctrl Pts',(-0.388337722225733,2.16552336726642,
8.6620415621173));
#33048=CARTESIAN_POINT('Ctrl Pts',(-0.391206066234724,2.14532639112539,
8.66306883459569));
#33049=CARTESIAN_POINT('Ctrl Pts',(-0.392499829559989,2.12507536231801,
8.66409610707408));
#33050=CARTESIAN_POINT('Ctrl Pts',(-0.393040345992751,2.11661476242546,
8.6645252873149));
#33051=CARTESIAN_POINT('Ctrl Pts',(-0.393306655044755,2.10814475890454,
8.66495446755571));
#33052=CARTESIAN_POINT('Ctrl Pts',(-0.393299873645868,2.0996847379755,8.66538364779653));
#33053=CARTESIAN_POINT('',(-0.393416716470155,2.1002762343866,8.79038364779653));
#33054=CARTESIAN_POINT('Ctrl Pts',(-0.393587260541253,2.09968450761139,
8.66538364779653));
#33055=CARTESIAN_POINT('Ctrl Pts',(-0.393770050696924,2.0787684143503,8.66644394667946));
#33056=CARTESIAN_POINT('Ctrl Pts',(-0.382732713030496,1.92738745922455,
8.67412769340335));
#33057=CARTESIAN_POINT('Ctrl Pts',(-0.186276276076986,1.67388242296857,
8.68843488796805));
#33058=CARTESIAN_POINT('Ctrl Pts',(0.257452574101791,1.71271042800903,8.70830523149091));
#33059=CARTESIAN_POINT('Ctrl Pts',(0.465003736545269,2.10682389063747,8.72817557501367));
#33060=CARTESIAN_POINT('Ctrl Pts',(0.245977275250812,2.49467736259462,8.74804591853647));
#33061=CARTESIAN_POINT('Ctrl Pts',(-0.198699849304038,2.52046808484241,
8.76791626205924));
#33062=CARTESIAN_POINT('Ctrl Pts',(-0.385062938840621,2.26483280350818,
8.78202883847928));
#33063=CARTESIAN_POINT('Ctrl Pts',(-0.39382877298102,2.11734147947392,8.78951796705837));
#33064=CARTESIAN_POINT('Ctrl Pts',(-0.393692564686641,2.10027642807121,
8.79038364779653));
#33065=CARTESIAN_POINT('',(-0.393299965593714,2.10016451134769,8.91538364779289));
#33066=CARTESIAN_POINT('Ctrl Pts',(-0.393299903050929,2.100276152367,8.79038364779653));
#33067=CARTESIAN_POINT('Ctrl Pts',(-0.393314122120435,2.08002516296271,
8.79141197759652));
#33068=CARTESIAN_POINT('Ctrl Pts',(-0.391759973089012,2.05971329987927,
8.79244030739651));
#33069=CARTESIAN_POINT('Ctrl Pts',(-0.388635608644073,2.03960750300037,
8.79346863719649));
#33070=CARTESIAN_POINT('Ctrl Pts',(-0.385515976401287,2.0195321586173,8.79449540947508));
#33071=CARTESIAN_POINT('Ctrl Pts',(-0.380830912048011,1.99966301204038,
8.79552218175366));
#33072=CARTESIAN_POINT('Ctrl Pts',(-0.37463042075924,1.98026304730053,8.79654895403225));
#33073=CARTESIAN_POINT('Ctrl Pts',(-0.368429200823891,1.96086080278683,
8.79757584697129));
#33074=CARTESIAN_POINT('Ctrl Pts',(-0.360712391440744,1.94192858389374,
8.79860273991033));
#33075=CARTESIAN_POINT('Ctrl Pts',(-0.351580247434861,1.92371551510799,
8.79962963284937));
#33076=CARTESIAN_POINT('Ctrl Pts',(-0.342448079966206,1.90550239952829,
8.80065652842676));
#33077=CARTESIAN_POINT('Ctrl Pts',(-0.331900931995182,1.88800910537307,
8.80168342400414));
#33078=CARTESIAN_POINT('Ctrl Pts',(-0.320085107705698,1.87146025766832,
8.80271031958153));
#33079=CARTESIAN_POINT('Ctrl Pts',(-0.308243682958548,1.85487555482009,
8.80373944005632));
#33080=CARTESIAN_POINT('Ctrl Pts',(-0.295128573858232,1.83923997386343,
8.80476856053111));
#33081=CARTESIAN_POINT('Ctrl Pts',(-0.280926850596252,1.82474558202624,
8.8057976810059));
#33082=CARTESIAN_POINT('Ctrl Pts',(-0.272374301224326,1.81601678204072,
8.80641743703888));
#33083=CARTESIAN_POINT('Ctrl Pts',(-0.263428410976905,1.80770115207403,
8.80703719307185));
#33084=CARTESIAN_POINT('Ctrl Pts',(-0.254135713613598,1.79983349776148,
8.80765694910483));
#33085=CARTESIAN_POINT('Ctrl Pts',(-0.23848241065873,1.78658064213909,8.80870091175239));
#33086=CARTESIAN_POINT('Ctrl Pts',(-0.221742997184422,1.77451604536762,
8.80974487439994));
#33087=CARTESIAN_POINT('Ctrl Pts',(-0.204124082495864,1.76381813114741,
8.81078883704749));
#33088=CARTESIAN_POINT('Ctrl Pts',(-0.186537579699419,1.75313989689317,
8.81183087921326));
#33089=CARTESIAN_POINT('Ctrl Pts',(-0.168075378184561,1.7438237830749,8.81287292137903));
#33090=CARTESIAN_POINT('Ctrl Pts',(-0.148974902208042,1.73600636198952,
8.8139149635448));
#33091=CARTESIAN_POINT('Ctrl Pts',(-0.129894939842656,1.72819733669157,
8.81495588657366));
#33092=CARTESIAN_POINT('Ctrl Pts',(-0.110178730435513,1.7218841127929,8.81599680960251));
#33093=CARTESIAN_POINT('Ctrl Pts',(-0.0900856348904587,1.71715607829511,
8.81703773263137));
#33094=CARTESIAN_POINT('Ctrl Pts',(-0.0699822200552296,1.71242561560202,
8.81807919025116));
#33095=CARTESIAN_POINT('Ctrl Pts',(-0.0495022449195084,1.70928215294598,
8.81912064787095));
#33096=CARTESIAN_POINT('Ctrl Pts',(-0.0289179025022455,1.70776455423449,
8.82016210549074));
#33097=CARTESIAN_POINT('Ctrl Pts',(-0.00832727067096913,1.70624649183043,
8.82120388132124));
#33098=CARTESIAN_POINT('Ctrl Pts',(0.0123670560961123,1.70635530029777,
8.82224565715174));
#33099=CARTESIAN_POINT('Ctrl Pts',(0.0328911129931427,1.70807773132154,
8.82328743298224));
#33100=CARTESIAN_POINT('Ctrl Pts',(0.053459533104898,1.70980388541905,8.82433146063484));
#33101=CARTESIAN_POINT('Ctrl Pts',(0.0738562218082703,1.71315050621404,
8.82537548828743));
#33102=CARTESIAN_POINT('Ctrl Pts',(0.0938149214189155,1.71805281710796,
8.82641951594003));
#33103=CARTESIAN_POINT('Ctrl Pts',(0.100874051857501,1.71978670021287,8.8267887748359));
#33104=CARTESIAN_POINT('Ctrl Pts',(0.107878530240366,1.72171473463223,8.82715803373176));
#33105=CARTESIAN_POINT('Ctrl Pts',(0.114817115658489,1.72383259052403,8.82752729262763));
#33106=CARTESIAN_POINT('Ctrl Pts',(0.134433769676722,1.72982015769892,8.82857125527518));
#33107=CARTESIAN_POINT('Ctrl Pts',(0.153639245627005,1.73736417203118,8.82961521792274));
#33108=CARTESIAN_POINT('Ctrl Pts',(0.172171680317429,1.7463874966907,8.83065918057029));
#33109=CARTESIAN_POINT('Ctrl Pts',(0.190670022597255,1.75539422197218,8.83170122273606));
#33110=CARTESIAN_POINT('Ctrl Pts',(0.208497101165738,1.7658745908189,8.83274326490183));
#33111=CARTESIAN_POINT('Ctrl Pts',(0.225409561550228,1.77770290171686,8.8337853070676));
#33112=CARTESIAN_POINT('Ctrl Pts',(0.242303858217949,1.78951850919473,8.83482623009645));
#33113=CARTESIAN_POINT('Ctrl Pts',(0.258284870307714,1.80267878890176,8.8358671531253));
#33114=CARTESIAN_POINT('Ctrl Pts',(0.273137042043731,1.81701405288672,8.83690807615416));
#33115=CARTESIAN_POINT('Ctrl Pts',(0.287996841468064,1.83135667908964,8.83794953377395));
#33116=CARTESIAN_POINT('Ctrl Pts',(0.301726101741667,1.84687499573061,8.83899099139374));
#33117=CARTESIAN_POINT('Ctrl Pts',(0.314144802395893,1.86336117578122,8.84003244901353));
#33118=CARTESIAN_POINT('Ctrl Pts',(0.326567297504571,1.87985239307857,8.84107422484403));
#33119=CARTESIAN_POINT('Ctrl Pts',(0.337678022398854,1.89731145353291,8.84211600067452));
#33120=CARTESIAN_POINT('Ctrl Pts',(0.347339814399537,1.91550083107804,8.84315777650502));
#33121=CARTESIAN_POINT('Ctrl Pts',(0.357022490582887,1.93372952537551,8.84420180415761));
#33122=CARTESIAN_POINT('Ctrl Pts',(0.365249688039197,1.95269101273338,8.84524583181021));
#33123=CARTESIAN_POINT('Ctrl Pts',(0.371931741996789,1.97212635418025,8.84628985946281));
#33124=CARTESIAN_POINT('Ctrl Pts',(0.37429509689488,1.97900037969637,8.84665911835867));
#33125=CARTESIAN_POINT('Ctrl Pts',(0.376465621746349,1.98593355040014,8.84702837725454));
#33126=CARTESIAN_POINT('Ctrl Pts',(0.378440872252739,1.99291407091225,8.84739763615041));
#33127=CARTESIAN_POINT('Ctrl Pts',(0.3840252678389,2.01264928313513,8.84844159879796));
#33128=CARTESIAN_POINT('Ctrl Pts',(0.388078396670224,2.03288130244609,8.84948556144552));
#33129=CARTESIAN_POINT('Ctrl Pts',(0.390523365497208,2.05334819402495,8.85052952409307));
#33130=CARTESIAN_POINT('Ctrl Pts',(0.392963836540573,2.07377743455131,8.85157156625884));
#33131=CARTESIAN_POINT('Ctrl Pts',(0.393801874513695,2.09443997441952,8.85261360842461));
#33132=CARTESIAN_POINT('Ctrl Pts',(0.393011439326963,2.11506315233106,8.85365565059038));
#33133=CARTESIAN_POINT('Ctrl Pts',(0.392221853055205,2.13566418127351,8.85469657361923));
#33134=CARTESIAN_POINT('Ctrl Pts',(0.389807264853583,2.15622519956534,8.85573749664809));
#33135=CARTESIAN_POINT('Ctrl Pts',(0.385793667153384,2.17647310889682,8.85677841967694));
#33136=CARTESIAN_POINT('Ctrl Pts',(0.381778008174011,2.1967314170268,8.85781987729673));
#33137=CARTESIAN_POINT('Ctrl Pts',(0.376161826354476,2.21667557007474,8.85886133491653));
#33138=CARTESIAN_POINT('Ctrl Pts',(0.369022418048841,2.23604170308176,8.85990279253632));
#33139=CARTESIAN_POINT('Ctrl Pts',(0.361880828342715,2.25541375328672,8.86094456836682));
#33140=CARTESIAN_POINT('Ctrl Pts',(0.35321537386231,2.27420675459767,8.86198634419732));
#33141=CARTESIAN_POINT('Ctrl Pts',(0.343151522140229,2.29217680102667,8.86302812002782));
#33142=CARTESIAN_POINT('Ctrl Pts',(0.33306591717428,2.3101856901188,8.86407214768041));
#33143=CARTESIAN_POINT('Ctrl Pts',(0.321576289749156,2.32736746076212,8.86511617533301));
#33144=CARTESIAN_POINT('Ctrl Pts',(0.308851823227105,2.34350655286725,8.86616020298561));
#33145=CARTESIAN_POINT('Ctrl Pts',(0.30435134620741,2.34921473819762,8.86652946188148));
#33146=CARTESIAN_POINT('Ctrl Pts',(0.299696756466525,2.35479280493104,8.86689872077734));
#33147=CARTESIAN_POINT('Ctrl Pts',(0.294896648627635,2.36023231280567,8.86726797967321));
#33148=CARTESIAN_POINT('Ctrl Pts',(0.281325863078232,2.37561079956858,8.86831194232076));
#33149=CARTESIAN_POINT('Ctrl Pts',(0.266508450871526,2.38997070048114,8.86935590496832));
#33150=CARTESIAN_POINT('Ctrl Pts',(0.250623027788763,2.40310557227143,8.87039986761587));
#33151=CARTESIAN_POINT('Ctrl Pts',(0.23476682765352,2.41621628104969,8.87144190978164));
#33152=CARTESIAN_POINT('Ctrl Pts',(0.217847039279517,2.42810592456112,8.87248395194741));
#33153=CARTESIAN_POINT('Ctrl Pts',(0.200078825197363,2.43860501134455,8.87352599411317));
#33154=CARTESIAN_POINT('Ctrl Pts',(0.182329693897984,2.44909282227373,8.87456691714203));
#33155=CARTESIAN_POINT('Ctrl Pts',(0.163734561363448,2.45819264399749,8.87560784017088));
#33156=CARTESIAN_POINT('Ctrl Pts',(0.14453712371496,2.46577849836781,8.87664876319974));
#33157=CARTESIAN_POINT('Ctrl Pts',(0.125329826762846,2.47336824863521,8.87769022081953));
#33158=CARTESIAN_POINT('Ctrl Pts',(0.105520285095474,2.4794421928199,8.87873167843932));
#33159=CARTESIAN_POINT('Ctrl Pts',(0.0853722030077162,2.48392248821033,
8.87977313605911));
#33160=CARTESIAN_POINT('Ctrl Pts',(0.0652179648025095,2.48840415252632,
8.8808149118896));
#33161=CARTESIAN_POINT('Ctrl Pts',(0.0447257057380876,2.49129107442718,
8.8818566877201));
#33162=CARTESIAN_POINT('Ctrl Pts',(0.0241684241785611,2.49255671854233,
8.8828984635506));
#33163=CARTESIAN_POINT('Ctrl Pts',(0.00356670758843661,2.49382509837597,
8.88394249120319));
#33164=CARTESIAN_POINT('Ctrl Pts',(-0.0170995757271018,2.49346521682634,
8.88498651885579));
#33165=CARTESIAN_POINT('Ctrl Pts',(-0.0375575969745094,2.49150263972226,
8.88603054650839));
#33166=CARTESIAN_POINT('Ctrl Pts',(-0.044793330931032,2.49080850192553,
8.88639980540425));
#33167=CARTESIAN_POINT('Ctrl Pts',(-0.0520030828421718,2.4899143478459,
8.88676906430012));
#33168=CARTESIAN_POINT('Ctrl Pts',(-0.0591751035598244,2.4888228351302,
8.88713832319599));
#33169=CARTESIAN_POINT('Ctrl Pts',(-0.0794517219988305,2.48573692842009,
8.88818228584354));
#33170=CARTESIAN_POINT('Ctrl Pts',(-0.0995467167524269,2.48105145677097,
8.88922624849109));
#33171=CARTESIAN_POINT('Ctrl Pts',(-0.119189818671564,2.47480485205643,
8.89027021113865));
#33172=CARTESIAN_POINT('Ctrl Pts',(-0.138796784988069,2.46856973864436,
8.89131225330442));
#33173=CARTESIAN_POINT('Ctrl Pts',(-0.157952797297252,2.46077935650606,
8.89235429547019));
#33174=CARTESIAN_POINT('Ctrl Pts',(-0.176398872778384,2.45152286935919,
8.89339633763596));
#33175=CARTESIAN_POINT('Ctrl Pts',(-0.194825137464267,2.44227632353407,
8.89443726066481));
#33176=CARTESIAN_POINT('Ctrl Pts',(-0.212542311730008,2.43156710108704,
8.89547818369367));
#33177=CARTESIAN_POINT('Ctrl Pts',(-0.229312553779454,2.41953191183221,
8.89651910672253));
#33178=CARTESIAN_POINT('Ctrl Pts',(-0.24609140858808,2.40749054161789,8.89756056434232));
#33179=CARTESIAN_POINT('Ctrl Pts',(-0.261921752449025,2.39412226004271,
8.89860202196211));
#33180=CARTESIAN_POINT('Ctrl Pts',(-0.276595385917055,2.37960665673298,
8.8996434795819));
#33181=CARTESIAN_POINT('Ctrl Pts',(-0.291273502819832,2.36508661827361,
8.9006852554124));
#33182=CARTESIAN_POINT('Ctrl Pts',(-0.304793708545817,2.34941910293927,
8.9017270312429));
#33183=CARTESIAN_POINT('Ctrl Pts',(-0.316985912733092,2.33281928856684,
8.9027688070734));
#33184=CARTESIAN_POINT('Ctrl Pts',(-0.329204470646399,2.31618359331893,
8.90381283472599));
#33185=CARTESIAN_POINT('Ctrl Pts',(-0.340088908370759,2.2986122019047,8.90485686237859));
#33186=CARTESIAN_POINT('Ctrl Pts',(-0.349513034957119,2.28034835290366,
8.90590089003119));
#33187=CARTESIAN_POINT('Ctrl Pts',(-0.352846225001586,2.27388866891003,
8.90627014892705));
#33188=CARTESIAN_POINT('Ctrl Pts',(-0.355997173223601,2.26734255865735,
8.90663940782292));
#33189=CARTESIAN_POINT('Ctrl Pts',(-0.358961754194026,2.26072133967196,
8.90700866671878));
#33190=CARTESIAN_POINT('Ctrl Pts',(-0.368144946689633,2.2402112139223,8.90815249633764));
#33191=CARTESIAN_POINT('Ctrl Pts',(-0.375583635340145,2.21887369636888,
8.90929632595649));
#33192=CARTESIAN_POINT('Ctrl Pts',(-0.381149004164054,2.19700683803088,
8.91044015557534));
#33193=CARTESIAN_POINT('Ctrl Pts',(-0.386678846079847,2.17527956826132,
8.91157668348049));
#33194=CARTESIAN_POINT('Ctrl Pts',(-0.390358983079574,2.15303014501776,
8.91271321138565));
#33195=CARTESIAN_POINT('Ctrl Pts',(-0.392110001369189,2.13057183060031,
8.9138497392908));
#33196=CARTESIAN_POINT('Ctrl Pts',(-0.392897752034933,2.12046825130662,
8.91436104212483));
#33197=CARTESIAN_POINT('Ctrl Pts',(-0.393295716606341,2.11032263485194,
8.91487234495886));
#33198=CARTESIAN_POINT('Ctrl Pts',(-0.393299965593714,2.10016451134769,
8.91538364779289));
#33199=CARTESIAN_POINT('',(-0.393299846669849,2.09965271125334,9.04038364779943));
#33200=CARTESIAN_POINT('Ctrl Pts',(-0.393299965593744,2.10016451127551,
8.91538364779652));
#33201=CARTESIAN_POINT('Ctrl Pts',(-0.39330879068897,2.07906620273691,8.9164456180457));
#33202=CARTESIAN_POINT('Ctrl Pts',(-0.391615565117182,2.05797632259616,
8.91750758829488));
#33203=CARTESIAN_POINT('Ctrl Pts',(-0.38825045884592,2.03717905440116,8.91856955854406));
#33204=CARTESIAN_POINT('Ctrl Pts',(-0.384882897301465,2.01636661195281,
8.91963230363565));
#33205=CARTESIAN_POINT('Ctrl Pts',(-0.379841181812565,1.99584788544338,
8.92069504872725));
#33206=CARTESIAN_POINT('Ctrl Pts',(-0.373206497384045,1.97589601009503,
8.92175779381885));
#33207=CARTESIAN_POINT('Ctrl Pts',(-0.366552785195639,1.95588691431706,
8.92282358678086));
#33208=CARTESIAN_POINT('Ctrl Pts',(-0.358297246682395,1.93644856117948,
8.92388937974288));
#33209=CARTESIAN_POINT('Ctrl Pts',(-0.34856954930456,1.91783480217776,8.9249551727049));
#33210=CARTESIAN_POINT('Ctrl Pts',(-0.342716470883866,1.9066350508996,8.92559645188379));
#33211=CARTESIAN_POINT('Ctrl Pts',(-0.336331328015612,1.89573336524099,
8.92623773106268));
#33212=CARTESIAN_POINT('Ctrl Pts',(-0.329449863585307,1.88517989529929,
8.92687901024156));
#33213=CARTESIAN_POINT('Ctrl Pts',(-0.318247267177633,1.8679995021352,8.92792297288912));
#33214=CARTESIAN_POINT('Ctrl Pts',(-0.305663770081435,1.85164658008582,
8.92896693553667));
#33215=CARTESIAN_POINT('Ctrl Pts',(-0.291846234603637,1.83635124626185,
8.93001089818423));
#33216=CARTESIAN_POINT('Ctrl Pts',(-0.278054117971273,1.82108404985262,
8.93105294035));
#33217=CARTESIAN_POINT('Ctrl Pts',(-0.263032912637363,1.80687115951435,
8.93209498251577));
#33218=CARTESIAN_POINT('Ctrl Pts',(-0.246970990128869,1.79391141799347,
8.93313702468154));
#33219=CARTESIAN_POINT('Ctrl Pts',(-0.230926317872829,1.7809655950314,8.9341779477104));
#33220=CARTESIAN_POINT('Ctrl Pts',(-0.213843698931939,1.7692707312228,8.93521887073926));
#33221=CARTESIAN_POINT('Ctrl Pts',(-0.195946034721089,1.75898674295992,
8.93625979376811));
#33222=CARTESIAN_POINT('Ctrl Pts',(-0.178039178736364,1.7486974731087,8.9373012513879));
#33223=CARTESIAN_POINT('Ctrl Pts',(-0.159317071170225,1.73982090691943,
8.9383427090077));
#33224=CARTESIAN_POINT('Ctrl Pts',(-0.140029376487857,1.73247222728014,
8.93938416662749));
#33225=CARTESIAN_POINT('Ctrl Pts',(-0.120735788573881,1.72512130229884,
8.94042594245799));
#33226=CARTESIAN_POINT('Ctrl Pts',(-0.10087696938326,1.7192994211612,8.94146771828849));
#33227=CARTESIAN_POINT('Ctrl Pts',(-0.0807192040880046,1.71507234434066,
8.94250949411899));
#33228=CARTESIAN_POINT('Ctrl Pts',(-0.0605178673256378,1.71083613059764,
8.94355352177159));
#33229=CARTESIAN_POINT('Ctrl Pts',(-0.0400170248655094,1.70820169721761,
8.94459754942419));
#33230=CARTESIAN_POINT('Ctrl Pts',(-0.019490333429555,1.70718322731481,
8.94564157707679));
#33231=CARTESIAN_POINT('Ctrl Pts',(-0.0122303117275964,1.70682300786006,
8.94601083597265));
#33232=CARTESIAN_POINT('Ctrl Pts',(-0.00496705512580053,1.70666445921509,
8.94638009486851));
#33233=CARTESIAN_POINT('Ctrl Pts',(0.00228742631401738,1.70670665187311,
8.94674935376437));
#33234=CARTESIAN_POINT('Ctrl Pts',(0.0227971763442628,1.70682593825855,
8.94779331641192));
#33235=CARTESIAN_POINT('Ctrl Pts',(0.0433586803398914,1.70855423573291,
8.94883727905948));
#33236=CARTESIAN_POINT('Ctrl Pts',(0.063698952493744,1.71189262638904,8.94988124170703));
#33237=CARTESIAN_POINT('Ctrl Pts',(0.0840018065251822,1.71522487571582,
8.9509232838728));
#33238=CARTESIAN_POINT('Ctrl Pts',(0.104083509057827,1.72016127975526,8.95196532603857));
#33239=CARTESIAN_POINT('Ctrl Pts',(0.12367490063912,1.72665108952629,8.95300736820434));
#33240=CARTESIAN_POINT('Ctrl Pts',(0.143245251373644,1.73313392934359,8.95404829123319));
#33241=CARTESIAN_POINT('Ctrl Pts',(0.162325632549298,1.74116666011048,8.95508921426204));
#33242=CARTESIAN_POINT('Ctrl Pts',(0.18066092303681,1.75064842795904,8.9561301372909));
#33243=CARTESIAN_POINT('Ctrl Pts',(0.199005630051624,1.76013506539644,8.95717159491069));
#33244=CARTESIAN_POINT('Ctrl Pts',(0.216603820945569,1.7710719029782,8.95821305253048));
#33245=CARTESIAN_POINT('Ctrl Pts',(0.233223499997948,1.78331136893045,8.95925451015027));
#33246=CARTESIAN_POINT('Ctrl Pts',(0.24984825708684,1.79555457457314,8.96029628598077));
#33247=CARTESIAN_POINT('Ctrl Pts',(0.265493336638524,1.80910073585399,8.96133806181127));
#33248=CARTESIAN_POINT('Ctrl Pts',(0.279959301094467,1.82376155276519,8.96237983764176));
#33249=CARTESIAN_POINT('Ctrl Pts',(0.29445653406085,1.83845405936483,8.96342386529436));
#33250=CARTESIAN_POINT('Ctrl Pts',(0.307769089265066,1.85426546837044,8.96446789294695));
#33251=CARTESIAN_POINT('Ctrl Pts',(0.319736905962473,1.87097336188656,8.96551192059955));
#33252=CARTESIAN_POINT('Ctrl Pts',(0.323969765857149,1.87688272482026,8.96588117949542));
#33253=CARTESIAN_POINT('Ctrl Pts',(0.328034808433888,1.88290397576896,8.96625043839128));
#33254=CARTESIAN_POINT('Ctrl Pts',(0.331926313975184,1.88902651329883,8.96661969728715));
#33255=CARTESIAN_POINT('Ctrl Pts',(0.342928314125601,1.90633605021451,8.9676636599347));
#33256=CARTESIAN_POINT('Ctrl Pts',(0.352605444300693,1.92456008956632,8.96870762258225));
#33257=CARTESIAN_POINT('Ctrl Pts',(0.360809022507467,1.94346968575638,8.96975158522981));
#33258=CARTESIAN_POINT('Ctrl Pts',(0.368997509348145,1.96234449570663,8.97079362739558));
#33259=CARTESIAN_POINT('Ctrl Pts',(0.375717480882778,1.9819017154483,8.97183566956135));
#33260=CARTESIAN_POINT('Ctrl Pts',(0.38086590688818,2.00188755955413,8.97287771172712));
#33261=CARTESIAN_POINT('Ctrl Pts',(0.386008803564934,2.02185193917737,8.97391863475597));
#33262=CARTESIAN_POINT('Ctrl Pts',(0.389583294806029,2.04224332759868,8.97495955778483));
#33263=CARTESIAN_POINT('Ctrl Pts',(0.391536078672314,2.06279262038375,8.97600048081368));
#33264=CARTESIAN_POINT('Ctrl Pts',(0.393489865437496,2.08335246675002,8.97704193843347));
#33265=CARTESIAN_POINT('Ctrl Pts',(0.393820195291432,2.10406964853755,8.97808339605326));
#33266=CARTESIAN_POINT('Ctrl Pts',(0.392525565748284,2.12466921632298,8.97912485367306));
#33267=CARTESIAN_POINT('Ctrl Pts',(0.391230540639369,2.14527507817442,8.98016662950356));
#33268=CARTESIAN_POINT('Ctrl Pts',(0.388309649948731,2.16576252304192,8.98120840533405));
#33269=CARTESIAN_POINT('Ctrl Pts',(0.383813260540295,2.18586193005883,8.98225018116455));
#33270=CARTESIAN_POINT('Ctrl Pts',(0.379307152084117,2.20600478240013,8.98329420881715));
#33271=CARTESIAN_POINT('Ctrl Pts',(0.373218962973318,2.2257572185577,8.98433823646975));
#33272=CARTESIAN_POINT('Ctrl Pts',(0.365649062383452,2.24486425776603,8.98538226412234));
#33273=CARTESIAN_POINT('Ctrl Pts',(0.36297168776921,2.25162216708365,8.98575152301821));
#33274=CARTESIAN_POINT('Ctrl Pts',(0.360109393162196,2.25829953959989,8.98612078191408));
#33275=CARTESIAN_POINT('Ctrl Pts',(0.35706799625136,2.26488582732618,8.98649004080994));
#33276=CARTESIAN_POINT('Ctrl Pts',(0.348469409171012,2.28350647113263,8.9875340034575));
#33277=CARTESIAN_POINT('Ctrl Pts',(0.338384716012229,2.30150817723554,8.98857796610505));
#33278=CARTESIAN_POINT('Ctrl Pts',(0.326925934083533,2.31864199876421,8.9896219287526));
#33279=CARTESIAN_POINT('Ctrl Pts',(0.315488231818954,2.3357443007819,8.99066397091837));
#33280=CARTESIAN_POINT('Ctrl Pts',(0.302681813314068,2.35198124958787,8.99170601308414));
#33281=CARTESIAN_POINT('Ctrl Pts',(0.288664293778539,2.36712883688838,8.99274805524991));
#33282=CARTESIAN_POINT('Ctrl Pts',(0.274661828838778,2.38226015591809,8.99378897827876));
#33283=CARTESIAN_POINT('Ctrl Pts',(0.259451321054667,2.39630387915413,8.99482990130762));
#33284=CARTESIAN_POINT('Ctrl Pts',(0.243230184949942,2.40906951827901,8.99587082433647));
#33285=CARTESIAN_POINT('Ctrl Pts',(0.227000718092483,2.42184171350343,8.99691228195626));
#33286=CARTESIAN_POINT('Ctrl Pts',(0.209760154235766,2.43333404559629,8.99795373957605));
#33287=CARTESIAN_POINT('Ctrl Pts',(0.191738862455026,2.44339641614969,8.99899519719585));
#33288=CARTESIAN_POINT('Ctrl Pts',(0.173712064384002,2.45346186119597,9.00003697302634));
#33289=CARTESIAN_POINT('Ctrl Pts',(0.154904723016358,2.46209614809795,9.00107874885684));
#33290=CARTESIAN_POINT('Ctrl Pts',(0.135570804897655,2.46919567556975,9.00212052468734));
#33291=CARTESIAN_POINT('Ctrl Pts',(0.116195096076183,2.47631054883129,9.00316455233994));
#33292=CARTESIAN_POINT('Ctrl Pts',(0.096291247327418,2.48188384101763,9.00420857999253));
#33293=CARTESIAN_POINT('Ctrl Pts',(0.0761279826925704,2.48586191863303,
9.00525260764513));
#33294=CARTESIAN_POINT('Ctrl Pts',(0.0689965002863075,2.48726891254193,
9.005621866541));
#33295=CARTESIAN_POINT('Ctrl Pts',(0.0618326341312234,2.48847682638425,
9.00599112543686));
#33296=CARTESIAN_POINT('Ctrl Pts',(0.0546484023851182,2.48948484196019,
9.00636038433273));
#33297=CARTESIAN_POINT('Ctrl Pts',(0.0343372611282992,2.49233468693674,
9.00740434698029));
#33298=CARTESIAN_POINT('Ctrl Pts',(0.0137420777018276,2.49359994515231,
9.00844830962784));
#33299=CARTESIAN_POINT('Ctrl Pts',(-0.00686719191505303,2.49324004332621,
9.00949227227539));
#33300=CARTESIAN_POINT('Ctrl Pts',(-0.027438548559685,2.49288080357831,
9.01053431444116));
#33301=CARTESIAN_POINT('Ctrl Pts',(-0.0480232115622961,2.49090229138008,
9.01157635660693));
#33302=CARTESIAN_POINT('Ctrl Pts',(-0.0683475107778663,2.48731577268486,
9.0126183987727));
#33303=CARTESIAN_POINT('Ctrl Pts',(-0.0886499820153858,2.48373310585437,
9.01365932180156));
#33304=CARTESIAN_POINT('Ctrl Pts',(-0.10869191865644,2.47854595971636,9.01470024483041));
#33305=CARTESIAN_POINT('Ctrl Pts',(-0.128206290664371,2.47181720916881,
9.01574116785926));
#33306=CARTESIAN_POINT('Ctrl Pts',(-0.147730684745145,2.46508500291036,
9.01678262547906));
#33307=CARTESIAN_POINT('Ctrl Pts',(-0.166726272064796,2.45680983515309,
9.01782408309885));
#33308=CARTESIAN_POINT('Ctrl Pts',(-0.184942144251628,2.44710415335978,
9.01886554071864));
#33309=CARTESIAN_POINT('Ctrl Pts',(-0.203163582181584,2.43739550605754,
9.01990731654914));
#33310=CARTESIAN_POINT('Ctrl Pts',(-0.220604198909779,2.42625585221344,
9.02094909237964));
#33311=CARTESIAN_POINT('Ctrl Pts',(-0.237039407940149,2.41384265019813,
9.02199086821014));
#33312=CARTESIAN_POINT('Ctrl Pts',(-0.253510142047781,2.40140261676498,
9.02303489586274));
#33313=CARTESIAN_POINT('Ctrl Pts',(-0.268970578871846,2.38768402813433,
9.02407892351533));
#33314=CARTESIAN_POINT('Ctrl Pts',(-0.283230157229812,2.37288379951103,
9.02512295116793));
#33315=CARTESIAN_POINT('Ctrl Pts',(-0.288273583183993,2.36764915264471,
9.0254922100638));
#33316=CARTESIAN_POINT('Ctrl Pts',(-0.293167148962151,2.36227951130538,
9.02586146895966));
#33317=CARTESIAN_POINT('Ctrl Pts',(-0.297903660961291,2.35678453766896,
9.02623072785553));
#33318=CARTESIAN_POINT('Ctrl Pts',(-0.311195734804249,2.34136399289811,
9.02726697911213));
#33319=CARTESIAN_POINT('Ctrl Pts',(-0.323330281225145,2.32485858760565,
9.02830323036874));
#33320=CARTESIAN_POINT('Ctrl Pts',(-0.334127681974604,2.30746947278643,
9.02933948162534));
#33321=CARTESIAN_POINT('Ctrl Pts',(-0.344904881002772,2.29011289265395,
9.03037379407653));
#33322=CARTESIAN_POINT('Ctrl Pts',(-0.354349454542564,2.27187647832869,
9.03140810652771));
#33323=CARTESIAN_POINT('Ctrl Pts',(-0.362323150777052,2.25299289006679,
9.0324424189789));
#33324=CARTESIAN_POINT('Ctrl Pts',(-0.370287998041917,2.23413025824642,
9.03347558358106));
#33325=CARTESIAN_POINT('Ctrl Pts',(-0.376784891220112,2.21462255238723,
9.03450874818322));
#33326=CARTESIAN_POINT('Ctrl Pts',(-0.381722503778977,2.1947249708826,9.03554191278537));
#33327=CARTESIAN_POINT('Ctrl Pts',(-0.386661872350672,2.17482031300087,
9.03657544482225));
#33328=CARTESIAN_POINT('Ctrl Pts',(-0.390040661394329,2.15452622553248,
9.03760897685914));
#33329=CARTESIAN_POINT('Ctrl Pts',(-0.391817972917354,2.13411108469304,
9.03864250889602));
#33330=CARTESIAN_POINT('Ctrl Pts',(-0.392816021718496,2.12264696792117,
9.03922288852952));
#33331=CARTESIAN_POINT('Ctrl Pts',(-0.393309994372249,2.11114484999877,
9.03980326816302));
#33332=CARTESIAN_POINT('Ctrl Pts',(-0.3932998466699,2.09965271131105,9.04038364779652));
#33333=CARTESIAN_POINT('',(-0.393299999929551,2.10000744414488,9.1653836477998));
#33334=CARTESIAN_POINT('Ctrl Pts',(-0.393299846669849,2.09965271125334,
9.04038364779943));
#33335=CARTESIAN_POINT('Ctrl Pts',(-0.393277423792018,2.07425910291527,
9.041666083863));
#33336=CARTESIAN_POINT('Ctrl Pts',(-0.390791705111248,2.04897530882568,
9.04294851992656));
#33337=CARTESIAN_POINT('Ctrl Pts',(-0.385929156388464,2.02421361435397,
9.04423095599012));
#33338=CARTESIAN_POINT('Ctrl Pts',(-0.383565548707071,2.01217734806765,
9.04485432778618));
#33339=CARTESIAN_POINT('Ctrl Pts',(-0.38064107672183,2.00026409950309,9.04547769958224));
#33340=CARTESIAN_POINT('Ctrl Pts',(-0.377169671296976,1.98851937812458,
9.04610107137829));
#33341=CARTESIAN_POINT('Ctrl Pts',(-0.371356098047462,1.96885045742165,
9.04714503402584));
#33342=CARTESIAN_POINT('Ctrl Pts',(-0.3639824965963,1.94957891206686,9.0481889966734));
#33343=CARTESIAN_POINT('Ctrl Pts',(-0.355123681233962,1.93096727823632,
9.04923295932095));
#33344=CARTESIAN_POINT('Ctrl Pts',(-0.346281162617074,1.91238988251172,
9.05027500148672));
#33345=CARTESIAN_POINT('Ctrl Pts',(-0.335959112373765,1.89447067102725,
9.05131704365249));
#33346=CARTESIAN_POINT('Ctrl Pts',(-0.324281071518415,1.87745410213875,
9.05235908581827));
#33347=CARTESIAN_POINT('Ctrl Pts',(-0.312615572695485,1.86045580877792,
9.05340000884712));
#33348=CARTESIAN_POINT('Ctrl Pts',(-0.299597364767039,1.84435885342254,
9.05444093187598));
#33349=CARTESIAN_POINT('Ctrl Pts',(-0.285394219692462,1.82938028644215,
9.05548185490483));
#33350=CARTESIAN_POINT('Ctrl Pts',(-0.271183780252756,1.81439402686016,
9.05652331252463));
#33351=CARTESIAN_POINT('Ctrl Pts',(-0.255787682487004,1.80052784812853,
9.05756477014442));
#33352=CARTESIAN_POINT('Ctrl Pts',(-0.239412150697716,1.78796360452938,
9.05860622776421));
#33353=CARTESIAN_POINT('Ctrl Pts',(-0.223031615469557,1.77539552200607,
9.05964800359471));
#33354=CARTESIAN_POINT('Ctrl Pts',(-0.205671655746578,1.76413058534215,
9.06068977942521));
#33355=CARTESIAN_POINT('Ctrl Pts',(-0.18756857332672,1.75430805577772,9.06173155525572));
#33356=CARTESIAN_POINT('Ctrl Pts',(-0.169426360683397,1.74446429459273,
9.06277558290831));
#33357=CARTESIAN_POINT('Ctrl Pts',(-0.150538491489484,1.7360694641524,9.06381961056091));
#33358=CARTESIAN_POINT('Ctrl Pts',(-0.131163100331721,1.72921551932238,
9.06486363821351));
#33359=CARTESIAN_POINT('Ctrl Pts',(-0.124310278447117,1.72679136887584,
9.06523289710938));
#33360=CARTESIAN_POINT('Ctrl Pts',(-0.117396605658614,1.72455951701898,
9.06560215600524));
#33361=CARTESIAN_POINT('Ctrl Pts',(-0.110433855231836,1.72252251243467,
9.0659714149011));
#33362=CARTESIAN_POINT('Ctrl Pts',(-0.0907488823003548,1.71676352673998,
9.06701537754866));
#33363=CARTESIAN_POINT('Ctrl Pts',(-0.0705535582228659,1.71253134714463,
9.06805934019621));
#33364=CARTESIAN_POINT('Ctrl Pts',(-0.0501091264440478,1.70990518402956,
9.06910330284376));
#33365=CARTESIAN_POINT('Ctrl Pts',(-0.0297023044004944,1.70728385202452,
9.07014534500953));
#33366=CARTESIAN_POINT('Ctrl Pts',(-0.00904799824759791,1.7062628237229,
9.0711873871753));
#33367=CARTESIAN_POINT('Ctrl Pts',(0.0115813720688393,1.70687055335297,
9.07222942934107));
#33368=CARTESIAN_POINT('Ctrl Pts',(0.0321885867656339,1.70747763029096,
9.07327035236992));
#33369=CARTESIAN_POINT('Ctrl Pts',(0.0527701862102576,1.70970999981279,
9.07431127539878));
#33370=CARTESIAN_POINT('Ctrl Pts',(0.073052852572784,1.71354408953804,9.07535219842763));
#33371=CARTESIAN_POINT('Ctrl Pts',(0.093345935584124,1.71738014835185,9.07639365604742));
#33372=CARTESIAN_POINT('Ctrl Pts',(0.1133390528375,1.72281944991755,9.07743511366721));
#33373=CARTESIAN_POINT('Ctrl Pts',(0.132767665055326,1.72978703815809,9.078476571287));
#33374=CARTESIAN_POINT('Ctrl Pts',(0.152202213561197,1.7367567553006,9.0795183471175));
#33375=CARTESIAN_POINT('Ctrl Pts',(0.171071233872581,1.7452554064944,9.080560122948));
#33376=CARTESIAN_POINT('Ctrl Pts',(0.189129718212506,1.75515968958247,9.08160189877849));
#33377=CARTESIAN_POINT('Ctrl Pts',(0.207227236376134,1.7650853810032,9.08264592643109));
#33378=CARTESIAN_POINT('Ctrl Pts',(0.224510104991437,1.77642236619478,9.08368995408368));
#33379=CARTESIAN_POINT('Ctrl Pts',(0.240761273844977,1.78900337780525,9.08473398173628));
#33380=CARTESIAN_POINT('Ctrl Pts',(0.246509099252161,1.79345311670307,9.08510324063215));
#33381=CARTESIAN_POINT('Ctrl Pts',(0.252128176255932,1.79805811483161,9.08547249952801));
#33382=CARTESIAN_POINT('Ctrl Pts',(0.257609988796705,1.80280985266641,9.08584175842388));
#33383=CARTESIAN_POINT('Ctrl Pts',(0.273108078612594,1.81624388733971,9.08688572107143));
#33384=CARTESIAN_POINT('Ctrl Pts',(0.287598664820426,1.8309335221233,9.08792968371898));
#33385=CARTESIAN_POINT('Ctrl Pts',(0.300873730116724,1.84670197686194,9.08897364636654));
#33386=CARTESIAN_POINT('Ctrl Pts',(0.31412437449994,1.86244142382894,9.09001568853231));
#33387=CARTESIAN_POINT('Ctrl Pts',(0.326163422497019,1.87925523317644,9.09105773069808));
#33388=CARTESIAN_POINT('Ctrl Pts',(0.336819483444385,1.8969297521244,9.09209977286385));
#33389=CARTESIAN_POINT('Ctrl Pts',(0.347464099949695,1.91458528891667,9.0931406958927));
#33390=CARTESIAN_POINT('Ctrl Pts',(0.356728275351814,1.93309908818909,9.09418161892156));
#33391=CARTESIAN_POINT('Ctrl Pts',(0.364483877850369,1.95222857926122,9.09522254195041));
#33392=CARTESIAN_POINT('Ctrl Pts',(0.372243463424232,1.9713678947414,9.0962639995702));
#33393=CARTESIAN_POINT('Ctrl Pts',(0.378492636902405,1.99112285791194,9.09730545719));
#33394=CARTESIAN_POINT('Ctrl Pts',(0.383151222805638,2.01123046433295,9.09834691480979));
#33395=CARTESIAN_POINT('Ctrl Pts',(0.387811232109963,2.03134421450434,9.09938869064029));
#33396=CARTESIAN_POINT('Ctrl Pts',(0.390879555659226,2.05181009807242,9.10043046647078));
#33397=CARTESIAN_POINT('Ctrl Pts',(0.392327240977996,2.07235536242607,9.10147224230128));
#33398=CARTESIAN_POINT('Ctrl Pts',(0.393778055501434,2.09294503583486,9.10251626995388));
#33399=CARTESIAN_POINT('Ctrl Pts',(0.393601244433702,2.11361369613625,9.10356029760648));
#33400=CARTESIAN_POINT('Ctrl Pts',(0.391819955956773,2.13408829878467,9.10460432525907));
#33401=CARTESIAN_POINT('Ctrl Pts',(0.391189937571169,2.14132989736541,9.10497358415494));
#33402=CARTESIAN_POINT('Ctrl Pts',(0.390359680607458,2.14854728661034,9.10534284305081));
#33403=CARTESIAN_POINT('Ctrl Pts',(0.389331738537403,2.15572869429157,9.10571210194668));
#33404=CARTESIAN_POINT('Ctrl Pts',(0.386425557706031,2.17603185139879,9.10675606459423));
#33405=CARTESIAN_POINT('Ctrl Pts',(0.381918265913698,2.19616756046058,9.10780002724179));
#33406=CARTESIAN_POINT('Ctrl Pts',(0.375845899555068,2.21586522251151,9.10884398988934));
#33407=CARTESIAN_POINT('Ctrl Pts',(0.36978470396869,2.23552664859055,9.10988603205511));
#33408=CARTESIAN_POINT('Ctrl Pts',(0.362164306241021,2.25475091450429,9.11092807422088));
#33409=CARTESIAN_POINT('Ctrl Pts',(0.353071572591811,2.27327825780387,9.11197011638665));
#33410=CARTESIAN_POINT('Ctrl Pts',(0.343988604395694,2.29178570302781,9.1130110394155));
#33411=CARTESIAN_POINT('Ctrl Pts',(0.333436736027456,2.30959704164456,9.11405196244436));
#33412=CARTESIAN_POINT('Ctrl Pts',(0.321550565199549,2.32647323024996,9.11509288547321));
#33413=CARTESIAN_POINT('Ctrl Pts',(0.309658289944099,2.34335808602597,9.116134343093));
#33414=CARTESIAN_POINT('Ctrl Pts',(0.296430753728987,2.35930622148777,9.11717580071279));
#33415=CARTESIAN_POINT('Ctrl Pts',(0.282045694960607,2.37410785460141,9.11821725833258));
#33416=CARTESIAN_POINT('Ctrl Pts',(0.267656240929639,2.38891401025926,9.11925903416308));
#33417=CARTESIAN_POINT('Ctrl Pts',(0.252109098574853,2.40257246420638,9.12030080999358));
#33418=CARTESIAN_POINT('Ctrl Pts',(0.235617930677045,2.41491122676632,9.12134258582408));
#33419=CARTESIAN_POINT('Ctrl Pts',(0.219091116745591,2.42727665984154,9.12238661347667));
#33420=CARTESIAN_POINT('Ctrl Pts',(0.201616826078801,2.43831631321023,9.12343064112927));
#33421=CARTESIAN_POINT('Ctrl Pts',(0.183437169948442,2.44790184633213,9.12447466878187));
#33422=CARTESIAN_POINT('Ctrl Pts',(0.177007263869615,2.45129212375253,9.12484392767773));
#33423=CARTESIAN_POINT('Ctrl Pts',(0.170489320673381,2.4545009320404,9.1252131865736));
#33424=CARTESIAN_POINT('Ctrl Pts',(0.163894620900134,2.45752404568085,9.12558244546946));
#33425=CARTESIAN_POINT('Ctrl Pts',(0.145250194693487,2.46607094260136,9.12662640811701));
#33426=CARTESIAN_POINT('Ctrl Pts',(0.125879851508083,2.47318095410641,9.12767037076457));
#33427=CARTESIAN_POINT('Ctrl Pts',(0.106030622950536,2.47873790013243,9.12871433341212));
#33428=CARTESIAN_POINT('Ctrl Pts',(0.0862179091877993,2.48428462355744,
9.12975637557789));
#33429=CARTESIAN_POINT('Ctrl Pts',(0.0659287432270489,2.48828369920904,
9.13079841774366));
#33430=CARTESIAN_POINT('Ctrl Pts',(0.0454285602405077,2.4906675516529,9.13184045990943));
#33431=CARTESIAN_POINT('Ctrl Pts',(0.0249503941284426,2.49304884387669,
9.13288138293829));
#33432=CARTESIAN_POINT('Ctrl Pts',(0.00426238471054755,2.49381824345169,
9.13392230596714));
#33433=CARTESIAN_POINT('Ctrl Pts',(-0.0163616158652496,2.4929595240305,
9.134963228996));
#33434=CARTESIAN_POINT('Ctrl Pts',(-0.036996208390216,2.4921003635934,9.13600468661579));
#33435=CARTESIAN_POINT('Ctrl Pts',(-0.0575659905876893,2.48961142820284,
9.13704614423558));
#33436=CARTESIAN_POINT('Ctrl Pts',(-0.0777983609566011,2.48552860468773,
9.13808760185537));
#33437=CARTESIAN_POINT('Ctrl Pts',(-0.0980369131967171,2.48144453369203,
9.13912937768587));
#33438=CARTESIAN_POINT('Ctrl Pts',(-0.117937134897336,2.4757657859523,9.14017115351637));
#33439=CARTESIAN_POINT('Ctrl Pts',(-0.137238754535256,2.46857891184061,
9.14121292934687));
#33440=CARTESIAN_POINT('Ctrl Pts',(-0.156582095062032,2.46137650313744,
9.14225695699947));
#33441=CARTESIAN_POINT('Ctrl Pts',(-0.175323582550946,2.45265977052075,
9.14330098465206));
#33442=CARTESIAN_POINT('Ctrl Pts',(-0.193224246771814,2.44256281242929,
9.14434501230466));
#33443=CARTESIAN_POINT('Ctrl Pts',(-0.199555477069242,2.43899165070078,
9.14471427120053));
#33444=CARTESIAN_POINT('Ctrl Pts',(-0.20578178095333,2.43524823326732,9.14508353009639));
#33445=CARTESIAN_POINT('Ctrl Pts',(-0.211893499175158,2.43133975766169,
9.14545278899226));
#33446=CARTESIAN_POINT('Ctrl Pts',(-0.229172447921879,2.4202897800259,9.14649675163981));
#33447=CARTESIAN_POINT('Ctrl Pts',(-0.245636189661819,2.40785162635901,
9.14754071428736));
#33448=CARTESIAN_POINT('Ctrl Pts',(-0.261053315445168,2.39417011489117,
9.14858467693491));
#33449=CARTESIAN_POINT('Ctrl Pts',(-0.276442079764349,2.38051377203795,
9.14962671910068));
#33450=CARTESIAN_POINT('Ctrl Pts',(-0.290787466309704,2.36561904994209,
9.15066876126645));
#33451=CARTESIAN_POINT('Ctrl Pts',(-0.303888971591314,2.34967255144523,
9.15171080343222));
#33452=CARTESIAN_POINT('Ctrl Pts',(-0.316976406062075,2.33374317923725,
9.15275172646107));
#33453=CARTESIAN_POINT('Ctrl Pts',(-0.328822124306866,2.31676482040477,
9.15379264948992));
#33454=CARTESIAN_POINT('Ctrl Pts',(-0.339264241806408,2.29895895112189,
9.15483357251877));
#33455=CARTESIAN_POINT('Ctrl Pts',(-0.34971172210534,2.28114393720863,9.15587503013856));
#33456=CARTESIAN_POINT('Ctrl Pts',(-0.358753775441977,2.26250119034864,
9.15691648775835));
#33457=CARTESIAN_POINT('Ctrl Pts',(-0.366273011986461,2.24327934495371,
9.15795794537814));
#33458=CARTESIAN_POINT('Ctrl Pts',(-0.373794545985521,2.22405162644702,
9.15899972120863));
#33459=CARTESIAN_POINT('Ctrl Pts',(-0.379792102792222,2.20424515498,9.16004149703913));
#33460=CARTESIAN_POINT('Ctrl Pts',(-0.384197565830724,2.18412562278965,
9.16108327286962));
#33461=CARTESIAN_POINT('Ctrl Pts',(-0.388612551377556,2.1639626017739,9.16212730052222));
#33462=CARTESIAN_POINT('Ctrl Pts',(-0.391428472340683,2.14348589867171,
9.16317132817481));
#33463=CARTESIAN_POINT('Ctrl Pts',(-0.392628722184836,2.12296903383913,
9.16421535582741));
#33464=CARTESIAN_POINT('Ctrl Pts',(-0.393053234822147,2.11571248767762,
9.16458461472329));
#33465=CARTESIAN_POINT('Ctrl Pts',(-0.393276113215156,2.10845092039755,
9.16495387361916));
#33466=CARTESIAN_POINT('Ctrl Pts',(-0.393298180452314,2.10119634982288,
9.16532313251504));
#33467=CARTESIAN_POINT('Ctrl Pts',(-0.393299385934505,2.1008000493904,9.16534330427554));
#33468=CARTESIAN_POINT('Ctrl Pts',(-0.393299992428502,2.10040374713497,
9.16536347603603));
#33469=CARTESIAN_POINT('Ctrl Pts',(-0.39329999992955,2.10000744420937,9.16538364779652));
#33470=CARTESIAN_POINT('',(-0.393299850244702,2.10034321639634,9.29038364779335));
#33471=CARTESIAN_POINT('Ctrl Pts',(-0.393299999929551,2.10000744414487,
9.1653836477998));
#33472=CARTESIAN_POINT('Ctrl Pts',(-0.39330038792013,2.07950855577125,9.16642703819617));
#33473=CARTESIAN_POINT('Ctrl Pts',(-0.391693847425995,2.05894822970895,
9.16747042859253));
#33474=CARTESIAN_POINT('Ctrl Pts',(-0.388477579848486,2.03859918603909,
9.16851381898889));
#33475=CARTESIAN_POINT('Ctrl Pts',(-0.385267228201931,2.01828757194696,
9.1695552901962));
#33476=CARTESIAN_POINT('Ctrl Pts',(-0.380453081344955,1.99818719758936,
9.1705967614035));
#33477=CARTESIAN_POINT('Ctrl Pts',(-0.374084194772206,1.97856728109101,
9.1716382326108));
#33478=CARTESIAN_POINT('Ctrl Pts',(-0.367722132165268,1.95896838642086,
9.17267858793014));
#33479=CARTESIAN_POINT('Ctrl Pts',(-0.359808835644594,1.93984963373444,
9.17371894324947));
#33480=CARTESIAN_POINT('Ctrl Pts',(-0.350443549068287,1.92146650477733,
9.17475929856881));
#33481=CARTESIAN_POINT('Ctrl Pts',(-0.341073433052452,1.90307389610927,
9.17580019037285));
#33482=CARTESIAN_POINT('Ctrl Pts',(-0.330250151491237,1.88541833259056,
9.1768410821769));
#33483=CARTESIAN_POINT('Ctrl Pts',(-0.318119796939728,1.86873243894782,
9.17788197398095));
#33484=CARTESIAN_POINT('Ctrl Pts',(-0.305985657120971,1.85204133848557,
9.17892319059444));
#33485=CARTESIAN_POINT('Ctrl Pts',(-0.292544094846466,1.83632108400085,
9.17996440720793));
#33486=CARTESIAN_POINT('Ctrl Pts',(-0.27798210897944,1.8217719692638,9.18100562382141));
#33487=CARTESIAN_POINT('Ctrl Pts',(-0.263388735792879,1.80719149495002,
9.18204908470288));
#33488=CARTESIAN_POINT('Ctrl Pts',(-0.247670679374745,1.79378767756556,
9.18309254558434));
#33489=CARTESIAN_POINT('Ctrl Pts',(-0.231049251744221,1.78172161042817,
9.18413600646581));
#33490=CARTESIAN_POINT('Ctrl Pts',(-0.225434393766891,1.77764559151889,
9.18448849632315));
#33491=CARTESIAN_POINT('Ctrl Pts',(-0.219716686710828,1.77372185895176,
9.18484098618049));
#33492=CARTESIAN_POINT('Ctrl Pts',(-0.2139053238769,1.76995545388975,9.18519347603783));
#33493=CARTESIAN_POINT('Ctrl Pts',(-0.196693918772264,1.75880056214355,
9.18623743868539));
#33494=CARTESIAN_POINT('Ctrl Pts',(-0.178556311766939,1.7489623879815,9.18728140133294));
#33495=CARTESIAN_POINT('Ctrl Pts',(-0.159720122492187,1.74059163550206,
9.1883253639805));
#33496=CARTESIAN_POINT('Ctrl Pts',(-0.140918584417327,1.73223628192382,
9.18936740614627));
#33497=CARTESIAN_POINT('Ctrl Pts',(-0.121421655609795,1.72534334143922,
9.19040944831204));
#33498=CARTESIAN_POINT('Ctrl Pts',(-0.101482198926803,1.72001808819237,
9.1914514904778));
#33499=CARTESIAN_POINT('Ctrl Pts',(-0.0815641569070532,1.71469855418386,
9.19249241350666));
#33500=CARTESIAN_POINT('Ctrl Pts',(-0.061205230328669,1.71094358175297,
9.19353333653551));
#33501=CARTESIAN_POINT('Ctrl Pts',(-0.0406740409346544,1.70880885440229,
9.19457425956436));
#33502=CARTESIAN_POINT('Ctrl Pts',(-0.0201323072568634,1.70667303071129,
9.19561571718416));
#33503=CARTESIAN_POINT('Ctrl Pts',(0.0005811358132983,1.70615920660784,
9.19665717480395));
#33504=CARTESIAN_POINT('Ctrl Pts',(0.021191362947472,1.70727131994667,9.19769863242374));
#33505=CARTESIAN_POINT('Ctrl Pts',(0.0418078874045685,1.70838377308462,
9.19874040825423));
#33506=CARTESIAN_POINT('Ctrl Pts',(0.0623204010020615,1.71112307692653,
9.19978218408473));
#33507=CARTESIAN_POINT('Ctrl Pts',(0.0824588473145895,1.71544125481333,
9.20082395991523));
#33508=CARTESIAN_POINT('Ctrl Pts',(0.10264082333581,1.71976876653961,9.20186798756783));
#33509=CARTESIAN_POINT('Ctrl Pts',(0.122446412133238,1.72568175505601,9.20291201522042));
#33510=CARTESIAN_POINT('Ctrl Pts',(0.141619753901276,1.73308211367536,9.20395604287302));
#33511=CARTESIAN_POINT('Ctrl Pts',(0.148401113565189,1.73569952351694,9.20432530176889));
#33512=CARTESIAN_POINT('Ctrl Pts',(0.155103577558642,1.73850255947007,9.20469456066475));
#33513=CARTESIAN_POINT('Ctrl Pts',(0.161716546775339,1.74148549750525,9.20506381956062));
#33514=CARTESIAN_POINT('Ctrl Pts',(0.180412624050508,1.74991881061851,9.20610778220817));
#33515=CARTESIAN_POINT('Ctrl Pts',(0.198502951430162,1.75984365389283,9.20715174485573));
#33516=CARTESIAN_POINT('Ctrl Pts',(0.215737599590802,1.7711502195184,9.20819570750328));
#33517=CARTESIAN_POINT('Ctrl Pts',(0.232940542759013,1.78243598549814,9.20923774966905));
#33518=CARTESIAN_POINT('Ctrl Pts',(0.249290290382995,1.79509807908818,9.21027979183482));
#33519=CARTESIAN_POINT('Ctrl Pts',(0.26456144684395,1.8089808754672,9.21132183400059));
#33520=CARTESIAN_POINT('Ctrl Pts',(0.27981620232277,1.82284876194101,9.21236275702945));
#33521=CARTESIAN_POINT('Ctrl Pts',(0.293994105192477,1.83793427749729,9.2134036800583));
#33522=CARTESIAN_POINT('Ctrl Pts',(0.306902925963941,1.8540417026511,9.21444460308716));
#33523=CARTESIAN_POINT('Ctrl Pts',(0.319818376369305,1.87015740015865,9.21548606070695));
#33524=CARTESIAN_POINT('Ctrl Pts',(0.33146296987723,1.88729549168208,9.21652751832674));
#33525=CARTESIAN_POINT('Ctrl Pts',(0.34168457342113,1.90522694671485,9.21756897594653));
#33526=CARTESIAN_POINT('Ctrl Pts',(0.351909300110537,1.92316388058887,9.21861075177703));
#33527=CARTESIAN_POINT('Ctrl Pts',(0.360709838642622,1.94189400395128,9.21965252760753));
#33528=CARTESIAN_POINT('Ctrl Pts',(0.36798034222869,1.96116427789198,9.22069430343803));
#33529=CARTESIAN_POINT('Ctrl Pts',(0.375266561173246,1.98047620496709,9.22173833109063));
#33530=CARTESIAN_POINT('Ctrl Pts',(0.38101593764056,2.0003299061597,9.22278235874323));
#33531=CARTESIAN_POINT('Ctrl Pts',(0.385172459953885,2.0204571430418,9.22382638639582));
#33532=CARTESIAN_POINT('Ctrl Pts',(0.386642567413423,2.02757588290406,9.22419564529169));
#33533=CARTESIAN_POINT('Ctrl Pts',(0.387913889462887,2.03472876864225,9.22456490418755));
#33534=CARTESIAN_POINT('Ctrl Pts',(0.388985501480998,2.04190378981744,9.22493416308341));
#33535=CARTESIAN_POINT('Ctrl Pts',(0.392015145267815,2.06218889110064,9.22597812573097));
#33536=CARTESIAN_POINT('Ctrl Pts',(0.393462780426647,2.08277205925253,9.22702208837852));
#33537=CARTESIAN_POINT('Ctrl Pts',(0.393285444071266,2.10338370827154,9.22806605102607));
#33538=CARTESIAN_POINT('Ctrl Pts',(0.393108433945221,2.12395743994115,9.22910809319185));
#33539=CARTESIAN_POINT('Ctrl Pts',(0.391312332757793,2.14455882052535,9.23015013535761));
#33540=CARTESIAN_POINT('Ctrl Pts',(0.387905981924002,2.16491409082454,9.23119217752338));
#33541=CARTESIAN_POINT('Ctrl Pts',(0.384503289457495,2.18524749988319,9.23223310055224));
#33542=CARTESIAN_POINT('Ctrl Pts',(0.379493872882747,2.20533459661122,9.23327402358109));
#33543=CARTESIAN_POINT('Ctrl Pts',(0.372938239351095,2.2249078045188,9.23431494660995));
#33544=CARTESIAN_POINT('Ctrl Pts',(0.366379239016921,2.24449106471581,9.23535640422974));
#33545=CARTESIAN_POINT('Ctrl Pts',(0.358272653687357,2.26355920603384,9.23639786184953));
#33546=CARTESIAN_POINT('Ctrl Pts',(0.348728703935136,2.28186033391512,9.23743931946932));
#33547=CARTESIAN_POINT('Ctrl Pts',(0.339181838090185,2.30016705358884,9.23848109529982));
#33548=CARTESIAN_POINT('Ctrl Pts',(0.328197105538829,2.31770565816276,9.23952287113032));
#33549=CARTESIAN_POINT('Ctrl Pts',(0.315929969147927,2.33425017522766,9.24056464696082));
#33550=CARTESIAN_POINT('Ctrl Pts',(0.30363631706334,2.35083045364164,9.24160867461341));
#33551=CARTESIAN_POINT('Ctrl Pts',(0.290055210998721,2.36641179950358,9.24265270226601));
#33552=CARTESIAN_POINT('Ctrl Pts',(0.275381870494289,2.38080191488497,9.24369672991861));
#33553=CARTESIAN_POINT('Ctrl Pts',(0.270192102292377,2.38589151007331,9.24406598881447));
#33554=CARTESIAN_POINT('Ctrl Pts',(0.264866017492327,2.39083244670933,9.24443524771034));
#33555=CARTESIAN_POINT('Ctrl Pts',(0.25941321417202,2.39561744588732,9.24480450660621));
#33556=CARTESIAN_POINT('Ctrl Pts',(0.243997138744853,2.4091455164803,9.24584846925377));
#33557=CARTESIAN_POINT('Ctrl Pts',(0.227474073502381,2.42150475487572,9.24689243190132));
#33558=CARTESIAN_POINT('Ctrl Pts',(0.21004743459489,2.43251310533587,9.24793639454887));
#33559=CARTESIAN_POINT('Ctrl Pts',(0.192652853867494,2.44350120474914,9.24897843671464));
#33560=CARTESIAN_POINT('Ctrl Pts',(0.174358582191037,2.45314291026621,9.25002047888041));
#33561=CARTESIAN_POINT('Ctrl Pts',(0.155399587219722,2.46129746510589,9.25106252104618));
#33562=CARTESIAN_POINT('Ctrl Pts',(0.136460953911176,2.46944326208177,9.25210344407503));
#33563=CARTESIAN_POINT('Ctrl Pts',(0.116859675628835,2.47610476334489,9.25314436710388));
#33564=CARTESIAN_POINT('Ctrl Pts',(0.0968534890904559,2.4811880004027,9.25418529013274));
#33565=CARTESIAN_POINT('Ctrl Pts',(0.076837027896091,2.48627384807857,9.25522674775253));
#33566=CARTESIAN_POINT('Ctrl Pts',(0.0564159521569811,2.48977961542495,
9.25626820537232));
#33567=CARTESIAN_POINT('Ctrl Pts',(0.0358617237148704,2.49166162279728,
9.25730966299211));
#33568=CARTESIAN_POINT('Ctrl Pts',(0.0153012150598787,2.49354420520491,
9.25835143882261));
#33569=CARTESIAN_POINT('Ctrl Pts',(-0.00539179189535383,2.4938020089592,
9.25939321465311));
#33570=CARTESIAN_POINT('Ctrl Pts',(-0.0259431406443975,2.4924434270739,
9.2604349904836));
#33571=CARTESIAN_POINT('Ctrl Pts',(-0.0465389116001311,2.49108190858302,
9.2614790181362));
#33572=CARTESIAN_POINT('Ctrl Pts',(-0.0669916842830418,2.48809713549467,
9.26252304578879));
#33573=CARTESIAN_POINT('Ctrl Pts',(-0.0870340952873548,2.48354915755026,
9.26356707344139));
#33574=CARTESIAN_POINT('Ctrl Pts',(-0.0941228333486487,2.48194059736508,
9.26393633233726));
#33575=CARTESIAN_POINT('Ctrl Pts',(-0.101160367275178,2.48013694818307,
9.26430559123313));
#33576=CARTESIAN_POINT('Ctrl Pts',(-0.108135381219693,2.47814234003675,
9.264674850129));
#33577=CARTESIAN_POINT('Ctrl Pts',(-0.127855025365576,2.47250321685096,
9.26571881277655));
#33578=CARTESIAN_POINT('Ctrl Pts',(-0.147191128061596,2.46530060682049,
9.2667627754241));
#33579=CARTESIAN_POINT('Ctrl Pts',(-0.165880500746236,2.45660699582619,
9.26780673807166));
#33580=CARTESIAN_POINT('Ctrl Pts',(-0.184535492315925,2.4479293776661,9.26884878023743));
#33581=CARTESIAN_POINT('Ctrl Pts',(-0.202545430758457,2.43776645590382,
9.2698908224032));
#33582=CARTESIAN_POINT('Ctrl Pts',(-0.219664773015213,2.42623960136099,
9.27093286456897));
#33583=CARTESIAN_POINT('Ctrl Pts',(-0.23676572936733,2.41472512647884,9.27197378759782));
#33584=CARTESIAN_POINT('Ctrl Pts',(-0.252977365006309,2.40185001174964,
9.27301471062668));
#33585=CARTESIAN_POINT('Ctrl Pts',(-0.268081151998824,2.38778009997737,
9.27405563365553));
#33586=CARTESIAN_POINT('Ctrl Pts',(-0.283192695902686,2.37370296226511,
9.27509709127532));
#33587=CARTESIAN_POINT('Ctrl Pts',(-0.29719470513914,2.35843029136667,9.27613854889511));
#33588=CARTESIAN_POINT('Ctrl Pts',(-0.309903505881037,2.34216669267809,
9.2771800065149));
#33589=CARTESIAN_POINT('Ctrl Pts',(-0.322616189715624,2.32589812475106,
9.2782217823454));
#33590=CARTESIAN_POINT('Ctrl Pts',(-0.334034454291829,2.30863862783796,
9.2792635581759));
#33591=CARTESIAN_POINT('Ctrl Pts',(-0.344016950735263,2.29062326092797,
9.2803053340064));
#33592=CARTESIAN_POINT('Ctrl Pts',(-0.354021024571285,2.27256895339359,
9.28134936165899));
#33593=CARTESIAN_POINT('Ctrl Pts',(-0.362582829329486,2.25375618432334,
9.28239338931159));
#33594=CARTESIAN_POINT('Ctrl Pts',(-0.369608127265093,2.23444226366582,
9.28343741696419));
#33595=CARTESIAN_POINT('Ctrl Pts',(-0.372092883059036,2.22761118309139,
9.28380667586005));
#33596=CARTESIAN_POINT('Ctrl Pts',(-0.374385886808147,2.22071755067123,
9.28417593475592));
#33597=CARTESIAN_POINT('Ctrl Pts',(-0.376484485645148,2.21377311663354,
9.28454519365178));
#33598=CARTESIAN_POINT('Ctrl Pts',(-0.383718590512525,2.1898348759429,9.28581807035828));
#33599=CARTESIAN_POINT('Ctrl Pts',(-0.38867394028947,2.1651777808366,9.28709094706477));
#33600=CARTESIAN_POINT('Ctrl Pts',(-0.391240571091593,2.14019583973404,
9.28836382377127));
#33601=CARTESIAN_POINT('Ctrl Pts',(-0.392598163313859,2.12698190615625,
9.2890370984453));
#33602=CARTESIAN_POINT('Ctrl Pts',(-0.393288214024346,2.11367743869001,
9.28971037311932));
#33603=CARTESIAN_POINT('Ctrl Pts',(-0.393299850244702,2.10034321639633,
9.29038364779335));
#33604=CARTESIAN_POINT('',(-0.393299960517904,2.09982377112743,9.41538364780035));
#33605=CARTESIAN_POINT('Ctrl Pts',(-0.393299850244757,2.10034321633353,
9.29038364779652));
#33606=CARTESIAN_POINT('Ctrl Pts',(-0.393317722140316,2.07986338143033,
9.29141772041544));
#33607=CARTESIAN_POINT('Ctrl Pts',(-0.391731641870721,2.05935355499808,
9.29245179303436));
#33608=CARTESIAN_POINT('Ctrl Pts',(-0.388554011035329,2.03908472680553,
9.29348586565328));
#33609=CARTESIAN_POINT('Ctrl Pts',(-0.38537523039336,2.01880856445958,9.29452031244514));
#33610=CARTESIAN_POINT('Ctrl Pts',(-0.380603838057588,1.99877431598211,
9.29555475923701));
#33611=CARTESIAN_POINT('Ctrl Pts',(-0.374303944301932,1.97924633637021,
9.29658920602887));
#33612=CARTESIAN_POINT('Ctrl Pts',(-0.368002981927405,1.95971504432665,
9.29762382828868));
#33613=CARTESIAN_POINT('Ctrl Pts',(-0.360173260756547,1.94069089294415,
9.29865845054849));
#33614=CARTESIAN_POINT('Ctrl Pts',(-0.35092797359622,1.92242058861554,9.29969307280829));
#33615=CARTESIAN_POINT('Ctrl Pts',(-0.341662002305568,1.90410940882799,
9.30073000978924));
#33616=CARTESIAN_POINT('Ctrl Pts',(-0.330974525908466,1.88655608541954,
9.30176694677018));
#33617=CARTESIAN_POINT('Ctrl Pts',(-0.319023789824703,1.86998106267987,
9.30280388375113));
#33618=CARTESIAN_POINT('Ctrl Pts',(-0.312832335224616,1.86139385097434,
9.30334110155894));
#33619=CARTESIAN_POINT('Ctrl Pts',(-0.30630249965348,1.85306870619157,9.30387831936676));
#33620=CARTESIAN_POINT('Ctrl Pts',(-0.299460328225751,1.84503254753023,
9.30441553717457));
#33621=CARTESIAN_POINT('Ctrl Pts',(-0.286164098475349,1.82941607065582,
9.30545949982212));
#33622=CARTESIAN_POINT('Ctrl Pts',(-0.271603393677206,1.81479593609752,
9.30650346246968));
#33623=CARTESIAN_POINT('Ctrl Pts',(-0.255953144490233,1.80138171886912,
9.30754742511723));
#33624=CARTESIAN_POINT('Ctrl Pts',(-0.240331685623043,1.78799217853877,
9.308589467283));
#33625=CARTESIAN_POINT('Ctrl Pts',(-0.223625174529091,1.77580467065087,
9.30963150944877));
#33626=CARTESIAN_POINT('Ctrl Pts',(-0.206045737474445,1.76499247162398,
9.31067355161454));
#33627=CARTESIAN_POINT('Ctrl Pts',(-0.188485180459032,1.75419188472898,
9.31171447464339));
#33628=CARTESIAN_POINT('Ctrl Pts',(-0.170054167058535,1.74476408252427,
9.31275539767224));
#33629=CARTESIAN_POINT('Ctrl Pts',(-0.150994123480303,1.73683934040921,
9.3137963207011));
#33630=CARTESIAN_POINT('Ctrl Pts',(-0.131924291160454,1.72891052835315,
9.31483777832089));
#33631=CARTESIAN_POINT('Ctrl Pts',(-0.112225456479429,1.72248661589742,
9.31587923594068));
#33632=CARTESIAN_POINT('Ctrl Pts',(-0.0921599033865566,1.71765010499834,
9.31692069356047));
#33633=CARTESIAN_POINT('Ctrl Pts',(-0.0720882193924271,1.71281211633433,
9.31796246939097));
#33634=CARTESIAN_POINT('Ctrl Pts',(-0.051650317092855,1.70956263188016,
9.31900424522146));
#33635=CARTESIAN_POINT('Ctrl Pts',(-0.0311186819455137,1.7079330189445,
9.32004602105196));
#33636=CARTESIAN_POINT('Ctrl Pts',(-0.0105426672028801,1.7062998835635,
9.32109004870456));
#33637=CARTESIAN_POINT('Ctrl Pts',(0.0101267484021445,1.70629361027658,
9.32213407635715));
#33638=CARTESIAN_POINT('Ctrl Pts',(0.0306163259953106,1.70789347036481,
9.32317810400975));
#33639=CARTESIAN_POINT('Ctrl Pts',(0.0378632210177484,1.70845931990746,
9.32354736290562));
#33640=CARTESIAN_POINT('Ctrl Pts',(0.0450876813134371,1.70922561461252,
9.32391662180149));
#33641=CARTESIAN_POINT('Ctrl Pts',(0.0522779124983442,1.71018990538364,
9.32428588069736));
#33642=CARTESIAN_POINT('Ctrl Pts',(0.0726060152693199,1.71291613231464,
9.32532984334491));
#33643=CARTESIAN_POINT('Ctrl Pts',(0.0927808587729757,1.71724489060391,
9.32637380599247));
#33644=CARTESIAN_POINT('Ctrl Pts',(0.112531535458932,1.72314254216315,9.32741776864002));
#33645=CARTESIAN_POINT('Ctrl Pts',(0.132245878646874,1.72902934435684,9.32845981080579));
#33646=CARTESIAN_POINT('Ctrl Pts',(0.151536889811539,1.73647915977044,9.32950185297157));
#33647=CARTESIAN_POINT('Ctrl Pts',(0.17014404725711,1.74540742649772,9.33054389513734));
#33648=CARTESIAN_POINT('Ctrl Pts',(0.188731220907897,1.75432610440679,9.3315848181662));
#33649=CARTESIAN_POINT('Ctrl Pts',(0.206635326381617,1.76471979078693,9.33262574119505));
#33650=CARTESIAN_POINT('Ctrl Pts',(0.22361613742165,1.77645601058802,9.33366666422391));
#33651=CARTESIAN_POINT('Ctrl Pts',(0.240605669363653,1.7881982578057,9.3347081218437));
#33652=CARTESIAN_POINT('Ctrl Pts',(0.256670345120845,1.80128401081605,9.33574957946349));
#33653=CARTESIAN_POINT('Ctrl Pts',(0.271598816530265,1.81553739637808,9.33679103708329));
#33654=CARTESIAN_POINT('Ctrl Pts',(0.286531849238524,1.8297951369708,9.33783281291379));
#33655=CARTESIAN_POINT('Ctrl Pts',(0.300327479751835,1.84522068650289,9.33887458874429));
#33656=CARTESIAN_POINT('Ctrl Pts',(0.312811832573712,1.86160191401382,9.33991636457479));
#33657=CARTESIAN_POINT('Ctrl Pts',(0.325323170607521,1.87801854991974,9.34096039222739));
#33658=CARTESIAN_POINT('Ctrl Pts',(0.336517173439119,1.89539436879011,9.34200441987999));
#33659=CARTESIAN_POINT('Ctrl Pts',(0.346263361006765,1.91348840565719,9.34304844753258));
#33660=CARTESIAN_POINT('Ctrl Pts',(0.349710459798716,1.91988802932471,9.34341770642844));
#33661=CARTESIAN_POINT('Ctrl Pts',(0.352976876386308,1.92637729406053,9.3437869653243));
#33662=CARTESIAN_POINT('Ctrl Pts',(0.356058285500431,1.93294495719526,9.34415622422015));
#33663=CARTESIAN_POINT('Ctrl Pts',(0.364769994420846,1.95151294586476,9.34520018686771));
#33664=CARTESIAN_POINT('Ctrl Pts',(0.372051304272281,1.97081955057842,9.34624414951526));
#33665=CARTESIAN_POINT('Ctrl Pts',(0.37778385140963,1.99061877851246,9.34728811216281));
#33666=CARTESIAN_POINT('Ctrl Pts',(0.383505852908803,2.01038158363322,9.34833015432858));
#33667=CARTESIAN_POINT('Ctrl Pts',(0.38768448763457,2.03063453090711,9.34937219649435));
#33668=CARTESIAN_POINT('Ctrl Pts',(0.390249831650448,2.05111279414001,9.35041423866012));
#33669=CARTESIAN_POINT('Ctrl Pts',(0.392812420527153,2.0715690640399,9.35145516168897));
#33670=CARTESIAN_POINT('Ctrl Pts',(0.393765038725769,2.09224944672371,9.35249608471783));
#33671=CARTESIAN_POINT('Ctrl Pts',(0.393089034827,2.11288024451545,9.35353700774668));
#33672=CARTESIAN_POINT('Ctrl Pts',(0.392412683750247,2.13352163774723,9.35457846536648));
#33673=CARTESIAN_POINT('Ctrl Pts',(0.390106047584464,2.15411265930102,9.35561992298627));
#33674=CARTESIAN_POINT('Ctrl Pts',(0.38620259712012,2.17438040049418,9.35666138060606));
#33675=CARTESIAN_POINT('Ctrl Pts',(0.382297953981481,2.19465433436588,9.35770315643656));
#33676=CARTESIAN_POINT('Ctrl Pts',(0.376795699818046,2.21460407618743,9.35874493226706));
#33677=CARTESIAN_POINT('Ctrl Pts',(0.369780076191529,2.23396859800635,9.35978670809756));
#33678=CARTESIAN_POINT('Ctrl Pts',(0.36274928813534,2.25337497667862,9.36083073575015));
#33679=CARTESIAN_POINT('Ctrl Pts',(0.354198904521378,2.27219293939679,9.36187476340275));
#33680=CARTESIAN_POINT('Ctrl Pts',(0.344260901793801,2.29018233749778,9.36291879105535));
#33681=CARTESIAN_POINT('Ctrl Pts',(0.340745960493972,2.29654495180546,9.36328804995121));
#33682=CARTESIAN_POINT('Ctrl Pts',(0.337057840837003,2.30280416961069,9.36365730884708));
#33683=CARTESIAN_POINT('Ctrl Pts',(0.333203654514282,2.30895026828967,9.36402656774294));
#33684=CARTESIAN_POINT('Ctrl Pts',(0.322307162641795,2.32632641689679,9.36507053039049));
#33685=CARTESIAN_POINT('Ctrl Pts',(0.310015328313207,2.34289968656694,9.36611449303804));
#33686=CARTESIAN_POINT('Ctrl Pts',(0.296470914319315,2.35843739466778,9.3671584556856));
#33687=CARTESIAN_POINT('Ctrl Pts',(0.282951416734462,2.37394651948028,9.36820049785136));
#33688=CARTESIAN_POINT('Ctrl Pts',(0.26818434653026,2.38842327668046,9.36924254001713));
#33689=CARTESIAN_POINT('Ctrl Pts',(0.252354523221998,2.40166551776661,9.3702845821829));
#33690=CARTESIAN_POINT('Ctrl Pts',(0.236541700895282,2.41489353689388,9.37132550521175));
#33691=CARTESIAN_POINT('Ctrl Pts',(0.219668934308881,2.42688918014886,9.37236642824061));
#33692=CARTESIAN_POINT('Ctrl Pts',(0.201956257018866,2.43748860758688,9.37340735126946));
#33693=CARTESIAN_POINT('Ctrl Pts',(0.184234482959447,2.44809347861457,9.37444880888925));
#33694=CARTESIAN_POINT('Ctrl Pts',(0.165672559532684,2.4573003096507,9.37549026650904));
#33695=CARTESIAN_POINT('Ctrl Pts',(0.146518071588861,2.46498951313412,9.37653172412883));
#33696=CARTESIAN_POINT('Ctrl Pts',(0.127357731113906,2.47268106600442,9.37757349995933));
#33697=CARTESIAN_POINT('Ctrl Pts',(0.10760516140445,2.47885382790631,9.37861527578982));
#33698=CARTESIAN_POINT('Ctrl Pts',(0.0875254409159908,2.48343733150603,
9.37965705162032));
#33699=CARTESIAN_POINT('Ctrl Pts',(0.0674023176560223,2.48803074245278,
9.38070107927292));
#33700=CARTESIAN_POINT('Ctrl Pts',(0.0469513605327151,2.49102793005919,
9.38174510692551));
#33701=CARTESIAN_POINT('Ctrl Pts',(0.026445932075582,2.49240986567192,9.38278913457811));
#33702=CARTESIAN_POINT('Ctrl Pts',(0.0191934308102392,2.49289863818408,
9.38315839347398));
#33703=CARTESIAN_POINT('Ctrl Pts',(0.0119341226015544,2.49318582883786,
9.38352765236985));
#33704=CARTESIAN_POINT('Ctrl Pts',(0.00468003209273598,2.49327215423878,
9.38389691126573));
#33705=CARTESIAN_POINT('Ctrl Pts',(-0.0158286127031104,2.49351621198553,
9.38494087391328));
#33706=CARTESIAN_POINT('Ctrl Pts',(-0.0364175065974294,2.49215242793676,
9.38598483656084));
#33707=CARTESIAN_POINT('Ctrl Pts',(-0.0568137257886784,2.48917488428984,
9.38702879920839));
#33708=CARTESIAN_POINT('Ctrl Pts',(-0.0771724239369054,2.48620281815531,
9.38807084137416));
#33709=CARTESIAN_POINT('Ctrl Pts',(-0.0973384225138492,2.48162293138315,
9.38911288353993));
#33710=CARTESIAN_POINT('Ctrl Pts',(-0.117041705296821,2.47548119689435,
9.3901549257057));
#33711=CARTESIAN_POINT('Ctrl Pts',(-0.136723827063587,2.46934605853191,
9.39119584873456));
#33712=CARTESIAN_POINT('Ctrl Pts',(-0.155943512111755,2.46165259273099,
9.39223677176341));
#33713=CARTESIAN_POINT('Ctrl Pts',(-0.174443892742717,2.45249711812264,
9.39327769479227));
#33714=CARTESIAN_POINT('Ctrl Pts',(-0.192953774687013,2.44333694150115,
9.39431915241206));
#33715=CARTESIAN_POINT('Ctrl Pts',(-0.210742947608435,2.43271356794082,
9.39536061003185));
#33716=CARTESIAN_POINT('Ctrl Pts',(-0.227576837991387,2.42077043630896,
9.39640206765164));
#33717=CARTESIAN_POINT('Ctrl Pts',(-0.244415871861747,2.40882365552972,
9.39744384348214));
#33718=CARTESIAN_POINT('Ctrl Pts',(-0.260298463478385,2.39555676881259,
9.39848561931264));
#33719=CARTESIAN_POINT('Ctrl Pts',(-0.275021870887769,2.38115451362799,
9.39952739514314));
#33720=CARTESIAN_POINT('Ctrl Pts',(-0.289777103276389,2.36672112764198,
9.40057142279574));
#33721=CARTESIAN_POINT('Ctrl Pts',(-0.303367664894849,2.35114802853795,
9.40161545044833));
#33722=CARTESIAN_POINT('Ctrl Pts',(-0.315629580034159,2.33465476387122,
9.40265947810093));
#33723=CARTESIAN_POINT('Ctrl Pts',(-0.319966458692713,2.32882131234833,
9.4030287369968));
#33724=CARTESIAN_POINT('Ctrl Pts',(-0.324137528436977,2.32287301752332,
9.40339799589266));
#33725=CARTESIAN_POINT('Ctrl Pts',(-0.328136882645062,2.316820377843,9.40376725478852));
#33726=CARTESIAN_POINT('Ctrl Pts',(-0.339658331581068,2.29938376798637,
9.40483102591043));
#33727=CARTESIAN_POINT('Ctrl Pts',(-0.349818092913587,2.28097840474098,
9.40589479703233));
#33728=CARTESIAN_POINT('Ctrl Pts',(-0.358459289317414,2.26183889489877,
9.40695856815424));
#33729=CARTESIAN_POINT('Ctrl Pts',(-0.367081814167475,2.24274074094877,
9.40802004072178));
#33730=CARTESIAN_POINT('Ctrl Pts',(-0.374191950452327,2.22291219397477,
9.40908151328933));
#33731=CARTESIAN_POINT('Ctrl Pts',(-0.379677967326944,2.20261350362638,
9.41014298585687));
#33732=CARTESIAN_POINT('Ctrl Pts',(-0.385155640934468,2.182345684017,9.41120284411127));
#33733=CARTESIAN_POINT('Ctrl Pts',(-0.389013881777438,2.16160980076571,
9.41226270236567));
#33734=CARTESIAN_POINT('Ctrl Pts',(-0.391190239428219,2.14068275526673,
9.41332256062008));
#33735=CARTESIAN_POINT('Ctrl Pts',(-0.392601013880606,2.12711727298338,
9.41400958967889));
#33736=CARTESIAN_POINT('Ctrl Pts',(-0.39330607589307,2.11347180629114,9.41469661873771));
#33737=CARTESIAN_POINT('Ctrl Pts',(-0.393299960517938,2.09982377120348,
9.41538364779652));
#33738=CARTESIAN_POINT('',(-0.393426948843716,2.09973322299738,9.54038364779652));
#33739=CARTESIAN_POINT('Ctrl Pts',(-0.393299960517904,2.09982377112743,
9.41538364780035));
#33740=CARTESIAN_POINT('Ctrl Pts',(-0.393289814354333,2.07718000297793,
9.41652351347478));
#33741=CARTESIAN_POINT('Ctrl Pts',(-0.391319955513586,2.05460099316646,
9.41766337914921));
#33742=CARTESIAN_POINT('Ctrl Pts',(-0.387448452243393,2.03240867767088,
9.41880324482365));
#33743=CARTESIAN_POINT('Ctrl Pts',(-0.383550246883438,2.0100632998739,9.4199509722493));
#33744=CARTESIAN_POINT('Ctrl Pts',(-0.377724278371578,1.98811043056177,
9.42109869967495));
#33745=CARTESIAN_POINT('Ctrl Pts',(-0.37007930774543,1.96686023892667,9.42224642710061));
#33746=CARTESIAN_POINT('Ctrl Pts',(-0.366990460804913,1.95827438652418,
9.42271015083751));
#33747=CARTESIAN_POINT('Ctrl Pts',(-0.363605213018767,1.9498029952863,9.42317387457441));
#33748=CARTESIAN_POINT('Ctrl Pts',(-0.359932879358728,1.94146542220533,
9.42363759831132));
#33749=CARTESIAN_POINT('Ctrl Pts',(-0.35166550189812,1.92269537837302,9.42468156095887));
#33750=CARTESIAN_POINT('Ctrl Pts',(-0.341901287220695,1.9045178491005,9.42572552360642));
#33751=CARTESIAN_POINT('Ctrl Pts',(-0.3307478250219,1.88718372655438,9.42676948625397));
#33752=CARTESIAN_POINT('Ctrl Pts',(-0.319614880818674,1.86988149199454,
9.42781152841974));
#33753=CARTESIAN_POINT('Ctrl Pts',(-0.307098105623127,1.85342022836891,
9.42885357058551));
#33754=CARTESIAN_POINT('Ctrl Pts',(-0.293351121657722,1.83802670093661,
9.42989561275128));
#33755=CARTESIAN_POINT('Ctrl Pts',(-0.279618901737133,1.82264970591094,
9.43093653578013));
#33756=CARTESIAN_POINT('Ctrl Pts',(-0.264659562032265,1.80833873581896,
9.43197745880898));
#33757=CARTESIAN_POINT('Ctrl Pts',(-0.248667111632916,1.79528774623894,
9.43301838183783));
#33758=CARTESIAN_POINT('Ctrl Pts',(-0.232666447927859,1.78223005401083,
9.43405983945762));
#33759=CARTESIAN_POINT('Ctrl Pts',(-0.215632173408295,1.77043411273341,
9.43510129707741));
#33760=CARTESIAN_POINT('Ctrl Pts',(-0.197791962042116,1.76005407819547,
9.43614275469719));
#33761=CARTESIAN_POINT('Ctrl Pts',(-0.179946299713597,1.74967087210445,
9.43718453052769));
#33762=CARTESIAN_POINT('Ctrl Pts',(-0.161294863939316,1.74070477244063,
9.43822630635818));
#33763=CARTESIAN_POINT('Ctrl Pts',(-0.142089746140225,1.7332638631907,9.43926808218868));
#33764=CARTESIAN_POINT('Ctrl Pts',(-0.122843116043193,1.72580687024658,
9.44031210984127));
#33765=CARTESIAN_POINT('Ctrl Pts',(-0.103041120146565,1.71988186059964,
9.44135613749387));
#33766=CARTESIAN_POINT('Ctrl Pts',(-0.0829514902189006,1.71554721971292,
9.44240016514646));
#33767=CARTESIAN_POINT('Ctrl Pts',(-0.0758460514431546,1.71401411404864,
9.44276942404234));
#33768=CARTESIAN_POINT('Ctrl Pts',(-0.0687047073434924,1.71267948354105,
9.44313868293822));
#33769=CARTESIAN_POINT('Ctrl Pts',(-0.0615394596976218,1.71154435916037,
9.4435079418341));
#33770=CARTESIAN_POINT('Ctrl Pts',(-0.0412819899758406,1.70833515427195,
9.44455190448165));
#33771=CARTESIAN_POINT('Ctrl Pts',(-0.0207124520729407,1.70670525575265,
9.4455958671292));
#33772=CARTESIAN_POINT('Ctrl Pts',(-0.000100040860850534,1.70670001272333,
9.44663982977675));
#33773=CARTESIAN_POINT('Ctrl Pts',(0.0204744515997068,1.70669477933914,
9.44768187194252));
#33774=CARTESIAN_POINT('Ctrl Pts',(0.0410909333620938,1.70830832859201,
9.44872391410829));
#33775=CARTESIAN_POINT('Ctrl Pts',(0.0614755776515536,1.71153424429892,
9.44976595627406));
#33776=CARTESIAN_POINT('Ctrl Pts',(0.0818383291532756,1.71475669542305,
9.45080687930291));
#33777=CARTESIAN_POINT('Ctrl Pts',(0.101969009916113,1.71958798939108,9.45184780233177));
#33778=CARTESIAN_POINT('Ctrl Pts',(0.121599517991356,1.72596999154577,9.45288872536062));
#33779=CARTESIAN_POINT('Ctrl Pts',(0.141240107783906,1.73235527133043,9.45393018298041));
#33780=CARTESIAN_POINT('Ctrl Pts',(0.160379306996292,1.74029263818211,9.4549716406002));
#33781=CARTESIAN_POINT('Ctrl Pts',(0.178764254648609,1.74967410706611,9.45601309821999));
#33782=CARTESIAN_POINT('Ctrl Pts',(0.197154819703953,1.75905844239786,9.45705487405049));
#33783=CARTESIAN_POINT('Ctrl Pts',(0.214790036028478,1.76988739178421,9.45809664988099));
#33784=CARTESIAN_POINT('Ctrl Pts',(0.231442563029828,1.78200750005985,9.45913842571149));
#33785=CARTESIAN_POINT('Ctrl Pts',(0.248131084846188,1.79415380622457,9.46018245336409));
#33786=CARTESIAN_POINT('Ctrl Pts',(0.263832117219195,1.80759636413703,9.46122648101668));
#33787=CARTESIAN_POINT('Ctrl Pts',(0.278351640562251,1.82214166523873,9.46227050866928));
#33788=CARTESIAN_POINT('Ctrl Pts',(0.283487005650375,1.82728614758221,9.46263976756515));
#33789=CARTESIAN_POINT('Ctrl Pts',(0.288474925473794,1.83256825795341,9.46300902646101));
#33790=CARTESIAN_POINT('Ctrl Pts',(0.293308036395142,1.83797846312559,9.46337828535688));
#33791=CARTESIAN_POINT('Ctrl Pts',(0.306972127713828,1.85327410577244,9.46442224800444));
#33792=CARTESIAN_POINT('Ctrl Pts',(0.319477238105998,1.86968704800722,9.46546621065199));
#33793=CARTESIAN_POINT('Ctrl Pts',(0.330639517170663,1.88701549426038,9.46651017329954));
#33794=CARTESIAN_POINT('Ctrl Pts',(0.341781262020188,1.90431206296942,9.46755221546532));
#33795=CARTESIAN_POINT('Ctrl Pts',(0.351584635012941,1.92252021332621,9.46859425763109));
#33796=CARTESIAN_POINT('Ctrl Pts',(0.359906803609566,1.94140623368005,9.46963629979686));
#33797=CARTESIAN_POINT('Ctrl Pts',(0.368220034327855,1.96027197074473,9.47067722282571));
#33798=CARTESIAN_POINT('Ctrl Pts',(0.375054897093438,1.97981347427841,9.47171814585457));
#33799=CARTESIAN_POINT('Ctrl Pts',(0.380315144137853,1.99977385002204,9.47275906888342));
#33800=CARTESIAN_POINT('Ctrl Pts',(0.385578092708052,2.01974447689443,9.47380052650322));
#33801=CARTESIAN_POINT('Ctrl Pts',(0.389264606902548,2.04013369836372,9.47484198412301));
#33802=CARTESIAN_POINT('Ctrl Pts',(0.391328604254572,2.06067045014027,9.4758834417428));
#33803=CARTESIAN_POINT('Ctrl Pts',(0.393393232247769,2.08121347678982,9.4769252175733));
#33804=CARTESIAN_POINT('Ctrl Pts',(0.393834318962646,2.10190338839271,9.4779669934038));
#33805=CARTESIAN_POINT('Ctrl Pts',(0.392657828679303,2.12246596485476,9.4790087692343));
#33806=CARTESIAN_POINT('Ctrl Pts',(0.391478795385515,2.14307298779246,9.48005279688689));
#33807=CARTESIAN_POINT('Ctrl Pts',(0.388675304535151,2.16355139641863,9.48109682453949));
#33808=CARTESIAN_POINT('Ctrl Pts',(0.384305035280898,2.18363330591187,9.48214085219209));
#33809=CARTESIAN_POINT('Ctrl Pts',(0.382759328330096,2.19073601407084,9.48251011108795));
#33810=CARTESIAN_POINT('Ctrl Pts',(0.38101808648348,2.19778924814953,9.48287936998382));
#33811=CARTESIAN_POINT('Ctrl Pts',(0.379085339378842,2.20478165616189,9.48324862887968));
#33812=CARTESIAN_POINT('Ctrl Pts',(0.373621108707589,2.22455047652922,9.48429259152723));
#33813=CARTESIAN_POINT('Ctrl Pts',(0.36659005522126,2.24394961943798,9.48533655417478));
#33814=CARTESIAN_POINT('Ctrl Pts',(0.358062330703742,2.26271526459126,9.48638051682234));
#33815=CARTESIAN_POINT('Ctrl Pts',(0.34955029385439,2.28144638831817,9.4874225589881));
#33816=CARTESIAN_POINT('Ctrl Pts',(0.339547297965382,2.29954564064235,9.48846460115387));
#33817=CARTESIAN_POINT('Ctrl Pts',(0.328172534142725,2.31676641306794,9.48950664331964));
#33818=CARTESIAN_POINT('Ctrl Pts',(0.316809986637721,2.33396869065449,9.49054756634849));
#33819=CARTESIAN_POINT('Ctrl Pts',(0.304078975301178,2.35029373459713,9.49158848937735));
#33820=CARTESIAN_POINT('Ctrl Pts',(0.290143400769497,2.36552155654468,9.4926294124062));
#33821=CARTESIAN_POINT('Ctrl Pts',(0.276200669289935,2.38075719910471,9.49367087002599));
#33822=CARTESIAN_POINT('Ctrl Pts',(0.261052623566681,2.39489394023539,9.49471232764578));
#33823=CARTESIAN_POINT('Ctrl Pts',(0.244902234035801,2.40774630097578,9.49575378526557));
#33824=CARTESIAN_POINT('Ctrl Pts',(0.228746909856824,2.42060258867269,9.49679556109607));
#33825=CARTESIAN_POINT('Ctrl Pts',(0.211589229949701,2.43217328527357,9.49783733692657));
#33826=CARTESIAN_POINT('Ctrl Pts',(0.193662992051958,2.4423149653601,9.49887911275706));
#33827=CARTESIAN_POINT('Ctrl Pts',(0.175698006184199,2.45247856691827,9.49992314040966));
#33828=CARTESIAN_POINT('Ctrl Pts',(0.156961813304875,2.46120667422723,9.50096716806226));
#33829=CARTESIAN_POINT('Ctrl Pts',(0.137710878535675,2.46840277405705,9.50201119571485));
#33830=CARTESIAN_POINT('Ctrl Pts',(0.130902075244271,2.47094794024218,9.50238045461072));
#33831=CARTESIAN_POINT('Ctrl Pts',(0.124029024073178,2.47330191597236,9.50274971350659));
#33832=CARTESIAN_POINT('Ctrl Pts',(0.117103451291254,2.47546194440406,9.50311897240246));
#33833=CARTESIAN_POINT('Ctrl Pts',(0.0975235863831054,2.48156874108674,
9.50416293505001));
#33834=CARTESIAN_POINT('Ctrl Pts',(0.077406403400487,2.48615801200553,9.50520689769757));
#33835=CARTESIAN_POINT('Ctrl Pts',(0.0570117016007467,2.48914593134271,
9.50625086034512));
#33836=CARTESIAN_POINT('Ctrl Pts',(0.0366545180526232,2.4921283540803,9.50729290251089));
#33837=CARTESIAN_POINT('Ctrl Pts',(0.0160215402250951,2.49351510835516,
9.50833494467666));
#33838=CARTESIAN_POINT('Ctrl Pts',(-0.00461535874382263,2.49327291854851,
9.50937698684243));
#33839=CARTESIAN_POINT('Ctrl Pts',(-0.0252300940074508,2.49303098884992,
9.51041790987129));
#33840=CARTESIAN_POINT('Ctrl Pts',(-0.0458480097155451,2.49116356783821,
9.51145883290014));
#33841=CARTESIAN_POINT('Ctrl Pts',(-0.0661954133476839,2.48768938243358,
9.512499755929));
#33842=CARTESIAN_POINT('Ctrl Pts',(-0.0865532668760106,2.48421341277787,
9.51354121354879));
#33843=CARTESIAN_POINT('Ctrl Pts',(-0.106639602786151,2.47912913812606,
9.51458267116858));
#33844=CARTESIAN_POINT('Ctrl Pts',(-0.126188595482363,2.47250681654191,
9.51562412878838));
#33845=CARTESIAN_POINT('Ctrl Pts',(-0.145743561248111,2.4658824715498,9.51666590461888));
#33846=CARTESIAN_POINT('Ctrl Pts',(-0.164760172269669,2.45771941422547,
9.51770768044937));
#33847=CARTESIAN_POINT('Ctrl Pts',(-0.182991274947575,2.44813658712215,
9.51874945627987));
#33848=CARTESIAN_POINT('Ctrl Pts',(-0.201261784567633,2.43853304652059,
9.51979348393247));
#33849=CARTESIAN_POINT('Ctrl Pts',(-0.218742773211489,2.42750400228088,
9.52083751158507));
#33850=CARTESIAN_POINT('Ctrl Pts',(-0.235214261623028,2.41521285051396,
9.52188153923767));
#33851=CARTESIAN_POINT('Ctrl Pts',(-0.241040011169962,2.41086563124339,
9.52225079813353));
#33852=CARTESIAN_POINT('Ctrl Pts',(-0.246739782897403,2.40636089635743,
9.5226200570294));
#33853=CARTESIAN_POINT('Ctrl Pts',(-0.252304911160714,2.40170701318362,
9.52298931592526));
#33854=CARTESIAN_POINT('Ctrl Pts',(-0.267819426598198,2.38873287513542,
9.52401873925017));
#33855=CARTESIAN_POINT('Ctrl Pts',(-0.282382930556754,2.37451483139563,
9.52504816257507));
#33856=CARTESIAN_POINT('Ctrl Pts',(-0.295787278418756,2.35921955158827,
9.52607758589997));
#33857=CARTESIAN_POINT('Ctrl Pts',(-0.30916686412036,2.34395252710343,9.52710510754747));
#33858=CARTESIAN_POINT('Ctrl Pts',(-0.32139099986214,2.32761273538655,9.52813262919496));
#33859=CARTESIAN_POINT('Ctrl Pts',(-0.332287146187854,2.31040471116002,
9.52916015084246));
#33860=CARTESIAN_POINT('Ctrl Pts',(-0.34317923556318,2.29320309397856,9.53018728991393));
#33861=CARTESIAN_POINT('Ctrl Pts',(-0.352743871297665,2.27513449803517,
9.5312144289854));
#33862=CARTESIAN_POINT('Ctrl Pts',(-0.36085089247073,2.25643376682506,9.53224156805687));
#33863=CARTESIAN_POINT('Ctrl Pts',(-0.368955606577506,2.23773835740031,
9.53326841482888));
#33864=CARTESIAN_POINT('Ctrl Pts',(-0.375603236691946,2.21841186921687,
9.53429526160089));
#33865=CARTESIAN_POINT('Ctrl Pts',(-0.380711562407097,2.19870965631359,
9.5353221083729));
#33866=CARTESIAN_POINT('Ctrl Pts',(-0.385828946432143,2.1789725065719,9.53635077599518));
#33867=CARTESIAN_POINT('Ctrl Pts',(-0.389401416802549,2.15885904512728,
9.53737944361746));
#33868=CARTESIAN_POINT('Ctrl Pts',(-0.391397696698209,2.13863590324215,
9.53840811123974));
#33869=CARTESIAN_POINT('Ctrl Pts',(-0.392675635858218,2.12568985043182,
9.53906662342533));
#33870=CARTESIAN_POINT('Ctrl Pts',(-0.393308701435708,2.11269901741784,
9.53972513561093));
#33871=CARTESIAN_POINT('Ctrl Pts',(-0.393299909580444,2.09973330914082,
9.54038364779652));
#33872=CARTESIAN_POINT('',(-0.39335257410733,2.10032199862207,9.66538364779652));
#33873=CARTESIAN_POINT('Ctrl Pts',(-0.393713022906921,2.09973302901478,
9.54038364779652));
#33874=CARTESIAN_POINT('Ctrl Pts',(-0.39383959327844,2.08346547400357,9.54120898501369));
#33875=CARTESIAN_POINT('Ctrl Pts',(-0.385530294422347,1.93677881389653,
9.54865777007186));
#33876=CARTESIAN_POINT('Ctrl Pts',(-0.201254141221434,1.68074851088445,
9.56273000297078));
#33877=CARTESIAN_POINT('Ctrl Pts',(0.243571655413408,1.7038335082775,9.58260034649366));
#33878=CARTESIAN_POINT('Ctrl Pts',(0.464953617493051,2.09034732862847,9.60247069001639));
#33879=CARTESIAN_POINT('Ctrl Pts',(0.259803933242123,2.48571616087013,9.62234103353921));
#33880=CARTESIAN_POINT('Ctrl Pts',(-0.183680490646769,2.52724292602718,
9.64221137706198));
#33881=CARTESIAN_POINT('Ctrl Pts',(-0.382233828622705,2.27422629591118,
9.65655891514776));
#33882=CARTESIAN_POINT('Ctrl Pts',(-0.393756568946857,2.12203738788098,
9.66428300539261));
#33883=CARTESIAN_POINT('Ctrl Pts',(-0.393564314774363,2.10032217195309,
9.66538364779652));
#33884=CARTESIAN_POINT('',(-0.393065748709506,2.1000925098763,9.7903836449317));
#33885=CARTESIAN_POINT('Ctrl Pts',(-0.393299868223561,2.10032195547701,
9.66538364779652));
#33886=CARTESIAN_POINT('Ctrl Pts',(-0.393316446318738,2.08007020294019,
9.6664108124149));
#33887=CARTESIAN_POINT('Ctrl Pts',(-0.391764536557221,2.05976190594462,
9.66743797703327));
#33888=CARTESIAN_POINT('Ctrl Pts',(-0.38864436446938,2.03966387511456,9.66846514165165));
#33889=CARTESIAN_POINT('Ctrl Pts',(-0.385528386016173,2.01959285683246,
9.66949092572017));
#33890=CARTESIAN_POINT('Ctrl Pts',(-0.380848399549848,1.99973229598539,
9.67051670978869));
#33891=CARTESIAN_POINT('Ctrl Pts',(-0.374656452113087,1.98034452419536,
9.67154249385721));
#33892=CARTESIAN_POINT('Ctrl Pts',(-0.368462833957878,1.96095152117423,
9.67256855470398));
#33893=CARTESIAN_POINT('Ctrl Pts',(-0.360756643960991,1.94203229391291,
9.67359461555075));
#33894=CARTESIAN_POINT('Ctrl Pts',(-0.351640021998056,1.92383477945631,
9.67462067639753));
#33895=CARTESIAN_POINT('Ctrl Pts',(-0.342521947302668,1.90563436522829,
9.67564690074695));
#33896=CARTESIAN_POINT('Ctrl Pts',(-0.331993363300273,1.8881565565742,9.67667312509638));
#33897=CARTESIAN_POINT('Ctrl Pts',(-0.320202169246142,1.87162429899382,
9.6776993494458));
#33898=CARTESIAN_POINT('Ctrl Pts',(-0.308386218692417,1.85505733069404,
9.67872772843051));
#33899=CARTESIAN_POINT('Ctrl Pts',(-0.295302856727771,1.83944045748286,
9.67975610741521));
#33900=CARTESIAN_POINT('Ctrl Pts',(-0.281140214503373,1.82496351189524,
9.68078448639991));
#33901=CARTESIAN_POINT('Ctrl Pts',(-0.275780327539312,1.81948467604632,
9.68117367896913));
#33902=CARTESIAN_POINT('Ctrl Pts',(-0.270266219843183,1.81416871195178,
9.68156287153835));
#33903=CARTESIAN_POINT('Ctrl Pts',(-0.264609301124671,1.8090243863168,9.68195206410757));
#33904=CARTESIAN_POINT('Ctrl Pts',(-0.249435291368448,1.79522534636968,
9.68299602675512));
#33905=CARTESIAN_POINT('Ctrl Pts',(-0.23313375991602,1.78257534514332,9.68403998940267));
#33906=CARTESIAN_POINT('Ctrl Pts',(-0.215904865923144,1.77126001327689,
9.68508395205022));
#33907=CARTESIAN_POINT('Ctrl Pts',(-0.198707666337281,1.75996549718273,
9.68612599421599));
#33908=CARTESIAN_POINT('Ctrl Pts',(-0.180587065928504,1.75000122589602,
9.68716803638176));
#33909=CARTESIAN_POINT('Ctrl Pts',(-0.161775502006798,1.7415120965075,9.68821007854753));
#33910=CARTESIAN_POINT('Ctrl Pts',(-0.142984141409238,1.73303208431059,
9.68925100157639));
#33911=CARTESIAN_POINT('Ctrl Pts',(-0.123503945868713,1.7260243963122,9.69029192460524));
#33912=CARTESIAN_POINT('Ctrl Pts',(-0.103590947029434,1.72058755200502,
9.69133284763409));
#33913=CARTESIAN_POINT('Ctrl Pts',(-0.0836677213929321,1.71514791547629,
9.69237430525388));
#33914=CARTESIAN_POINT('Ctrl Pts',(-0.0633119539506658,1.71128094368098,
9.69341576287367));
#33915=CARTESIAN_POINT('Ctrl Pts',(-0.0427942901722567,1.70903511829238,
9.69445722049347));
#33916=CARTESIAN_POINT('Ctrl Pts',(-0.0222703573530727,1.70678860670622,
9.69549899632396));
#33917=CARTESIAN_POINT('Ctrl Pts',(-0.00158516445215278,1.70616427163879,
9.69654077215446));
#33918=CARTESIAN_POINT('Ctrl Pts',(0.0189870263641044,1.70715857801162,
9.69758254798496));
#33919=CARTESIAN_POINT('Ctrl Pts',(0.0396036844376565,1.70815503360025,
9.69862657563756));
#33920=CARTESIAN_POINT('Ctrl Pts',(0.0601061222521713,1.7107770222481,9.69967060329015));
#33921=CARTESIAN_POINT('Ctrl Pts',(0.0802259545891204,1.71496923991678,
9.70071463094275));
#33922=CARTESIAN_POINT('Ctrl Pts',(0.0873420755609822,1.71645197235565,
9.70108388983862));
#33923=CARTESIAN_POINT('Ctrl Pts',(0.0944104563888153,1.71813067024748,
9.70145314873449));
#33924=CARTESIAN_POINT('Ctrl Pts',(0.101419709838481,1.72000140466539,9.70182240763036));
#33925=CARTESIAN_POINT('Ctrl Pts',(0.121236155347336,1.72529031409351,9.70286637027791));
#33926=CARTESIAN_POINT('Ctrl Pts',(0.140696816394127,1.73214925937274,9.70391033292547));
#33927=CARTESIAN_POINT('Ctrl Pts',(0.159537261646172,1.74051042832032,9.70495429557302));
#33928=CARTESIAN_POINT('Ctrl Pts',(0.178343047869007,1.74885621599665,9.70599633773879));
#33929=CARTESIAN_POINT('Ctrl Pts',(0.19653019399076,1.75869850116809,9.70703837990456));
#33930=CARTESIAN_POINT('Ctrl Pts',(0.213851045427472,1.76992028179608,9.70808042207033));
#33931=CARTESIAN_POINT('Ctrl Pts',(0.231153294541837,1.78113001040797,9.70912134509918));
#33932=CARTESIAN_POINT('Ctrl Pts',(0.247590465910109,1.79371591946494,9.71016226812803));
#33933=CARTESIAN_POINT('Ctrl Pts',(0.262941128023705,1.80751606335797,9.71120319115689));
#33934=CARTESIAN_POINT('Ctrl Pts',(0.278299673837276,1.82132329464522,9.71224464877668));
#33935=CARTESIAN_POINT('Ctrl Pts',(0.292570037680396,1.83634552666361,9.71328610639647));
#33936=CARTESIAN_POINT('Ctrl Pts',(0.30556495001116,1.85238143986228,9.71432756401626));
#33937=CARTESIAN_POINT('Ctrl Pts',(0.318563832854169,1.86842225273154,9.71536933984675));
#33938=CARTESIAN_POINT('Ctrl Pts',(0.330286053632177,1.88547676942525,9.71641111567725));
#33939=CARTESIAN_POINT('Ctrl Pts',(0.340586121636195,1.90331247180155,9.71745289150775));
#33940=CARTESIAN_POINT('Ctrl Pts',(0.350908453470948,1.92118672645329,9.71849691916034));
#33941=CARTESIAN_POINT('Ctrl Pts',(0.359802178515282,1.93984487308267,9.71954094681294));
#33942=CARTESIAN_POINT('Ctrl Pts',(0.367168515626677,1.95903131151741,9.72058497446553));
#33943=CARTESIAN_POINT('Ctrl Pts',(0.36977389250688,1.96581730330075,9.72095423336141));
#33944=CARTESIAN_POINT('Ctrl Pts',(0.372188655523025,1.9726692339568,9.72132349225728));
#33945=CARTESIAN_POINT('Ctrl Pts',(0.374409944071579,1.97957540209609,9.72169275115315));
#33946=CARTESIAN_POINT('Ctrl Pts',(0.380689934344148,1.99910040651919,9.7227367138007));
#33947=CARTESIAN_POINT('Ctrl Pts',(0.385457217804642,2.01917614977143,9.72378067644826));
#33948=CARTESIAN_POINT('Ctrl Pts',(0.388625670692114,2.039543585294,9.72482463909581));
#33949=CARTESIAN_POINT('Ctrl Pts',(0.391788294869081,2.05987355272421,9.72586668126158));
#33950=CARTESIAN_POINT('Ctrl Pts',(0.393357756093461,2.08049343761516,9.72690872342735));
#33951=CARTESIAN_POINT('Ctrl Pts',(0.393298371872983,2.10113167224099,9.72795076559312));
#33952=CARTESIAN_POINT('Ctrl Pts',(0.393239051430224,2.12174774172704,9.72899168862198));
#33953=CARTESIAN_POINT('Ctrl Pts',(0.39155433161465,2.14238138969642,9.73003261165083));
#33954=CARTESIAN_POINT('Ctrl Pts',(0.388260514317251,2.16275876848779,9.73107353467968));
#33955=CARTESIAN_POINT('Ctrl Pts',(0.384965005401136,2.18314661256979,9.73211499229948));
#33956=CARTESIAN_POINT('Ctrl Pts',(0.380058849553642,2.20327719561725,9.73315644991927));
#33957=CARTESIAN_POINT('Ctrl Pts',(0.373609947470832,2.22288408013588,9.73419790753906));
#33958=CARTESIAN_POINT('Ctrl Pts',(0.367159074967286,2.24249695541253,9.73523968336956));
#33959=CARTESIAN_POINT('Ctrl Pts',(0.359164781894791,2.26158512656372,9.73628145920006));
#33960=CARTESIAN_POINT('Ctrl Pts',(0.349743816920492,2.27990039612487,9.73732323503056));
#33961=CARTESIAN_POINT('Ctrl Pts',(0.340302488316614,2.29825525455681,9.73836726268316));
#33962=CARTESIAN_POINT('Ctrl Pts',(0.329428718633892,2.31583324971255,9.73941129033576));
#33963=CARTESIAN_POINT('Ctrl Pts',(0.317283949056236,2.33241296364721,9.74045531798835));
#33964=CARTESIAN_POINT('Ctrl Pts',(0.31298850324731,2.33827699114303,9.74082457688421));
#33965=CARTESIAN_POINT('Ctrl Pts',(0.308534432124841,2.34401644099237,9.74119383578008));
#33966=CARTESIAN_POINT('Ctrl Pts',(0.303930025930211,2.34962257377501,9.74156309467594));
#33967=CARTESIAN_POINT('Ctrl Pts',(0.290912524834874,2.3654721397242,9.74260705732349));
#33968=CARTESIAN_POINT('Ctrl Pts',(0.276613097141096,2.38034791958114,9.74365101997105));
#33969=CARTESIAN_POINT('Ctrl Pts',(0.261202933485644,2.3940372723627,9.7446949826186));
#33970=CARTESIAN_POINT('Ctrl Pts',(0.245821118486778,2.40770144210469,9.74573702478437));
#33971=CARTESIAN_POINT('Ctrl Pts',(0.229333127803274,2.42018298947153,9.74677906695014));
#33972=CARTESIAN_POINT('Ctrl Pts',(0.21194798486347,2.4313049074679,9.74782110911591));
#33973=CARTESIAN_POINT('Ctrl Pts',(0.194581513294059,2.44241488069908,9.74886203214476));
#33974=CARTESIAN_POINT('Ctrl Pts',(0.176320403371528,2.45216770458646,9.74990295517362));
#33975=CARTESIAN_POINT('Ctrl Pts',(0.157403735620761,2.46042884736468,9.75094387820247));
#33976=CARTESIAN_POINT('Ctrl Pts',(0.138477352762478,2.46869423285051,9.75198533582226));
#33977=CARTESIAN_POINT('Ctrl Pts',(0.118895407301652,2.47546609751238,9.75302679344205));
#33978=CARTESIAN_POINT('Ctrl Pts',(0.0989186805275231,2.4806573060414,9.75406825106184));
#33979=CARTESIAN_POINT('Ctrl Pts',(0.0789358499924424,2.48585010071094,
9.75511002689234));
#33980=CARTESIAN_POINT('Ctrl Pts',(0.0585587186387426,2.48946112790821,
9.75615180272284));
#33981=CARTESIAN_POINT('Ctrl Pts',(0.0380591735014942,2.49145419823063,
9.75719357855334));
#33982=CARTESIAN_POINT('Ctrl Pts',(0.0175153181322421,2.49345157661978,
9.75823760620593));
#33983=CARTESIAN_POINT('Ctrl Pts',(-0.00315074292368206,2.49382400277443,
9.75928163385853));
#33984=CARTESIAN_POINT('Ctrl Pts',(-0.0236654464639412,2.49258736179819,
9.76032566151113));
#33985=CARTESIAN_POINT('Ctrl Pts',(-0.030921228204479,2.49214997809448,
9.76069492040699));
#33986=CARTESIAN_POINT('Ctrl Pts',(-0.0381581295777627,2.49151178325602,
9.76106417930286));
#33987=CARTESIAN_POINT('Ctrl Pts',(-0.0453643146653507,2.49067501706014,
9.76143343819873));
#33988=CARTESIAN_POINT('Ctrl Pts',(-0.0657375220463668,2.48830932550062,
9.76247740084628));
#33989=CARTESIAN_POINT('Ctrl Pts',(-0.0859858826766692,2.4843386390981,
9.76352136349384));
#33990=CARTESIAN_POINT('Ctrl Pts',(-0.10583793562551,2.47879179159867,9.76456532614139));
#33991=CARTESIAN_POINT('Ctrl Pts',(-0.125653468583777,2.47325514812292,
9.76560736830716));
#33992=CARTESIAN_POINT('Ctrl Pts',(-0.145073424360301,2.46614823746583,
9.76664941047293));
#33993=CARTESIAN_POINT('Ctrl Pts',(-0.163835824145666,2.4575509931835,9.7676914526387));
#33994=CARTESIAN_POINT('Ctrl Pts',(-0.182578073408403,2.44896298220649,
9.76873237566755));
#33995=CARTESIAN_POINT('Ctrl Pts',(-0.200663491109591,2.43888809382229,
9.76977329869641));
#33996=CARTESIAN_POINT('Ctrl Pts',(-0.217849541924163,2.4274545267414,9.77081422172526));
#33997=CARTESIAN_POINT('Ctrl Pts',(-0.235044419046517,2.41601508767844,
9.77185567934505));
#33998=CARTESIAN_POINT('Ctrl Pts',(-0.251338385001536,2.4032159700336,9.77289713696484));
#33999=CARTESIAN_POINT('Ctrl Pts',(-0.266517009237516,2.38922927546687,
9.77393859458463));
#34000=CARTESIAN_POINT('Ctrl Pts',(-0.281700271204945,2.37523830735516,
9.77498037041513));
#34001=CARTESIAN_POINT('Ctrl Pts',(-0.295766996918788,2.36005956474198,
9.77602214624563));
#34002=CARTESIAN_POINT('Ctrl Pts',(-0.308539580316651,2.34390206513686,
9.77706392207613));
#34003=CARTESIAN_POINT('Ctrl Pts',(-0.321339771943368,2.32770964072969,
9.77810794972873));
#34004=CARTESIAN_POINT('Ctrl Pts',(-0.332839826783865,2.3105348475876,9.77915197738132));
#34005=CARTESIAN_POINT('Ctrl Pts',(-0.342905016613257,2.29261630144269,
9.78019600503392));
#34006=CARTESIAN_POINT('Ctrl Pts',(-0.346464942323886,2.28627874654312,
9.78056526392979));
#34007=CARTESIAN_POINT('Ctrl Pts',(-0.349845802153086,2.27984836389872,
9.78093452282565));
#34008=CARTESIAN_POINT('Ctrl Pts',(-0.353043072349212,2.27333631779356,
9.78130378172152));
#34009=CARTESIAN_POINT('Ctrl Pts',(-0.362743512461029,2.25357892809122,
9.7824241042421));
#34010=CARTESIAN_POINT('Ctrl Pts',(-0.370801759049986,2.23296418808786,
9.78354442676268));
#34011=CARTESIAN_POINT('Ctrl Pts',(-0.377083179295149,2.21177283163928,
9.78466474928327));
#34012=CARTESIAN_POINT('Ctrl Pts',(-0.383333005235826,2.1906880635325,9.78577943680261));
#34013=CARTESIAN_POINT('Ctrl Pts',(-0.387823576188697,2.16903297057527,
9.78689412432196));
#34014=CARTESIAN_POINT('Ctrl Pts',(-0.390468833763719,2.14710604907229,
9.78800881184131));
#34015=CARTESIAN_POINT('Ctrl Pts',(-0.392347399310581,2.13153434835279,
9.78880042230266));
#34016=CARTESIAN_POINT('Ctrl Pts',(-0.393296284805524,2.11582603520907,
9.78959203276402));
#34017=CARTESIAN_POINT('Ctrl Pts',(-0.39329998909922,2.10009259888561,9.79038364322537));
#34018=CARTESIAN_POINT('',(-0.393299834084712,2.09963873979202,9.91538365013564));
#34019=CARTESIAN_POINT('Ctrl Pts',(-0.392672473494722,2.10009236043514,
9.79038364779652));
#34020=CARTESIAN_POINT('Ctrl Pts',(-0.392522896058815,2.02871865682851,
9.79398047361245));
#34021=CARTESIAN_POINT('Ctrl Pts',(-0.339736212547102,1.82570629495234,
9.80420074726931));
#34022=CARTESIAN_POINT('Ctrl Pts',(-0.0137707264308251,1.63515012361188,
9.8210444687671));
#34023=CARTESIAN_POINT('Ctrl Pts',(0.383399755879578,1.8367896892674,9.84091481228989));
#34024=CARTESIAN_POINT('Ctrl Pts',(0.428853157334091,2.279888882172,9.86078515581266));
#34025=CARTESIAN_POINT('Ctrl Pts',(0.0808921700199272,2.55796451534366,
9.88065549933548));
#34026=CARTESIAN_POINT('Ctrl Pts',(-0.305777301598321,2.42786420633564,
9.8988549966634));
#34027=CARTESIAN_POINT('Ctrl Pts',(-0.392338317521313,2.19756855304251,
9.91043104615043));
#34028=CARTESIAN_POINT('Ctrl Pts',(-0.393224617787252,2.09963885513283,
9.91538364779652));
#34029=CARTESIAN_POINT('',(-0.393532055459869,2.10009220002109,10.0403836856852));
#34030=CARTESIAN_POINT('Ctrl Pts',(-0.393299834084712,2.09963873979202,
9.91538365013564));
#34031=CARTESIAN_POINT('Ctrl Pts',(-0.393275337824574,2.07296994307694,
9.91673212643577));
#34032=CARTESIAN_POINT('Ctrl Pts',(-0.390534469167157,2.04642365724893,
9.9180806027359));
#34033=CARTESIAN_POINT('Ctrl Pts',(-0.385173622860435,2.02046277442249,
9.91942907903603));
#34034=CARTESIAN_POINT('Ctrl Pts',(-0.383892049517696,2.01425652013338,
9.91975144815103));
#34035=CARTESIAN_POINT('Ctrl Pts',(-0.382460952053443,2.0080836142271,9.92007381726604));
#34036=CARTESIAN_POINT('Ctrl Pts',(-0.380882036249165,2.00195019396914,
9.92039618638104));
#34037=CARTESIAN_POINT('Ctrl Pts',(-0.375768863036924,1.9820876781355,9.92144014902859));
#34038=CARTESIAN_POINT('Ctrl Pts',(-0.369082564124017,1.96256702585223,
9.92248411167614));
#34039=CARTESIAN_POINT('Ctrl Pts',(-0.360888606771479,1.94365325874026,
9.92352807432368));
#34040=CARTESIAN_POINT('Ctrl Pts',(-0.352709723086441,1.92477428554096,
9.92457011648945));
#34041=CARTESIAN_POINT('Ctrl Pts',(-0.343028920867443,1.90650067260202,
9.92561215865521));
#34042=CARTESIAN_POINT('Ctrl Pts',(-0.331961003905475,1.88908110116429,
9.92665420082097));
#34043=CARTESIAN_POINT('Ctrl Pts',(-0.320904973712453,1.87168023807262,
9.92769512384982));
#34044=CARTESIAN_POINT('Ctrl Pts',(-0.308465154437204,1.85513222895444,
9.92873604687867));
#34045=CARTESIAN_POINT('Ctrl Pts',(-0.294801523954965,1.83965993110197,
9.92977696990752));
#34046=CARTESIAN_POINT('Ctrl Pts',(-0.281130876188233,1.82417968708059,
9.93081842752731));
#34047=CARTESIAN_POINT('Ctrl Pts',(-0.266235636533031,1.809776820191,9.93185988514709));
#34048=CARTESIAN_POINT('Ctrl Pts',(-0.250315457859235,1.7966403758627,9.93290134276688));
#34049=CARTESIAN_POINT('Ctrl Pts',(-0.234390414876792,1.78349991777797,
9.93394311859737));
#34050=CARTESIAN_POINT('Ctrl Pts',(-0.217440399509737,1.77162709255911,
9.93498489442787));
#34051=CARTESIAN_POINT('Ctrl Pts',(-0.199696632060677,1.76116944479043,
9.93602667025836));
#34052=CARTESIAN_POINT('Ctrl Pts',(-0.181914511055617,1.7506891925788,9.93707069791095));
#34053=CARTESIAN_POINT('Ctrl Pts',(-0.163335874611733,1.74163054760894,
9.93811472556354));
#34054=CARTESIAN_POINT('Ctrl Pts',(-0.144215437897276,1.73409455118556,
9.93915875321614));
#34055=CARTESIAN_POINT('Ctrl Pts',(-0.137452790056707,1.73142916803034,
9.93952801211204));
#34056=CARTESIAN_POINT('Ctrl Pts',(-0.130622517524043,1.72895380719259,
9.93989727100793));
#34057=CARTESIAN_POINT('Ctrl Pts',(-0.123736295891238,1.72667143281137,
9.94026652990383));
#34058=CARTESIAN_POINT('Ctrl Pts',(-0.104267683903116,1.72021874168276,
9.94131049255139));
#34059=CARTESIAN_POINT('Ctrl Pts',(-0.0842349555426453,1.71527381972604,
9.94235445519894));
#34060=CARTESIAN_POINT('Ctrl Pts',(-0.063896384345083,1.71192508188801,
9.9433984178465));
#34061=CARTESIAN_POINT('Ctrl Pts',(-0.0435952281408463,1.70858250441409,
9.94444046001226));
#34062=CARTESIAN_POINT('Ctrl Pts',(-0.0229900540417418,1.70683045938156,
9.94548250217804));
#34063=CARTESIAN_POINT('Ctrl Pts',(-0.0023521030540002,1.70670703335653,
9.94652454434381));
#34064=CARTESIAN_POINT('Ctrl Pts',(0.0182636830986,1.70658373988911,9.94756546737266));
#34065=CARTESIAN_POINT('Ctrl Pts',(0.0389114443941607,1.70808562632387,
9.94860639040152));
#34066=CARTESIAN_POINT('Ctrl Pts',(0.0593171995167528,1.71119881707807,
9.94964731343037));
#34067=CARTESIAN_POINT('Ctrl Pts',(0.0797334345033376,1.71431360668591,
9.95068877105016));
#34068=CARTESIAN_POINT('Ctrl Pts',(0.0999066852239352,1.71904125878756,
9.95173022866995));
#34069=CARTESIAN_POINT('Ctrl Pts',(0.1195699231907,1.7253162353822,9.95277168628974));
#34070=CARTESIAN_POINT('Ctrl Pts',(0.139239169133913,1.73159312925575,9.95381346212024));
#34071=CARTESIAN_POINT('Ctrl Pts',(0.158397402739161,1.73941803083677,9.95485523795074));
#34072=CARTESIAN_POINT('Ctrl Pts',(0.176795402150575,1.74867639450442,9.95589701378124));
#34073=CARTESIAN_POINT('Ctrl Pts',(0.195233169255211,1.75795477033522,9.95694104143384));
#34074=CARTESIAN_POINT('Ctrl Pts',(0.21290679173709,1.76867241229492,9.95798506908643));
#34075=CARTESIAN_POINT('Ctrl Pts',(0.229593430335173,1.78066984679343,9.95902909673903));
#34076=CARTESIAN_POINT('Ctrl Pts',(0.235495275682921,1.78491318211611,9.95939835563489));
#34077=CARTESIAN_POINT('Ctrl Pts',(0.241273953331664,1.78931624000458,9.95976761453075));
#34078=CARTESIAN_POINT('Ctrl Pts',(0.246920650771322,1.79387080795411,9.96013687342662));
#34079=CARTESIAN_POINT('Ctrl Pts',(0.262884900448396,1.8067474071866,9.96118083607417));
#34080=CARTESIAN_POINT('Ctrl Pts',(0.277886757195359,1.82091450826151,9.96222479872173));
#34081=CARTESIAN_POINT('Ctrl Pts',(0.291712072010568,1.83620281077445,9.96326876136928));
#34082=CARTESIAN_POINT('Ctrl Pts',(0.305511953669411,1.8514629888075,9.96431080353505));
#34083=CARTESIAN_POINT('Ctrl Pts',(0.31813905755377,1.86783977447944,9.96535284570082));
#34084=CARTESIAN_POINT('Ctrl Pts',(0.329414532139265,1.88512572044223,9.96639488786659));
#34085=CARTESIAN_POINT('Ctrl Pts',(0.340677897042187,1.90239310157061,9.96743581089545));
#34086=CARTESIAN_POINT('Ctrl Pts',(0.350592090308146,1.92056710721788,9.9684767339243));
#34087=CARTESIAN_POINT('Ctrl Pts',(0.359020467738701,1.93940985788448,9.96951765695316));
#34088=CARTESIAN_POINT('Ctrl Pts',(0.367453173764235,1.95826228569671,9.97055911457295));
#34089=CARTESIAN_POINT('Ctrl Pts',(0.374398224354034,1.9777834795981,9.97160057219274));
#34090=CARTESIAN_POINT('Ctrl Pts',(0.379766177687244,1.99771344035104,9.97264202981254));
#34091=CARTESIAN_POINT('Ctrl Pts',(0.385135771164221,2.01764949057586,9.97368380564304));
#34092=CARTESIAN_POINT('Ctrl Pts',(0.388927151832685,2.03799383702034,9.97472558147354));
#34093=CARTESIAN_POINT('Ctrl Pts',(0.391101723407775,2.05847492387162,9.97576735730404));
#34094=CARTESIAN_POINT('Ctrl Pts',(0.393280995368673,2.07900028105691,9.97681138495664));
#34095=CARTESIAN_POINT('Ctrl Pts',(0.393836461307713,2.0996622325233,9.97785541260923));
#34096=CARTESIAN_POINT('Ctrl Pts',(0.392781582556244,2.1201870850945,9.97889944026183));
#34097=CARTESIAN_POINT('Ctrl Pts',(0.392408485768947,2.12744645641409,9.97926869915769));
#34098=CARTESIAN_POINT('Ctrl Pts',(0.391834418487633,2.13468872683798,9.97963795805355));
#34099=CARTESIAN_POINT('Ctrl Pts',(0.391061515562374,2.14190204107271,9.98000721694941));
#34100=CARTESIAN_POINT('Ctrl Pts',(0.388876377186018,2.16229540386114,9.98105117959696));
#34101=CARTESIAN_POINT('Ctrl Pts',(0.385085201072507,2.18257814140808,9.98209514224452));
#34102=CARTESIAN_POINT('Ctrl Pts',(0.379714415309066,2.20247854803077,9.98313910489207));
#34103=CARTESIAN_POINT('Ctrl Pts',(0.374353509684772,2.22234234571108,9.98418114705784));
#34104=CARTESIAN_POINT('Ctrl Pts',(0.367418894565462,2.2418244907315,9.98522318922361));
#34105=CARTESIAN_POINT('Ctrl Pts',(0.358988179833785,2.26066230653027,9.98626523138937));
#34106=CARTESIAN_POINT('Ctrl Pts',(0.350566519557285,2.27947989081081,9.98730615441823));
#34107=CARTESIAN_POINT('Ctrl Pts',(0.340652222167683,2.29765383965664,9.98834707744708));
#34108=CARTESIAN_POINT('Ctrl Pts',(0.329371333033667,2.31494049170788,9.98938800047594));
#34109=CARTESIAN_POINT('Ctrl Pts',(0.318084650329008,2.33223602173306,9.99042945809573));
#34110=CARTESIAN_POINT('Ctrl Pts',(0.305430362355158,2.34864271960023,9.99147091571552));
#34111=CARTESIAN_POINT('Ctrl Pts',(0.29157866465248,2.36394463873979,9.99251237333531));
#34112=CARTESIAN_POINT('Ctrl Pts',(0.277722734652274,2.37925123328275,9.99355414916581));
#34113=CARTESIAN_POINT('Ctrl Pts',(0.262669186770547,2.39345185636053,9.99459592499631));
#34114=CARTESIAN_POINT('Ctrl Pts',(0.246625457130397,2.40636705745759,9.9956377008268));
#34115=CARTESIAN_POINT('Ctrl Pts',(0.230547048604549,2.4193101750549,9.9966817284794));
#34116=CARTESIAN_POINT('Ctrl Pts',(0.213474793621571,2.43096190842826,9.997725756132));
#34117=CARTESIAN_POINT('Ctrl Pts',(0.195646105166284,2.44118542104443,9.9987697837846));
#34118=CARTESIAN_POINT('Ctrl Pts',(0.189340331753627,2.44480134344953,9.99913904268047));
#34119=CARTESIAN_POINT('Ctrl Pts',(0.18294014812053,2.44823902924116,9.99950830157634));
#34120=CARTESIAN_POINT('Ctrl Pts',(0.176456678042913,2.45149385595492,9.99987756047221));
#34121=CARTESIAN_POINT('Ctrl Pts',(0.15812671859372,2.46069584824659,10.0009215231198));
#34122=CARTESIAN_POINT('Ctrl Pts',(0.139020397581867,2.46848757181165,10.0019654857673));
#34123=CARTESIAN_POINT('Ctrl Pts',(0.119380476011277,2.47474416866353,10.0030094484149));
#34124=CARTESIAN_POINT('Ctrl Pts',(0.0997766841927412,2.48098925583132,
10.0040514905806));
#34125=CARTESIAN_POINT('Ctrl Pts',(0.0796419153791249,2.48570454439856,
10.0050935327464));
#34126=CARTESIAN_POINT('Ctrl Pts',(0.0592390443584112,2.48881309857501,
10.0061355749122));
#34127=CARTESIAN_POINT('Ctrl Pts',(0.0388580857006548,2.49191831421311,
10.007176497941));
#34128=CARTESIAN_POINT('Ctrl Pts',(0.0182103158007307,2.49342008235121,
10.0082174209699));
#34129=CARTESIAN_POINT('Ctrl Pts',(-0.00243115987178641,2.49329248589527,
10.0092583439988));
#34130=CARTESIAN_POINT('Ctrl Pts',(-0.023083236468227,2.49316482390911,
10.0102998016186));
#34131=CARTESIAN_POINT('Ctrl Pts',(-0.0437282765154819,2.49140611401917,
10.0113412592383));
#34132=CARTESIAN_POINT('Ctrl Pts',(-0.0640925783502209,2.48804256390301,
10.0123827168581));
#34133=CARTESIAN_POINT('Ctrl Pts',(-0.0844631023669823,2.48467798607565,
10.0134244926886));
#34134=CARTESIAN_POINT('Ctrl Pts',(-0.104551997972933,2.47970774735316,
10.0144662685191));
#34135=CARTESIAN_POINT('Ctrl Pts',(-0.124096091040081,2.47320912393532,
10.0155080443496));
#34136=CARTESIAN_POINT('Ctrl Pts',(-0.143682429107908,2.4666964535955,10.0165520720022));
#34137=CARTESIAN_POINT('Ctrl Pts',(-0.162720935243703,2.45864908974604,
10.0175960996548));
#34138=CARTESIAN_POINT('Ctrl Pts',(-0.180968038901883,2.44919258138742,
10.0186401273074));
#34139=CARTESIAN_POINT('Ctrl Pts',(-0.187421800287246,2.44584793833455,
10.0190093862033));
#34140=CARTESIAN_POINT('Ctrl Pts',(-0.193776803094997,2.44232743077858,
10.0193786450991));
#34141=CARTESIAN_POINT('Ctrl Pts',(-0.200023139173413,2.43863790956597,
10.019747903995));
#34142=CARTESIAN_POINT('Ctrl Pts',(-0.217682677299445,2.42820695617139,
10.0207918666426));
#34143=CARTESIAN_POINT('Ctrl Pts',(-0.234576694771981,2.416359820131,10.0218358292901));
#34144=CARTESIAN_POINT('Ctrl Pts',(-0.250468797842574,2.40323303135921,
10.0228797919377));
#34145=CARTESIAN_POINT('Ctrl Pts',(-0.266331665677096,2.39013039072986,
10.0239218341034));
#34146=CARTESIAN_POINT('Ctrl Pts',(-0.281195678899764,2.37575318751205,
10.0249638762692));
#34147=CARTESIAN_POINT('Ctrl Pts',(-0.294853849648067,2.36028080480073,
10.026005918435));
#34148=CARTESIAN_POINT('Ctrl Pts',(-0.308497351735555,2.34482503918537,
10.0270468414638));
#34149=CARTESIAN_POINT('Ctrl Pts',(-0.320937076202657,2.32827695879629,
10.0280877644927));
#34150=CARTESIAN_POINT('Ctrl Pts',(-0.332003394567297,2.31085216621081,
10.0291286875215));
#34151=CARTESIAN_POINT('Ctrl Pts',(-0.343075396304625,2.293418424706,10.0301701451413));
#34152=CARTESIAN_POINT('Ctrl Pts',(-0.352772174750329,2.27510768395625,
10.0312116027611));
#34153=CARTESIAN_POINT('Ctrl Pts',(-0.3609676061331,2.25616426390996,10.0322530603809));
#34154=CARTESIAN_POINT('Ctrl Pts',(-0.369165541577451,2.23721505582297,
10.0332948362114));
#34155=CARTESIAN_POINT('Ctrl Pts',(-0.375860958045332,2.21763347269119,
10.0343366120419));
#34156=CARTESIAN_POINT('Ctrl Pts',(-0.380976369838367,2.19768262703664,
10.0353783878724));
#34157=CARTESIAN_POINT('Ctrl Pts',(-0.386102838710076,2.17768865717647,
10.036422415525));
#34158=CARTESIAN_POINT('Ctrl Pts',(-0.389642358477646,2.15732455688644,
10.0374664431776));
#34159=CARTESIAN_POINT('Ctrl Pts',(-0.391568643851175,2.13686308658471,
10.0385104708302));
#34160=CARTESIAN_POINT('Ctrl Pts',(-0.39224994573852,2.12962613274288,10.0388797297261));
#34161=CARTESIAN_POINT('Ctrl Pts',(-0.392729917800397,2.12237701824811,
10.0392489886219));
#34162=CARTESIAN_POINT('Ctrl Pts',(-0.393008956889611,2.11512778253875,
10.0396182475178));
#34163=CARTESIAN_POINT('Ctrl Pts',(-0.39320175440833,2.11011904107064,10.0398733809441));
#34164=CARTESIAN_POINT('Ctrl Pts',(-0.393298804877452,2.1051065904132,10.0401285143703));
#34165=CARTESIAN_POINT('Ctrl Pts',(-0.393299989030347,2.10009289095292,
10.0403836477965));
#34166=CARTESIAN_POINT('',(-0.393202477937398,2.10031103147611,10.1653836091462));
#34167=CARTESIAN_POINT('Ctrl Pts',(-0.393923156018864,2.10009103559663,
10.040383749539));
#34168=CARTESIAN_POINT('Ctrl Pts',(-0.39352309280741,1.97474775194909,10.0467520300395));
#34169=CARTESIAN_POINT('Ctrl Pts',(-0.260911319827819,1.7183126572773,10.059743758381));
#34170=CARTESIAN_POINT('Ctrl Pts',(0.176083159449116,1.66957025957435,10.0793589345633));
#34171=CARTESIAN_POINT('Ctrl Pts',(0.457230028159891,2.01505447726103,10.0992292780861));
#34172=CARTESIAN_POINT('Ctrl Pts',(0.318930592281517,2.43846464777199,10.1190996216089));
#34173=CARTESIAN_POINT('Ctrl Pts',(-0.11194424353566,2.55137958175324,10.1389699651317));
#34174=CARTESIAN_POINT('Ctrl Pts',(-0.366754511395233,2.3175460488061,10.1543979270584));
#34175=CARTESIAN_POINT('Ctrl Pts',(-0.393263485699074,2.14351739557072,
10.1632024411441));
#34176=CARTESIAN_POINT('Ctrl Pts',(-0.392946047468718,2.10031284482443,
10.1653835073888));
#34177=CARTESIAN_POINT('',(-0.393130899880172,2.09975969803041,10.2903836983485));
#34178=CARTESIAN_POINT('Ctrl Pts',(-0.393299877558333,2.10031034271459,
10.1653836477965));
#34179=CARTESIAN_POINT('Ctrl Pts',(-0.393316137078467,2.07970451896758,
10.1664229484123));
#34180=CARTESIAN_POINT('Ctrl Pts',(-0.391708693976257,2.05907847120989,
10.1674622490281));
#34181=CARTESIAN_POINT('Ctrl Pts',(-0.388494396308227,2.03870567695858,
10.168501549644));
#34182=CARTESIAN_POINT('Ctrl Pts',(-0.385277877255557,2.0183188031736,10.1695415685151));
#34183=CARTESIAN_POINT('Ctrl Pts',(-0.380452391197413,1.99818626229835,
10.1705815873863));
#34184=CARTESIAN_POINT('Ctrl Pts',(-0.374086359525959,1.97857395000818,
10.1716216062574));
#34185=CARTESIAN_POINT('Ctrl Pts',(-0.367717552787176,1.9589530883595,10.1726620784914));
#34186=CARTESIAN_POINT('Ctrl Pts',(-0.359807131823567,1.93985359354466,
10.1737025507254));
#34187=CARTESIAN_POINT('Ctrl Pts',(-0.350472277064807,1.9215229062064,10.1747430229595));
#34188=CARTESIAN_POINT('Ctrl Pts',(-0.341116449486835,1.90315103491815,
10.1757858328449));
#34189=CARTESIAN_POINT('Ctrl Pts',(-0.330330191756566,1.88555204354073,
10.1768286427302));
#34190=CARTESIAN_POINT('Ctrl Pts',(-0.31827520167265,1.86894635687738,10.1778714526156));
#34191=CARTESIAN_POINT('Ctrl Pts',(-0.315041457108724,1.86449189041959,
10.1781511858029));
#34192=CARTESIAN_POINT('Ctrl Pts',(-0.311716639803177,1.86010871273235,
10.1784309189901));
#34193=CARTESIAN_POINT('Ctrl Pts',(-0.308304338982045,1.85580064585498,
10.1787106521773));
#34194=CARTESIAN_POINT('Ctrl Pts',(-0.295569651922344,1.83972296501987,
10.1797546148249));
#34195=CARTESIAN_POINT('Ctrl Pts',(-0.281535989030201,1.82459620844249,
10.1807985774724));
#34196=CARTESIAN_POINT('Ctrl Pts',(-0.266370747194188,1.81063601634065,
10.18184254012));
#34197=CARTESIAN_POINT('Ctrl Pts',(-0.251233403454677,1.79670150551647,
10.1828845822857));
#34198=CARTESIAN_POINT('Ctrl Pts',(-0.234969107732109,1.78392983584885,
10.1839266244515));
#34199=CARTESIAN_POINT('Ctrl Pts',(-0.217783715017697,1.77250168935842,
10.1849686666173));
#34200=CARTESIAN_POINT('Ctrl Pts',(-0.200616779145092,1.76108581651778,
10.1860095896461));
#34201=CARTESIAN_POINT('Ctrl Pts',(-0.182531303722437,1.75101103175003,
10.187050512675));
#34202=CARTESIAN_POINT('Ctrl Pts',(-0.163763948559705,1.74241608096541,
10.1880914357038));
#34203=CARTESIAN_POINT('Ctrl Pts',(-0.144986954972491,1.73381671603809,
10.1891328933236));
#34204=CARTESIAN_POINT('Ctrl Pts',(-0.125528044281525,1.72669902443544,
10.1901743509434));
#34205=CARTESIAN_POINT('Ctrl Pts',(-0.105646413272996,1.7211547474726,10.1912158085632));
#34206=CARTESIAN_POINT('Ctrl Pts',(-0.0857587075594246,1.71560877649144,
10.1922575843937));
#34207=CARTESIAN_POINT('Ctrl Pts',(-0.0654487422604584,1.71163733982698,
10.1932993602242));
#34208=CARTESIAN_POINT('Ctrl Pts',(-0.0449877206602062,1.70928143761807,
10.1943411360547));
#34209=CARTESIAN_POINT('Ctrl Pts',(-0.0244824720974497,1.70692044307309,
10.1953851637073));
#34210=CARTESIAN_POINT('Ctrl Pts',(-0.00382625137647264,1.70618198093199,
10.1964291913599));
#34211=CARTESIAN_POINT('Ctrl Pts',(0.0167071398267035,1.70705501469186,
10.1974732190125));
#34212=CARTESIAN_POINT('Ctrl Pts',(0.023969531148709,1.70736379528922,10.1978424779084));
#34213=CARTESIAN_POINT('Ctrl Pts',(0.031216602388322,1.70787368997157,10.1982117368043));
#34214=CARTESIAN_POINT('Ctrl Pts',(0.0384364798072488,1.70858266898357,
10.1985809957001));
#34215=CARTESIAN_POINT('Ctrl Pts',(0.0588483979210042,1.71058708272879,
10.1996249583477));
#34216=CARTESIAN_POINT('Ctrl Pts',(0.0791639209822469,1.71419845109411,
10.2006689209952));
#34217=CARTESIAN_POINT('Ctrl Pts',(0.0991111198744934,1.71939275372476,
10.2017128836428));
#34218=CARTESIAN_POINT('Ctrl Pts',(0.119021623744943,1.72457750087599,10.2027549258086));
#34219=CARTESIAN_POINT('Ctrl Pts',(0.138564429422154,1.73133927636122,10.2037969679743));
#34220=CARTESIAN_POINT('Ctrl Pts',(0.157476183201892,1.73960280006059,10.2048390101401));
#34221=CARTESIAN_POINT('Ctrl Pts',(0.176367626055164,1.74785744886533,10.205879933169));
#34222=CARTESIAN_POINT('Ctrl Pts',(0.194628680100807,1.75761037737541,10.2069208561978));
#34223=CARTESIAN_POINT('Ctrl Pts',(0.212014577061992,1.76873770345356,10.2079617792267));
#34224=CARTESIAN_POINT('Ctrl Pts',(0.229409402966725,1.77987074423637,10.2090032368465));
#34225=CARTESIAN_POINT('Ctrl Pts',(0.24592754546134,1.7923792096721,10.2100446944662));
#34226=CARTESIAN_POINT('Ctrl Pts',(0.261351558901751,1.80609482369372,10.211086152086));
#34227=CARTESIAN_POINT('Ctrl Pts',(0.276780285050694,1.81981462843337,10.2121279279165));
#34228=CARTESIAN_POINT('Ctrl Pts',(0.29111369129841,1.83474180046838,10.213169703747));
#34229=CARTESIAN_POINT('Ctrl Pts',(0.304170496756044,1.85067050133773,10.2142114795775));
#34230=CARTESIAN_POINT('Ctrl Pts',(0.317255524794978,1.86663363245548,10.2152555072301));
#34231=CARTESIAN_POINT('Ctrl Pts',(0.329058022495414,1.88360200977445,10.2162995348827));
#34232=CARTESIAN_POINT('Ctrl Pts',(0.339439055752096,1.90133944168475,10.2173435625353));
#34233=CARTESIAN_POINT('Ctrl Pts',(0.343110691142987,1.90761293885359,10.2177128214312));
#34234=CARTESIAN_POINT('Ctrl Pts',(0.346604933172984,1.91398242131096,10.218082080327));
#34235=CARTESIAN_POINT('Ctrl Pts',(0.349917061027627,1.92043680666187,10.2184513392229));
#34236=CARTESIAN_POINT('Ctrl Pts',(0.359281054157792,1.93868453825249,10.2194953018705));
#34237=CARTESIAN_POINT('Ctrl Pts',(0.367241710688164,1.95772109272876,10.220539264518));
#34238=CARTESIAN_POINT('Ctrl Pts',(0.373672027218917,1.97730482456875,10.2215832271656));
#34239=CARTESIAN_POINT('Ctrl Pts',(0.380090514489504,1.99685253002375,10.2226252693313));
#34240=CARTESIAN_POINT('Ctrl Pts',(0.384983966425265,2.01694474218674,10.2236673114971));
#34241=CARTESIAN_POINT('Ctrl Pts',(0.388273121780206,2.03731927805893,10.2247093536629));
#34242=CARTESIAN_POINT('Ctrl Pts',(0.391558744633968,2.05767193199968,10.2257502766917));
#34243=CARTESIAN_POINT('Ctrl Pts',(0.393243346233729,2.07830558962094,10.2267911997206));
#34244=CARTESIAN_POINT('Ctrl Pts',(0.393298591407606,2.09894738573383,10.2278321227494));
#34245=CARTESIAN_POINT('Ctrl Pts',(0.393353864953964,2.1195997829352,10.2288735803692));
#34246=CARTESIAN_POINT('Ctrl Pts',(0.391778092255447,2.14025959124585,10.229915037989));
#34247=CARTESIAN_POINT('Ctrl Pts',(0.388595055585969,2.16065288759934,10.2309564956088));
#34248=CARTESIAN_POINT('Ctrl Pts',(0.385411046360019,2.18105241499393,10.2319982714393));
#34249=CARTESIAN_POINT('Ctrl Pts',(0.380618944641255,2.20118454753727,10.2330400472698));
#34250=CARTESIAN_POINT('Ctrl Pts',(0.374293692472436,2.22078543693405,10.2340818231002));
#34251=CARTESIAN_POINT('Ctrl Pts',(0.367954768127517,2.24042869409806,10.2351258507528));
#34252=CARTESIAN_POINT('Ctrl Pts',(0.360076357932214,2.25953773472292,10.2361698784054));
#34253=CARTESIAN_POINT('Ctrl Pts',(0.35078184847944,2.27786788573924,10.237213906058));
#34254=CARTESIAN_POINT('Ctrl Pts',(0.347494502316144,2.28435101988659,10.2375831649539));
#34255=CARTESIAN_POINT('Ctrl Pts',(0.344030423772152,2.29073695709101,10.2379524238498));
#34256=CARTESIAN_POINT('Ctrl Pts',(0.340396375661423,2.29701572890652,10.2383216827456));
#34257=CARTESIAN_POINT('Ctrl Pts',(0.330122254903612,2.31476696881248,10.2393656453932));
#34258=CARTESIAN_POINT('Ctrl Pts',(0.318425226282013,2.33176526226058,10.2404096080407));
#34259=CARTESIAN_POINT('Ctrl Pts',(0.305439720442846,2.34777301543105,10.2414535706883));
#34260=CARTESIAN_POINT('Ctrl Pts',(0.292478102840944,2.36375132061463,10.2424956128541));
#34261=CARTESIAN_POINT('Ctrl Pts',(0.27823312506752,2.37874210010351,10.2435376550198));
#34262=CARTESIAN_POINT('Ctrl Pts',(0.262882329737576,2.39253678522836,10.2445796971856));
#34263=CARTESIAN_POINT('Ctrl Pts',(0.247548020920653,2.4063166550781,10.2456206202144));
#34264=CARTESIAN_POINT('Ctrl Pts',(0.231110777444544,2.41890246996186,10.2466615432433));
#34265=CARTESIAN_POINT('Ctrl Pts',(0.213784690905028,2.43012269830268,10.2477024662722));
#34266=CARTESIAN_POINT('Ctrl Pts',(0.196449706139038,2.44134868906034,10.248743923892));
#34267=CARTESIAN_POINT('Ctrl Pts',(0.178225575176194,2.4512072786998,10.2497853815117));
#34268=CARTESIAN_POINT('Ctrl Pts',(0.159355491209759,2.45957018427742,10.2508268391315));
#34269=CARTESIAN_POINT('Ctrl Pts',(0.140479641609996,2.46793564508729,10.251868614962));
#34270=CARTESIAN_POINT('Ctrl Pts',(0.120958132865967,2.47480424727279,10.2529103907925));
#34271=CARTESIAN_POINT('Ctrl Pts',(0.101053380830248,2.48009617759559,10.253952166623));
#34272=CARTESIAN_POINT('Ctrl Pts',(0.08110560422132,2.48539954654586,10.2549961942756));
#34273=CARTESIAN_POINT('Ctrl Pts',(0.0607736549357756,2.48911930716426,
10.2560402219282));
#34274=CARTESIAN_POINT('Ctrl Pts',(0.0403300498632668,2.49122675915385,
10.2570842495808));
#34275=CARTESIAN_POINT('Ctrl Pts',(0.0330994147188781,2.49197213729861,
10.2574535084767));
#34276=CARTESIAN_POINT('Ctrl Pts',(0.0258548360733349,2.49251630123194,
10.2578227673726));
#34277=CARTESIAN_POINT('Ctrl Pts',(0.0186083564078811,2.49285954114899,
10.2581920262684));
#34278=CARTESIAN_POINT('Ctrl Pts',(-0.00187877113783579,2.49382994336967,
10.259235988916));
#34279=CARTESIAN_POINT('Ctrl Pts',(-0.0225030535577246,2.49319635565967,
10.2602799515635));
#34280=CARTESIAN_POINT('Ctrl Pts',(-0.0429919479763473,2.49094319588554,
10.2613239142111));
#34281=CARTESIAN_POINT('Ctrl Pts',(-0.0634431508658882,2.48869418104161,
10.2623659563769));
#34282=CARTESIAN_POINT('Ctrl Pts',(-0.0837587305199895,2.48483152848569,
10.2634079985426));
#34283=CARTESIAN_POINT('Ctrl Pts',(-0.103667211641671,2.47939161723797,
10.2644500407084));
#34284=CARTESIAN_POINT('Ctrl Pts',(-0.123554311367365,2.47395754836947,
10.2654909637373));
#34285=CARTESIAN_POINT('Ctrl Pts',(-0.143034466758624,2.46694974876387,
10.2665318867661));
#34286=CARTESIAN_POINT('Ctrl Pts',(-0.161847559345197,2.45845537732611,
10.267572809795));
#34287=CARTESIAN_POINT('Ctrl Pts',(-0.180670313845794,2.44995664340056,
10.2686142674148));
#34288=CARTESIAN_POINT('Ctrl Pts',(-0.198824643905938,2.43997010050044,
10.2696557250345));
#34289=CARTESIAN_POINT('Ctrl Pts',(-0.21607104206007,2.42863078794154,10.2706971826543));
#34290=CARTESIAN_POINT('Ctrl Pts',(-0.233322709740733,2.41728801072829,
10.2717389584848));
#34291=CARTESIAN_POINT('Ctrl Pts',(-0.249665298850806,2.40459207512652,
10.2727807343153));
#34292=CARTESIAN_POINT('Ctrl Pts',(-0.26488965054794,2.39072042073544,10.2738225101458));
#34293=CARTESIAN_POINT('Ctrl Pts',(-0.280146910026749,2.3768187824486,10.2748665377984));
#34294=CARTESIAN_POINT('Ctrl Pts',(-0.294280602877999,2.36173688909286,
10.275910565451));
#34295=CARTESIAN_POINT('Ctrl Pts',(-0.307119079061731,2.34568834175897,
10.2769545931036));
#34296=CARTESIAN_POINT('Ctrl Pts',(-0.311659879804395,2.34001218092731,
10.2773238519995));
#34297=CARTESIAN_POINT('Ctrl Pts',(-0.316039043904594,2.33421537526186,
10.2776931108954));
#34298=CARTESIAN_POINT('Ctrl Pts',(-0.320250296550904,2.32830820738436,
10.2780623697912));
#34299=CARTESIAN_POINT('Ctrl Pts',(-0.332267798420901,2.31145113254785,
10.2791161107668));
#34300=CARTESIAN_POINT('Ctrl Pts',(-0.34298584099648,2.29359358210619,10.2801698517423));
#34301=CARTESIAN_POINT('Ctrl Pts',(-0.352241230061416,2.27496001213083,
10.2812235927178));
#34302=CARTESIAN_POINT('Ctrl Pts',(-0.361477954782044,2.25636401846515,
10.2822752087276));
#34303=CARTESIAN_POINT('Ctrl Pts',(-0.369257510879528,2.2369957190811,10.2833268247374));
#34304=CARTESIAN_POINT('Ctrl Pts',(-0.37546086600497,2.21710690884315,10.2843784407472));
#34305=CARTESIAN_POINT('Ctrl Pts',(-0.381658138137299,2.19723760151826,
10.2854290255452));
#34306=CARTESIAN_POINT('Ctrl Pts',(-0.386282022236364,2.17684946460557,
10.2864796103432));
#34307=CARTESIAN_POINT('Ctrl Pts',(-0.389262129579668,2.15621284973297,
10.2875301951412));
#34308=CARTESIAN_POINT('Ctrl Pts',(-0.391960180934149,2.13752941309972,
10.2884813460263));
#34309=CARTESIAN_POINT('Ctrl Pts',(-0.393311420851984,2.11864292265643,
10.2894324969114));
#34310=CARTESIAN_POINT('Ctrl Pts',(-0.393299927137564,2.09976059743748,
10.2903836477965));
#34311=CARTESIAN_POINT('',(-0.393480327863744,2.09979784797213,10.4153835873822));
#34312=CARTESIAN_POINT('Ctrl Pts',(-0.392802840044818,2.09975795239874,
10.2903837964633));
#34313=CARTESIAN_POINT('Ctrl Pts',(-0.393078666905956,2.04986700265937,
10.2929001020802));
#34314=CARTESIAN_POINT('Ctrl Pts',(-0.36107951247964,1.86899388280721,10.302039855538));
#34315=CARTESIAN_POINT('Ctrl Pts',(-0.0889922105537249,1.64354033371482,
10.3178030568369));
#34316=CARTESIAN_POINT('Ctrl Pts',(0.335626368481811,1.77808389095263,10.3376734003596));
#34317=CARTESIAN_POINT('Ctrl Pts',(0.452353445839552,2.20794165332066,10.3575437438824));
#34318=CARTESIAN_POINT('Ctrl Pts',(0.154107819000222,2.53877764369605,10.3774140874052));
#34319=CARTESIAN_POINT('Ctrl Pts',(-0.272447788613133,2.46922488414649,
10.3966939973457));
#34320=CARTESIAN_POINT('Ctrl Pts',(-0.393070870679608,2.21862714459167,
10.4093504594452));
#34321=CARTESIAN_POINT('Ctrl Pts',(-0.393819740132955,2.09979991159289,
10.4153834737038));
#34322=CARTESIAN_POINT('',(-0.393299843557239,2.10035079602495,10.5403836477997));
#34323=CARTESIAN_POINT('Ctrl Pts',(-0.393299947482771,2.09979675126253,
10.4153836477965));
#34324=CARTESIAN_POINT('Ctrl Pts',(-0.39329394627344,2.08818400845285,10.4159740233479));
#34325=CARTESIAN_POINT('Ctrl Pts',(-0.392773668395661,2.07658491143399,
10.4165643988994));
#34326=CARTESIAN_POINT('Ctrl Pts',(-0.391742435504716,2.06503209721997,
10.4171547744508));
#34327=CARTESIAN_POINT('Ctrl Pts',(-0.389918903658791,2.04460322531887,
10.4181987370984));
#34328=CARTESIAN_POINT('Ctrl Pts',(-0.386487626392958,2.02425651071807,
10.4192426997459));
#34329=CARTESIAN_POINT('Ctrl Pts',(-0.381470214444904,2.00426408463195,
10.4202866623935));
#34330=CARTESIAN_POINT('Ctrl Pts',(-0.376462032566783,1.98430843676791,
10.4213287045592));
#34331=CARTESIAN_POINT('Ctrl Pts',(-0.369873627250801,1.96470650378052,
10.422370746725));
#34332=CARTESIAN_POINT('Ctrl Pts',(-0.361777942947447,1.9457222958535,10.4234127888907));
#34333=CARTESIAN_POINT('Ctrl Pts',(-0.353690953281854,1.92675847666757,
10.4244537119196));
#34334=CARTESIAN_POINT('Ctrl Pts',(-0.344100158875096,1.9084117502013,10.4254946349484));
#34335=CARTESIAN_POINT('Ctrl Pts',(-0.333127268913106,1.89092797244372,
10.4265355579773));
#34336=CARTESIAN_POINT('Ctrl Pts',(-0.322148743560819,1.87343521547356,
10.4275770155971));
#34337=CARTESIAN_POINT('Ctrl Pts',(-0.309787082088958,1.85680692438022,
10.4286184732169));
#34338=CARTESIAN_POINT('Ctrl Pts',(-0.296208627888156,1.84126202682131,
10.4296599308367));
#34339=CARTESIAN_POINT('Ctrl Pts',(-0.282626024877622,1.8257123796185,10.4307017066671));
#34340=CARTESIAN_POINT('Ctrl Pts',(-0.267826399889048,1.81124731481315,
10.4317434824976));
#34341=CARTESIAN_POINT('Ctrl Pts',(-0.252013977571094,1.79804992944396,
10.4327852583281));
#34342=CARTESIAN_POINT('Ctrl Pts',(-0.236167376343474,1.78482401762682,
10.4338292859807));
#34343=CARTESIAN_POINT('Ctrl Pts',(-0.219304208043086,1.77287168163419,
10.4348733136333));
#34344=CARTESIAN_POINT('Ctrl Pts',(-0.201659424373089,1.76233394224247,
10.4359173412859));
#34345=CARTESIAN_POINT('Ctrl Pts',(-0.195418695672471,1.7586068819457,10.4362866001818));
#34346=CARTESIAN_POINT('Ctrl Pts',(-0.189080414146325,1.7550563578388,10.4366558590777));
#34347=CARTESIAN_POINT('Ctrl Pts',(-0.182655619939169,1.75168718871589,
10.4370251179735));
#34348=CARTESIAN_POINT('Ctrl Pts',(-0.164491547941026,1.7421619294548,10.4380690806211));
#34349=CARTESIAN_POINT('Ctrl Pts',(-0.14552625362603,1.7340329645596,10.4391130432686));
#34350=CARTESIAN_POINT('Ctrl Pts',(-0.12600024807438,1.72742943287856,10.4401570059162));
#34351=CARTESIAN_POINT('Ctrl Pts',(-0.106510162713992,1.72083804910561,
10.441199048082));
#34352=CARTESIAN_POINT('Ctrl Pts',(-0.0864620836551864,1.7157668177461,
10.4422410902477));
#34353=CARTESIAN_POINT('Ctrl Pts',(-0.0661174815364688,1.71229731928284,
10.4432831324135));
#34354=CARTESIAN_POINT('Ctrl Pts',(-0.0457947292008156,1.70883154700642,
10.4443240554423));
#34355=CARTESIAN_POINT('Ctrl Pts',(-0.0251768027941027,1.70696424412038,
10.4453649784712));
#34356=CARTESIAN_POINT('Ctrl Pts',(-0.00453630581528488,1.70672616165126,
10.4464059015001));
#34357=CARTESIAN_POINT('Ctrl Pts',(0.0161147915848249,1.70648795690919,
10.4474473591199));
#34358=CARTESIAN_POINT('Ctrl Pts',(0.0367877471711825,1.70788066877968,
10.4484888167396));
#34359=CARTESIAN_POINT('Ctrl Pts',(0.0572084379665225,1.71088294225846,
10.4495302743594));
#34360=CARTESIAN_POINT('Ctrl Pts',(0.0776353681731634,1.71388613306268,
10.4505720501899));
#34361=CARTESIAN_POINT('Ctrl Pts',(0.097809158068138,1.71849972178497,10.4516138260204));
#34362=CARTESIAN_POINT('Ctrl Pts',(0.117465305890651,1.72465110641962,10.4526556018509));
#34363=CARTESIAN_POINT('Ctrl Pts',(0.13716394092274,1.73081578741175,10.4536996295035));
#34364=CARTESIAN_POINT('Ctrl Pts',(0.156342016723673,1.73852462580554,10.4547436571561));
#34365=CARTESIAN_POINT('Ctrl Pts',(0.174753776897547,1.74765640709665,10.4557876848087));
#34366=CARTESIAN_POINT('Ctrl Pts',(0.181265775134261,1.75088619844219,10.4561569437046));
#34367=CARTESIAN_POINT('Ctrl Pts',(0.187682145688885,1.75429357617944,10.4565262026005));
#34368=CARTESIAN_POINT('Ctrl Pts',(0.193992860603331,1.75787186605756,10.4568954614963));
#34369=CARTESIAN_POINT('Ctrl Pts',(0.211834409510512,1.76798834806158,10.4579394241439));
#34370=CARTESIAN_POINT('Ctrl Pts',(0.228935645232347,1.7795343515047,10.4589833867914));
#34371=CARTESIAN_POINT('Ctrl Pts',(0.245057792519578,1.79237755555644,10.460027349439));
#34372=CARTESIAN_POINT('Ctrl Pts',(0.261150281379612,1.80519713315039,10.4610693916048));
#34373=CARTESIAN_POINT('Ctrl Pts',(0.276266650944304,1.81930876780531,10.4621114337705));
#34374=CARTESIAN_POINT('Ctrl Pts',(0.290196768101947,1.83453677131628,10.4631534759363));
#34375=CARTESIAN_POINT('Ctrl Pts',(0.304111924532597,1.8497484201907,10.4641943989652));
#34376=CARTESIAN_POINT('Ctrl Pts',(0.316842842338324,1.86607353707251,10.465235321994));
#34377=CARTESIAN_POINT('Ctrl Pts',(0.328216100305829,1.88329955814527,10.4662762450229));
#34378=CARTESIAN_POINT('Ctrl Pts',(0.339595199282202,1.90053442605349,10.4673177026427));
#34379=CARTESIAN_POINT('Ctrl Pts',(0.34961482660134,1.91867051734725,10.4683591602625));
#34380=CARTESIAN_POINT('Ctrl Pts',(0.358144550212507,1.93746578466956,10.4694006178822));
#34381=CARTESIAN_POINT('Ctrl Pts',(0.366676880026103,1.95626679476545,10.4704423937127));
#34382=CARTESIAN_POINT('Ctrl Pts',(0.37371812901234,1.97572669744607,10.4714841695432));
#34383=CARTESIAN_POINT('Ctrl Pts',(0.379186162655151,1.99558379411767,10.4725259453737));
#34384=CARTESIAN_POINT('Ctrl Pts',(0.384666015576766,2.01548381235434,10.4735699730263));
#34385=CARTESIAN_POINT('Ctrl Pts',(0.388565725190146,2.03578201537182,10.4746140006789));
#34386=CARTESIAN_POINT('Ctrl Pts',(0.390854178443174,2.05620615119093,10.4756580283315));
#34387=CARTESIAN_POINT('Ctrl Pts',(0.39166357436229,2.06342990031563,10.4760272872274));
#34388=CARTESIAN_POINT('Ctrl Pts',(0.392271887471484,2.07066937469568,10.4763965461233));
#34389=CARTESIAN_POINT('Ctrl Pts',(0.392679301285457,2.07791252975181,10.4767658050191));
#34390=CARTESIAN_POINT('Ctrl Pts',(0.393831134886887,2.09839025801692,10.4778097676667));
#34391=CARTESIAN_POINT('Ctrl Pts',(0.393380256363785,2.11901934348574,10.4788537303142));
#34392=CARTESIAN_POINT('Ctrl Pts',(0.391308670082716,2.13952739199715,10.4798976929618));
#34393=CARTESIAN_POINT('Ctrl Pts',(0.389240894707837,2.15999771374345,10.4809397351276));
#34394=CARTESIAN_POINT('Ctrl Pts',(0.385558343610689,2.18034671074249,10.4819817772933));
#34395=CARTESIAN_POINT('Ctrl Pts',(0.380294989729315,2.20030259611187,10.4830238194591));
#34396=CARTESIAN_POINT('Ctrl Pts',(0.375037288607326,2.22023704917385,10.484064742488));
#34397=CARTESIAN_POINT('Ctrl Pts',(0.368202313883265,2.23977851354841,10.4851056655168));
#34398=CARTESIAN_POINT('Ctrl Pts',(0.359874916983526,2.25866610893981,10.4861465885457));
#34399=CARTESIAN_POINT('Ctrl Pts',(0.351543243349778,2.27756340450793,10.4871880461655));
#34400=CARTESIAN_POINT('Ctrl Pts',(0.341717898385468,2.2958054804688,10.4882295037853));
#34401=CARTESIAN_POINT('Ctrl Pts',(0.330531794616224,2.31315164261103,10.489270961405));
#34402=CARTESIAN_POINT('Ctrl Pts',(0.319342273004604,2.33050310476201,10.4903127372355));
#34403=CARTESIAN_POINT('Ctrl Pts',(0.306791593716707,2.34695750991802,10.491354513066));
#34404=CARTESIAN_POINT('Ctrl Pts',(0.293055336718086,2.36230413572998,10.4923962888965));
#34405=CARTESIAN_POINT('Ctrl Pts',(0.27928938848825,2.37768393362188,10.4934403165491));
#34406=CARTESIAN_POINT('Ctrl Pts',(0.264333279241318,2.39195066334533,10.4944843442017));
#34407=CARTESIAN_POINT('Ctrl Pts',(0.248399081258619,2.40493078957343,10.4955283718543));
#34408=CARTESIAN_POINT('Ctrl Pts',(0.2427633642937,2.40952169007999,10.4958976307502));
#34409=CARTESIAN_POINT('Ctrl Pts',(0.237005575494178,2.41395202892457,10.4962668896461));
#34410=CARTESIAN_POINT('Ctrl Pts',(0.231135941497791,2.41821544046122,10.4966361485419));
#34411=CARTESIAN_POINT('Ctrl Pts',(0.214541409272148,2.43026888709514,10.4976801111895));
#34412=CARTESIAN_POINT('Ctrl Pts',(0.196952036167494,2.44105667706841,10.498724073837));
#34413=CARTESIAN_POINT('Ctrl Pts',(0.178587114710008,2.45041622744895,10.4997680364846));
#34414=CARTESIAN_POINT('Ctrl Pts',(0.160255977504472,2.45975855992802,10.5008100786504));
#34415=CARTESIAN_POINT('Ctrl Pts',(0.141152745043059,2.46767748479036,10.5018521208161));
#34416=CARTESIAN_POINT('Ctrl Pts',(0.121524330767905,2.4740544439402,10.5028941629819));
#34417=CARTESIAN_POINT('Ctrl Pts',(0.101916997101322,2.4804245543361,10.5039350860108));
#34418=CARTESIAN_POINT('Ctrl Pts',(0.0817862886590113,2.48525573296991,
10.5049760090396));
#34419=CARTESIAN_POINT('Ctrl Pts',(0.0613974898748184,2.48847810522225,
10.5060169320685));
#34420=CARTESIAN_POINT('Ctrl Pts',(0.0409982199349738,2.491702132401,10.5070583896883));
#34421=CARTESIAN_POINT('Ctrl Pts',(0.0203413190920445,2.49331557176928,
10.5080998473081));
#34422=CARTESIAN_POINT('Ctrl Pts',(-0.000298884699839051,2.49329988643265,
10.5091413049278));
#34423=CARTESIAN_POINT('Ctrl Pts',(-0.0209453949738137,2.49328419630347,
10.5101830807583));
#34424=CARTESIAN_POINT('Ctrl Pts',(-0.0415744629098813,2.49163842726921,
10.5112248565888));
#34425=CARTESIAN_POINT('Ctrl Pts',(-0.0619138647762143,2.4883961422935,
10.5122666324193));
#34426=CARTESIAN_POINT('Ctrl Pts',(-0.0822972307212442,2.48514684904524,
10.5133106600719));
#34427=CARTESIAN_POINT('Ctrl Pts',(-0.102388964684835,2.48029432319326,
10.5143546877245));
#34428=CARTESIAN_POINT('Ctrl Pts',(-0.121928356499301,2.47392294110068,
10.5153987153771));
#34429=CARTESIAN_POINT('Ctrl Pts',(-0.128839183266563,2.47166946676903,
10.515767974273));
#34430=CARTESIAN_POINT('Ctrl Pts',(-0.13568108660344,2.46922643732443,10.5161372331689));
#34431=CARTESIAN_POINT('Ctrl Pts',(-0.142443178297055,2.46659900566782,
10.5165064920647));
#34432=CARTESIAN_POINT('Ctrl Pts',(-0.161560852174292,2.45917077431253,
10.5175504547123));
#34433=CARTESIAN_POINT('Ctrl Pts',(-0.180152864613886,2.45022094011477,
10.5185944173598));
#34434=CARTESIAN_POINT('Ctrl Pts',(-0.197963805968831,2.43984587907805,
10.5196383800074));
#34435=CARTESIAN_POINT('Ctrl Pts',(-0.21574198217792,2.42948990408409,10.5206804221732));
#34436=CARTESIAN_POINT('Ctrl Pts',(-0.232741280890506,2.41771422131281,
10.5217224643389));
#34437=CARTESIAN_POINT('Ctrl Pts',(-0.24872835762929,2.40466226236775,10.5227645065047));
#34438=CARTESIAN_POINT('Ctrl Pts',(-0.264698264498812,2.39162432102156,
10.5238054295336));
#34439=CARTESIAN_POINT('Ctrl Pts',(-0.279657522212033,2.37731326522368,
10.5248463525624));
#34440=CARTESIAN_POINT('Ctrl Pts',(-0.293403775680491,2.36191432648183,
10.5258872755913));
#34441=CARTESIAN_POINT('Ctrl Pts',(-0.307157088866454,2.3465074792464,10.5269287332111));
#34442=CARTESIAN_POINT('Ctrl Pts',(-0.319695651247729,2.33001217105164,
10.5279701908308));
#34443=CARTESIAN_POINT('Ctrl Pts',(-0.330855377993217,2.31264902739718,
10.5290116484506));
#34444=CARTESIAN_POINT('Ctrl Pts',(-0.342018514521751,2.29528057854535,
10.5300534242811));
#34445=CARTESIAN_POINT('Ctrl Pts',(-0.351801609668667,2.27704440435856,
10.5310952001116));
#34446=CARTESIAN_POINT('Ctrl Pts',(-0.360085524149898,2.25818756366318,
10.5321369759421));
#34447=CARTESIAN_POINT('Ctrl Pts',(-0.368387344500269,2.23928996347872,
10.5331810035947));
#34448=CARTESIAN_POINT('Ctrl Pts',(-0.375183272511529,2.21976971390877,
10.5342250312473));
#34449=CARTESIAN_POINT('Ctrl Pts',(-0.380403126216002,2.19989169918012,
10.5352690588999));
#34450=CARTESIAN_POINT('Ctrl Pts',(-0.382249320050743,2.19286110592663,
10.5356383177958));
#34451=CARTESIAN_POINT('Ctrl Pts',(-0.383898823054406,2.18578585511974,
10.5360075766917));
#34452=CARTESIAN_POINT('Ctrl Pts',(-0.385350073891993,2.17867789112219,
10.5363768355876));
#34453=CARTESIAN_POINT('Ctrl Pts',(-0.390599227118804,2.15296848845556,
10.5377124396572));
#34454=CARTESIAN_POINT('Ctrl Pts',(-0.393276326782456,2.1267169504976,10.5390480437269));
#34455=CARTESIAN_POINT('Ctrl Pts',(-0.393299843557183,2.10035079608795,
10.5403836477965));
#34456=CARTESIAN_POINT('',(-0.393299999656376,2.1000164406377,10.6653836477933));
#34457=CARTESIAN_POINT('Ctrl Pts',(-0.393299843557239,2.10035079602495,
10.5403836477997));
#34458=CARTESIAN_POINT('Ctrl Pts',(-0.393317932042654,2.08007063895956,
10.5414109595528));
#34459=CARTESIAN_POINT('Ctrl Pts',(-0.391763135488696,2.05973973232589,
10.542438271306));
#34460=CARTESIAN_POINT('Ctrl Pts',(-0.388638377742624,2.03962532529627,
10.5434655830591));
#34461=CARTESIAN_POINT('Ctrl Pts',(-0.38539857970124,2.01877039131615,10.5445307160634));
#34462=CARTESIAN_POINT('Ctrl Pts',(-0.38047079879135,1.99814908177945,10.5455958490676));
#34463=CARTESIAN_POINT('Ctrl Pts',(-0.373917289109901,1.97805431166006,
10.5466609820719));
#34464=CARTESIAN_POINT('Ctrl Pts',(-0.36760091349782,1.95868665645206,10.5476875739988));
#34465=CARTESIAN_POINT('Ctrl Pts',(-0.359774888340862,1.93980879168581,
10.5487141659257));
#34466=CARTESIAN_POINT('Ctrl Pts',(-0.35054562487635,1.92166701124007,10.5497407578526));
#34467=CARTESIAN_POINT('Ctrl Pts',(-0.341313014370206,1.90351865158086,
10.5507677220785));
#34468=CARTESIAN_POINT('Ctrl Pts',(-0.330676536465045,1.8861075620019,10.5517946863044));
#34469=CARTESIAN_POINT('Ctrl Pts',(-0.318787818793444,1.86965413702669,
10.5528216505303));
#34470=CARTESIAN_POINT('Ctrl Pts',(-0.306874829414054,1.85316712115176,
10.5538507113807));
#34471=CARTESIAN_POINT('Ctrl Pts',(-0.293705002890454,1.83764223713916,
10.554879772231));
#34472=CARTESIAN_POINT('Ctrl Pts',(-0.27946933195069,1.82326586314834,10.5559088330813));
#34473=CARTESIAN_POINT('Ctrl Pts',(-0.277909144740444,1.82169025530203,
10.556021615091));
#34474=CARTESIAN_POINT('Ctrl Pts',(-0.276336188231771,1.82012840325817,
10.5561343971006));
#34475=CARTESIAN_POINT('Ctrl Pts',(-0.274750737366453,1.81858052249961,
10.5562471791103));
#34476=CARTESIAN_POINT('Ctrl Pts',(-0.260075068010066,1.80425261949579,
10.5572911417578));
#34477=CARTESIAN_POINT('Ctrl Pts',(-0.244231881104207,1.79103309274978,
10.5583351044054));
#34478=CARTESIAN_POINT('Ctrl Pts',(-0.227414634405084,1.77911454682644,
10.5593790670529));
#34479=CARTESIAN_POINT('Ctrl Pts',(-0.210628324843434,1.76721792635263,
10.5604211092187));
#34480=CARTESIAN_POINT('Ctrl Pts',(-0.1928720714548,1.75661800526572,10.5614631513845));
#34481=CARTESIAN_POINT('Ctrl Pts',(-0.17437303283508,1.74746782356798,10.5625051935502));
#34482=CARTESIAN_POINT('Ctrl Pts',(-0.155893861892215,1.73832746902163,
10.5635461165791));
#34483=CARTESIAN_POINT('Ctrl Pts',(-0.136674132766392,1.73063411333564,
10.564587039608));
#34484=CARTESIAN_POINT('Ctrl Pts',(-0.116966226458038,1.724495283827,10.5656279626368));
#34485=CARTESIAN_POINT('Ctrl Pts',(-0.0972481986826536,1.71835330157552,
10.5666694202566));
#34486=CARTESIAN_POINT('Ctrl Pts',(-0.0770421905450604,1.71376767466379,
10.5677108778764));
#34487=CARTESIAN_POINT('Ctrl Pts',(-0.0566169602373726,1.71079644167418,
10.5687523354962));
#34488=CARTESIAN_POINT('Ctrl Pts',(-0.0361854891313576,1.70782430084336,
10.5697941113267));
#34489=CARTESIAN_POINT('Ctrl Pts',(-0.015535395219666,1.70646760593883,
10.5708358871572));
#34490=CARTESIAN_POINT('Ctrl Pts',(0.00505910623880618,1.70673253955601,
10.5718776629877));
#34491=CARTESIAN_POINT('Ctrl Pts',(0.0256981231795252,1.70699804583321,
10.5729216906403));
#34492=CARTESIAN_POINT('Ctrl Pts',(0.0462805743857226,1.70889211107832,
10.5739657182929));
#34493=CARTESIAN_POINT('Ctrl Pts',(0.0665362839956814,1.71236897323351,
10.5750097459456));
#34494=CARTESIAN_POINT('Ctrl Pts',(0.0737004629778612,1.71359869380394,
10.5753790048414));
#34495=CARTESIAN_POINT('Ctrl Pts',(0.0808238736536021,1.71502594797986,
10.5757482637373));
#34496=CARTESIAN_POINT('Ctrl Pts',(0.0878949967574936,1.71664721268132,
10.5761175226332));
#34497=CARTESIAN_POINT('Ctrl Pts',(0.107886359130526,1.72123082545024,10.5771614852807));
#34498=CARTESIAN_POINT('Ctrl Pts',(0.12757777724642,1.72739609197389,10.5782054479283));
#34499=CARTESIAN_POINT('Ctrl Pts',(0.146702583559594,1.7350846098382,10.5792494105758));
#34500=CARTESIAN_POINT('Ctrl Pts',(0.165792207730737,1.74275898384541,10.5802914527416));
#34501=CARTESIAN_POINT('Ctrl Pts',(0.184316591960079,1.7519508307966,10.5813334949074));
#34502=CARTESIAN_POINT('Ctrl Pts',(0.202024092421189,1.76255199499568,10.5823755370731));
#34503=CARTESIAN_POINT('Ctrl Pts',(0.219712575304979,1.77314177371095,10.583416460102));
#34504=CARTESIAN_POINT('Ctrl Pts',(0.236585273164828,1.78513751363441,10.5844573831308));
#34505=CARTESIAN_POINT('Ctrl Pts',(0.252415156711633,1.79838521478177,10.5854983061597));
#34506=CARTESIAN_POINT('Ctrl Pts',(0.268253170074052,1.81163971960315,10.5865397637795));
#34507=CARTESIAN_POINT('Ctrl Pts',(0.283046724588536,1.82614701031703,10.5875812213993));
#34508=CARTESIAN_POINT('Ctrl Pts',(0.296601536710333,1.84171252755685,10.5886226790191));
#34509=CARTESIAN_POINT('Ctrl Pts',(0.31016049041818,1.8572828007408,10.5896644548496));
#34510=CARTESIAN_POINT('Ctrl Pts',(0.322479492742613,1.87391136596323,10.5907062306801));
#34511=CARTESIAN_POINT('Ctrl Pts',(0.333404907572315,1.89137100487541,10.5917480065105));
#34512=CARTESIAN_POINT('Ctrl Pts',(0.344353937934095,1.9088683831933,10.5927920341631));
#34513=CARTESIAN_POINT('Ctrl Pts',(0.353903026703146,1.92719976842434,10.5938360618157));
#34514=CARTESIAN_POINT('Ctrl Pts',(0.361944400361301,1.94611322003792,10.5948800894683));
#34515=CARTESIAN_POINT('Ctrl Pts',(0.364788528819829,1.95280265996074,10.5952493483642));
#34516=CARTESIAN_POINT('Ctrl Pts',(0.367444498865245,1.95956474967142,10.5956186072601));
#34517=CARTESIAN_POINT('Ctrl Pts',(0.36990903717972,1.96638789645855,10.5959878661559));
#34518=CARTESIAN_POINT('Ctrl Pts',(0.376876739170362,1.98567818428725,10.5970318288035));
#34519=CARTESIAN_POINT('Ctrl Pts',(0.382352193119457,2.00557245137034,10.598075791451));
#34520=CARTESIAN_POINT('Ctrl Pts',(0.386240152861614,2.02581486457897,10.5991197540986));
#34521=CARTESIAN_POINT('Ctrl Pts',(0.390120960282875,2.04602003968726,10.6001617962644));
#34522=CARTESIAN_POINT('Ctrl Pts',(0.392419874689684,2.06657138645579,10.6012038384301));
#34523=CARTESIAN_POINT('Ctrl Pts',(0.393091615977614,2.08719877161722,10.6022458805959));
#34524=CARTESIAN_POINT('Ctrl Pts',(0.393762635825953,2.10780400329104,10.6032868036247));
#34525=CARTESIAN_POINT('Ctrl Pts',(0.392809899143816,2.12848438051671,10.6043277266536));
#34526=CARTESIAN_POINT('Ctrl Pts',(0.390239996818926,2.14896565002902,10.6053686496825));
#34527=CARTESIAN_POINT('Ctrl Pts',(0.387668774659185,2.16945743818753,10.6064101073023));
#34528=CARTESIAN_POINT('Ctrl Pts',(0.383478803244115,2.18974918228631,10.607451564922));
#34529=CARTESIAN_POINT('Ctrl Pts',(0.377728502379318,2.20957220674184,10.6084930225418));
#34530=CARTESIAN_POINT('Ctrl Pts',(0.37197644454691,2.22940128799557,10.6095347983723));
#34531=CARTESIAN_POINT('Ctrl Pts',(0.364663347732142,2.24876066852812,10.6105765742028));
#34532=CARTESIAN_POINT('Ctrl Pts',(0.355897095187741,2.26739817094857,10.6116183500333));
#34533=CARTESIAN_POINT('Ctrl Pts',(0.347111894189543,2.28607595875343,10.6126623776859));
#34534=CARTESIAN_POINT('Ctrl Pts',(0.3368676315669,2.30402811361368,10.6137064053385));
#34535=CARTESIAN_POINT('Ctrl Pts',(0.325317803676073,2.32102763766411,10.6147504329911));
#34536=CARTESIAN_POINT('Ctrl Pts',(0.321232780943391,2.32704014649516,10.615119691887));
#34537=CARTESIAN_POINT('Ctrl Pts',(0.316984819419497,2.33293377500648,10.6154889507829));
#34538=CARTESIAN_POINT('Ctrl Pts',(0.312581894557631,2.33869949558967,10.6158582096787));
#34539=CARTESIAN_POINT('Ctrl Pts',(0.300134018156454,2.35500024553087,10.6169021723263));
#34540=CARTESIAN_POINT('Ctrl Pts',(0.286370524356214,2.37037323148458,10.6179461349738));
#34541=CARTESIAN_POINT('Ctrl Pts',(0.271454963761862,2.38459988167434,10.6189900976214));
#34542=CARTESIAN_POINT('Ctrl Pts',(0.256566841948458,2.39880036040807,10.6200321397871));
#34543=CARTESIAN_POINT('Ctrl Pts',(0.240531345533421,2.41185814414704,10.6210741819529));
#34544=CARTESIAN_POINT('Ctrl Pts',(0.223551096465811,2.42358893255013,10.6221162241187));
#34545=CARTESIAN_POINT('Ctrl Pts',(0.206589083918966,2.43530712227075,10.6231571471475));
#34546=CARTESIAN_POINT('Ctrl Pts',(0.188684918897334,2.44570070607319,10.6241980701764));
#34547=CARTESIAN_POINT('Ctrl Pts',(0.170072766223247,2.45462676744596,10.6252389932052));
#34548=CARTESIAN_POINT('Ctrl Pts',(0.151451054832624,2.46355741301122,10.626280450825));
#34549=CARTESIAN_POINT('Ctrl Pts',(0.132121285848229,2.4710186977558,10.6273219084448));
#34550=CARTESIAN_POINT('Ctrl Pts',(0.112340990207518,2.47691430315019,10.6283633660646));
#34551=CARTESIAN_POINT('Ctrl Pts',(0.0925546508241235,2.48281170990906,
10.6294051418951));
#34552=CARTESIAN_POINT('Ctrl Pts',(0.072318225609469,2.48714230965479,10.6304469177255));
#34553=CARTESIAN_POINT('Ctrl Pts',(0.05190214898293,2.4898603043796,10.631488693556));
#34554=CARTESIAN_POINT('Ctrl Pts',(0.0314419425434746,2.49258417411169,
10.6325327212086));
#34555=CARTESIAN_POINT('Ctrl Pts',(0.0108020448549819,2.49368844048206,
10.6335767488612));
#34556=CARTESIAN_POINT('Ctrl Pts',(-0.00974358986208664,2.49317928792931,
10.6346207765138));
#34557=CARTESIAN_POINT('Ctrl Pts',(-0.0170103115543989,2.49299920734525,
10.6349900354097));
#34558=CARTESIAN_POINT('Ctrl Pts',(-0.0242652782571971,2.49261777284311,
10.6353592943056));
#34559=CARTESIAN_POINT('Ctrl Pts',(-0.0314965821387619,2.49203680351923,
10.6357285532014));
#34560=CARTESIAN_POINT('Ctrl Pts',(-0.0519408049590046,2.4903942966486,
10.636772515849));
#34561=CARTESIAN_POINT('Ctrl Pts',(-0.0723171146773218,2.48714337970345,
10.6378164784965));
#34562=CARTESIAN_POINT('Ctrl Pts',(-0.0923531993330601,2.48230325210878,
10.6388604411441));
#34563=CARTESIAN_POINT('Ctrl Pts',(-0.112352425452054,2.47747202845037,
10.6399024833098));
#34564=CARTESIAN_POINT('Ctrl Pts',(-0.132011947763811,2.47105751023603,
10.6409445254756));
#34565=CARTESIAN_POINT('Ctrl Pts',(-0.151067120319559,2.46313030052359,
10.6419865676414));
#34566=CARTESIAN_POINT('Ctrl Pts',(-0.170101827919337,2.45521160450986,
10.6430274906702));
#34567=CARTESIAN_POINT('Ctrl Pts',(-0.188532787305078,2.44578369670904,
10.6440684136991));
#34568=CARTESIAN_POINT('Ctrl Pts',(-0.206113074065671,2.43496610380634,
10.6451093367279));
#34569=CARTESIAN_POINT('Ctrl Pts',(-0.223702389603354,2.42414295526986,
10.6461507943477));
#34570=CARTESIAN_POINT('Ctrl Pts',(-0.240439524624304,2.4119290676693,10.6471922519675));
#34571=CARTESIAN_POINT('Ctrl Pts',(-0.256104086634659,2.39848883866742,
10.6482337095873));
#34572=CARTESIAN_POINT('Ctrl Pts',(-0.271773434851617,2.38504450308965,
10.6492754854178));
#34573=CARTESIAN_POINT('Ctrl Pts',(-0.28636902327221,2.37037358633983,10.6503172612483));
#34574=CARTESIAN_POINT('Ctrl Pts',(-0.299705953073875,2.35467868323062,
10.6513590370788));
#34575=CARTESIAN_POINT('Ctrl Pts',(-0.313071710951967,2.33894985523216,
10.6524030647314));
#34576=CARTESIAN_POINT('Ctrl Pts',(-0.325172947445456,2.32219321905018,
10.653447092384));
#34577=CARTESIAN_POINT('Ctrl Pts',(-0.335866566171454,2.30464246804658,
10.6544911200366));
#34578=CARTESIAN_POINT('Ctrl Pts',(-0.339648758945623,2.29843499746736,
10.6548603789325));
#34579=CARTESIAN_POINT('Ctrl Pts',(-0.343255286552126,2.29212841417969,
10.6552296378284));
#34580=CARTESIAN_POINT('Ctrl Pts',(-0.346681232595258,2.28573371521141,
10.6555988967243));
#34581=CARTESIAN_POINT('Ctrl Pts',(-0.356893907206437,2.26667124925972,
10.6566996498895));
#34582=CARTESIAN_POINT('Ctrl Pts',(-0.365553831017984,2.24672094907881,
10.6578004030547));
#34583=CARTESIAN_POINT('Ctrl Pts',(-0.372520334458991,2.22614868376072,
10.6589011562199));
#34584=CARTESIAN_POINT('Ctrl Pts',(-0.379459197939549,2.2056580399626,10.6599975420904));
#34585=CARTESIAN_POINT('Ctrl Pts',(-0.384717760168914,2.18455089922893,
10.6610939279609));
#34586=CARTESIAN_POINT('Ctrl Pts',(-0.388203047708099,2.16311326128591,
10.6621903138313));
#34587=CARTESIAN_POINT('Ctrl Pts',(-0.391586797707641,2.14230017009492,
10.6632547584853));
#34588=CARTESIAN_POINT('Ctrl Pts',(-0.393299115142935,2.12117615124244,
10.6643192031393));
#34589=CARTESIAN_POINT('Ctrl Pts',(-0.393299999656376,2.1000164406377,10.6653836477933));
#34590=CARTESIAN_POINT('',(-0.393299837322886,2.09964228252567,10.7903836477965));
#34591=CARTESIAN_POINT('Ctrl Pts',(-0.393299999656379,2.10001644057314,
10.6653836477965));
#34592=CARTESIAN_POINT('Ctrl Pts',(-0.393300903919296,2.07838418954183,
10.6664718637175));
#34593=CARTESIAN_POINT('Ctrl Pts',(-0.391512781482813,2.05678450351341,
10.6675600796385));
#34594=CARTESIAN_POINT('Ctrl Pts',(-0.387977325474063,2.03551368425788,
10.6686482955595));
#34595=CARTESIAN_POINT('Ctrl Pts',(-0.384283948480357,2.01329274464465,
10.6697851196741));
#34596=CARTESIAN_POINT('Ctrl Pts',(-0.378683490893823,1.99143152671946,
10.6709219437887));
#34597=CARTESIAN_POINT('Ctrl Pts',(-0.371281621402311,1.97025082809948,
10.6720587679033));
#34598=CARTESIAN_POINT('Ctrl Pts',(-0.363879751910796,1.94907012947949,
10.6731955920179));
#34599=CARTESIAN_POINT('Ctrl Pts',(-0.354676875977424,1.92857061784174,
10.6743324161325));
#34600=CARTESIAN_POINT('Ctrl Pts',(-0.343833048533687,1.90904522855914,
10.6754692402471));
#34601=CARTESIAN_POINT('Ctrl Pts',(-0.333874999031955,1.8911147705151,10.6765132028946));
#34602=CARTESIAN_POINT('Ctrl Pts',(-0.322480926677385,1.87391193429824,
10.6775571655422));
#34603=CARTESIAN_POINT('Ctrl Pts',(-0.309781032102686,1.85767665785279,
10.6786011281898));
#34604=CARTESIAN_POINT('Ctrl Pts',(-0.297104500352545,1.84147124794781,
10.6796431703555));
#34605=CARTESIAN_POINT('Ctrl Pts',(-0.283127316027989,1.82623047435161,
10.6806852125213));
#34606=CARTESIAN_POINT('Ctrl Pts',(-0.26802329913917,1.81216601813101,10.6817272546871));
#34607=CARTESIAN_POINT('Ctrl Pts',(-0.252935503727212,1.79811666691546,
10.6827681777159));
#34608=CARTESIAN_POINT('Ctrl Pts',(-0.236723794323403,1.78524164506732,
10.6838091007448));
#34609=CARTESIAN_POINT('Ctrl Pts',(-0.219599190286858,1.77371624982945,
10.6848500237736));
#34610=CARTESIAN_POINT('Ctrl Pts',(-0.202465791499996,1.76218493544898,
10.6858914813934));
#34611=CARTESIAN_POINT('Ctrl Pts',(-0.184419162849741,1.75200505659938,
10.6869329390132));
#34612=CARTESIAN_POINT('Ctrl Pts',(-0.165700186865509,1.74330918420467,
10.687974396633));
#34613=CARTESIAN_POINT('Ctrl Pts',(-0.146975491418038,1.73461065484185,
10.6890161724635));
#34614=CARTESIAN_POINT('Ctrl Pts',(-0.127578721642701,1.7273973115178,10.690057948294));
#34615=CARTESIAN_POINT('Ctrl Pts',(-0.107770838341297,1.72175360358199,
10.6910997241245));
#34616=CARTESIAN_POINT('Ctrl Pts',(-0.0879201398506443,1.71609769664339,
10.6921437517771));
#34617=CARTESIAN_POINT('Ctrl Pts',(-0.06765727571691,1.7120183440099,10.6931877794297));
#34618=CARTESIAN_POINT('Ctrl Pts',(-0.0472542116476989,1.70954906904765,
10.6942318070823));
#34619=CARTESIAN_POINT('Ctrl Pts',(-0.0400379153251642,1.7086757188602,
10.6946010659781));
#34620=CARTESIAN_POINT('Ctrl Pts',(-0.0328041132268868,1.70800330430401,
10.694970324874));
#34621=CARTESIAN_POINT('Ctrl Pts',(-0.0255648510851573,1.70753174855921,
10.6953395837698));
#34622=CARTESIAN_POINT('Ctrl Pts',(-0.0050981288021612,1.70619857395095,
10.6963835464174));
#34623=CARTESIAN_POINT('Ctrl Pts',(0.0155341411384485,1.70646670791081,
10.6974275090649));
#34624=CARTESIAN_POINT('Ctrl Pts',(0.0360597346621666,1.70835655816024,
10.6984714717125));
#34625=CARTESIAN_POINT('Ctrl Pts',(0.0565475691448373,1.71024293182649,
10.6995135138782));
#34626=CARTESIAN_POINT('Ctrl Pts',(0.0769283868876979,1.71374509252851,
10.700555556044));
#34627=CARTESIAN_POINT('Ctrl Pts',(0.0969301107475258,1.71883147607591,
10.7015975982098));
#34628=CARTESIAN_POINT('Ctrl Pts',(0.116910353070145,1.72391239692728,10.7026385212386));
#34629=CARTESIAN_POINT('Ctrl Pts',(0.136511593186629,1.73057401049135,10.7036794442675));
#34630=CARTESIAN_POINT('Ctrl Pts',(0.155472209444625,1.73873377947778,10.7047203672964));
#34631=CARTESIAN_POINT('Ctrl Pts',(0.174442563380965,1.7468977391089,10.7057618249162));
#34632=CARTESIAN_POINT('Ctrl Pts',(0.192770953952402,1.75656111523172,10.7068032825359));
#34633=CARTESIAN_POINT('Ctrl Pts',(0.210215519086775,1.76759313253924,10.7078447401557));
#34634=CARTESIAN_POINT('Ctrl Pts',(0.227665414296312,1.778628520609,10.7088865159862));
#34635=CARTESIAN_POINT('Ctrl Pts',(0.244230344470396,1.7910329588451,10.7099282918167));
#34636=CARTESIAN_POINT('Ctrl Pts',(0.259698040286721,1.8046327406918,10.7109700676472));
#34637=CARTESIAN_POINT('Ctrl Pts',(0.275199169878563,1.81826191877559,10.7120140952998));
#34638=CARTESIAN_POINT('Ctrl Pts',(0.289597817093409,1.83309107044353,10.7130581229525));
#34639=CARTESIAN_POINT('Ctrl Pts',(0.302718574933163,1.84890966886311,10.714102150605));
#34640=CARTESIAN_POINT('Ctrl Pts',(0.30735921499739,1.85450449977778,10.7144714095009));
#34641=CARTESIAN_POINT('Ctrl Pts',(0.31184038097793,1.86022281995002,10.7148406683968));
#34642=CARTESIAN_POINT('Ctrl Pts',(0.316155616893762,1.86605445952845,10.7152099272926));
#34643=CARTESIAN_POINT('Ctrl Pts',(0.328355580556014,1.88254157456363,10.7162538899402));
#34644=CARTESIAN_POINT('Ctrl Pts',(0.339298749242088,1.90003470229508,10.7172978525877));
#34645=CARTESIAN_POINT('Ctrl Pts',(0.348820603964078,1.91831599891533,10.7183418152353));
#34646=CARTESIAN_POINT('Ctrl Pts',(0.358324942208264,1.93656366512051,10.7193838574011));
#34647=CARTESIAN_POINT('Ctrl Pts',(0.366412767688192,1.95559600445267,10.7204258995668));
#34648=CARTESIAN_POINT('Ctrl Pts',(0.372963339866515,1.97516716331183,10.7214679417326));
#34649=CARTESIAN_POINT('Ctrl Pts',(0.379506876833226,1.99471730305384,10.7225088647615));
#34650=CARTESIAN_POINT('Ctrl Pts',(0.384516178323465,2.01480442848181,10.7235497877903));
#34651=CARTESIAN_POINT('Ctrl Pts',(0.387919022641102,2.03516388449967,10.7245907108192));
#34652=CARTESIAN_POINT('Ctrl Pts',(0.391323614570892,2.0555337966035,10.7256321684389));
#34653=CARTESIAN_POINT('Ctrl Pts',(0.393119963899375,2.07617559565587,10.7266736260587));
#34654=CARTESIAN_POINT('Ctrl Pts',(0.393287104536297,2.09681512865945,10.7277150836785));
#34655=CARTESIAN_POINT('Ctrl Pts',(0.39345429624197,2.11746096794018,10.728756859509));
#34656=CARTESIAN_POINT('Ctrl Pts',(0.391991318491797,2.13810380436656,10.7297986353395));
#34657=CARTESIAN_POINT('Ctrl Pts',(0.388929321648321,2.15847112759454,10.73084041117));
#34658=CARTESIAN_POINT('Ctrl Pts',(0.385860706229182,2.17888247525387,10.7318844388226));
#34659=CARTESIAN_POINT('Ctrl Pts',(0.381186337904448,2.19901640337461,10.7329284664752));
#34660=CARTESIAN_POINT('Ctrl Pts',(0.374988280426774,2.21861146463378,10.7339724941278));
#34661=CARTESIAN_POINT('Ctrl Pts',(0.372796108739457,2.22554198095415,10.7343417530237));
#34662=CARTESIAN_POINT('Ctrl Pts',(0.370413778870354,2.23240525557609,10.7347110119195));
#34663=CARTESIAN_POINT('Ctrl Pts',(0.367846347073399,2.23919035507088,10.7350802708154));
#34664=CARTESIAN_POINT('Ctrl Pts',(0.36058774632988,2.25837307622284,10.736124233463));
#34665=CARTESIAN_POINT('Ctrl Pts',(0.351802946269833,2.27704363450668,10.7371681961105));
#34666=CARTESIAN_POINT('Ctrl Pts',(0.341586056766116,2.29494577662257,10.7382121587581));
#34667=CARTESIAN_POINT('Ctrl Pts',(0.331387962331579,2.31281498581896,10.7392542009239));
#34668=CARTESIAN_POINT('Ctrl Pts',(0.319763316728726,2.32991792346314,10.7402962430896));
#34669=CARTESIAN_POINT('Ctrl Pts',(0.306853479031764,2.34601998375356,10.7413382852554));
#34670=CARTESIAN_POINT('Ctrl Pts',(0.293957506297671,2.3621047506842,10.7423792082843));
#34671=CARTESIAN_POINT('Ctrl Pts',(0.279779516999117,2.37719018501119,10.7434201313131));
#34672=CARTESIAN_POINT('Ctrl Pts',(0.264502942970299,2.39107229885383,10.744461054342));
#34673=CARTESIAN_POINT('Ctrl Pts',(0.24921852329122,2.40496154218831,10.7455025119618));
#34674=CARTESIAN_POINT('Ctrl Pts',(0.232834925418655,2.41764572366694,10.7465439695816));
#34675=CARTESIAN_POINT('Ctrl Pts',(0.215571312777791,2.42895881065456,10.7475854272014));
#34676=CARTESIAN_POINT('Ctrl Pts',(0.198302425350644,2.44027535428345,10.7486272030319));
#34677=CARTESIAN_POINT('Ctrl Pts',(0.180153622595453,2.45021959674736,10.7496689788624));
#34678=CARTESIAN_POINT('Ctrl Pts',(0.161370898342717,2.45867021505565,10.7507107546929));
#34679=CARTESIAN_POINT('Ctrl Pts',(0.142547574805271,2.46713909956718,10.7517547823455));
#34680=CARTESIAN_POINT('Ctrl Pts',(0.123088287520985,2.47410766607676,10.7527988099981));
#34681=CARTESIAN_POINT('Ctrl Pts',(0.103257288672177,2.47950338909695,10.7538428376507));
#34682=CARTESIAN_POINT('Ctrl Pts',(0.096243324319536,2.48141178560329,10.7542120965465));
#34683=CARTESIAN_POINT('Ctrl Pts',(0.0891829619311183,2.48312389455941,
10.7545813554424));
#34684=CARTESIAN_POINT('Ctrl Pts',(0.0820881315711749,2.48463804889162,
10.7549506143382));
#34685=CARTESIAN_POINT('Ctrl Pts',(0.0620297444348467,2.488918840995,10.7559945769858));
#34686=CARTESIAN_POINT('Ctrl Pts',(0.0415758337412953,2.49163913437268,
10.7570385396333));
#34687=CARTESIAN_POINT('Ctrl Pts',(0.0209928052276988,2.49273934374935,
10.7580825022809));
#34688=CARTESIAN_POINT('Ctrl Pts',(0.000447641413002693,2.49383752917232,
10.7591245444467));
#34689=CARTESIAN_POINT('Ctrl Pts',(-0.0202254454845265,2.49332144819461,
10.7601665866124));
#34690=CARTESIAN_POINT('Ctrl Pts',(-0.0407526744854151,2.49118296169732,
10.7612086287782));
#34691=CARTESIAN_POINT('Ctrl Pts',(-0.0612578575648515,2.48904677190093,
10.7622495518071));
#34692=CARTESIAN_POINT('Ctrl Pts',(-0.0816167626296247,2.48529168282829,
10.7632904748359));
#34693=CARTESIAN_POINT('Ctrl Pts',(-0.101558578051101,2.47996150492417,
10.7643313978648));
#34694=CARTESIAN_POINT('Ctrl Pts',(-0.12151063506921,2.4746285895796,10.7653728554845));
#34695=CARTESIAN_POINT('Ctrl Pts',(-0.14104445952005,2.4677191437732,10.7664143131043));
#34696=CARTESIAN_POINT('Ctrl Pts',(-0.159901811069196,2.45932756757142,
10.7674557707241));
#34697=CARTESIAN_POINT('Ctrl Pts',(-0.178764924361347,2.45093342737726,
10.7684975465546));
#34698=CARTESIAN_POINT('Ctrl Pts',(-0.196950496329909,2.44105658720445,
10.7695393223851));
#34699=CARTESIAN_POINT('Ctrl Pts',(-0.214223355526875,2.42983820874302,
10.7705810982156));
#34700=CARTESIAN_POINT('Ctrl Pts',(-0.231533550400975,2.41859558150197,
10.7716251258682));
#34701=CARTESIAN_POINT('Ctrl Pts',(-0.247926509704076,2.40600607531257,
10.7726691535208));
#34702=CARTESIAN_POINT('Ctrl Pts',(-0.263198208226789,2.39225261878417,
10.7737131811734));
#34703=CARTESIAN_POINT('Ctrl Pts',(-0.268599607816748,2.38738820148688,
10.7740824400693));
#34704=CARTESIAN_POINT('Ctrl Pts',(-0.27386108141518,2.38237851789273,10.7744516989651));
#34705=CARTESIAN_POINT('Ctrl Pts',(-0.278974769357337,2.37723269659624,
10.774820957861));
#34706=CARTESIAN_POINT('Ctrl Pts',(-0.293233924883227,2.36288393949469,
10.7758506100583));
#34707=CARTESIAN_POINT('Ctrl Pts',(-0.306431222875898,2.34738350856294,
10.7768802622555));
#34708=CARTESIAN_POINT('Ctrl Pts',(-0.318374647887716,2.33091659442832,
10.7779099144527));
#34709=CARTESIAN_POINT('Ctrl Pts',(-0.330432044486473,2.3142925427612,10.7789493922314));
#34710=CARTESIAN_POINT('Ctrl Pts',(-0.341210903503436,2.29668397029978,
10.77998887001));
#34711=CARTESIAN_POINT('Ctrl Pts',(-0.350553101672658,2.27831829100706,
10.7810283477887));
#34712=CARTESIAN_POINT('Ctrl Pts',(-0.359783125904629,2.26017313267945,
10.7820553443169));
#34713=CARTESIAN_POINT('Ctrl Pts',(-0.367610470850558,2.24128964931751,
10.7830823408451));
#34714=CARTESIAN_POINT('Ctrl Pts',(-0.373927706534286,2.22191374116977,
10.7841093373733));
#34715=CARTESIAN_POINT('Ctrl Pts',(-0.380360103757361,2.20218461532995,
10.7851550557771));
#34716=CARTESIAN_POINT('Ctrl Pts',(-0.385226426293683,2.18194566437344,
10.786200774181));
#34717=CARTESIAN_POINT('Ctrl Pts',(-0.388466071386825,2.16147358279201,
10.7872464925849));
#34718=CARTESIAN_POINT('Ctrl Pts',(-0.391705716479968,2.14100150121058,
10.7882922109888));
#34719=CARTESIAN_POINT('Ctrl Pts',(-0.393318623483942,2.12029711383068,
10.7893379293926));
#34720=CARTESIAN_POINT('Ctrl Pts',(-0.393299837322886,2.09964228252567,
10.7903836477965));
#34721=CARTESIAN_POINT('',(-0.393454859789483,2.10017238244214,10.9153836477965));
#34722=CARTESIAN_POINT('Ctrl Pts',(-0.393365501908144,2.09964222280185,
10.7903836477965));
#34723=CARTESIAN_POINT('Ctrl Pts',(-0.393628539003501,2.07127590643749,
10.7918195323256));
#34724=CARTESIAN_POINT('Ctrl Pts',(-0.377873717533349,1.91235128146771,
10.7998788646957));
#34725=CARTESIAN_POINT('Ctrl Pts',(-0.161856479690965,1.66402119264042,
10.8145616449065));
#34726=CARTESIAN_POINT('Ctrl Pts',(0.278962950142402,1.72790496787461,10.8344319884294));
#34727=CARTESIAN_POINT('Ctrl Pts',(0.463871850595977,2.13313527891918,10.8543023319521));
#34728=CARTESIAN_POINT('Ctrl Pts',(0.223241478578169,2.50796848251641,10.8741726754749));
#34729=CARTESIAN_POINT('Ctrl Pts',(-0.22218255845236,2.50854614329848,10.8940430189977));
#34730=CARTESIAN_POINT('Ctrl Pts',(-0.389209440306793,2.2498445668232,10.9077800097716));
#34731=CARTESIAN_POINT('Ctrl Pts',(-0.393910523469697,2.10982310132666,
10.9148935527045));
#34732=CARTESIAN_POINT('Ctrl Pts',(-0.393857559113655,2.10017255887481,
10.9153836477965));
#34733=CARTESIAN_POINT('',(-0.393299911892188,2.10026325956176,11.0403836477918));
#34734=CARTESIAN_POINT('Ctrl Pts',(-0.393299962252333,2.10017231457764,
10.9153836477965));
#34735=CARTESIAN_POINT('Ctrl Pts',(-0.393308860645182,2.07986214918405,
10.9164165483161));
#34736=CARTESIAN_POINT('Ctrl Pts',(-0.391740229032019,2.05948767802324,
10.9174494488357));
#34737=CARTESIAN_POINT('Ctrl Pts',(-0.388590402319534,2.03931730703782,
10.9184823493553));
#34738=CARTESIAN_POINT('Ctrl Pts',(-0.385446002585379,2.01918168849316,
10.9195134702441));
#34739=CARTESIAN_POINT('Ctrl Pts',(-0.380725869940055,1.9992502169752,10.9205445911328));
#34740=CARTESIAN_POINT('Ctrl Pts',(-0.374478210275068,1.97978785406964,
10.9215757120216));
#34741=CARTESIAN_POINT('Ctrl Pts',(-0.368231000004424,1.96032689109242,
10.9226067587418));
#34742=CARTESIAN_POINT('Ctrl Pts',(-0.360456661425524,1.94133570028298,
10.923637805462));
#34743=CARTESIAN_POINT('Ctrl Pts',(-0.351253818214342,1.92306598633998,
10.9246688521823));
#34744=CARTESIAN_POINT('Ctrl Pts',(-0.342052869418203,1.90480003323698,
10.9256996866604));
#34745=CARTESIAN_POINT('Ctrl Pts',(-0.331424349561752,1.88725592944221,
10.9267305211386));
#34746=CARTESIAN_POINT('Ctrl Pts',(-0.319513281200284,1.87066148789044,
10.9277613556167));
#34747=CARTESIAN_POINT('Ctrl Pts',(-0.307574770851816,1.85402881429805,
10.9287945650411));
#34748=CARTESIAN_POINT('Ctrl Pts',(-0.294348272970208,1.8383507713546,10.9298277744654));
#34749=CARTESIAN_POINT('Ctrl Pts',(-0.280020318160216,1.82382340537719,
10.9308609838898));
#34750=CARTESIAN_POINT('Ctrl Pts',(-0.266510107499354,1.81012516460906,
10.9318352246076));
#34751=CARTESIAN_POINT('Ctrl Pts',(-0.25202134251128,1.79745002976386,10.9328094653255));
#34752=CARTESIAN_POINT('Ctrl Pts',(-0.236736783861808,1.78592901253575,
10.9337837060434));
#34753=CARTESIAN_POINT('Ctrl Pts',(-0.22035837961134,1.77358348906557,10.9348276686909));
#34754=CARTESIAN_POINT('Ctrl Pts',(-0.202962869780021,1.76248580027779,
10.9358716313385));
#34755=CARTESIAN_POINT('Ctrl Pts',(-0.184766632364385,1.75280238830786,
10.936915593986));
#34756=CARTESIAN_POINT('Ctrl Pts',(-0.166603868888234,1.7431367900177,10.9379576361518));
#34757=CARTESIAN_POINT('Ctrl Pts',(-0.147643915980189,1.73488069849844,
10.9389996783176));
#34758=CARTESIAN_POINT('Ctrl Pts',(-0.128131548108157,1.72815702725558,
10.9400417204833));
#34759=CARTESIAN_POINT('Ctrl Pts',(-0.108640136212677,1.72144057713001,
10.9410826435122));
#34760=CARTESIAN_POINT('Ctrl Pts',(-0.0885981698533844,1.71625354581778,
10.942123566541));
#34761=CARTESIAN_POINT('Ctrl Pts',(-0.0682696540235158,1.71267049642519,
10.9431644895699));
#34762=CARTESIAN_POINT('Ctrl Pts',(-0.0479306979977496,1.70908560687182,
10.9442059471897));
#34763=CARTESIAN_POINT('Ctrl Pts',(-0.0273056203105137,1.7071064885264,
10.9452474048095));
#34764=CARTESIAN_POINT('Ctrl Pts',(-0.00666837749199288,1.70675653502998,
10.9462888624293));
#34765=CARTESIAN_POINT('Ctrl Pts',(0.0139751709039052,1.70640647460752,
10.9473306382597));
#34766=CARTESIAN_POINT('Ctrl Pts',(0.0346301561646096,1.70768654628708,
10.9483724140902));
#34767=CARTESIAN_POINT('Ctrl Pts',(0.0550238027152715,1.71056801475129,
10.9494141899207));
#34768=CARTESIAN_POINT('Ctrl Pts',(0.0754615305957612,1.71345571157498,
10.9504582175733));
#34769=CARTESIAN_POINT('Ctrl Pts',(0.0956360731470906,1.71795155561728,
10.9515022452259));
#34770=CARTESIAN_POINT('Ctrl Pts',(0.1152852664044,1.72397580217482,10.9525462728785));
#34771=CARTESIAN_POINT('Ctrl Pts',(0.12223492850275,1.72610649921789,10.9529155317744));
#34772=CARTESIAN_POINT('Ctrl Pts',(0.129119035910486,1.72842794259158,10.9532847906703));
#34773=CARTESIAN_POINT('Ctrl Pts',(0.135926610840863,1.73093517308565,10.9536540495661));
#34774=CARTESIAN_POINT('Ctrl Pts',(0.155172874173353,1.73802357370082,10.9546980122137));
#34775=CARTESIAN_POINT('Ctrl Pts',(0.17392051339201,1.74664265035955,10.9557419748612));
#34776=CARTESIAN_POINT('Ctrl Pts',(0.191912451650082,1.75670056670356,10.9567859375088));
#34777=CARTESIAN_POINT('Ctrl Pts',(0.209871291798986,1.76673998042666,10.9578279796746));
#34778=CARTESIAN_POINT('Ctrl Pts',(0.227076526462355,1.77821267678054,10.9588700218403));
#34779=CARTESIAN_POINT('Ctrl Pts',(0.243292306921786,1.79097938031148,10.9599120640061));
#34780=CARTESIAN_POINT('Ctrl Pts',(0.259490671887751,1.8037323726034,10.9609529870349));
#34781=CARTESIAN_POINT('Ctrl Pts',(0.274701099211307,1.81777618298433,10.9619939100638));
#34782=CARTESIAN_POINT('Ctrl Pts',(0.288717984224568,1.83292919368583,10.9630348330927));
#34783=CARTESIAN_POINT('Ctrl Pts',(0.302742067944637,1.84808998657868,10.9640762907124));
#34784=CARTESIAN_POINT('Ctrl Pts',(0.315570873307961,1.86436058865663,10.9651177483322));
#34785=CARTESIAN_POINT('Ctrl Pts',(0.327036432902423,1.88152331576468,10.966159205952));
#34786=CARTESIAN_POINT('Ctrl Pts',(0.338505495725203,1.89869128683411,10.9672009817825));
#34787=CARTESIAN_POINT('Ctrl Pts',(0.348610105271661,1.91675129418567,10.968242757613));
#34788=CARTESIAN_POINT('Ctrl Pts',(0.357226764363725,1.93545842828567,10.9692845334435));
#34789=CARTESIAN_POINT('Ctrl Pts',(0.365862048559952,1.95420599828053,10.9703285610961));
#34790=CARTESIAN_POINT('Ctrl Pts',(0.373002706807748,1.97360279648528,10.9713725887487));
#34791=CARTESIAN_POINT('Ctrl Pts',(0.378573875790318,1.99338522349554,10.9724166164013));
#34792=CARTESIAN_POINT('Ctrl Pts',(0.380544325233959,2.00038200862594,10.9727858752972));
#34793=CARTESIAN_POINT('Ctrl Pts',(0.382318905809099,2.00742692863409,10.973155134193));
#34794=CARTESIAN_POINT('Ctrl Pts',(0.383895844834153,2.01450806869025,10.9735243930889));
#34795=CARTESIAN_POINT('Ctrl Pts',(0.388354140783265,2.03452775082497,10.9745683557365));
#34796=CARTESIAN_POINT('Ctrl Pts',(0.391255502666754,2.05495676347717,10.975612318384));
#34797=CARTESIAN_POINT('Ctrl Pts',(0.392537987796697,2.07552923915117,10.9766562810316));
#34798=CARTESIAN_POINT('Ctrl Pts',(0.393818113657047,2.09606386953937,10.9776983231973));
#34799=CARTESIAN_POINT('Ctrl Pts',(0.393485169553287,2.11674071672829,10.9787403653631));
#34800=CARTESIAN_POINT('Ctrl Pts',(0.39152859160775,2.13728608257315,10.9797824075289));
#34801=CARTESIAN_POINT('Ctrl Pts',(0.38957411499619,2.15780938301784,10.9808233305577));
#34802=CARTESIAN_POINT('Ctrl Pts',(0.385999506927345,2.17820075095957,10.9818642535866));
#34803=CARTESIAN_POINT('Ctrl Pts',(0.380846177350917,2.19818899733266,10.9829051766154));
#34804=CARTESIAN_POINT('Ctrl Pts',(0.375690201158729,2.21818750914814,10.9839466342352));
#34805=CARTESIAN_POINT('Ctrl Pts',(0.368954051761435,2.23778176928542,10.984988091855));
#34806=CARTESIAN_POINT('Ctrl Pts',(0.360729838098909,2.25671271137063,10.9860295494748));
#34807=CARTESIAN_POINT('Ctrl Pts',(0.352503111580559,2.27564943768398,10.9870713253053));
#34808=CARTESIAN_POINT('Ctrl Pts',(0.342787741772241,2.29392178261049,10.9881131011358));
#34809=CARTESIAN_POINT('Ctrl Pts',(0.331722801740919,2.31129333355588,10.9891548769662));
#34810=CARTESIAN_POINT('Ctrl Pts',(0.320633944590629,2.32870243350283,10.9901989046188));
#34811=CARTESIAN_POINT('Ctrl Pts',(0.308190136705372,2.3452062641528,10.9912429322714));
#34812=CARTESIAN_POINT('Ctrl Pts',(0.294572492317858,2.36059918796812,10.992286959924));
#34813=CARTESIAN_POINT('Ctrl Pts',(0.289756109994744,2.36604346335493,10.9926562188199));
#34814=CARTESIAN_POINT('Ctrl Pts',(0.284793227646956,2.37134910496925,10.9930254777158));
#34815=CARTESIAN_POINT('Ctrl Pts',(0.279692903892098,2.37650817259605,10.9933947366116));
#34816=CARTESIAN_POINT('Ctrl Pts',(0.265273352866704,2.39109380332532,10.9944386992592));
#34817=CARTESIAN_POINT('Ctrl Pts',(0.249666832871676,2.40459191402152,10.9954826619067));
#34818=CARTESIAN_POINT('Ctrl Pts',(0.233063359361353,2.41680650328426,10.9965266245543));
#34819=CARTESIAN_POINT('Ctrl Pts',(0.216490429729673,2.42899862249386,10.99756866672));
#34820=CARTESIAN_POINT('Ctrl Pts',(0.198924737747735,2.43991142812055,10.9986107088858));
#34821=CARTESIAN_POINT('Ctrl Pts',(0.180590695298224,2.44938788011564,10.9996527510516));
#34822=CARTESIAN_POINT('Ctrl Pts',(0.162276343322299,2.45885415455016,11.0006936740804));
#34823=CARTESIAN_POINT('Ctrl Pts',(0.143195916125291,2.46688677600022,11.0017345971093));
#34824=CARTESIAN_POINT('Ctrl Pts',(0.123599850283095,2.47337376315161,11.0027755201382));
#34825=CARTESIAN_POINT('Ctrl Pts',(0.103993720412203,2.47986408185054,11.0038169777579));
#34826=CARTESIAN_POINT('Ctrl Pts',(0.0838721162823775,2.48480693388882,
11.0048584353777));
#34827=CARTESIAN_POINT('Ctrl Pts',(0.0635027257726444,2.48813952880304,
11.0058998929975));
#34828=CARTESIAN_POINT('Ctrl Pts',(0.0431271115260769,2.49147314197029,
11.006941668828));
#34829=CARTESIAN_POINT('Ctrl Pts',(0.0225042915339611,2.4931954355568,11.0079834446585));
#34830=CARTESIAN_POINT('Ctrl Pts',(0.00190832850244365,2.49329537027828,
11.009025220489));
#34831=CARTESIAN_POINT('Ctrl Pts',(-0.018732153170544,2.49339552101093,
11.0100692481416));
#34832=CARTESIAN_POINT('Ctrl Pts',(-0.0393449275255872,2.49186636627842,
11.0111132757942));
#34833=CARTESIAN_POINT('Ctrl Pts',(-0.0596590504325071,2.4887488748556,
11.0121573034468));
#34834=CARTESIAN_POINT('Ctrl Pts',(-0.0668438894322014,2.48764625900265,
11.0125265623427));
#34835=CARTESIAN_POINT('Ctrl Pts',(-0.0739914657842849,2.48634541833996,
11.0128958212386));
#34836=CARTESIAN_POINT('Ctrl Pts',(-0.0810901996203999,2.48484967133353,
11.0132650801344));
#34837=CARTESIAN_POINT('Ctrl Pts',(-0.101159622599137,2.48062092011757,
11.014309042782));
#34838=CARTESIAN_POINT('Ctrl Pts',(-0.120957167013114,2.47480544989585,
11.0153530054296));
#34839=CARTESIAN_POINT('Ctrl Pts',(-0.140215172576819,2.46745692996493,
11.0163969680771));
#34840=CARTESIAN_POINT('Ctrl Pts',(-0.159437750964121,2.46012192842828,
11.0174390102429));
#34841=CARTESIAN_POINT('Ctrl Pts',(-0.178122059783856,2.45125967897456,
11.0184810524086));
#34842=CARTESIAN_POINT('Ctrl Pts',(-0.196014578744431,2.44097386251683,
11.0195230945744));
#34843=CARTESIAN_POINT('Ctrl Pts',(-0.213887881420712,2.43069909286439,
11.0205640176033));
#34844=CARTESIAN_POINT('Ctrl Pts',(-0.230970433358254,2.419004131185,11.0216049406321));
#34845=CARTESIAN_POINT('Ctrl Pts',(-0.247032512819492,2.40603893152684,
11.022645863661));
#34846=CARTESIAN_POINT('Ctrl Pts',(-0.263102841346124,2.39306707328003,
11.0236873212808));
#34847=CARTESIAN_POINT('Ctrl Pts',(-0.27815106772843,2.37882412338271,11.0247287789006));
#34848=CARTESIAN_POINT('Ctrl Pts',(-0.29197949233482,2.36350116898394,11.0257702365204));
#34849=CARTESIAN_POINT('Ctrl Pts',(-0.305812142127802,2.34817353275456,
11.0268120123509));
#34850=CARTESIAN_POINT('Ctrl Pts',(-0.318423782504393,2.33176580510451,
11.0278537881814));
#34851=CARTESIAN_POINT('Ctrl Pts',(-0.329656776341884,2.31450244709997,
11.0288955640119));
#34852=CARTESIAN_POINT('Ctrl Pts',(-0.340914050550457,2.29720177395537,
11.0299395916645));
#34853=CARTESIAN_POINT('Ctrl Pts',(-0.350786377080374,2.2790424251318,11.0309836193171));
#34854=CARTESIAN_POINT('Ctrl Pts',(-0.359161536257712,2.26027439244309,
11.0320276469697));
#34855=CARTESIAN_POINT('Ctrl Pts',(-0.362123720279164,2.25363638528795,
11.0323969058655));
#34856=CARTESIAN_POINT('Ctrl Pts',(-0.364899062387056,2.24692240656288,
11.0327661647614));
#34857=CARTESIAN_POINT('Ctrl Pts',(-0.367484084415039,2.24014398917414,
11.0331354236572));
#34858=CARTESIAN_POINT('Ctrl Pts',(-0.375941032129185,2.21796827042949,
11.034343461013));
#34859=CARTESIAN_POINT('Ctrl Pts',(-0.382399795014722,2.19499045153081,
11.0355514983688));
#34860=CARTESIAN_POINT('Ctrl Pts',(-0.386735574710299,2.17155756601153,
11.0367595357245));
#34861=CARTESIAN_POINT('Ctrl Pts',(-0.391071354405876,2.14812468049226,
11.0379675730803));
#34862=CARTESIAN_POINT('Ctrl Pts',(-0.393283864787408,2.12423703226915,
11.0391756104361));
#34863=CARTESIAN_POINT('Ctrl Pts',(-0.393299911892188,2.10026325956174,
11.0403836477918));
#34864=CARTESIAN_POINT('',(-0.393299891708519,2.09970814032956,11.165383647801));
#34865=CARTESIAN_POINT('Ctrl Pts',(-0.39329991189225,2.1002632594691,11.0403836477965));
#34866=CARTESIAN_POINT('Ctrl Pts',(-0.39331388416996,2.07938919324474,11.0414354910785));
#34867=CARTESIAN_POINT('Ctrl Pts',(-0.391661618617504,2.0585053384122,11.0424873343604));
#34868=CARTESIAN_POINT('Ctrl Pts',(-0.388365281852791,2.03789285184939,
11.0435391776424));
#34869=CARTESIAN_POINT('Ctrl Pts',(-0.385083289625895,2.01737006382592,
11.0445864436597));
#34870=CARTESIAN_POINT('Ctrl Pts',(-0.380171680434979,1.99711699783367,
11.045633709677));
#34871=CARTESIAN_POINT('Ctrl Pts',(-0.373703802948097,1.97740164086689,
11.0466809756944));
#34872=CARTESIAN_POINT('Ctrl Pts',(-0.36719352192696,1.95755702962525,11.0477351076086));
#34873=CARTESIAN_POINT('Ctrl Pts',(-0.359106746809468,1.93825789928112,
11.0487892395229));
#34874=CARTESIAN_POINT('Ctrl Pts',(-0.349567488074763,1.91975721573084,
11.0498433714372));
#34875=CARTESIAN_POINT('Ctrl Pts',(-0.340028229340057,1.90125653218055,
11.0508975033515));
#34876=CARTESIAN_POINT('Ctrl Pts',(-0.329036932527729,1.8835548881979,11.0519516352657));
#34877=CARTESIAN_POINT('Ctrl Pts',(-0.316761350199374,1.86687527582886,
11.05300576718));
#34878=CARTESIAN_POINT('Ctrl Pts',(-0.304604191067691,1.85035657256891,
11.0540497298276));
#34879=CARTESIAN_POINT('Ctrl Pts',(-0.291115185860461,1.83474218185906,
11.0550936924751));
#34880=CARTESIAN_POINT('Ctrl Pts',(-0.276453987570692,1.82025353843835,
11.0561376551227));
#34881=CARTESIAN_POINT('Ctrl Pts',(-0.261819760135011,1.80579154843846,
11.0571796972884));
#34882=CARTESIAN_POINT('Ctrl Pts',(-0.246018095568352,1.79245174865092,
11.0582217394542));
#34883=CARTESIAN_POINT('Ctrl Pts',(-0.229248319187245,1.78042199989702,
11.05926378162));
#34884=CARTESIAN_POINT('Ctrl Pts',(-0.212496553282527,1.76840517090429,
11.0603047046488));
#34885=CARTESIAN_POINT('Ctrl Pts',(-0.194779317661103,1.75769604996397,
11.0613456276777));
#34886=CARTESIAN_POINT('Ctrl Pts',(-0.17632820866795,1.7484416793362,11.0623865507065));
#34887=CARTESIAN_POINT('Ctrl Pts',(-0.157867623666118,1.73918255590487,
11.0634280083263));
#34888=CARTESIAN_POINT('Ctrl Pts',(-0.138673062795551,1.73138001964964,
11.0644694659461));
#34889=CARTESIAN_POINT('Ctrl Pts',(-0.119000310322095,1.725134936086,11.0655109235659));
#34890=CARTESIAN_POINT('Ctrl Pts',(-0.0993215469651018,1.71888794437708,
11.0665526993964));
#34891=CARTESIAN_POINT('Ctrl Pts',(-0.0791650127848176,1.71419954065486,
11.0675944752269));
#34892=CARTESIAN_POINT('Ctrl Pts',(-0.0588002884634068,1.7111203064229,
11.0686362510574));
#34893=CARTESIAN_POINT('Ctrl Pts',(-0.0383915453282304,1.70803441635627,
11.06968027871));
#34894=CARTESIAN_POINT('Ctrl Pts',(-0.0177744482470587,1.70656469231682,
11.0707243063626));
#34895=CARTESIAN_POINT('Ctrl Pts',(0.00277698199232742,1.70670980387122,
11.0717683340152));
#34896=CARTESIAN_POINT('Ctrl Pts',(0.0100457534851455,1.70676112792593,
11.0721375929111));
#34897=CARTESIAN_POINT('Ctrl Pts',(0.0173063387704855,1.70701398253939,
11.072506851807));
#34898=CARTESIAN_POINT('Ctrl Pts',(0.0245467996603237,1.70746675984519,
11.0728761107028));
#34899=CARTESIAN_POINT('Ctrl Pts',(0.0450169110224329,1.70874684436091,
11.0739200733504));
#34900=CARTESIAN_POINT('Ctrl Pts',(0.0654476125468863,1.71163628962611,
11.074964035998));
#34901=CARTESIAN_POINT('Ctrl Pts',(0.0855662948905743,1.71612072317107,
11.0760079986455));
#34902=CARTESIAN_POINT('Ctrl Pts',(0.105647966750178,1.72059690711731,11.0770500408113));
#34903=CARTESIAN_POINT('Ctrl Pts',(0.125418035800352,1.72666215494416,11.078092082977));
#34904=CARTESIAN_POINT('Ctrl Pts',(0.144610646903623,1.73425056281367,11.0791341251428));
#34905=CARTESIAN_POINT('Ctrl Pts',(0.163782645444069,1.74183082085234,11.0801750481717));
#34906=CARTESIAN_POINT('Ctrl Pts',(0.182377725842926,1.75093074911251,11.0812159712005));
#34907=CARTESIAN_POINT('Ctrl Pts',(0.20014688504895,1.76143521387303,11.0822568942294));
#34908=CARTESIAN_POINT('Ctrl Pts',(0.217925170032028,1.77194507345288,11.0832983518492));
#34909=CARTESIAN_POINT('Ctrl Pts',(0.234876044837998,1.78386055004182,11.084339809469));
#34910=CARTESIAN_POINT('Ctrl Pts',(0.250776239290656,1.79702117597556,11.0853812670887));
#34911=CARTESIAN_POINT('Ctrl Pts',(0.266681291945907,1.81018582305426,11.0864230429192));
#34912=CARTESIAN_POINT('Ctrl Pts',(0.281534481895788,1.82459588023449,11.0874648187497));
#34913=CARTESIAN_POINT('Ctrl Pts',(0.295147350412218,1.84005205993383,11.0885065945802));
#34914=CARTESIAN_POINT('Ctrl Pts',(0.308789643452868,1.85554164851633,11.0895506222328));
#34915=CARTESIAN_POINT('Ctrl Pts',(0.321185820917087,1.87208128469986,11.0905946498854));
#34916=CARTESIAN_POINT('Ctrl Pts',(0.33218866905337,1.88943984671227,11.091638677538));
#34917=CARTESIAN_POINT('Ctrl Pts',(0.336080232216586,1.89557934256437,11.0920079364339));
#34918=CARTESIAN_POINT('Ctrl Pts',(0.3397979135357,1.90182104743952,11.0923771953298));
#34919=CARTESIAN_POINT('Ctrl Pts',(0.343336602576712,1.90815405312835,11.0927464542256));
#34920=CARTESIAN_POINT('Ctrl Pts',(0.353341125748525,1.92605862214438,11.0937904168732));
#34921=CARTESIAN_POINT('Ctrl Pts',(0.361971136330359,1.9448012307163,11.0948343795207));
#34922=CARTESIAN_POINT('Ctrl Pts',(0.369091150588893,1.96414488394997,11.0958783421683));
#34923=CARTESIAN_POINT('Ctrl Pts',(0.376198066813973,1.98345295244912,11.0969203843341));
#34924=CARTESIAN_POINT('Ctrl Pts',(0.381800193445969,2.00335920871818,11.0979624264998));
#34925=CARTESIAN_POINT('Ctrl Pts',(0.385809031422191,2.0236044420593,11.0990044686656));
#34926=CARTESIAN_POINT('Ctrl Pts',(0.389813563969406,2.04382793233787,11.1000453916945));
#34927=CARTESIAN_POINT('Ctrl Pts',(0.392228034371326,2.06438896446323,11.1010863147233));
#34928=CARTESIAN_POINT('Ctrl Pts',(0.393014459271252,2.08501584824805,11.1021272377522));
#34929=CARTESIAN_POINT('Ctrl Pts',(0.393801288058509,2.10565332546277,11.103168695372));
#34930=CARTESIAN_POINT('Ctrl Pts',(0.392958356818582,2.12635598727122,11.1042101529918));
#34931=CARTESIAN_POINT('Ctrl Pts',(0.390499729456089,2.14684924006557,11.1052516106116));
#34932=CARTESIAN_POINT('Ctrl Pts',(0.388040350875748,2.16734875444209,11.1062933864421));
#34933=CARTESIAN_POINT('Ctrl Pts',(0.383964416895371,2.18763800681407,11.1073351622726));
#34934=CARTESIAN_POINT('Ctrl Pts',(0.378337475967636,2.20745065973943,11.1083769381031));
#34935=CARTESIAN_POINT('Ctrl Pts',(0.372698372279397,2.22730613816368,11.1094209657557));
#34936=CARTESIAN_POINT('Ctrl Pts',(0.365501824890359,2.24668227003993,11.1104649934083));
#34937=CARTESIAN_POINT('Ctrl Pts',(0.356862475660956,2.26533016501877,11.1115090210608));
#34938=CARTESIAN_POINT('Ctrl Pts',(0.353806851081012,2.2719256810407,11.1118782799567));
#34939=CARTESIAN_POINT('Ctrl Pts',(0.350571161940436,2.27843032168585,11.1122475388526));
#34940=CARTESIAN_POINT('Ctrl Pts',(0.347161813686725,2.28483388519896,11.1126167977484));
#34941=CARTESIAN_POINT('Ctrl Pts',(0.337522960650935,2.30293793413005,11.113660760396));
#34942=CARTESIAN_POINT('Ctrl Pts',(0.326435420451159,2.32033991421969,11.1147047230435));
#34943=CARTESIAN_POINT('Ctrl Pts',(0.314025122844744,2.33679761870075,11.1157486856911));
#34944=CARTESIAN_POINT('Ctrl Pts',(0.301637655318063,2.35322504746099,11.1167907278569));
#34945=CARTESIAN_POINT('Ctrl Pts',(0.287932651007697,2.36871103203746,11.1178327700226));
#34946=CARTESIAN_POINT('Ctrl Pts',(0.273080152767697,2.38304084539934,11.1188748121884));
#34947=CARTESIAN_POINT('Ctrl Pts',(0.258243605877466,2.3973552687668,11.1199157352173));
#34948=CARTESIAN_POINT('Ctrl Pts',(0.24226251838913,2.41051545691407,11.1209566582461));
#34949=CARTESIAN_POINT('Ctrl Pts',(0.225344771199342,2.42234240194724,11.121997581275));
#34950=CARTESIAN_POINT('Ctrl Pts',(0.208418335495539,2.43417542099113,11.1230390388948));
#34951=CARTESIAN_POINT('Ctrl Pts',(0.190554872867629,2.44467339422271,11.1240804965146));
#34952=CARTESIAN_POINT('Ctrl Pts',(0.17199287958319,2.45369950434328,11.1251219541343));
#34953=CARTESIAN_POINT('Ctrl Pts',(0.153425214800552,2.46272837233401,11.1261637299648));
#34954=CARTESIAN_POINT('Ctrl Pts',(0.134159271428605,2.4702841929787,11.1272055057953));
#34955=CARTESIAN_POINT('Ctrl Pts',(0.114454473319069,2.47627790732018,11.1282472816258));
#34956=CARTESIAN_POINT('Ctrl Pts',(0.0947070828412857,2.48228457721121,
11.1292913092784));
#34957=CARTESIAN_POINT('Ctrl Pts',(0.0745196631070063,2.48672224160587,
11.130335336931));
#34958=CARTESIAN_POINT('Ctrl Pts',(0.054163543288737,2.4895525645897,11.1313793645836));
#34959=CARTESIAN_POINT('Ctrl Pts',(0.0469638505320102,2.4905536127299,11.1317486234795));
#34960=CARTESIAN_POINT('Ctrl Pts',(0.039743095218919,2.49135406688011,11.1321178823754));
#34961=CARTESIAN_POINT('Ctrl Pts',(0.0325133225523991,2.49195379046082,
11.1324871412712));
#34962=CARTESIAN_POINT('Ctrl Pts',(0.0120734287579877,2.4936493190564,11.1335311039188));
#34963=CARTESIAN_POINT('Ctrl Pts',(-0.00856035352241005,2.49374672299721,
11.1345750665663));
#34964=CARTESIAN_POINT('Ctrl Pts',(-0.0291162044493577,2.49222077537844,
11.1356190292139));
#34965=CARTESIAN_POINT('Ctrl Pts',(-0.0496342406735042,2.49069763490475,
11.1366610713797));
#34966=CARTESIAN_POINT('Ctrl Pts',(-0.0700739002393444,2.48755706516615,
11.1377031135454));
#34967=CARTESIAN_POINT('Ctrl Pts',(-0.0901625895454327,2.48282580561721,
11.1387451557112));
#34968=CARTESIAN_POINT('Ctrl Pts',(-0.11022970391479,2.47809962736669,11.1397860787401));
#34969=CARTESIAN_POINT('Ctrl Pts',(-0.129945877151433,2.47178629050859,
11.1408270017689));
#34970=CARTESIAN_POINT('Ctrl Pts',(-0.149048066527609,2.46396368481537,
11.1418679247978));
#34971=CARTESIAN_POINT('Ctrl Pts',(-0.168160066290393,2.45613706163574,
11.1429093824176));
#34972=CARTESIAN_POINT('Ctrl Pts',(-0.186656765236036,2.44679988502048,
11.1439508400374));
#34973=CARTESIAN_POINT('Ctrl Pts',(-0.204294022591169,2.43607862522558,
11.1449922976571));
#34974=CARTESIAN_POINT('Ctrl Pts',(-0.221936668897339,2.42535408961841,
11.1460340734876));
#34975=CARTESIAN_POINT('Ctrl Pts',(-0.238718741438448,2.41324504172642,
11.1470758493181));
#34976=CARTESIAN_POINT('Ctrl Pts',(-0.254424927030318,2.39992140054624,
11.1481176251486));
#34977=CARTESIAN_POINT('Ctrl Pts',(-0.270165061898765,2.38656896001329,
11.1491616528012));
#34978=CARTESIAN_POINT('Ctrl Pts',(-0.284824144641143,2.37199720397771,
11.1502056804538));
#34979=CARTESIAN_POINT('Ctrl Pts',(-0.29822306635052,2.35641351894253,11.1512497081064));
#34980=CARTESIAN_POINT('Ctrl Pts',(-0.302962089329329,2.35090177381274,
11.1516189670023));
#34981=CARTESIAN_POINT('Ctrl Pts',(-0.307543850832177,2.34526373375715,
11.1519882258981));
#34982=CARTESIAN_POINT('Ctrl Pts',(-0.311961715734576,2.33950945266511,
11.152357484794));
#34983=CARTESIAN_POINT('Ctrl Pts',(-0.324948951561612,2.32259354255731,
11.1534429983775));
#34984=CARTESIAN_POINT('Ctrl Pts',(-0.336597542900089,2.30456456151901,
11.1545285119611));
#34985=CARTESIAN_POINT('Ctrl Pts',(-0.346718674991621,2.28566381018404,
11.1556140255446));
#34986=CARTESIAN_POINT('Ctrl Pts',(-0.356448637914021,2.267493549384,11.156657585378));
#34987=CARTESIAN_POINT('Ctrl Pts',(-0.364766744947935,2.24851841758935,
11.1577011452115));
#34988=CARTESIAN_POINT('Ctrl Pts',(-0.371548357285401,2.22898336403785,
11.1587447050449));
#34989=CARTESIAN_POINT('Ctrl Pts',(-0.378321739649224,2.20947201767689,
11.1597869984435));
#34990=CARTESIAN_POINT('Ctrl Pts',(-0.383562061465708,2.18940277634239,
11.1608292918422));
#34991=CARTESIAN_POINT('Ctrl Pts',(-0.387192915306281,2.16904010672517,
11.1618715852408));
#34992=CARTESIAN_POINT('Ctrl Pts',(-0.390822952250089,2.14868201845429,
11.1629136441364));
#34993=CARTESIAN_POINT('Ctrl Pts',(-0.392844102813498,2.12803135043112,
11.1639557030321));
#34994=CARTESIAN_POINT('Ctrl Pts',(-0.393231083751943,2.10736238896501,
11.1649977619277));
#34995=CARTESIAN_POINT('Ctrl Pts',(-0.393278851517683,2.10481107438773,
11.1651263905506));
#34996=CARTESIAN_POINT('Ctrl Pts',(-0.393301785008165,2.10225948554673,
11.1652550191736));
#34997=CARTESIAN_POINT('Ctrl Pts',(-0.393299891708585,2.09970814041908,
11.1653836477965));
#34998=CARTESIAN_POINT('',(-0.393441883900895,2.09987214517031,11.2903836477965));
#34999=CARTESIAN_POINT('Ctrl Pts',(-0.393299891708519,2.09970814032956,
11.165383647801));
#35000=CARTESIAN_POINT('Ctrl Pts',(-0.393282117129534,2.07575573889103,
11.1665912321375));
#35001=CARTESIAN_POINT('Ctrl Pts',(-0.391072133920177,2.05189347906682,
11.1677988164739));
#35002=CARTESIAN_POINT('Ctrl Pts',(-0.386743192868008,2.02848361886771,
11.1690064008103));
#35003=CARTESIAN_POINT('Ctrl Pts',(-0.382893808230515,2.0076670831075,11.1700802099791));
#35004=CARTESIAN_POINT('Ctrl Pts',(-0.377369766906101,1.98720811105829,
11.1711540191479));
#35005=CARTESIAN_POINT('Ctrl Pts',(-0.370254349587689,1.96734779831681,
11.1722278283167));
#35006=CARTESIAN_POINT('Ctrl Pts',(-0.363336705263321,1.94803950288335,
11.1732717909643));
#35007=CARTESIAN_POINT('Ctrl Pts',(-0.35488402826661,1.92921625368693,11.1743157536118));
#35008=CARTESIAN_POINT('Ctrl Pts',(-0.344985874235674,1.91113593095073,
11.1753597162594));
#35009=CARTESIAN_POINT('Ctrl Pts',(-0.335105928925666,1.89308886891648,
11.1764017584251));
#35010=CARTESIAN_POINT('Ctrl Pts',(-0.32378608197909,1.8757826871725,11.1774438005909));
#35011=CARTESIAN_POINT('Ctrl Pts',(-0.31116351430148,1.85945445884916,11.1784858427567));
#35012=CARTESIAN_POINT('Ctrl Pts',(-0.298554503063261,1.84314376678652,
11.1795267657855));
#35013=CARTESIAN_POINT('Ctrl Pts',(-0.284645973490244,1.82780953989057,
11.1805676888144));
#35014=CARTESIAN_POINT('Ctrl Pts',(-0.269617715035238,1.81365898348442,
11.1816086118432));
#35015=CARTESIAN_POINT('Ctrl Pts',(-0.254581738458369,1.7995011597213,11.182650069463));
#35016=CARTESIAN_POINT('Ctrl Pts',(-0.238425408781422,1.78652873703318,
11.1836915270828));
#35017=CARTESIAN_POINT('Ctrl Pts',(-0.221364913809522,1.77491160443027,
11.1847329847026));
#35018=CARTESIAN_POINT('Ctrl Pts',(-0.204299206112636,1.76329092228688,
11.1857747605331));
#35019=CARTESIAN_POINT('Ctrl Pts',(-0.186329411169498,1.75302673847489,
11.1868165363636));
#35020=CARTESIAN_POINT('Ctrl Pts',(-0.167699335001218,1.74424471467011,
11.1878583121941));
#35021=CARTESIAN_POINT('Ctrl Pts',(-0.149028989500528,1.73544370832159,
11.1889023398467));
#35022=CARTESIAN_POINT('Ctrl Pts',(-0.129696202265947,1.72813151859826,
11.1899463674993));
#35023=CARTESIAN_POINT('Ctrl Pts',(-0.10996389924166,1.72238534077241,11.1909903951519));
#35024=CARTESIAN_POINT('Ctrl Pts',(-0.10298484230805,1.72035299299486,11.1913596540478));
#35025=CARTESIAN_POINT('Ctrl Pts',(-0.0959559174314416,1.71851608003603,
11.1917289129437));
#35026=CARTESIAN_POINT('Ctrl Pts',(-0.0888890232722175,1.7168764800463,
11.1920981718396));
#35027=CARTESIAN_POINT('Ctrl Pts',(-0.0689096169019349,1.7122410300535,
11.1931421344871));
#35028=CARTESIAN_POINT('Ctrl Pts',(-0.0485071051703846,1.70915882730775,
11.1941860971347));
#35029=CARTESIAN_POINT('Ctrl Pts',(-0.0279467964714988,1.70769416704951,
11.1952300597822));
#35030=CARTESIAN_POINT('Ctrl Pts',(-0.00742431067596596,1.70623220119164,
11.196272101948));
#35031=CARTESIAN_POINT('Ctrl Pts',(0.0132546744797402,1.70638198229833,
11.1973141441138));
#35032=CARTESIAN_POINT('Ctrl Pts',(0.033816565160104,1.70815649817718,11.1983561862795));
#35033=CARTESIAN_POINT('Ctrl Pts',(0.0543563726929092,1.70992910825385,
11.1993971093084));
#35034=CARTESIAN_POINT('Ctrl Pts',(0.0747786035859954,1.71332295485183,
11.2004380323372));
#35035=CARTESIAN_POINT('Ctrl Pts',(0.0948117126143965,1.71829903176554,
11.2014789553661));
#35036=CARTESIAN_POINT('Ctrl Pts',(0.114855110125461,1.72327766426266,11.2025204129859));
#35037=CARTESIAN_POINT('Ctrl Pts',(0.13450826856536,1.7298399887263,11.2035618706057));
#35038=CARTESIAN_POINT('Ctrl Pts',(0.153511315847371,1.73789619457011,11.2046033282255));
#35039=CARTESIAN_POINT('Ctrl Pts',(0.172520169388787,1.74595486193603,11.205645104056));
#35040=CARTESIAN_POINT('Ctrl Pts',(0.19087785360811,1.75550799910288,11.2066868798864));
#35041=CARTESIAN_POINT('Ctrl Pts',(0.208346733313902,1.76641863253859,11.2077286557169));
#35042=CARTESIAN_POINT('Ctrl Pts',(0.225853372399599,1.77735284955607,11.2087726833695));
#35043=CARTESIAN_POINT('Ctrl Pts',(0.242466779490609,1.78964998278444,11.2098167110221));
#35044=CARTESIAN_POINT('Ctrl Pts',(0.257979720855493,1.80313074657802,11.2108607386747));
#35045=CARTESIAN_POINT('Ctrl Pts',(0.263466444876461,1.8078987160293,11.2112299975706));
#35046=CARTESIAN_POINT('Ctrl Pts',(0.268815838221317,1.81281440773856,11.2115992564665));
#35047=CARTESIAN_POINT('Ctrl Pts',(0.274019880747731,1.81786883377585,11.2119685153623));
#35048=CARTESIAN_POINT('Ctrl Pts',(0.288732663769763,1.83215862353258,11.2130124780099));
#35049=CARTESIAN_POINT('Ctrl Pts',(0.302368483273617,1.84764496865274,11.2140564406574));
#35050=CARTESIAN_POINT('Ctrl Pts',(0.3147296624425,1.86413959726391,11.215100403305));
#35051=CARTESIAN_POINT('Ctrl Pts',(0.327068101890308,1.88060388222836,11.2161424454707));
#35052=CARTESIAN_POINT('Ctrl Pts',(0.338136071564399,1.8980722224112,11.2171844876365));
#35053=CARTESIAN_POINT('Ctrl Pts',(0.347774549796921,1.91632160575193,11.2182265298023));
#35054=CARTESIAN_POINT('Ctrl Pts',(0.357402676455242,1.93455138954165,11.2192674528311));
#35055=CARTESIAN_POINT('Ctrl Pts',(0.365603992059651,1.95355991741043,11.22030837586));
#35056=CARTESIAN_POINT('Ctrl Pts',(0.37226430138939,1.97309775450738,11.2213492988889));
#35057=CARTESIAN_POINT('Ctrl Pts',(0.378928031280413,1.99264562572825,11.2223907565087));
#35058=CARTESIAN_POINT('Ctrl Pts',(0.384048921150567,2.01272265802806,11.2234322141284));
#35059=CARTESIAN_POINT('Ctrl Pts',(0.387561811892712,2.0330617302103,11.2244736717482));
#35060=CARTESIAN_POINT('Ctrl Pts',(0.391075775976127,2.0534070168658,11.2255154475787));
#35061=CARTESIAN_POINT('Ctrl Pts',(0.392980673373426,2.07401377220309,11.2265572234092));
#35062=CARTESIAN_POINT('Ctrl Pts',(0.393263037659875,2.09460804205064,11.2275989992397));
#35063=CARTESIAN_POINT('Ctrl Pts',(0.393546012283137,2.11524682687982,11.2286430268923));
#35064=CARTESIAN_POINT('Ctrl Pts',(0.392199499935705,2.13587233742638,11.2296870545449));
#35065=CARTESIAN_POINT('Ctrl Pts',(0.389262067835153,2.15621327729906,11.2307310821975));
#35066=CARTESIAN_POINT('Ctrl Pts',(0.388223136604324,2.16340760110799,11.2311003410934));
#35067=CARTESIAN_POINT('Ctrl Pts',(0.386985658277728,2.17056641955304,11.2314695999893));
#35068=CARTESIAN_POINT('Ctrl Pts',(0.385552848619826,2.17767812382607,11.2318388588851));
#35069=CARTESIAN_POINT('Ctrl Pts',(0.381502032835427,2.19778421660975,11.2328828215327));
#35070=CARTESIAN_POINT('Ctrl Pts',(0.375862152065989,2.21763249622357,11.2339267841802));
#35071=CARTESIAN_POINT('Ctrl Pts',(0.368684502639998,2.23695483749433,11.2349707468278));
#35072=CARTESIAN_POINT('Ctrl Pts',(0.361520057273563,2.25624163323621,11.2360127889936));
#35073=CARTESIAN_POINT('Ctrl Pts',(0.352823656058063,2.27500370847721,11.2370548311593));
#35074=CARTESIAN_POINT('Ctrl Pts',(0.342696730224722,2.29298663449391,11.2380968733251));
#35075=CARTESIAN_POINT('Ctrl Pts',(0.332580680550633,2.31095024713056,11.239137796354));
#35076=CARTESIAN_POINT('Ctrl Pts',(0.321037490307621,2.32813571972793,11.2401787193828));
#35077=CARTESIAN_POINT('Ctrl Pts',(0.308215072847903,2.344312011308,11.2412196424117));
#35078=CARTESIAN_POINT('Ctrl Pts',(0.29538607012877,2.36049661060983,11.2422611000315));
#35079=CARTESIAN_POINT('Ctrl Pts',(0.281276972119512,2.37567040685188,11.2433025576513));
#35080=CARTESIAN_POINT('Ctrl Pts',(0.266077107302757,2.38963401555998,11.2443440152711));
#35081=CARTESIAN_POINT('Ctrl Pts',(0.25087259826464,2.4036018907593,11.2453857911015));
#35082=CARTESIAN_POINT('Ctrl Pts',(0.234577224806245,2.41635837160149,11.246427566932));
#35083=CARTESIAN_POINT('Ctrl Pts',(0.217414042880951,2.42774383893242,11.2474693427625));
#35084=CARTESIAN_POINT('Ctrl Pts',(0.200213762348447,2.43915391620935,11.2485133704151));
#35085=CARTESIAN_POINT('Ctrl Pts',(0.182142572330235,2.44918670605734,11.2495573980677));
#35086=CARTESIAN_POINT('Ctrl Pts',(0.163449460821231,2.45772777884482,11.2506014257203));
#35087=CARTESIAN_POINT('Ctrl Pts',(0.156837952305214,2.46074864433547,11.2509706846162));
#35088=CARTESIAN_POINT('Ctrl Pts',(0.150148820204391,2.46358334817812,11.2513399435121));
#35089=CARTESIAN_POINT('Ctrl Pts',(0.143393566163912,2.46622831018751,11.2517092024079));
#35090=CARTESIAN_POINT('Ctrl Pts',(0.124295223586484,2.47370610306648,11.2527531650555));
#35091=CARTESIAN_POINT('Ctrl Pts',(0.104553465349265,2.47970822272757,11.253797127703));
#35092=CARTESIAN_POINT('Ctrl Pts',(0.084421503527998,2.48413265904121,11.2548410903506));
#35093=CARTESIAN_POINT('Ctrl Pts',(0.0643265766198458,2.4885489561275,11.2558831325164));
#35094=CARTESIAN_POINT('Ctrl Pts',(0.0438435687218423,2.49139311661894,
11.2569251746821));
#35095=CARTESIAN_POINT('Ctrl Pts',(0.0232413146182522,2.49261269884559,
11.2579672168479));
#35096=CARTESIAN_POINT('Ctrl Pts',(0.00266118701191055,2.49383097126008,
11.2590081398768));
#35097=CARTESIAN_POINT('Ctrl Pts',(-0.0180372034940253,2.49342805706877,
11.2600490629056));
#35098=CARTESIAN_POINT('Ctrl Pts',(-0.0385795253384346,2.49140325781048,
11.2610899859345));
#35099=CARTESIAN_POINT('Ctrl Pts',(-0.059132397183938,2.48937741866807,
11.2621314435543));
#35100=CARTESIAN_POINT('Ctrl Pts',(-0.0795283064293706,2.48572808652609,
11.2631729011741));
#35101=CARTESIAN_POINT('Ctrl Pts',(-0.0994971201104013,2.48050652174403,
11.2642143587939));
#35102=CARTESIAN_POINT('Ctrl Pts',(-0.119472035134574,2.47528336154628,
11.2652561346244));
#35103=CARTESIAN_POINT('Ctrl Pts',(-0.139018892715362,2.46848723335869,
11.2662979104549));
#35104=CARTESIAN_POINT('Ctrl Pts',(-0.157882737992171,2.46021928188826,
11.2673396862854));
#35105=CARTESIAN_POINT('Ctrl Pts',(-0.176787357898624,2.45193345905311,
11.268383713938));
#35106=CARTESIAN_POINT('Ctrl Pts',(-0.195005368916282,2.44216980935798,
11.2694277415906));
#35107=CARTESIAN_POINT('Ctrl Pts',(-0.212305774861567,2.4310757435398,11.2704717692432));
#35108=CARTESIAN_POINT('Ctrl Pts',(-0.218424701674887,2.42715191787823,
11.270841028139));
#35109=CARTESIAN_POINT('Ctrl Pts',(-0.224429119490491,2.42306205225298,
11.2712102870349));
#35110=CARTESIAN_POINT('Ctrl Pts',(-0.230309791976158,2.41881387943422,
11.2715795459307));
#35111=CARTESIAN_POINT('Ctrl Pts',(-0.246801243074373,2.4069005252272,11.2726150763124));
#35112=CARTESIAN_POINT('Ctrl Pts',(-0.262418861882085,2.39366574277209,
11.2736506066941));
#35113=CARTESIAN_POINT('Ctrl Pts',(-0.276941775913723,2.37926357219257,
11.2746861370758));
#35114=CARTESIAN_POINT('Ctrl Pts',(-0.291437973362016,2.36488789607482,
11.2757197624794));
#35115=CARTESIAN_POINT('Ctrl Pts',(-0.304842892466673,2.34934956990205,
11.2767533878829));
#35116=CARTESIAN_POINT('Ctrl Pts',(-0.316968640225888,2.33284280343904,
11.2777870132865));
#35117=CARTESIAN_POINT('Ctrl Pts',(-0.329283192815779,2.31607901717742,
11.278836732829));
#35118=CARTESIAN_POINT('Ctrl Pts',(-0.340277802284048,2.29831690485719,
11.2798864523715));
#35119=CARTESIAN_POINT('Ctrl Pts',(-0.349797924201985,2.27979516740998,
11.280936171914));
#35120=CARTESIAN_POINT('Ctrl Pts',(-0.359166996768876,2.26156730187384,
11.2819692362648));
#35121=CARTESIAN_POINT('Ctrl Pts',(-0.367107770865079,2.24260447085751,
11.2830023006156));
#35122=CARTESIAN_POINT('Ctrl Pts',(-0.373519603111344,2.22315841867913,
11.2840353649664));
#35123=CARTESIAN_POINT('Ctrl Pts',(-0.380086493890814,2.20324209899973,
11.2850934121047));
#35124=CARTESIAN_POINT('Ctrl Pts',(-0.385049188178705,2.18281963576225,
11.2861514592431));
#35125=CARTESIAN_POINT('Ctrl Pts',(-0.388354250310891,2.1621760907863,11.2872095063814));
#35126=CARTESIAN_POINT('Ctrl Pts',(-0.391659312443079,2.14153254581033,
11.2882675535198));
#35127=CARTESIAN_POINT('Ctrl Pts',(-0.393306737388483,2.12066875645485,
11.2893256006581));
#35128=CARTESIAN_POINT('Ctrl Pts',(-0.393299979233323,2.09987219128435,
11.2903836477965));
#35129=CARTESIAN_POINT('',(-0.393299833502872,2.10036189309685,11.4153836477965));
#35130=CARTESIAN_POINT('Ctrl Pts',(-0.393899443331936,2.09987199647952,
11.2903836477965));
#35131=CARTESIAN_POINT('Ctrl Pts',(-0.393929117802885,2.09287546046937,
11.2907390616822));
#35132=CARTESIAN_POINT('Ctrl Pts',(-0.39375888735456,2.08588039805356,11.2910944755679));
#35133=CARTESIAN_POINT('Ctrl Pts',(-0.386401867339676,1.94874160309987,
11.2980733372944));
#35134=CARTESIAN_POINT('Ctrl Pts',(-0.230433513831742,1.69605020585767,
11.3113202329764));
#35135=CARTESIAN_POINT('Ctrl Pts',(0.214910394680641,1.68758205332127,11.3311905764991));
#35136=CARTESIAN_POINT('Ctrl Pts',(0.463103273481829,2.05745122122909,11.3510609200219));
#35137=CARTESIAN_POINT('Ctrl Pts',(0.286461944681156,2.46635310116605,11.3709312635446));
#35138=CARTESIAN_POINT('Ctrl Pts',(-0.152969220092249,2.53917588525426,
11.3908016070675));
#35139=CARTESIAN_POINT('Ctrl Pts',(-0.376012290477261,2.29304678368391,
11.4056190660244));
#35140=CARTESIAN_POINT('Ctrl Pts',(-0.393569766291279,2.13140534042234,
11.4138130771406));
#35141=CARTESIAN_POINT('Ctrl Pts',(-0.393284377485805,2.10036202476101,
11.4153836404157));
#35142=CARTESIAN_POINT('',(-0.39306000785858,2.09993937222327,11.5403836637865));
#35143=CARTESIAN_POINT('Ctrl Pts',(-0.393299833502872,2.10036189309685,
11.4153836477965));
#35144=CARTESIAN_POINT('Ctrl Pts',(-0.393318545155974,2.08002635723286,
11.4164124453626));
#35145=CARTESIAN_POINT('Ctrl Pts',(-0.39175578397594,2.05964716809563,11.4174412429287));
#35146=CARTESIAN_POINT('Ctrl Pts',(-0.388617730630256,2.03949256706991,
11.4184700404948));
#35147=CARTESIAN_POINT('Ctrl Pts',(-0.385479911390416,2.0193394696228,11.4194987613102));
#35148=CARTESIAN_POINT('Ctrl Pts',(-0.380767098308162,1.99941168018583,
11.4205274821257));
#35149=CARTESIAN_POINT('Ctrl Pts',(-0.374537338097605,1.97997220167494,
11.4215562029412));
#35150=CARTESIAN_POINT('Ctrl Pts',(-0.368308813458114,1.96053657866674,
11.4225847197267));
#35151=CARTESIAN_POINT('Ctrl Pts',(-0.360564182220411,1.94158979100163,
11.4236132365122));
#35152=CARTESIAN_POINT('Ctrl Pts',(-0.351411029419831,1.92337843166223,
11.4246417532978));
#35153=CARTESIAN_POINT('Ctrl Pts',(-0.342236955454333,1.90512544700962,
11.425672620942));
#35154=CARTESIAN_POINT('Ctrl Pts',(-0.331648297244273,1.88761191302799,
11.4267034885863));
#35155=CARTESIAN_POINT('Ctrl Pts',(-0.319798523303929,1.87105940837714,
11.4277343562306));
#35156=CARTESIAN_POINT('Ctrl Pts',(-0.309039486379814,1.85603051334321,
11.4286703355247));
#35157=CARTESIAN_POINT('Ctrl Pts',(-0.297241658399242,1.84179382727624,
11.4296063148189));
#35158=CARTESIAN_POINT('Ctrl Pts',(-0.284547292283978,1.82848991095384,
11.430542294113));
#35159=CARTESIAN_POINT('Ctrl Pts',(-0.270388384986038,1.81365113001762,
11.4315862567606));
#35160=CARTESIAN_POINT('Ctrl Pts',(-0.255023429813726,1.79987867158512,
11.4326302194081));
#35161=CARTESIAN_POINT('Ctrl Pts',(-0.238638940285526,1.78737187237966,
11.4336741820557));
#35162=CARTESIAN_POINT('Ctrl Pts',(-0.222284591791345,1.77488808077901,
11.4347162242214));
#35163=CARTESIAN_POINT('Ctrl Pts',(-0.204914973989729,1.76366581546066,
11.4357582663872));
#35164=CARTESIAN_POINT('Ctrl Pts',(-0.186751681621276,1.75386606723462,
11.436800308553));
#35165=CARTESIAN_POINT('Ctrl Pts',(-0.168607896343485,1.74407684378423,
11.4378412315818));
#35166=CARTESIAN_POINT('Ctrl Pts',(-0.149672759229649,1.73570747750828,
11.4388821546107));
#35167=CARTESIAN_POINT('Ctrl Pts',(-0.130194683834731,1.72887436857423,
11.4399230776396));
#35168=CARTESIAN_POINT('Ctrl Pts',(-0.11070660500795,1.72203775033353,11.4409645352593));
#35169=CARTESIAN_POINT('Ctrl Pts',(-0.0906757198006848,1.71673922442125,
11.4420059928791));
#35170=CARTESIAN_POINT('Ctrl Pts',(-0.070368561768369,1.71304631347582,
11.4430474504989));
#35171=CARTESIAN_POINT('Ctrl Pts',(-0.050055199013961,1.70935227418511,
11.4440892263294));
#35172=CARTESIAN_POINT('Ctrl Pts',(-0.029466125156578,1.70726492243702,
11.4451310021599));
#35173=CARTESIAN_POINT('Ctrl Pts',(-0.00887516433844985,1.70680015074015,
11.4461727779904));
#35174=CARTESIAN_POINT('Ctrl Pts',(0.0117603043087581,1.70633437442872,
11.447216805643));
#35175=CARTESIAN_POINT('Ctrl Pts',(0.0323969327501948,1.70749813874247,
11.4482608332956));
#35176=CARTESIAN_POINT('Ctrl Pts',(0.0527630936196593,1.71025528104709,
11.4493048609482));
#35177=CARTESIAN_POINT('Ctrl Pts',(0.0599663377646051,1.7112304461403,11.4496741198441));
#35178=CARTESIAN_POINT('Ctrl Pts',(0.0671358366151855,1.71240446503712,
11.45004337874));
#35179=CARTESIAN_POINT('Ctrl Pts',(0.0742599533342948,1.71377422492694,
11.4504126376358));
#35180=CARTESIAN_POINT('Ctrl Pts',(0.0944011383803014,1.71764678744903,
11.4514566002834));
#35181=CARTESIAN_POINT('Ctrl Pts',(0.11429859587963,1.72311063625593,11.4525005629309));
#35182=CARTESIAN_POINT('Ctrl Pts',(0.133683756808683,1.73011685201199,11.4535445255785));
#35183=CARTESIAN_POINT('Ctrl Pts',(0.153033256645336,1.73711017907921,11.4545865677443));
#35184=CARTESIAN_POINT('Ctrl Pts',(0.171871626217857,1.74564004972883,11.45562860991));
#35185=CARTESIAN_POINT('Ctrl Pts',(0.189943548333678,1.75560729036983,11.4566706520758));
#35186=CARTESIAN_POINT('Ctrl Pts',(0.20799606148904,1.76556382635095,11.4577115751047));
#35187=CARTESIAN_POINT('Ctrl Pts',(0.225283106358137,1.77695433946821,11.4587524981335));
#35188=CARTESIAN_POINT('Ctrl Pts',(0.241572340850244,1.78963296867075,11.4597934211624));
#35189=CARTESIAN_POINT('Ctrl Pts',(0.257869941068643,1.80231810928681,11.4608348787822));
#35190=CARTESIAN_POINT('Ctrl Pts',(0.273168116620351,1.81629224839513,11.461876336402));
#35191=CARTESIAN_POINT('Ctrl Pts',(0.287265813832512,1.83136783103443,11.4629177940217));
#35192=CARTESIAN_POINT('Ctrl Pts',(0.301367818505782,1.84644801992148,11.4639595698522));
#35193=CARTESIAN_POINT('Ctrl Pts',(0.314268138928285,1.86262976063816,11.4650013456827));
#35194=CARTESIAN_POINT('Ctrl Pts',(0.325805186438368,1.87969141984512,11.4660431215132));
#35195=CARTESIAN_POINT('Ctrl Pts',(0.33736717153845,1.89678995821562,11.4670871491658));
#35196=CARTESIAN_POINT('Ctrl Pts',(0.347559637522531,1.91477157154622,11.4681311768184));
#35197=CARTESIAN_POINT('Ctrl Pts',(0.356265953779684,1.93338829519673,11.469175204471));
#35198=CARTESIAN_POINT('Ctrl Pts',(0.359345263719599,1.9399727863285,11.4695444633669));
#35199=CARTESIAN_POINT('Ctrl Pts',(0.362239106883503,1.94663654696954,11.4699137222628));
#35200=CARTESIAN_POINT('Ctrl Pts',(0.364943801348106,1.95336810763823,11.4702829811586));
#35201=CARTESIAN_POINT('Ctrl Pts',(0.372590468837211,1.9723994647064,11.4713269438062));
#35202=CARTESIAN_POINT('Ctrl Pts',(0.378767220202153,1.99208728330822,11.4723709064537));
#35203=CARTESIAN_POINT('Ctrl Pts',(0.383369806431004,2.01217926487979,11.4734148691013));
#35204=CARTESIAN_POINT('Ctrl Pts',(0.38796392570653,2.03223428508622,11.4744569112671));
#35205=CARTESIAN_POINT('Ctrl Pts',(0.390989407579595,2.05269129661982,11.4754989534328));
#35206=CARTESIAN_POINT('Ctrl Pts',(0.392391431171545,2.07328193975703,11.4765409955986));
#35207=CARTESIAN_POINT('Ctrl Pts',(0.393791949012181,2.09385046886697,11.4775819186275));
#35208=CARTESIAN_POINT('Ctrl Pts',(0.393572391387792,2.1145516162707,11.4786228416563));
#35209=CARTESIAN_POINT('Ctrl Pts',(0.391729629909612,2.13511106735601,11.4796637646852));
#35210=CARTESIAN_POINT('Ctrl Pts',(0.389885922037165,2.15568107723956,11.480705222305));
#35211=CARTESIAN_POINT('Ctrl Pts',(0.386417394523157,2.17610851114386,11.4817466799248));
#35212=CARTESIAN_POINT('Ctrl Pts',(0.38137291295117,2.19612279265158,11.4827881375445));
#35213=CARTESIAN_POINT('Ctrl Pts',(0.376326890070137,2.21614318939487,11.4838299133751));
#35214=CARTESIAN_POINT('Ctrl Pts',(0.369704169290134,2.23574947841387,11.4848716892055));
#35215=CARTESIAN_POINT('Ctrl Pts',(0.361603633028839,2.25468581893743,11.485913465036));
#35216=CARTESIAN_POINT('Ctrl Pts',(0.353485587274598,2.27366309079075,11.4869574926886));
#35217=CARTESIAN_POINT('Ctrl Pts',(0.343883690839864,2.29196687088298,11.4880015203412));
#35218=CARTESIAN_POINT('Ctrl Pts',(0.332943302576687,2.30936486636809,11.4890455479938));
#35219=CARTESIAN_POINT('Ctrl Pts',(0.329073830651941,2.3155183093225,11.4894148068897));
#35220=CARTESIAN_POINT('Ctrl Pts',(0.32503731098751,2.32155871850864,11.4897840657856));
#35221=CARTESIAN_POINT('Ctrl Pts',(0.320841394237289,2.32747678946185,11.4901533246814));
#35222=CARTESIAN_POINT('Ctrl Pts',(0.308978767748014,2.34420826185136,11.491197287329));
#35223=CARTESIAN_POINT('Ctrl Pts',(0.295768484490001,2.36005915693541,11.4922412499765));
#35224=CARTESIAN_POINT('Ctrl Pts',(0.281366249739214,2.37480524650685,11.4932852126241));
#35225=CARTESIAN_POINT('Ctrl Pts',(0.266990509451176,2.38952420905755,11.4943272547899));
#35226=CARTESIAN_POINT('Ctrl Pts',(0.251427635888406,2.4031418383637,11.4953692969556));
#35227=CARTESIAN_POINT('Ctrl Pts',(0.234873595179144,2.41546677208166,11.4964113391214));
#35228=CARTESIAN_POINT('Ctrl Pts',(0.218337333249554,2.42777846901443,11.4974522621503));
#35229=CARTESIAN_POINT('Ctrl Pts',(0.200812587361982,2.43879976616843,11.4984931851791));
#35230=CARTESIAN_POINT('Ctrl Pts',(0.182528312700421,2.44837954168225,11.499534108208));
#35231=CARTESIAN_POINT('Ctrl Pts',(0.164234647711941,2.4579642371191,11.5005755658278));
#35232=CARTESIAN_POINT('Ctrl Pts',(0.145181318928943,2.46610557615619,11.5016170234476));
#35233=CARTESIAN_POINT('Ctrl Pts',(0.125622283670958,2.47269817794738,11.5026584810673));
#35234=CARTESIAN_POINT('Ctrl Pts',(0.106057272275004,2.47929279406582,11.5037002568978));
#35235=CARTESIAN_POINT('Ctrl Pts',(0.0859869550061474,2.4843375303674,11.5047420327283));
#35236=CARTESIAN_POINT('Ctrl Pts',(0.0656799742048062,2.48777703772717,
11.5057838085588));
#35237=CARTESIAN_POINT('Ctrl Pts',(0.0453290994036211,2.49122397966014,
11.5068278362114));
#35238=CARTESIAN_POINT('Ctrl Pts',(0.024741273348776,2.49305870011403,11.507871863864));
#35239=CARTESIAN_POINT('Ctrl Pts',(0.00419049739736034,2.49327767509937,
11.5089158915166));
#35240=CARTESIAN_POINT('Ctrl Pts',(-0.00307804268214043,2.49335512368141,
11.5092851504125));
#35241=CARTESIAN_POINT('Ctrl Pts',(-0.010341967905338,2.49323092831189,
11.5096544093084));
#35242=CARTESIAN_POINT('Ctrl Pts',(-0.01758931347456,2.49290648512272,11.5100236682042));
#35243=CARTESIAN_POINT('Ctrl Pts',(-0.0380788890890574,2.49198922470049,
11.5110676308518));
#35244=CARTESIAN_POINT('Ctrl Pts',(-0.0585575704984534,2.48946215793166,
11.5121115934993));
#35245=CARTESIAN_POINT('Ctrl Pts',(-0.0787525365322312,2.48533482582001,
11.5131555561469));
#35246=CARTESIAN_POINT('Ctrl Pts',(-0.0989103517498564,2.48121508638053,
11.5141975983127));
#35247=CARTESIAN_POINT('Ctrl Pts',(-0.11878476294852,2.47550101244367,11.5152396404784));
#35248=CARTESIAN_POINT('Ctrl Pts',(-0.138108789237371,2.46825378794438,
11.5162816826442));
#35249=CARTESIAN_POINT('Ctrl Pts',(-0.157412061825551,2.46101434685037,
11.5173226056731));
#35250=CARTESIAN_POINT('Ctrl Pts',(-0.176165427403162,2.45224525402999,
11.5183635287019));
#35251=CARTESIAN_POINT('Ctrl Pts',(-0.194117882425333,2.44205721410709,
11.5194044517308));
#35252=CARTESIAN_POINT('Ctrl Pts',(-0.212079557360518,2.43186394187241,
11.5204459093505));
#35253=CARTESIAN_POINT('Ctrl Pts',(-0.229238852130596,2.420250615819,11.5214873669703));
#35254=CARTESIAN_POINT('Ctrl Pts',(-0.245369688947589,2.40737372325195,
11.5225288245901));
#35255=CARTESIAN_POINT('Ctrl Pts',(-0.261505454438471,2.39449289623283,
11.5235706004206));
#35256=CARTESIAN_POINT('Ctrl Pts',(-0.276611584428988,2.38034822103917,
11.5246123762511));
#35257=CARTESIAN_POINT('Ctrl Pts',(-0.290496119430963,2.36513561547923,
11.5256541520816));
#35258=CARTESIAN_POINT('Ctrl Pts',(-0.304410666170423,2.34989012752716,
11.5266981797342));
#35259=CARTESIAN_POINT('Ctrl Pts',(-0.317097894219481,2.33357268210092,
11.5277422073868));
#35260=CARTESIAN_POINT('Ctrl Pts',(-0.328406518659218,2.31641175684822,
11.5287862350394));
#35261=CARTESIAN_POINT('Ctrl Pts',(-0.33240623089295,2.31034216252743,11.5291554939353));
#35262=CARTESIAN_POINT('Ctrl Pts',(-0.336233899176785,2.30416729494598,
11.5295247528311));
#35263=CARTESIAN_POINT('Ctrl Pts',(-0.339884220642279,2.29789797007143,
11.529894011727));
#35264=CARTESIAN_POINT('Ctrl Pts',(-0.350604217101314,2.2794866764111,11.5309784241804));
#35265=CARTESIAN_POINT('Ctrl Pts',(-0.35985098890901,2.26015666987324,11.5320628366339));
#35266=CARTESIAN_POINT('Ctrl Pts',(-0.367477689652263,2.24016075630445,
11.5331472490873));
#35267=CARTESIAN_POINT('Ctrl Pts',(-0.375085032562881,2.22021559568392,
11.5342289091219));
#35268=CARTESIAN_POINT('Ctrl Pts',(-0.381080186982307,2.19960846920468,
11.5353105691565));
#35269=CARTESIAN_POINT('Ctrl Pts',(-0.38536290260287,2.17861503226159,11.5363922291911));
#35270=CARTESIAN_POINT('Ctrl Pts',(-0.389634913556175,2.15767406851004,
11.5374711856115));
#35271=CARTESIAN_POINT('Ctrl Pts',(-0.392202824028884,2.13634934251665,
11.5385501420318));
#35272=CARTESIAN_POINT('Ctrl Pts',(-0.393016510875971,2.11493024376485,
11.5396290984522));
#35273=CARTESIAN_POINT('Ctrl Pts',(-0.393206190108389,2.10993721945226,
11.5398806149003));
#35274=CARTESIAN_POINT('Ctrl Pts',(-0.39330076247864,2.10493911161085,11.5401321313484));
#35275=CARTESIAN_POINT('Ctrl Pts',(-0.393299995370208,2.09993965272061,
11.5403836477965));
#35276=CARTESIAN_POINT('',(-0.393506066767946,2.09966341860499,11.6653836477965));
#35277=CARTESIAN_POINT('Ctrl Pts',(-0.39266098561946,2.09993890584618,11.5403836903727));
#35278=CARTESIAN_POINT('Ctrl Pts',(-0.392745546116008,2.03788589116262,
11.543510578665));
#35279=CARTESIAN_POINT('Ctrl Pts',(-0.34960937735406,1.84450213648791,11.5532609147986));
#35280=CARTESIAN_POINT('Ctrl Pts',(-0.0466491534524713,1.63729177988004,
11.5696346987724));
#35281=CARTESIAN_POINT('Ctrl Pts',(0.363801326322039,1.81030423639476,11.5895050422954));
#35282=CARTESIAN_POINT('Ctrl Pts',(0.440513616274446,2.24907311750052,11.6093753858181));
#35283=CARTESIAN_POINT('Ctrl Pts',(0.113114633808556,2.55108770777179,11.629245729341));
#35284=CARTESIAN_POINT('Ctrl Pts',(-0.291992820397266,2.44604751618319,
11.6479151500004));
#35285=CARTESIAN_POINT('Ctrl Pts',(-0.392534688237482,2.20668854395861,
11.6599611228189));
#35286=CARTESIAN_POINT('Ctrl Pts',(-0.393506066767946,2.09966341860499,
11.6653836477965));
#35287=CARTESIAN_POINT('',(-0.393451127689227,2.10024138252102,11.7903836477965));
#35288=CARTESIAN_POINT('Ctrl Pts',(-0.393506066767946,2.09966341860499,
11.6653836477965));
#35289=CARTESIAN_POINT('Ctrl Pts',(-0.393721197300494,2.07596063797799,
11.6665845706598));
#35290=CARTESIAN_POINT('Ctrl Pts',(-0.38096993553427,1.9217609719386,11.6744089413645));
#35291=CARTESIAN_POINT('Ctrl Pts',(-0.177198995273587,1.67002842354576,
11.688856759909));
#35292=CARTESIAN_POINT('Ctrl Pts',(0.265606781934669,1.71825652870706,11.7087271034323));
#35293=CARTESIAN_POINT('Ctrl Pts',(0.4647544958161,2.11668229909881,11.7285974469549));
#35294=CARTESIAN_POINT('Ctrl Pts',(0.237553230397542,2.49980433115734,11.7484677904776));
#35295=CARTESIAN_POINT('Ctrl Pts',(-0.207570783958694,2.51616031782387,
11.7683381340004));
#35296=CARTESIAN_POINT('Ctrl Pts',(-0.386668906132234,2.25921693343521,
11.7823100864401));
#35297=CARTESIAN_POINT('Ctrl Pts',(-0.393864405022987,2.11452798323012,
11.7896585910388));
#35298=CARTESIAN_POINT('Ctrl Pts',(-0.393761364200694,2.10024157285132,
11.7903836477965));
#35299=CARTESIAN_POINT('',(-0.39310814853926,2.10020427938886,11.9153836449369));
#35300=CARTESIAN_POINT('Ctrl Pts',(-0.393299925984296,2.10024128975868,
11.7903836477965));
#35301=CARTESIAN_POINT('Ctrl Pts',(-0.393312358087271,2.07997708456835,
11.7914132981653));
#35302=CARTESIAN_POINT('Ctrl Pts',(-0.391754378673078,2.05965018812199,
11.792442948534));
#35303=CARTESIAN_POINT('Ctrl Pts',(-0.388623230446764,2.03952790100285,
11.7934725989028));
#35304=CARTESIAN_POINT('Ctrl Pts',(-0.385497099732515,2.01943785886577,
11.7945005993072));
#35305=CARTESIAN_POINT('Ctrl Pts',(-0.380802862960053,1.99955252466687,
11.7955285997115));
#35306=CARTESIAN_POINT('Ctrl Pts',(-0.374589626192585,1.98013548503039,
11.7965566001159));
#35307=CARTESIAN_POINT('Ctrl Pts',(-0.368376152079289,1.96071770366243,
11.7975846397899));
#35308=CARTESIAN_POINT('Ctrl Pts',(-0.360643749500282,1.94176898604104,
11.7986126794639));
#35309=CARTESIAN_POINT('Ctrl Pts',(-0.351491849216906,1.92353932468088,
11.7996407191379));
#35310=CARTESIAN_POINT('Ctrl Pts',(-0.342340698207265,1.90531115579835,
11.8006686746454));
#35311=CARTESIAN_POINT('Ctrl Pts',(-0.331770637105692,1.88780259463896,
11.801696630153));
#35312=CARTESIAN_POINT('Ctrl Pts',(-0.319927294380957,1.87123939082508,
11.8027245856605));
#35313=CARTESIAN_POINT('Ctrl Pts',(-0.308057729623245,1.85463951485819,
11.8037548171372));
#35314=CARTESIAN_POINT('Ctrl Pts',(-0.294909727505328,1.8389897697705,11.8047850486139));
#35315=CARTESIAN_POINT('Ctrl Pts',(-0.280669978286549,1.82448366057777,
11.8058152800907));
#35316=CARTESIAN_POINT('Ctrl Pts',(-0.270241171337324,1.81385977879227,
11.8065697937425));
#35317=CARTESIAN_POINT('Ctrl Pts',(-0.259227669239505,1.80384861854286,
11.8073243073943));
#35318=CARTESIAN_POINT('Ctrl Pts',(-0.247713843480614,1.79451228871187,
11.8080788210461));
#35319=CARTESIAN_POINT('Ctrl Pts',(-0.231783046212682,1.78159432548412,
11.8091227836936));
#35320=CARTESIAN_POINT('Ctrl Pts',(-0.214791578465285,1.76988738384627,
11.8101667463412));
#35321=CARTESIAN_POINT('Ctrl Pts',(-0.196949786389058,1.7595654664384,11.8112107089887));
#35322=CARTESIAN_POINT('Ctrl Pts',(-0.179140816211926,1.74926253730985,
11.8122527511545));
#35323=CARTESIAN_POINT('Ctrl Pts',(-0.160485226611759,1.74033999069353,
11.8132947933203));
#35324=CARTESIAN_POINT('Ctrl Pts',(-0.141223284345155,1.73292933383507,
11.814336835486));
#35325=CARTESIAN_POINT('Ctrl Pts',(-0.12198202910195,1.72552663590565,11.8153777585149));
#35326=CARTESIAN_POINT('Ctrl Pts',(-0.102136386848528,1.71963289406112,
11.8164186815437));
#35327=CARTESIAN_POINT('Ctrl Pts',(-0.0819475555604086,1.71533197671541,
11.8174596045726));
#35328=CARTESIAN_POINT('Ctrl Pts',(-0.061748355814717,1.71102885053065,
11.8185010621924));
#35329=CARTESIAN_POINT('Ctrl Pts',(-0.0412063311912306,1.70832035216473,
11.8195425198122));
#35330=CARTESIAN_POINT('Ctrl Pts',(-0.0205944375822625,1.7072395652046,
11.820583977432));
#35331=CARTESIAN_POINT('Ctrl Pts',(2.3753858809171E-5,1.70615844801694,
11.8216257532625));
#35332=CARTESIAN_POINT('Ctrl Pts',(0.0207111207399054,1.70670603467909,
11.8226675290929));
#35333=CARTESIAN_POINT('Ctrl Pts',(0.0411940407681122,1.70886327070295,
11.8237093049234));
#35334=CARTESIAN_POINT('Ctrl Pts',(0.0617212350927722,1.71102516964142,
11.824753332576));
#35335=CARTESIAN_POINT('Ctrl Pts',(0.0820423762315913,1.71480352955339,
11.8257973602286));
#35336=CARTESIAN_POINT('Ctrl Pts',(0.10189263988648,1.72012794267416,11.8268413878812));
#35337=CARTESIAN_POINT('Ctrl Pts',(0.10891341794883,1.72201111780388,11.8272106467771));
#35338=CARTESIAN_POINT('Ctrl Pts',(0.115875439456983,1.72408724175438,11.827579905673));
#35339=CARTESIAN_POINT('Ctrl Pts',(0.122767557839216,1.72635174730477,11.8279491645688));
#35340=CARTESIAN_POINT('Ctrl Pts',(0.142252841021652,1.7327539199708,11.8289931272164));
#35341=CARTESIAN_POINT('Ctrl Pts',(0.161294035664333,1.740703471235,11.8300370898639));
#35342=CARTESIAN_POINT('Ctrl Pts',(0.179630973060031,1.75011772906089,11.8310810525115));
#35343=CARTESIAN_POINT('Ctrl Pts',(0.197934177683471,1.75951466834507,11.8321230946773));
#35344=CARTESIAN_POINT('Ctrl Pts',(0.215535022366861,1.77037068639414,11.833165136843));
#35345=CARTESIAN_POINT('Ctrl Pts',(0.232192872726832,1.78255494986555,11.8342071790088));
#35346=CARTESIAN_POINT('Ctrl Pts',(0.248832832817209,1.79472612762942,11.8352481020377));
#35347=CARTESIAN_POINT('Ctrl Pts',(0.264531201223698,1.8082223100065,11.8362890250665));
#35348=CARTESIAN_POINT('Ctrl Pts',(0.279076068698541,1.82286927655028,11.8373299480954));
#35349=CARTESIAN_POINT('Ctrl Pts',(0.293628406038229,1.83752376539432,11.8383714057152));
#35350=CARTESIAN_POINT('Ctrl Pts',(0.307025529057808,1.85332970838511,11.839412863335));
#35351=CARTESIAN_POINT('Ctrl Pts',(0.319091864528525,1.87007550806469,11.8404543209547));
#35352=CARTESIAN_POINT('Ctrl Pts',(0.331161886790774,1.88682642431613,11.8414960967852));
#35353=CARTESIAN_POINT('Ctrl Pts',(0.341899911610759,1.9045171513388,11.8425378726157));
#35354=CARTESIAN_POINT('Ctrl Pts',(0.351173843652062,1.92290730807106,11.8435796484462));
#35355=CARTESIAN_POINT('Ctrl Pts',(0.360467821507927,1.94133721554444,11.8446236760988));
#35356=CARTESIAN_POINT('Ctrl Pts',(0.368291109722894,1.96046888934245,11.8456677037514));
#35357=CARTESIAN_POINT('Ctrl Pts',(0.374559554228507,1.98004154745854,11.846711731404));
#35358=CARTESIAN_POINT('Ctrl Pts',(0.376776620884906,1.98696414008059,11.8470809902999));
#35359=CARTESIAN_POINT('Ctrl Pts',(0.378799646733713,1.99394177582292,11.8474502491958));
#35360=CARTESIAN_POINT('Ctrl Pts',(0.380626438135335,2.00096261012927,11.8478195080916));
#35361=CARTESIAN_POINT('Ctrl Pts',(0.385791112594161,2.02081179684508,11.8488634707392));
#35362=CARTESIAN_POINT('Ctrl Pts',(0.389414330272041,2.04112520996009,11.8499074333867));
#35363=CARTESIAN_POINT('Ctrl Pts',(0.391424769275268,2.06163934309995,11.8509513960343));
#35364=CARTESIAN_POINT('Ctrl Pts',(0.393431509859312,2.08211573828138,11.8519934382001));
#35365=CARTESIAN_POINT('Ctrl Pts',(0.393831230767547,2.10279140234921,11.8530354803658));
#35366=CARTESIAN_POINT('Ctrl Pts',(0.392603679277159,2.12339318315316,11.8540775225316));
#35367=CARTESIAN_POINT('Ctrl Pts',(0.391377446157789,2.14397283796818,11.8551184455605));
#35368=CARTESIAN_POINT('Ctrl Pts',(0.38852742484426,2.16447803457521,11.8561593685893));
#35369=CARTESIAN_POINT('Ctrl Pts',(0.38408539270256,2.18463628720898,11.8572002916182));
#35370=CARTESIAN_POINT('Ctrl Pts',(0.379641079248923,2.20480489259592,11.858241749238));
#35371=CARTESIAN_POINT('Ctrl Pts',(0.373603264147745,2.2246254760342,11.8592832068578));
#35372=CARTESIAN_POINT('Ctrl Pts',(0.366054821369077,2.24383587088224,11.8603246644775));
#35373=CARTESIAN_POINT('Ctrl Pts',(0.358504072212052,2.26305213534342,11.861366440308));
#35374=CARTESIAN_POINT('Ctrl Pts',(0.349442079048673,2.28165716905833,11.8624082161385));
#35375=CARTESIAN_POINT('Ctrl Pts',(0.338999452987024,2.29940978129094,11.863449991969));
#35376=CARTESIAN_POINT('Ctrl Pts',(0.328534254952179,2.31720076619773,11.8644940196216));
#35377=CARTESIAN_POINT('Ctrl Pts',(0.316682888350589,2.3341350477143,11.8655380472742));
#35378=CARTESIAN_POINT('Ctrl Pts',(0.303619069244698,2.35000070158098,11.8665820749268));
#35379=CARTESIAN_POINT('Ctrl Pts',(0.298998567664272,2.35561217539054,11.8669513338227));
#35380=CARTESIAN_POINT('Ctrl Pts',(0.294226747047553,2.36109029205047,11.8673205927186));
#35381=CARTESIAN_POINT('Ctrl Pts',(0.289312379052769,2.366426795437,11.8676898516144));
#35382=CARTESIAN_POINT('Ctrl Pts',(0.275418559078957,2.38151406961361,11.868733814262));
#35383=CARTESIAN_POINT('Ctrl Pts',(0.260299990829136,2.39555655346789,11.8697777769095));
#35384=CARTESIAN_POINT('Ctrl Pts',(0.244139627350994,2.40835163751295,11.8708217395571));
#35385=CARTESIAN_POINT('Ctrl Pts',(0.228008992602849,2.42112318362216,11.8718637817229));
#35386=CARTESIAN_POINT('Ctrl Pts',(0.210840900219715,2.43265138666402,11.8729058238886));
#35387=CARTESIAN_POINT('Ctrl Pts',(0.192854058255359,2.44277135559209,11.8739478660544));
#35388=CARTESIAN_POINT('Ctrl Pts',(0.174886533876714,2.45288045583251,11.8749887890833));
#35389=CARTESIAN_POINT('Ctrl Pts',(0.15610262940298,2.46158394031299,11.8760297121121));
#35390=CARTESIAN_POINT('Ctrl Pts',(0.136748657406688,2.46876102654357,11.877070635141));
#35391=CARTESIAN_POINT('Ctrl Pts',(0.117384745714798,2.47594179873858,11.8781120927608));
#35392=CARTESIAN_POINT('Ctrl Pts',(0.0974508658738936,2.48159433564851,
11.8791535503805));
#35393=CARTESIAN_POINT('Ctrl Pts',(0.0772123134675798,2.48564640365104,
11.8801950080003));
#35394=CARTESIAN_POINT('Ctrl Pts',(0.0569675773011836,2.48969970973701,
11.8812367838308));
#35395=CARTESIAN_POINT('Ctrl Pts',(0.0364187112028805,2.49215146455734,
11.8822785596613));
#35396=CARTESIAN_POINT('Ctrl Pts',(0.0158392148146877,2.49298092736678,
11.8833203354918));
#35397=CARTESIAN_POINT('Ctrl Pts',(-0.00478476462195937,2.49381218307891,
11.8843643631444));
#35398=CARTESIAN_POINT('Ctrl Pts',(-0.0254387706010218,2.49301417441685,
11.885408390797));
#35399=CARTESIAN_POINT('Ctrl Pts',(-0.0458505777671413,2.4906182465252,
11.8864524184496));
#35400=CARTESIAN_POINT('Ctrl Pts',(-0.0530699664088936,2.48977083823515,
11.8868216773455));
#35401=CARTESIAN_POINT('Ctrl Pts',(-0.0602591377000667,2.4887240095554,
11.8871909362414));
#35402=CARTESIAN_POINT('Ctrl Pts',(-0.0674064014868825,2.48748066666427,
11.8875601951372));
#35403=CARTESIAN_POINT('Ctrl Pts',(-0.0876130275401507,2.48396550819155,
11.8886041577848));
#35404=CARTESIAN_POINT('Ctrl Pts',(-0.107604153555675,2.47885499556035,
11.8896481204323));
#35405=CARTESIAN_POINT('Ctrl Pts',(-0.127110386058818,2.47219328279266,
11.8906920830799));
#35406=CARTESIAN_POINT('Ctrl Pts',(-0.146580734745346,2.46554382496345,
11.8917341252457));
#35407=CARTESIAN_POINT('Ctrl Pts',(-0.165567252883045,2.45734901011157,
11.8927761674114));
#35408=CARTESIAN_POINT('Ctrl Pts',(-0.183812906506485,2.44770347338161,
11.8938182095772));
#35409=CARTESIAN_POINT('Ctrl Pts',(-0.202038964584578,2.43806829580657,
11.8948591326061));
#35410=CARTESIAN_POINT('Ctrl Pts',(-0.219525077061563,2.42698580602208,
11.8959000556349));
#35411=CARTESIAN_POINT('Ctrl Pts',(-0.236036354411226,2.41459772630497,
11.8969409786638));
#35412=CARTESIAN_POINT('Ctrl Pts',(-0.252556111522601,2.40220328439299,
11.8979824362836));
#35413=CARTESIAN_POINT('Ctrl Pts',(-0.2680994351019,2.38850234168312,11.8990238939034));
#35414=CARTESIAN_POINT('Ctrl Pts',(-0.282461980533189,2.37367886208706,
11.9000653515231));
#35415=CARTESIAN_POINT('Ctrl Pts',(-0.296828914348269,2.35885085327173,
11.9011071273536));
#35416=CARTESIAN_POINT('Ctrl Pts',(-0.310013866211834,2.34290017792611,
11.9021489031841));
#35417=CARTESIAN_POINT('Ctrl Pts',(-0.321851346635873,2.32604557210588,
11.9031906790146));
#35418=CARTESIAN_POINT('Ctrl Pts',(-0.333714414042464,2.30915453467271,
11.9042347066672));
#35419=CARTESIAN_POINT('Ctrl Pts',(-0.34422382070222,2.29135630014038,11.9052787343198));
#35420=CARTESIAN_POINT('Ctrl Pts',(-0.353258561670272,2.27289672815485,
11.9063227619724));
#35421=CARTESIAN_POINT('Ctrl Pts',(-0.35645403112551,2.26636781950709,11.9066920208683));
#35422=CARTESIAN_POINT('Ctrl Pts',(-0.359465467148731,2.25975636828849,
11.9070612797642));
#35423=CARTESIAN_POINT('Ctrl Pts',(-0.36228898521523,2.25307377695647,11.90743053866));
#35424=CARTESIAN_POINT('Ctrl Pts',(-0.371160264491516,2.23207758263456,
11.9085907220601));
#35425=CARTESIAN_POINT('Ctrl Pts',(-0.378217950532817,2.21027158304454,
11.9097509054601));
#35426=CARTESIAN_POINT('Ctrl Pts',(-0.383336557191521,2.18796575424875,
11.9109110888601));
#35427=CARTESIAN_POINT('Ctrl Pts',(-0.388417242785302,2.16582517760815,
11.9120626770715));
#35428=CARTESIAN_POINT('Ctrl Pts',(-0.391587266064288,2.1431925567704,11.9132142652829));
#35429=CARTESIAN_POINT('Ctrl Pts',(-0.392771028312522,2.12039140304942,
11.9143658534942));
#35430=CARTESIAN_POINT('Ctrl Pts',(-0.393119770227964,2.11367407612434,
11.9147051167873));
#35431=CARTESIAN_POINT('Ctrl Pts',(-0.393296445026141,2.10694223489702,
11.9150443800805));
#35432=CARTESIAN_POINT('Ctrl Pts',(-0.393299946880902,2.1002044100772,11.9153836433736));
#35433=CARTESIAN_POINT('',(-0.393236352003104,2.09966893770289,12.0403836508529));
#35434=CARTESIAN_POINT('Ctrl Pts',(-0.392757315398087,2.10020404033675,
11.9153836477965));
#35435=CARTESIAN_POINT('Ctrl Pts',(-0.392387812223022,2.02141992873627,
11.9193560592586));
#35436=CARTESIAN_POINT('Ctrl Pts',(-0.331161934722823,1.81074557558215,
11.9299519185616));
#35437=CARTESIAN_POINT('Ctrl Pts',(0.0125649746725957,1.63511596941171,
11.9471712257055));
#35438=CARTESIAN_POINT('Ctrl Pts',(0.397684464205737,1.85891472999403,11.9670415692284));
#35439=CARTESIAN_POINT('Ctrl Pts',(0.417982597681194,2.30387640501092,11.9869119127511));
#35440=CARTESIAN_POINT('Ctrl Pts',(0.0548386009764254,2.5618092336966,12.0067822562739));
#35441=CARTESIAN_POINT('Ctrl Pts',(-0.316031342189213,2.41316174940269,
12.0246061679557));
#35442=CARTESIAN_POINT('Ctrl Pts',(-0.392293930819629,2.19029546669872,
12.0358066317966));
#35443=CARTESIAN_POINT('Ctrl Pts',(-0.39301380866462,2.09966918558721,12.0403836477965));
#35444=CARTESIAN_POINT('',(-0.393542333918762,2.09995565468233,12.1653836477965));
#35445=CARTESIAN_POINT('Ctrl Pts',(-0.393299860603728,2.09966886696257,
12.0403836517251));
#35446=CARTESIAN_POINT('Ctrl Pts',(-0.393278992343729,2.07488280571045,
12.0416345529641));
#35447=CARTESIAN_POINT('Ctrl Pts',(-0.390911039572184,2.05019917076539,
12.042885454203));
#35448=CARTESIAN_POINT('Ctrl Pts',(-0.386277243284786,2.02600823478044,
12.044136355442));
#35449=CARTESIAN_POINT('Ctrl Pts',(-0.383330311450925,2.01062364838013,
12.0449318847345));
#35450=CARTESIAN_POINT('Ctrl Pts',(-0.379467960270538,1.99543790614008,
12.045727414027));
#35451=CARTESIAN_POINT('Ctrl Pts',(-0.374721036216391,1.98054693383209,
12.0465229433195));
#35452=CARTESIAN_POINT('Ctrl Pts',(-0.368491710093453,1.96100570634752,
12.0475669059671));
#35453=CARTESIAN_POINT('Ctrl Pts',(-0.360711132460197,1.94189484371864,
12.0486108686146));
#35454=CARTESIAN_POINT('Ctrl Pts',(-0.351459667605607,1.92347523673276,
12.0496548312622));
#35455=CARTESIAN_POINT('Ctrl Pts',(-0.34222522181752,1.90508951459875,12.050696873428));
#35456=CARTESIAN_POINT('Ctrl Pts',(-0.33152553318996,1.88739320072474,12.0517389155937));
#35457=CARTESIAN_POINT('Ctrl Pts',(-0.319489298458345,1.87062807894035,
12.0527809577595));
#35458=CARTESIAN_POINT('Ctrl Pts',(-0.307465990453748,1.85388096263339,
12.0538218807884));
#35459=CARTESIAN_POINT('Ctrl Pts',(-0.294109389451292,1.83806366453776,
12.0548628038172));
#35460=CARTESIAN_POINT('Ctrl Pts',(-0.2795918320278,1.82338962878565,12.0559037268461));
#35461=CARTESIAN_POINT('Ctrl Pts',(-0.265066818765183,1.80870805683123,
12.0569451844659));
#35462=CARTESIAN_POINT('Ctrl Pts',(-0.249380163951019,1.79517145460707,
12.0579866420857));
#35463=CARTESIAN_POINT('Ctrl Pts',(-0.232741901561904,1.78295726272733,
12.0590280997055));
#35464=CARTESIAN_POINT('Ctrl Pts',(-0.216098555458261,1.77073933887947,
12.060069875536));
#35465=CARTESIAN_POINT('Ctrl Pts',(-0.198503636978505,1.75984503562868,
12.0611116513665));
#35466=CARTESIAN_POINT('Ctrl Pts',(-0.180196347689156,1.75040857235984,
12.062153427197));
#35467=CARTESIAN_POINT('Ctrl Pts',(-0.161849486778567,1.7409517119615,12.0631974548496));
#35468=CARTESIAN_POINT('Ctrl Pts',(-0.142787860101782,1.73295926745141,
12.0642414825022));
#35469=CARTESIAN_POINT('Ctrl Pts',(-0.123271494020737,1.7265176995333,12.0652855101548));
#35470=CARTESIAN_POINT('Ctrl Pts',(-0.116368811154175,1.72423940139535,
12.0656547690507));
#35471=CARTESIAN_POINT('Ctrl Pts',(-0.109409368565569,1.72215464889553,
12.0660240279465));
#35472=CARTESIAN_POINT('Ctrl Pts',(-0.102404990915842,1.72026574050327,
12.0663932868423));
#35473=CARTESIAN_POINT('Ctrl Pts',(-0.0826023301861622,1.71492544991475,
12.0674372494899));
#35474=CARTESIAN_POINT('Ctrl Pts',(-0.0623218074606997,1.71112244364286,
12.0684812121374));
#35475=CARTESIAN_POINT('Ctrl Pts',(-0.041826287026211,1.70893037485174,
12.069525174785));
#35476=CARTESIAN_POINT('Ctrl Pts',(-0.0213684703100815,1.70674233860736,
12.0705672169508));
#35477=CARTESIAN_POINT('Ctrl Pts',(-0.000697157978116574,1.70615949392462,
12.0716092591165));
#35478=CARTESIAN_POINT('Ctrl Pts',(0.019914687928456,1.70720451223988,12.0726513012823));
#35479=CARTESIAN_POINT('Ctrl Pts',(0.0405043970363343,1.70824840822188,
12.0736922243112));
#35480=CARTESIAN_POINT('Ctrl Pts',(0.0610340339351239,1.7109166882268,12.07473314734));
#35481=CARTESIAN_POINT('Ctrl Pts',(0.08123084207394,1.71517998974071,12.0757740703689));
#35482=CARTESIAN_POINT('Ctrl Pts',(0.101438022767024,1.71944548077517,12.0768155279887));
#35483=CARTESIAN_POINT('Ctrl Pts',(0.121311309972315,1.72530749362791,12.0778569856085));
#35484=CARTESIAN_POINT('Ctrl Pts',(0.140587813257872,1.73268547978147,12.0788984432282));
#35485=CARTESIAN_POINT('Ctrl Pts',(0.159870206355562,1.74006572023145,12.0799402190587));
#35486=CARTESIAN_POINT('Ctrl Pts',(0.178554778877644,1.74896255951808,12.0809819948892));
#35487=CARTESIAN_POINT('Ctrl Pts',(0.196399192632152,1.75924752805968,12.0820237707197));
#35488=CARTESIAN_POINT('Ctrl Pts',(0.214282177491934,1.76955472779418,12.0830677983723));
#35489=CARTESIAN_POINT('Ctrl Pts',(0.231320770877661,1.78125563016296,12.0841118260249));
#35490=CARTESIAN_POINT('Ctrl Pts',(0.247301518113519,1.79417840308646,12.0851558536775));
#35491=CARTESIAN_POINT('Ctrl Pts',(0.252953698939172,1.798749018481,12.0855251125734));
#35492=CARTESIAN_POINT('Ctrl Pts',(0.258473868190067,1.80347212821718,12.0858943714693));
#35493=CARTESIAN_POINT('Ctrl Pts',(0.263853692369344,1.80833903411141,12.0862636303651));
#35494=CARTESIAN_POINT('Ctrl Pts',(0.279063442375129,1.82209867001886,12.0873075930127));
#35495=CARTESIAN_POINT('Ctrl Pts',(0.293239291536087,1.83709226062575,12.0883515556602));
#35496=CARTESIAN_POINT('Ctrl Pts',(0.306177017765042,1.85313865472192,12.0893955183078));
#35497=CARTESIAN_POINT('Ctrl Pts',(0.319090943652483,1.86915552974705,12.0904375604736));
#35498=CARTESIAN_POINT('Ctrl Pts',(0.330770764769411,1.88622083490477,12.0914796026393));
#35499=CARTESIAN_POINT('Ctrl Pts',(0.341049659281186,1.90411733128174,12.0925216448051));
#35500=CARTESIAN_POINT('Ctrl Pts',(0.351317514421732,1.92199460710275,12.0935625678339));
#35501=CARTESIAN_POINT('Ctrl Pts',(0.360187040219998,1.94070068155717,12.0946034908628));
#35502=CARTESIAN_POINT('Ctrl Pts',(0.367535277154023,1.95999032159413,12.0956444138917));
#35503=CARTESIAN_POINT('Ctrl Pts',(0.374887287951018,1.97928986828746,12.0966858715114));
#35504=CARTESIAN_POINT('Ctrl Pts',(0.380716172040446,1.99917289746567,12.0977273291312));
#35505=CARTESIAN_POINT('Ctrl Pts',(0.384947348717024,2.01937476377874,12.098768786751));
#35506=CARTESIAN_POINT('Ctrl Pts',(0.389179818202539,2.0395828026427,12.0998105625815));
#35507=CARTESIAN_POINT('Ctrl Pts',(0.39181349315293,2.06010914561655,12.100852338412));
#35508=CARTESIAN_POINT('Ctrl Pts',(0.392825211050546,2.08068048750372,12.1018941142425));
#35509=CARTESIAN_POINT('Ctrl Pts',(0.393839115799356,2.10129629481321,12.1029381418951));
#35510=CARTESIAN_POINT('Ctrl Pts',(0.393224086057792,2.12195655907155,12.1039821695477));
#35511=CARTESIAN_POINT('Ctrl Pts',(0.391009054441986,2.14238878795606,12.1050261972003));
#35512=CARTESIAN_POINT('Ctrl Pts',(0.39022562679355,2.14961539949202,12.1053954560962));
#35513=CARTESIAN_POINT('Ctrl Pts',(0.389242518921626,2.15681356127486,12.105764714992));
#35514=CARTESIAN_POINT('Ctrl Pts',(0.388062533342288,2.16397155786727,12.1061339738879));
#35515=CARTESIAN_POINT('Ctrl Pts',(0.38472649761437,2.18420852753092,12.1071779365355));
#35516=CARTESIAN_POINT('Ctrl Pts',(0.379793261473248,2.20424413682783,12.108221899183));
#35517=CARTESIAN_POINT('Ctrl Pts',(0.373304590993985,2.22380861174738,12.1092658618306));
#35518=CARTESIAN_POINT('Ctrl Pts',(0.366827857123262,2.24333709570713,12.1103079039963));
#35519=CARTESIAN_POINT('Ctrl Pts',(0.358801541214424,2.26239545645464,12.1113499461621));
#35520=CARTESIAN_POINT('Ctrl Pts',(0.34931799796196,2.28072583185546,12.1123919883279));
#35521=CARTESIAN_POINT('Ctrl Pts',(0.339844639885968,2.29903652072106,12.1134329113567));
#35522=CARTESIAN_POINT('Ctrl Pts',(0.328917472140692,2.31662011291515,12.1144738343856));
#35523=CARTESIAN_POINT('Ctrl Pts',(0.316676130855067,2.33324047278863,12.1155147574144));
#35524=CARTESIAN_POINT('Ctrl Pts',(0.304428502735605,2.34986936844577,12.1165562150342));
#35525=CARTESIAN_POINT('Ctrl Pts',(0.290865776088012,2.36553344150845,12.117597672654));
#35526=CARTESIAN_POINT('Ctrl Pts',(0.276170097577517,2.38002672587456,12.1186391302738));
#35527=CARTESIAN_POINT('Ctrl Pts',(0.261469928896557,2.3945244385709,12.1196809061043));
#35528=CARTESIAN_POINT('Ctrl Pts',(0.245636668050709,2.40785015996275,12.1207226819348));
#35529=CARTESIAN_POINT('Ctrl Pts',(0.228887576653288,2.41983646954934,12.1217644577653));
#35530=CARTESIAN_POINT('Ctrl Pts',(0.21210228171473,2.4318486878161,12.1228084854178));
#35531=CARTESIAN_POINT('Ctrl Pts',(0.194397834904987,2.44251533414798,12.1238525130704));
#35532=CARTESIAN_POINT('Ctrl Pts',(0.176019014395658,2.45171323058876,12.124896540723));
#35533=CARTESIAN_POINT('Ctrl Pts',(0.169518666486625,2.45496640599607,12.1252657996189));
#35534=CARTESIAN_POINT('Ctrl Pts',(0.162934149126423,2.45803628633091,12.1256350585148));
#35535=CARTESIAN_POINT('Ctrl Pts',(0.156276829917091,2.46091888622108,12.1260043174106));
#35536=CARTESIAN_POINT('Ctrl Pts',(0.137455367075572,2.46906852498915,12.1270482800582));
#35537=CARTESIAN_POINT('Ctrl Pts',(0.117938618192391,2.47576620904804,12.1280922427057));
#35538=CARTESIAN_POINT('Ctrl Pts',(0.097976022816915,2.48090102251501,12.1291362053533));
#35539=CARTESIAN_POINT('Ctrl Pts',(0.0780501507867196,2.4860263899393,12.130178247519));
#35540=CARTESIAN_POINT('Ctrl Pts',(0.0576807500142376,2.48959435485226,
12.1312202896848));
#35541=CARTESIAN_POINT('Ctrl Pts',(0.0371346288638493,2.49154298530193,
12.1322623318506));
#35542=CARTESIAN_POINT('Ctrl Pts',(0.0166105739248071,2.4934895229531,12.1333032548794));
#35543=CARTESIAN_POINT('Ctrl Pts',(-0.00408909855726484,2.49382008083868,
12.1343441779083));
#35544=CARTESIAN_POINT('Ctrl Pts',(-0.0246902539410924,2.49252424302242,
12.1353851009372));
#35545=CARTESIAN_POINT('Ctrl Pts',(-0.0453019895413941,2.49122773969763,
12.1364265585569));
#35546=CARTESIAN_POINT('Ctrl Pts',(-0.0658143716253239,2.48830320208075,
12.1374680161767));
#35547=CARTESIAN_POINT('Ctrl Pts',(-0.0859556209254608,2.48379228917647,
12.1385094737965));
#35548=CARTESIAN_POINT('Ctrl Pts',(-0.106103024255346,2.47927999799165,
12.139551249627));
#35549=CARTESIAN_POINT('Ctrl Pts',(-0.125878359575164,2.4731805625576,12.1405930254575));
#35550=CARTESIAN_POINT('Ctrl Pts',(-0.145023249093352,2.4655860325866,12.141634801288));
#35551=CARTESIAN_POINT('Ctrl Pts',(-0.164209520724682,2.45797508686672,
12.1426788289406));
#35552=CARTESIAN_POINT('Ctrl Pts',(-0.18276196489742,2.4488629193954,12.1437228565932));
#35553=CARTESIAN_POINT('Ctrl Pts',(-0.200444508533405,2.43838866558855,
12.1447668842458));
#35554=CARTESIAN_POINT('Ctrl Pts',(-0.206698592439045,2.434684059311,12.1451361431417));
#35555=CARTESIAN_POINT('Ctrl Pts',(-0.21284412101073,2.43080946091724,12.1455054020376));
#35556=CARTESIAN_POINT('Ctrl Pts',(-0.218871589787769,2.4267722711366,12.1458746609334));
#35557=CARTESIAN_POINT('Ctrl Pts',(-0.235859404920921,2.41539385737989,
12.1469153800299));
#35558=CARTESIAN_POINT('Ctrl Pts',(-0.252009714550351,2.40265218981606,
12.1479560991263));
#35559=CARTESIAN_POINT('Ctrl Pts',(-0.267095036879578,2.38869556850478,
12.1489968182227));
#35560=CARTESIAN_POINT('Ctrl Pts',(-0.282152609210813,2.374764620905,12.1500356228785));
#35561=CARTESIAN_POINT('Ctrl Pts',(-0.296148503569641,2.35962360806551,
12.1510744275344));
#35562=CARTESIAN_POINT('Ctrl Pts',(-0.308886923198884,2.34346202717616,
12.1521132321902));
#35563=CARTESIAN_POINT('Ctrl Pts',(-0.321611824317927,2.32731759758991,
12.1531509344259));
#35564=CARTESIAN_POINT('Ctrl Pts',(-0.333081420598854,2.31015531091151,
12.1541886366615));
#35565=CARTESIAN_POINT('Ctrl Pts',(-0.343139227393768,2.29219875291897,
12.1552263388971));
#35566=CARTESIAN_POINT('Ctrl Pts',(-0.353202254929823,2.27423287415273,
12.1562645797765));
#35567=CARTESIAN_POINT('Ctrl Pts',(-0.361851654557597,2.25547253991361,
12.1573028206559));
#35568=CARTESIAN_POINT('Ctrl Pts',(-0.368976013497073,2.23616751251237,
12.1583410615353));
#35569=CARTESIAN_POINT('Ctrl Pts',(-0.376102798245648,2.21685591184447,
12.1593796559306));
#35570=CARTESIAN_POINT('Ctrl Pts',(-0.38170328924997,2.19699995663281,12.1604182503259));
#35571=CARTESIAN_POINT('Ctrl Pts',(-0.385715712151455,2.17686533288483,
12.1614568447212));
#35572=CARTESIAN_POINT('Ctrl Pts',(-0.389736625277397,2.15668810458615,
12.162497636766));
#35573=CARTESIAN_POINT('Ctrl Pts',(-0.392162681036991,2.13623176724534,
12.1635384288109));
#35574=CARTESIAN_POINT('Ctrl Pts',(-0.392983771039473,2.11576850340379,
12.1645792208558));
#35575=CARTESIAN_POINT('Ctrl Pts',(-0.393195310870127,2.1104964925955,12.1648473631694));
#35576=CARTESIAN_POINT('Ctrl Pts',(-0.393300591151716,2.10522401439645,
12.1651155054829));
#35577=CARTESIAN_POINT('Ctrl Pts',(-0.393299997503069,2.09995568198939,
12.1653836477965));
#35578=CARTESIAN_POINT('',(-0.393299839507982,2.10035530690372,12.2903836477965));
#35579=CARTESIAN_POINT('Ctrl Pts',(-0.393943705169969,2.09995560945483,
12.1653836477965));
#35580=CARTESIAN_POINT('Ctrl Pts',(-0.393947486574571,2.09758514782183,
12.1655041000164));
#35581=CARTESIAN_POINT('Ctrl Pts',(-0.393927945909171,2.0952147502193,12.1656245522363));
#35582=CARTESIAN_POINT('Ctrl Pts',(-0.391517524700006,1.96252442555434,
12.1723684522972));
#35583=CARTESIAN_POINT('Ctrl Pts',(-0.244598393841188,1.70446660543666,
12.185615347979));
#35584=CARTESIAN_POINT('Ctrl Pts',(0.200166029731868,1.68022791776267,12.2054856915018));
#35585=CARTESIAN_POINT('Ctrl Pts',(0.461305371170257,2.04107296873276,12.2253560350246));
#35586=CARTESIAN_POINT('Ctrl Pts',(0.299259835615228,2.45597554869975,12.2452263785474));
#35587=CARTESIAN_POINT('Ctrl Pts',(-0.137315858568866,2.54431902442941,
12.2650967220702));
#35588=CARTESIAN_POINT('Ctrl Pts',(-0.372610321006317,2.30247066778261,
12.2801491210047));
#35589=CARTESIAN_POINT('Ctrl Pts',(-0.393458625209538,2.13607564144017,
12.2885780720982));
#35590=CARTESIAN_POINT('Ctrl Pts',(-0.393146135639666,2.10035660126003,
12.2903835753508));
#35591=CARTESIAN_POINT('',(-0.393077234676447,2.09986488121323,12.4153836834263));
#35592=CARTESIAN_POINT('Ctrl Pts',(-0.393299839507982,2.10035530690372,
12.2903836477965));
#35593=CARTESIAN_POINT('Ctrl Pts',(-0.39331828485987,2.07993759516899,12.291415314833));
#35594=CARTESIAN_POINT('Ctrl Pts',(-0.391742474161141,2.059484472507,12.2924469818694));
#35595=CARTESIAN_POINT('Ctrl Pts',(-0.388582344254501,2.03926572850789,
12.2934786489059));
#35596=CARTESIAN_POINT('Ctrl Pts',(-0.385421623636996,2.01904320509715,
12.2945105087879));
#35597=CARTESIAN_POINT('Ctrl Pts',(-0.380676071652342,1.99905589466593,
12.2955423686699));
#35598=CARTESIAN_POINT('Ctrl Pts',(-0.374407400948638,1.97956749560486,
12.2965742285519));
#35599=CARTESIAN_POINT('Ctrl Pts',(-0.368138578638465,1.960078625221,12.2976061133892));
#35600=CARTESIAN_POINT('Ctrl Pts',(-0.360346816786855,1.941089398043,12.2986379982265));
#35601=CARTESIAN_POINT('Ctrl Pts',(-0.351143090919384,1.92284633873504,
12.2996698830638));
#35602=CARTESIAN_POINT('Ctrl Pts',(-0.341918686932898,1.90456229253145,
12.3007040862489));
#35603=CARTESIAN_POINT('Ctrl Pts',(-0.331276362675052,1.88702841307074,
12.3017382894339));
#35604=CARTESIAN_POINT('Ctrl Pts',(-0.319372463074704,1.87046542781185,
12.302772492619));
#35605=CARTESIAN_POINT('Ctrl Pts',(-0.311449919737479,1.85944206799592,
12.3034607981179));
#35606=CARTESIAN_POINT('Ctrl Pts',(-0.302969490447348,1.84884816990448,
12.3041491036168));
#35607=CARTESIAN_POINT('Ctrl Pts',(-0.293986668735287,1.83874011290302,
12.3048374091157));
#35608=CARTESIAN_POINT('Ctrl Pts',(-0.280362296487944,1.82340908043909,
12.3058813717633));
#35609=CARTESIAN_POINT('Ctrl Pts',(-0.265494859934947,1.80910097822167,
12.3069253344108));
#35610=CARTESIAN_POINT('Ctrl Pts',(-0.249563694235651,1.79602162491477,
12.3079692970584));
#35611=CARTESIAN_POINT('Ctrl Pts',(-0.233661835632341,1.78296633248767,
12.3090113392242));
#35612=CARTESIAN_POINT('Ctrl Pts',(-0.216700656659647,1.77113580970523,
12.3100533813899));
#35613=CARTESIAN_POINT('Ctrl Pts',(-0.1988959100457,1.76069879610132,12.3110954235557));
#35614=CARTESIAN_POINT('Ctrl Pts',(-0.181110285449925,1.75027299168607,
12.3121363465845));
#35615=CARTESIAN_POINT('Ctrl Pts',(-0.162483508710738,1.74123812048123,
12.3131772696134));
#35616=CARTESIAN_POINT('Ctrl Pts',(-0.143259714116111,1.73371930939323,
12.3142181926422));
#35617=CARTESIAN_POINT('Ctrl Pts',(-0.124026046681599,1.72619663683982,
12.315259650262));
#35618=CARTESIAN_POINT('Ctrl Pts',(-0.104195428206946,1.72019186291053,
12.3163011078818));
#35619=CARTESIAN_POINT('Ctrl Pts',(-0.0840318330442134,1.71578190954195,
12.3173425655016));
#35620=CARTESIAN_POINT('Ctrl Pts',(-0.0638620770240899,1.71137060874035,
12.3183843413321));
#35621=CARTESIAN_POINT('Ctrl Pts',(-0.0433598676905176,1.70855522030048,
12.3194261171626));
#35622=CARTESIAN_POINT('Ctrl Pts',(-0.0227982943508453,1.70736132669502,
12.3204678929931));
#35623=CARTESIAN_POINT('Ctrl Pts',(-0.0021922767038096,1.70616485246145,
12.3215119206457));
#35624=CARTESIAN_POINT('Ctrl Pts',(0.018472624810372,1.70659685502673,12.3225559482983));
#35625=CARTESIAN_POINT('Ctrl Pts',(0.0389236722817217,1.70863081657327,
12.3235999759509));
#35626=CARTESIAN_POINT('Ctrl Pts',(0.0461569397051607,1.70935020211163,
12.3239692348468));
#35627=CARTESIAN_POINT('Ctrl Pts',(0.0533635272051451,1.71026951204017,
12.3243384937427));
#35628=CARTESIAN_POINT('Ctrl Pts',(0.0605316949800335,1.71138604772494,
12.3247077526385));
#35629=CARTESIAN_POINT('Ctrl Pts',(0.0807974204426804,1.7145426989596,12.3257517152861));
#35630=CARTESIAN_POINT('Ctrl Pts',(0.100875941008522,1.71929827154436,12.3267956779336));
#35631=CARTESIAN_POINT('Ctrl Pts',(0.120497123297663,1.7256133906281,12.3278396405812));
#35632=CARTESIAN_POINT('Ctrl Pts',(0.140082210307686,1.73191689236979,12.328881682747));
#35633=CARTESIAN_POINT('Ctrl Pts',(0.159210918328371,1.73977407958339,12.3299237249127));
#35634=CARTESIAN_POINT('Ctrl Pts',(0.17762457728834,1.74909488527076,12.3309657670785));
#35635=CARTESIAN_POINT('Ctrl Pts',(0.196018460267855,1.75840568055925,12.3320066901074));
#35636=CARTESIAN_POINT('Ctrl Pts',(0.213698152554131,1.7691766689096,12.3330476131362));
#35637=CARTESIAN_POINT('Ctrl Pts',(0.230426290902619,1.78127031129676,12.3340885361651));
#35638=CARTESIAN_POINT('Ctrl Pts',(0.247163020386969,1.79337016466345,12.3351299937849));
#35639=CARTESIAN_POINT('Ctrl Pts',(0.262946613915361,1.80679361110466,12.3361714514047));
#35640=CARTESIAN_POINT('Ctrl Pts',(0.277569500059795,1.82136033549303,12.3372129090244));
#35641=CARTESIAN_POINT('Ctrl Pts',(0.292196854133464,1.83593151065078,12.3382546848549));
#35642=CARTESIAN_POINT('Ctrl Pts',(0.305662299505186,1.85164611470455,12.3392964606854));
#35643=CARTESIAN_POINT('Ctrl Pts',(0.317796497797404,1.86828837752995,12.3403382365159));
#35644=CARTESIAN_POINT('Ctrl Pts',(0.329956924434584,1.88496661298409,12.3413822641685));
#35645=CARTESIAN_POINT('Ctrl Pts',(0.340779973523657,1.90257588296395,12.3424262918211));
#35646=CARTESIAN_POINT('Ctrl Pts',(0.350140303761709,1.92087250997779,12.3434703194737));
#35647=CARTESIAN_POINT('Ctrl Pts',(0.353450929874014,1.92734378712492,12.3438395783696));
#35648=CARTESIAN_POINT('Ctrl Pts',(0.356579013654895,1.93390085399953,12.3442088372655));
#35649=CARTESIAN_POINT('Ctrl Pts',(0.35952046919734,1.94053237874689,12.3445780961613));
#35650=CARTESIAN_POINT('Ctrl Pts',(0.367836503692704,1.95928091591162,12.3456220588089));
#35651=CARTESIAN_POINT('Ctrl Pts',(0.374706799095974,1.97873757286482,12.3466660214564));
#35652=CARTESIAN_POINT('Ctrl Pts',(0.38001823440743,1.99865390230571,12.347709984104));
#35653=CARTESIAN_POINT('Ctrl Pts',(0.38531989876129,2.0185335935125,12.3487520262698));
#35654=CARTESIAN_POINT('Ctrl Pts',(0.389068150359415,2.03887059111312,12.3497940684355));
#35655=CARTESIAN_POINT('Ctrl Pts',(0.391198696362921,2.05939864578673,12.3508361106013));
#35656=CARTESIAN_POINT('Ctrl Pts',(0.393326954193488,2.0799046536521,12.3518770336302));
#35657=CARTESIAN_POINT('Ctrl Pts',(0.393840851226927,2.10060058608385,12.352917956659));
#35658=CARTESIAN_POINT('Ctrl Pts',(0.392727543724899,2.12121241145669,12.3539588796879));
#35659=CARTESIAN_POINT('Ctrl Pts',(0.391613664457153,2.14183482252585,12.3550003373077));
#35660=CARTESIAN_POINT('Ctrl Pts',(0.388870934719196,2.16237230466497,12.3560417949275));
#35661=CARTESIAN_POINT('Ctrl Pts',(0.384538604533982,2.18255272026443,12.3570832525472));
#35662=CARTESIAN_POINT('Ctrl Pts',(0.380204950633023,2.20273930186065,12.3581250283777));
#35663=CARTESIAN_POINT('Ctrl Pts',(0.374280919069172,2.22256788853888,12.3591668042082));
#35664=CARTESIAN_POINT('Ctrl Pts',(0.366856267302736,2.24177929729232,12.3602085800387));
#35665=CARTESIAN_POINT('Ctrl Pts',(0.35941556698302,2.26103223194173,12.3612526076913));
#35666=CARTESIAN_POINT('Ctrl Pts',(0.350468089532821,2.27966466141527,12.3622966353439));
#35667=CARTESIAN_POINT('Ctrl Pts',(0.340150873838033,2.29743928947204,12.3633406629965));
#35668=CARTESIAN_POINT('Ctrl Pts',(0.336501809882322,2.30372594243024,12.3637099218924));
#35669=CARTESIAN_POINT('Ctrl Pts',(0.332681798925405,2.30990555005749,12.3640791807883));
#35670=CARTESIAN_POINT('Ctrl Pts',(0.328698157218337,2.31596854271229,12.3644484396841));
#35671=CARTESIAN_POINT('Ctrl Pts',(0.317435671222777,2.3331097353413,12.3654924023317));
#35672=CARTESIAN_POINT('Ctrl Pts',(0.304795180737228,2.34941864269302,12.3665363649792));
#35673=CARTESIAN_POINT('Ctrl Pts',(0.290924350259353,2.36466566159246,12.3675803276268));
#35674=CARTESIAN_POINT('Ctrl Pts',(0.277079036668816,2.37988463195767,12.3686223697926));
#35675=CARTESIAN_POINT('Ctrl Pts',(0.262008321281486,2.39404501327894,12.3696644119583));
#35676=CARTESIAN_POINT('Ctrl Pts',(0.245901268417969,2.40694862141804,12.3707064541241));
#35677=CARTESIAN_POINT('Ctrl Pts',(0.229811514276188,2.41983837128471,12.371747377153));
#35678=CARTESIAN_POINT('Ctrl Pts',(0.212688185489378,2.43147354728851,12.3727883001818));
#35679=CARTESIAN_POINT('Ctrl Pts',(0.194754740206817,2.4416950119141,12.3738292232107));
#35680=CARTESIAN_POINT('Ctrl Pts',(0.176812084774155,2.45192172601751,12.3748706808305));
#35681=CARTESIAN_POINT('Ctrl Pts',(0.158059112915481,2.46073289991761,12.3759121384503));
#35682=CARTESIAN_POINT('Ctrl Pts',(0.138745889552052,2.46801422273115,12.37695359607));
#35683=CARTESIAN_POINT('Ctrl Pts',(0.119426765156904,2.47529777030624,12.3779953719005));
#35684=CARTESIAN_POINT('Ctrl Pts',(0.0995477491332538,2.48105031074997,
12.379037147731));
#35685=CARTESIAN_POINT('Ctrl Pts',(0.0793753545288147,2.4852070132973,12.3800789235615));
#35686=CARTESIAN_POINT('Ctrl Pts',(0.0591593568356653,2.48937270065151,
12.3811229512141));
#35687=CARTESIAN_POINT('Ctrl Pts',(0.0386494453176911,2.49193557215298,
12.3821669788667));
#35688=CARTESIAN_POINT('Ctrl Pts',(0.0181193245279482,2.49288239980769,
12.3832110065193));
#35689=CARTESIAN_POINT('Ctrl Pts',(0.0108580899083783,2.49321728033838,
12.3835802654152));
#35690=CARTESIAN_POINT('Ctrl Pts',(0.00359432421909314,2.49335047999792,
12.3839495243111));
#35691=CARTESIAN_POINT('Ctrl Pts',(-0.00365996579511119,2.49328297020133,
12.3843187832069));
#35692=CARTESIAN_POINT('Ctrl Pts',(-0.0241691746296765,2.49309210762017,
12.3853627458545));
#35693=CARTESIAN_POINT('Ctrl Pts',(-0.0447245218309344,2.49129206313246,
12.386406708502));
#35694=CARTESIAN_POINT('Ctrl Pts',(-0.0650530194777359,2.48788270734441,
12.3874506711496));
#35695=CARTESIAN_POINT('Ctrl Pts',(-0.0853441206626011,2.48447962343371,
12.3884927133154));
#35696=CARTESIAN_POINT('Ctrl Pts',(-0.105408473360152,2.47947316637522,
12.3895347554811));
#35697=CARTESIAN_POINT('Ctrl Pts',(-0.124977096865666,2.47291502417981,
12.3905767976469));
#35698=CARTESIAN_POINT('Ctrl Pts',(-0.144524703976956,2.46636392532609,
12.3916177206758));
#35699=CARTESIAN_POINT('Ctrl Pts',(-0.163576935552843,2.45826465490463,
12.3926586437046));
#35700=CARTESIAN_POINT('Ctrl Pts',(-0.181879023987313,2.44871895651573,
12.3936995667335));
#35701=CARTESIAN_POINT('Ctrl Pts',(-0.200190511897392,2.43916835570493,
12.3947410243533));
#35702=CARTESIAN_POINT('Ctrl Pts',(-0.217750427183038,2.42817016884568,
12.395782481973));
#35703=CARTESIAN_POINT('Ctrl Pts',(-0.234327290546682,2.41587277645446,
12.3968239395928));
#35704=CARTESIAN_POINT('Ctrl Pts',(-0.250909218864775,2.40357162667374,
12.3978657154233));
#35705=CARTESIAN_POINT('Ctrl Pts',(-0.266506928430191,2.38997094816352,
12.3989074912538));
#35706=CARTESIAN_POINT('Ctrl Pts',(-0.280921640046613,2.37525973580152,
12.3999492670843));
#35707=CARTESIAN_POINT('Ctrl Pts',(-0.295367509389291,2.36051672482017,
12.4009932947369));
#35708=CARTESIAN_POINT('Ctrl Pts',(-0.308624803329615,2.34465895265043,
12.4020373223895));
#35709=CARTESIAN_POINT('Ctrl Pts',(-0.320534238313284,2.32790939442884,
12.4030813500421));
#35710=CARTESIAN_POINT('Ctrl Pts',(-0.324746449361074,2.32198529523495,
12.403450608938));
#35711=CARTESIAN_POINT('Ctrl Pts',(-0.328790453635197,2.31594989437262,
12.4038198678338));
#35712=CARTESIAN_POINT('Ctrl Pts',(-0.332660568450896,2.30981381317236,
12.4041891267297));
#35713=CARTESIAN_POINT('Ctrl Pts',(-0.343883239717833,2.29202022681716,
12.4052599143931));
#35714=CARTESIAN_POINT('Ctrl Pts',(-0.353704393768988,2.27327671702817,
12.4063307020566));
#35715=CARTESIAN_POINT('Ctrl Pts',(-0.361970923399411,2.25382438237606,
12.40740148972));
#35716=CARTESIAN_POINT('Ctrl Pts',(-0.370218634500474,2.23441633043353,
12.4084698397645));
#35717=CARTESIAN_POINT('Ctrl Pts',(-0.376918430054792,2.21430325676297,
12.409538189809));
#35718=CARTESIAN_POINT('Ctrl Pts',(-0.381962909938574,2.19375086896268,
12.4106065398535));
#35719=CARTESIAN_POINT('Ctrl Pts',(-0.386997980238035,2.17323681800393,
12.4116728970801));
#35720=CARTESIAN_POINT('Ctrl Pts',(-0.390383670121265,2.15228573180286,
12.4127392543067));
#35721=CARTESIAN_POINT('Ctrl Pts',(-0.392062200302088,2.13117885652627,
12.4138056115333));
#35722=CARTESIAN_POINT('Ctrl Pts',(-0.392890184717364,2.12076726906489,
12.414331623621));
#35723=CARTESIAN_POINT('Ctrl Pts',(-0.393303551202367,2.1103179756868,12.4148576357088));
#35724=CARTESIAN_POINT('Ctrl Pts',(-0.393299977006061,2.09986551196329,
12.4153836477965));
#35725=CARTESIAN_POINT('',(-0.393390187309037,2.09970304505391,12.5403836071275));
#35726=CARTESIAN_POINT('Ctrl Pts',(-0.392695458149876,2.09986380011846,
12.4153837444951));
#35727=CARTESIAN_POINT('Ctrl Pts',(-0.392870617776604,2.04248652105401,
12.4182756530809));
#35728=CARTESIAN_POINT('Ctrl Pts',(-0.354200996982992,1.85392122723629,
12.4277910095078));
#35729=CARTESIAN_POINT('Ctrl Pts',(-0.0630108380886311,1.63923468580215,
12.4439298137753));
#35730=CARTESIAN_POINT('Ctrl Pts',(0.353310820705713,1.79759876908859,12.4638001572982));
#35731=CARTESIAN_POINT('Ctrl Pts',(0.445517900427544,2.23337481352617,12.4836705008209));
#35732=CARTESIAN_POINT('Ctrl Pts',(0.129022958292381,2.5467976238947,12.5035408443436));
#35733=CARTESIAN_POINT('Ctrl Pts',(-0.284692123815817,2.45503358678244,
12.5224451756817));
#35734=CARTESIAN_POINT('Ctrl Pts',(-0.392699784792383,2.21126854754101,
12.534726059179));
#35735=CARTESIAN_POINT('Ctrl Pts',(-0.393639516850345,2.09970507070382,
12.5403834948351));
#35736=CARTESIAN_POINT('',(-0.393391798196894,2.10029574838795,12.6653836890739));
#35737=CARTESIAN_POINT('Ctrl Pts',(-0.393299887339814,2.09970231142193,
12.5403836477965));
#35738=CARTESIAN_POINT('Ctrl Pts',(-0.3932854820339,2.08067032426963,12.5413496089941));
#35739=CARTESIAN_POINT('Ctrl Pts',(-0.391889466207624,2.06168959049348,
12.5423155701917));
#35740=CARTESIAN_POINT('Ctrl Pts',(-0.389134880197745,2.04291291727994,
12.5432815313893));
#35741=CARTESIAN_POINT('Ctrl Pts',(-0.386157861130145,2.02262002608602,
12.5443254940369));
#35742=CARTESIAN_POINT('Ctrl Pts',(-0.381580325228403,2.00250016963069,
12.5453694566844));
#35743=CARTESIAN_POINT('Ctrl Pts',(-0.375439253030338,1.9828238194682,12.546413419332));
#35744=CARTESIAN_POINT('Ctrl Pts',(-0.369309477996323,1.96318366607209,
12.5474554614977));
#35745=CARTESIAN_POINT('Ctrl Pts',(-0.36162203596023,1.94398611163449,12.5484975036635));
#35746=CARTESIAN_POINT('Ctrl Pts',(-0.352464699157093,1.92549061386819,
12.5495395458292));
#35747=CARTESIAN_POINT('Ctrl Pts',(-0.343317197189826,1.90701497997595,
12.5505804688581));
#35748=CARTESIAN_POINT('Ctrl Pts',(-0.332703233336234,1.88924057476259,
12.5516213918869));
#35749=CARTESIAN_POINT('Ctrl Pts',(-0.320758238726044,1.87240597044438,
12.5526623149158));
#35750=CARTESIAN_POINT('Ctrl Pts',(-0.308807109477952,1.85556272031216,
12.5537037725355));
#35751=CARTESIAN_POINT('Ctrl Pts',(-0.295523996459302,1.83966084471345,
12.5547452301553));
#35752=CARTESIAN_POINT('Ctrl Pts',(-0.281087369111873,1.82490950411589,
12.5557866877751));
#35753=CARTESIAN_POINT('Ctrl Pts',(-0.266646330745397,1.81015365634067,
12.5568284636056));
#35754=CARTESIAN_POINT('Ctrl Pts',(-0.251051616466253,1.79654954350039,
12.557870239436));
#35755=CARTESIAN_POINT('Ctrl Pts',(-0.234517487980402,1.78426840856297,
12.5589120152665));
#35756=CARTESIAN_POINT('Ctrl Pts',(-0.21794762060063,1.77196072767368,12.5599560429191));
#35757=CARTESIAN_POINT('Ctrl Pts',(-0.200434909090465,1.76098212501383,
12.5610000705717));
#35758=CARTESIAN_POINT('Ctrl Pts',(-0.182221911142592,1.75146009539862,
12.5620440982243));
#35759=CARTESIAN_POINT('Ctrl Pts',(-0.17578021249898,1.74809227833564,12.5624133571202));
#35760=CARTESIAN_POINT('Ctrl Pts',(-0.169251110582697,1.74490623654066,
12.5627826160161));
#35761=CARTESIAN_POINT('Ctrl Pts',(-0.162645900612064,1.74190615613489,
12.563151874912));
#35762=CARTESIAN_POINT('Ctrl Pts',(-0.143971760151691,1.73342437839599,
12.5641958375595));
#35763=CARTESIAN_POINT('Ctrl Pts',(-0.124576721715779,1.72638201069807,
12.5652398002071));
#35764=CARTESIAN_POINT('Ctrl Pts',(-0.104708220863087,1.72089437028226,
12.5662837628547));
#35765=CARTESIAN_POINT('Ctrl Pts',(-0.0848762702586617,1.71541682497231,
12.5673258050204));
#35766=CARTESIAN_POINT('Ctrl Pts',(-0.0645732714895317,1.71148858078031,
12.5683678471862));
#35767=CARTESIAN_POINT('Ctrl Pts',(-0.0440648939428253,1.70917628638757,
12.569409889352));
#35768=CARTESIAN_POINT('Ctrl Pts',(-0.0235785420714202,1.70686647536269,
12.5704508123808));
#35769=CARTESIAN_POINT('Ctrl Pts',(-0.00288797351194347,1.70616927950223,
12.5714917354097));
#35770=CARTESIAN_POINT('Ctrl Pts',(0.0177329046270695,1.70709996933891,
12.5725326584386));
#35771=CARTESIAN_POINT('Ctrl Pts',(0.038364373111642,1.70803113715363,12.5735741160583));
#35772=CARTESIAN_POINT('Ctrl Pts',(0.0589253439161157,1.71059184381556,
12.5746155736781));
#35773=CARTESIAN_POINT('Ctrl Pts',(0.0791433424408346,1.71474525136308,
12.5756570312979));
#35774=CARTESIAN_POINT('Ctrl Pts',(0.0993675184455364,1.71889992795769,
12.5766988071285));
#35775=CARTESIAN_POINT('Ctrl Pts',(0.119247800712942,1.72464809084637,12.577740582959));
#35776=CARTESIAN_POINT('Ctrl Pts',(0.138524221356739,1.73190228186321,12.5787823587895));
#35777=CARTESIAN_POINT('Ctrl Pts',(0.157842308421191,1.73917215297855,12.5798263864421));
#35778=CARTESIAN_POINT('Ctrl Pts',(0.176553261277886,1.7479542383803,12.5808704140947));
#35779=CARTESIAN_POINT('Ctrl Pts',(0.194418579141684,1.75811360646477,12.5819144417473));
#35780=CARTESIAN_POINT('Ctrl Pts',(0.200737307895772,1.76170684178966,12.5822837006431));
#35781=CARTESIAN_POINT('Ctrl Pts',(0.206950509720769,1.76547196558809,12.582652959539));
#35782=CARTESIAN_POINT('Ctrl Pts',(0.213048550545228,1.76940174666133,12.5830222184349));
#35783=CARTESIAN_POINT('Ctrl Pts',(0.230288830780609,1.78051195876333,12.5840661810824));
#35784=CARTESIAN_POINT('Ctrl Pts',(0.246709064381734,1.79300749345407,12.58511014373));
#35785=CARTESIAN_POINT('Ctrl Pts',(0.262078349208762,1.80674272579182,12.5861541063775));
#35786=CARTESIAN_POINT('Ctrl Pts',(0.277419360580215,1.82045269068964,12.5871961485433));
#35787=CARTESIAN_POINT('Ctrl Pts',(0.291712678715274,1.8353973860074,12.5882381907091));
#35788=CARTESIAN_POINT('Ctrl Pts',(0.30475845256979,1.85138951030323,12.5892802328748));
#35789=CARTESIAN_POINT('Ctrl Pts',(0.317790215468133,1.8673644593088,12.5903211559037));
#35790=CARTESIAN_POINT('Ctrl Pts',(0.329576608846557,1.88438405508869,12.5913620789325));
#35791=CARTESIAN_POINT('Ctrl Pts',(0.339956522100723,1.90222625785717,12.5924030019614));
#35792=CARTESIAN_POINT('Ctrl Pts',(0.350341766207803,1.92007762391596,12.5934444595812));
#35793=CARTESIAN_POINT('Ctrl Pts',(0.359318703208209,1.93875181308501,12.594485917201));
#35794=CARTESIAN_POINT('Ctrl Pts',(0.366770811695528,1.95799978278818,12.5955273748208));
#35795=CARTESIAN_POINT('Ctrl Pts',(0.374225197126873,1.97725363358524,12.5965691506513));
#35796=CARTESIAN_POINT('Ctrl Pts',(0.38015359485801,1.99708091529422,12.5976109264818));
#35797=CARTESIAN_POINT('Ctrl Pts',(0.384488815966542,2.01721569957627,12.5986527023123));
#35798=CARTESIAN_POINT('Ctrl Pts',(0.388833407753879,2.03739400565147,12.5996967299648));
#35799=CARTESIAN_POINT('Ctrl Pts',(0.39157784997706,2.05788041133163,12.6007407576174));
#35800=CARTESIAN_POINT('Ctrl Pts',(0.39270649075991,2.07840133997127,12.60178478527));
#35801=CARTESIAN_POINT('Ctrl Pts',(0.393105676210853,2.08565932344772,12.6021540441659));
#35802=CARTESIAN_POINT('Ctrl Pts',(0.393303211122216,2.09292162432936,12.6025233030618));
#35803=CARTESIAN_POINT('Ctrl Pts',(0.393299960518412,2.10017622773788,12.6028925619576));
#35804=CARTESIAN_POINT('Ctrl Pts',(0.39329077046506,2.12068632259594,12.6039365246052));
#35805=CARTESIAN_POINT('Ctrl Pts',(0.391672870315327,2.14125680770998,12.6049804872527));
#35806=CARTESIAN_POINT('Ctrl Pts',(0.388443712627104,2.16161470701441,12.6060244499003));
#35807=CARTESIAN_POINT('Ctrl Pts',(0.385220495322409,2.18193515576939,12.607066492066));
#35808=CARTESIAN_POINT('Ctrl Pts',(0.380391959294063,2.2020430671794,12.6081085342318));
#35809=CARTESIAN_POINT('Ctrl Pts',(0.37400740796664,2.22166901325348,12.6091505763976));
#35810=CARTESIAN_POINT('Ctrl Pts',(0.367629713547045,2.24127388136979,12.6101914994264));
#35811=CARTESIAN_POINT('Ctrl Pts',(0.359699520392321,2.26039710667069,12.6112324224553));
#35812=CARTESIAN_POINT('Ctrl Pts',(0.350316311448575,2.27878303032745,12.6122733454842));
#35813=CARTESIAN_POINT('Ctrl Pts',(0.340928283533272,2.2971783965154,12.6133148031039));
#35814=CARTESIAN_POINT('Ctrl Pts',(0.330086069131397,2.31483504189024,12.6143562607237));
#35815=CARTESIAN_POINT('Ctrl Pts',(0.317935992557206,2.33152018192085,12.6153977183435));
#35816=CARTESIAN_POINT('Ctrl Pts',(0.305782203604921,2.34821041998915,12.616439494174));
#35817=CARTESIAN_POINT('Ctrl Pts',(0.292320218959994,2.36392798879112,12.6174812700045));
#35818=CARTESIAN_POINT('Ctrl Pts',(0.277737265353293,2.37847244286298,12.618523045835));
#35819=CARTESIAN_POINT('Ctrl Pts',(0.263122790361445,2.39304833510237,12.6195670734876));
#35820=CARTESIAN_POINT('Ctrl Pts',(0.247383069833464,2.4064455728217,12.6206111011402));
#35821=CARTESIAN_POINT('Ctrl Pts',(0.23073965926772,2.41850290366183,12.6216551287928));
#35822=CARTESIAN_POINT('Ctrl Pts',(0.224853103108243,2.42276742353553,12.6220243876887));
#35823=CARTESIAN_POINT('Ctrl Pts',(0.218853759716514,2.42686472911455,12.6223936465846));
#35824=CARTESIAN_POINT('Ctrl Pts',(0.212752199670672,2.43078904385619,12.6227629054804));
#35825=CARTESIAN_POINT('Ctrl Pts',(0.195501969951427,2.44188380163538,12.623806868128));
#35826=CARTESIAN_POINT('Ctrl Pts',(0.177330139180993,2.4516586174993,12.6248508307755));
#35827=CARTESIAN_POINT('Ctrl Pts',(0.158464851546329,2.45996358263636,12.6258947934231));
#35828=CARTESIAN_POINT('Ctrl Pts',(0.13963426864112,2.46825326989513,12.6269368355889));
#35829=CARTESIAN_POINT('Ctrl Pts',(0.120113402909539,2.47507812612367,12.6279788777546));
#35830=CARTESIAN_POINT('Ctrl Pts',(0.100155483064891,2.48033376028436,12.6290209199204));
#35831=CARTESIAN_POINT('Ctrl Pts',(0.080218997712619,2.48558374997652,12.6300618429493));
#35832=CARTESIAN_POINT('Ctrl Pts',(0.0598470906458656,2.48926764897692,
12.6311027659781));
#35833=CARTESIAN_POINT('Ctrl Pts',(0.039308576301513,2.49133071158439,12.632143689007));
#35834=CARTESIAN_POINT('Ctrl Pts',(0.018759513911499,2.49339483372705,12.6331851466268));
#35835=CARTESIAN_POINT('Ctrl Pts',(-0.00195559621317298,2.4938363669115,
12.6342266042466));
#35836=CARTESIAN_POINT('Ctrl Pts',(-0.0225618166756512,2.49265233276818,
12.6352680618664));
#35837=CARTESIAN_POINT('Ctrl Pts',(-0.0431743332368318,2.49146793685081,
12.6363098376969));
#35838=CARTESIAN_POINT('Ctrl Pts',(-0.0636771620298553,2.48865706312374,
12.6373516135274));
#35839=CARTESIAN_POINT('Ctrl Pts',(-0.0838004157075394,2.4842686304231,
12.6383933893579));
#35840=CARTESIAN_POINT('Ctrl Pts',(-0.103967166254713,2.47987071202559,
12.6394374170105));
#35841=CARTESIAN_POINT('Ctrl Pts',(-0.123751998718944,2.47388864004582,
12.640481444663));
#35842=CARTESIAN_POINT('Ctrl Pts',(-0.142899397235013,2.466421413498,12.6415254723156));
#35843=CARTESIAN_POINT('Ctrl Pts',(-0.14967158111068,2.46378035334663,12.6418947312115));
#35844=CARTESIAN_POINT('Ctrl Pts',(-0.156364221980266,2.46095394355193,
12.6422639901074));
#35845=CARTESIAN_POINT('Ctrl Pts',(-0.162966740778297,2.45794794509831,
12.6426332490032));
#35846=CARTESIAN_POINT('Ctrl Pts',(-0.181633272802725,2.44944943595106,
12.6436772116508));
#35847=CARTESIAN_POINT('Ctrl Pts',(-0.199688853333332,2.43946151973071,
12.6447211742983));
#35848=CARTESIAN_POINT('Ctrl Pts',(-0.216883937786604,2.42809487580603,
12.6457651369459));
#35849=CARTESIAN_POINT('Ctrl Pts',(-0.234047390029146,2.41674914204768,
12.6468071791117));
#35850=CARTESIAN_POINT('Ctrl Pts',(-0.250352848681105,2.40403006662534,
12.6478492212774));
#35851=CARTESIAN_POINT('Ctrl Pts',(-0.265575462610926,2.39009406002018,
12.6488912634432));
#35852=CARTESIAN_POINT('Ctrl Pts',(-0.280781727692532,2.37617302046718,
12.6499321864721));
#35853=CARTESIAN_POINT('Ctrl Pts',(-0.294906897322246,2.36103811735178,
12.6509731095009));
#35854=CARTESIAN_POINT('Ctrl Pts',(-0.307759426222471,2.34488573982822,
12.6520140325298));
#35855=CARTESIAN_POINT('Ctrl Pts',(-0.320618555846558,2.32872506686456,
12.6530554901495));
#35856=CARTESIAN_POINT('Ctrl Pts',(-0.332203268262198,2.31154644127121,
12.6540969477693));
#35857=CARTESIAN_POINT('Ctrl Pts',(-0.342362230622209,2.29357942308878,
12.6551384053891));
#35858=CARTESIAN_POINT('Ctrl Pts',(-0.35252429698812,2.27560691519899,12.6561801812196));
#35859=CARTESIAN_POINT('Ctrl Pts',(-0.361259415719716,2.25684619292158,
12.6572219570501));
#35860=CARTESIAN_POINT('Ctrl Pts',(-0.368462623752698,2.23755066302013,
12.6582637328806));
#35861=CARTESIAN_POINT('Ctrl Pts',(-0.375681401683303,2.21821342539294,
12.6593077605332));
#35862=CARTESIAN_POINT('Ctrl Pts',(-0.381361455759539,2.19833978036997,
12.6603517881858));
#35863=CARTESIAN_POINT('Ctrl Pts',(-0.385447710770332,2.17819816022075,
12.6613958158384));
#35864=CARTESIAN_POINT('Ctrl Pts',(-0.386892965606033,2.17107433318533,
12.6617650747343));
#35865=CARTESIAN_POINT('Ctrl Pts',(-0.388139317076599,2.1639170542226,12.6621343336301));
#35866=CARTESIAN_POINT('Ctrl Pts',(-0.389185882481578,2.15673833692518,
12.662503592526));
#35867=CARTESIAN_POINT('Ctrl Pts',(-0.391906797485739,2.13807473547968,
12.6634636109495));
#35868=CARTESIAN_POINT('Ctrl Pts',(-0.393285629476647,2.1192108351539,12.664423629373));
#35869=CARTESIAN_POINT('Ctrl Pts',(-0.393299888242884,2.10029649306013,
12.6653836477965));
#35870=CARTESIAN_POINT('',(-0.393077839436675,2.10013693750963,12.7903836117785));
#35871=CARTESIAN_POINT('Ctrl Pts',(-0.393642737751318,2.10029371522729,
12.6653838017726));
#35872=CARTESIAN_POINT('Ctrl Pts',(-0.392704612486157,1.98861543350834,
12.6710471798646));
#35873=CARTESIAN_POINT('Ctrl Pts',(-0.284503920525053,1.74474015797601,
12.6833340057978));
#35874=CARTESIAN_POINT('Ctrl Pts',(0.129423303771996,1.6533181793209,12.7022442795714));
#35875=CARTESIAN_POINT('Ctrl Pts',(0.445637245252665,1.9670244904942,12.7221146230944));
#35876=CARTESIAN_POINT('Ctrl Pts',(0.353039682245798,2.40271772865816,12.7419849666171));
#35877=CARTESIAN_POINT('Ctrl Pts',(-0.0634237272071889,2.56070866207559,
12.7618553101399));
#35878=CARTESIAN_POINT('Ctrl Pts',(-0.354314217530218,2.34584041188345,
12.7779881712589));
#35879=CARTESIAN_POINT('Ctrl Pts',(-0.39287385494239,2.15739695435976,12.787497584537));
#35880=CARTESIAN_POINT('Ctrl Pts',(-0.392696668310428,2.10013803163933,
12.7903835499741));
#35881=CARTESIAN_POINT('',(-0.393299839860298,2.09964508330049,12.9153836477965));
#35882=CARTESIAN_POINT('Ctrl Pts',(-0.393299976382332,2.10013629987835,
12.7903836477965));
#35883=CARTESIAN_POINT('Ctrl Pts',(-0.393307320618343,2.07894414707162,
12.7914501378907));
#35884=CARTESIAN_POINT('Ctrl Pts',(-0.391597482747587,2.0577651672122,12.7925166279849));
#35885=CARTESIAN_POINT('Ctrl Pts',(-0.388202863252538,2.03688560415776,
12.7935831180791));
#35886=CARTESIAN_POINT('Ctrl Pts',(-0.384805099452868,2.01598670117238,
12.7946505960218));
#35887=CARTESIAN_POINT('Ctrl Pts',(-0.379719606119362,1.99538843537396,
12.7957180739645));
#35888=CARTESIAN_POINT('Ctrl Pts',(-0.373029699516558,1.97536560154361,
12.7967855519072));
#35889=CARTESIAN_POINT('Ctrl Pts',(-0.366320071011017,1.95528374022532,
12.7978561767842));
#35890=CARTESIAN_POINT('Ctrl Pts',(-0.357996851840173,1.93578133184653,
12.7989268016611));
#35891=CARTESIAN_POINT('Ctrl Pts',(-0.348191675533187,1.9171135677821,12.799997426538));
#35892=CARTESIAN_POINT('Ctrl Pts',(-0.34331157626416,1.90782250162348,12.8005302834205));
#35893=CARTESIAN_POINT('Ctrl Pts',(-0.338065089716678,1.89873778525007,
12.8010631403031));
#35894=CARTESIAN_POINT('Ctrl Pts',(-0.332472410414027,1.8898881576077,12.8015959971856));
#35895=CARTESIAN_POINT('Ctrl Pts',(-0.321515343921992,1.87255014245255,
12.8026399598332));
#35896=CARTESIAN_POINT('Ctrl Pts',(-0.309165745435914,1.85601987094724,
12.8036839224809));
#35897=CARTESIAN_POINT('Ctrl Pts',(-0.295567188915755,1.84052952607967,
12.8047278851286));
#35898=CARTESIAN_POINT('Ctrl Pts',(-0.281993648405637,1.82506767737067,
12.8057699272944));
#35899=CARTESIAN_POINT('Ctrl Pts',(-0.267176145730319,1.81064254388779,
12.8068119694603));
#35900=CARTESIAN_POINT('Ctrl Pts',(-0.25130020475716,1.79745562790062,12.8078540116262));
#35901=CARTESIAN_POINT('Ctrl Pts',(-0.235441314295202,1.78428287445405,
12.8088949346552));
#35902=CARTESIAN_POINT('Ctrl Pts',(-0.21852678689345,1.77234618847189,12.8099358576841));
#35903=CARTESIAN_POINT('Ctrl Pts',(-0.200777226552667,1.76180864100658,
12.8109767807131));
#35904=CARTESIAN_POINT('Ctrl Pts',(-0.183018550500336,1.75126568173155,
12.812018238333));
#35905=CARTESIAN_POINT('Ctrl Pts',(-0.164424609212882,1.74212368596976,
12.8130596959529));
#35906=CARTESIAN_POINT('Ctrl Pts',(-0.145243403381224,1.73450137650842,
12.8141011535728));
#35907=CARTESIAN_POINT('Ctrl Pts',(-0.126056336854973,1.72687673809925,
12.8151429294034));
#35908=CARTESIAN_POINT('Ctrl Pts',(-0.106282345125238,1.72077294822902,
12.816184705234));
#35909=CARTESIAN_POINT('Ctrl Pts',(-0.0861867509570695,1.71625954870582,
12.8172264810646));
#35910=CARTESIAN_POINT('Ctrl Pts',(-0.066047719706139,1.71173639336713,
12.8182705087173));
#35911=CARTESIAN_POINT('Ctrl Pts',(-0.0455864272438703,1.70881059575511,
12.81931453637));
#35912=CARTESIAN_POINT('Ctrl Pts',(-0.0250763008431699,1.70750023040004,
12.8203585640227));
#35913=CARTESIAN_POINT('Ctrl Pts',(-0.0178221379903036,1.70703677135075,
12.8207278229179));
#35914=CARTESIAN_POINT('Ctrl Pts',(-0.0105618717355667,1.70677491668709,
12.8210970818131));
#35915=CARTESIAN_POINT('Ctrl Pts',(-0.00330752414799727,1.70671390784314,
12.8214663407083));
#35916=CARTESIAN_POINT('Ctrl Pts',(0.0172018474903776,1.70654142464756,
12.8225103033557));
#35917=CARTESIAN_POINT('Ctrl Pts',(0.0377858565357733,1.70797705351697,
12.8235542660032));
#35918=CARTESIAN_POINT('Ctrl Pts',(0.0581715601962042,1.71102575974193,
12.8245982286506));
#35919=CARTESIAN_POINT('Ctrl Pts',(0.0785197621580826,1.71406885754328,
12.8256402708162));
#35920=CARTESIAN_POINT('Ctrl Pts',(0.0986696545932957,1.71871909368904,
12.8266823129819));
#35921=CARTESIAN_POINT('Ctrl Pts',(0.118351383364296,1.72492955320932,12.8277243551475));
#35922=CARTESIAN_POINT('Ctrl Pts',(0.138011974267798,1.73113334279365,12.8287652781763));
#35923=CARTESIAN_POINT('Ctrl Pts',(0.157204692866169,1.73889383646972,12.829806201205));
#35924=CARTESIAN_POINT('Ctrl Pts',(0.175673009167233,1.74811381975115,12.8308471242337));
#35925=CARTESIAN_POINT('Ctrl Pts',(0.194150810314275,1.75733853817572,12.8318885818534));
#35926=CARTESIAN_POINT('Ctrl Pts',(0.211902800420434,1.76802392942791,12.8329300394731));
#35927=CARTESIAN_POINT('Ctrl Pts',(0.22869490798557,1.78002573687643,12.8339714970928));
#35928=CARTESIAN_POINT('Ctrl Pts',(0.245492146271674,1.79203121140039,12.8350132729231));
#35929=CARTESIAN_POINT('Ctrl Pts',(0.261328341094543,1.80535344593764,12.8360550487535));
#35930=CARTESIAN_POINT('Ctrl Pts',(0.27600139645014,1.81980699659418,12.8370968245839));
#35931=CARTESIAN_POINT('Ctrl Pts',(0.290706167947926,1.83429178892853,12.8381408522364));
#35932=CARTESIAN_POINT('Ctrl Pts',(0.304242298286553,1.84991222285872,12.8391848798889));
#35933=CARTESIAN_POINT('Ctrl Pts',(0.316446578954081,1.86644817990806,12.8402289075414));
#35934=CARTESIAN_POINT('Ctrl Pts',(0.320763073064432,1.87229673117929,12.840598166438));
#35935=CARTESIAN_POINT('Ctrl Pts',(0.324913358478234,1.87825954639764,12.8409674253346));
#35936=CARTESIAN_POINT('Ctrl Pts',(0.328891565248036,1.88432610656666,12.8413366842311));
#35937=CARTESIAN_POINT('Ctrl Pts',(0.340138685655048,1.90147738517673,12.8423806468785));
#35938=CARTESIAN_POINT('Ctrl Pts',(0.350074079222775,1.91956192037248,12.843424609526));
#35939=CARTESIAN_POINT('Ctrl Pts',(0.358545822180928,1.93835290476905,12.8444685721734));
#35940=CARTESIAN_POINT('Ctrl Pts',(0.367001980455002,1.95710932112493,12.845510614339));
#35941=CARTESIAN_POINT('Ctrl Pts',(0.373999479504436,1.97656896830518,12.8465526565046));
#35942=CARTESIAN_POINT('Ctrl Pts',(0.37943168935525,1.99647955219851,12.8475946986702));
#35943=CARTESIAN_POINT('Ctrl Pts',(0.384858065098019,2.01636875243751,12.8486356216989));
#35944=CARTESIAN_POINT('Ctrl Pts',(0.388722268436086,2.03670722931816,12.8496765447276));
#35945=CARTESIAN_POINT('Ctrl Pts',(0.39096717473016,2.05722666387203,12.8507174677563));
#35946=CARTESIAN_POINT('Ctrl Pts',(0.393213233949594,2.07775663667264,12.851758925376));
#35947=CARTESIAN_POINT('Ctrl Pts',(0.393838238672249,2.09846702314922,12.8528003829956));
#35948=CARTESIAN_POINT('Ctrl Pts',(0.392836775324064,2.11908292307251,12.8538418406152));
#35949=CARTESIAN_POINT('Ctrl Pts',(0.391835005985166,2.13970512205198,12.8548836164456));
#35950=CARTESIAN_POINT('Ctrl Pts',(0.389205851059815,2.1602320444683,12.8559253922759));
#35951=CARTESIAN_POINT('Ctrl Pts',(0.384995836875683,2.18039338025231,12.8569671681063));
#35952=CARTESIAN_POINT('Ctrl Pts',(0.38077672265035,2.20059829522116,12.8580111957587));
#35953=CARTESIAN_POINT('Ctrl Pts',(0.374970134062881,2.22043533909527,12.8590552234111));
#35954=CARTESIAN_POINT('Ctrl Pts',(0.367672802953046,2.23964812912693,12.8600992510636));
#35955=CARTESIAN_POINT('Ctrl Pts',(0.365091832584362,2.24644344114239,12.8604685099604));
#35956=CARTESIAN_POINT('Ctrl Pts',(0.36232481527227,2.25316085504905,12.8608377688571));
#35957=CARTESIAN_POINT('Ctrl Pts',(0.359377418068716,2.25978974116715,12.8612070277539));
#35958=CARTESIAN_POINT('Ctrl Pts',(0.351044585421646,2.27853081841046,12.8622509904022));
#35959=CARTESIAN_POINT('Ctrl Pts',(0.341216992486097,2.29667416089257,12.8632949530506));
#35960=CARTESIAN_POINT('Ctrl Pts',(0.330003103890568,2.3139692534515,12.8643389156989));
#35961=CARTESIAN_POINT('Ctrl Pts',(0.318809844451445,2.33123252982406,12.8653809578654));
#35962=CARTESIAN_POINT('Ctrl Pts',(0.306235697347738,2.34765001095391,12.866423000032));
#35963=CARTESIAN_POINT('Ctrl Pts',(0.292435075254193,2.36299546908849,12.8674650421985));
#35964=CARTESIAN_POINT('Ctrl Pts',(0.278649274811979,2.37832444644209,12.8685059652281));
#35965=CARTESIAN_POINT('Ctrl Pts',(0.263640082374575,2.39258312282989,12.8695468882577));
#35966=CARTESIAN_POINT('Ctrl Pts',(0.247602182735681,2.40557822092637,12.8705878112874));
#35967=CARTESIAN_POINT('Ctrl Pts',(0.231556046449694,2.41857999296641,12.8716292689079));
#35968=CARTESIAN_POINT('Ctrl Pts',(0.214480709023903,2.43031641454184,12.8726707265285));
#35969=CARTESIAN_POINT('Ctrl Pts',(0.196604381027897,2.44063412536127,12.873712184149));
#35970=CARTESIAN_POINT('Ctrl Pts',(0.178722591034438,2.45095498869111,12.8747539599803));
#35971=CARTESIAN_POINT('Ctrl Pts',(0.160039978057417,2.4598559421548,12.8757957358115));
#35972=CARTESIAN_POINT('Ctrl Pts',(0.140809009184932,2.46722978219687,12.8768375116428));
#35973=CARTESIAN_POINT('Ctrl Pts',(0.121536472137206,2.47461956096137,12.8778815392961));
#35974=CARTESIAN_POINT('Ctrl Pts',(0.10171391913597,2.48047542758616,12.8789255669495));
#35975=CARTESIAN_POINT('Ctrl Pts',(0.0816092840789526,2.48473993132,12.8799695946028));
#35976=CARTESIAN_POINT('Ctrl Pts',(0.0744985382792814,2.48624823037279,
12.8803388534941));
#35977=CARTESIAN_POINT('Ctrl Pts',(0.0673525800331886,2.48755793017658,
12.8807081123853));
#35978=CARTESIAN_POINT('Ctrl Pts',(0.0601834146428161,2.48866804165242,
12.8810773712766));
#35979=CARTESIAN_POINT('Ctrl Pts',(0.0399148685066659,2.49180653050562,
12.8821213339231));
#35980=CARTESIAN_POINT('Ctrl Pts',(0.0193397677068456,2.49336463352435,
12.8831652965696));
#35981=CARTESIAN_POINT('Ctrl Pts',(-0.00127253626072525,2.49329794132625,
12.8842092592161));
#35982=CARTESIAN_POINT('Ctrl Pts',(-0.021846921674124,2.49323137181563,
12.8852513013808));
#35983=CARTESIAN_POINT('Ctrl Pts',(-0.0424576467489466,2.49154588299042,
12.8862933435455));
#35984=CARTESIAN_POINT('Ctrl Pts',(-0.0628309087702101,2.48824884662174,
12.8873353857102));
#35985=CARTESIAN_POINT('Ctrl Pts',(-0.0831822902282565,2.4849553512183,
12.888376308738));
#35986=CARTESIAN_POINT('Ctrl Pts',(-0.103295987665238,2.48005383267414,
12.8894172317658));
#35987=CARTESIAN_POINT('Ctrl Pts',(-0.122904103649506,2.4736033609406,12.8904581547936));
#35988=CARTESIAN_POINT('Ctrl Pts',(-0.142522289851617,2.46714957641273,
12.8914996124124));
#35989=CARTESIAN_POINT('Ctrl Pts',(-0.161633671903684,2.45914546407377,
12.8925410700312));
#35990=CARTESIAN_POINT('Ctrl Pts',(-0.179985767222745,2.44969989075955,
12.89358252765));
#35991=CARTESIAN_POINT('Ctrl Pts',(-0.198343469907265,2.44025143141075,
12.8946243034795));
#35992=CARTESIAN_POINT('Ctrl Pts',(-0.215940786907783,2.4293610028965,12.8956660793089));
#35993=CARTESIAN_POINT('Ctrl Pts',(-0.232550914559593,2.4171828528428,12.8967078551384));
#35994=CARTESIAN_POINT('Ctrl Pts',(-0.249196945379844,2.40497837944097,
12.8977518827901));
#35995=CARTESIAN_POINT('Ctrl Pts',(-0.264850968986824,2.3914811084241,12.8987959104417));
#35996=CARTESIAN_POINT('Ctrl Pts',(-0.279319642300925,2.37688522428054,
12.8998399380933));
#35997=CARTESIAN_POINT('Ctrl Pts',(-0.284437022490672,2.37172285128706,
12.9002091969954));
#35998=CARTESIAN_POINT('Ctrl Pts',(-0.289406478001018,2.3664233656682,12.9005784558974));
#35999=CARTESIAN_POINT('Ctrl Pts',(-0.294220678509066,2.36099632629151,
12.9009477147994));
#36000=CARTESIAN_POINT('Ctrl Pts',(-0.307707358188683,2.34579281709828,
12.9019821703694));
#36001=CARTESIAN_POINT('Ctrl Pts',(-0.320056576268256,2.32949124904495,
12.9030166259395));
#36002=CARTESIAN_POINT('Ctrl Pts',(-0.331086220149197,2.31228943644778,
12.9040510815095));
#36003=CARTESIAN_POINT('Ctrl Pts',(-0.3420960322969,2.29511855338582,12.9050836770877));
#36004=CARTESIAN_POINT('Ctrl Pts',(-0.351790522206156,2.27705122675409,
12.9061162726659));
#36005=CARTESIAN_POINT('Ctrl Pts',(-0.360028444154879,2.2583174323927,12.9071488682442));
#36006=CARTESIAN_POINT('Ctrl Pts',(-0.368257398146856,2.23960403199214,
12.9081803397194));
#36007=CARTESIAN_POINT('Ctrl Pts',(-0.375032603801925,2.22022627634804,
12.9092118111947));
#36008=CARTESIAN_POINT('Ctrl Pts',(-0.380259424142445,2.20043734539929,
12.91024328267));
#36009=CARTESIAN_POINT('Ctrl Pts',(-0.38548888546593,2.18063841559347,12.9112752753222));
#36010=CARTESIAN_POINT('Ctrl Pts',(-0.389168195733384,2.16042861870346,
12.9123072679745));
#36011=CARTESIAN_POINT('Ctrl Pts',(-0.391252958431796,2.14007508600573,
12.9133392606268));
#36012=CARTESIAN_POINT('Ctrl Pts',(-0.39262960328261,2.12663490597684,12.9140207230167));
#36013=CARTESIAN_POINT('Ctrl Pts',(-0.393312010835634,2.11313231187333,
12.9147021854066));
#36014=CARTESIAN_POINT('Ctrl Pts',(-0.393299839860298,2.09964508330049,
12.9153836477965));
#36015=CARTESIAN_POINT('',(-0.393541630724459,2.10004216970008,13.0403836477965));
#36016=CARTESIAN_POINT('Ctrl Pts',(-0.393142733542287,2.09964376269932,
12.9153837217147));
#36017=CARTESIAN_POINT('Ctrl Pts',(-0.393455688614957,2.06380637641479,
12.9171951672506));
#36018=CARTESIAN_POINT('Ctrl Pts',(-0.372521700895207,1.8972908910741,12.9256300606271));
#36019=CARTESIAN_POINT('Ctrl Pts',(-0.136917627666675,1.65555809852058,
12.9406884018452));
#36020=CARTESIAN_POINT('Ctrl Pts',(0.299578723250621,1.74429277563225,12.9605587453678));
#36021=CARTESIAN_POINT('Ctrl Pts',(0.461252377310549,2.15934040607319,12.9804290888907));
#36022=CARTESIAN_POINT('Ctrl Pts',(0.19978977333452,2.5199512921437,13.0002994324134));
#36023=CARTESIAN_POINT('Ctrl Pts',(-0.244952757047327,2.49531403938879,
13.0201697759362));
#36024=CARTESIAN_POINT('Ctrl Pts',(-0.392908567496978,2.23489280799354,
13.0335311810639));
#36025=CARTESIAN_POINT('Ctrl Pts',(-0.39394771448153,2.10229571354889,13.0402691383507));
#36026=CARTESIAN_POINT('Ctrl Pts',(-0.393944288396229,2.1000422128466,13.0403836477965));
#36027=CARTESIAN_POINT('',(-0.393238269502415,2.10033186658782,13.1653836447486));
#36028=CARTESIAN_POINT('Ctrl Pts',(-0.393299997742054,2.10004214380805,
13.0403836477965));
#36029=CARTESIAN_POINT('Ctrl Pts',(-0.393302189049272,2.07959213788605,
13.0414244974294));
#36030=CARTESIAN_POINT('Ctrl Pts',(-0.391705092139561,2.05907940249458,
13.0424653470622));
#36031=CARTESIAN_POINT('Ctrl Pts',(-0.388505413481191,2.03877554658628,
13.0435061966951));
#36032=CARTESIAN_POINT('Ctrl Pts',(-0.385311597575711,2.01850889331693,
13.0445451391851));
#36033=CARTESIAN_POINT('Ctrl Pts',(-0.380521082138016,1.99845109263691,
13.0455840816752));
#36034=CARTESIAN_POINT('Ctrl Pts',(-0.374182434352757,1.97887033467459,
13.0466230241652));
#36035=CARTESIAN_POINT('Ctrl Pts',(-0.367850471108373,1.95931022597083,
13.0476608710188));
#36036=CARTESIAN_POINT('Ctrl Pts',(-0.359973815974987,1.9402268713692,13.0486987178724));
#36037=CARTESIAN_POINT('Ctrl Pts',(-0.350651231867759,1.92187475308193,
13.049736564726));
#36038=CARTESIAN_POINT('Ctrl Pts',(-0.341323709487897,1.90351291348107,
13.0507749613382));
#36039=CARTESIAN_POINT('Ctrl Pts',(-0.330549051033115,1.88588375069158,
13.0518133579503));
#36040=CARTESIAN_POINT('Ctrl Pts',(-0.318472847162838,1.86921885774614,
13.0528517545625));
#36041=CARTESIAN_POINT('Ctrl Pts',(-0.306392475521783,1.85254821336966,
13.0538905095488));
#36042=CARTESIAN_POINT('Ctrl Pts',(-0.293010130277935,1.83684307719353,
13.0549292645352));
#36043=CARTESIAN_POINT('Ctrl Pts',(-0.278512250093498,1.82230265296936,
13.0559680195215));
#36044=CARTESIAN_POINT('Ctrl Pts',(-0.263983526389957,1.80773129471575,
13.0570089844074));
#36045=CARTESIAN_POINT('Ctrl Pts',(-0.248335096783645,1.79433007213102,
13.0580499492932));
#36046=CARTESIAN_POINT('Ctrl Pts',(-0.231787549495608,1.78225887597162,
13.0590909141791));
#36047=CARTESIAN_POINT('Ctrl Pts',(-0.227444936614511,1.77909100275031,
13.0593640971133));
#36048=CARTESIAN_POINT('Ctrl Pts',(-0.223040549547636,1.77601449326531,
13.0596372800476));
#36049=CARTESIAN_POINT('Ctrl Pts',(-0.218578668352261,1.77303172058845,
13.0599104629818));
#36050=CARTESIAN_POINT('Ctrl Pts',(-0.201527694796042,1.76163312528515,
13.0609544251097));
#36051=CARTESIAN_POINT('Ctrl Pts',(-0.183531882943273,1.75153793738519,
13.0619983872377));
#36052=CARTESIAN_POINT('Ctrl Pts',(-0.164816685327661,1.74290008367741,
13.0630423493656));
#36053=CARTESIAN_POINT('Ctrl Pts',(-0.14613591633572,1.73427812023275,13.0640843910126));
#36054=CARTESIAN_POINT('Ctrl Pts',(-0.126739024042769,1.72710852830456,
13.0651264326597));
#36055=CARTESIAN_POINT('Ctrl Pts',(-0.10687734793002,1.72150016842878,13.0661684743068));
#36056=CARTESIAN_POINT('Ctrl Pts',(-0.0870370029068725,1.71589783183251,
13.0672093968195));
#36057=CARTESIAN_POINT('Ctrl Pts',(-0.0667335616766056,1.71185362533106,
13.0682503193322));
#36058=CARTESIAN_POINT('Ctrl Pts',(-0.0462348264664314,1.70942704801584,
13.0692912418449));
#36059=CARTESIAN_POINT('Ctrl Pts',(-0.0257255634438634,1.70699922445052,
13.0703326989583));
#36060=CARTESIAN_POINT('Ctrl Pts',(-0.00502153484719317,1.70619079230346,
13.0713741560716));
#36061=CARTESIAN_POINT('Ctrl Pts',(0.015602418044393,1.70700959992492,13.072415613185));
#36062=CARTESIAN_POINT('Ctrl Pts',(0.0362326725539908,1.70782865773183,
13.073457388514));
#36063=CARTESIAN_POINT('Ctrl Pts',(0.056782069505377,1.71027587979938,13.074499163843));
#36064=CARTESIAN_POINT('Ctrl Pts',(0.0769798975387362,1.7143071359554,13.075540939172));
#36065=CARTESIAN_POINT('Ctrl Pts',(0.0972213839447773,1.71834710582476,
13.076584966338));
#36066=CARTESIAN_POINT('Ctrl Pts',(0.117109075645695,1.72397774490345,13.077628993504));
#36067=CARTESIAN_POINT('Ctrl Pts',(0.136385743363226,1.73110459611529,13.0786730206699));
#36068=CARTESIAN_POINT('Ctrl Pts',(0.143203707534823,1.73362529196017,13.0790422826148));
#36069=CARTESIAN_POINT('Ctrl Pts',(0.149945423373895,1.73633272053559,13.0794115445597));
#36070=CARTESIAN_POINT('Ctrl Pts',(0.15660021115429,1.73922130901835,13.0797808065045));
#36071=CARTESIAN_POINT('Ctrl Pts',(0.175414365851484,1.74738781294976,13.0808247693751));
#36072=CARTESIAN_POINT('Ctrl Pts',(0.193644049227042,1.75705431354917,13.0818687322457));
#36073=CARTESIAN_POINT('Ctrl Pts',(0.211037795122978,1.76811456942247,13.0829126951163));
#36074=CARTESIAN_POINT('Ctrl Pts',(0.228399543248293,1.77915447869921,13.0839547374986));
#36075=CARTESIAN_POINT('Ctrl Pts',(0.244927760586449,1.79158271370629,13.084996779881));
#36076=CARTESIAN_POINT('Ctrl Pts',(0.260394860435468,1.80524687167259,13.0860388222633));
#36077=CARTESIAN_POINT('Ctrl Pts',(0.275845348761198,1.81889635445864,13.0870797455017));
#36078=CARTESIAN_POINT('Ctrl Pts',(0.290236414266017,1.83377866206034,13.0881206687401));
#36079=CARTESIAN_POINT('Ctrl Pts',(0.303373062655239,1.84970082929586,13.0891615919785));
#36080=CARTESIAN_POINT('Ctrl Pts',(0.316516457524256,1.86563117354704,13.0902030497953));
#36081=CARTESIAN_POINT('Ctrl Pts',(0.328403667579282,1.88260188702379,13.091244507612));
#36082=CARTESIAN_POINT('Ctrl Pts',(0.33887931702491,1.90038612650236,13.0922859654287));
#36083=CARTESIAN_POINT('Ctrl Pts',(0.349358167166871,1.91817579972042,13.0933277414491));
#36084=CARTESIAN_POINT('Ctrl Pts',(0.358424256170585,1.93677884197119,13.0943695174695));
#36085=CARTESIAN_POINT('Ctrl Pts',(0.365968148299018,1.95594374560406,13.0954112934899));
#36086=CARTESIAN_POINT('Ctrl Pts',(0.373528346623202,1.97515007436137,13.0964553213193));
#36087=CARTESIAN_POINT('Ctrl Pts',(0.379559564362063,1.99491998470172,13.0974993491486));
#36088=CARTESIAN_POINT('Ctrl Pts',(0.384001979624431,2.01498606205734,13.098543376978));
#36089=CARTESIAN_POINT('Ctrl Pts',(0.385573198246311,2.02208314608645,13.0989126346611));
#36090=CARTESIAN_POINT('Ctrl Pts',(0.386946138599605,2.02921720008482,13.0992818923442));
#36091=CARTESIAN_POINT('Ctrl Pts',(0.388119705309467,2.03637622810229,13.0996511500273));
#36092=CARTESIAN_POINT('Ctrl Pts',(0.391437609261143,2.05661620862466,13.1006951141375));
#36093=CARTESIAN_POINT('Ctrl Pts',(0.393177899969202,2.07717673006261,13.1017390782477));
#36094=CARTESIAN_POINT('Ctrl Pts',(0.393293784326227,2.09778884411339,13.1027830423579));
#36095=CARTESIAN_POINT('Ctrl Pts',(0.393409455502914,2.1183630402123,13.1038250859964));
#36096=CARTESIAN_POINT('Ctrl Pts',(0.391906588329872,2.13898791341175,13.1048671296349));
#36097=CARTESIAN_POINT('Ctrl Pts',(0.388790129405108,2.15938960580067,13.1059091732735));
#36098=CARTESIAN_POINT('Ctrl Pts',(0.385677017488246,2.17976938722356,13.1069500977802));
#36099=CARTESIAN_POINT('Ctrl Pts',(0.380953836115718,2.1999257356621,13.1079910222869));
#36100=CARTESIAN_POINT('Ctrl Pts',(0.374677280338413,2.21959024039699,13.1090319467936));
#36101=CARTESIAN_POINT('Ctrl Pts',(0.36839750114873,2.23926484411135,13.1100734058816));
#36102=CARTESIAN_POINT('Ctrl Pts',(0.360562962183608,2.25844639365872,13.1111148649695));
#36103=CARTESIAN_POINT('Ctrl Pts',(0.351280289951746,2.27688145151886,13.1121563240575));
#36104=CARTESIAN_POINT('Ctrl Pts',(0.341994781496254,2.29532214201854,13.1131981013524));
#36105=CARTESIAN_POINT('Ctrl Pts',(0.331260621878094,2.31301524643091,13.1142398786473));
#36106=CARTESIAN_POINT('Ctrl Pts',(0.319230044069069,2.32973260317957,13.1152816559422));
#36107=CARTESIAN_POINT('Ctrl Pts',(0.307173462249178,2.34648609437941,13.1163256850316));
#36108=CARTESIAN_POINT('Ctrl Pts',(0.293815343749129,2.36225906524756,13.1173697141209));
#36109=CARTESIAN_POINT('Ctrl Pts',(0.279348153227717,2.37685645971923,13.1184137432102));
#36110=CARTESIAN_POINT('Ctrl Pts',(0.274231426314988,2.3820192369038,13.1187829933235));
#36111=CARTESIAN_POINT('Ctrl Pts',(0.26897628854097,2.38703531663029,13.1191522434368));
#36112=CARTESIAN_POINT('Ctrl Pts',(0.263592232763096,2.3918972847201,13.1195214935501));
#36113=CARTESIAN_POINT('Ctrl Pts',(0.248370213741312,2.40564323643377,13.1205654523203));
#36114=CARTESIAN_POINT('Ctrl Pts',(0.232024695912387,2.41823623162151,13.1216094110905));
#36115=CARTESIAN_POINT('Ctrl Pts',(0.214756483154807,2.42949133970862,13.1226533698606));
#36116=CARTESIAN_POINT('Ctrl Pts',(0.197520037206229,2.4407257427654,13.1236954081519));
#36117=CARTESIAN_POINT('Ctrl Pts',(0.179364842576409,2.45062669703958,13.1247374464431));
#36118=CARTESIAN_POINT('Ctrl Pts',(0.160523839093104,2.45905011778693,13.1257794847343));
#36119=CARTESIAN_POINT('Ctrl Pts',(0.141703070347353,2.46746449200403,13.1268204039041));
#36120=CARTESIAN_POINT('Ctrl Pts',(0.122198611456366,2.47440415774629,13.1278613230739));
#36121=CARTESIAN_POINT('Ctrl Pts',(0.102266834682567,2.47977148987781,13.1289022422437));
#36122=CARTESIAN_POINT('Ctrl Pts',(0.0823248201470075,2.48514157888686,
13.1299436960714));
#36123=CARTESIAN_POINT('Ctrl Pts',(0.061955755525126,2.48893751396757,13.1309851498991));
#36124=CARTESIAN_POINT('Ctrl Pts',(0.0414304522452797,2.49111175848695,
13.1320266037268));
#36125=CARTESIAN_POINT('Ctrl Pts',(0.0208988768998916,2.49328666740597,
13.133068375799));
#36126=CARTESIAN_POINT('Ctrl Pts',(0.000211702737125122,2.49383885777713,
13.1341101478713));
#36127=CARTESIAN_POINT('Ctrl Pts',(-0.0203568237301628,2.49277282203281,
13.1351519199436));
#36128=CARTESIAN_POINT('Ctrl Pts',(-0.0409698117976874,2.49170448191073,
13.1361959439445));
#36129=CARTESIAN_POINT('Ctrl Pts',(-0.0614629099310601,2.48901102804192,
13.1372399679454));
#36130=CARTESIAN_POINT('Ctrl Pts',(-0.0815679292918496,2.48474870098681,
13.1382839919463));
#36131=CARTESIAN_POINT('Ctrl Pts',(-0.0886792752952678,2.48324107336783,
13.1386532736552));
#36132=CARTESIAN_POINT('Ctrl Pts',(-0.095742191761906,2.48153762390391,
13.1390225553641));
#36133=CARTESIAN_POINT('Ctrl Pts',(-0.102745303105613,2.47964232204766,
13.1393918370729));
#36134=CARTESIAN_POINT('Ctrl Pts',(-0.122543211064429,2.47428427333719,
13.1404358023798));
#36135=CARTESIAN_POINT('Ctrl Pts',(-0.141979855005472,2.46735743365101,
13.1414797676867));
#36136=CARTESIAN_POINT('Ctrl Pts',(-0.160791040950966,2.45893053805702,
13.1425237329936));
#36137=CARTESIAN_POINT('Ctrl Pts',(-0.179567620997308,2.45051914495714,
13.1435657777751));
#36138=CARTESIAN_POINT('Ctrl Pts',(-0.197720338777932,2.44061341671961,
13.1446078225567));
#36139=CARTESIAN_POINT('Ctrl Pts',(-0.215001948648293,2.42933121940903,
13.1456498673383));
#36140=CARTESIAN_POINT('Ctrl Pts',(-0.232264997538626,2.41806113952503,
13.1466907929318));
#36141=CARTESIAN_POINT('Ctrl Pts',(-0.248658167111771,2.40541790144835,
13.1477317185253));
#36142=CARTESIAN_POINT('Ctrl Pts',(-0.263960591461509,2.39156422303721,
13.1487726441188));
#36143=CARTESIAN_POINT('Ctrl Pts',(-0.279270873193604,2.37770343113569,
13.1498141041995));
#36144=CARTESIAN_POINT('Ctrl Pts',(-0.293488734540599,2.36263143908251,
13.1508555642802));
#36145=CARTESIAN_POINT('Ctrl Pts',(-0.306427608728904,2.34655021924283,
13.1518970243609));
#36146=CARTESIAN_POINT('Ctrl Pts',(-0.319370435593064,2.33046408677717,
13.1529388025956));
#36147=CARTESIAN_POINT('Ctrl Pts',(-0.331033064811712,2.3133687082097,13.1539805808302));
#36148=CARTESIAN_POINT('Ctrl Pts',(-0.341270816983217,2.29549710861189,
13.1550223590649));
#36149=CARTESIAN_POINT('Ctrl Pts',(-0.351530697063042,2.27758688128498,
13.1560663890022));
#36150=CARTESIAN_POINT('Ctrl Pts',(-0.360359236985173,2.25889774933996,
13.1571104189395));
#36151=CARTESIAN_POINT('Ctrl Pts',(-0.367658547116141,2.23968565686014,
13.1581544488767));
#36152=CARTESIAN_POINT('Ctrl Pts',(-0.370240106983396,2.23289088228254,
13.1585236927831));
#36153=CARTESIAN_POINT('Ctrl Pts',(-0.372630839426149,2.22603083974788,
13.1588929366894));
#36154=CARTESIAN_POINT('Ctrl Pts',(-0.374827924988285,2.21911723909232,
13.1592621805957));
#36155=CARTESIAN_POINT('Ctrl Pts',(-0.382278322486661,2.19567296640825,
13.160514300187));
#36156=CARTESIAN_POINT('Ctrl Pts',(-0.387534363760182,2.17149952030509,
13.1617664197783));
#36157=CARTESIAN_POINT('Ctrl Pts',(-0.390484665621148,2.14697463054394,
13.1630185393695));
#36158=CARTESIAN_POINT('Ctrl Pts',(-0.392342255036592,2.13153310022531,
13.1638069075465));
#36159=CARTESIAN_POINT('Ctrl Pts',(-0.393286676415921,2.11595266695904,
13.1645952757234));
#36160=CARTESIAN_POINT('Ctrl Pts',(-0.393299859927403,2.10033193536341,
13.1653836439004));
#36161=CARTESIAN_POINT('',(-0.393168444855454,2.09979799896453,13.2903836510805));
#36162=CARTESIAN_POINT('Ctrl Pts',(-0.393016960555868,2.1003316194609,13.1653836477965));
#36163=CARTESIAN_POINT('Ctrl Pts',(-0.392294146464799,2.00958948971456,
13.1699666065705));
#36164=CARTESIAN_POINT('Ctrl Pts',(-0.31587487389345,1.7866046526642,13.1811730131854));
#36165=CARTESIAN_POINT('Ctrl Pts',(0.0552540808467619,1.63823999361116,
13.1990028676414));
#36166=CARTESIAN_POINT('Ctrl Pts',(0.41816195164139,1.89649844744964,13.2188732111641));
#36167=CARTESIAN_POINT('Ctrl Pts',(0.397474384784138,2.34144118050984,13.2387435546869));
#36168=CARTESIAN_POINT('Ctrl Pts',(0.0121365597886237,2.56489583068018,
13.2586138982096));
#36169=CARTESIAN_POINT('Ctrl Pts',(-0.331284324819889,2.3890171423689,13.2758272625795));
#36170=CARTESIAN_POINT('Ctrl Pts',(-0.392396098076996,2.17846515087843,
13.2864171791085));
#36171=CARTESIAN_POINT('Ctrl Pts',(-0.392766706913104,2.09979827052114,
13.2903836477965));
#36172=CARTESIAN_POINT('',(0.386061278380631,2.17511044757631,13.3566999406454));
#36173=CARTESIAN_POINT('Ctrl Pts',(-0.393299948079913,2.09979791007433,
13.2903836521554));
#36174=CARTESIAN_POINT('Ctrl Pts',(-0.393288194121441,2.07692279029185,
13.2915354796105));
#36175=CARTESIAN_POINT('Ctrl Pts',(-0.391276592848532,2.05411783564869,
13.2926873070656));
#36176=CARTESIAN_POINT('Ctrl Pts',(-0.387326160418207,2.03171138121407,
13.2938391345206));
#36177=CARTESIAN_POINT('Ctrl Pts',(-0.38334552455176,2.0091336159351,13.2949997683906));
#36178=CARTESIAN_POINT('Ctrl Pts',(-0.377396497655504,1.98696088882726,
13.2961604022605));
#36179=CARTESIAN_POINT('Ctrl Pts',(-0.369590783055106,1.96551006327344,
13.2973210361305));
#36180=CARTESIAN_POINT('Ctrl Pts',(-0.367273776316445,1.95914271449086,
13.2976655525054));
#36181=CARTESIAN_POINT('Ctrl Pts',(-0.364793491675445,1.95283882330262,
13.2980100688803));
#36182=CARTESIAN_POINT('Ctrl Pts',(-0.362153634920279,1.94660627550636,
13.2983545852552));
#36183=CARTESIAN_POINT('Ctrl Pts',(-0.354165085623896,1.92774577664974,
13.2993971365372));
#36184=CARTESIAN_POINT('Ctrl Pts',(-0.344675022130477,1.90945389785774,
13.3004396878193));
#36185=CARTESIAN_POINT('Ctrl Pts',(-0.33378684723082,1.8919826194384,13.3014822391013));
#36186=CARTESIAN_POINT('Ctrl Pts',(-0.322918758472639,1.87454357145008,
13.3025228671195));
#36187=CARTESIAN_POINT('Ctrl Pts',(-0.310658012177592,1.85792277018594,
13.3035634951377));
#36188=CARTESIAN_POINT('Ctrl Pts',(-0.297154417031168,1.84234879693883,
13.304604123156));
#36189=CARTESIAN_POINT('Ctrl Pts',(-0.283665320897661,1.8267915457007,13.3056436338363));
#36190=CARTESIAN_POINT('Ctrl Pts',(-0.268936483837422,1.81227946511035,
13.3066831445166));
#36191=CARTESIAN_POINT('Ctrl Pts',(-0.253158594444117,1.79900894355633,
13.3077226551969));
#36192=CARTESIAN_POINT('Ctrl Pts',(-0.237372305983092,1.7857313576855,13.3087627192415));
#36193=CARTESIAN_POINT('Ctrl Pts',(-0.220536403997549,1.77369713855338,
13.3098027832861));
#36194=CARTESIAN_POINT('Ctrl Pts',(-0.202875827346148,1.76306337587223,
13.3108428473307));
#36195=CARTESIAN_POINT('Ctrl Pts',(-0.185209694911656,1.75242626795043,
13.3118832385656));
#36196=CARTESIAN_POINT('Ctrl Pts',(-0.166719022153088,1.74319084209225,
13.3129236298006));
#36197=CARTESIAN_POINT('Ctrl Pts',(-0.147653809061824,1.73546846135137,
13.3139640210355));
#36198=CARTESIAN_POINT('Ctrl Pts',(-0.128546706716977,1.72772911333279,
13.3150066981727));
#36199=CARTESIAN_POINT('Ctrl Pts',(-0.108863248517147,1.72150966889204,
13.3160493753098));
#36200=CARTESIAN_POINT('Ctrl Pts',(-0.0888697560011624,1.71687201033037,
13.3170920524469));
#36201=CARTESIAN_POINT('Ctrl Pts',(-0.0816287307463324,1.71519239368803,
13.3174696778906));
#36202=CARTESIAN_POINT('Ctrl Pts',(-0.0743471254598987,1.71371976480426,
13.3178473033343));
#36203=CARTESIAN_POINT('Ctrl Pts',(-0.0670377807939903,1.71245538844384,
13.318224928778));
#36204=CARTESIAN_POINT('Ctrl Pts',(-0.0467922450206122,1.70895329926814,
13.3192708815657));
#36205=CARTESIAN_POINT('Ctrl Pts',(-0.0262122163330918,1.707031660208,13.3203168343534));
#36206=CARTESIAN_POINT('Ctrl Pts',(-0.00556709706753582,1.70673940264725,
13.3213627871411));
#36207=CARTESIAN_POINT('Ctrl Pts',(0.0150398900019641,1.70644768489557,
13.3224068080205));
#36208=CARTESIAN_POINT('Ctrl Pts',(0.0357110053059775,1.70777944339817,
13.3234508288999));
#36209=CARTESIAN_POINT('Ctrl Pts',(0.0561715495447083,1.7107319085492,13.3244948497794));
#36210=CARTESIAN_POINT('Ctrl Pts',(0.0766098110257722,1.71368115828892,
13.3255377336575));
#36211=CARTESIAN_POINT('Ctrl Pts',(0.0968372310438449,1.71824753486853,
13.3265806175357));
#36212=CARTESIAN_POINT('Ctrl Pts',(0.116584129853373,1.72437647748533,13.3276235014139));
#36213=CARTESIAN_POINT('Ctrl Pts',(0.136340226437917,1.73050827486103,13.3286668710499));
#36214=CARTESIAN_POINT('Ctrl Pts',(0.155614649935592,1.73820389117585,13.3297102406859));
#36215=CARTESIAN_POINT('Ctrl Pts',(0.174152259224977,1.7473587083071,13.3307536103219));
#36216=CARTESIAN_POINT('Ctrl Pts',(0.192695060688043,1.75651608959858,13.3317972721939));
#36217=CARTESIAN_POINT('Ctrl Pts',(0.210499995805076,1.76713313037676,13.3328409340659));
#36218=CARTESIAN_POINT('Ctrl Pts',(0.227336745970714,1.77905936073559,13.3338845959379));
#36219=CARTESIAN_POINT('Ctrl Pts',(0.244208748436968,1.79101056189067,13.334930442999));
#36220=CARTESIAN_POINT('Ctrl Pts',(0.260107954319876,1.80427595693448,13.33597629006));
#36221=CARTESIAN_POINT('Ctrl Pts',(0.27483673790471,1.81866451077424,13.3370221371211));
#36222=CARTESIAN_POINT('Ctrl Pts',(0.279874432996801,1.82358583687312,13.3373798488477));
#36223=CARTESIAN_POINT('Ctrl Pts',(0.284775536428784,1.82863824945768,13.3377375605743));
#36224=CARTESIAN_POINT('Ctrl Pts',(0.289533219254565,1.83381321417454,13.3380952723008));
#36225=CARTESIAN_POINT('Ctrl Pts',(0.303298904154541,1.84878624543143,13.3391302607802));
#36226=CARTESIAN_POINT('Ctrl Pts',(0.315943783334727,1.86487772602899,13.3401652492595));
#36227=CARTESIAN_POINT('Ctrl Pts',(0.327282668995372,1.88189235553226,13.3412002377389));
#36228=CARTESIAN_POINT('Ctrl Pts',(0.338601061227082,1.89887623350394,13.3422333556233));
#36229=CARTESIAN_POINT('Ctrl Pts',(0.348617681618409,1.91677936705804,13.3432664735076));
#36230=CARTESIAN_POINT('Ctrl Pts',(0.357187760401041,1.93537377541932,13.344299591392));
#36231=CARTESIAN_POINT('Ctrl Pts',(0.365759867841031,1.95397258533679,13.3453329538297));
#36232=CARTESIAN_POINT('Ctrl Pts',(0.372884379614551,1.97326234353729,13.3463663162675));
#36233=CARTESIAN_POINT('Ctrl Pts',(0.378462415407803,1.99299023351258,13.3473996787053));
#36234=CARTESIAN_POINT('Ctrl Pts',(0.384036418815935,2.01270386211471,13.3484322941211));
#36235=CARTESIAN_POINT('Ctrl Pts',(0.388065981863659,2.03285426537309,13.3494649095369));
#36236=CARTESIAN_POINT('Ctrl Pts',(0.390502626407998,2.0531749130438,13.3504975249528));
#36237=CARTESIAN_POINT('Ctrl Pts',(0.392944704640702,2.07354087551722,13.3515324430887));
#36238=CARTESIAN_POINT('Ctrl Pts',(0.393786700096242,2.09407709007872,13.3525673612246));
#36239=CARTESIAN_POINT('Ctrl Pts',(0.393032175547103,2.11451202896604,13.3536022793605));
#36240=CARTESIAN_POINT('Ctrl Pts',(0.392279374784967,2.13490028218605,13.3546348331221));
#36241=CARTESIAN_POINT('Ctrl Pts',(0.389937501447389,2.15518699244151,13.3556673868838));
#36242=CARTESIAN_POINT('Ctrl Pts',(0.386061278380631,2.17511044757631,13.3566999406454));
#36243=CARTESIAN_POINT('Ctrl Pts',(0.386061278380631,2.17511044757631,13.3567));
#36244=CARTESIAN_POINT('Ctrl Pts',(0.385531328553113,2.17769530268049,13.3567));
#36245=CARTESIAN_POINT('Ctrl Pts',(0.385001378725595,2.18028015778468,13.3567));
#36246=CARTESIAN_POINT('Ctrl Pts',(0.384471428898077,2.18286501288886,13.3567));
#36247=CARTESIAN_POINT('',(-0.3933,2.1,13.4067));
#36248=CARTESIAN_POINT('Origin',(0.,2.1,13.4067));
#36249=CARTESIAN_POINT('Origin',(0.,2.1,4.03722265507267));
#36250=CARTESIAN_POINT('',(-0.322274998938081,2.10002616218071,13.100028292361));
#36251=CARTESIAN_POINT('',(-0.304247867982273,1.99372483614108,13.3567));
#36252=CARTESIAN_POINT('Ctrl Pts',(-0.322274998940427,2.10002613326275,
13.1000282941516));
#36253=CARTESIAN_POINT('Ctrl Pts',(-0.322275002368696,2.09998385590746,
13.1000309118996));
#36254=CARTESIAN_POINT('Ctrl Pts',(-0.322274997477792,2.09994157852145,
13.1000335291818));
#36255=CARTESIAN_POINT('Ctrl Pts',(-0.322274843812231,2.09944978993456,
13.1000639690949));
#36256=CARTESIAN_POINT('Ctrl Pts',(-0.322273762884423,2.0990002763328,13.1000917395794));
#36257=CARTESIAN_POINT('Ctrl Pts',(-0.322263476054635,2.09671275874497,
13.1002327981922));
#36258=CARTESIAN_POINT('Ctrl Pts',(-0.322239486612913,2.09487480804254,
13.1003452742039));
#36259=CARTESIAN_POINT('Ctrl Pts',(-0.321507714129348,2.06101285841063,
13.1024032971133));
#36260=CARTESIAN_POINT('Ctrl Pts',(-0.316045174157482,2.02926498944136,
13.104112479787));
#36261=CARTESIAN_POINT('Ctrl Pts',(-0.300735410555515,1.98295606854878,
13.1068806919687));
#36262=CARTESIAN_POINT('Ctrl Pts',(-0.294255879988497,1.96750688529557,
13.1078528274757));
#36263=CARTESIAN_POINT('Ctrl Pts',(-0.286004525178468,1.95145934939636,
13.1089488438727));
#36264=CARTESIAN_POINT('Ctrl Pts',(-0.285394560335216,1.95029075461181,
13.1090291601988));
#36265=CARTESIAN_POINT('Ctrl Pts',(-0.284516939401083,1.94863422952304,
13.1091437417129));
#36266=CARTESIAN_POINT('Ctrl Pts',(-0.284255156766297,1.94814318874716,
13.1091777986978));
#36267=CARTESIAN_POINT('Ctrl Pts',(-0.283802169922842,1.94729877077789,
13.1092365240531));
#36268=CARTESIAN_POINT('Ctrl Pts',(-0.283611573614604,1.94694506748116,
13.1092611707669));
#36269=CARTESIAN_POINT('Ctrl Pts',(-0.283246264998223,1.94627016332486,
13.1093082920872));
#36270=CARTESIAN_POINT('Ctrl Pts',(-0.283071666396078,1.94594890132931,
13.1093307626127));
#36271=CARTESIAN_POINT('Ctrl Pts',(-0.282662705435276,1.94519945462188,
13.1093832767361));
#36272=CARTESIAN_POINT('Ctrl Pts',(-0.28242791671866,1.94477150471925,13.1094133355378));
#36273=CARTESIAN_POINT('Ctrl Pts',(-0.281618205814068,1.94330356129304,
13.1095166917221));
#36274=CARTESIAN_POINT('Ctrl Pts',(-0.28103850947434,1.94226622466587,13.1095901600136));
#36275=CARTESIAN_POINT('Ctrl Pts',(-0.27476257576315,1.93118019684787,13.1103799954219));
#36276=CARTESIAN_POINT('Ctrl Pts',(-0.26853643292989,1.92144264618825,13.1111155954051));
#36277=CARTESIAN_POINT('Ctrl Pts',(-0.259453713912288,1.9087902781968,13.1121309662091));
#36278=CARTESIAN_POINT('Ctrl Pts',(-0.257044660048004,1.90556381979863,
13.1123954170968));
#36279=CARTESIAN_POINT('Ctrl Pts',(-0.253968458756467,1.90160096071808,
13.1127270520547));
#36280=CARTESIAN_POINT('Ctrl Pts',(-0.253357455578584,1.90082129504387,
13.1127926350144));
#36281=CARTESIAN_POINT('Ctrl Pts',(-0.23874504855636,1.88235128025021,13.1143542303163));
#36282=CARTESIAN_POINT('Ctrl Pts',(-0.222929361289476,1.86617837262526,
13.11590202832));
#36283=CARTESIAN_POINT('Ctrl Pts',(-0.202226214283227,1.84903303288053,
13.1176948547406));
#36284=CARTESIAN_POINT('Ctrl Pts',(-0.19884178749188,1.84634313208145,13.1179811821564));
#36285=CARTESIAN_POINT('Ctrl Pts',(-0.190315934567189,1.83984242850949,
13.1186841043337));
#36286=CARTESIAN_POINT('Ctrl Pts',(-0.185112877733177,1.83611488722322,
13.1190971017542));
#36287=CARTESIAN_POINT('Ctrl Pts',(-0.178877127044097,1.83192278968225,
13.1195705224224));
#36288=CARTESIAN_POINT('Ctrl Pts',(-0.177949143736069,1.83130589957853,
13.119640429617));
#36289=CARTESIAN_POINT('Ctrl Pts',(-0.176712515090817,1.83049304972884,
13.1197328456181));
#36290=CARTESIAN_POINT('Ctrl Pts',(-0.176406723529106,1.83029279369831,
13.1197556381718));
#36291=CARTESIAN_POINT('Ctrl Pts',(-0.175929208574289,1.82998123941053,
13.1197911361329));
#36292=CARTESIAN_POINT('Ctrl Pts',(-0.175757719987975,1.82986958452437,
13.1198038655069));
#36293=CARTESIAN_POINT('Ctrl Pts',(-0.175410654143129,1.82964408305688,
13.1198295893424));
#36294=CARTESIAN_POINT('Ctrl Pts',(-0.175235073691105,1.82953024501472,
13.1198425831398));
#36295=CARTESIAN_POINT('Ctrl Pts',(-0.174832512429986,1.82926979992011,
13.1198723292715));
#36296=CARTESIAN_POINT('Ctrl Pts',(-0.174605458371492,1.82912330748837,
13.1198890738459));
#36297=CARTESIAN_POINT('Ctrl Pts',(-0.173937633682946,1.8286936239447,13.1199382280543));
#36298=CARTESIAN_POINT('Ctrl Pts',(-0.173496353764188,1.82841122015232,
13.1199705851969));
#36299=CARTESIAN_POINT('Ctrl Pts',(-0.170655059918173,1.82660264194096,
13.1201781513914));
#36300=CARTESIAN_POINT('Ctrl Pts',(-0.168235524922132,1.82510715841391,
13.1203513660593));
#36301=CARTESIAN_POINT('Ctrl Pts',(-0.146263235101439,1.81192515877966,
13.1218957105008));
#36302=CARTESIAN_POINT('Ctrl Pts',(-0.12553966536828,1.80230863438546,13.123152969081));
#36303=CARTESIAN_POINT('Ctrl Pts',(-0.0801845046078889,1.7868495092839,
13.1258331491801));
#36304=CARTESIAN_POINT('Ctrl Pts',(-0.0555340376343538,1.78155300784509,
13.1272548768699));
#36305=CARTESIAN_POINT('Ctrl Pts',(-0.0293712670059871,1.77906412332862,
13.1288529741022));
#36306=CARTESIAN_POINT('Ctrl Pts',(-0.0282214899131648,1.77896097478164,
13.1289233627152));
#36307=CARTESIAN_POINT('Ctrl Pts',(-0.0265459716102778,1.7788197315584,
13.1290261734174));
#36308=CARTESIAN_POINT('Ctrl Pts',(-0.0260206428446681,1.7787767449488,
13.1290584417069));
#36309=CARTESIAN_POINT('Ctrl Pts',(-0.025099767409725,1.778703665344,13.1291150665734));
#36310=CARTESIAN_POINT('Ctrl Pts',(-0.0247042651843215,1.77867301347875,
13.1291394055409));
#36311=CARTESIAN_POINT('Ctrl Pts',(-0.0239371262816572,1.77861498405498,
13.1291866528768));
#36312=CARTESIAN_POINT('Ctrl Pts',(-0.0235654965410722,1.77858752068477,
13.1292095585108));
#36313=CARTESIAN_POINT('Ctrl Pts',(-0.0226795762349534,1.778523596089,13.1292642044297));
#36314=CARTESIAN_POINT('Ctrl Pts',(-0.022165245357576,1.77848772442867,
13.1292959631807));
#36315=CARTESIAN_POINT('Ctrl Pts',(-0.0206141440500869,1.77838328357096,
13.1293918421999));
#36316=CARTESIAN_POINT('Ctrl Pts',(-0.0195771334775212,1.77831849443,13.1294560809539));
#36317=CARTESIAN_POINT('Ctrl Pts',(-0.00882555581054929,1.77769895160184,
13.1301235550778));
#36318=CARTESIAN_POINT('Ctrl Pts',(0.000908137531323761,1.77757946929876,
13.1307403894243));
#36319=CARTESIAN_POINT('Ctrl Pts',(0.0396114779545556,1.77885695122998,
13.1332464644097));
#36320=CARTESIAN_POINT('Ctrl Pts',(0.0683277008459709,1.78372044169004,
13.1352406106739));
#36321=CARTESIAN_POINT('Ctrl Pts',(0.101923147754386,1.79420372707678,13.1375914010035));
#36322=CARTESIAN_POINT('Ctrl Pts',(0.107793009829547,1.79622316732652,13.1380020943538));
#36323=CARTESIAN_POINT('Ctrl Pts',(0.118451622629756,1.80023800524931,13.1387435707093));
#36324=CARTESIAN_POINT('Ctrl Pts',(0.123257618230174,1.80218192235977,13.1390762569213));
#36325=CARTESIAN_POINT('Ctrl Pts',(0.128917104841652,1.80463154860443,13.1394643046045));
#36326=CARTESIAN_POINT('Ctrl Pts',(0.129817488808469,1.80502616783916,13.139525926346));
#36327=CARTESIAN_POINT('Ctrl Pts',(0.131034367354442,1.80556615095718,13.1396090402527));
#36328=CARTESIAN_POINT('Ctrl Pts',(0.131352440572687,1.80570791167876,13.1396307492936));
#36329=CARTESIAN_POINT('Ctrl Pts',(0.13185664158092,1.80593360718472,13.1396651363002));
#36330=CARTESIAN_POINT('Ctrl Pts',(0.132042919289206,1.80601720326092,13.1396778350777));
#36331=CARTESIAN_POINT('Ctrl Pts',(0.132426478835396,1.80618977185241,13.1397039711755));
#36332=CARTESIAN_POINT('Ctrl Pts',(0.132623750025104,1.80627876585039,13.13971740704));
#36333=CARTESIAN_POINT('Ctrl Pts',(0.133079752809487,1.8064850332405,13.1397484502752));
#36334=CARTESIAN_POINT('Ctrl Pts',(0.133338419930862,1.80660245043373,13.1397660487443));
#36335=CARTESIAN_POINT('Ctrl Pts',(0.134132668270098,1.8069642521859,13.1398200534769));
#36336=CARTESIAN_POINT('Ctrl Pts',(0.134667739178919,1.80720976411161,13.1398563905862));
#36337=CARTESIAN_POINT('Ctrl Pts',(0.138983883981192,1.80920451872364,13.1401491640672));
#36338=CARTESIAN_POINT('Ctrl Pts',(0.142731601938089,1.81102556211661,13.1404012727305));
#36339=CARTESIAN_POINT('Ctrl Pts',(0.172774049806691,1.82635053717589,13.1424134214274));
#36340=CARTESIAN_POINT('Ctrl Pts',(0.197135322277393,1.84334248799633,13.1440006445294));
#36341=CARTESIAN_POINT('Ctrl Pts',(0.231247387429444,1.87489678116242,13.1466382850647));
#36342=CARTESIAN_POINT('Ctrl Pts',(0.242730402707627,1.88732973862727,13.1476207852567));
#36343=CARTESIAN_POINT('Ctrl Pts',(0.253910992039204,1.90152642215609,13.1487194874641));
#36344=CARTESIAN_POINT('Ctrl Pts',(0.254632068482555,1.9024523788456,13.148791040873));
#36345=CARTESIAN_POINT('Ctrl Pts',(0.255671819258296,1.90380270626667,13.1488952402997));
#36346=CARTESIAN_POINT('Ctrl Pts',(0.255994534219415,1.90422396552286,13.1489277265531));
#36347=CARTESIAN_POINT('Ctrl Pts',(0.256557018170268,1.90496197838828,13.1489846047204));
#36348=CARTESIAN_POINT('Ctrl Pts',(0.256797245317798,1.90527838270614,13.14900897854));
#36349=CARTESIAN_POINT('Ctrl Pts',(0.257261074819815,1.90589164590104,13.1490561991587));
#36350=CARTESIAN_POINT('Ctrl Pts',(0.257484750028722,1.90618844913343,13.1490790430485));
#36351=CARTESIAN_POINT('Ctrl Pts',(0.258015219121175,1.90689488807573,13.1491333926211));
#36352=CARTESIAN_POINT('Ctrl Pts',(0.258321550915546,1.90730486805008,13.149164916309));
#36353=CARTESIAN_POINT('Ctrl Pts',(0.259401953665918,1.90875803419428,13.1492765894412));
#36354=CARTESIAN_POINT('Ctrl Pts',(0.260170684701439,1.90980515834106,13.1493569464142));
#36355=CARTESIAN_POINT('Ctrl Pts',(0.273056757340544,1.92758218595751,13.1507193709368));
#36356=CARTESIAN_POINT('Ctrl Pts',(0.28354192636524,1.94543099935899,13.1520653646861));
#36357=CARTESIAN_POINT('Ctrl Pts',(0.304068469423984,1.98959080521796,13.155329549031));
#36358=CARTESIAN_POINT('Ctrl Pts',(0.312520218092005,2.01645930589435,13.1572707371285));
#36359=CARTESIAN_POINT('Ctrl Pts',(0.317726993876248,2.0460132057395,13.1591756431431));
#36360=CARTESIAN_POINT('Ctrl Pts',(0.318049436064414,2.04794643846475,13.1592991715826));
#36361=CARTESIAN_POINT('Ctrl Pts',(0.318423607378717,2.05032323574633,13.1594496203989));
#36362=CARTESIAN_POINT('Ctrl Pts',(0.318492068609554,2.05076406920446,13.1594774647636));
#36363=CARTESIAN_POINT('Ctrl Pts',(0.31859147974066,2.05141307836185,13.1595183685132));
#36364=CARTESIAN_POINT('Ctrl Pts',(0.318623141064951,2.05162114205434,13.1595314681635));
#36365=CARTESIAN_POINT('Ctrl Pts',(0.318687011110921,2.0520436490427,13.1595580414137));
#36366=CARTESIAN_POINT('Ctrl Pts',(0.318719207152378,2.05225809345008,13.1595715142184));
#36367=CARTESIAN_POINT('Ctrl Pts',(0.318787251917256,2.05271444782472,13.1596001544743));
#36368=CARTESIAN_POINT('Ctrl Pts',(0.31882304162232,2.05295636534958,13.1596153184984));
#36369=CARTESIAN_POINT('Ctrl Pts',(0.318918332434982,2.05360557909043,13.1596559640351));
#36370=CARTESIAN_POINT('Ctrl Pts',(0.318977328901456,2.05401295067085,13.1596814168783));
#36371=CARTESIAN_POINT('Ctrl Pts',(0.319239256268139,2.05584631927787,13.1597957393549));
#36372=CARTESIAN_POINT('Ctrl Pts',(0.319433410440474,2.05727358264205,13.1598841193034));
#36373=CARTESIAN_POINT('Ctrl Pts',(0.323121445303702,2.08581651541562,13.1616400716805));
#36374=CARTESIAN_POINT('Ctrl Pts',(0.323161033818841,2.11327156868801,13.1631282644955));
#36375=CARTESIAN_POINT('Ctrl Pts',(0.316950491520289,2.16241599995751,13.1659079770247));
#36376=CARTESIAN_POINT('Ctrl Pts',(0.311904261492362,2.18407662552179,13.1671761672507));
#36377=CARTESIAN_POINT('Ctrl Pts',(0.304300538618862,2.20613045917093,13.168594768159));
#36378=CARTESIAN_POINT('Ctrl Pts',(0.303920754150156,2.20721318627414,13.1686647329452));
#36379=CARTESIAN_POINT('Ctrl Pts',(0.303358515084277,2.20878907765674,13.1687670394483));
#36380=CARTESIAN_POINT('Ctrl Pts',(0.303180619710128,2.20928386851932,13.1687992295271));
#36381=CARTESIAN_POINT('Ctrl Pts',(0.302866449162211,2.21015101823665,13.1688557653961));
#36382=CARTESIAN_POINT('Ctrl Pts',(0.30273069582072,2.21052356604963,13.168880093755));
#36383=CARTESIAN_POINT('Ctrl Pts',(0.302465885548909,2.21124613645369,13.1689273560864));
#36384=CARTESIAN_POINT('Ctrl Pts',(0.302336907644422,2.21159618752874,13.1689502873901));
#36385=CARTESIAN_POINT('Ctrl Pts',(0.302027710623407,2.21243088991442,13.1690050512688));
#36386=CARTESIAN_POINT('Ctrl Pts',(0.301846932761477,2.21291533185923,13.169036902488));
#36387=CARTESIAN_POINT('Ctrl Pts',(0.30119681906715,2.21464476477485,13.1691508526744));
#36388=CARTESIAN_POINT('Ctrl Pts',(0.300720945040233,2.21588726865104,13.1692331704195));
#36389=CARTESIAN_POINT('Ctrl Pts',(0.292334952281257,2.23738353731727,13.17066527293));
#36390=CARTESIAN_POINT('Ctrl Pts',(0.282404457371426,2.25678437813968,13.1720862914891));
#36391=CARTESIAN_POINT('Ctrl Pts',(0.262028823322614,2.28828456714812,13.174606664647));
#36392=CARTESIAN_POINT('Ctrl Pts',(0.252496981220199,2.3008866584972,13.1756825023987));
#36393=CARTESIAN_POINT('Ctrl Pts',(0.234455428947308,2.32141647237794,13.1775126468732));
#36394=CARTESIAN_POINT('Ctrl Pts',(0.226368457612949,2.32967800313671,13.1782741659965));
#36395=CARTESIAN_POINT('Ctrl Pts',(0.217088154515517,2.33819107873137,13.179070995298));
#36396=CARTESIAN_POINT('Ctrl Pts',(0.21631850115342,2.33889027386052,13.1791365336938));
#36397=CARTESIAN_POINT('Ctrl Pts',(0.214986406528519,2.34008870475396,13.1792490081594));
#36398=CARTESIAN_POINT('Ctrl Pts',(0.214425582467213,2.34058971456196,13.1792960715749));
#36399=CARTESIAN_POINT('Ctrl Pts',(0.21363175387852,2.3412938973872,13.1793622747434));
#36400=CARTESIAN_POINT('Ctrl Pts',(0.213400208352938,2.34149870032436,13.1793815356462));
#36401=CARTESIAN_POINT('Ctrl Pts',(0.213014552338626,2.34183882686326,13.179413533527));
#36402=CARTESIAN_POINT('Ctrl Pts',(0.212860607346183,2.34197433650576,13.1794262845246));
#36403=CARTESIAN_POINT('Ctrl Pts',(0.212539549983822,2.34225640285186,13.1794528315255));
#36404=CARTESIAN_POINT('Ctrl Pts',(0.212372415099037,2.34240293384303,13.1794666255679));
#36405=CARTESIAN_POINT('Ctrl Pts',(0.21196793764384,2.34275680908801,13.1794999463602));
#36406=CARTESIAN_POINT('Ctrl Pts',(0.211730441615963,2.34296397889956,13.1795194599925));
#36407=CARTESIAN_POINT('Ctrl Pts',(0.210927328858837,2.34366246916725,13.1795852756171));
#36408=CARTESIAN_POINT('Ctrl Pts',(0.210360297414463,2.34415217025104,13.179631457841));
#36409=CARTESIAN_POINT('Ctrl Pts',(0.201177618098627,2.35202679996756,13.1803748344916));
#36410=CARTESIAN_POINT('Ctrl Pts',(0.19217842681585,2.3589545488804,13.1810395216439));
#36411=CARTESIAN_POINT('Ctrl Pts',(0.178016111897704,2.36871105466462,13.1820242125751));
#36412=CARTESIAN_POINT('Ctrl Pts',(0.173111284483999,2.37189677126632,13.1823548795258));
#36413=CARTESIAN_POINT('Ctrl Pts',(0.154200742874493,2.38346002092454,13.1836011716372));
#36414=CARTESIAN_POINT('Ctrl Pts',(0.139652925356227,2.39090292206267,13.1845034252282));
#36415=CARTESIAN_POINT('Ctrl Pts',(0.109073237023004,2.40372323925584,13.1863858614907));
#36416=CARTESIAN_POINT('Ctrl Pts',(0.0930582244146317,2.40900618144362,
13.1873650263045));
#36417=CARTESIAN_POINT('Ctrl Pts',(0.0755658154721046,2.41329276963923,
13.1884600329017));
#36418=CARTESIAN_POINT('Ctrl Pts',(0.0744248458547879,2.41356577338527,
13.1885315600744));
#36419=CARTESIAN_POINT('Ctrl Pts',(0.072765774141958,2.41395317997857,13.1886357257984));
#36420=CARTESIAN_POINT('Ctrl Pts',(0.0722488309123698,2.41407254501407,
13.1886682046928));
#36421=CARTESIAN_POINT('Ctrl Pts',(0.071344352680709,2.41427904279586,13.1887250718279));
#36422=CARTESIAN_POINT('Ctrl Pts',(0.0709569459069465,2.41436673683038,
13.1887494419835));
#36423=CARTESIAN_POINT('Ctrl Pts',(0.0702067813063998,2.41453508799919,
13.1887966568519));
#36424=CARTESIAN_POINT('Ctrl Pts',(0.0698440439528597,2.41461583438628,
13.1888194986584));
#36425=CARTESIAN_POINT('Ctrl Pts',(0.0689814297210626,2.41480628947348,
13.1888738453948));
#36426=CARTESIAN_POINT('Ctrl Pts',(0.0684814307218341,2.41491543496611,
13.1889053683344));
#36427=CARTESIAN_POINT('Ctrl Pts',(0.0667112453192996,2.41529743608114,
13.1890170500196));
#36428=CARTESIAN_POINT('Ctrl Pts',(0.065439684174189,2.41556379879081,13.189097416381));
#36429=CARTESIAN_POINT('Ctrl Pts',(0.0438295462181028,2.41995439293981,
13.190465764114));
#36430=CARTESIAN_POINT('Ctrl Pts',(0.0231450745828925,2.4221115472394,13.1918183050712));
#36431=CARTESIAN_POINT('Ctrl Pts',(-0.00216728645454903,2.4223000820675,
13.1935154006768));
#36432=CARTESIAN_POINT('Ctrl Pts',(-0.00673504506051571,2.42223699013039,
13.1938230864147));
#36433=CARTESIAN_POINT('Ctrl Pts',(-0.0271023102383277,2.42152241881947,
13.195199387668));
#36434=CARTESIAN_POINT('Ctrl Pts',(-0.0428429370357241,2.41980574345981,
13.196275987723));
#36435=CARTESIAN_POINT('Ctrl Pts',(-0.0646624397054319,2.41578563541496,
13.1977443581534));
#36436=CARTESIAN_POINT('Ctrl Pts',(-0.0708953762043883,2.41444499626468,
13.1981608138686));
#36437=CARTESIAN_POINT('Ctrl Pts',(-0.0800195295578282,2.41219735016752,
13.1987621617263));
#36438=CARTESIAN_POINT('Ctrl Pts',(-0.0829440210275808,2.41143314139955,
13.1989536302863));
#36439=CARTESIAN_POINT('Ctrl Pts',(-0.0863457283848059,2.41049291044949,
13.1991745000902));
#36440=CARTESIAN_POINT('Ctrl Pts',(-0.0868336868203381,2.41035679965358,
13.1992061382819));
#36441=CARTESIAN_POINT('Ctrl Pts',(-0.0875775841786026,2.41014740567287,
13.1992543008954));
#36442=CARTESIAN_POINT('Ctrl Pts',(-0.0878337537599031,2.41007495577335,
13.199270873542));
#36443=CARTESIAN_POINT('Ctrl Pts',(-0.088279135392221,2.40994839668533,
13.1992996646235));
#36444=CARTESIAN_POINT('Ctrl Pts',(-0.088468387136638,2.40989443175303,
13.1993118914649));
#36445=CARTESIAN_POINT('Ctrl Pts',(-0.0888962129169217,2.40977201383681,
13.1993395156271));
#36446=CARTESIAN_POINT('Ctrl Pts',(-0.0891347568762895,2.40970345872316,
13.1993549068576));
#36447=CARTESIAN_POINT('Ctrl Pts',(-0.0897804840358736,2.40951707544482,
13.199396540317));
#36448=CARTESIAN_POINT('Ctrl Pts',(-0.0901875161493704,2.40939871887472,
13.1994227516542));
#36449=CARTESIAN_POINT('Ctrl Pts',(-0.0920105050184408,2.40886472810304,
13.1995400058776));
#36450=CARTESIAN_POINT('Ctrl Pts',(-0.0934238595329029,2.40844016594039,
13.1996305352916));
#36451=CARTESIAN_POINT('Ctrl Pts',(-0.125906286536871,2.39843890444091,
13.2017034876592));
#36452=CARTESIAN_POINT('Ctrl Pts',(-0.155357663903889,2.38422353518025,
13.2034360692372));
#36453=CARTESIAN_POINT('Ctrl Pts',(-0.194804724683445,2.35718923139032,
13.206150109739));
#36454=CARTESIAN_POINT('Ctrl Pts',(-0.206789772936656,2.3476551642339,13.2070370015348));
#36455=CARTESIAN_POINT('Ctrl Pts',(-0.219846175937913,2.33565817071051,
13.2081066420595));
#36456=CARTESIAN_POINT('Ctrl Pts',(-0.221621845306997,2.33398904178676,
13.2082544908054));
#36457=CARTESIAN_POINT('Ctrl Pts',(-0.223887445556888,2.33181045300906,
13.2084463055136));
#36458=CARTESIAN_POINT('Ctrl Pts',(-0.224394899915125,2.33131926699224,
13.2084894773868));
#36459=CARTESIAN_POINT('Ctrl Pts',(-0.225211372436159,2.33052375464129,
13.2085592791024));
#36460=CARTESIAN_POINT('Ctrl Pts',(-0.225521399900627,2.33022046371347,
13.2085858636074));
#36461=CARTESIAN_POINT('Ctrl Pts',(-0.226111638489387,2.32964071396988,
13.2086366287326));
#36462=CARTESIAN_POINT('Ctrl Pts',(-0.226391957385034,2.3293643655892,13.2086608044731));
#36463=CARTESIAN_POINT('Ctrl Pts',(-0.227031178984468,2.32873188460738,
13.2087160850871));
#36464=CARTESIAN_POINT('Ctrl Pts',(-0.227389750644248,2.32837542022823,
13.2087472045869));
#36465=CARTESIAN_POINT('Ctrl Pts',(-0.228485278063448,2.32728119309091,
13.208842620816));
#36466=CARTESIAN_POINT('Ctrl Pts',(-0.229219487703784,2.32654070150954,
13.208907038621));
#36467=CARTESIAN_POINT('Ctrl Pts',(-0.234652677725241,2.32100757066395,
13.209387276282));
#36468=CARTESIAN_POINT('Ctrl Pts',(-0.239204201552291,2.31607305361624,
13.2098094698477));
#36469=CARTESIAN_POINT('Ctrl Pts',(-0.244863527809933,2.30953940908034,
13.2103614634661));
#36470=CARTESIAN_POINT('Ctrl Pts',(-0.246115761277302,2.30806715985257,
13.2104854022711));
#36471=CARTESIAN_POINT('Ctrl Pts',(-0.263521375524284,2.28722641365731,
13.2122336704529));
#36472=CARTESIAN_POINT('Ctrl Pts',(-0.277357893443123,2.26604055207158,
13.2139468567067));
#36473=CARTESIAN_POINT('Ctrl Pts',(-0.292298157336018,2.23598773543766,
13.2162121926337));
#36474=CARTESIAN_POINT('Ctrl Pts',(-0.295722949980194,2.22836988379563,
13.216772671429));
#36475=CARTESIAN_POINT('Ctrl Pts',(-0.301737337741392,2.21346953571121,
13.2178332323034));
#36476=CARTESIAN_POINT('Ctrl Pts',(-0.304368693351965,2.20620959036298,
13.2183343352683));
#36477=CARTESIAN_POINT('Ctrl Pts',(-0.307119522869414,2.19767460973626,
13.2189000436941));
#36478=CARTESIAN_POINT('Ctrl Pts',(-0.307495179388808,2.19648546775468,
13.2189783409417));
#36479=CARTESIAN_POINT('Ctrl Pts',(-0.307976702761597,2.19492982478192,
13.2190800639565));
#36480=CARTESIAN_POINT('Ctrl Pts',(-0.308088828191964,2.19456529502895,
13.2191038499748));
#36481=CARTESIAN_POINT('Ctrl Pts',(-0.308270085292133,2.19397226786407,
13.2191424627275));
#36482=CARTESIAN_POINT('Ctrl Pts',(-0.308339610219882,2.19374389251507,
13.2191573125466));
#36483=CARTESIAN_POINT('Ctrl Pts',(-0.30847306478934,2.19330376653323,13.219185892396));
#36484=CARTESIAN_POINT('Ctrl Pts',(-0.308537030028967,2.19309202785927,
13.2191996244642));
#36485=CARTESIAN_POINT('Ctrl Pts',(-0.308684432511372,2.19260227321381,
13.2192313472234));
#36486=CARTESIAN_POINT('Ctrl Pts',(-0.308767712465595,2.19232420928218,
13.2192493286352));
#36487=CARTESIAN_POINT('Ctrl Pts',(-0.308990620692099,2.1915762645651,13.2192976170855));
#36488=CARTESIAN_POINT('Ctrl Pts',(-0.309129553480925,2.19110617476075,
13.2193278835812));
#36489=CARTESIAN_POINT('Ctrl Pts',(-0.310112108354956,2.18775350044511,
13.2195431631885));
#36490=CARTESIAN_POINT('Ctrl Pts',(-0.310916505185332,2.18485944231975,
13.2197259380808));
#36491=CARTESIAN_POINT('Ctrl Pts',(-0.320491591038072,2.14844449924624,
13.2219924530133));
#36492=CARTESIAN_POINT('Ctrl Pts',(-0.323842776910861,2.11372797121006,
13.2238224967533));
#36493=CARTESIAN_POINT('Ctrl Pts',(-0.320833182380519,2.06733103721908,
13.2264943429057));
#36494=CARTESIAN_POINT('Ctrl Pts',(-0.31941758761162,2.05557535261493,13.2271885200427));
#36495=CARTESIAN_POINT('Ctrl Pts',(-0.317003691010174,2.04191380023851,
13.2280271387493));
#36496=CARTESIAN_POINT('Ctrl Pts',(-0.316629228389137,2.03990608891751,
13.2281511864198));
#36497=CARTESIAN_POINT('Ctrl Pts',(-0.316103296798389,2.03722776368256,
13.2283177883289));
#36498=CARTESIAN_POINT('Ctrl Pts',(-0.315968722900876,2.03655384932107,
13.2283598033556));
#36499=CARTESIAN_POINT('Ctrl Pts',(-0.315755076555664,2.03550149832686,
13.2284255622288));
#36500=CARTESIAN_POINT('Ctrl Pts',(-0.3156774763623,2.03512276204876,13.2284492590064));
#36501=CARTESIAN_POINT('Ctrl Pts',(-0.315527743167163,2.03439860186007,
13.2284946269214));
#36502=CARTESIAN_POINT('Ctrl Pts',(-0.315455723909256,2.03405315475784,
13.2285162943932));
#36503=CARTESIAN_POINT('Ctrl Pts',(-0.315286018791363,2.03324578745157,
13.2285669949671));
#36504=CARTESIAN_POINT('Ctrl Pts',(-0.315187885113132,2.03278396313053,
13.2285960423648));
#36505=CARTESIAN_POINT('Ctrl Pts',(-0.314903928008363,2.03146193589925,
13.2286793267996));
#36506=CARTESIAN_POINT('Ctrl Pts',(-0.314715596556258,2.03060228126632,
13.2287336440924));
#36507=CARTESIAN_POINT('Ctrl Pts',(-0.313471512159119,2.025032780693,13.2290866116284));
#36508=CARTESIAN_POINT('Ctrl Pts',(-0.312313631880659,2.02034659973759,
13.2293885277008));
#36509=CARTESIAN_POINT('Ctrl Pts',(-0.308526419612287,2.00637443043774,
13.2303042101087));
#36510=CARTESIAN_POINT('Ctrl Pts',(-0.30558500700906,1.99717941853793,13.2309277713388));
#36511=CARTESIAN_POINT('Ctrl Pts',(-0.296506832716131,1.97265299170292,
13.2326475297276));
#36512=CARTESIAN_POINT('Ctrl Pts',(-0.28959778341036,1.95763918347249,13.2337634509625));
#36513=CARTESIAN_POINT('Ctrl Pts',(-0.273472215704942,1.92867801569639,
13.2360063135293));
#36514=CARTESIAN_POINT('Ctrl Pts',(-0.264258759393619,1.91478204835129,
13.2371296950493));
#36515=CARTESIAN_POINT('Ctrl Pts',(-0.251867972717343,1.89891336124446,
13.2384228471367));
#36516=CARTESIAN_POINT('Ctrl Pts',(-0.249679458469861,1.89620234930712,
13.2386441080038));
#36517=CARTESIAN_POINT('Ctrl Pts',(-0.247082166797389,1.89308962496345,
13.2388980274663));
#36518=CARTESIAN_POINT('Ctrl Pts',(-0.246715863689308,1.89265298877747,
13.2389336429125));
#36519=CARTESIAN_POINT('Ctrl Pts',(-0.246168322665017,1.89200382082237,
13.2389865866025));
#36520=CARTESIAN_POINT('Ctrl Pts',(-0.245987966144664,1.89179055220853,
13.2390039787743));
#36521=CARTESIAN_POINT('Ctrl Pts',(-0.245665770348604,1.8914105639849,13.2390349644316));
#36522=CARTESIAN_POINT('Ctrl Pts',(-0.245524038407464,1.89124375433705,
13.2390485658056));
#36523=CARTESIAN_POINT('Ctrl Pts',(-0.245222359741969,1.89088942960377,
13.2390774547672));
#36524=CARTESIAN_POINT('Ctrl Pts',(-0.245062368216546,1.89070195401311,
13.239092738922));
#36525=CARTESIAN_POINT('Ctrl Pts',(-0.244631233432553,1.89019792904867,
13.2391338274935));
#36526=CARTESIAN_POINT('Ctrl Pts',(-0.244359689722565,1.88988172047741,
13.2391596023144));
#36527=CARTESIAN_POINT('Ctrl Pts',(-0.243041871773518,1.88835315100923,
13.2392841907315));
#36528=CARTESIAN_POINT('Ctrl Pts',(-0.241987160764741,1.88714804582244,
13.2393823888207));
#36529=CARTESIAN_POINT('Ctrl Pts',(-0.233010240374893,1.87704405485538,
13.2402059929506));
#36530=CARTESIAN_POINT('Ctrl Pts',(-0.224608174224842,1.86858184652406,
13.2408977411943));
#36531=CARTESIAN_POINT('Ctrl Pts',(-0.192015589123711,1.83920781575204,
13.2433939586018));
#36532=CARTESIAN_POINT('Ctrl Pts',(-0.165226656512624,1.82146314127373,
13.2451183260423));
#36533=CARTESIAN_POINT('Ctrl Pts',(-0.131041458441012,1.80551311970321,
13.2473538942219));
#36534=CARTESIAN_POINT('Ctrl Pts',(-0.125754903120121,1.80321710890451,
13.2476997988164));
#36535=CARTESIAN_POINT('Ctrl Pts',(-0.11949788015101,1.80069681099245,13.2481104516411));
#36536=CARTESIAN_POINT('Ctrl Pts',(-0.118584213644656,1.80033364127531,
13.2481704461446));
#36537=CARTESIAN_POINT('Ctrl Pts',(-0.117203327516454,1.79979206247822,
13.2482611700817));
#36538=CARTESIAN_POINT('Ctrl Pts',(-0.116737325271348,1.79961054842747,
13.2482917949193));
#36539=CARTESIAN_POINT('Ctrl Pts',(-0.115904710359728,1.79928846396228,
13.2483465289436));
#36540=CARTESIAN_POINT('Ctrl Pts',(-0.11553825896239,1.79914747715282,13.2483706240814));
#36541=CARTESIAN_POINT('Ctrl Pts',(-0.114764357424741,1.79885135236284,
13.2484215222192));
#36542=CARTESIAN_POINT('Ctrl Pts',(-0.114356848583648,1.79869637093482,
13.2484483304136));
#36543=CARTESIAN_POINT('Ctrl Pts',(-0.113277746132655,1.79828847741656,
13.2485193390946));
#36544=CARTESIAN_POINT('Ctrl Pts',(-0.112605622895469,1.79803698188767,
13.2485635869149));
#36545=CARTESIAN_POINT('Ctrl Pts',(-0.109538973172311,1.79690116335904,
13.2487655682254));
#36546=CARTESIAN_POINT('Ctrl Pts',(-0.107134885553436,1.79604308346307,
13.2489241747789));
#36547=CARTESIAN_POINT('Ctrl Pts',(-0.0966104146836363,1.792427001985,13.2496198301654));
#36548=CARTESIAN_POINT('Ctrl Pts',(-0.0883926046461903,1.78996541088462,
13.2501665460423));
#36549=CARTESIAN_POINT('Ctrl Pts',(-0.0660917983424246,1.78424406978137,
13.251660491625));
#36550=CARTESIAN_POINT('Ctrl Pts',(-0.0518723850401837,1.78159913439141,
13.2526245763627));
#36551=CARTESIAN_POINT('Ctrl Pts',(-0.0129311996467933,1.77703386832622,
13.2552704081916));
#36552=CARTESIAN_POINT('Ctrl Pts',(0.0119147229375276,1.77699444672677,
13.2569688229929));
#36553=CARTESIAN_POINT('Ctrl Pts',(0.0378626493634233,1.77995403862979,
13.2586184066659));
#36554=CARTESIAN_POINT('Ctrl Pts',(0.0392028157741224,1.78011543176669,
13.258703232091));
#36555=CARTESIAN_POINT('Ctrl Pts',(0.0409479913379044,1.78033673162865,
13.2588131714256));
#36556=CARTESIAN_POINT('Ctrl Pts',(0.0413539306085327,1.78038899335582,
13.2588387072496));
#36557=CARTESIAN_POINT('Ctrl Pts',(0.0419782888144332,1.78047058436149,
13.2588779250693));
#36558=CARTESIAN_POINT('Ctrl Pts',(0.0421967771750812,1.78049936434053,
13.2588916380938));
#36559=CARTESIAN_POINT('Ctrl Pts',(0.0426313411542964,1.78055706002362,
13.2589188908167));
#36560=CARTESIAN_POINT('Ctrl Pts',(0.0428474154018679,1.78058597065381,
13.2589324306268));
#36561=CARTESIAN_POINT('Ctrl Pts',(0.0433301604808671,1.78065106037633,
13.258962656751));
#36562=CARTESIAN_POINT('Ctrl Pts',(0.0435968147746435,1.78068735416706,
13.2589793364339));
#36563=CARTESIAN_POINT('Ctrl Pts',(0.0443789317289334,1.78079480454234,
13.2590282120503));
#36564=CARTESIAN_POINT('Ctrl Pts',(0.0448942709807827,1.78086687600528,
13.2590603562572));
#36565=CARTESIAN_POINT('Ctrl Pts',(0.0487283439531174,1.78141255144116,
13.2592990737063));
#36566=CARTESIAN_POINT('Ctrl Pts',(0.0520398374056291,1.78193668655603,
13.2595028429308));
#36567=CARTESIAN_POINT('Ctrl Pts',(0.0631478979208892,1.78387298318018,
13.2601800572255));
#36568=CARTESIAN_POINT('Ctrl Pts',(0.0709009005361706,1.78552101824546,
13.2606422488961));
#36569=CARTESIAN_POINT('Ctrl Pts',(0.107840562099311,1.79480902034258,13.2628272620334));
#36570=CARTESIAN_POINT('Ctrl Pts',(0.135917534323478,1.80623526056136,13.2644508740788));
#36571=CARTESIAN_POINT('Ctrl Pts',(0.170125446169387,1.82612610334544,13.2667573100406));
#36572=CARTESIAN_POINT('Ctrl Pts',(0.178042120665504,1.83120536488094,13.2673158022855));
#36573=CARTESIAN_POINT('Ctrl Pts',(0.186660537323343,1.83728279454425,13.2679571344166));
#36574=CARTESIAN_POINT('Ctrl Pts',(0.187592601095877,1.83794752014631,13.2680269443166));
#36575=CARTESIAN_POINT('Ctrl Pts',(0.188942657742257,1.83892124201081,13.2681287274504));
#36576=CARTESIAN_POINT('Ctrl Pts',(0.189363483330773,1.83922631082924,13.2681605490507));
#36577=CARTESIAN_POINT('Ctrl Pts',(0.190104537932795,1.83976626275833,13.268216753822));
#36578=CARTESIAN_POINT('Ctrl Pts',(0.190425075033036,1.84000072281287,13.2682411205599));
#36579=CARTESIAN_POINT('Ctrl Pts',(0.191086565153946,1.84048645578685,13.2682915219504));
#36580=CARTESIAN_POINT('Ctrl Pts',(0.191427457688659,1.84073780944277,13.2683175597141));
#36581=CARTESIAN_POINT('Ctrl Pts',(0.192298300361876,1.84138257034721,13.2683842399728));
#36582=CARTESIAN_POINT('Ctrl Pts',(0.192827537364962,1.84177693351349,13.2684249197307));
#36583=CARTESIAN_POINT('Ctrl Pts',(0.194978415629963,1.84338996911338,13.2685908878316));
#36584=CARTESIAN_POINT('Ctrl Pts',(0.196589717470629,1.84462229307194,13.2687167109769));
#36585=CARTESIAN_POINT('Ctrl Pts',(0.207120971923618,1.85283533028714,13.2695490916004));
#36586=CARTESIAN_POINT('Ctrl Pts',(0.215678256035746,1.86026616855722,13.2702736652006));
#36587=CARTESIAN_POINT('Ctrl Pts',(0.246927706024237,1.89043167323565,13.2731144002436));
#36588=CARTESIAN_POINT('Ctrl Pts',(0.266563150661782,1.9160548621442,13.2753496251217));
#36589=CARTESIAN_POINT('Ctrl Pts',(0.28277181708008,1.94539314521262,13.2775349921177));
#36590=CARTESIAN_POINT('Ctrl Pts',(0.283448303490417,1.94663690318856,13.277626957818));
#36591=CARTESIAN_POINT('Ctrl Pts',(0.284291970606341,1.94821268449843,13.2777425819444));
#36592=CARTESIAN_POINT('Ctrl Pts',(0.284466792532364,1.94854057425565,13.2777665926034));
#36593=CARTESIAN_POINT('Ctrl Pts',(0.286623869228038,1.95260321940963,13.2780634849976));
#36594=CARTESIAN_POINT('Ctrl Pts',(0.288533126039736,1.95637655908958,13.278332902583));
#36595=CARTESIAN_POINT('Ctrl Pts',(0.290624353423767,1.96071966804988,13.2786349390143));
#36596=CARTESIAN_POINT('Ctrl Pts',(0.290879563145679,1.96125344894926,13.2786719229933));
#36597=CARTESIAN_POINT('Ctrl Pts',(0.291255517372583,1.96204536820673,13.2787265862069));
#36598=CARTESIAN_POINT('Ctrl Pts',(0.291377389951216,1.96230296495601,13.2787443348773));
#36599=CARTESIAN_POINT('Ctrl Pts',(0.291591273284423,1.96275659628188,13.2787755333272));
#36600=CARTESIAN_POINT('Ctrl Pts',(0.29168342801291,1.96295256170431,13.2787889920552));
#36601=CARTESIAN_POINT('Ctrl Pts',(0.29187480401475,1.96336058687352,13.2788169757109));
#36602=CARTESIAN_POINT('Ctrl Pts',(0.291973991410148,1.96357266117431,13.278831498507));
#36603=CARTESIAN_POINT('Ctrl Pts',(0.29223140406459,1.96412460616443,13.2788692390282));
#36604=CARTESIAN_POINT('Ctrl Pts',(0.292389268108418,1.96446464642047,13.2788924343716));
#36605=CARTESIAN_POINT('Ctrl Pts',(0.293042812909677,1.96587884234628,13.2789886735287));
#36606=CARTESIAN_POINT('Ctrl Pts',(0.293533178692765,1.96695546521373,13.2790613939057));
#36607=CARTESIAN_POINT('Ctrl Pts',(0.301129965871642,1.98388105587522,13.2801964606125));
#36608=CARTESIAN_POINT('Ctrl Pts',(0.306950749323379,2.00027895469877,13.2811848256562));
#36609=CARTESIAN_POINT('Ctrl Pts',(0.317610770460845,2.04030905876824,13.2835123068745));
#36610=CARTESIAN_POINT('Ctrl Pts',(0.321178432826951,2.06416768577558,13.2848377434887));
#36611=CARTESIAN_POINT('Ctrl Pts',(0.32215438466193,2.09080622367152,13.2863991425299));
#36612=CARTESIAN_POINT('Ctrl Pts',(0.322218217573961,2.09341267798522,13.2865526905281));
#36613=CARTESIAN_POINT('Ctrl Pts',(0.322322909530261,2.10188840214809,13.2870548552787));
#36614=CARTESIAN_POINT('Ctrl Pts',(0.322235059836258,2.10775780721272,13.2874070753915));
#36615=CARTESIAN_POINT('Ctrl Pts',(0.3219451268441,2.11461140096026,13.2878246840979));
#36616=CARTESIAN_POINT('Ctrl Pts',(0.321898674125451,2.1156013236187,13.2878851565429));
#36617=CARTESIAN_POINT('Ctrl Pts',(0.321821772788813,2.11709312661381,13.2879765248342));
#36618=CARTESIAN_POINT('Ctrl Pts',(0.321794714040184,2.11759518200107,13.2880073146335));
#36619=CARTESIAN_POINT('Ctrl Pts',(0.321744349462104,2.11849066086518,13.2880623050691));
#36620=CARTESIAN_POINT('Ctrl Pts',(0.321721496563834,2.1188841096313,13.2880864914868));
#36621=CARTESIAN_POINT('Ctrl Pts',(0.321671783293538,2.11971371119004,13.2881375428814));
#36622=CARTESIAN_POINT('Ctrl Pts',(0.321644757457155,2.12014985293917,13.2881644129906));
#36623=CARTESIAN_POINT('Ctrl Pts',(0.321570993652707,2.12130227473176,13.2882354951546));
#36624=CARTESIAN_POINT('Ctrl Pts',(0.321522749715472,2.12201845293495,13.2882797542807));
#36625=CARTESIAN_POINT('Ctrl Pts',(0.321293041500956,2.12526659638077,13.2884808759018));
#36626=CARTESIAN_POINT('Ctrl Pts',(0.32108406240864,2.1277964689326,13.2886385979543));
#36627=CARTESIAN_POINT('Ctrl Pts',(0.320041679956877,2.13882563301227,13.2893310641673));
#36628=CARTESIAN_POINT('Ctrl Pts',(0.318900579807654,2.14729169995432,13.2898753681984));
#36629=CARTESIAN_POINT('Ctrl Pts',(0.314941127734568,2.16985518027476,13.2913614172381));
#36630=CARTESIAN_POINT('Ctrl Pts',(0.311513939663806,2.1838251083527,13.2923198015192));
#36631=CARTESIAN_POINT('Ctrl Pts',(0.300361758639017,2.2189525790881,13.2948062389792));
#36632=CARTESIAN_POINT('Ctrl Pts',(0.291331775562052,2.23961671405938,13.2963461465302));
#36633=CARTESIAN_POINT('Ctrl Pts',(0.278482219273848,2.2622382665128,13.2980176282241));
#36634=CARTESIAN_POINT('Ctrl Pts',(0.276690920222358,2.26527473723107,13.2982415535531));
#36635=CARTESIAN_POINT('Ctrl Pts',(0.274557315584081,2.26875950467236,13.2984974856627));
#36636=CARTESIAN_POINT('Ctrl Pts',(0.274263310686198,2.26923689426567,13.2985325233897));
#36637=CARTESIAN_POINT('Ctrl Pts',(0.273821605988517,2.2699499369256,13.2985848190297));
#36638=CARTESIAN_POINT('Ctrl Pts',(0.273674846480638,2.27018616680665,13.2986021382795));
#36639=CARTESIAN_POINT('Ctrl Pts',(0.273413885318743,2.27060500968234,13.2986328343962));
#36640=CARTESIAN_POINT('Ctrl Pts',(0.273299806298809,2.27078769830258,13.2986462193896));
#36641=CARTESIAN_POINT('Ctrl Pts',(0.273061216871858,2.27116892938551,13.2986741426149));
#36642=CARTESIAN_POINT('Ctrl Pts',(0.272936673235062,2.27136745008958,13.2986886784835));
#36643=CARTESIAN_POINT('Ctrl Pts',(0.272607423120428,2.2718910004424,13.2987270011957));
#36644=CARTESIAN_POINT('Ctrl Pts',(0.272402350927641,2.27221580179012,13.298750763591));
#36645=CARTESIAN_POINT('Ctrl Pts',(0.271506096007834,2.2736297191016,13.2988541552198));
#36646=CARTESIAN_POINT('Ctrl Pts',(0.270808946155987,2.274715066149,13.2989333902238));
#36647=CARTESIAN_POINT('Ctrl Pts',(0.265630958450031,2.28267087910922,13.2995134654401));
#36648=CARTESIAN_POINT('Ctrl Pts',(0.260895364419495,2.2893728882114,13.2999980971152));
#36649=CARTESIAN_POINT('Ctrl Pts',(0.246455521633568,2.30823719723952,13.3013730589431));
#36650=CARTESIAN_POINT('Ctrl Pts',(0.236120113209579,2.31988726984462,13.3022367865324));
#36651=CARTESIAN_POINT('Ctrl Pts',(0.213426316652339,2.34201429321112,13.3040064251962));
#36652=CARTESIAN_POINT('Ctrl Pts',(0.201039831968825,2.35239778410238,13.3049106062132));
#36653=CARTESIAN_POINT('Ctrl Pts',(0.185592405341932,2.36348606082858,13.3060154871071));
#36654=CARTESIAN_POINT('Ctrl Pts',(0.183233974858488,2.36513158043407,13.3061835478911));
#36655=CARTESIAN_POINT('Ctrl Pts',(0.180368195179146,2.36707458532761,13.3063871989529));
#36656=CARTESIAN_POINT('Ctrl Pts',(0.179881607027661,2.36740255684497,13.3064217580238));
#36657=CARTESIAN_POINT('Ctrl Pts',(0.177786687557818,2.36880627469434,13.3065704680477));
#36658=CARTESIAN_POINT('Ctrl Pts',(0.1761696049791,2.3698688378451,13.3066850617583));
#36659=CARTESIAN_POINT('Ctrl Pts',(0.170403142930759,2.37358398647841,13.307093148083));
#36660=CARTESIAN_POINT('Ctrl Pts',(0.166202802667764,2.37615584929755,13.3073894136506));
#36661=CARTESIAN_POINT('Ctrl Pts',(0.161211239626043,2.37905704223633,13.3077409690505));
#36662=CARTESIAN_POINT('Ctrl Pts',(0.160475448754023,2.3794808167457,13.3077927773409));
#36663=CARTESIAN_POINT('Ctrl Pts',(0.159294650871496,2.38015469012894,13.3078759013984));
#36664=CARTESIAN_POINT('Ctrl Pts',(0.158850706008351,2.38040665005201,13.3079071495277));
#36665=CARTESIAN_POINT('Ctrl Pts',(0.158063695002334,2.38085084759829,13.307962538832));
#36666=CARTESIAN_POINT('Ctrl Pts',(0.157720871288638,2.38104351448171,13.3079866644034));
#36667=CARTESIAN_POINT('Ctrl Pts',(0.157008938695551,2.38144190761101,13.308036761302));
#36668=CARTESIAN_POINT('Ctrl Pts',(0.156639776306437,2.38164753623273,13.3080627360959));
#36669=CARTESIAN_POINT('Ctrl Pts',(0.155688534258917,2.38217494269321,13.3081296617048));
#36670=CARTESIAN_POINT('Ctrl Pts',(0.155105863127844,2.38249564456165,13.3081706511882));
#36671=CARTESIAN_POINT('Ctrl Pts',(0.152682693196762,2.38381959900697,13.3083410982904));
#36672=CARTESIAN_POINT('Ctrl Pts',(0.150833453699553,2.38480666862155,13.308471134781));
#36673=CARTESIAN_POINT('Ctrl Pts',(0.138336650841771,2.39132124871586,13.3093497799342));
#36674=CARTESIAN_POINT('Ctrl Pts',(0.127398486029302,2.39626789231732,13.3101188123888));
#36675=CARTESIAN_POINT('Ctrl Pts',(0.0997208249173376,2.40696825237916,
13.3120654669599));
#36676=CARTESIAN_POINT('Ctrl Pts',(0.0827351846189903,2.4119752107131,13.3132620137301));
#36677=CARTESIAN_POINT('Ctrl Pts',(0.0594515538423541,2.41680265712882,
13.3148714962036));
#36678=CARTESIAN_POINT('Ctrl Pts',(0.0534424711182091,2.41787153975798,
13.3152839441848));
#36679=CARTESIAN_POINT('Ctrl Pts',(0.0343476700455006,2.42071127159424,
13.3165796962642));
#36680=CARTESIAN_POINT('Ctrl Pts',(0.0211799489830165,2.421849317678,13.3174516881898));
#36681=CARTESIAN_POINT('Ctrl Pts',(0.00714357649414458,2.42219689889339,
13.3183341627897));
#36682=CARTESIAN_POINT('Ctrl Pts',(0.00630904854883794,2.42221432042184,
13.3183864520476));
#36683=CARTESIAN_POINT('Ctrl Pts',(0.005145336440725,2.42223409112913,13.3184591100335));
#36684=CARTESIAN_POINT('Ctrl Pts',(0.00481621137220232,2.42223917838035,
13.3184796307488));
#36685=CARTESIAN_POINT('Ctrl Pts',(0.00426235170572277,2.42224689058909,
13.3185141146055));
#36686=CARTESIAN_POINT('Ctrl Pts',(0.00403762212661081,2.42224978470929,
13.3185280929315));
#36687=CARTESIAN_POINT('Ctrl Pts',(0.00359227569525369,2.42225505404386,
13.3185557667465));
#36688=CARTESIAN_POINT('Ctrl Pts',(0.00337166025017408,2.42225743778746,
13.3185694626837));
#36689=CARTESIAN_POINT('Ctrl Pts',(0.00292761510799275,2.42226177964352,
13.3185970032096));
#36690=CARTESIAN_POINT('Ctrl Pts',(0.00270418546231148,2.42226373195093,
13.3186108474634));
#36691=CARTESIAN_POINT('Ctrl Pts',(0.00190994003425121,2.42226984593815,
13.3186600142412));
#36692=CARTESIAN_POINT('Ctrl Pts',(0.00133911108802614,2.42227272342722,
13.3186952650754));
#36693=CARTESIAN_POINT('Ctrl Pts',(-0.00425503190026124,2.42228605935975,
13.3190399114128));
#36694=CARTESIAN_POINT('Ctrl Pts',(-0.0092782734663582,2.42218058577684,
13.3193429620839));
#36695=CARTESIAN_POINT('Ctrl Pts',(-0.0236659034809866,2.42154166748611,
13.3201977314319));
#36696=CARTESIAN_POINT('Ctrl Pts',(-0.0330126164451058,2.42071687438639,
13.3207369834546));
#36697=CARTESIAN_POINT('Ctrl Pts',(-0.0485215048691819,2.41866297208185,
13.3216238336867));
#36698=CARTESIAN_POINT('Ctrl Pts',(-0.0547071341289445,2.4176595016193,
13.3219754068292));
#36699=CARTESIAN_POINT('Ctrl Pts',(-0.0836978928970217,2.41208446015627,
13.323627611145));
#36700=CARTESIAN_POINT('Ctrl Pts',(-0.105991362608536,2.40523395823029,
13.324917175608));
#36701=CARTESIAN_POINT('Ctrl Pts',(-0.133922292476707,2.39321858326136,
13.3267079426474));
#36702=CARTESIAN_POINT('Ctrl Pts',(-0.14039530966298,2.3901748836482,13.3271356157394));
#36703=CARTESIAN_POINT('Ctrl Pts',(-0.147710583639609,2.3864330564264,13.3276357136852));
#36704=CARTESIAN_POINT('Ctrl Pts',(-0.148657356723442,2.38594283096855,
13.3277007670064));
#36705=CARTESIAN_POINT('Ctrl Pts',(-0.15005016218335,2.38521286935792,13.3277969596101));
#36706=CARTESIAN_POINT('Ctrl Pts',(-0.150498096721495,2.38497676203023,
13.3278279711796));
#36707=CARTESIAN_POINT('Ctrl Pts',(-0.151295902465212,2.38455383117248,
13.3278833406439));
#36708=CARTESIAN_POINT('Ctrl Pts',(-0.15164598948692,2.38436741516568,13.3279076841217));
#36709=CARTESIAN_POINT('Ctrl Pts',(-0.152377363899488,2.38397623475382,
13.327958638715));
#36710=CARTESIAN_POINT('Ctrl Pts',(-0.152758584496747,2.38377134773188,
13.3279852541323));
#36711=CARTESIAN_POINT('Ctrl Pts',(-0.153751313946428,2.38323522511471,
13.3280547093998));
#36712=CARTESIAN_POINT('Ctrl Pts',(-0.154362162974006,2.38290277820476,
13.3280975921348));
#36713=CARTESIAN_POINT('Ctrl Pts',(-0.157001188711173,2.38145542965283,
13.3282834908116));
#36714=CARTESIAN_POINT('Ctrl Pts',(-0.159018358734871,2.38032069719605,
13.328427211055));
#36715=CARTESIAN_POINT('Ctrl Pts',(-0.173161401824821,2.37216293482577,
13.3294466283498));
#36716=CARTESIAN_POINT('Ctrl Pts',(-0.184828488828499,2.36437827139864,
13.330349998307));
#36717=CARTESIAN_POINT('Ctrl Pts',(-0.208509633131971,2.34624203535987,
13.3323203537741));
#36718=CARTESIAN_POINT('Ctrl Pts',(-0.220342473068241,2.33571283128132,
13.3333910432132));
#36719=CARTESIAN_POINT('Ctrl Pts',(-0.237272731053398,2.31825470799072,
13.3350340857633));
#36720=CARTESIAN_POINT('Ctrl Pts',(-0.242948202527085,2.3119189642645,13.3356069872501));
#36721=CARTESIAN_POINT('Ctrl Pts',(-0.254953255373636,2.29740022822919,
13.336858826803));
#36722=CARTESIAN_POINT('Ctrl Pts',(-0.261153638419859,2.28912122889594,
13.3375333369435));
#36723=CARTESIAN_POINT('Ctrl Pts',(-0.267361038546912,2.27994387918258,
13.3382285982005));
#36724=CARTESIAN_POINT('Ctrl Pts',(-0.267774033371893,2.27932872515409,
13.338274957594));
#36725=CARTESIAN_POINT('Ctrl Pts',(-0.268360279763345,2.27844897277762,
13.3383409045595));
#36726=CARTESIAN_POINT('Ctrl Pts',(-0.268535265125195,2.27818554101334,
13.3383606066346));
#36727=CARTESIAN_POINT('Ctrl Pts',(-0.268834518137468,2.27773358845282,
13.3383943305701));
#36728=CARTESIAN_POINT('Ctrl Pts',(-0.268958975100083,2.27754519514732,
13.3384083650659));
#36729=CARTESIAN_POINT('Ctrl Pts',(-0.269210146181475,2.27716412164922,
13.338436707058));
#36730=CARTESIAN_POINT('Ctrl Pts',(-0.269336851848363,2.2769714356725,13.3384510140019));
#36731=CARTESIAN_POINT('Ctrl Pts',(-0.269650757755236,2.27649294941179,
13.3384864828059));
#36732=CARTESIAN_POINT('Ctrl Pts',(-0.269837711091967,2.27620698631211,
13.3385076284309));
#36733=CARTESIAN_POINT('Ctrl Pts',(-0.270513702732569,2.27516939333368,
13.3385841673609));
#36734=CARTESIAN_POINT('Ctrl Pts',(-0.271000063826336,2.27441601181311,
13.3386393877078));
#36735=CARTESIAN_POINT('Ctrl Pts',(-0.281811921276165,2.25751385592853,
13.3398706030303));
#36736=CARTESIAN_POINT('Ctrl Pts',(-0.290681186503799,2.24047510466773,
13.3409570247485));
#36737=CARTESIAN_POINT('Ctrl Pts',(-0.306018856020226,2.20324082872203,
13.3432232905128));
#36738=CARTESIAN_POINT('Ctrl Pts',(-0.312118573380971,2.18299479425078,
13.3443981638694));
#36739=CARTESIAN_POINT('Ctrl Pts',(-0.317875867065161,2.15377362982812,
13.3461416142945));
#36740=CARTESIAN_POINT('Ctrl Pts',(-0.319209911596244,2.14518497722302,
13.3466590579368));
#36741=CARTESIAN_POINT('Ctrl Pts',(-0.32032380239195,2.13542768839048,13.3472564584957));
#36742=CARTESIAN_POINT('Ctrl Pts',(-0.320446380109866,2.1343012668521,13.3473255654185));
#36743=CARTESIAN_POINT('Ctrl Pts',(-0.320616793409913,2.13265456108935,
13.3474268054853));
#36744=CARTESIAN_POINT('Ctrl Pts',(-0.320669308925578,2.13213476131231,
13.3474587939726));
#36745=CARTESIAN_POINT('Ctrl Pts',(-0.320760051283632,2.13121421446549,
13.3475155002185));
#36746=CARTESIAN_POINT('Ctrl Pts',(-0.320798791732582,2.13081351821522,
13.3475402020509));
#36747=CARTESIAN_POINT('Ctrl Pts',(-0.320877611296746,2.12998201781723,
13.3475915010323));
#36748=CARTESIAN_POINT('Ctrl Pts',(-0.320917573814974,2.12955120365997,
13.3476181017331));
#36749=CARTESIAN_POINT('Ctrl Pts',(-0.321018221485092,2.12844189065102,
13.3476866533823));
#36750=CARTESIAN_POINT('Ctrl Pts',(-0.321077622921942,2.12776328000895,
13.3477286439287));
#36751=CARTESIAN_POINT('Ctrl Pts',(-0.321315490036934,2.12494294169138,
13.3479033902646));
#36752=CARTESIAN_POINT('Ctrl Pts',(-0.321474678016385,2.12279968240715,
13.3480367404471));
#36753=CARTESIAN_POINT('Ctrl Pts',(-0.322400548880522,2.10838326463028,
13.3489376106644));
#36754=CARTESIAN_POINT('Ctrl Pts',(-0.322485575474556,2.09607794736713,
13.349726153015));
#36755=CARTESIAN_POINT('Ctrl Pts',(-0.320321010611323,2.05307409786068,
13.3525523025489));
#36756=CARTESIAN_POINT('Ctrl Pts',(-0.314384246460146,2.02274357795218,
13.3546890337174));
#36757=CARTESIAN_POINT('Ctrl Pts',(-0.304247867982273,1.99372483614108,
13.3567));
#36758=CARTESIAN_POINT('',(-0.203204102907281,2.3501384980099,13.3567));
#36759=CARTESIAN_POINT('Origin',(0.,2.1,13.3567));
#36760=CARTESIAN_POINT('',(-0.322274957492435,2.09983447583549,13.2493773449307));
#36761=CARTESIAN_POINT('Ctrl Pts',(-0.322274957492435,2.09983447583549,
13.2493773449307));
#36762=CARTESIAN_POINT('Ctrl Pts',(-0.32226483878068,2.08013338016583,13.2505879758328));
#36763=CARTESIAN_POINT('Ctrl Pts',(-0.320444039314449,2.06049592730386,
13.2517986067348));
#36764=CARTESIAN_POINT('Ctrl Pts',(-0.316871812603967,2.04123410851458,
13.2530092376369));
#36765=CARTESIAN_POINT('Ctrl Pts',(-0.313271733721456,2.02182210791043,
13.2542293076656));
#36766=CARTESIAN_POINT('Ctrl Pts',(-0.307893024034668,2.00279206168637,
13.2554493776942));
#36767=CARTESIAN_POINT('Ctrl Pts',(-0.300845432144591,1.98444394614416,
13.2566694477229));
#36768=CARTESIAN_POINT('Ctrl Pts',(-0.299538362453334,1.98104104397687,
13.2568957259439));
#36769=CARTESIAN_POINT('Ctrl Pts',(-0.29817401836561,1.97766153425079,13.257122004165));
#36770=CARTESIAN_POINT('Ctrl Pts',(-0.296753274075577,1.97430723986472,
13.2573482823861));
#36771=CARTESIAN_POINT('Ctrl Pts',(-0.289873171352211,1.95806371870298,
13.2584440583226));
#36772=CARTESIAN_POINT('Ctrl Pts',(-0.281633490705982,1.94233506417864,
13.2595398342591));
#36773=CARTESIAN_POINT('Ctrl Pts',(-0.272133799288446,1.92736057544745,
13.2606356101957));
#36774=CARTESIAN_POINT('Ctrl Pts',(-0.262652330660647,1.91241481153979,
13.2617292841592));
#36775=CARTESIAN_POINT('Ctrl Pts',(-0.251916004330233,1.89822102456005,
13.2628229581228));
#36776=CARTESIAN_POINT('Ctrl Pts',(-0.24007054260555,1.88499462751346,13.2639166320864));
#36777=CARTESIAN_POINT('Ctrl Pts',(-0.228064507295878,1.87158893733,13.2650251315716));
#36778=CARTESIAN_POINT('Ctrl Pts',(-0.21491946217764,1.85917776405065,13.2661336310568));
#36779=CARTESIAN_POINT('Ctrl Pts',(-0.200829887600173,1.84795133035165,
13.267242130542));
#36780=CARTESIAN_POINT('Ctrl Pts',(-0.1869352002943,1.83688018090353,13.2683352972406));
#36781=CARTESIAN_POINT('Ctrl Pts',(-0.172122628296553,1.8269616217329,13.2694284639392));
#36782=CARTESIAN_POINT('Ctrl Pts',(-0.156611467290689,1.81833703839863,
13.2705216306378));
#36783=CARTESIAN_POINT('Ctrl Pts',(-0.14077396631965,1.80953100209484,13.2716377965163));
#36784=CARTESIAN_POINT('Ctrl Pts',(-0.124208846012644,1.80207448238125,
13.2727539623948));
#36785=CARTESIAN_POINT('Ctrl Pts',(-0.107173813964848,1.7960675252211,13.2738701282733));
#36786=CARTESIAN_POINT('Ctrl Pts',(-0.0901387819170519,1.79006056806095,
13.2749862941518));
#36787=CARTESIAN_POINT('Ctrl Pts',(-0.0726346771758236,1.78550332968368,
13.2761024600303));
#36788=CARTESIAN_POINT('Ctrl Pts',(-0.0549316064210603,1.78244103816614,
13.2772186259088));
#36789=CARTESIAN_POINT('Ctrl Pts',(-0.0374952283451083,1.77942487936417,
13.2783179770057));
#36790=CARTESIAN_POINT('Ctrl Pts',(-0.0197559757355919,1.77783976901579,
13.2794173281027));
#36791=CARTESIAN_POINT('Ctrl Pts',(-0.00197043232130345,1.77773102379927,
13.2805166791996));
#36792=CARTESIAN_POINT('Ctrl Pts',(0.0157809453715159,1.77762248748043,
13.281613918462));
#36793=CARTESIAN_POINT('Ctrl Pts',(0.0335776760126947,1.77898475464975,
13.2827111577245));
#36794=CARTESIAN_POINT('Ctrl Pts',(0.0511584206520158,1.78181138986225,
13.283808396987));
#36795=CARTESIAN_POINT('Ctrl Pts',(0.0688909821816445,1.78466243422106,
13.2849151113574));
#36796=CARTESIAN_POINT('Ctrl Pts',(0.0864030118068149,1.78900325792153,
13.2860218257277));
#36797=CARTESIAN_POINT('Ctrl Pts',(0.10343179270322,1.79477378899708,13.2871285400981));
#36798=CARTESIAN_POINT('Ctrl Pts',(0.120305488659644,1.80049176654746,13.2882251753717));
#36799=CARTESIAN_POINT('Ctrl Pts',(0.136703982565598,1.80761320475385,13.2893218106452));
#36800=CARTESIAN_POINT('Ctrl Pts',(0.152388340046847,1.81602998495833,13.2904184459188));
#36801=CARTESIAN_POINT('Ctrl Pts',(0.168288928250003,1.82456280220557,13.2915301998376));
#36802=CARTESIAN_POINT('Ctrl Pts',(0.183454807723234,1.83442659769339,13.2926419537564));
#36803=CARTESIAN_POINT('Ctrl Pts',(0.197665413300553,1.84546206567641,13.2937537076752));
#36804=CARTESIAN_POINT('Ctrl Pts',(0.211876018877872,1.85649753365943,13.294865461594));
#36805=CARTESIAN_POINT('Ctrl Pts',(0.225130784671371,1.86870408322537,13.2959772155128));
#36806=CARTESIAN_POINT('Ctrl Pts',(0.237247185952831,1.88188317721353,13.2970889694316));
#36807=CARTESIAN_POINT('Ctrl Pts',(0.249220469872859,1.89490660145175,13.2981875914572));
#36808=CARTESIAN_POINT('Ctrl Pts',(0.26015467709715,1.9089585061543,13.2992862134828));
#36809=CARTESIAN_POINT('Ctrl Pts',(0.269873121224844,1.92384758285689,13.3003848355085));
#36810=CARTESIAN_POINT('Ctrl Pts',(0.279573317837768,1.93870870357769,13.3014813947428));
#36811=CARTESIAN_POINT('Ctrl Pts',(0.288061813739083,1.95440327127342,13.3025779539772));
#36812=CARTESIAN_POINT('Ctrl Pts',(0.295202914764986,1.97070802523259,13.3036745132115));
#36813=CARTESIAN_POINT('Ctrl Pts',(0.302412442995074,1.98716901402506,13.3047815798568));
#36814=CARTESIAN_POINT('Ctrl Pts',(0.308248181548252,2.00425127227537,13.305888646502));
#36815=CARTESIAN_POINT('Ctrl Pts',(0.312618619957343,2.02170074022721,13.3069957131473));
#36816=CARTESIAN_POINT('Ctrl Pts',(0.316945703283351,2.03897710812319,13.3080917976067));
#36817=CARTESIAN_POINT('Ctrl Pts',(0.3198363087186,2.0566126553897,13.3091878820662));
#36818=CARTESIAN_POINT('Ctrl Pts',(0.321252477112893,2.07434806880895,13.3102839665257));
#36819=CARTESIAN_POINT('Ctrl Pts',(0.322689929393039,2.09235003140153,13.3113965242639));
#36820=CARTESIAN_POINT('Ctrl Pts',(0.322608154631673,2.11045407645896,13.312509082002));
#36821=CARTESIAN_POINT('Ctrl Pts',(0.321022286249014,2.12838780295226,13.3136216397401));
#36822=CARTESIAN_POINT('Ctrl Pts',(0.319436417866355,2.14632152944555,13.3147341974782));
#36823=CARTESIAN_POINT('Ctrl Pts',(0.316346651383024,2.16408413715393,13.3158467552163));
#36824=CARTESIAN_POINT('Ctrl Pts',(0.311821906718333,2.18141421322806,13.3169593129544));
#36825=CARTESIAN_POINT('Ctrl Pts',(0.307406464415695,2.19832565391172,13.3180449951011));
#36826=CARTESIAN_POINT('Ctrl Pts',(0.301595565345558,2.21493620643441,13.3191306772479));
#36827=CARTESIAN_POINT('Ctrl Pts',(0.294449846721818,2.23099795185612,13.3202163593946));
#36828=CARTESIAN_POINT('Ctrl Pts',(0.287317896864584,2.24702874861695,13.3212999495888));
#36829=CARTESIAN_POINT('Ctrl Pts',(0.278856483092462,2.2625120937275,13.3223835397831));
#36830=CARTESIAN_POINT('Ctrl Pts',(0.269175515635444,2.27721658333066,13.3234671299773));
#36831=CARTESIAN_POINT('Ctrl Pts',(0.259226937221565,2.29232754909959,13.3245806738523));
#36832=CARTESIAN_POINT('Ctrl Pts',(0.247990648795134,2.3066151140032,13.3256942177273));
#36833=CARTESIAN_POINT('Ctrl Pts',(0.235635590836591,2.31985687152348,13.3268077616023));
#36834=CARTESIAN_POINT('Ctrl Pts',(0.223616150494876,2.33273892477394,13.3278910567368));
#36835=CARTESIAN_POINT('Ctrl Pts',(0.210538642062222,2.34463078399106,13.3289743518713));
#36836=CARTESIAN_POINT('Ctrl Pts',(0.196597171399358,2.35536391253028,13.3300576470059));
#36837=CARTESIAN_POINT('Ctrl Pts',(0.182071771323903,2.36654659116323,13.3311863152511));
#36838=CARTESIAN_POINT('Ctrl Pts',(0.166609069782128,2.37647061849798,13.3323149834963));
#36839=CARTESIAN_POINT('Ctrl Pts',(0.150461755109173,2.38499550149865,13.3334436517415));
#36840=CARTESIAN_POINT('Ctrl Pts',(0.134314440436219,2.39352038449932,13.3345723199868));
#36841=CARTESIAN_POINT('Ctrl Pts',(0.117483428649364,2.40064583038671,13.335700988232));
#36842=CARTESIAN_POINT('Ctrl Pts',(0.100242319425589,2.40628851271502,13.3368296564772));
#36843=CARTESIAN_POINT('Ctrl Pts',(0.0830172659067363,2.41192594032095,
13.3379572736552));
#36844=CARTESIAN_POINT('Ctrl Pts',(0.0652712419742939,2.41612062749411,
13.3390848908333));
#36845=CARTESIAN_POINT('Ctrl Pts',(0.0472633934003619,2.41879044413107,
13.3402125080113));
#36846=CARTESIAN_POINT('Ctrl Pts',(0.0292958691642339,2.42145428234214,
13.3413376001561));
#36847=CARTESIAN_POINT('Ctrl Pts',(0.0110683824425036,2.42259987165385,
13.3424626923009));
#36848=CARTESIAN_POINT('Ctrl Pts',(-0.0071482943072423,2.42219571305884,
13.3435877844457));
#36849=CARTESIAN_POINT('Ctrl Pts',(-0.0253420927399112,2.42179206204646,
13.3447114635877));
#36850=CARTESIAN_POINT('Ctrl Pts',(-0.0435243899744615,2.4198425030032,
13.3458351427298));
#36851=CARTESIAN_POINT('Ctrl Pts',(-0.0614226686174823,2.41636755744688,
13.3469588218718));
#36852=CARTESIAN_POINT('Ctrl Pts',(-0.0793049610672264,2.41289571560531,
13.3480814973781));
#36853=CARTESIAN_POINT('Ctrl Pts',(-0.0969030296939914,2.40790131785739,
13.3492041728844));
#36854=CARTESIAN_POINT('Ctrl Pts',(-0.113953079311686,2.40145625112176,
13.3503268483907));
#36855=CARTESIAN_POINT('Ctrl Pts',(-0.131016296558478,2.39500620690804,
13.3514503909311));
#36856=CARTESIAN_POINT('Ctrl Pts',(-0.147529969748812,2.38710350153777,
13.3525739334715));
#36857=CARTESIAN_POINT('Ctrl Pts',(-0.163248172020791,2.37786905181555,
13.3536974760119));
#36858=CARTESIAN_POINT('Ctrl Pts',(-0.177249801591024,2.36964308919856,
13.3546983173413));
#36859=CARTESIAN_POINT('Ctrl Pts',(-0.1906201923099,2.36036124374616,13.3556991586706));
#36860=CARTESIAN_POINT('Ctrl Pts',(-0.203204102907283,2.35013849800989,
13.3567));
#36861=CARTESIAN_POINT('',(-0.32227499814981,2.10003453317044,12.9993773449273));
#36862=CARTESIAN_POINT('Ctrl Pts',(-0.322274964711977,2.0998491858969,13.2496290980342));
#36863=CARTESIAN_POINT('Ctrl Pts',(-0.322279096760105,2.10867896797313,
13.2491131692747));
#36864=CARTESIAN_POINT('Ctrl Pts',(-0.321920350415243,2.11750462929075,
13.2485878344569));
#36865=CARTESIAN_POINT('Ctrl Pts',(-0.321135494975524,2.12708854194888,
13.2480030121234));
#36866=CARTESIAN_POINT('Ctrl Pts',(-0.321068373910397,2.12787282718828,
13.2479550502186));
#36867=CARTESIAN_POINT('Ctrl Pts',(-0.320953752144539,2.12915675745422,
13.2478763601958));
#36868=CARTESIAN_POINT('Ctrl Pts',(-0.320907956107554,2.12965655447462,
13.247845685479));
#36869=CARTESIAN_POINT('Ctrl Pts',(-0.320824851200874,2.1305407868138,13.2477913394896));
#36870=CARTESIAN_POINT('Ctrl Pts',(-0.320788018295633,2.13092526674389,
13.2477676831771));
#36871=CARTESIAN_POINT('Ctrl Pts',(-0.320713928190224,2.13168427926963,
13.2477209314442));
#36872=CARTESIAN_POINT('Ctrl Pts',(-0.320676705866237,2.13205881471408,
13.2476978371539));
#36873=CARTESIAN_POINT('Ctrl Pts',(-0.320601295512739,2.13280432935961,
13.2476518185281));
#36874=CARTESIAN_POINT('Ctrl Pts',(-0.320563119470224,2.13317530923575,
13.2476288946017));
#36875=CARTESIAN_POINT('Ctrl Pts',(-0.32047071803939,2.13405817780325,13.2475742812828));
#36876=CARTESIAN_POINT('Ctrl Pts',(-0.320415910126827,2.13457000330722,
13.2475425736246));
#36877=CARTESIAN_POINT('Ctrl Pts',(-0.32021696124988,2.13638676961118,13.2474298575485));
#36878=CARTESIAN_POINT('Ctrl Pts',(-0.320066074203459,2.13769094502954,
13.2473486372935));
#36879=CARTESIAN_POINT('Ctrl Pts',(-0.319526418107202,2.14211827317617,
13.2470718543437));
#36880=CARTESIAN_POINT('Ctrl Pts',(-0.319099879757327,2.14523656059779,
13.2468751088991));
#36881=CARTESIAN_POINT('Ctrl Pts',(-0.318214624174351,2.15107065737437,
13.246503519785));
#36882=CARTESIAN_POINT('Ctrl Pts',(-0.317766625696212,2.15378782325487,
13.246329027528));
#36883=CARTESIAN_POINT('Ctrl Pts',(-0.317111742987272,2.15746548616636,
13.2460908843058));
#36884=CARTESIAN_POINT('Ctrl Pts',(-0.316935198554853,2.15843132314595,
13.2460281577341));
#36885=CARTESIAN_POINT('Ctrl Pts',(-0.316346789335334,2.16156924627687,
13.2458237618279));
#36886=CARTESIAN_POINT('Ctrl Pts',(-0.315916993487235,2.16373786995476,
13.2456815626518));
#36887=CARTESIAN_POINT('Ctrl Pts',(-0.310324212617377,2.19050989458346,
13.2439144471589));
#36888=CARTESIAN_POINT('Ctrl Pts',(-0.302322265015784,2.21442925934373,
13.2422036375887));
#36889=CARTESIAN_POINT('Ctrl Pts',(-0.285036700002335,2.25117822255731,
13.2394677211623));
#36890=CARTESIAN_POINT('Ctrl Pts',(-0.27744678242937,2.26469421964319,13.2384376730576));
#36891=CARTESIAN_POINT('Ctrl Pts',(-0.268397569404883,2.27839505939664,
13.2374050602449));
#36892=CARTESIAN_POINT('Ctrl Pts',(-0.26787808281707,2.27917417581001,13.2373463839986));
#36893=CARTESIAN_POINT('Ctrl Pts',(-0.267163986518146,2.28023511644934,
13.2372665565599));
#36894=CARTESIAN_POINT('Ctrl Pts',(-0.266972319121646,2.28051890127954,
13.2372452111875));
#36895=CARTESIAN_POINT('Ctrl Pts',(-0.266650739143972,2.28099340371458,
13.2372095334631));
#36896=CARTESIAN_POINT('Ctrl Pts',(-0.266521073965429,2.28118428741845,
13.2371951844409));
#36897=CARTESIAN_POINT('Ctrl Pts',(-0.266265313025881,2.2815599315386,13.2371669538127));
#36898=CARTESIAN_POINT('Ctrl Pts',(-0.266139230206618,2.28174469952761,
13.2371530714535));
#36899=CARTESIAN_POINT('Ctrl Pts',(-0.265860228253173,2.28215264986376,
13.2371224277996));
#36900=CARTESIAN_POINT('Ctrl Pts',(-0.265707219923848,2.28237577169351,
13.2371056725679));
#36901=CARTESIAN_POINT('Ctrl Pts',(-0.265183414701852,2.28313754345954,
13.2370484831727));
#36902=CARTESIAN_POINT('Ctrl Pts',(-0.264811256220294,2.28367526195429,
13.2370081409302));
#36903=CARTESIAN_POINT('Ctrl Pts',(-0.261040237666083,2.28908858672199,
13.2366022348204));
#36904=CARTESIAN_POINT('Ctrl Pts',(-0.257508494216956,2.29387079632716,
13.236245516732));
#36905=CARTESIAN_POINT('Ctrl Pts',(-0.251490179513832,2.30156509945613,
13.2356697645654));
#36906=CARTESIAN_POINT('Ctrl Pts',(-0.249080618848116,2.30453519774991,
13.2354470507446));
#36907=CARTESIAN_POINT('Ctrl Pts',(-0.227921873930415,2.3296874985036,13.2335502049417));
#36908=CARTESIAN_POINT('Ctrl Pts',(-0.206306182745667,2.34928439089276,
13.2319863617403));
#36909=CARTESIAN_POINT('Ctrl Pts',(-0.175724206183174,2.37027184458794,
13.2298440779071));
#36910=CARTESIAN_POINT('Ctrl Pts',(-0.168924958401285,2.37457277729758,
13.2293725702221));
#36911=CARTESIAN_POINT('Ctrl Pts',(-0.159612980318856,2.37998628535088,
13.2287287631247));
#36912=CARTESIAN_POINT('Ctrl Pts',(-0.157236357768794,2.38132783470637,
13.2285646240746));
#36913=CARTESIAN_POINT('Ctrl Pts',(-0.153239324349628,2.38351759894937,
13.2282887090762));
#36914=CARTESIAN_POINT('Ctrl Pts',(-0.151628188883919,2.38438250924227,
13.2281775291729));
#36915=CARTESIAN_POINT('Ctrl Pts',(-0.149450151561957,2.38552798053293,
13.2280272467451));
#36916=CARTESIAN_POINT('Ctrl Pts',(-0.148889635844594,2.38582066370049,
13.227988573316));
#36917=CARTESIAN_POINT('Ctrl Pts',(-0.148002691761106,2.38628048020011,
13.2279273787445));
#36918=CARTESIAN_POINT('Ctrl Pts',(-0.147676831227424,2.38644871029385,
13.2279048962942));
#36919=CARTESIAN_POINT('Ctrl Pts',(-0.147000794286862,2.38679626372173,
13.2278582539206));
#36920=CARTESIAN_POINT('Ctrl Pts',(-0.146650575398872,2.38697550268047,
13.2278340910791));
#36921=CARTESIAN_POINT('Ctrl Pts',(-0.145851351666812,2.38738269330252,
13.2277789495913));
#36922=CARTESIAN_POINT('Ctrl Pts',(-0.145402139816339,2.38761023438864,
13.2277479566028));
#36923=CARTESIAN_POINT('Ctrl Pts',(-0.144030454665508,2.38830100467042,
13.2276533167197));
#36924=CARTESIAN_POINT('Ctrl Pts',(-0.143106294166735,2.38876085208229,
13.2275895516774));
#36925=CARTESIAN_POINT('Ctrl Pts',(-0.136364047529785,2.39207536947543,
13.2271243128556));
#36926=CARTESIAN_POINT('Ctrl Pts',(-0.130463600126605,2.39475822995283,
13.2267169066211));
#36927=CARTESIAN_POINT('Ctrl Pts',(-0.105322239585872,2.40528689077244,
13.224978134888));
#36928=CARTESIAN_POINT('Ctrl Pts',(-0.0854296244791532,2.41143921684941,
13.2235911177663));
#36929=CARTESIAN_POINT('Ctrl Pts',(-0.062997392440134,2.41606495390252,
13.2220422259398));
#36930=CARTESIAN_POINT('Ctrl Pts',(-0.0609038418287308,2.41647503622835,
13.221897863492));
#36931=CARTESIAN_POINT('Ctrl Pts',(-0.0564022552593713,2.41731047904094,
13.2215879942009));
#36932=CARTESIAN_POINT('Ctrl Pts',(-0.0539931288313977,2.4177292819042,
13.2214224910965));
#36933=CARTESIAN_POINT('Ctrl Pts',(-0.0435408139573372,2.41942400013965,
13.2207062958807));
#36934=CARTESIAN_POINT('Ctrl Pts',(-0.0354553710290919,2.42042225236733,
13.2201569582779));
#36935=CARTESIAN_POINT('Ctrl Pts',(-0.0217979875431622,2.42158508388674,
13.2192443399585));
#36936=CARTESIAN_POINT('Ctrl Pts',(-0.016243823534985,2.42191344044718,
13.2188774446051));
#36937=CARTESIAN_POINT('Ctrl Pts',(-0.00533430417689137,2.42227529849871,
13.2181683785087));
#36938=CARTESIAN_POINT('Ctrl Pts',(1.90551163048386E-5,2.42231945467463,
13.2178259027443));
#36939=CARTESIAN_POINT('Ctrl Pts',(0.00594829671087206,2.42222061741735,
13.217454434595));
#36940=CARTESIAN_POINT('Ctrl Pts',(0.00652516779550501,2.42220945163058,
13.2174183759355));
#36941=CARTESIAN_POINT('Ctrl Pts',(0.00738255421381879,2.42219055271838,
13.2173649086578));
#36942=CARTESIAN_POINT('Ctrl Pts',(0.00766309044230832,2.42218400241788,
13.2173474341973));
#36943=CARTESIAN_POINT('Ctrl Pts',(0.00814210509455091,2.42217219180168,
13.2173176311726));
#36944=CARTESIAN_POINT('Ctrl Pts',(0.00834058738309613,2.42216711447422,
13.217305292268));
#36945=CARTESIAN_POINT('Ctrl Pts',(0.00874875374904936,2.42215629581398,
13.217279939067));
#36946=CARTESIAN_POINT('Ctrl Pts',(0.00895843649401029,2.42215053319981,
13.2172669260097));
#36947=CARTESIAN_POINT('Ctrl Pts',(0.00952459711261236,2.42213442047981,
13.2172318200005));
#36948=CARTESIAN_POINT('Ctrl Pts',(0.00988106501800944,2.4221236833346,
13.2172097488915));
#36949=CARTESIAN_POINT('Ctrl Pts',(0.011197895396698,2.42208183125278,13.2171283333454));
#36950=CARTESIAN_POINT('Ctrl Pts',(0.0121581474168493,2.42204701270314,
13.2170691947901));
#36951=CARTESIAN_POINT('Ctrl Pts',(0.0133507180898196,2.42199842870043,
13.2169960194764));
#36952=CARTESIAN_POINT('Ctrl Pts',(0.0135831830166143,2.42198870616678,
13.2169817683792));
#36953=CARTESIAN_POINT('Ctrl Pts',(0.0327486286671742,2.42116634483214,
13.2158078839908));
#36954=CARTESIAN_POINT('Ctrl Pts',(0.0515763005692398,2.4186854391674,13.2147372668815));
#36955=CARTESIAN_POINT('Ctrl Pts',(0.0863009112098291,2.41094940647918,
13.2127445220053));
#36956=CARTESIAN_POINT('Ctrl Pts',(0.102218588373151,2.4060861281953,13.2118230268691));
#36957=CARTESIAN_POINT('Ctrl Pts',(0.126801722989407,2.39644275553252,13.2103120140148));
#36958=CARTESIAN_POINT('Ctrl Pts',(0.135745619543746,2.39245527165815,13.2097428740567));
#36959=CARTESIAN_POINT('Ctrl Pts',(0.147383728801952,2.38661762997997,13.2089676883943));
#36960=CARTESIAN_POINT('Ctrl Pts',(0.150251698682107,2.38512463107413,13.2087737800204));
#36961=CARTESIAN_POINT('Ctrl Pts',(0.154319881571491,2.38292840467492,13.2084943467172));
#36962=CARTESIAN_POINT('Ctrl Pts',(0.155538817366452,2.38226013572395,13.2084100511051));
#36963=CARTESIAN_POINT('Ctrl Pts',(0.15740539956484,2.3812210388538,13.2082800720528));
#36964=CARTESIAN_POINT('Ctrl Pts',(0.158056155129065,2.38085580698524,13.208234588334));
#36965=CARTESIAN_POINT('Ctrl Pts',(0.159263304780322,2.38017277872948,13.208149899586));
#36966=CARTESIAN_POINT('Ctrl Pts',(0.159820032024022,2.37985557622644,13.208110716023));
#36967=CARTESIAN_POINT('Ctrl Pts',(0.160735856784765,2.37933014924153,13.2080460492966));
#36968=CARTESIAN_POINT('Ctrl Pts',(0.161095506356642,2.37912288648688,13.2080206009424));
#36969=CARTESIAN_POINT('Ctrl Pts',(0.16179753380385,2.37871650570222,13.2079708215053));
#36970=CARTESIAN_POINT('Ctrl Pts',(0.162139947139263,2.37851745014507,13.2079464927194));
#36971=CARTESIAN_POINT('Ctrl Pts',(0.162928257195209,2.37805723450644,13.2078903692799));
#36972=CARTESIAN_POINT('Ctrl Pts',(0.163373893592153,2.37779563268996,13.207858558606));
#36973=CARTESIAN_POINT('Ctrl Pts',(0.16479336888695,2.37695776148477,13.20775696395));
#36974=CARTESIAN_POINT('Ctrl Pts',(0.165764794604688,2.37637743918968,13.2076870323102));
#36975=CARTESIAN_POINT('Ctrl Pts',(0.174463034386662,2.37111882153216,13.2070571750442));
#36976=CARTESIAN_POINT('Ctrl Pts',(0.181992345668761,2.36612313963779,13.2064855800994));
#36977=CARTESIAN_POINT('Ctrl Pts',(0.190088539838872,2.3602469378859,13.2058400666763));
#36978=CARTESIAN_POINT('Ctrl Pts',(0.190873105205912,2.35967206113675,13.2057771818182));
#36979=CARTESIAN_POINT('Ctrl Pts',(0.213642754672032,2.3428290456307,13.203942479105));
#36980=CARTESIAN_POINT('Ctrl Pts',(0.23346866267692,2.3238328322786,13.2020678405428));
#36981=CARTESIAN_POINT('Ctrl Pts',(0.253567017407664,2.2989633489604,13.1999235837407));
#36982=CARTESIAN_POINT('Ctrl Pts',(0.25640156704276,2.29529691709814,13.1996146376598));
#36983=CARTESIAN_POINT('Ctrl Pts',(0.262571558963039,2.28695016637314,13.1989291453272));
#36984=CARTESIAN_POINT('Ctrl Pts',(0.265863020899388,2.28223899394042,13.1985542713795));
#36985=CARTESIAN_POINT('Ctrl Pts',(0.270738766509925,2.27484668186106,13.1979872136151));
#36986=CARTESIAN_POINT('Ctrl Pts',(0.272413020193182,2.27222656602066,13.197790177345));
#36987=CARTESIAN_POINT('Ctrl Pts',(0.27431747495842,2.2691489241659,13.1975636664284));
#36988=CARTESIAN_POINT('Ctrl Pts',(0.274584754747601,2.26871469432964,13.1975318205444));
#36989=CARTESIAN_POINT('Ctrl Pts',(0.274990271116812,2.26805236550117,13.1974834201294));
#36990=CARTESIAN_POINT('Ctrl Pts',(0.275129255395169,2.26782472876896,13.1974668165278));
#36991=CARTESIAN_POINT('Ctrl Pts',(0.275370255986218,2.26742889965142,13.1974379996797));
#36992=CARTESIAN_POINT('Ctrl Pts',(0.275472400489772,2.26726078706444,13.1974257779592));
#36993=CARTESIAN_POINT('Ctrl Pts',(0.275686360584953,2.26690791727649,13.1974001602889));
#36994=CARTESIAN_POINT('Ctrl Pts',(0.275798144013824,2.266723141829,13.1973867664853));
#36995=CARTESIAN_POINT('Ctrl Pts',(0.276109705297572,2.26620696736693,13.1973494074915));
#36996=CARTESIAN_POINT('Ctrl Pts',(0.276309072990298,2.26587531928466,13.1973254693052));
#36997=CARTESIAN_POINT('Ctrl Pts',(0.27710915226221,2.26453894275921,13.1972292699536));
#36998=CARTESIAN_POINT('Ctrl Pts',(0.277704994491041,2.26353128778696,13.1971573232983));
#36999=CARTESIAN_POINT('Ctrl Pts',(0.288224106363828,2.24551865660134,13.1958812809199));
#37000=CARTESIAN_POINT('Ctrl Pts',(0.296575668554731,2.22763988250608,13.1947726313028));
#37001=CARTESIAN_POINT('Ctrl Pts',(0.308784109651684,2.19370899862269,13.192754278719));
#37002=CARTESIAN_POINT('Ctrl Pts',(0.313143591071176,2.17791063254559,13.1918453988327));
#37003=CARTESIAN_POINT('Ctrl Pts',(0.318671921027294,2.14964035505235,13.1901940816162));
#37004=CARTESIAN_POINT('Ctrl Pts',(0.320350329878614,2.13730375395253,13.189465719512));
#37005=CARTESIAN_POINT('Ctrl Pts',(0.321421511985437,2.12348222747628,13.188628039931));
#37006=CARTESIAN_POINT('Ctrl Pts',(0.32152213037569,2.12206179849046,13.188541706775));
#37007=CARTESIAN_POINT('Ctrl Pts',(0.321661985134296,2.1198826568207,13.1884088655862));
#37008=CARTESIAN_POINT('Ctrl Pts',(0.321707958718722,2.11912438245705,13.1883625679059));
#37009=CARTESIAN_POINT('Ctrl Pts',(0.321779171870183,2.11787680686395,13.1882862724147));
#37010=CARTESIAN_POINT('Ctrl Pts',(0.321805977575803,2.11738759515941,13.1882563236448));
#37011=CARTESIAN_POINT('Ctrl Pts',(0.321855651404073,2.11644154815703,13.1881983473708));
#37012=CARTESIAN_POINT('Ctrl Pts',(0.321878662741033,2.11598472130233,13.1881703244192));
#37013=CARTESIAN_POINT('Ctrl Pts',(0.321919150891103,2.11514538006495,13.1881187861475));
#37014=CARTESIAN_POINT('Ctrl Pts',(0.321936918697785,2.11476287997605,13.188095279992));
#37015=CARTESIAN_POINT('Ctrl Pts',(0.321974403078859,2.11392366213582,13.1880436637399));
#37016=CARTESIAN_POINT('Ctrl Pts',(0.321993829631447,2.11346693287672,13.1880155446054));
#37017=CARTESIAN_POINT('Ctrl Pts',(0.322044177814712,2.11222077399748,13.1879387462635));
#37018=CARTESIAN_POINT('Ctrl Pts',(0.322073168321577,2.11143127337538,13.1878900066494));
#37019=CARTESIAN_POINT('Ctrl Pts',(0.322198926036979,2.1076248755538,13.1876546069605));
#37020=CARTESIAN_POINT('Ctrl Pts',(0.322256205657304,2.10460690621253,13.1874667145118));
#37021=CARTESIAN_POINT('Ctrl Pts',(0.322276998411832,2.1003889410247,13.1872022789311));
#37022=CARTESIAN_POINT('Ctrl Pts',(0.322276213121028,2.09918921377692,13.1871268577795));
#37023=CARTESIAN_POINT('Ctrl Pts',(0.322263229994967,2.09710807890913,13.1869956629524));
#37024=CARTESIAN_POINT('Ctrl Pts',(0.322254114776638,2.09622665940697,13.1869399850383));
#37025=CARTESIAN_POINT('Ctrl Pts',(0.322218656853498,2.09377193648883,13.1867846063821));
#37026=CARTESIAN_POINT('Ctrl Pts',(0.322184407674301,2.09219878778271,13.1866846659551));
#37027=CARTESIAN_POINT('Ctrl Pts',(0.32123049791921,2.05941765234215,13.1845944719271));
#37028=CARTESIAN_POINT('Ctrl Pts',(0.315791810869729,2.02851068592621,13.1824553493103));
#37029=CARTESIAN_POINT('Ctrl Pts',(0.302228035049034,1.98746631691699,13.1795571754119));
#37030=CARTESIAN_POINT('Ctrl Pts',(0.297821129502904,1.9762734584719,13.1787635063836));
#37031=CARTESIAN_POINT('Ctrl Pts',(0.292126235947137,1.96388964734301,13.1779008269239));
#37032=CARTESIAN_POINT('Ctrl Pts',(0.291442855257529,1.96243245948172,13.1777995718464));
#37033=CARTESIAN_POINT('Ctrl Pts',(0.290568308307015,1.96060341303054,13.1776728572627));
#37034=CARTESIAN_POINT('Ctrl Pts',(0.290387312074675,1.96022675777576,13.1776467833436));
#37035=CARTESIAN_POINT('Ctrl Pts',(0.290098206548865,1.95962811126287,13.1776053758506));
#37036=CARTESIAN_POINT('Ctrl Pts',(0.289990574648707,1.95940589199261,13.1775900126853));
#37037=CARTESIAN_POINT('Ctrl Pts',(0.289787030902136,1.95898687907789,13.1775610584638));
#37038=CARTESIAN_POINT('Ctrl Pts',(0.289691174682163,1.95879006103359,13.1775474641382));
#37039=CARTESIAN_POINT('Ctrl Pts',(0.289472680526909,1.95834259384912,13.1775165708343));
#37040=CARTESIAN_POINT('Ctrl Pts',(0.289349917800132,1.95809200671105,13.1774992798084));
#37041=CARTESIAN_POINT('Ctrl Pts',(0.288984145472422,1.95734782870726,13.1774479576333));
#37042=CARTESIAN_POINT('Ctrl Pts',(0.288740195667025,1.95685469715812,13.1774139850255));
#37043=CARTESIAN_POINT('Ctrl Pts',(0.287053077269109,1.95346613820736,13.1771807745509));
#37044=CARTESIAN_POINT('Ctrl Pts',(0.285567579417923,1.9505918297393,13.1769841269981));
#37045=CARTESIAN_POINT('Ctrl Pts',(0.267766696179407,1.917384467472,13.1747202927847));
#37046=CARTESIAN_POINT('Ctrl Pts',(0.246731427960973,1.88982893112825,13.1729000995787));
#37047=CARTESIAN_POINT('Ctrl Pts',(0.213156448041101,1.85799791883507,13.170241273147));
#37048=CARTESIAN_POINT('Ctrl Pts',(0.204145711070526,1.8503499248823,13.1695483304205));
#37049=CARTESIAN_POINT('Ctrl Pts',(0.193636140072587,1.84237987789917,13.1687510075561));
#37050=CARTESIAN_POINT('Ctrl Pts',(0.192530646211191,1.84155265094913,13.1686672719658));
#37051=CARTESIAN_POINT('Ctrl Pts',(0.190822306579979,1.84029136577644,13.1685380631465));
#37052=CARTESIAN_POINT('Ctrl Pts',(0.190223209779657,1.83985223847697,13.1684927864428));
#37053=CARTESIAN_POINT('Ctrl Pts',(0.189106138489201,1.83903936697325,13.1684084268837));
#37054=CARTESIAN_POINT('Ctrl Pts',(0.188588559705034,1.83866508319182,13.1683693651045));
#37055=CARTESIAN_POINT('Ctrl Pts',(0.187733104604984,1.83805033108631,13.1683048433984));
#37056=CARTESIAN_POINT('Ctrl Pts',(0.187395869067517,1.83780897066737,13.1682794179192));
#37057=CARTESIAN_POINT('Ctrl Pts',(0.186735091745805,1.83733797658044,13.1682296187032));
#37058=CARTESIAN_POINT('Ctrl Pts',(0.18641158982547,1.83710828804872,13.1682052471355));
#37059=CARTESIAN_POINT('Ctrl Pts',(0.185663919414702,1.83657951099812,13.1681489404626));
#37060=CARTESIAN_POINT('Ctrl Pts',(0.18523945175659,1.83628084918552,13.1681169890894));
#37061=CARTESIAN_POINT('Ctrl Pts',(0.183878627009978,1.83532825888816,13.1680146011897));
#37062=CARTESIAN_POINT('Ctrl Pts',(0.182939522369073,1.83467828751532,13.1679440139995));
#37063=CARTESIAN_POINT('Ctrl Pts',(0.17429067854855,1.82876001380216,13.1672945380636));
#37064=CARTESIAN_POINT('Ctrl Pts',(0.166359545756294,1.82382461523632,13.1667031769179));
#37065=CARTESIAN_POINT('Ctrl Pts',(0.152383581031761,1.81594825377416,13.1656666821713));
#37066=CARTESIAN_POINT('Ctrl Pts',(0.146440157357755,1.81283903243551,13.1652275873111));
#37067=CARTESIAN_POINT('Ctrl Pts',(0.12042370678694,1.80024666675599,13.1633146309699));
#37068=CARTESIAN_POINT('Ctrl Pts',(0.0994977094055758,1.79266628304339,
13.161793517804));
#37069=CARTESIAN_POINT('Ctrl Pts',(0.0671131119549469,1.78459230919784,
13.159560977551));
#37070=CARTESIAN_POINT('Ctrl Pts',(0.0561298973154182,1.7824536686134,13.1588249075766));
#37071=CARTESIAN_POINT('Ctrl Pts',(0.0440448436074629,1.78074732351417,
13.1580528492691));
#37072=CARTESIAN_POINT('Ctrl Pts',(0.0430323937090804,1.78060927870665,
13.1579884575212));
#37073=CARTESIAN_POINT('Ctrl Pts',(0.0412840281338727,1.78037935829573,
13.1578777799429));
#37074=CARTESIAN_POINT('Ctrl Pts',(0.040548427256948,1.78028520419719,13.1578313719749));
#37075=CARTESIAN_POINT('Ctrl Pts',(0.0395038875445841,1.78015517010413,
13.1577657041466));
#37076=CARTESIAN_POINT('Ctrl Pts',(0.0391952187420621,1.78011719775523,
13.1577463274058));
#37077=CARTESIAN_POINT('Ctrl Pts',(0.0386644096994556,1.78005267762069,
13.1577130554387));
#37078=CARTESIAN_POINT('Ctrl Pts',(0.0384422963018082,1.78002591428169,
13.1576991479614));
#37079=CARTESIAN_POINT('Ctrl Pts',(0.0380164320243075,1.77997505001049,
13.1576725116372));
#37080=CARTESIAN_POINT('Ctrl Pts',(0.0378126863099761,1.77995091239896,
13.1576597806995));
#37081=CARTESIAN_POINT('Ctrl Pts',(0.0373319664819103,1.77989442731473,
13.157629772725));
#37082=CARTESIAN_POINT('Ctrl Pts',(0.0370549726278806,1.77986224466571,
13.1576125050623));
#37083=CARTESIAN_POINT('Ctrl Pts',(0.0362345377804529,1.77976800116962,
13.1575614271024));
#37084=CARTESIAN_POINT('Ctrl Pts',(0.0356909766952838,1.77970696386599,
13.1575276742666));
#37085=CARTESIAN_POINT('Ctrl Pts',(0.0308395887537717,1.77917469743018,
13.1572271853582));
#37086=CARTESIAN_POINT('Ctrl Pts',(0.0265225662064618,1.77878898996396,
13.1569651504885));
#37087=CARTESIAN_POINT('Ctrl Pts',(-0.00745675486368154,1.77644286677046,
13.1549354959716));
#37088=CARTESIAN_POINT('Ctrl Pts',(-0.0372567417464889,1.77850774781622,
13.1533404233214));
#37089=CARTESIAN_POINT('Ctrl Pts',(-0.080973642123726,1.78770586424096,
13.1508021649634));
#37090=CARTESIAN_POINT('Ctrl Pts',(-0.0953594772313317,1.79179415623468,
13.1499349706324));
#37091=CARTESIAN_POINT('Ctrl Pts',(-0.110899772519987,1.79740302611123,
13.1489381186997));
#37092=CARTESIAN_POINT('Ctrl Pts',(-0.112386717573886,1.797952133385,13.1488421243433));
#37093=CARTESIAN_POINT('Ctrl Pts',(-0.114985459082477,1.79893365720745,
13.1486732500931));
#37094=CARTESIAN_POINT('Ctrl Pts',(-0.116099026324078,1.79936132219953,
13.1486005291913));
#37095=CARTESIAN_POINT('Ctrl Pts',(-0.117707671663017,1.79998939205323,
13.1484949494165));
#37096=CARTESIAN_POINT('Ctrl Pts',(-0.118204675336389,1.80018486433785,
13.1484622564439));
#37097=CARTESIAN_POINT('Ctrl Pts',(-0.119070908759118,1.80052804395081,
13.1484051466468));
#37098=CARTESIAN_POINT('Ctrl Pts',(-0.119440356285209,1.80067520139351,
13.1483807483987));
#37099=CARTESIAN_POINT('Ctrl Pts',(-0.120153470884081,1.800960777946,13.1483335748189));
#37100=CARTESIAN_POINT('Ctrl Pts',(-0.120497173692491,1.80109910668836,
13.1483108025689));
#37101=CARTESIAN_POINT('Ctrl Pts',(-0.121311385508265,1.80142843197987,
13.1482567711376));
#37102=CARTESIAN_POINT('Ctrl Pts',(-0.12178168208099,1.80161994807168,13.1482254944164));
#37103=CARTESIAN_POINT('Ctrl Pts',(-0.123432484548044,1.80229674761582,
13.1481154697758));
#37104=CARTESIAN_POINT('Ctrl Pts',(-0.124610546548384,1.80278792700235,
13.1480365221996));
#37105=CARTESIAN_POINT('Ctrl Pts',(-0.141732461682995,1.81004640413557,
13.1468827293306));
#37106=CARTESIAN_POINT('Ctrl Pts',(-0.157105573400245,1.81808008338434,
13.1457636687784));
#37107=CARTESIAN_POINT('Ctrl Pts',(-0.181832283745838,1.83365439735847,
13.1438210455253));
#37108=CARTESIAN_POINT('Ctrl Pts',(-0.191547690559377,1.84055363580459,
13.1430164424767));
#37109=CARTESIAN_POINT('Ctrl Pts',(-0.210159366238616,1.85538670186657,
13.1414058370563));
#37110=CARTESIAN_POINT('Ctrl Pts',(-0.219043076928487,1.86330868294766,
13.1406010764666));
#37111=CARTESIAN_POINT('Ctrl Pts',(-0.233378553863066,1.87759221472451,
13.139261565831));
#37112=CARTESIAN_POINT('Ctrl Pts',(-0.239057998629047,1.88370836184933,
13.1387185403232));
#37113=CARTESIAN_POINT('Ctrl Pts',(-0.245345128406196,1.89102954823742,
13.1381094099944));
#37114=CARTESIAN_POINT('Ctrl Pts',(-0.246190089423904,1.89202567045372,
13.1380273700341));
#37115=CARTESIAN_POINT('Ctrl Pts',(-0.247278040055303,1.89332417432803,
13.1379215393394));
#37116=CARTESIAN_POINT('Ctrl Pts',(-0.247526557228097,1.89362187741586,
13.1378973512053));
#37117=CARTESIAN_POINT('Ctrl Pts',(-0.247928042885322,1.8941045925644,13.1378582537083));
#37118=CARTESIAN_POINT('Ctrl Pts',(-0.248081342120482,1.89428932710085,
13.1378433201413));
#37119=CARTESIAN_POINT('Ctrl Pts',(-0.248375036564697,1.89464405184302,
13.1378147007844));
#37120=CARTESIAN_POINT('Ctrl Pts',(-0.248515463315888,1.89481401430634,
13.1378010127143));
#37121=CARTESIAN_POINT('Ctrl Pts',(-0.24883809811766,1.89520532539957,13.1377695543678));
#37122=CARTESIAN_POINT('Ctrl Pts',(-0.249020185838086,1.89542677382854,
13.1377517929243));
#37123=CARTESIAN_POINT('Ctrl Pts',(-0.249583483061063,1.89611370178924,
13.137696824039));
#37124=CARTESIAN_POINT('Ctrl Pts',(-0.249963687524055,1.89658000946777,
13.13765968937));
#37125=CARTESIAN_POINT('Ctrl Pts',(-0.25310157907732,1.90045060697281,13.1373529126579));
#37126=CARTESIAN_POINT('Ctrl Pts',(-0.255791054563873,1.90390994258175,
13.1370880602181));
#37127=CARTESIAN_POINT('Ctrl Pts',(-0.258519376379704,1.90757094400929,
13.1368160750597));
#37128=CARTESIAN_POINT('Ctrl Pts',(-0.258629317155157,1.90771873242204,
13.1368051093541));
#37129=CARTESIAN_POINT('Ctrl Pts',(-0.259217291643297,1.90851053655655,
13.1367464322878));
#37130=CARTESIAN_POINT('Ctrl Pts',(-0.259693050873104,1.90915624650303,
13.1366988426192));
#37131=CARTESIAN_POINT('Ctrl Pts',(-0.260341359482322,1.91004305736347,
13.1366338299425));
#37132=CARTESIAN_POINT('Ctrl Pts',(-0.260515990228434,1.91028262507251,
13.1366163015428));
#37133=CARTESIAN_POINT('Ctrl Pts',(-0.277871270752546,1.9341606662873,13.1348726132801));
#37134=CARTESIAN_POINT('Ctrl Pts',(-0.29175920876836,1.9600281575405,13.1333031384424));
#37135=CARTESIAN_POINT('Ctrl Pts',(-0.307457857108944,2.00213483659472,
13.1307435365567));
#37136=CARTESIAN_POINT('Ctrl Pts',(-0.311861221815125,2.01723286754563,
13.12982714177));
#37137=CARTESIAN_POINT('Ctrl Pts',(-0.315393806445226,2.03374802692001,
13.1288003774934));
#37138=CARTESIAN_POINT('Ctrl Pts',(-0.315635042852909,2.03490701461971,
13.1287282041958));
#37139=CARTESIAN_POINT('Ctrl Pts',(-0.315975515215974,2.0365891734354,13.1286232722474));
#37140=CARTESIAN_POINT('Ctrl Pts',(-0.316079850795476,2.03711131216712,
13.1285906765864));
#37141=CARTESIAN_POINT('Ctrl Pts',(-0.316259809667588,2.03802366259876,
13.128533676587));
#37142=CARTESIAN_POINT('Ctrl Pts',(-0.316336006158008,2.03841376116076,
13.1285092905967));
#37143=CARTESIAN_POINT('Ctrl Pts',(-0.316481931661086,2.03916826314085,
13.1284620970564));
#37144=CARTESIAN_POINT('Ctrl Pts',(-0.316551753491421,2.03953264817315,
13.1284392925077));
#37145=CARTESIAN_POINT('Ctrl Pts',(-0.316715987653266,2.04039783139133,
13.1283851160599));
#37146=CARTESIAN_POINT('Ctrl Pts',(-0.316809841422015,2.04089873341936,
13.12835372641));
#37147=CARTESIAN_POINT('Ctrl Pts',(-0.317136477369064,2.04266514112886,
13.1282429465762));
#37148=CARTESIAN_POINT('Ctrl Pts',(-0.317362865792543,2.04393180350001,
13.1281633531708));
#37149=CARTESIAN_POINT('Ctrl Pts',(-0.320721263789985,2.06339459902744,
13.126937904173));
#37150=CARTESIAN_POINT('Ctrl Pts',(-0.322290923176652,2.08182222789064,
13.1257415472982));
#37151=CARTESIAN_POINT('Ctrl Pts',(-0.322253006248937,2.1254414566591,13.1228329141351));
#37152=CARTESIAN_POINT('Ctrl Pts',(-0.319284709249872,2.15051232414512,
13.1210974374452));
#37153=CARTESIAN_POINT('Ctrl Pts',(-0.313323395040868,2.17543101939966,
13.1194202283871));
#37154=CARTESIAN_POINT('Ctrl Pts',(-0.313215065641186,2.17587958373119,
13.1193900557357));
#37155=CARTESIAN_POINT('Ctrl Pts',(-0.311632950742687,2.1823695985687,13.118953794462));
#37156=CARTESIAN_POINT('Ctrl Pts',(-0.30998544133701,2.18836789935263,13.118554197901));
#37157=CARTESIAN_POINT('Ctrl Pts',(-0.307969276497932,2.19495550916034,
13.1181221692465));
#37158=CARTESIAN_POINT('Ctrl Pts',(-0.307771318510728,2.19559518558902,
13.118080290219));
#37159=CARTESIAN_POINT('Ctrl Pts',(-0.307491176693233,2.19649053837735,
13.1180217781899));
#37160=CARTESIAN_POINT('Ctrl Pts',(-0.30741066653164,2.19674673040679,13.1180050480017));
#37161=CARTESIAN_POINT('Ctrl Pts',(-0.307262748794474,2.19721537175826,
13.117974466834));
#37162=CARTESIAN_POINT('Ctrl Pts',(-0.307195440914091,2.19742785220539,
13.1179606099689));
#37163=CARTESIAN_POINT('Ctrl Pts',(-0.30705812660608,2.19785977501212,13.1179324598245));
#37164=CARTESIAN_POINT('Ctrl Pts',(-0.306988105311617,2.19807921226357,
13.1179181674523));
#37165=CARTESIAN_POINT('Ctrl Pts',(-0.30681304730563,2.19862579624533,13.1178825899624));
#37166=CARTESIAN_POINT('Ctrl Pts',(-0.306707722241865,2.19895285140819,
13.1178613219114));
#37167=CARTESIAN_POINT('Ctrl Pts',(-0.306309056872683,2.20018403462883,
13.1177813331873));
#37168=CARTESIAN_POINT('Ctrl Pts',(-0.306012236388668,2.20108704343583,
13.1177228156871));
#37169=CARTESIAN_POINT('Ctrl Pts',(-0.303709753905448,2.2079887386341,13.1172766221947));
#37170=CARTESIAN_POINT('Ctrl Pts',(-0.301531721568479,2.21392899514777,
13.1168986965569));
#37171=CARTESIAN_POINT('Ctrl Pts',(-0.294696281257612,2.23099909341191,
13.11582010347));
#37172=CARTESIAN_POINT('Ctrl Pts',(-0.289587036975815,2.24193679376754,
13.1151381732785));
#37173=CARTESIAN_POINT('Ctrl Pts',(-0.272109580616609,2.27445735314753,
13.1130676153323));
#37174=CARTESIAN_POINT('Ctrl Pts',(-0.257850809630431,2.29491499395365,
13.1116967463171));
#37175=CARTESIAN_POINT('Ctrl Pts',(-0.241062068602797,2.31389364109768,
13.1102041849633));
#37176=CARTESIAN_POINT('Ctrl Pts',(-0.240740059711737,2.31425600170733,
13.1101756000938));
#37177=CARTESIAN_POINT('Ctrl Pts',(-0.236027419658964,2.31953515737534,
13.1097578665379));
#37178=CARTESIAN_POINT('Ctrl Pts',(-0.231488026074143,2.32431654530755,
13.1093631427797));
#37179=CARTESIAN_POINT('Ctrl Pts',(-0.226068716071867,2.32968497266832,
13.1088988886345));
#37180=CARTESIAN_POINT('Ctrl Pts',(-0.225328463125049,2.33041122959249,
13.1088356196183));
#37181=CARTESIAN_POINT('Ctrl Pts',(-0.224223004852126,2.33148536474811,
13.1087413467001));
#37182=CARTESIAN_POINT('Ctrl Pts',(-0.223860462286072,2.33183598387218,
13.108710462523));
#37183=CARTESIAN_POINT('Ctrl Pts',(-0.223213707639791,2.33245853623972,
13.1086554252819));
#37184=CARTESIAN_POINT('Ctrl Pts',(-0.222929817313236,2.33273080350381,
13.108631286793));
#37185=CARTESIAN_POINT('Ctrl Pts',(-0.222331578477663,2.33330245022302,
13.1085804613781));
#37186=CARTESIAN_POINT('Ctrl Pts',(-0.222017122330506,2.33360171544228,
13.1085537695836));
#37187=CARTESIAN_POINT('Ctrl Pts',(-0.22118787285423,2.3343877182231,13.1084834430083));
#37188=CARTESIAN_POINT('Ctrl Pts',(-0.220672079589491,2.33487339318971,
13.1084397626066));
#37189=CARTESIAN_POINT('Ctrl Pts',(-0.218358157672523,2.33703784968652,
13.1082440812253));
#37190=CARTESIAN_POINT('Ctrl Pts',(-0.216542482121872,2.33869767511017,
13.1080912735306));
#37191=CARTESIAN_POINT('Ctrl Pts',(-0.203113995651687,2.35069420324249,
13.1069662180705));
#37192=CARTESIAN_POINT('Ctrl Pts',(-0.190787464491034,2.3601977997522,13.1059594533601));
#37193=CARTESIAN_POINT('Ctrl Pts',(-0.150962634025548,2.38654652239965,
13.1027875471387));
#37194=CARTESIAN_POINT('Ctrl Pts',(-0.121589723911327,2.40019076005394,
13.1005384838953));
#37195=CARTESIAN_POINT('Ctrl Pts',(-0.0892470126214924,2.40967464362763,
13.09840682535));
#37196=CARTESIAN_POINT('Ctrl Pts',(-0.0878083411675966,2.41008564880571,
13.0983127252413));
#37197=CARTESIAN_POINT('Ctrl Pts',(-0.0859563561977601,2.41060080807551,
13.0981925618348));
#37198=CARTESIAN_POINT('Ctrl Pts',(-0.0855456567573275,2.41071417373993,
13.0981659753228));
#37199=CARTESIAN_POINT('Ctrl Pts',(-0.0848949273519165,2.41089240703937,
13.0981239486413));
#37200=CARTESIAN_POINT('Ctrl Pts',(-0.0846550468944974,2.41095781141678,
13.0981084772973));
#37201=CARTESIAN_POINT('Ctrl Pts',(-0.084225280111226,2.41107445490901,
13.0980807970893));
#37202=CARTESIAN_POINT('Ctrl Pts',(-0.0840354239436804,2.41112579743518,
13.0980685822451));
#37203=CARTESIAN_POINT('Ctrl Pts',(-0.0835892051609647,2.41124602948818,
13.0980399048934));
#37204=CARTESIAN_POINT('Ctrl Pts',(-0.0833328047323441,2.41131477598768,
13.0980234508257));
#37205=CARTESIAN_POINT('Ctrl Pts',(-0.0825901501201167,2.41151291451913,
13.0979758613039));
#37206=CARTESIAN_POINT('Ctrl Pts',(-0.082103674687822,2.41164148539618,
13.0979447735235));
#37207=CARTESIAN_POINT('Ctrl Pts',(-0.0787640224052549,2.41251576130564,
13.097731931086));
#37208=CARTESIAN_POINT('Ctrl Pts',(-0.075900909784012,2.4132234436762,13.0975523366848));
#37209=CARTESIAN_POINT('Ctrl Pts',(-0.0668910435168518,2.41531963065269,
13.096995011878));
#37210=CARTESIAN_POINT('Ctrl Pts',(-0.0607127345015744,2.41656730078298,
13.0966241992132));
#37211=CARTESIAN_POINT('Ctrl Pts',(-0.0392078355984223,2.42025724177956,
13.0953603168399));
#37212=CARTESIAN_POINT('Ctrl Pts',(-0.0237436830089551,2.42177361073879,
13.0944974048763));
#37213=CARTESIAN_POINT('Ctrl Pts',(0.00791816849111961,2.42258239136098,
13.0927267098881));
#37214=CARTESIAN_POINT('Ctrl Pts',(0.0240732424119309,2.42178023592525,
13.0918206258763));
#37215=CARTESIAN_POINT('Ctrl Pts',(0.0498711807509808,2.41854518807796,
13.0903080928411));
#37216=CARTESIAN_POINT('Ctrl Pts',(0.0595811165778582,2.41687258058835,
13.0897238604599));
#37217=CARTESIAN_POINT('Ctrl Pts',(0.0702162387756829,2.41453448319897,
13.089061727398));
#37218=CARTESIAN_POINT('Ctrl Pts',(0.0712327970479158,2.41430582223988,
13.0889982127875));
#37219=CARTESIAN_POINT('Ctrl Pts',(0.0727513047835294,2.41395650935331,
13.0889029939564));
#37220=CARTESIAN_POINT('Ctrl Pts',(0.0732541091407909,2.41383957303393,
13.0888714090847));
#37221=CARTESIAN_POINT('Ctrl Pts',(0.0741194658921079,2.4136361256758,13.088816951874));
#37222=CARTESIAN_POINT('Ctrl Pts',(0.0744821542365156,2.41355019255528,
13.0887940981617));
#37223=CARTESIAN_POINT('Ctrl Pts',(0.0752302827170993,2.41337156435153,
13.0887468956383));
#37224=CARTESIAN_POINT('Ctrl Pts',(0.0756157023975147,2.4132787869144,13.0887225442077));
#37225=CARTESIAN_POINT('Ctrl Pts',(0.07651225269705,2.4130612202743,13.088665819798));
#37226=CARTESIAN_POINT('Ctrl Pts',(0.0770232497612231,2.41293589030885,
13.0886334294292));
#37227=CARTESIAN_POINT('Ctrl Pts',(0.0786501089781209,2.41253265168059,
13.0885301164451));
#37228=CARTESIAN_POINT('Ctrl Pts',(0.0797647821857898,2.41225002398189,
13.0884590416309));
#37229=CARTESIAN_POINT('Ctrl Pts',(0.103335565093096,2.40613915463422,13.0869499064733));
#37230=CARTESIAN_POINT('Ctrl Pts',(0.125093999268113,2.39791021857387,13.0854299383529));
#37231=CARTESIAN_POINT('Ctrl Pts',(0.167131032246705,2.37658938942965,13.0822569474135));
#37232=CARTESIAN_POINT('Ctrl Pts',(0.18721232471678,2.36341247202198,13.0806119040556));
#37233=CARTESIAN_POINT('Ctrl Pts',(0.208387877028438,2.34586240063223,13.0788445023761));
#37234=CARTESIAN_POINT('Ctrl Pts',(0.211088871349678,2.34354736361537,13.0786185171938));
#37235=CARTESIAN_POINT('Ctrl Pts',(0.214180244910568,2.34080765582103,13.0783597825881));
#37236=CARTESIAN_POINT('Ctrl Pts',(0.21460836056838,2.34042619657217,13.0783239492136));
#37237=CARTESIAN_POINT('Ctrl Pts',(0.215243955217368,2.33985681921156,13.0782707499646));
#37238=CARTESIAN_POINT('Ctrl Pts',(0.215452208195212,2.33966977273978,13.0782533192241));
#37239=CARTESIAN_POINT('Ctrl Pts',(0.215819219694456,2.33933926927883,13.0782226008915));
#37240=CARTESIAN_POINT('Ctrl Pts',(0.21597807896954,2.33919592558004,13.0782093047717));
#37241=CARTESIAN_POINT('Ctrl Pts',(0.216314533114263,2.33889172401483,13.0781811448852));
#37242=CARTESIAN_POINT('Ctrl Pts',(0.216492090888996,2.33873082671207,13.0781662842343));
#37243=CARTESIAN_POINT('Ctrl Pts',(0.216855957544523,2.33840036234422,13.0781358305881));
#37244=CARTESIAN_POINT('Ctrl Pts',(0.217042247442515,2.33823077449094,13.0781202391854));
#37245=CARTESIAN_POINT('Ctrl Pts',(0.217504479164869,2.33780899249834,13.0780815525566));
#37246=CARTESIAN_POINT('Ctrl Pts',(0.217780182271521,2.33755653555087,13.078058477083));
#37247=CARTESIAN_POINT('Ctrl Pts',(0.218548874194158,2.33685019370729,13.0779941367495));
#37248=CARTESIAN_POINT('Ctrl Pts',(0.219040891016237,2.33639524688971,13.077952950656));
#37249=CARTESIAN_POINT('Ctrl Pts',(0.223433722231753,2.33230789487173,13.0775851598428));
#37250=CARTESIAN_POINT('Ctrl Pts',(0.227245548325914,2.32858052159811,13.077265497385));
#37251=CARTESIAN_POINT('Ctrl Pts',(0.23555682967224,2.32003984970661,13.0765624730784));
#37252=CARTESIAN_POINT('Ctrl Pts',(0.240004739919378,2.31517966925828,13.076182002696));
#37253=CARTESIAN_POINT('Ctrl Pts',(0.262616274645169,2.28889814962329,13.0742039340899));
#37254=CARTESIAN_POINT('Ctrl Pts',(0.278070515415464,2.26530790843284,13.0726836389549));
#37255=CARTESIAN_POINT('Ctrl Pts',(0.29137208088291,2.23773125916035,13.0709041826914));
#37256=CARTESIAN_POINT('Ctrl Pts',(0.292445386241801,2.23543738359043,13.0707562524421));
#37257=CARTESIAN_POINT('Ctrl Pts',(0.296656654435833,2.22615351838009,13.070157470565));
#37258=CARTESIAN_POINT('Ctrl Pts',(0.299571723524877,2.21906573273273,13.0697000858954));
#37259=CARTESIAN_POINT('Ctrl Pts',(0.302569700958455,2.21096712023805,13.069174691213));
#37260=CARTESIAN_POINT('Ctrl Pts',(0.302903935112911,2.21005149600274,13.0691152524391));
#37261=CARTESIAN_POINT('Ctrl Pts',(0.303403045243259,2.20866469957226,13.0690251646235));
#37262=CARTESIAN_POINT('Ctrl Pts',(0.303570990791344,2.20819463175939,13.0689946177078));
#37263=CARTESIAN_POINT('Ctrl Pts',(0.303860955567561,2.2073770504376,13.0689414684775));
#37264=CARTESIAN_POINT('Ctrl Pts',(0.303983472752198,2.20702971349488,13.0689188827426));
#37265=CARTESIAN_POINT('Ctrl Pts',(0.304237567888071,2.20630539655903,13.0688717706871));
#37266=CARTESIAN_POINT('Ctrl Pts',(0.304369041149942,2.20592838070719,13.0688472409385));
#37267=CARTESIAN_POINT('Ctrl Pts',(0.304677723340702,2.20503787696982,13.0687892843774));
#37268=CARTESIAN_POINT('Ctrl Pts',(0.304854334911626,2.20452418465708,13.0687558378483));
#37269=CARTESIAN_POINT('Ctrl Pts',(0.305430864233008,2.20283340060768,13.068645703436));
#37270=CARTESIAN_POINT('Ctrl Pts',(0.305825266099085,2.2016544522028,13.0685688335494));
#37271=CARTESIAN_POINT('Ctrl Pts',(0.306733067795013,2.19888774077777,13.0683882497277));
#37272=CARTESIAN_POINT('Ctrl Pts',(0.307240972822584,2.19729822508886,13.0682843569049));
#37273=CARTESIAN_POINT('Ctrl Pts',(0.310271565259121,2.187553433495,13.0676464781159));
#37274=CARTESIAN_POINT('Ctrl Pts',(0.31248154029603,2.17930518827934,13.0671023839154));
#37275=CARTESIAN_POINT('Ctrl Pts',(0.317526473993992,2.15696167328448,13.0656164428712));
#37276=CARTESIAN_POINT('Ctrl Pts',(0.319750092552013,2.14274921581793,13.0646579277367));
#37277=CARTESIAN_POINT('Ctrl Pts',(0.322992987195578,2.10614126152995,13.0621784741338));
#37278=CARTESIAN_POINT('Ctrl Pts',(0.322640031807941,2.08369904038748,13.0606459833613));
#37279=CARTESIAN_POINT('Ctrl Pts',(0.319536149627843,2.05792118456938,13.0589772314738));
#37280=CARTESIAN_POINT('Ctrl Pts',(0.319049266320506,2.05437603780318,13.0587498865492));
#37281=CARTESIAN_POINT('Ctrl Pts',(0.318415788733078,2.0502718278368,13.0584897628732));
#37282=CARTESIAN_POINT('Ctrl Pts',(0.31832664197396,2.04970432779171,13.0584538633312));
#37283=CARTESIAN_POINT('Ctrl Pts',(0.318191765364524,2.04886044041541,13.058400584733));
#37284=CARTESIAN_POINT('Ctrl Pts',(0.31814719238745,2.04858387336923,13.0583831405327));
#37285=CARTESIAN_POINT('Ctrl Pts',(0.318067965212445,2.04809633113808,13.0583524193016));
#37286=CARTESIAN_POINT('Ctrl Pts',(0.318033461695653,2.04788533240428,13.0583391336911));
#37287=CARTESIAN_POINT('Ctrl Pts',(0.317959877205087,2.04743813713453,13.0583109970614));
#37288=CARTESIAN_POINT('Ctrl Pts',(0.317920743111636,2.047201950411,13.0582961491507));
#37289=CARTESIAN_POINT('Ctrl Pts',(0.317839933054891,2.04671758347836,13.0582657245643));
#37290=CARTESIAN_POINT('Ctrl Pts',(0.317798229495703,2.0464694079506,13.0582501494724));
#37291=CARTESIAN_POINT('Ctrl Pts',(0.317693960495412,2.04585332550601,13.0582115183003));
#37292=CARTESIAN_POINT('Ctrl Pts',(0.317631046428263,2.04548547677745,13.0581884818852));
#37293=CARTESIAN_POINT('Ctrl Pts',(0.317453649135773,2.04445899555445,13.0581242787384));
#37294=CARTESIAN_POINT('Ctrl Pts',(0.317337754528671,2.04380060415333,13.0580831903538));
#37295=CARTESIAN_POINT('Ctrl Pts',(0.316283443627598,2.03791837710243,13.0577168804707));
#37296=CARTESIAN_POINT('Ctrl Pts',(0.315218100570476,2.03271774801417,13.0573985426621));
#37297=CARTESIAN_POINT('Ctrl Pts',(0.312556923473534,2.0211839590057,13.0567001487743));
#37298=CARTESIAN_POINT('Ctrl Pts',(0.310896088541645,2.01486815856367,13.0563228910691));
#37299=CARTESIAN_POINT('Ctrl Pts',(0.300901074344268,1.98107018423994,13.0543113624356));
#37300=CARTESIAN_POINT('Ctrl Pts',(0.289114371763786,1.95474593840934,13.0527584892853));
#37301=CARTESIAN_POINT('Ctrl Pts',(0.268968128504277,1.92221219030782,13.0505295305729));
#37302=CARTESIAN_POINT('Ctrl Pts',(0.263582917995622,1.91432184430516,13.0499625820578));
#37303=CARTESIAN_POINT('Ctrl Pts',(0.25717567109151,1.90577555432751,13.0493130376319));
#37304=CARTESIAN_POINT('Ctrl Pts',(0.256490791181818,1.90487200332691,13.0492439062031));
#37305=CARTESIAN_POINT('Ctrl Pts',(0.255510205231541,1.90359241496058,13.0491453414699));
#37306=CARTESIAN_POINT('Ctrl Pts',(0.255218402321414,1.90321338574209,13.0491160621781));
#37307=CARTESIAN_POINT('Ctrl Pts',(0.254681324888904,1.90251896798081,13.049062265996));
#37308=CARTESIAN_POINT('Ctrl Pts',(0.254436305283572,1.90220338272382,13.0490377592348));
#37309=CARTESIAN_POINT('Ctrl Pts',(0.253938331920387,1.90156444938872,13.0489880236215));
#37310=CARTESIAN_POINT('Ctrl Pts',(0.253685345948721,1.90124112746016,13.0489627935157));
#37311=CARTESIAN_POINT('Ctrl Pts',(0.253060502880787,1.900445699949,13.0489005691146));
#37312=CARTESIAN_POINT('Ctrl Pts',(0.252687942804198,1.89997415081872,13.0488635468015));
#37313=CARTESIAN_POINT('Ctrl Pts',(0.251320872298043,1.8982537647919,13.0487279817749));
#37314=CARTESIAN_POINT('Ctrl Pts',(0.250318417745873,1.89701129621758,13.0486291207624));
#37315=CARTESIAN_POINT('Ctrl Pts',(0.236771416629674,1.88047374417353,13.0473002457689));
#37316=CARTESIAN_POINT('Ctrl Pts',(0.222856206323393,1.86636067777752,13.0460120568462));
#37317=CARTESIAN_POINT('Ctrl Pts',(0.185539591629949,1.83489757100428,13.0427438513796));
#37318=CARTESIAN_POINT('Ctrl Pts',(0.160913873015246,1.81926690872778,13.0407305193064));
#37319=CARTESIAN_POINT('Ctrl Pts',(0.13315434731878,1.80651511377369,13.03879822242));
#37320=CARTESIAN_POINT('Ctrl Pts',(0.131776865250896,1.80589403839773,13.0387031840369));
#37321=CARTESIAN_POINT('Ctrl Pts',(0.130008523928478,1.80511165169672,13.0385823057028));
#37322=CARTESIAN_POINT('Ctrl Pts',(0.129621674802877,1.80494140296332,13.0385559305887));
#37323=CARTESIAN_POINT('Ctrl Pts',(0.129005175166487,1.80467153359935,13.0385140086579));
#37324=CARTESIAN_POINT('Ctrl Pts',(0.128775743263671,1.8045714194019,13.038498431649));
#37325=CARTESIAN_POINT('Ctrl Pts',(0.128350200187613,1.80438632065108,13.0384695853292));
#37326=CARTESIAN_POINT('Ctrl Pts',(0.12815412259156,1.80430126451135,13.0384563116932));
#37327=CARTESIAN_POINT('Ctrl Pts',(0.127714004802703,1.80411086661788,13.0384265575442));
#37328=CARTESIAN_POINT('Ctrl Pts',(0.127469919388127,1.80400563193066,13.0384100836778));
#37329=CARTESIAN_POINT('Ctrl Pts',(0.126960483511842,1.80378674138531,13.0383757575334));
#37330=CARTESIAN_POINT('Ctrl Pts',(0.126695109803024,1.80367313974897,13.0383579085725));
#37331=CARTESIAN_POINT('Ctrl Pts',(0.12600503124198,1.8033788261836,13.0383115765733));
#37332=CARTESIAN_POINT('Ctrl Pts',(0.125580088328562,1.8031986690123,13.0382831269264));
#37333=CARTESIAN_POINT('Ctrl Pts',(0.124327276875871,1.8026707041373,13.0381994865187));
#37334=CARTESIAN_POINT('Ctrl Pts',(0.12349833189717,1.80232543942091,13.0381444453988));
#37335=CARTESIAN_POINT('Ctrl Pts',(0.114453106214344,1.79860229069937,13.0375470115137));
#37336=CARTESIAN_POINT('Ctrl Pts',(0.106101123925351,1.7955617044105,13.037023679848));
#37337=CARTESIAN_POINT('Ctrl Pts',(0.0819762463610353,1.78789266429104,
13.0355630691195));
#37338=CARTESIAN_POINT('Ctrl Pts',(0.0659605269880235,1.78411969386218,
13.0346528875474));
#37339=CARTESIAN_POINT('Ctrl Pts',(0.0385740729033675,1.77984282292276,
13.0331015182396));
#37340=CARTESIAN_POINT('Ctrl Pts',(0.0273386758454484,1.77868838453489,
13.0324666541269));
#37341=CARTESIAN_POINT('Ctrl Pts',(0.0154194326313917,1.77809343549193,
13.0317807120393));
#37342=CARTESIAN_POINT('Ctrl Pts',(0.0147724170681609,1.77806309490285,
13.0317434394454));
#37343=CARTESIAN_POINT('Ctrl Pts',(0.00895827483731269,1.7778080158524,
13.0314081496997));
#37344=CARTESIAN_POINT('Ctrl Pts',(0.00378672053054447,1.77770575192817,
13.0311073823492));
#37345=CARTESIAN_POINT('Ctrl Pts',(-0.00221113729222063,1.77773152619727,
13.0307545336235));
#37346=CARTESIAN_POINT('Ctrl Pts',(-0.00303737053497946,1.7777382543671,
13.0307058388947));
#37347=CARTESIAN_POINT('Ctrl Pts',(-0.0104114484344289,1.777826664162,13.0302704251714));
#37348=CARTESIAN_POINT('Ctrl Pts',(-0.0169550291985275,1.77810471530703,
13.029878256878));
#37349=CARTESIAN_POINT('Ctrl Pts',(-0.0245175380833472,1.77865729007696,
13.0294167650025));
#37350=CARTESIAN_POINT('Ctrl Pts',(-0.0255494286636264,1.77873768731747,
13.0293536178997));
#37351=CARTESIAN_POINT('Ctrl Pts',(-0.0270831415515609,1.77886461883149,
13.0292594917865));
#37352=CARTESIAN_POINT('Ctrl Pts',(-0.0275852779382948,1.77890736222851,
13.0292286319535));
#37353=CARTESIAN_POINT('Ctrl Pts',(-0.0284791133003946,1.77898556042512,
13.0291736220837));
#37354=CARTESIAN_POINT('Ctrl Pts',(-0.0288708523799717,1.7790205548783,
13.029149486569));
#37355=CARTESIAN_POINT('Ctrl Pts',(-0.0296950436186146,1.77909570174745,
13.0290986510387));
#37356=CARTESIAN_POINT('Ctrl Pts',(-0.0301274803351692,1.77913601140329,
13.0290719461219));
#37357=CARTESIAN_POINT('Ctrl Pts',(-0.0312660519308131,1.77924446553055,
13.02900154786));
#37358=CARTESIAN_POINT('Ctrl Pts',(-0.0319720426862349,1.77931406739657,
13.0289578087248));
#37359=CARTESIAN_POINT('Ctrl Pts',(-0.0351342189382954,1.77963636443293,
13.0287615017033));
#37360=CARTESIAN_POINT('Ctrl Pts',(-0.0375876290833089,1.77991494579042,
13.0286081207465));
#37361=CARTESIAN_POINT('Ctrl Pts',(-0.055561697716967,1.78216537209679,
13.0274762778186));
#37362=CARTESIAN_POINT('Ctrl Pts',(-0.070921326847603,1.78523661447709,
13.0264628455106));
#37363=CARTESIAN_POINT('Ctrl Pts',(-0.0995741890199547,1.79316995814285,
13.0244873830651));
#37364=CARTESIAN_POINT('Ctrl Pts',(-0.112891171137942,1.79781588693697,
13.0235326116357));
#37365=CARTESIAN_POINT('Ctrl Pts',(-0.139325694513887,1.80903013221806,
13.021590467278));
#37366=CARTESIAN_POINT('Ctrl Pts',(-0.152387464847363,1.81565294516366,
13.0206055100016));
#37367=CARTESIAN_POINT('Ctrl Pts',(-0.168832614573602,1.82545110249935,
13.0193676139911));
#37368=CARTESIAN_POINT('Ctrl Pts',(-0.172661495499823,1.8278427623984,13.0190796351122));
#37369=CARTESIAN_POINT('Ctrl Pts',(-0.176953441869582,1.83065072337242,
13.0187582110946));
#37370=CARTESIAN_POINT('Ctrl Pts',(-0.177466826844408,1.83098870136393,
13.0187197866268));
#37371=CARTESIAN_POINT('Ctrl Pts',(-0.178216765169868,1.83148549125072,
13.0186636946089));
#37372=CARTESIAN_POINT('Ctrl Pts',(-0.178454075929436,1.83164314880713,
13.0186459503258));
#37373=CARTESIAN_POINT('Ctrl Pts',(-0.17887009584438,1.831920327777,13.0186148536351));
#37374=CARTESIAN_POINT('Ctrl Pts',(-0.179048894663105,1.8320397134507,13.0186014920557));
#37375=CARTESIAN_POINT('Ctrl Pts',(-0.179422552713927,1.83228974946524,
13.0185735757498));
#37376=CARTESIAN_POINT('Ctrl Pts',(-0.179617388360722,1.83242043339769,
13.0185590233876));
#37377=CARTESIAN_POINT('Ctrl Pts',(-0.180015156777663,1.8326878625357,13.0185293216267));
#37378=CARTESIAN_POINT('Ctrl Pts',(-0.18021807690784,1.83282462639305,13.0185141735055));
#37379=CARTESIAN_POINT('Ctrl Pts',(-0.180716181781151,1.83316116416408,
13.0184769992732));
#37380=CARTESIAN_POINT('Ctrl Pts',(-0.181011192113998,1.83336119749714,
13.0184549905759));
#37381=CARTESIAN_POINT('Ctrl Pts',(-0.181823879645668,1.83391421496085,
13.0183943827026));
#37382=CARTESIAN_POINT('Ctrl Pts',(-0.182340863583443,1.8342682222764,13.0183558512888));
#37383=CARTESIAN_POINT('Ctrl Pts',(-0.183979226213123,1.83539713174827,
13.0182338065228));
#37384=CARTESIAN_POINT('Ctrl Pts',(-0.185096740101167,1.83617765349205,
13.0181506568005));
#37385=CARTESIAN_POINT('Ctrl Pts',(-0.209487237327741,1.85344433520756,
13.0163371731466));
#37386=CARTESIAN_POINT('Ctrl Pts',(-0.230478768121008,1.87294337030669,
13.0147946684863));
#37387=CARTESIAN_POINT('Ctrl Pts',(-0.261393140611049,1.91042908455911,
13.0120590819876));
#37388=CARTESIAN_POINT('Ctrl Pts',(-0.272680515351522,1.92705879364602,
13.0109057066521));
#37389=CARTESIAN_POINT('Ctrl Pts',(-0.282973628979109,1.94576387642268,
13.0096089577418));
#37390=CARTESIAN_POINT('Ctrl Pts',(-0.28359181294541,1.94690349426797,13.0095299713568));
#37391=CARTESIAN_POINT('Ctrl Pts',(-0.284444155350767,1.94849765844747,
13.0094194955218));
#37392=CARTESIAN_POINT('Ctrl Pts',(-0.284684139749583,1.94894908944532,
13.0093882129521));
#37393=CARTESIAN_POINT('Ctrl Pts',(-0.285096616000628,1.94972946686435,
13.0093341376605));
#37394=CARTESIAN_POINT('Ctrl Pts',(-0.285269615754226,1.95005814490462,
13.0093113629625));
#37395=CARTESIAN_POINT('Ctrl Pts',(-0.285626434377593,1.95073890874086,
13.009264192583));
#37396=CARTESIAN_POINT('Ctrl Pts',(-0.285810171270957,1.95109103661971,
13.0092397940537));
#37397=CARTESIAN_POINT('Ctrl Pts',(-0.286237941058301,1.95191455680242,
13.0091827341107));
#37398=CARTESIAN_POINT('Ctrl Pts',(-0.286481460661861,1.95238621311006,
13.0091500546756));
#37399=CARTESIAN_POINT('Ctrl Pts',(-0.287260284378128,1.95390384922752,
13.0090449034622));
#37400=CARTESIAN_POINT('Ctrl Pts',(-0.287791029086278,1.95495214661916,
13.0089722717302));
#37401=CARTESIAN_POINT('Ctrl Pts',(-0.296028904342663,1.97144635541009,
13.0078294069265));
#37402=CARTESIAN_POINT('Ctrl Pts',(-0.302487259792097,1.98748141111869,
13.006715226017));
#37403=CARTESIAN_POINT('Ctrl Pts',(-0.311719902453299,2.01705310471501,
13.0046572594936));
#37404=CARTESIAN_POINT('Ctrl Pts',(-0.314968563061163,2.03039933803388,
13.0037279718904));
#37405=CARTESIAN_POINT('Ctrl Pts',(-0.32062983445731,2.0624314153751,13.0015273956094));
#37406=CARTESIAN_POINT('Ctrl Pts',(-0.322275899729781,2.08120454186863,
13.0002603718331));
#37407=CARTESIAN_POINT('Ctrl Pts',(-0.322274999631057,2.10001542082731,
12.9990742422863));
#37408=CARTESIAN_POINT('',(-0.322274868779446,2.0997091767017,12.8743773449311));
#37409=CARTESIAN_POINT('Ctrl Pts',(-0.322274868779446,2.0997091767017,12.8743773449311));
#37410=CARTESIAN_POINT('Ctrl Pts',(-0.32225477015569,2.07743695377,12.8757506912526));
#37411=CARTESIAN_POINT('Ctrl Pts',(-0.319921917552464,2.05526885992465,
12.8771240375741));
#37412=CARTESIAN_POINT('Ctrl Pts',(-0.315363309840923,2.03361356741639,
12.8784973838957));
#37413=CARTESIAN_POINT('Ctrl Pts',(-0.313909026430378,2.02670511320448,
12.8789355077481));
#37414=CARTESIAN_POINT('Ctrl Pts',(-0.312228581490867,2.01984867270576,
12.8793736316006));
#37415=CARTESIAN_POINT('Ctrl Pts',(-0.310325794918933,2.01305704955011,
12.879811755453));
#37416=CARTESIAN_POINT('Ctrl Pts',(-0.305560360746364,1.99604776771548,
12.8809090148141));
#37417=CARTESIAN_POINT('Ctrl Pts',(-0.299377391867214,1.97937816504062,
12.8820062741752));
#37418=CARTESIAN_POINT('Ctrl Pts',(-0.291845741122565,1.96329872343822,
12.8831035335364));
#37419=CARTESIAN_POINT('Ctrl Pts',(-0.284328498231357,1.94725004139251,
12.8841986938686));
#37420=CARTESIAN_POINT('Ctrl Pts',(-0.275467960777509,1.93178999933012,
12.8852938542009));
#37421=CARTESIAN_POINT('Ctrl Pts',(-0.265381773584942,1.917151183012,12.8863890145332));
#37422=CARTESIAN_POINT('Ctrl Pts',(-0.255179573497405,1.90234398875011,
12.8874967715701));
#37423=CARTESIAN_POINT('Ctrl Pts',(-0.243723683465363,1.88837777039137,
12.888604528607));
#37424=CARTESIAN_POINT('Ctrl Pts',(-0.231182240909558,1.87546504255899,
12.8897122856439));
#37425=CARTESIAN_POINT('Ctrl Pts',(-0.218789416356174,1.86270533251606,
12.8908069155913));
#37426=CARTESIAN_POINT('Ctrl Pts',(-0.205337238028378,1.85097478606144,
12.8919015455388));
#37427=CARTESIAN_POINT('Ctrl Pts',(-0.191025630177961,1.84044194437446,
12.8929961754862));
#37428=CARTESIAN_POINT('Ctrl Pts',(-0.176456579495077,1.82971963378739,
12.8941104960678));
#37429=CARTESIAN_POINT('Ctrl Pts',(-0.160997509866063,1.82023907717878,
12.8952248166494));
#37430=CARTESIAN_POINT('Ctrl Pts',(-0.144889561086191,1.81213164343184,
12.896339137231));
#37431=CARTESIAN_POINT('Ctrl Pts',(-0.128781612306314,1.80402420968491,
12.8974534578126));
#37432=CARTESIAN_POINT('Ctrl Pts',(-0.112025581744362,1.79729015799452,
12.8985677783942));
#37433=CARTESIAN_POINT('Ctrl Pts',(-0.0948817706989104,1.79200872542548,
12.8996820989758));
#37434=CARTESIAN_POINT('Ctrl Pts',(-0.0780004465863533,1.78680815626729,
12.9007793583222));
#37435=CARTESIAN_POINT('Ctrl Pts',(-0.0606373936470627,1.7829833500994,
12.9018766176687));
#37436=CARTESIAN_POINT('Ctrl Pts',(-0.0430404928385636,1.78061200460691,
12.9029738770151));
#37437=CARTESIAN_POINT('Ctrl Pts',(-0.0254772544471081,1.77824519543715,
12.9040690373328));
#37438=CARTESIAN_POINT('Ctrl Pts',(-0.00768180547187218,1.7773264938092,
12.9051641976504));
#37439=CARTESIAN_POINT('Ctrl Pts',(0.0100866085518973,1.77788288472526,
12.906259357968));
#37440=CARTESIAN_POINT('Ctrl Pts',(0.0280593979987197,1.77844567534749,
12.9073671150122));
#37441=CARTESIAN_POINT('Ctrl Pts',(0.0460037248759171,1.7805178263984,12.9084748720565));
#37442=CARTESIAN_POINT('Ctrl Pts',(0.0636498872489975,1.78407300292917,
12.9095826291007));
#37443=CARTESIAN_POINT('Ctrl Pts',(0.0810869395700782,1.78758605000803,
12.9106772590338));
#37444=CARTESIAN_POINT('Ctrl Pts',(0.0982321000672225,1.79254692552035,
12.911771888967));
#37445=CARTESIAN_POINT('Ctrl Pts',(0.114835433694952,1.79887876396193,12.9128665189002));
#37446=CARTESIAN_POINT('Ctrl Pts',(0.131737435115925,1.80532450219358,12.9139808394999));
#37447=CARTESIAN_POINT('Ctrl Pts',(0.14807713087735,1.81319076820556,12.9150951600996));
#37448=CARTESIAN_POINT('Ctrl Pts',(0.163613530327581,1.82234591967928,12.9162094806994));
#37449=CARTESIAN_POINT('Ctrl Pts',(0.179149929777806,1.83150107115299,12.9173238012991));
#37450=CARTESIAN_POINT('Ctrl Pts',(0.193882383350925,1.84194457795324,12.9184381218989));
#37451=CARTESIAN_POINT('Ctrl Pts',(0.207603361298644,1.8535004665268,12.9195524424986));
#37452=CARTESIAN_POINT('Ctrl Pts',(0.22111425879022,1.86487942410084,12.9206497018524));
#37453=CARTESIAN_POINT('Ctrl Pts',(0.233729158635664,1.87740815327334,12.9217469612061));
#37454=CARTESIAN_POINT('Ctrl Pts',(0.245248548787146,1.89092029045649,12.9228442205599));
#37455=CARTESIAN_POINT('Ctrl Pts',(0.256745902640785,1.90440657926784,12.9239393808846));
#37456=CARTESIAN_POINT('Ctrl Pts',(0.26715136151924,1.91887200168266,12.9250345412094));
#37457=CARTESIAN_POINT('Ctrl Pts',(0.276301901655129,1.93411318688106,12.9261297015342));
#37458=CARTESIAN_POINT('Ctrl Pts',(0.285557692822547,1.94952967872147,12.9272374585748));
#37459=CARTESIAN_POINT('Ctrl Pts',(0.293528979425782,1.96573928278836,12.9283452156154));
#37460=CARTESIAN_POINT('Ctrl Pts',(0.3000919098322,1.98250097328802,12.929452972656));
#37461=CARTESIAN_POINT('Ctrl Pts',(0.306577068447082,1.99906403503214,12.9305476025957));
#37462=CARTESIAN_POINT('Ctrl Pts',(0.311686860661269,2.01616540460373,12.9316422325354));
#37463=CARTESIAN_POINT('Ctrl Pts',(0.31535062200815,2.03355332345352,12.9327368624751));
#37464=CARTESIAN_POINT('Ctrl Pts',(0.319080288593584,2.05125402330382,12.9338511830661));
#37465=CARTESIAN_POINT('Ctrl Pts',(0.321311163799205,2.06925088384046,12.9349655036572));
#37466=CARTESIAN_POINT('Ctrl Pts',(0.322023482246868,2.08727001545166,12.9360798242482));
#37467=CARTESIAN_POINT('Ctrl Pts',(0.322735800694531,2.10528914706285,12.9371941448393));
#37468=CARTESIAN_POINT('Ctrl Pts',(0.321929656509605,2.12332971661026,12.9383084654303));
#37469=CARTESIAN_POINT('Ctrl Pts',(0.319640671798446,2.14112197170903,12.9394227860214));
#37470=CARTESIAN_POINT('Ctrl Pts',(0.317386733394382,2.15864181221583,12.9405200454143));
#37471=CARTESIAN_POINT('Ctrl Pts',(0.313681026625055,2.17603067396092,12.9416173048073));
#37472=CARTESIAN_POINT('Ctrl Pts',(0.308555433511349,2.19303074801174,12.9427145642002));
#37473=CARTESIAN_POINT('Ctrl Pts',(0.303439645524016,2.20999830136286,12.9438097245645));
#37474=CARTESIAN_POINT('Ctrl Pts',(0.296909521902379,2.22657779252613,12.9449048849287));
#37475=CARTESIAN_POINT('Ctrl Pts',(0.28904781277566,2.24252205988761,12.946000045293));
#37476=CARTESIAN_POINT('Ctrl Pts',(0.281095677393468,2.25864971999111,12.9471078023139));
#37477=CARTESIAN_POINT('Ctrl Pts',(0.271781353589384,2.27412667164002,12.9482155593348));
#37478=CARTESIAN_POINT('Ctrl Pts',(0.261240457029716,2.28871830657333,12.9493233163558));
#37479=CARTESIAN_POINT('Ctrl Pts',(0.250824471247107,2.30313702903684,12.9504179463349));
#37480=CARTESIAN_POINT('Ctrl Pts',(0.23921135584914,2.31669071449423,12.9515125763139));
#37481=CARTESIAN_POINT('Ctrl Pts',(0.226574541989169,2.32918366553356,12.952607206293));
#37482=CARTESIAN_POINT('Ctrl Pts',(0.213710412980391,2.34190134387014,12.9537215268349));
#37483=CARTESIAN_POINT('Ctrl Pts',(0.199785944014845,2.35351912880811,12.9548358473767));
#37484=CARTESIAN_POINT('Ctrl Pts',(0.185020726982867,2.36387213989304,12.9559501679186));
#37485=CARTESIAN_POINT('Ctrl Pts',(0.170255509950889,2.37422515097797,12.9570644884605));
#37486=CARTESIAN_POINT('Ctrl Pts',(0.154650296321501,2.38331301635944,12.9581788090023));
#37487=CARTESIAN_POINT('Ctrl Pts',(0.138451181570716,2.39101966591052,12.9592931295442));
#37488=CARTESIAN_POINT('Ctrl Pts',(0.122500089953329,2.39860831966992,12.9603903888283));
#37489=CARTESIAN_POINT('Ctrl Pts',(0.105873259244491,2.40490539970148,12.9614876481124));
#37490=CARTESIAN_POINT('Ctrl Pts',(0.0888047180756005,2.40979815634137,
12.9625849073965));
#37491=CARTESIAN_POINT('Ctrl Pts',(0.0717688285844593,2.41468155326437,
12.9636800676519));
#37492=CARTESIAN_POINT('Ctrl Pts',(0.054293623314285,2.41816568666105,12.9647752279074));
#37493=CARTESIAN_POINT('Ctrl Pts',(0.0366317142711716,2.42018634126795,
12.9658703881629));
#37494=CARTESIAN_POINT('Ctrl Pts',(0.0187666533278381,2.42223023797298,
12.9669781452382));
#37495=CARTESIAN_POINT('Ctrl Pts',(0.000711342416110285,2.42277654184563,
12.9680859023136));
#37496=CARTESIAN_POINT('Ctrl Pts',(-0.0172635443498445,2.42181228326694,
12.9691936593889));
#37497=CARTESIAN_POINT('Ctrl Pts',(-0.0350254241429703,2.42085945139728,
12.9702882892616));
#37498=CARTESIAN_POINT('Ctrl Pts',(-0.0527079932519415,2.41843179160619,
12.9713829191343));
#37499=CARTESIAN_POINT('Ctrl Pts',(-0.0700528244136611,2.41456919336875,
12.972477549007));
#37500=CARTESIAN_POINT('Ctrl Pts',(-0.0877096639345393,2.41063711259056,
12.9735918696836));
#37501=CARTESIAN_POINT('Ctrl Pts',(-0.105015674487834,2.4052180864362,12.9747061903603));
#37502=CARTESIAN_POINT('Ctrl Pts',(-0.121713352459767,2.3984074989976,12.975820511037));
#37503=CARTESIAN_POINT('Ctrl Pts',(-0.138411030431706,2.391596911559,12.9769348317137));
#37504=CARTESIAN_POINT('Ctrl Pts',(-0.154499656379204,2.38339519339613,
12.9780491523903));
#37505=CARTESIAN_POINT('Ctrl Pts',(-0.169748420447812,2.37394643523958,
12.979163473067));
#37506=CARTESIAN_POINT('Ctrl Pts',(-0.184763711413957,2.36464234657043,
12.9802607324327));
#37507=CARTESIAN_POINT('Ctrl Pts',(-0.19905881373056,2.35407093203492,12.9813579917984));
#37508=CARTESIAN_POINT('Ctrl Pts',(-0.2124122415145,2.34236793368716,12.9824552511641));
#37509=CARTESIAN_POINT('Ctrl Pts',(-0.225740124523122,2.33068732288426,
12.9835504115));
#37510=CARTESIAN_POINT('Ctrl Pts',(-0.238129291142844,2.31787988075899,
12.9846455718358));
#37511=CARTESIAN_POINT('Ctrl Pts',(-0.249389004567557,2.30412324714692,
12.9857407321716));
#37512=CARTESIAN_POINT('Ctrl Pts',(-0.260778228910836,2.29020838266447,
12.9868484892065));
#37513=CARTESIAN_POINT('Ctrl Pts',(-0.271011236232546,2.2753228786545,12.9879562462413));
#37514=CARTESIAN_POINT('Ctrl Pts',(-0.279930600684152,2.25968730201744,
12.9890640032762));
#37515=CARTESIAN_POINT('Ctrl Pts',(-0.288744269334159,2.2442370093,12.9901586332246));
#37516=CARTESIAN_POINT('Ctrl Pts',(-0.296274943808381,2.22805505132666,
12.9912532631731));
#37517=CARTESIAN_POINT('Ctrl Pts',(-0.302416272518608,2.21138031128054,
12.9923478931215));
#37518=CARTESIAN_POINT('Ctrl Pts',(-0.308668073840186,2.19440561951984,
12.9934622136996));
#37519=CARTESIAN_POINT('Ctrl Pts',(-0.313479715083512,2.17692100071793,
12.9945765342776));
#37520=CARTESIAN_POINT('Ctrl Pts',(-0.31679200553615,2.15919460155609,12.9956908548557));
#37521=CARTESIAN_POINT('Ctrl Pts',(-0.320104295988786,2.14146820239425,
12.9968051754337));
#37522=CARTESIAN_POINT('Ctrl Pts',(-0.321917208225557,2.12350086086223,
12.9979194960118));
#37523=CARTESIAN_POINT('Ctrl Pts',(-0.322226954727219,2.10556464484248,
12.9990338165898));
#37524=CARTESIAN_POINT('Ctrl Pts',(-0.32225878479565,2.10372148929352,12.9991483260357));
#37525=CARTESIAN_POINT('Ctrl Pts',(-0.322274800607892,2.10187805985517,
12.9992628354815));
#37526=CARTESIAN_POINT('Ctrl Pts',(-0.32227499814981,2.10003453317044,12.9993773449273));
#37527=CARTESIAN_POINT('',(-0.322555864543089,2.10024316196973,12.6243773449273));
#37528=CARTESIAN_POINT('Ctrl Pts',(-0.322274872504986,2.09971333487317,
12.8744514725916));
#37529=CARTESIAN_POINT('Ctrl Pts',(-0.322294798337445,2.12211436839394,
12.8731948915496));
#37530=CARTESIAN_POINT('Ctrl Pts',(-0.319979252500182,2.14445352842172,
12.8719154443998));
#37531=CARTESIAN_POINT('Ctrl Pts',(-0.315200854949327,2.16715834777632,
12.8705046719139));
#37532=CARTESIAN_POINT('Ctrl Pts',(-0.315032253003373,2.16794484664868,
12.870455670392));
#37533=CARTESIAN_POINT('Ctrl Pts',(-0.314752217117301,2.16922771292375,
12.8703755245491));
#37534=CARTESIAN_POINT('Ctrl Pts',(-0.314642548503174,2.16972446545997,
12.8703444367166));
#37535=CARTESIAN_POINT('Ctrl Pts',(-0.314447146601967,2.17059970411111,
12.8702895669105));
#37536=CARTESIAN_POINT('Ctrl Pts',(-0.314361904779475,2.17097829983898,
12.870265800726));
#37537=CARTESIAN_POINT('Ctrl Pts',(-0.314188225474058,2.17174323436838,
12.8702177181107));
#37538=CARTESIAN_POINT('Ctrl Pts',(-0.314099758743251,2.17212956577808,
12.8701934007776));
#37539=CARTESIAN_POINT('Ctrl Pts',(-0.313926666095136,2.17287909862558,
12.8701461572907));
#37540=CARTESIAN_POINT('Ctrl Pts',(-0.313842121908859,2.17324231847787,
12.8701232337988));
#37541=CARTESIAN_POINT('Ctrl Pts',(-0.313638876291029,2.17410869151184,
12.8700684844704));
#37542=CARTESIAN_POINT('Ctrl Pts',(-0.313519594545015,2.17461170625347,
12.8700366399912));
#37543=CARTESIAN_POINT('Ctrl Pts',(-0.313088972824143,2.17640838449785,
12.8699226915661));
#37544=CARTESIAN_POINT('Ctrl Pts',(-0.312770835197441,2.17770039054188,
12.8698403687799));
#37545=CARTESIAN_POINT('Ctrl Pts',(-0.307111492576687,2.2000857973967,12.8684072984508));
#37546=CARTESIAN_POINT('Ctrl Pts',(-0.299656721557315,2.2205825125988,12.8669852048862));
#37547=CARTESIAN_POINT('Ctrl Pts',(-0.287724429957582,2.24528636866053,
12.8651420378203));
#37548=CARTESIAN_POINT('Ctrl Pts',(-0.285117622275454,2.25033767293752,
12.8647582171332));
#37549=CARTESIAN_POINT('Ctrl Pts',(-0.279787039351144,2.26002907664861,
12.8640100273077));
#37550=CARTESIAN_POINT('Ctrl Pts',(-0.277077891269175,2.26467524177196,
12.8636458371482));
#37551=CARTESIAN_POINT('Ctrl Pts',(-0.266632672176858,2.28160059456275,
12.862302458274));
#37552=CARTESIAN_POINT('Ctrl Pts',(-0.258185362980705,2.29342224180021,
12.8613301513551));
#37553=CARTESIAN_POINT('Ctrl Pts',(-0.24697580343239,2.30706033594075,12.8601994571681));
#37554=CARTESIAN_POINT('Ctrl Pts',(-0.24494708254618,2.30945634095366,12.8600004798228));
#37555=CARTESIAN_POINT('Ctrl Pts',(-0.24254565442415,2.31220990901419,12.8597718040688));
#37556=CARTESIAN_POINT('Ctrl Pts',(-0.242206795593599,2.31259658544019,
12.8597396916465));
#37557=CARTESIAN_POINT('Ctrl Pts',(-0.24169004535362,2.31318341705031,12.8596909590196));
#37558=CARTESIAN_POINT('Ctrl Pts',(-0.24151282944834,2.31338416188037,12.8596742888225));
#37559=CARTESIAN_POINT('Ctrl Pts',(-0.24119091964426,2.31374789684954,12.8596440847185));
#37560=CARTESIAN_POINT('Ctrl Pts',(-0.24104631111361,2.31391096050881,12.859630544534));
#37561=CARTESIAN_POINT('Ctrl Pts',(-0.240754565061393,2.31423926806511,
12.859603283995));
#37562=CARTESIAN_POINT('Ctrl Pts',(-0.240607423445389,2.31440450639542,
12.8595895640782));
#37563=CARTESIAN_POINT('Ctrl Pts',(-0.240184933232937,2.31487797536065,
12.85955025216));
#37564=CARTESIAN_POINT('Ctrl Pts',(-0.239909160424916,2.31518582944966,
12.8595246920494));
#37565=CARTESIAN_POINT('Ctrl Pts',(-0.238708080539584,2.3165214548443,12.8594137988775));
#37566=CARTESIAN_POINT('Ctrl Pts',(-0.237776737929243,2.3175438144005,12.8593289137375));
#37567=CARTESIAN_POINT('Ctrl Pts',(-0.220167182346014,2.33662609483042,
12.8577437933958));
#37568=CARTESIAN_POINT('Ctrl Pts',(-0.201480136395958,2.3527284638963,12.8563897808667));
#37569=CARTESIAN_POINT('Ctrl Pts',(-0.17388286426215,2.37148283091152,12.8545233038542));
#37570=CARTESIAN_POINT('Ctrl Pts',(-0.166426831463961,2.37611642503389,
12.8540310146772));
#37571=CARTESIAN_POINT('Ctrl Pts',(-0.149192108432061,2.38587510396397,
12.8529044601625));
#37572=CARTESIAN_POINT('Ctrl Pts',(-0.139321065774814,2.39081345803224,
12.8522668597802));
#37573=CARTESIAN_POINT('Ctrl Pts',(-0.125872574071606,2.39669950746404,
12.8513954682407));
#37574=CARTESIAN_POINT('Ctrl Pts',(-0.122503724504924,2.39810625372167,
12.8511770017648));
#37575=CARTESIAN_POINT('Ctrl Pts',(-0.116980424016449,2.40030320932826,
12.8508181425325));
#37576=CARTESIAN_POINT('Ctrl Pts',(-0.114840098055629,2.4011281929577,12.8506789191371));
#37577=CARTESIAN_POINT('Ctrl Pts',(-0.112210384543954,2.40210969630715,
12.8505076064953));
#37578=CARTESIAN_POINT('Ctrl Pts',(-0.111729153557894,2.40228800049416,
12.8504762463275));
#37579=CARTESIAN_POINT('Ctrl Pts',(-0.110881791546671,2.40259966253182,
12.8504210075836));
#37580=CARTESIAN_POINT('Ctrl Pts',(-0.110515839819288,2.40273350757374,
12.8503971452843));
#37581=CARTESIAN_POINT('Ctrl Pts',(-0.109776402774381,2.40300243358327,
12.8503489164489));
#37582=CARTESIAN_POINT('Ctrl Pts',(-0.109402908753309,2.40313748847263,
12.8503245490949));
#37583=CARTESIAN_POINT('Ctrl Pts',(-0.108679610914486,2.4033975210493,12.850277346658));
#37584=CARTESIAN_POINT('Ctrl Pts',(-0.10832983860777,2.40352258511156,12.8502545144928));
#37585=CARTESIAN_POINT('Ctrl Pts',(-0.10749803075371,2.4038183841019,12.8502002017231));
#37586=CARTESIAN_POINT('Ctrl Pts',(-0.107015804611268,2.40398857658275,
12.8501687031532));
#37587=CARTESIAN_POINT('Ctrl Pts',(-0.105308886907108,2.40458643557149,
12.8500571661655));
#37588=CARTESIAN_POINT('Ctrl Pts',(-0.104082032870247,2.40500785030952,
12.8499769208359));
#37589=CARTESIAN_POINT('Ctrl Pts',(-0.0836837798919911,2.41187708736274,
12.8486413420139));
#37590=CARTESIAN_POINT('Ctrl Pts',(-0.063953534988268,2.41651217980907,
12.8473248596033));
#37591=CARTESIAN_POINT('Ctrl Pts',(-0.0259853823046345,2.4217355477075,
12.8447582876782));
#37592=CARTESIAN_POINT('Ctrl Pts',(-0.00787289940778402,2.42268715141514,
12.8435211252291));
#37593=CARTESIAN_POINT('Ctrl Pts',(0.0193635842491699,2.4218227074341,12.841700225228));
#37594=CARTESIAN_POINT('Ctrl Pts',(0.0284881730753215,2.42114367072974,
12.841097395038));
#37595=CARTESIAN_POINT('Ctrl Pts',(0.0406020883521112,2.41972167962587,
12.8403166783615));
#37596=CARTESIAN_POINT('Ctrl Pts',(0.0436268559760407,2.41932300434967,
12.8401233918411));
#37597=CARTESIAN_POINT('Ctrl Pts',(0.0471505928940003,2.41880755582274,
12.8399005101506));
#37598=CARTESIAN_POINT('Ctrl Pts',(0.0476553753261181,2.4187324917089,12.8398686369114));
#37599=CARTESIAN_POINT('Ctrl Pts',(0.0484239556834199,2.41861633262442,
12.8398201928404));
#37600=CARTESIAN_POINT('Ctrl Pts',(0.0486878814064416,2.4185761088099,12.8398035729111));
#37601=CARTESIAN_POINT('Ctrl Pts',(0.0491463023560506,2.41850565981011,
12.8397747324617));
#37602=CARTESIAN_POINT('Ctrl Pts',(0.0493408194042368,2.41847558447639,
12.8397625034295));
#37603=CARTESIAN_POINT('Ctrl Pts',(0.0497486927689843,2.41841213831531,
12.8397368789214));
#37604=CARTESIAN_POINT('Ctrl Pts',(0.0499620424284265,2.41837873134961,
12.8397234855741));
#37605=CARTESIAN_POINT('Ctrl Pts',(0.0505576321794122,2.41828485860364,
12.8396861248128));
#37606=CARTESIAN_POINT('Ctrl Pts',(0.0509397988042087,2.41822391847477,
12.8396621844141));
#37607=CARTESIAN_POINT('Ctrl Pts',(0.0524778680162669,2.41797581688993,
12.8395659614733));
#37608=CARTESIAN_POINT('Ctrl Pts',(0.0536328748788254,2.41778304169577,
12.8394939936818));
#37609=CARTESIAN_POINT('Ctrl Pts',(0.07415216161304,2.41424323272159,12.8382202074648));
#37610=CARTESIAN_POINT('Ctrl Pts',(0.0931746927149973,2.40913763883687,
12.8371134851007));
#37611=CARTESIAN_POINT('Ctrl Pts',(0.122599371135456,2.3982744552928,12.8353578368062));
#37612=CARTESIAN_POINT('Ctrl Pts',(0.133353684710301,2.39362398612088,12.8347063708794));
#37613=CARTESIAN_POINT('Ctrl Pts',(0.155540500420522,2.38255892655562,12.8333047490035));
#37614=CARTESIAN_POINT('Ctrl Pts',(0.166882479261162,2.37601192186967,12.8325531344663));
#37615=CARTESIAN_POINT('Ctrl Pts',(0.182574784628207,2.36563221398936,12.8314373372663));
#37616=CARTESIAN_POINT('Ctrl Pts',(0.18726965939977,2.36234346468265,12.8310930913317));
#37617=CARTESIAN_POINT('Ctrl Pts',(0.192611641789871,2.35838493309092,12.8306880940477));
#37618=CARTESIAN_POINT('Ctrl Pts',(0.193346798810902,2.35783528378327,12.8306320595801));
#37619=CARTESIAN_POINT('Ctrl Pts',(0.194391635989917,2.35704711681272,12.8305519890433));
#37620=CARTESIAN_POINT('Ctrl Pts',(0.194703250722833,2.35681116128472,12.8305280535126));
#37621=CARTESIAN_POINT('Ctrl Pts',(0.195331146289716,2.35633391731906,12.8304797123047));
#37622=CARTESIAN_POINT('Ctrl Pts',(0.195647411114207,2.35609260903237,12.8304553058722));
#37623=CARTESIAN_POINT('Ctrl Pts',(0.196257294313261,2.35562548241471,12.8304081291823));
#37624=CARTESIAN_POINT('Ctrl Pts',(0.196550971917827,2.35539974210498,12.8303853620308));
#37625=CARTESIAN_POINT('Ctrl Pts',(0.197245982518356,2.35486360160357,12.830331362526));
#37626=CARTESIAN_POINT('Ctrl Pts',(0.197646972082191,2.35455275968651,12.8303001126906));
#37627=CARTESIAN_POINT('Ctrl Pts',(0.199051955638438,2.35345831338486,12.8301902858797));
#37628=CARTESIAN_POINT('Ctrl Pts',(0.200052027068166,2.3526697133782,12.8301115102332));
#37629=CARTESIAN_POINT('Ctrl Pts',(0.214377880965699,2.3412347832568,12.8289742993041));
#37630=CARTESIAN_POINT('Ctrl Pts',(0.226840364854264,2.32955473259397,12.8278730427438));
#37631=CARTESIAN_POINT('Ctrl Pts',(0.253516605080675,2.30025035121218,12.825240734852));
#37632=CARTESIAN_POINT('Ctrl Pts',(0.266916867367605,2.28200594613907,12.82369097945));
#37633=CARTESIAN_POINT('Ctrl Pts',(0.282141150478601,2.25593447543346,12.8216815462283));
#37634=CARTESIAN_POINT('Ctrl Pts',(0.285747900495652,2.24922246768539,12.8211811816926));
#37635=CARTESIAN_POINT('Ctrl Pts',(0.290568133186489,2.23943519259995,12.8204816332445));
#37636=CARTESIAN_POINT('Ctrl Pts',(0.291977353175279,2.23645966536536,12.8202728153829));
#37637=CARTESIAN_POINT('Ctrl Pts',(0.293558289813493,2.23298489360371,12.8200338469683));
#37638=CARTESIAN_POINT('Ctrl Pts',(0.293774616617726,2.23250632469958,12.8200010411197));
#37639=CARTESIAN_POINT('Ctrl Pts',(0.294100421651276,2.23178084290423,12.81995147289));
#37640=CARTESIAN_POINT('Ctrl Pts',(0.29421075961816,2.23153432060948,12.8199346578796));
#37641=CARTESIAN_POINT('Ctrl Pts',(0.294401110194699,2.23110759252099,12.8199056009178));
#37642=CARTESIAN_POINT('Ctrl Pts',(0.29448126720316,2.23092745230739,12.8198933500404));
#37643=CARTESIAN_POINT('Ctrl Pts',(0.294648231685222,2.23055129699269,12.8198678006857));
#37644=CARTESIAN_POINT('Ctrl Pts',(0.294735008631728,2.23035526943408,12.8198545041202));
#37645=CARTESIAN_POINT('Ctrl Pts',(0.294947952123556,2.22987293425737,12.8198218314042));
#37646=CARTESIAN_POINT('Ctrl Pts',(0.295073897776521,2.22958652849506,12.819802468867));
#37647=CARTESIAN_POINT('Ctrl Pts',(0.295561422485904,2.22847348067334,12.8197273675001));
#37648=CARTESIAN_POINT('Ctrl Pts',(0.295919950993991,2.22764549481936,12.81967181384));
#37649=CARTESIAN_POINT('Ctrl Pts',(0.302546739078168,2.21216360281485,12.8186387015698));
#37650=CARTESIAN_POINT('Ctrl Pts',(0.307723861557192,2.19706379715061,12.8177248300039));
#37651=CARTESIAN_POINT('Ctrl Pts',(0.316212620434076,2.1646476848214,12.8158363005609));
#37652=CARTESIAN_POINT('Ctrl Pts',(0.319265758241281,2.14731938135108,12.8148671895422));
#37653=CARTESIAN_POINT('Ctrl Pts',(0.322281284058626,2.11487875086428,12.8130164791697));
#37654=CARTESIAN_POINT('Ctrl Pts',(0.322624385960057,2.09985196986792,12.8121451498433));
#37655=CARTESIAN_POINT('Ctrl Pts',(0.321844346021484,2.08326919318544,12.8111435318882));
#37656=CARTESIAN_POINT('Ctrl Pts',(0.321757899432826,2.08168178567307,12.8110472575976));
#37657=CARTESIAN_POINT('Ctrl Pts',(0.321586465717361,2.07891144613579,12.8108785248203));
#37658=CARTESIAN_POINT('Ctrl Pts',(0.32150668659176,2.07772821393267,12.8108062298208));
#37659=CARTESIAN_POINT('Ctrl Pts',(0.321381679545725,2.07601512067632,12.8107012214256));
#37660=CARTESIAN_POINT('Ctrl Pts',(0.321341667437633,2.07548487922013,12.8106686718477));
#37661=CARTESIAN_POINT('Ctrl Pts',(0.321269321853031,2.07455677295298,12.8106116154829));
#37662=CARTESIAN_POINT('Ctrl Pts',(0.321237561056537,2.0741588635969,12.810587126736));
#37663=CARTESIAN_POINT('Ctrl Pts',(0.321175062986253,2.07339379219501,12.8105399895523));
#37664=CARTESIAN_POINT('Ctrl Pts',(0.321144435160048,2.07302662160633,12.8105173445917));
#37665=CARTESIAN_POINT('Ctrl Pts',(0.321070784690939,2.07216159935117,12.8104639403661));
#37666=CARTESIAN_POINT('Ctrl Pts',(0.321027233731924,2.07166379470218,12.8104331645303));
#37667=CARTESIAN_POINT('Ctrl Pts',(0.320895129117275,2.07019319009003,12.8103421199722));
#37668=CARTESIAN_POINT('Ctrl Pts',(0.320803310768753,2.06922069568139,12.8102817486766));
#37669=CARTESIAN_POINT('Ctrl Pts',(0.319946577898176,2.06056719828913,12.8097430619174));
#37670=CARTESIAN_POINT('Ctrl Pts',(0.318910415135014,2.05291614794123,12.8092562430717));
#37671=CARTESIAN_POINT('Ctrl Pts',(0.31678603845607,2.04057923964921,12.8084531337641));
#37672=CARTESIAN_POINT('Ctrl Pts',(0.315865818340726,2.03586730899957,12.8081420660488));
#37673=CARTESIAN_POINT('Ctrl Pts',(0.308981607262987,2.00437409448425,12.8060342900635));
#37674=CARTESIAN_POINT('Ctrl Pts',(0.299723488107712,1.97842923616108,12.8041442608572));
#37675=CARTESIAN_POINT('Ctrl Pts',(0.282898017303006,1.945326029564,12.8016727225593));
#37676=CARTESIAN_POINT('Ctrl Pts',(0.278112616825124,1.93687815089933,12.801037605369));
#37677=CARTESIAN_POINT('Ctrl Pts',(0.272197009653912,1.92745439978341,12.8003345075261));
#37678=CARTESIAN_POINT('Ctrl Pts',(0.271433289850888,1.92625545891521,12.8002451616514));
#37679=CARTESIAN_POINT('Ctrl Pts',(0.270442207240963,1.92472207329882,12.8001310695506));
#37680=CARTESIAN_POINT('Ctrl Pts',(0.270222128836323,1.92438297309927,12.8001058498632));
#37681=CARTESIAN_POINT('Ctrl Pts',(0.269868321454398,1.9238400609642,12.8000654913053));
#37682=CARTESIAN_POINT('Ctrl Pts',(0.269734999180581,1.92363598648333,12.8000503253229));
#37683=CARTESIAN_POINT('Ctrl Pts',(0.269481210209441,1.92324847630247,12.800021535702));
#37684=CARTESIAN_POINT('Ctrl Pts',(0.269360788691905,1.92306501391504,12.8000079092662));
#37685=CARTESIAN_POINT('Ctrl Pts',(0.26908398215702,1.92264423622231,12.7999766647861));
#37686=CARTESIAN_POINT('Ctrl Pts',(0.268927470763725,1.92240700501213,12.7999590553954));
#37687=CARTESIAN_POINT('Ctrl Pts',(0.26844228150179,1.92167369445557,12.7999046401988));
#37688=CARTESIAN_POINT('Ctrl Pts',(0.268112540915502,1.92117831461427,12.7998679055396));
#37689=CARTESIAN_POINT('Ctrl Pts',(0.26553705631142,1.91733221972438,12.7995828708176));
#37690=CARTESIAN_POINT('Ctrl Pts',(0.263229831986759,1.91402283627209,12.7993386212626));
#37691=CARTESIAN_POINT('Ctrl Pts',(0.260362541519931,1.91007042612646,12.7990470087596));
#37692=CARTESIAN_POINT('Ctrl Pts',(0.259861411499974,1.90938535496712,12.7989964671431));
#37693=CARTESIAN_POINT('Ctrl Pts',(0.257822019165564,1.90662038835086,12.7987924588947));
#37694=CARTESIAN_POINT('Ctrl Pts',(0.256261408480435,1.90455701846726,12.7986401685053));
#37695=CARTESIAN_POINT('Ctrl Pts',(0.251532889154093,1.89845920760348,12.7981892328105));
#37696=CARTESIAN_POINT('Ctrl Pts',(0.248293244609554,1.89448125560719,12.7978938899385));
#37697=CARTESIAN_POINT('Ctrl Pts',(0.229027081004777,1.87194526764538,12.7962030526133));
#37698=CARTESIAN_POINT('Ctrl Pts',(0.211019549998739,1.8551874390649,12.7948681101692));
#37699=CARTESIAN_POINT('Ctrl Pts',(0.181451524726275,1.8333807551702,12.7927601774063));
#37700=CARTESIAN_POINT('Ctrl Pts',(0.17121428858235,1.82669413979487,12.792044300411));
#37701=CARTESIAN_POINT('Ctrl Pts',(0.159401752754256,1.81990315747046,12.7912208624954));
#37702=CARTESIAN_POINT('Ctrl Pts',(0.158175938246972,1.81920909480776,12.7911354497365));
#37703=CARTESIAN_POINT('Ctrl Pts',(0.15600551226607,1.81799891071448,12.7909842639244));
#37704=CARTESIAN_POINT('Ctrl Pts',(0.15506278575154,1.81747944031178,12.7909186114017));
#37705=CARTESIAN_POINT('Ctrl Pts',(0.153669483224819,1.81672076362164,12.7908215959574));
#37706=CARTESIAN_POINT('Ctrl Pts',(0.153220906514812,1.81647788509581,12.7907903640199));
#37707=CARTESIAN_POINT('Ctrl Pts',(0.152423451174443,1.81604855408418,12.790734845027));
#37708=CARTESIAN_POINT('Ctrl Pts',(0.152074801549055,1.81586167657782,12.7907105731414));
#37709=CARTESIAN_POINT('Ctrl Pts',(0.151395480458144,1.81549916641149,12.7906632828383));
#37710=CARTESIAN_POINT('Ctrl Pts',(0.151064845093423,1.81532346708805,12.7906402668332));
#37711=CARTESIAN_POINT('Ctrl Pts',(0.150272021668474,1.81490393162464,12.7905850789375));
#37712=CARTESIAN_POINT('Ctrl Pts',(0.149809546366781,1.81466064324797,12.7905528877185));
#37713=CARTESIAN_POINT('Ctrl Pts',(0.148137278417831,1.81378612118715,12.7904364906724));
#37714=CARTESIAN_POINT('Ctrl Pts',(0.146924084400398,1.81316145479842,12.7903520535319));
#37715=CARTESIAN_POINT('Ctrl Pts',(0.125250447984287,1.80217540580457,12.7888435831714));
#37716=CARTESIAN_POINT('Ctrl Pts',(0.103749911909894,1.79402169774127,12.7873397614731));
#37717=CARTESIAN_POINT('Ctrl Pts',(0.0673270662363956,1.78449245784487,
12.7848049970899));
#37718=CARTESIAN_POINT('Ctrl Pts',(0.0528449351368403,1.7817463954164,12.7838021723191));
#37719=CARTESIAN_POINT('Ctrl Pts',(0.0293869323174163,1.77894420343887,
12.7822209543241));
#37720=CARTESIAN_POINT('Ctrl Pts',(0.0205073360428285,1.77825492783069,
12.7816324253688));
#37721=CARTESIAN_POINT('Ctrl Pts',(0.00778265093736817,1.77779622428641,
12.7808130616387));
#37722=CARTESIAN_POINT('Ctrl Pts',(0.00395300021213832,1.77772648300974,
12.7805695799996));
#37723=CARTESIAN_POINT('Ctrl Pts',(-0.000414578155192063,1.7777248186117,
12.7802961344325));
#37724=CARTESIAN_POINT('Ctrl Pts',(-0.000951973252704545,1.77772595796316,
12.7802625623382));
#37725=CARTESIAN_POINT('Ctrl Pts',(-0.00176198122830027,1.77772970138882,
12.7802120724391));
#37726=CARTESIAN_POINT('Ctrl Pts',(-0.00203459437469886,1.77773130718012,
12.7801950990197));
#37727=CARTESIAN_POINT('Ctrl Pts',(-0.00252545891919314,1.77773482142982,
12.7801645719383));
#37728=CARTESIAN_POINT('Ctrl Pts',(-0.00274370991875125,1.77773660568031,
12.7801510113279));
#37729=CARTESIAN_POINT('Ctrl Pts',(-0.00321292090836895,1.77774091828092,
12.7801218847612));
#37730=CARTESIAN_POINT('Ctrl Pts',(-0.00346387904177128,1.77774351805712,
12.7801063229106));
#37731=CARTESIAN_POINT('Ctrl Pts',(-0.00414022903178649,1.77775131480055,
12.7800644265646));
#37732=CARTESIAN_POINT('Ctrl Pts',(-0.00456561592331929,1.77775706095342,
12.780038122924));
#37733=CARTESIAN_POINT('Ctrl Pts',(-0.00652796604187311,1.77778745502861,
12.779916992775));
#37734=CARTESIAN_POINT('Ctrl Pts',(-0.00806478485520179,1.77782225721948,
12.7798227266898));
#37735=CARTESIAN_POINT('Ctrl Pts',(-0.0386408573612863,1.77873359498489,
12.7779580846699));
#37736=CARTESIAN_POINT('Ctrl Pts',(-0.0674354029734516,1.78352201012447,
12.776388274738));
#37737=CARTESIAN_POINT('Ctrl Pts',(-0.114665652532731,1.79812580354504,
12.7736052269428));
#37738=CARTESIAN_POINT('Ctrl Pts',(-0.133511925421488,1.805975140956,12.7724335132134));
#37739=CARTESIAN_POINT('Ctrl Pts',(-0.152496191545028,1.81608559883235,
12.7711254711677));
#37740=CARTESIAN_POINT('Ctrl Pts',(-0.153499686134291,1.81662688566048,
12.7710559449282));
#37741=CARTESIAN_POINT('Ctrl Pts',(-0.154960410723947,1.81742483895959,
12.7709541698236));
#37742=CARTESIAN_POINT('Ctrl Pts',(-0.155419927956753,1.81767731845009,
12.7709220704237));
#37743=CARTESIAN_POINT('Ctrl Pts',(-0.156225552197426,1.81812252768252,
12.7708656474279));
#37744=CARTESIAN_POINT('Ctrl Pts',(-0.156571924684937,1.81831477682053,
12.7708413410783));
#37745=CARTESIAN_POINT('Ctrl Pts',(-0.157243979830494,1.81868941405107,
12.7707940871838));
#37746=CARTESIAN_POINT('Ctrl Pts',(-0.157569701974109,1.81887173038303,
12.770771142242));
#37747=CARTESIAN_POINT('Ctrl Pts',(-0.158346910146726,1.81930853188089,
12.7707162909197));
#37748=CARTESIAN_POINT('Ctrl Pts',(-0.158798099423586,1.81956354045466,
12.7706843657373));
#37749=CARTESIAN_POINT('Ctrl Pts',(-0.160412303274585,1.82048102022052,
12.770569850424));
#37750=CARTESIAN_POINT('Ctrl Pts',(-0.161571791127033,1.82114963990678,
12.7704870385978));
#37751=CARTESIAN_POINT('Ctrl Pts',(-0.17700632936119,1.83017856499719,12.769377160884));
#37752=CARTESIAN_POINT('Ctrl Pts',(-0.19061886661846,1.83961732083457,12.7683099364981));
#37753=CARTESIAN_POINT('Ctrl Pts',(-0.209923162783697,1.85533041284295,
12.7666585372885));
#37754=CARTESIAN_POINT('Ctrl Pts',(-0.216193343477245,1.86085283167352,
12.7660977226627));
#37755=CARTESIAN_POINT('Ctrl Pts',(-0.233885142392716,1.87769971653058,
12.7644485746494));
#37756=CARTESIAN_POINT('Ctrl Pts',(-0.244682821479849,1.88964311045779,
12.7633533654514));
#37757=CARTESIAN_POINT('Ctrl Pts',(-0.259691931728857,1.90897193653139,
12.7617331682992));
#37758=CARTESIAN_POINT('Ctrl Pts',(-0.264579190612359,1.91580038043099,
12.7611867309191));
#37759=CARTESIAN_POINT('Ctrl Pts',(-0.269915437390255,1.92390755000385,
12.7605740719818));
#37760=CARTESIAN_POINT('Ctrl Pts',(-0.270629541952309,1.92500701314151,
12.7604917287081));
#37761=CARTESIAN_POINT('Ctrl Pts',(-0.271546472468741,1.92643779291042,
12.7603855630568));
#37762=CARTESIAN_POINT('Ctrl Pts',(-0.271755423229029,1.92676514095191,
12.7603613402616));
#37763=CARTESIAN_POINT('Ctrl Pts',(-0.272092655439282,1.92729556989709,
12.7603221991707));
#37764=CARTESIAN_POINT('Ctrl Pts',(-0.272221301649726,1.92749841667333,
12.7603072565806));
#37765=CARTESIAN_POINT('Ctrl Pts',(-0.272467573732861,1.92788769514869,
12.7602786302581));
#37766=CARTESIAN_POINT('Ctrl Pts',(-0.272585234733785,1.92807410310701,
12.7602649442258));
#37767=CARTESIAN_POINT('Ctrl Pts',(-0.272855354150572,1.92850302221004,
12.760233502966));
#37768=CARTESIAN_POINT('Ctrl Pts',(-0.273007680997734,1.92874561670577,
12.7602157565404));
#37769=CARTESIAN_POINT('Ctrl Pts',(-0.273478318129193,1.92949737332277,
12.7601608757268));
#37770=CARTESIAN_POINT('Ctrl Pts',(-0.273795531305651,1.93000722591426,
12.7601238137817));
#37771=CARTESIAN_POINT('Ctrl Pts',(-0.276398715824301,1.93421747955254,
12.7598190473085));
#37772=CARTESIAN_POINT('Ctrl Pts',(-0.27861111930298,1.93796314331041,12.7595560630485));
#37773=CARTESIAN_POINT('Ctrl Pts',(-0.281261584416215,1.94266534272298,
12.759234447152));
#37774=CARTESIAN_POINT('Ctrl Pts',(-0.281771579301667,1.94358053062314,
12.7591722451662));
#37775=CARTESIAN_POINT('Ctrl Pts',(-0.298003790445098,1.97304630936764,
12.7571816555366));
#37776=CARTESIAN_POINT('Ctrl Pts',(-0.309310561368489,2.00381759938031,
12.7554484724751));
#37777=CARTESIAN_POINT('Ctrl Pts',(-0.318092910704573,2.04699607174501,
12.7529126429641));
#37778=CARTESIAN_POINT('Ctrl Pts',(-0.31977625636406,2.05833924538311,12.7522394874613));
#37779=CARTESIAN_POINT('Ctrl Pts',(-0.321043663119327,2.07178094364901,
12.7514231559741));
#37780=CARTESIAN_POINT('Ctrl Pts',(-0.321216083520347,2.07381649067866,
12.7512990480815));
#37781=CARTESIAN_POINT('Ctrl Pts',(-0.321418694191573,2.07651306478306,
12.7511339502529));
#37782=CARTESIAN_POINT('Ctrl Pts',(-0.321466220303422,2.0771727729399,12.7510935052819));
#37783=CARTESIAN_POINT('Ctrl Pts',(-0.321540852753819,2.07825522859776,
12.7510270520601));
#37784=CARTESIAN_POINT('Ctrl Pts',(-0.321569157189131,2.07867789374977,
12.7510010814739));
#37785=CARTESIAN_POINT('Ctrl Pts',(-0.321622348306308,2.07949639062806,
12.7509507446949));
#37786=CARTESIAN_POINT('Ctrl Pts',(-0.321647337796222,2.07989221509692,
12.7509263817767));
#37787=CARTESIAN_POINT('Ctrl Pts',(-0.321703294719823,2.08080535577262,
12.7508701313624));
#37788=CARTESIAN_POINT('Ctrl Pts',(-0.321733745071581,2.0813227015386,12.7508382276983));
#37789=CARTESIAN_POINT('Ctrl Pts',(-0.321811944325856,2.08270826229849,
12.7507526891531));
#37790=CARTESIAN_POINT('Ctrl Pts',(-0.321857427274629,2.08357659633482,
12.7506989833232));
#37791=CARTESIAN_POINT('Ctrl Pts',(-0.322151852056877,2.08966954076648,
12.7503214346279));
#37792=CARTESIAN_POINT('Ctrl Pts',(-0.322277069779807,2.09489908999244,
12.7499937336023));
#37793=CARTESIAN_POINT('Ctrl Pts',(-0.322270858283079,2.11040090480719,
12.7490107673536));
#37794=CARTESIAN_POINT('Ctrl Pts',(-0.32177566869535,2.12066562122389,12.7483446080737));
#37795=CARTESIAN_POINT('Ctrl Pts',(-0.317483520666422,2.16524176671075,
12.745388357424));
#37796=CARTESIAN_POINT('Ctrl Pts',(-0.308679940777706,2.19883680377138,
12.7429673497424));
#37797=CARTESIAN_POINT('Ctrl Pts',(-0.294193486321486,2.2315790475234,12.7407070839352));
#37798=CARTESIAN_POINT('Ctrl Pts',(-0.293662297977832,2.23276034054669,
12.7406257194122));
#37799=CARTESIAN_POINT('Ctrl Pts',(-0.292956578761065,2.23430480575694,
12.740519611485));
#37800=CARTESIAN_POINT('Ctrl Pts',(-0.292788477815313,2.23467087714721,
12.7404944816792));
#37801=CARTESIAN_POINT('Ctrl Pts',(-0.292527867487607,2.2352356106612,12.7404557463465));
#37802=CARTESIAN_POINT('Ctrl Pts',(-0.292435841857345,2.23543449355916,
12.7404421110324));
#37803=CARTESIAN_POINT('Ctrl Pts',(-0.292251793430961,2.23583119104158,
12.7404149261675));
#37804=CARTESIAN_POINT('Ctrl Pts',(-0.292159773263715,2.23602900466564,
12.7404013766651));
#37805=CARTESIAN_POINT('Ctrl Pts',(-0.291952818973589,2.23647271078912,
12.7403709983576));
#37806=CARTESIAN_POINT('Ctrl Pts',(-0.291837775319167,2.23671855102661,
12.7403541764921));
#37807=CARTESIAN_POINT('Ctrl Pts',(-0.291496483398094,2.23744547434984,
12.7403044635083));
#37808=CARTESIAN_POINT('Ctrl Pts',(-0.291269353764116,2.2379261462526,12.7402716268644));
#37809=CARTESIAN_POINT('Ctrl Pts',(-0.289469286846647,2.24171133157789,
12.7400133098462));
#37810=CARTESIAN_POINT('Ctrl Pts',(-0.287841273360165,2.24498956392793,
12.7397911798443));
#37811=CARTESIAN_POINT('Ctrl Pts',(-0.281843657943182,2.25656720370941,
12.7390098917046));
#37812=CARTESIAN_POINT('Ctrl Pts',(-0.277167769857751,2.26470335392474,
12.7384667421102));
#37813=CARTESIAN_POINT('Ctrl Pts',(-0.264265181171557,2.28504432835819,
12.737094776661));
#37814=CARTESIAN_POINT('Ctrl Pts',(-0.255545947242584,2.29691060871783,
12.7362800029481));
#37815=CARTESIAN_POINT('Ctrl Pts',(-0.237041839132695,2.31878466718948,
12.7346741001606));
#37816=CARTESIAN_POINT('Ctrl Pts',(-0.227356549554287,2.32883294675853,
12.7338855995298));
#37817=CARTESIAN_POINT('Ctrl Pts',(-0.21034972029776,2.34432841998635,12.7325426643839));
#37818=CARTESIAN_POINT('Ctrl Pts',(-0.203393526719695,2.35014881845531,
12.7320036011275));
#37819=CARTESIAN_POINT('Ctrl Pts',(-0.195302537861792,2.35635791183437,
12.7313833309925));
#37820=CARTESIAN_POINT('Ctrl Pts',(-0.194399749656025,2.35704318224302,
12.7313142147422));
#37821=CARTESIAN_POINT('Ctrl Pts',(-0.193079620064435,2.35803430707788,
12.7312132748753));
#37822=CARTESIAN_POINT('Ctrl Pts',(-0.192665120293248,2.35834394657286,
12.7311815995305));
#37823=CARTESIAN_POINT('Ctrl Pts',(-0.19193167579708,2.3588890971858,12.7311255822123));
#37824=CARTESIAN_POINT('Ctrl Pts',(-0.191613037968386,2.35912502097299,
12.7311012563954));
#37825=CARTESIAN_POINT('Ctrl Pts',(-0.190952768598169,2.35961200961382,
12.7310508703488));
#37826=CARTESIAN_POINT('Ctrl Pts',(-0.190611075522273,2.35986298939353,
12.7310248068777));
#37827=CARTESIAN_POINT('Ctrl Pts',(-0.189733764755043,2.36050472878076,
12.7309579169297));
#37828=CARTESIAN_POINT('Ctrl Pts',(-0.189197436589199,2.36089450968321,
12.7309170526456));
#37829=CARTESIAN_POINT('Ctrl Pts',(-0.186993168925861,2.36248610780821,
12.7307492133639));
#37830=CARTESIAN_POINT('Ctrl Pts',(-0.185314979742844,2.36367358605934,
12.7306216876413));
#37831=CARTESIAN_POINT('Ctrl Pts',(-0.174109977673614,2.37144237792792,
12.7297717653415));
#37832=CARTESIAN_POINT('Ctrl Pts',(-0.164246846310098,2.37752147305494,
12.7290305104738));
#37833=CARTESIAN_POINT('Ctrl Pts',(-0.124942825128483,2.39891624594211,
12.7261005811851));
#37834=CARTESIAN_POINT('Ctrl Pts',(-0.0935381426399251,2.41018025238688,
12.7237844048989));
#37835=CARTESIAN_POINT('Ctrl Pts',(-0.0608254647214458,2.41648295436013,
12.7216279247192));
#37836=CARTESIAN_POINT('Ctrl Pts',(-0.0606800181313171,2.41651087336589,
12.7216183420291));
#37837=CARTESIAN_POINT('Ctrl Pts',(-0.0603166475295293,2.41658036400689,
12.7215944151184));
#37838=CARTESIAN_POINT('Ctrl Pts',(-0.0600986994030898,2.41662181095834,
12.7215800760894));
#37839=CARTESIAN_POINT('Ctrl Pts',(-0.0556300762085716,2.4174668237735,
12.7212863337734));
#37840=CARTESIAN_POINT('Ctrl Pts',(-0.0513634264563727,2.4181849973752,
12.7210105550523));
#37841=CARTESIAN_POINT('Ctrl Pts',(-0.0465424715136856,2.41889696284348,
12.7207051798045));
#37842=CARTESIAN_POINT('Ctrl Pts',(-0.0460013764860825,2.41897546604275,
12.7206709931862));
#37843=CARTESIAN_POINT('Ctrl Pts',(-0.045184049981826,2.41909192247915,
12.720619489867));
#37844=CARTESIAN_POINT('Ctrl Pts',(-0.0449079681481661,2.41913089440299,
12.7206021161082));
#37845=CARTESIAN_POINT('Ctrl Pts',(-0.0444286350722031,2.41919792309505,
12.720571992766));
#37846=CARTESIAN_POINT('Ctrl Pts',(-0.044225407561986,2.41922614405636,
12.7205592338562));
#37847=CARTESIAN_POINT('Ctrl Pts',(-0.043800496915967,2.41928473524476,
12.7205325842717));
#37848=CARTESIAN_POINT('Ctrl Pts',(-0.0435788092353001,2.41931506866474,
12.7205186957714));
#37849=CARTESIAN_POINT('Ctrl Pts',(-0.0430488143718693,2.41938702539646,
12.7204855284205));
#37850=CARTESIAN_POINT('Ctrl Pts',(-0.04274047709039,2.4194284333469,12.720466261838));
#37851=CARTESIAN_POINT('Ctrl Pts',(-0.0416963825037867,2.41956711049236,
12.7204011189465));
#37852=CARTESIAN_POINT('Ctrl Pts',(-0.0409603423033512,2.41966228555527,
12.7203553604523));
#37853=CARTESIAN_POINT('Ctrl Pts',(-0.0392092061358328,2.41988257192766,
12.7202468716592));
#37854=CARTESIAN_POINT('Ctrl Pts',(-0.0381938234744561,2.4200053961753,
12.7201842659374));
#37855=CARTESIAN_POINT('Ctrl Pts',(-0.0260526719490014,2.42141542126039,
12.7194390827068));
#37856=CARTESIAN_POINT('Ctrl Pts',(-0.0148663570043847,2.42212678279148,
12.7187865790783));
#37857=CARTESIAN_POINT('Ctrl Pts',(0.0239225773776201,2.42256787326939,
12.7165729937292));
#37858=CARTESIAN_POINT('Ctrl Pts',(0.0514353445574283,2.41933810346185,
12.7150784566859));
#37859=CARTESIAN_POINT('Ctrl Pts',(0.0884705579172079,2.4100744909077,12.7128643718395));
#37860=CARTESIAN_POINT('Ctrl Pts',(0.0986059675968008,2.4070017203914,12.7122377628991));
#37861=CARTESIAN_POINT('Ctrl Pts',(0.109680877358072,2.40303905690927,12.7115226275228));
#37862=CARTESIAN_POINT('Ctrl Pts',(0.110788441748999,2.40263589672669,12.7114507676475));
#37863=CARTESIAN_POINT('Ctrl Pts',(0.112342347476113,2.40206059227251,12.7113494592059));
#37864=CARTESIAN_POINT('Ctrl Pts',(0.112790564475416,2.40189351268598,12.7113201797891));
#37865=CARTESIAN_POINT('Ctrl Pts',(0.113612467228913,2.40158505026827,12.711266383435));
#37866=CARTESIAN_POINT('Ctrl Pts',(0.113986265795373,2.40144396902725,12.7112418766272));
#37867=CARTESIAN_POINT('Ctrl Pts',(0.114743619069936,2.401156514204,12.7111921409791));
#37868=CARTESIAN_POINT('Ctrl Pts',(0.115127158289912,2.40101010213343,12.7111669108853));
#37869=CARTESIAN_POINT('Ctrl Pts',(0.116071452568792,2.40064755891778,12.7111046866247));
#37870=CARTESIAN_POINT('Ctrl Pts',(0.116631883181514,2.40043059198818,12.7110676644404));
#37871=CARTESIAN_POINT('Ctrl Pts',(0.118678841640688,2.39963153500491,12.7109321005294));
#37872=CARTESIAN_POINT('Ctrl Pts',(0.120161626574517,2.39903997654881,12.7108332405108));
#37873=CARTESIAN_POINT('Ctrl Pts',(0.139958245769743,2.39097108445333,12.7095043638443));
#37874=CARTESIAN_POINT('Ctrl Pts',(0.157546728757828,2.38183550461061,12.7082161720322));
#37875=CARTESIAN_POINT('Ctrl Pts',(0.198618277278576,2.35545124590271,12.7049475942317));
#37876=CARTESIAN_POINT('Ctrl Pts',(0.220818504250289,2.33652452852572,12.7029338638387));
#37877=CARTESIAN_POINT('Ctrl Pts',(0.241187353923832,2.31375711571281,12.7010016026221));
#37878=CARTESIAN_POINT('Ctrl Pts',(0.242183755866325,2.312627544818,12.7009068678861));
#37879=CARTESIAN_POINT('Ctrl Pts',(0.243449252418657,2.31117247766962,12.7007863216411));
#37880=CARTESIAN_POINT('Ctrl Pts',(0.243725655883097,2.31085340523103,12.7007599785039));
#37881=CARTESIAN_POINT('Ctrl Pts',(0.244164884948457,2.31034435382241,12.7007180958952));
#37882=CARTESIAN_POINT('Ctrl Pts',(0.244328116418331,2.31015472812991,12.7007025263277));
#37883=CARTESIAN_POINT('Ctrl Pts',(0.24463202642518,2.3098008437612,12.7006735299879));
#37884=CARTESIAN_POINT('Ctrl Pts',(0.244772759380092,2.30963663482715,12.7006600991993));
#37885=CARTESIAN_POINT('Ctrl Pts',(0.245086986398828,2.30926924309419,12.7006301034972));
#37886=CARTESIAN_POINT('Ctrl Pts',(0.245260392734177,2.30906598662717,12.7006135451364));
#37887=CARTESIAN_POINT('Ctrl Pts',(0.245769457081035,2.30846778704644,12.7005649190285));
#37888=CARTESIAN_POINT('Ctrl Pts',(0.246104417332713,2.30807224718382,12.7005329027107));
#37889=CARTESIAN_POINT('Ctrl Pts',(0.246863601991946,2.30717136136361,12.700460286179));
#37890=CARTESIAN_POINT('Ctrl Pts',(0.247287233242557,2.30666551538809,12.7004197285185));
#37891=CARTESIAN_POINT('Ctrl Pts',(0.251025882491353,2.30217334634081,12.7000614312949));
#37892=CARTESIAN_POINT('Ctrl Pts',(0.254246032364896,2.29810860135809,12.6997502627613));
#37893=CARTESIAN_POINT('Ctrl Pts',(0.261105646015792,2.28900689039399,12.6990772124062));
#37894=CARTESIAN_POINT('Ctrl Pts',(0.264700385988307,2.28393878625517,12.6987176277412));
#37895=CARTESIAN_POINT('Ctrl Pts',(0.279536150612351,2.26168579952436,12.6971884363827));
#37896=CARTESIAN_POINT('Ctrl Pts',(0.289267370979552,2.24355213158384,12.6960629947269));
#37897=CARTESIAN_POINT('Ctrl Pts',(0.304143724761689,2.20807201516693,12.6938863882927));
#37898=CARTESIAN_POINT('Ctrl Pts',(0.309685754581759,2.19098107927744,12.6928478260964));
#37899=CARTESIAN_POINT('Ctrl Pts',(0.314069602660388,2.17227104789943,12.6916805379382));
#37900=CARTESIAN_POINT('Ctrl Pts',(0.314354651685597,2.17102093050411,12.6916024166488));
#37901=CARTESIAN_POINT('Ctrl Pts',(0.314742386399003,2.16927239520752,12.6914929585882));
#37902=CARTESIAN_POINT('Ctrl Pts',(0.314851365817075,2.16877537329861,12.691461823697));
#37903=CARTESIAN_POINT('Ctrl Pts',(0.315037724818665,2.16791572023286,12.6914079348117));
#37904=CARTESIAN_POINT('Ctrl Pts',(0.315115656704324,2.16755320874398,12.6913851985492));
#37905=CARTESIAN_POINT('Ctrl Pts',(0.315275851077469,2.16680173211615,12.6913380425478));
#37906=CARTESIAN_POINT('Ctrl Pts',(0.315358019742335,2.16641274778478,12.6913136198477));
#37907=CARTESIAN_POINT('Ctrl Pts',(0.315548697814019,2.16550174964194,12.691256390038));
#37908=CARTESIAN_POINT('Ctrl Pts',(0.315656631745686,2.1649796177874,12.691223564586));
#37909=CARTESIAN_POINT('Ctrl Pts',(0.31600083677188,2.16329342500347,12.6911174759556));
#37910=CARTESIAN_POINT('Ctrl Pts',(0.316231966110548,2.16212833523045,12.6910440487884));
#37911=CARTESIAN_POINT('Ctrl Pts',(0.319789327093048,2.14366190689422,12.6898782062644));
#37912=CARTESIAN_POINT('Ctrl Pts',(0.321697211899241,2.12612072780041,12.6887399424266));
#37913=CARTESIAN_POINT('Ctrl Pts',(0.322896336572627,2.08074693582228,12.6857215332683));
#37914=CARTESIAN_POINT('Ctrl Pts',(0.320037440726205,2.05300341902457,12.6837975962204));
#37915=CARTESIAN_POINT('Ctrl Pts',(0.313477510586859,2.02520937129726,12.6819436929028));
#37916=CARTESIAN_POINT('Ctrl Pts',(0.313295011307161,2.02444853609156,12.6818930120875));
#37917=CARTESIAN_POINT('Ctrl Pts',(0.312894083096318,2.0228035113205,12.681783591494));
#37918=CARTESIAN_POINT('Ctrl Pts',(0.312674672367909,2.02191956455509,12.6817248937903));
#37919=CARTESIAN_POINT('Ctrl Pts',(0.31157987672749,2.01758755329321,12.681437755011));
#37920=CARTESIAN_POINT('Ctrl Pts',(0.310651145150706,2.01415304568063,12.6812117370444));
#37921=CARTESIAN_POINT('Ctrl Pts',(0.309506854177506,2.01018345550559,12.6809529685311));
#37922=CARTESIAN_POINT('Ctrl Pts',(0.309346550333297,2.00963288066616,12.6809171331943));
#37923=CARTESIAN_POINT('Ctrl Pts',(0.309105805559018,2.00881417349964,12.680863931437));
#37924=CARTESIAN_POINT('Ctrl Pts',(0.309026484527284,2.00854571717531,12.6808465001436));
#37925=CARTESIAN_POINT('Ctrl Pts',(0.308884498576148,2.00806746983367,12.680815471657));
#37926=CARTESIAN_POINT('Ctrl Pts',(0.308821969686714,2.00785763947397,12.6808018665102));
#37927=CARTESIAN_POINT('Ctrl Pts',(0.30869010871261,2.00741679102963,12.680773300529));
#37928=CARTESIAN_POINT('Ctrl Pts',(0.308620731321345,2.00718578772705,12.6807583424441));
#37929=CARTESIAN_POINT('Ctrl Pts',(0.308442352732378,2.00659425860689,12.6807200654912));
#37930=CARTESIAN_POINT('Ctrl Pts',(0.308332978348298,2.00623384432227,12.6806967685287));
#37931=CARTESIAN_POINT('Ctrl Pts',(0.308087707462199,2.00543068880162,12.6806449068712));
#37932=CARTESIAN_POINT('Ctrl Pts',(0.307951487610129,2.0049880460427,12.6806163609016));
#37933=CARTESIAN_POINT('Ctrl Pts',(0.307547099997746,2.00368400537686,12.6805323670296));
#37934=CARTESIAN_POINT('Ctrl Pts',(0.307276266163541,2.00282342960248,12.6804770702883));
#37935=CARTESIAN_POINT('Ctrl Pts',(0.30427741567572,1.9934324664209,12.6798749926308));
#37936=CARTESIAN_POINT('Ctrl Pts',(0.301198279006492,1.98501733199069,12.679347580168));
#37937=CARTESIAN_POINT('Ctrl Pts',(0.291768628981438,1.96223701163983,12.677925578984));
#37938=CARTESIAN_POINT('Ctrl Pts',(0.284713056773765,1.94819055658742,12.6770545096981));
#37939=CARTESIAN_POINT('Ctrl Pts',(0.264125894669908,1.91373112846354,12.6748090552013));
#37940=CARTESIAN_POINT('Ctrl Pts',(0.249246347445778,1.89424628660456,12.6734262111375));
#37941=CARTESIAN_POINT('Ctrl Pts',(0.231270508978587,1.87555095633149,12.6718531054586));
#37942=CARTESIAN_POINT('Ctrl Pts',(0.230224297779887,1.87447795203033,12.6717618851207));
#37943=CARTESIAN_POINT('Ctrl Pts',(0.228788339010278,1.87302562426727,12.6716371196519));
#37944=CARTESIAN_POINT('Ctrl Pts',(0.228405047547426,1.8726399209283,12.6716038587613));
#37945=CARTESIAN_POINT('Ctrl Pts',(0.227752117998115,1.87198620017677,12.6715472696857));
#37946=CARTESIAN_POINT('Ctrl Pts',(0.22748297753402,1.87171768554549,12.6715239635638));
#37947=CARTESIAN_POINT('Ctrl Pts',(0.226962325160456,1.87120007891595,12.6714789163482));
#37948=CARTESIAN_POINT('Ctrl Pts',(0.226710876605779,1.87095092369237,12.6714571780889));
#37949=CARTESIAN_POINT('Ctrl Pts',(0.226114488235349,1.87036191884447,12.6714056595011));
#37950=CARTESIAN_POINT('Ctrl Pts',(0.225769192675481,1.87002243209101,12.6713758633001));
#37951=CARTESIAN_POINT('Ctrl Pts',(0.224752604973225,1.86902744210202,12.6712882325723));
#37952=CARTESIAN_POINT('Ctrl Pts',(0.224079218108836,1.86837409487254,12.6712303040307));
#37953=CARTESIAN_POINT('Ctrl Pts',(0.218950725517841,1.8634415184044,12.6707899955996));
#37954=CARTESIAN_POINT('Ctrl Pts',(0.21437652834929,1.8592884901205,12.6704022100983));
#37955=CARTESIAN_POINT('Ctrl Pts',(0.205611153919882,1.85177827690984,12.6696673542998));
#37956=CARTESIAN_POINT('Ctrl Pts',(0.201449877432279,1.84838936424058,12.669321742861));
#37957=CARTESIAN_POINT('Ctrl Pts',(0.185326038360252,1.83591468623627,12.667994811072));
#37958=CARTESIAN_POINT('Ctrl Pts',(0.172819057310317,1.82756599952935,12.6669891042642));
#37959=CARTESIAN_POINT('Ctrl Pts',(0.145573845088344,1.81201233009996,12.6648691191675));
#37960=CARTESIAN_POINT('Ctrl Pts',(0.13077376418729,1.80499676526009,12.6637560853862));
#37961=CARTESIAN_POINT('Ctrl Pts',(0.11425437003661,1.79865483582613,12.6625909335711));
#37962=CARTESIAN_POINT('Ctrl Pts',(0.113001153961262,1.79818265731498,12.6625030144126));
#37963=CARTESIAN_POINT('Ctrl Pts',(0.105573479386464,1.79543685564542,12.6619848581212));
#37964=CARTESIAN_POINT('Ctrl Pts',(0.0993329737775362,1.79334474788145,
12.6615614341212));
#37965=CARTESIAN_POINT('Ctrl Pts',(0.0924467617944067,1.79126848904973,
12.6611103419266));
#37966=CARTESIAN_POINT('Ctrl Pts',(0.0918607387770176,1.79109361562805,
12.6610720800819));
#37967=CARTESIAN_POINT('Ctrl Pts',(0.0909912654010182,1.79083685166463,
12.6610155026688));
#37968=CARTESIAN_POINT('Ctrl Pts',(0.0907081989301965,1.79075368180613,
12.6609971132553));
#37969=CARTESIAN_POINT('Ctrl Pts',(0.0902239783409053,1.7906121314146,12.6609657075822));
#37970=CARTESIAN_POINT('Ctrl Pts',(0.0900228814852149,1.79055355826065,
12.6609526800409));
#37971=CARTESIAN_POINT('Ctrl Pts',(0.0896307847982094,1.79043976745867,
12.6609273089579));
#37972=CARTESIAN_POINT('Ctrl Pts',(0.0894397915376084,1.79038453067644,
12.6609149643517));
#37973=CARTESIAN_POINT('Ctrl Pts',(0.0890437692126625,1.79027039486817,
12.6608893964575));
#37974=CARTESIAN_POINT('Ctrl Pts',(0.088838732379173,1.79021152255029,12.6608761747367));
#37975=CARTESIAN_POINT('Ctrl Pts',(0.0881847645862222,1.7900244511367,12.660834053848));
#37976=CARTESIAN_POINT('Ctrl Pts',(0.0877356108046971,1.78989702323027,
12.6608051997071));
#37977=CARTESIAN_POINT('Ctrl Pts',(0.0850872172821791,1.78915187100529,
12.6606354972821));
#37978=CARTESIAN_POINT('Ctrl Pts',(0.0828816657773448,1.78855654762444,
12.6604959303619));
#37979=CARTESIAN_POINT('Ctrl Pts',(0.0762912027958152,1.78685261842885,
12.6600836031961));
#37980=CARTESIAN_POINT('Ctrl Pts',(0.0718889212248584,1.78581276652288,
12.6598143622473));
#37981=CARTESIAN_POINT('Ctrl Pts',(0.0547956051997901,1.78215331756569,
12.6587876189092));
#37982=CARTESIAN_POINT('Ctrl Pts',(0.0419720889116463,1.78020714458005,
12.6580565142472));
#37983=CARTESIAN_POINT('Ctrl Pts',(0.005409857505952,1.77689618010248,12.6559995533956));
#37984=CARTESIAN_POINT('Ctrl Pts',(-0.0184077162975488,1.77737575342825,
12.6546865021522));
#37985=CARTESIAN_POINT('Ctrl Pts',(-0.0493395550389234,1.78143722189983,
12.6528522675982));
#37986=CARTESIAN_POINT('Ctrl Pts',(-0.0566869767453593,1.78266231153574,
12.6524074304611));
#37987=CARTESIAN_POINT('Ctrl Pts',(-0.0649325281241641,1.78433264796437,
12.6518955500821));
#37988=CARTESIAN_POINT('Ctrl Pts',(-0.0658792161887074,1.78452886155427,
12.6518365911073));
#37989=CARTESIAN_POINT('Ctrl Pts',(-0.0673113236936698,1.78483241209612,
12.6517471092636));
#37990=CARTESIAN_POINT('Ctrl Pts',(-0.0677974070490249,1.78493661851049,
12.651716686581));
#37991=CARTESIAN_POINT('Ctrl Pts',(-0.0686426883493315,1.78511987640807,
12.6516636932915));
#37992=CARTESIAN_POINT('Ctrl Pts',(-0.0690019966403035,1.78519841907175,
12.6516411390238));
#37993=CARTESIAN_POINT('Ctrl Pts',(-0.0697514783881423,1.78536359614808,
12.6515940339977));
#37994=CARTESIAN_POINT('Ctrl Pts',(-0.0701416265266435,1.78545034161177,
12.6515694797097));
#37995=CARTESIAN_POINT('Ctrl Pts',(-0.0710638396406129,1.78565718739193,
12.6515113599366));
#37996=CARTESIAN_POINT('Ctrl Pts',(-0.0715957618047044,1.78577791288869,
12.6514777744244));
#37997=CARTESIAN_POINT('Ctrl Pts',(-0.0733513243900375,1.7861810460031,
12.6513667196834));
#37998=CARTESIAN_POINT('Ctrl Pts',(-0.0745736090558756,1.7864692528024,
12.6512890642116));
#37999=CARTESIAN_POINT('Ctrl Pts',(-0.0950365845363402,1.79142071770933,
12.6499832722463));
#38000=CARTESIAN_POINT('Ctrl Pts',(-0.113805296649084,1.7978390851135,12.6486966595016));
#38001=CARTESIAN_POINT('Ctrl Pts',(-0.139903283602466,1.80954195707377,
12.6467835617785));
#38002=CARTESIAN_POINT('Ctrl Pts',(-0.147791214723686,1.81347504213293,
12.6461883148161));
#38003=CARTESIAN_POINT('Ctrl Pts',(-0.164165111723942,1.82249560916032,
12.6449233106211));
#38004=CARTESIAN_POINT('Ctrl Pts',(-0.172598591702555,1.82766086073706,
12.6442539267819));
#38005=CARTESIAN_POINT('Ctrl Pts',(-0.184296708382683,1.8355875777654,12.6433098837101));
#38006=CARTESIAN_POINT('Ctrl Pts',(-0.187764609461418,1.83803882030308,
12.6430279864428));
#38007=CARTESIAN_POINT('Ctrl Pts',(-0.191705027663266,1.84094251947338,
12.6427061257315));
#38008=CARTESIAN_POINT('Ctrl Pts',(-0.192225729275967,1.8413286547306,12.6426635621124));
#38009=CARTESIAN_POINT('Ctrl Pts',(-0.194282966337951,1.8428638766497,12.6424952823922));
#38010=CARTESIAN_POINT('Ctrl Pts',(-0.195810421801844,1.84402512629723,
12.6423700822728));
#38011=CARTESIAN_POINT('Ctrl Pts',(-0.198185554477325,1.84586452510421,
12.6421751088282));
#38012=CARTESIAN_POINT('Ctrl Pts',(-0.199040310760639,1.84653341766826,
12.6421048822281));
#38013=CARTESIAN_POINT('Ctrl Pts',(-0.203096257690227,1.84974058263086,
12.6417714218089));
#38014=CARTESIAN_POINT('Ctrl Pts',(-0.206252549160517,1.8523353967536,12.6415112532114));
#38015=CARTESIAN_POINT('Ctrl Pts',(-0.20976783025766,1.85533916854319,12.6412215417368));
#38016=CARTESIAN_POINT('Ctrl Pts',(-0.210175967488279,1.85568968961498,
12.6411879059524));
#38017=CARTESIAN_POINT('Ctrl Pts',(-0.21079258546576,1.85622194925309,12.6411370924412));
#38018=CARTESIAN_POINT('Ctrl Pts',(-0.211001710642537,1.85640293470438,
12.6411198597673));
#38019=CARTESIAN_POINT('Ctrl Pts',(-0.211365142854505,1.8567182829014,12.6410899131889));
#38020=CARTESIAN_POINT('Ctrl Pts',(-0.211519554966323,1.85685252344359,
12.641077190221));
#38021=CARTESIAN_POINT('Ctrl Pts',(-0.211829823873968,1.85712277971408,
12.6410516264236));
#38022=CARTESIAN_POINT('Ctrl Pts',(-0.211985677444673,1.85725879835744,
12.6410387858907));
#38023=CARTESIAN_POINT('Ctrl Pts',(-0.21230658669911,1.85753941140907,12.6410123476971));
#38024=CARTESIAN_POINT('Ctrl Pts',(-0.212471626170902,1.85768402477619,
12.6409987514317));
#38025=CARTESIAN_POINT('Ctrl Pts',(-0.212856360537317,1.85802183777206,
12.6409670572247));
#38026=CARTESIAN_POINT('Ctrl Pts',(-0.213075940750248,1.85821516860771,
12.6409489690446));
#38027=CARTESIAN_POINT('Ctrl Pts',(-0.214322703550612,1.85931590651822,
12.6408462675182));
#38028=CARTESIAN_POINT('Ctrl Pts',(-0.215344373102298,1.86022957804808,
12.6407621158182));
#38029=CARTESIAN_POINT('Ctrl Pts',(-0.222733415671263,1.86692287150594,
12.6401532915388));
#38030=CARTESIAN_POINT('Ctrl Pts',(-0.22887364789554,1.87294933499325,12.6396461842112));
#38031=CARTESIAN_POINT('Ctrl Pts',(-0.239115342780323,1.88383956437788,
12.6387825210659));
#38032=CARTESIAN_POINT('Ctrl Pts',(-0.243327269256387,1.88859203560086,
12.6384215133403));
#38033=CARTESIAN_POINT('Ctrl Pts',(-0.261554233234643,1.91042515595422,
12.6368169446537));
#38034=CARTESIAN_POINT('Ctrl Pts',(-0.27393050852774,1.92879453648479,12.6356046307471));
#38035=CARTESIAN_POINT('Ctrl Pts',(-0.286391385280005,1.9521476635516,12.6340807282555));
#38036=CARTESIAN_POINT('Ctrl Pts',(-0.288373216098588,1.95605131132475,
12.6338267181539));
#38037=CARTESIAN_POINT('Ctrl Pts',(-0.291064666902309,1.96163150468679,
12.6334637986043));
#38038=CARTESIAN_POINT('Ctrl Pts',(-0.291840587455013,1.96327563440083,
12.6333568925903));
#38039=CARTESIAN_POINT('Ctrl Pts',(-0.295345725427335,1.97086861273787,
12.6328631156283));
#38040=CARTESIAN_POINT('Ctrl Pts',(-0.297907083236376,1.97689283849018,
12.6324711441923));
#38041=CARTESIAN_POINT('Ctrl Pts',(-0.30065887570407,1.98395480606048,12.6320098650307));
#38042=CARTESIAN_POINT('Ctrl Pts',(-0.301029958345309,1.98492085021364,
12.6319467272545));
#38043=CARTESIAN_POINT('Ctrl Pts',(-0.301574807989261,1.98635993333962,
12.6318526123332));
#38044=CARTESIAN_POINT('Ctrl Pts',(-0.301752131290522,1.98683162623151,
12.6318217543231));
#38045=CARTESIAN_POINT('Ctrl Pts',(-0.302065878713144,1.98767219745387,
12.6317667464572));
#38046=CARTESIAN_POINT('Ctrl Pts',(-0.302202735570087,1.98804091408301,
12.6317426111193));
#38047=CARTESIAN_POINT('Ctrl Pts',(-0.302489306685563,1.98881734124193,
12.6316917746865));
#38048=CARTESIAN_POINT('Ctrl Pts',(-0.302638872267206,1.98922510547277,
12.631665068688));
#38049=CARTESIAN_POINT('Ctrl Pts',(-0.303030586127574,1.99029975900531,
12.6315946646836));
#38050=CARTESIAN_POINT('Ctrl Pts',(-0.303271356258478,1.99096714502778,
12.6315509208745));
#38051=CARTESIAN_POINT('Ctrl Pts',(-0.304340411217701,1.99396137500652,
12.6313545645777));
#38052=CARTESIAN_POINT('Ctrl Pts',(-0.305144116780036,1.9962968499079,12.6312011385203));
#38053=CARTESIAN_POINT('Ctrl Pts',(-0.310843940760075,2.01350005836985,
12.6300687619498));
#38054=CARTESIAN_POINT('Ctrl Pts',(-0.314677184054625,2.02869547292112,
12.6290548053835));
#38055=CARTESIAN_POINT('Ctrl Pts',(-0.320654555095514,2.06263845251039,
12.6267647108128));
#38056=CARTESIAN_POINT('Ctrl Pts',(-0.322288461322062,2.08141875410052,
12.6254806111673));
#38057=CARTESIAN_POINT('Ctrl Pts',(-0.322274916475093,2.10023202580047,
12.6242160103981));
#38058=CARTESIAN_POINT('',(-0.322553225215846,2.09975585955174,12.4993773449273));
#38059=CARTESIAN_POINT('Ctrl Pts',(-0.322553225215846,2.09975585955174,
12.4993773449273));
#38060=CARTESIAN_POINT('Ctrl Pts',(-0.322684578197607,2.08414723200036,
12.5003433061249));
#38061=CARTESIAN_POINT('Ctrl Pts',(-0.314554479716074,1.96165005111452,
12.5079327151634));
#38062=CARTESIAN_POINT('Ctrl Pts',(-0.157588690559167,1.75304050246825,
12.5221455720428));
#38063=CARTESIAN_POINT('Ctrl Pts',(0.206424151974156,1.77968116227517,12.5420159155657));
#38064=CARTESIAN_POINT('Ctrl Pts',(0.38107093718189,2.10017074822258,12.5618862590884));
#38065=CARTESIAN_POINT('Ctrl Pts',(0.206137015648765,2.42050369592105,12.5817566026112));
#38066=CARTESIAN_POINT('Ctrl Pts',(-0.157899554721464,2.44681813525015,
12.601626946134));
#38067=CARTESIAN_POINT('Ctrl Pts',(-0.314612782206414,2.23815528960921,
12.6158338602394));
#38068=CARTESIAN_POINT('Ctrl Pts',(-0.322686048272827,2.11575543190525,
12.6234173265038));
#38069=CARTESIAN_POINT('Ctrl Pts',(-0.322555864543089,2.10024316196973,
12.6243773449273));
#38070=CARTESIAN_POINT('',(-0.322274864054643,2.10029601277207,12.2494497673494));
#38071=CARTESIAN_POINT('Ctrl Pts',(-0.322274900757235,2.09974708318754,
12.4992173059391));
#38072=CARTESIAN_POINT('Ctrl Pts',(-0.322290026286624,2.11902052901133,
12.4981254716813));
#38073=CARTESIAN_POINT('Ctrl Pts',(-0.320576212832934,2.13825717465125,
12.4970659124543));
#38074=CARTESIAN_POINT('Ctrl Pts',(-0.314206619257685,2.17355803539727,
12.4950292330845));
#38075=CARTESIAN_POINT('Ctrl Pts',(-0.310003156025341,2.18963542280539,
12.4940645046333));
#38076=CARTESIAN_POINT('Ctrl Pts',(-0.304151340170072,2.20655921977322,
12.4929768269527));
#38077=CARTESIAN_POINT('Ctrl Pts',(-0.303713988176344,2.20779943576773,
12.4928967005569));
#38078=CARTESIAN_POINT('Ctrl Pts',(-0.303081013869604,2.20955995426099,
12.4927823501861));
#38079=CARTESIAN_POINT('Ctrl Pts',(-0.302891613247663,2.21008249254088,
12.4927483333191));
#38080=CARTESIAN_POINT('Ctrl Pts',(-0.30256304839729,2.21098170397983,12.49268966222));
#38081=CARTESIAN_POINT('Ctrl Pts',(-0.302424529723917,2.21135861301506,
12.4926650295648));
#38082=CARTESIAN_POINT('Ctrl Pts',(-0.302158550878916,2.21207818440519,
12.4926179248569));
#38083=CARTESIAN_POINT('Ctrl Pts',(-0.302031211250172,2.2124208909316,12.4925954568629));
#38084=CARTESIAN_POINT('Ctrl Pts',(-0.30173242725774,2.21322083033487,12.4925429334093));
#38085=CARTESIAN_POINT('Ctrl Pts',(-0.301560526636234,2.21367789077588,
12.4925128627138));
#38086=CARTESIAN_POINT('Ctrl Pts',(-0.300966146598159,2.21524743090018,
12.4924093912459));
#38087=CARTESIAN_POINT('Ctrl Pts',(-0.300538548479867,2.21635795006759,
12.492335819011));
#38088=CARTESIAN_POINT('Ctrl Pts',(-0.295864224466337,2.22830001311935,
12.491540699915));
#38089=CARTESIAN_POINT('Ctrl Pts',(-0.291040592977938,2.23889510499578,
12.4907996357478));
#38090=CARTESIAN_POINT('Ctrl Pts',(-0.275061774079559,2.2694867432541,12.4885488944374));
#38091=CARTESIAN_POINT('Ctrl Pts',(-0.262339239984499,2.28858055893766,
12.4869902824885));
#38092=CARTESIAN_POINT('Ctrl Pts',(-0.243632780222619,2.31105630630737,
12.4850189630426));
#38093=CARTESIAN_POINT('Ctrl Pts',(-0.239416423400156,2.31582742674833,
12.4845919886044));
#38094=CARTESIAN_POINT('Ctrl Pts',(-0.229124665998932,2.32680028979355,
12.4835947001165));
#38095=CARTESIAN_POINT('Ctrl Pts',(-0.222934096261984,2.33288817645456,
12.4830289971766));
#38096=CARTESIAN_POINT('Ctrl Pts',(-0.215508708151894,2.33962257899729,
12.4823959998899));
#38097=CARTESIAN_POINT('Ctrl Pts',(-0.214507033841069,2.3405196795231,12.4823115224198));
#38098=CARTESIAN_POINT('Ctrl Pts',(-0.213281847524685,2.34160321554687,
12.4822093312029));
#38099=CARTESIAN_POINT('Ctrl Pts',(-0.213063679794022,2.34179563395634,
12.4821911775951));
#38100=CARTESIAN_POINT('Ctrl Pts',(-0.212680939456152,2.34213228100004,
12.4821594065718));
#38101=CARTESIAN_POINT('Ctrl Pts',(-0.212516480358375,2.34227663751795,
12.4821457796296));
#38102=CARTESIAN_POINT('Ctrl Pts',(-0.212195998997101,2.34255736759563,
12.4821192730835));
#38103=CARTESIAN_POINT('Ctrl Pts',(-0.212039991817014,2.34269375854451,
12.4821063921715));
#38104=CARTESIAN_POINT('Ctrl Pts',(-0.211729254575457,2.34296489556985,
12.4820807801458));
#38105=CARTESIAN_POINT('Ctrl Pts',(-0.211574527559349,2.34309964420167,
12.4820680488256));
#38106=CARTESIAN_POINT('Ctrl Pts',(-0.211209237752952,2.34341715480014,
12.4820380429911));
#38107=CARTESIAN_POINT('Ctrl Pts',(-0.210998565859277,2.34359979180998,
12.4820207778431));
#38108=CARTESIAN_POINT('Ctrl Pts',(-0.210374074214234,2.34413976213594,
12.4819697163317));
#38109=CARTESIAN_POINT('Ctrl Pts',(-0.2099595792029,2.3444963183129,12.4819359773638));
#38110=CARTESIAN_POINT('Ctrl Pts',(-0.206257636224627,2.34766444091444,
12.4816359798046));
#38111=CARTESIAN_POINT('Ctrl Pts',(-0.20291460438456,2.35041077369261,12.4813744047309));
#38112=CARTESIAN_POINT('Ctrl Pts',(-0.199342750985433,2.35322656365423,
12.4811033563741));
#38113=CARTESIAN_POINT('Ctrl Pts',(-0.199168264649428,2.35336382391263,
12.4810901363439));
#38114=CARTESIAN_POINT('Ctrl Pts',(-0.198876360551659,2.35359296336294,
12.4810680545548));
#38115=CARTESIAN_POINT('Ctrl Pts',(-0.198759020869685,2.35368494136734,
12.4810591873984));
#38116=CARTESIAN_POINT('Ctrl Pts',(-0.196494501763941,2.35545747404113,
12.4808882397285));
#38117=CARTESIAN_POINT('Ctrl Pts',(-0.194326080410058,2.35711084304287,
12.4807276329801));
#38118=CARTESIAN_POINT('Ctrl Pts',(-0.18797264894187,2.3618288796417,12.4802650956061));
#38119=CARTESIAN_POINT('Ctrl Pts',(-0.183734199615987,2.3648203679699,12.4799664510617));
#38120=CARTESIAN_POINT('Ctrl Pts',(-0.168619979991341,2.37495031770507,
12.4789289373896));
#38121=CARTESIAN_POINT('Ctrl Pts',(-0.157385817704502,2.38153171016061,
12.4782057642214));
#38122=CARTESIAN_POINT('Ctrl Pts',(-0.13280015327219,2.39400213602806,12.4766636875476));
#38123=CARTESIAN_POINT('Ctrl Pts',(-0.119385368028905,2.39970022859808,
12.4758451034907));
#38124=CARTESIAN_POINT('Ctrl Pts',(-0.0975152182488424,2.40728776891555,
12.474501508541));
#38125=CARTESIAN_POINT('Ctrl Pts',(-0.089289508312883,2.40977791272939,
12.4739944467603));
#38126=CARTESIAN_POINT('Ctrl Pts',(-0.0793419929761372,2.41236015899325,
12.4733749100982));
#38127=CARTESIAN_POINT('Ctrl Pts',(-0.0777060693319513,2.41277114220925,
12.4732728270014));
#38128=CARTESIAN_POINT('Ctrl Pts',(-0.0748484897124004,2.41346523192363,
12.4730941345731));
#38129=CARTESIAN_POINT('Ctrl Pts',(-0.0736282578422544,2.41375408780568,
12.4730177108634));
#38130=CARTESIAN_POINT('Ctrl Pts',(-0.0718751972222612,2.41415828623365,
12.4729077347383));
#38131=CARTESIAN_POINT('Ctrl Pts',(-0.0713437025634769,2.41427941212203,
12.4728743682547));
#38132=CARTESIAN_POINT('Ctrl Pts',(-0.0704220533971347,2.41448699450864,
12.4728164662337));
#38133=CARTESIAN_POINT('Ctrl Pts',(-0.0700320395028736,2.41457407515638,
12.4727919507851));
#38134=CARTESIAN_POINT('Ctrl Pts',(-0.0692826901099888,2.41473992406874,
12.4727448227742));
#38135=CARTESIAN_POINT('Ctrl Pts',(-0.0689233794986877,2.41481880297786,
12.4727222138016));
#38136=CARTESIAN_POINT('Ctrl Pts',(-0.0680779000958508,2.41500289296054,
12.4726689867348));
#38137=CARTESIAN_POINT('Ctrl Pts',(-0.0675916222496276,2.41510759377109,
12.4726383523395));
#38138=CARTESIAN_POINT('Ctrl Pts',(-0.0661583709685047,2.41541271772961,
12.47254799839));
#38139=CARTESIAN_POINT('Ctrl Pts',(-0.0652107409874402,2.41560999949604,
12.4724881784425));
#38140=CARTESIAN_POINT('Ctrl Pts',(-0.0569343896900057,2.41729414087804,
12.4719650063401));
#38141=CARTESIAN_POINT('Ctrl Pts',(-0.0495574007219953,2.41852966194042,
12.4714936802498));
#38142=CARTESIAN_POINT('Ctrl Pts',(-0.0186826131266899,2.42260219662153,
12.469497956932));
#38143=CARTESIAN_POINT('Ctrl Pts',(0.00504550425815098,2.42310279770829,
12.4679016658535));
#38144=CARTESIAN_POINT('Ctrl Pts',(0.0415061952087167,2.41985315812628,
12.4654252927583));
#38145=CARTESIAN_POINT('Ctrl Pts',(0.0543222232273812,2.41792758160035,
12.4645520674005));
#38146=CARTESIAN_POINT('Ctrl Pts',(0.0705689334140489,2.41447511945697,
12.4634654619567));
#38147=CARTESIAN_POINT('Ctrl Pts',(0.074136451731667,2.4136532544204,12.4632281838213));
#38148=CARTESIAN_POINT('Ctrl Pts',(0.0797086102165182,2.41226918209775,
12.4628604486367));
#38149=CARTESIAN_POINT('Ctrl Pts',(0.0817230325195258,2.41174805709163,
12.4627281013187));
#38150=CARTESIAN_POINT('Ctrl Pts',(0.0845583286985679,2.41098520277602,
12.4625427996151));
#38151=CARTESIAN_POINT('Ctrl Pts',(0.0853834549580555,2.4107596707358,12.4624889905468));
#38152=CARTESIAN_POINT('Ctrl Pts',(0.0868115907755423,2.41036320036786,
12.4623960726099));
#38153=CARTESIAN_POINT('Ctrl Pts',(0.0874150129769259,2.41019378452422,
12.4623568792882));
#38154=CARTESIAN_POINT('Ctrl Pts',(0.0883028957406706,2.40994170737687,
12.4622993121272));
#38155=CARTESIAN_POINT('Ctrl Pts',(0.0885877380825749,2.40986041378495,
12.4622808595028));
#38156=CARTESIAN_POINT('Ctrl Pts',(0.0890860327096472,2.40971745795855,
12.4622486067419));
#38157=CARTESIAN_POINT('Ctrl Pts',(0.0892995337620247,2.4096559675823,12.4622347965273));
#38158=CARTESIAN_POINT('Ctrl Pts',(0.0897121036771894,2.40953668126229,
12.4622081270728));
#38159=CARTESIAN_POINT('Ctrl Pts',(0.0899111798673848,2.40947891419049,
12.462195266163));
#38160=CARTESIAN_POINT('Ctrl Pts',(0.090385693998628,2.40934072521842,12.4621646295082));
#38161=CARTESIAN_POINT('Ctrl Pts',(0.0906610811077255,2.40926012729114,
12.4621468641018));
#38162=CARTESIAN_POINT('Ctrl Pts',(0.0916404506219502,2.40897207327173,
12.4620837356401));
#38163=CARTESIAN_POINT('Ctrl Pts',(0.0923438384569645,2.40876257832882,
12.4620384908834));
#38164=CARTESIAN_POINT('Ctrl Pts',(0.102784348805078,2.40561413905456,12.4613682345227));
#38165=CARTESIAN_POINT('Ctrl Pts',(0.112378875572752,2.40221790261043,12.4607693152175));
#38166=CARTESIAN_POINT('Ctrl Pts',(0.143209097334117,2.38963282032531,12.458852532942));
#38167=CARTESIAN_POINT('Ctrl Pts',(0.163618345664013,2.37861294966487,12.4575916325838));
#38168=CARTESIAN_POINT('Ctrl Pts',(0.196750278942803,2.35581727309351,12.4553100454899));
#38169=CARTESIAN_POINT('Ctrl Pts',(0.210032812175859,2.3450290576798,12.4543172764806));
#38170=CARTESIAN_POINT('Ctrl Pts',(0.223246425643824,2.33242974796044,12.4532072132991));
#38171=CARTESIAN_POINT('Ctrl Pts',(0.224091763809188,2.33161484329695,12.4531356258133));
#38172=CARTESIAN_POINT('Ctrl Pts',(0.225312649999349,2.33042497038078,12.4530313925262));
#38173=CARTESIAN_POINT('Ctrl Pts',(0.225691761636345,2.33005365884696,12.452998906682));
#38174=CARTESIAN_POINT('Ctrl Pts',(0.226353001772631,2.32940281590998,12.452942035723));
#38175=CARTESIAN_POINT('Ctrl Pts',(0.226635534617074,2.32912369542555,12.4529176687143));
#38176=CARTESIAN_POINT('Ctrl Pts',(0.227181326279846,2.32858249846448,12.4528704660266));
#38177=CARTESIAN_POINT('Ctrl Pts',(0.227444649490961,2.32832048754037,12.4528476332635));
#38178=CARTESIAN_POINT('Ctrl Pts',(0.228069422328669,2.32769667492192,12.4527933176231));
#38179=CARTESIAN_POINT('Ctrl Pts',(0.228430464078042,2.32733446779604,12.452761816776));
#38180=CARTESIAN_POINT('Ctrl Pts',(0.229704395509317,2.32605032546645,12.4526502640619));
#38181=CARTESIAN_POINT('Ctrl Pts',(0.230612569078438,2.32512374788962,12.4525700052067));
#38182=CARTESIAN_POINT('Ctrl Pts',(0.245623124152832,2.30962286183139,12.4512310856986));
#38183=CARTESIAN_POINT('Ctrl Pts',(0.258321717526134,2.29375776996131,12.449910934293));
#38184=CARTESIAN_POINT('Ctrl Pts',(0.284978085243346,2.25313513107307,12.4466567642006));
#38185=CARTESIAN_POINT('Ctrl Pts',(0.297324711375373,2.22751857426121,12.4446957041301));
#38186=CARTESIAN_POINT('Ctrl Pts',(0.306588638485943,2.19932985946696,12.4428106627899));
#38187=CARTESIAN_POINT('Ctrl Pts',(0.307003857071948,2.19803900306387,12.4427249369398));
#38188=CARTESIAN_POINT('Ctrl Pts',(0.307687621994381,2.19586632606344,12.4425816945084));
#38189=CARTESIAN_POINT('Ctrl Pts',(0.307960550560082,2.19498591763744,12.4425239369798));
#38190=CARTESIAN_POINT('Ctrl Pts',(0.308328608240422,2.19378038012545,12.4424452534898));
#38191=CARTESIAN_POINT('Ctrl Pts',(0.308427004144702,2.19345626502695,12.4424241388146));
#38192=CARTESIAN_POINT('Ctrl Pts',(0.308583865830456,2.19293661831519,12.4423903505375));
#38193=CARTESIAN_POINT('Ctrl Pts',(0.308642656847939,2.19274118636902,12.4423776578203));
#38194=CARTESIAN_POINT('Ctrl Pts',(0.308764860524416,2.19233355608487,12.4423512140617));
#38195=CARTESIAN_POINT('Ctrl Pts',(0.308828239955441,2.19212134866684,12.4423374650717));
#38196=CARTESIAN_POINT('Ctrl Pts',(0.308974925122138,2.19162836376462,12.4423055643036));
#38197=CARTESIAN_POINT('Ctrl Pts',(0.309058067190835,2.19134753694711,12.4422874221764));
#38198=CARTESIAN_POINT('Ctrl Pts',(0.309326623957569,2.19043587597952,12.4422286227424));
#38199=CARTESIAN_POINT('Ctrl Pts',(0.309510492462696,2.18980458243663,12.4421880555103));
#38200=CARTESIAN_POINT('Ctrl Pts',(0.31129414499497,2.18361004602388,12.4417914142068));
#38201=CARTESIAN_POINT('Ctrl Pts',(0.312745817945078,2.1780047950456,12.4414437396001));
#38202=CARTESIAN_POINT('Ctrl Pts',(0.320479924283225,2.14443983202386,12.4394116308283));
#38203=CARTESIAN_POINT('Ctrl Pts',(0.323161959155335,2.11578050504518,12.4378701329498));
#38204=CARTESIAN_POINT('Ctrl Pts',(0.321377099112435,2.07108185415861,12.4353249612468));
#38205=CARTESIAN_POINT('Ctrl Pts',(0.319535478305687,2.05509491381871,12.434388354495));
#38206=CARTESIAN_POINT('Ctrl Pts',(0.316286256584576,2.03814867899337,12.4333393448164));
#38207=CARTESIAN_POINT('Ctrl Pts',(0.316056516197759,2.03698523566139,12.433267045383));
#38208=CARTESIAN_POINT('Ctrl Pts',(0.315714256426155,2.03530094422519,12.4331619645296));
#38209=CARTESIAN_POINT('Ctrl Pts',(0.315606856684791,2.03477905599402,12.4331293467709));
#38210=CARTESIAN_POINT('Ctrl Pts',(0.315417073123507,2.0338682857997,12.4330723222247));
#38211=CARTESIAN_POINT('Ctrl Pts',(0.315335262907165,2.03347928438561,12.4330479338382));
#38212=CARTESIAN_POINT('Ctrl Pts',(0.315175731403202,2.03272763185277,12.433000745886));
#38213=CARTESIAN_POINT('Ctrl Pts',(0.315098103343966,2.03236496138148,12.4329779493404));
#38214=CARTESIAN_POINT('Ctrl Pts',(0.314912415842221,2.03150470643102,12.432923807928));
#38215=CARTESIAN_POINT('Ctrl Pts',(0.314803803104114,2.03100724357499,12.4328924453605));
#38216=CARTESIAN_POINT('Ctrl Pts',(0.314417092773972,2.02925597720847,12.4327818449955));
#38217=CARTESIAN_POINT('Ctrl Pts',(0.31413268268596,2.0280035932764,12.4327024048208));
#38218=CARTESIAN_POINT('Ctrl Pts',(0.30971062648175,2.00905645776845,12.4314952245629));
#38219=CARTESIAN_POINT('Ctrl Pts',(0.304091886191966,1.99174418950717,12.4303186304509));
#38220=CARTESIAN_POINT('Ctrl Pts',(0.290663614268348,1.95983373276787,12.428011793656));
#38221=CARTESIAN_POINT('Ctrl Pts',(0.283129557936342,1.94517904450121,12.4268915142553));
#38222=CARTESIAN_POINT('Ctrl Pts',(0.266491842701544,1.91812771905889,12.424751469655));
#38223=CARTESIAN_POINT('Ctrl Pts',(0.25755390985221,1.90567671745366,12.4237332386531));
#38224=CARTESIAN_POINT('Ctrl Pts',(0.247362680939358,1.89342489802427,12.4227309828571));
#38225=CARTESIAN_POINT('Ctrl Pts',(0.246960347169611,1.89294407610735,12.4226916501911));
#38226=CARTESIAN_POINT('Ctrl Pts',(0.246236392167622,1.89208400239844,12.4226212998441));
#38227=CARTESIAN_POINT('Ctrl Pts',(0.245915292804973,1.89170431675404,12.4225902453808));
#38228=CARTESIAN_POINT('Ctrl Pts',(0.245423232877895,1.89112520165268,12.4225428850124));
#38229=CARTESIAN_POINT('Ctrl Pts',(0.245252906964426,1.89092523765994,12.4225265328323));
#38230=CARTESIAN_POINT('Ctrl Pts',(0.244954447611766,1.89057571056123,12.4224979521194));
#38231=CARTESIAN_POINT('Ctrl Pts',(0.244826421815556,1.89042605697884,12.422485715683));
#38232=CARTESIAN_POINT('Ctrl Pts',(0.24455809955657,1.89011298764975,12.4224601190365));
#38233=CARTESIAN_POINT('Ctrl Pts',(0.244417776896874,1.88994959569315,12.4224467608771));
#38234=CARTESIAN_POINT('Ctrl Pts',(0.244026715316692,1.88949516535379,12.4224096106649));
#38235=CARTESIAN_POINT('Ctrl Pts',(0.243775618600757,1.88920443321279,12.4223858451214));
#38236=CARTESIAN_POINT('Ctrl Pts',(0.242771979841304,1.88804656249271,12.4222912017266));
#38237=CARTESIAN_POINT('Ctrl Pts',(0.242015314317958,1.88718298565185,12.4222206256285));
#38238=CARTESIAN_POINT('Ctrl Pts',(0.228353229259573,1.87175764647997,12.4209598091936));
#38239=CARTESIAN_POINT('Ctrl Pts',(0.214157565312173,1.85838760035137,12.419862942759));
#38240=CARTESIAN_POINT('Ctrl Pts',(0.185954565646599,1.83627633873239,12.4178565601304));
#38241=CARTESIAN_POINT('Ctrl Pts',(0.172318068100565,1.82717088161644,12.4169476693011));
#38242=CARTESIAN_POINT('Ctrl Pts',(0.145963516883332,1.81234021676456,12.4152155501483));
#38243=CARTESIAN_POINT('Ctrl Pts',(0.133452758760993,1.80632707829239,12.414402548287));
#38244=CARTESIAN_POINT('Ctrl Pts',(0.119429354491756,1.80066843774786,12.4134836604013));
#38245=CARTESIAN_POINT('Ctrl Pts',(0.118261244617346,1.80020501534176,12.413407071664));
#38246=CARTESIAN_POINT('Ctrl Pts',(0.116582145275752,1.7995502093278,12.4132969001715));
#38247=CARTESIAN_POINT('Ctrl Pts',(0.116073323491315,1.79935326896843,12.4132635042679));
#38248=CARTESIAN_POINT('Ctrl Pts',(0.115190884527432,1.79901429351208,12.4132055675852));
#38249=CARTESIAN_POINT('Ctrl Pts',(0.114817497567415,1.79887165919118,12.4131810469619));
#38250=CARTESIAN_POINT('Ctrl Pts',(0.114100058219928,1.79859912477645,12.4131339205454));
#38251=CARTESIAN_POINT('Ctrl Pts',(0.113756046713933,1.79846911815605,12.4131113183636));
#38252=CARTESIAN_POINT('Ctrl Pts',(0.112946614506063,1.79816480507354,12.4130581248289));
#38253=CARTESIAN_POINT('Ctrl Pts',(0.112481012624485,1.79799098619539,12.413027517226));
#38254=CARTESIAN_POINT('Ctrl Pts',(0.111108983577949,1.79748239211648,12.4129372938686));
#38255=CARTESIAN_POINT('Ctrl Pts',(0.110201456668662,1.79715061791905,12.4128775781307));
#38256=CARTESIAN_POINT('Ctrl Pts',(0.102300268360973,1.79430231441866,12.4123573281569));
#38257=CARTESIAN_POINT('Ctrl Pts',(0.0952234886330571,1.7920245264706,12.4118889177847));
#38258=CARTESIAN_POINT('Ctrl Pts',(0.0841737473577247,1.78888522694789,
12.4111529321127));
#38259=CARTESIAN_POINT('Ctrl Pts',(0.080252315188744,1.78785070011569,12.4108908774919));
#38260=CARTESIAN_POINT('Ctrl Pts',(0.0496201198374673,1.78038487634848,
12.4088374199338));
#38261=CARTESIAN_POINT('Ctrl Pts',(0.0222067609649575,1.77731985982936,
12.4069482854065));
#38262=CARTESIAN_POINT('Ctrl Pts',(-0.0168461864125599,1.77795693509862,
12.4043402650436));
#38263=CARTESIAN_POINT('Ctrl Pts',(-0.0284186537932631,1.7787711457504,
12.4035799449124));
#38264=CARTESIAN_POINT('Ctrl Pts',(-0.0406630980736328,1.78029975942349,
12.4028054495856));
#38265=CARTESIAN_POINT('Ctrl Pts',(-0.0414025247065735,1.78039467722863,
12.4027587968817));
#38266=CARTESIAN_POINT('Ctrl Pts',(-0.0424506183693955,1.78053291599362,
12.4026928433818));
#38267=CARTESIAN_POINT('Ctrl Pts',(-0.0427595550149776,1.78057411936356,
12.4026734243439));
#38268=CARTESIAN_POINT('Ctrl Pts',(-0.0432902825347482,1.78064568708836,
12.4026401014833));
#38269=CARTESIAN_POINT('Ctrl Pts',(-0.0435121020223595,1.78067583443164,
12.4026261853172));
#38270=CARTESIAN_POINT('Ctrl Pts',(-0.043937048360315,1.78073403962603,
12.4025995474618));
#38271=CARTESIAN_POINT('Ctrl Pts',(-0.0441401795365313,1.78076206017579,
12.4025868236526));
#38272=CARTESIAN_POINT('Ctrl Pts',(-0.0446189727882375,1.78082857213866,
12.4025568549538));
#38273=CARTESIAN_POINT('Ctrl Pts',(-0.0448946125427213,1.78086722690749,
12.4025396193738));
#38274=CARTESIAN_POINT('Ctrl Pts',(-0.0457096991685293,1.78098260875728,
12.4024887027934));
#38275=CARTESIAN_POINT('Ctrl Pts',(-0.0462490053559496,1.78106034735832,
12.4024550787309));
#38276=CARTESIAN_POINT('Ctrl Pts',(-0.0510157849502292,1.78175980246951,
12.4021584405468));
#38277=CARTESIAN_POINT('Ctrl Pts',(-0.0552309486542478,1.78246420634107,
12.4018999953036));
#38278=CARTESIAN_POINT('Ctrl Pts',(-0.0596870585361504,1.78330030235255,
12.4016297022023));
#38279=CARTESIAN_POINT('Ctrl Pts',(-0.0599429604798284,1.7833486381895,
12.4016141903038));
#38280=CARTESIAN_POINT('Ctrl Pts',(-0.0603204949564488,1.78342042255194,
12.4015913202584));
#38281=CARTESIAN_POINT('Ctrl Pts',(-0.0604421723909528,1.7834436309822,
12.4015839516291));
#38282=CARTESIAN_POINT('Ctrl Pts',(-0.0614290730691154,1.78363245955405,
12.4015242043827));
#38283=CARTESIAN_POINT('Ctrl Pts',(-0.0622936358762339,1.78380155815278,
12.4014719769428));
#38284=CARTESIAN_POINT('Ctrl Pts',(-0.0883293179160923,1.78900476838662,
12.3999023136815));
#38285=CARTESIAN_POINT('Ctrl Pts',(-0.11281270690571,1.79702523189865,12.3985082595602));
#38286=CARTESIAN_POINT('Ctrl Pts',(-0.147102073554181,1.81299857443853,
12.3963745956976));
#38287=CARTESIAN_POINT('Ctrl Pts',(-0.157817272638603,1.81874831816142,
12.3956799637302));
#38288=CARTESIAN_POINT('Ctrl Pts',(-0.174608347743744,1.82902055400519,
12.3945223613654));
#38289=CARTESIAN_POINT('Ctrl Pts',(-0.18089472592584,1.83317605157413,12.394072135403));
#38290=CARTESIAN_POINT('Ctrl Pts',(-0.18782941374598,1.83811786611662,12.3935536718632));
#38291=CARTESIAN_POINT('Ctrl Pts',(-0.188626828305283,1.83869163747512,
12.3934937193264));
#38292=CARTESIAN_POINT('Ctrl Pts',(-0.18982073281737,1.83955901165978,12.3934034475937));
#38293=CARTESIAN_POINT('Ctrl Pts',(-0.190219197384165,1.83984989725697,
12.3933732336415));
#38294=CARTESIAN_POINT('Ctrl Pts',(-0.190903406482155,1.84035179339406,
12.3933212042604));
#38295=CARTESIAN_POINT('Ctrl Pts',(-0.191189473786501,1.84056236411855,
12.3932994059581));
#38296=CARTESIAN_POINT('Ctrl Pts',(-0.191777974666696,1.84099705454615,
12.3932544694453));
#38297=CARTESIAN_POINT('Ctrl Pts',(-0.192080364794332,1.84122123197673,
12.3932313290028));
#38298=CARTESIAN_POINT('Ctrl Pts',(-0.192807580535545,1.84176233150446,
12.3931755561862));
#38299=CARTESIAN_POINT('Ctrl Pts',(-0.193232017392648,1.84207977203989,
12.3931429035605));
#38300=CARTESIAN_POINT('Ctrl Pts',(-0.194783643135526,1.84324622811512,
12.3930231621745));
#38301=CARTESIAN_POINT('Ctrl Pts',(-0.19590602259413,1.84410158808627,12.3929358244279));
#38302=CARTESIAN_POINT('Ctrl Pts',(-0.215881062186123,1.85953290464592,
12.3913683610573));
#38303=CARTESIAN_POINT('Ctrl Pts',(-0.2330612849956,1.87614502260686,12.3898016482174));
#38304=CARTESIAN_POINT('Ctrl Pts',(-0.257863258200955,1.90610587732993,
12.3871792712474));
#38305=CARTESIAN_POINT('Ctrl Pts',(-0.266648866503839,1.91837735945161,
12.3861525365442));
#38306=CARTESIAN_POINT('Ctrl Pts',(-0.278769650686272,1.93809330566276,
12.3846094623814));
#38307=CARTESIAN_POINT('Ctrl Pts',(-0.282736560540412,1.94512471438944,
12.3840783999449));
#38308=CARTESIAN_POINT('Ctrl Pts',(-0.287984080354277,1.95530113757531,
12.38334385278));
#38309=CARTESIAN_POINT('Ctrl Pts',(-0.289485335073529,1.95832842788299,
12.383129471457));
#38310=CARTESIAN_POINT('Ctrl Pts',(-0.291162997825407,1.96184951658988,
12.3828853311461));
#38311=CARTESIAN_POINT('Ctrl Pts',(-0.291386081890458,1.96232066727819,
12.3828527697961));
#38312=CARTESIAN_POINT('Ctrl Pts',(-0.291722666349328,1.96303601177082,
12.3828034960315));
#38313=CARTESIAN_POINT('Ctrl Pts',(-0.291837004147715,1.96327980710604,
12.3827867319244));
#38314=CARTESIAN_POINT('Ctrl Pts',(-0.292043367533353,1.96372126122609,
12.3827564286768));
#38315=CARTESIAN_POINT('Ctrl Pts',(-0.292135497806559,1.96391886947774,
12.3827428830503));
#38316=CARTESIAN_POINT('Ctrl Pts',(-0.292320340948617,1.9643163884191,12.3827156722394));
#38317=CARTESIAN_POINT('Ctrl Pts',(-0.292413048901168,1.96451629981072,
12.3827020073775));
#38318=CARTESIAN_POINT('Ctrl Pts',(-0.292677185669697,1.96508740686366,
12.3826630245014));
#38319=CARTESIAN_POINT('Ctrl Pts',(-0.292848114015169,1.96545883559131,
12.3826377375316));
#38320=CARTESIAN_POINT('Ctrl Pts',(-0.293578379517358,1.96705369379375,
12.3825294385826));
#38321=CARTESIAN_POINT('Ctrl Pts',(-0.294130770780488,1.96828031626675,
12.3824468491483));
#38322=CARTESIAN_POINT('Ctrl Pts',(-0.303997422645833,1.99056147924542,
12.3809587312885));
#38323=CARTESIAN_POINT('Ctrl Pts',(-0.31103842916825,2.01255469288941,12.379681987296));
#38324=CARTESIAN_POINT('Ctrl Pts',(-0.318730994436393,2.04997944678461,
12.3775463056297));
#38325=CARTESIAN_POINT('Ctrl Pts',(-0.320732575812288,2.06504179493686,
12.3766965896928));
#38326=CARTESIAN_POINT('Ctrl Pts',(-0.322069846210219,2.08675385496259,
12.3754388283474));
#38327=CARTESIAN_POINT('Ctrl Pts',(-0.322273096087557,2.09332994929834,
12.3750537678569));
#38328=CARTESIAN_POINT('Ctrl Pts',(-0.322276461705378,2.1050389730816,12.3743576554723));
#38329=CARTESIAN_POINT('Ctrl Pts',(-0.32215537060393,2.11016964417602,12.3740490550513));
#38330=CARTESIAN_POINT('Ctrl Pts',(-0.321870831240938,2.11615829627295,
12.373683958331));
#38331=CARTESIAN_POINT('Ctrl Pts',(-0.321826342566203,2.11702139094832,
12.3736312216135));
#38332=CARTESIAN_POINT('Ctrl Pts',(-0.321749710133317,2.11840017986138,
12.3735467821712));
#38333=CARTESIAN_POINT('Ctrl Pts',(-0.321719796728216,2.11891599793951,
12.3735151494289));
#38334=CARTESIAN_POINT('Ctrl Pts',(-0.321664744458097,2.11982737749388,
12.3734591816648));
#38335=CARTESIAN_POINT('Ctrl Pts',(-0.321640116001363,2.12022296966275,
12.3734348627071));
#38336=CARTESIAN_POINT('Ctrl Pts',(-0.321587614932111,2.12104189961484,
12.373384465578));
#38337=CARTESIAN_POINT('Ctrl Pts',(-0.321559636043543,2.12146522960347,
12.373358384116));
#38338=CARTESIAN_POINT('Ctrl Pts',(-0.321485701802137,2.12255128555685,
12.3732913952818));
#38339=CARTESIAN_POINT('Ctrl Pts',(-0.321438533224841,2.12321392451062,
12.3732504498849));
#38340=CARTESIAN_POINT('Ctrl Pts',(-0.321236209336698,2.12593731295027,
12.3730818630893));
#38341=CARTESIAN_POINT('Ctrl Pts',(-0.321063285472976,2.12799665683,12.3729536647719));
#38342=CARTESIAN_POINT('Ctrl Pts',(-0.319781573546354,2.14168074161831,
12.3720968790595));
#38343=CARTESIAN_POINT('Ctrl Pts',(-0.318061596280838,2.15323818446407,
12.3713491044441));
#38344=CARTESIAN_POINT('Ctrl Pts',(-0.308959903202273,2.19766864721991,
12.368378481486));
#38345=CARTESIAN_POINT('Ctrl Pts',(-0.297073256600571,2.22939244412999,
12.3660239643655));
#38346=CARTESIAN_POINT('Ctrl Pts',(-0.278475297815029,2.26226356671525,
12.3635881606904));
#38347=CARTESIAN_POINT('Ctrl Pts',(-0.27639016025259,2.26579034890125,12.3633272734452));
#38348=CARTESIAN_POINT('Ctrl Pts',(-0.273955425703913,2.26973476436015,
12.3630368396401));
#38349=CARTESIAN_POINT('Ctrl Pts',(-0.273671475562494,2.27019221186175,
12.3630031778772));
#38350=CARTESIAN_POINT('Ctrl Pts',(-0.273239876536263,2.27088365060094,
12.3629523318112));
#38351=CARTESIAN_POINT('Ctrl Pts',(-0.273093072271738,2.27111816400035,
12.3629350924626));
#38352=CARTESIAN_POINT('Ctrl Pts',(-0.272837163323071,2.27152579925237,
12.3629051375315));
#38353=CARTESIAN_POINT('Ctrl Pts',(-0.27272819571163,2.27169900629816,12.3628924128735));
#38354=CARTESIAN_POINT('Ctrl Pts',(-0.272499476948899,2.2720617940404,12.3628657679937));
#38355=CARTESIAN_POINT('Ctrl Pts',(-0.272379692942661,2.27225135348857,
12.3628518500565));
#38356=CARTESIAN_POINT('Ctrl Pts',(-0.272091874502325,2.27270577825777,
12.3628184947943));
#38357=CARTESIAN_POINT('Ctrl Pts',(-0.27192365043759,2.27297052450779,12.3627990701009));
#38358=CARTESIAN_POINT('Ctrl Pts',(-0.271347965626978,2.27387360543697,
12.3627328358612));
#38359=CARTESIAN_POINT('Ctrl Pts',(-0.270938637579908,2.27451075557445,
12.3626861495704));
#38360=CARTESIAN_POINT('Ctrl Pts',(-0.263550196199281,2.28592276637011,
12.3618506281738));
#38361=CARTESIAN_POINT('Ctrl Pts',(-0.255934672004761,2.29627407750246,
12.3611034909171));
#38362=CARTESIAN_POINT('Ctrl Pts',(-0.227817783086908,2.33006171692015,
12.3586011541544));
#38363=CARTESIAN_POINT('Ctrl Pts',(-0.20455732329365,2.35096956232152,12.3569210539585));
#38364=CARTESIAN_POINT('Ctrl Pts',(-0.173124994607485,2.37190649017438,
12.3546922815772));
#38365=CARTESIAN_POINT('Ctrl Pts',(-0.167477629447395,2.3754208363688,12.3542941209579));
#38366=CARTESIAN_POINT('Ctrl Pts',(-0.160826570176197,2.37927955699399,
12.3538261519073));
#38367=CARTESIAN_POINT('Ctrl Pts',(-0.159924739146724,2.37979695208943,
12.3537627200538));
#38368=CARTESIAN_POINT('Ctrl Pts',(-0.158581285565393,2.38055909609915,
12.3536682511151));
#38369=CARTESIAN_POINT('Ctrl Pts',(-0.158141559866103,2.38080718932049,
12.3536373344888));
#38370=CARTESIAN_POINT('Ctrl Pts',(-0.157358158821926,2.38124676043204,
12.3535822607654));
#38371=CARTESIAN_POINT('Ctrl Pts',(-0.157014711674405,2.38143864467583,
12.3535581183145));
#38372=CARTESIAN_POINT('Ctrl Pts',(-0.156291808879971,2.38184079602012,
12.3535073063399));
#38373=CARTESIAN_POINT('Ctrl Pts',(-0.155912278559379,2.38205092663511,
12.353480631991));
#38374=CARTESIAN_POINT('Ctrl Pts',(-0.154912926458348,2.38260159409755,
12.3534104006092));
#38375=CARTESIAN_POINT('Ctrl Pts',(-0.154292408544179,2.38294085675854,
12.3533667981793));
#38376=CARTESIAN_POINT('Ctrl Pts',(-0.151519091321392,2.3844453072291,12.3531719439067));
#38377=CARTESIAN_POINT('Ctrl Pts',(-0.149354220142093,2.38558796234007,
12.3530198937103));
#38378=CARTESIAN_POINT('Ctrl Pts',(-0.133460614693063,2.39374673162533,
12.3519037430355));
#38379=CARTESIAN_POINT('Ctrl Pts',(-0.119259160883542,2.39979327276105,
12.3509057154518));
#38380=CARTESIAN_POINT('Ctrl Pts',(-0.0883844415753198,2.41039697703056,
12.3487381981583));
#38381=CARTESIAN_POINT('Ctrl Pts',(-0.0716654959918706,2.41467775159411,
12.3475654738115));
#38382=CARTESIAN_POINT('Ctrl Pts',(-0.0390890883744199,2.42028688794024,
12.3453362534991));
#38383=CARTESIAN_POINT('Ctrl Pts',(-0.0233134248564113,2.42182023995543,
12.3442815894348));
#38384=CARTESIAN_POINT('Ctrl Pts',(-0.00658607211306412,2.42220895644832,
12.3432294321605));
#38385=CARTESIAN_POINT('Ctrl Pts',(-0.00568492162010916,2.42222611575352,
12.3431729545758));
#38386=CARTESIAN_POINT('Ctrl Pts',(-0.00447100000889573,2.42224413661959,
12.3430971618197));
#38387=CARTESIAN_POINT('Ctrl Pts',(-0.00415829349260601,2.42224832353952,
12.3430776632413));
#38388=CARTESIAN_POINT('Ctrl Pts',(-0.00363125913339092,2.42225461287934,
12.3430448442142));
#38389=CARTESIAN_POINT('Ctrl Pts',(-0.00341693525146551,2.42225695666504,
12.3430315102305));
#38390=CARTESIAN_POINT('Ctrl Pts',(-0.00300543908141589,2.42226104611096,
12.3430059329806));
#38391=CARTESIAN_POINT('Ctrl Pts',(-0.00280826898654971,2.42226282461703,
12.3429936879865));
#38392=CARTESIAN_POINT('Ctrl Pts',(-0.00234093621502636,2.42226661110576,
12.3429646895244));
#38393=CARTESIAN_POINT('Ctrl Pts',(-0.00207077286777499,2.42226846031991,
12.3429479451057));
#38394=CARTESIAN_POINT('Ctrl Pts',(-0.00127503832141977,2.42227290629625,
12.3428986829334));
#38395=CARTESIAN_POINT('Ctrl Pts',(-0.000749459525098847,2.42227455713259,
12.3428662181729));
#38396=CARTESIAN_POINT('Ctrl Pts',(0.00326785903834728,2.42227734784248,
12.3426186097039));
#38397=CARTESIAN_POINT('Ctrl Pts',(0.00675957556747228,2.42222302585975,
12.3424065116362));
#38398=CARTESIAN_POINT('Ctrl Pts',(0.0188651441933347,2.42183781586057,
12.3416798627528));
#38399=CARTESIAN_POINT('Ctrl Pts',(0.0274666734445083,2.4212181189898,12.3411787685483));
#38400=CARTESIAN_POINT('Ctrl Pts',(0.0718192360720136,2.41622775382,12.3386274515187));
#38401=CARTESIAN_POINT('Ctrl Pts',(0.106674869151872,2.40623302521987,12.3366996135462));
#38402=CARTESIAN_POINT('Ctrl Pts',(0.139751374585636,2.39039827991158,12.3344977435956));
#38403=CARTESIAN_POINT('Ctrl Pts',(0.140343369906351,2.39011264396422,12.3344582166111));
#38404=CARTESIAN_POINT('Ctrl Pts',(0.143333897636095,2.38865842783097,12.3342579352018));
#38405=CARTESIAN_POINT('Ctrl Pts',(0.145718671783204,2.38746193174845,12.3340962424619));
#38406=CARTESIAN_POINT('Ctrl Pts',(0.148758020935467,2.38588948123213,12.333887515734));
#38407=CARTESIAN_POINT('Ctrl Pts',(0.149426557726388,2.38554062425975,12.333841437929));
#38408=CARTESIAN_POINT('Ctrl Pts',(0.150490887341073,2.38498047256803,12.3337678128664));
#38409=CARTESIAN_POINT('Ctrl Pts',(0.150887476772373,2.38477069067558,12.3337403192061));
#38410=CARTESIAN_POINT('Ctrl Pts',(0.151628943197061,2.38437649719668,12.3336888047028));
#38411=CARTESIAN_POINT('Ctrl Pts',(0.151973925452723,2.38419228447172,12.3336647909542));
#38412=CARTESIAN_POINT('Ctrl Pts',(0.152734150101069,2.38378456159807,12.3336117716826));
#38413=CARTESIAN_POINT('Ctrl Pts',(0.153149238382994,2.38356076736291,12.3335827560863));
#38414=CARTESIAN_POINT('Ctrl Pts',(0.154345502208729,2.38291241058491,12.3334989410395));
#38415=CARTESIAN_POINT('Ctrl Pts',(0.155125409331093,2.38248552789397,12.3334440588869));
#38416=CARTESIAN_POINT('Ctrl Pts',(0.156878872580975,2.38151631726688,12.3333201238913));
#38417=CARTESIAN_POINT('Ctrl Pts',(0.15785139845159,2.38097215788493,12.3332510057651));
#38418=CARTESIAN_POINT('Ctrl Pts',(0.165923145325354,2.3764006226304,12.3326741410611));
#38419=CARTESIAN_POINT('Ctrl Pts',(0.172869272585666,2.3721102524518,12.3321569242951));
#38420=CARTESIAN_POINT('Ctrl Pts',(0.186104822008574,2.36322370498861,12.3311288096778));
#38421=CARTESIAN_POINT('Ctrl Pts',(0.192405396613111,2.3586539627675,12.3306190863669));
#38422=CARTESIAN_POINT('Ctrl Pts',(0.216913149678283,2.33948747143721,12.3285560766956));
#38423=CARTESIAN_POINT('Ctrl Pts',(0.23367538902042,2.32316196148891,12.3269532314582));
#38424=CARTESIAN_POINT('Ctrl Pts',(0.255162546005965,2.29713411745301,12.3247079394858));
#38425=CARTESIAN_POINT('Ctrl Pts',(0.261404353680891,2.28877923655543,12.3240271832591));
#38426=CARTESIAN_POINT('Ctrl Pts',(0.26764303197325,2.27952416771744,12.3233265712654));
#38427=CARTESIAN_POINT('Ctrl Pts',(0.268053097212222,2.2789113089181,12.3232804200175));
#38428=CARTESIAN_POINT('Ctrl Pts',(0.268620131858981,2.27805752737708,12.3232164683218));
#38429=CARTESIAN_POINT('Ctrl Pts',(0.26877888374771,2.27781779986406,12.3231985491066));
#38430=CARTESIAN_POINT('Ctrl Pts',(0.26905161903196,2.27740474896056,12.3231677389522));
#38431=CARTESIAN_POINT('Ctrl Pts',(0.269165755925846,2.27723152793705,12.3231548376485));
#38432=CARTESIAN_POINT('Ctrl Pts',(0.269401736500291,2.27687263585666,12.323128148415));
#38433=CARTESIAN_POINT('Ctrl Pts',(0.269523555304116,2.27668694937862,12.3231143622353));
#38434=CARTESIAN_POINT('Ctrl Pts',(0.269810422084073,2.27624869585435,12.3230818771019));
#38435=CARTESIAN_POINT('Ctrl Pts',(0.269975308030901,2.27599602186112,12.3230631891056));
#38436=CARTESIAN_POINT('Ctrl Pts',(0.27049929600999,2.27519058474166,12.3230037481725));
#38437=CARTESIAN_POINT('Ctrl Pts',(0.270857060027102,2.27463694676547,12.3229630844526));
#38438=CARTESIAN_POINT('Ctrl Pts',(0.275594818122077,2.26725570895044,12.3224234743239));
#38439=CARTESIAN_POINT('Ctrl Pts',(0.279717654045023,2.26026551744576,12.3219411581942));
#38440=CARTESIAN_POINT('Ctrl Pts',(0.287302177045821,2.24621985476806,12.3210122207659));
#38441=CARTESIAN_POINT('Ctrl Pts',(0.29077833374161,2.23917887879653,12.3205652549226));
#38442=CARTESIAN_POINT('Ctrl Pts',(0.304150427732204,2.20940016272012,12.3187240484361));
#38443=CARTESIAN_POINT('Ctrl Pts',(0.311662495319964,2.1856874934315,12.3173667496005));
#38444=CARTESIAN_POINT('Ctrl Pts',(0.318242538080686,2.15175313277524,12.3153552292708));
#38445=CARTESIAN_POINT('Ctrl Pts',(0.31966544401802,2.14207938440594,12.3147753200863));
#38446=CARTESIAN_POINT('Ctrl Pts',(0.320750987375719,2.13132189719268,12.3141178572602));
#38447=CARTESIAN_POINT('Ctrl Pts',(0.320850390211302,2.1302867001808,12.3140544637939));
#38448=CARTESIAN_POINT('Ctrl Pts',(0.320991589559972,2.1287374499988,12.3139593968405));
#38449=CARTESIAN_POINT('Ctrl Pts',(0.321037166119318,2.12822374117423,12.3139278421692));
#38450=CARTESIAN_POINT('Ctrl Pts',(0.321113546448796,2.12733870416159,12.3138734229338));
#38451=CARTESIAN_POINT('Ctrl Pts',(0.321144939784693,2.12696742677662,12.3138505769352));
#38452=CARTESIAN_POINT('Ctrl Pts',(0.321208411436013,2.12620094020098,12.3138033771844));
#38453=CARTESIAN_POINT('Ctrl Pts',(0.32124040439261,2.12580572471652,12.3137790207896));
#38454=CARTESIAN_POINT('Ctrl Pts',(0.321312358587386,2.12489598711545,12.3137229105413));
#38455=CARTESIAN_POINT('Ctrl Pts',(0.321351813382894,2.12438142707116,12.3136911408363));
#38456=CARTESIAN_POINT('Ctrl Pts',(0.321471696455759,2.12276708153775,12.3135913640183));
#38457=CARTESIAN_POINT('Ctrl Pts',(0.321547715459162,2.12166698544912,12.3135232186595));
#38458=CARTESIAN_POINT('Ctrl Pts',(0.321710850975623,2.1191158828462,12.3133648291437));
#38459=CARTESIAN_POINT('Ctrl Pts',(0.321793798738509,2.11766464249429,12.3132744553582));
#38460=CARTESIAN_POINT('Ctrl Pts',(0.322515221507821,2.10334259081287,12.3123798281188));
#38461=CARTESIAN_POINT('Ctrl Pts',(0.322390911846858,2.090446631611,12.3115517077522));
#38462=CARTESIAN_POINT('Ctrl Pts',(0.320181833962088,2.05874934582598,12.3094606026357));
#38463=CARTESIAN_POINT('Ctrl Pts',(0.31721420442595,2.04005787319945,12.3081772277891));
#38464=CARTESIAN_POINT('Ctrl Pts',(0.309706361623461,2.01006766575015,12.3060891857521));
#38465=CARTESIAN_POINT('Ctrl Pts',(0.306134117098912,1.99857119530979,12.3052823131422));
#38466=CARTESIAN_POINT('Ctrl Pts',(0.301550693359492,1.98629197902112,12.3044304182303));
#38467=CARTESIAN_POINT('Ctrl Pts',(0.301169148885928,1.98528522972201,12.3043606502367));
#38468=CARTESIAN_POINT('Ctrl Pts',(0.299224737321257,1.98023124506068,12.3040108613566));
#38469=CARTESIAN_POINT('Ctrl Pts',(0.297585209461193,1.97621370920541,12.3037342692817));
#38470=CARTESIAN_POINT('Ctrl Pts',(0.295627082900686,1.97167945033083,12.3034247713452));
#38471=CARTESIAN_POINT('Ctrl Pts',(0.295387670153801,1.97112928980316,12.3033872639484));
#38472=CARTESIAN_POINT('Ctrl Pts',(0.295031725050041,1.97031754614533,12.3033319934783));
#38473=CARTESIAN_POINT('Ctrl Pts',(0.294916379989371,1.97005544859725,12.3033141585056));
#38474=CARTESIAN_POINT('Ctrl Pts',(0.294711630388784,1.969591874779,12.3032826333765));
#38475=CARTESIAN_POINT('Ctrl Pts',(0.294622368380299,1.969390336264,12.3032689344561));
#38476=CARTESIAN_POINT('Ctrl Pts',(0.294435383065221,1.96896932213148,12.3032403313998));
#38477=CARTESIAN_POINT('Ctrl Pts',(0.294337621315708,1.96874986467602,12.3032254297132));
#38478=CARTESIAN_POINT('Ctrl Pts',(0.294081105505361,1.96817576100857,12.30318646691));
#38479=CARTESIAN_POINT('Ctrl Pts',(0.293921954705788,1.96782129087247,12.3031624302255));
#38480=CARTESIAN_POINT('Ctrl Pts',(0.293266573671614,1.96636862394841,12.3030640041036));
#38481=CARTESIAN_POINT('Ctrl Pts',(0.292764818389349,1.9652729087392,12.3029899499804));
#38482=CARTESIAN_POINT('Ctrl Pts',(0.289433497539623,1.95810458546837,12.302506539083));
#38483=CARTESIAN_POINT('Ctrl Pts',(0.286421083364148,1.95211816935647,12.3021078400876));
#38484=CARTESIAN_POINT('Ctrl Pts',(0.279790509090775,1.93990556451551,12.3012961121901));
#38485=CARTESIAN_POINT('Ctrl Pts',(0.276146000741318,1.93369800260942,12.3008844282648));
#38486=CARTESIAN_POINT('Ctrl Pts',(0.261866043913477,1.91114130508282,12.2993730652622));
#38487=CARTESIAN_POINT('Ctrl Pts',(0.249961758877574,1.89564596255504,12.2983012611015));
#38488=CARTESIAN_POINT('Ctrl Pts',(0.233222372681876,1.87752479522032,12.2968987906593));
#38489=CARTESIAN_POINT('Ctrl Pts',(0.229624393963316,1.87381307177378,12.2966027559472));
#38490=CARTESIAN_POINT('Ctrl Pts',(0.223433738157265,1.86772670962211,12.2961004177346));
#38491=CARTESIAN_POINT('Ctrl Pts',(0.220888623953633,1.86530502480585,12.295895783679));
#38492=CARTESIAN_POINT('Ctrl Pts',(0.216994154326212,1.86171889403754,12.2955850208604));
#38493=CARTESIAN_POINT('Ctrl Pts',(0.215673855374263,1.86052320277745,12.295480064171));
#38494=CARTESIAN_POINT('Ctrl Pts',(0.214035704254371,1.85906419304752,12.2953502850332));
#38495=CARTESIAN_POINT('Ctrl Pts',(0.213727153566522,1.85879044464686,12.2953258599934));
#38496=CARTESIAN_POINT('Ctrl Pts',(0.213165611263555,1.85829416365103,12.2952814422058));
#38497=CARTESIAN_POINT('Ctrl Pts',(0.212912794274646,1.85807143371757,12.295261457017));
#38498=CARTESIAN_POINT('Ctrl Pts',(0.208572337142748,1.85425959569122,12.294918554917));
#38499=CARTESIAN_POINT('Ctrl Pts',(0.204395021423741,1.85077432725717,12.2945917241251));
#38500=CARTESIAN_POINT('Ctrl Pts',(0.199441583216768,1.84684983567982,12.2942069347975));
#38501=CARTESIAN_POINT('Ctrl Pts',(0.198749245222525,1.84630591589338,12.2941532147827));
#38502=CARTESIAN_POINT('Ctrl Pts',(0.197643333775411,1.84544438692515,12.2940674986986));
#38503=CARTESIAN_POINT('Ctrl Pts',(0.197231199929601,1.84512493000873,12.2940355760091));
#38504=CARTESIAN_POINT('Ctrl Pts',(0.196503813049271,1.84456393205277,12.2939792701984));
#38505=CARTESIAN_POINT('Ctrl Pts',(0.196188884664472,1.84432197027684,12.293954903771));
#38506=CARTESIAN_POINT('Ctrl Pts',(0.195538136832002,1.84382390620373,12.2939045781487));
#38507=CARTESIAN_POINT('Ctrl Pts',(0.195202259756554,1.84356788077216,12.2938786159918));
#38508=CARTESIAN_POINT('Ctrl Pts',(0.194354123655839,1.84292401303357,12.2938130898862));
#38509=CARTESIAN_POINT('Ctrl Pts',(0.193841207944696,1.8425370423735,12.293773491825));
#38510=CARTESIAN_POINT('Ctrl Pts',(0.19180392251793,1.84100954565989,12.2936163222143));
#38511=CARTESIAN_POINT('Ctrl Pts',(0.190270640570015,1.83988102103127,12.2934982834932));
#38512=CARTESIAN_POINT('Ctrl Pts',(0.186397567777461,1.8370829330404,12.293200694271));
#38513=CARTESIAN_POINT('Ctrl Pts',(0.184045308669641,1.83543099034943,12.2930204769172));
#38514=CARTESIAN_POINT('Ctrl Pts',(0.174556488715929,1.82895497121465,12.2922953860837));
#38515=CARTESIAN_POINT('Ctrl Pts',(0.167250415221558,1.8243867710029,12.2917411705884));
#38516=CARTESIAN_POINT('Ctrl Pts',(0.146200563886629,1.8123705051892,12.2901557531709));
#38517=CARTESIAN_POINT('Ctrl Pts',(0.132086239725396,1.80562188765775,12.2891046297023));
#38518=CARTESIAN_POINT('Ctrl Pts',(0.10041966889317,1.79321811506809,12.2868036894158));
#38519=CARTESIAN_POINT('Ctrl Pts',(0.0827559233496249,1.7879891000378,12.2855554124849));
#38520=CARTESIAN_POINT('Ctrl Pts',(0.0607357642610242,1.78347344068038,
12.2841057500113));
#38521=CARTESIAN_POINT('Ctrl Pts',(0.0567145821016261,1.78272826178682,
12.2838453439549));
#38522=CARTESIAN_POINT('Ctrl Pts',(0.0521491910143933,1.7819718140105,12.2835553937908));
#38523=CARTESIAN_POINT('Ctrl Pts',(0.0516180766465092,1.78188517893618,
12.2835217494151));
#38524=CARTESIAN_POINT('Ctrl Pts',(0.0508136401664482,1.78175602738491,
12.2834709251376));
#38525=CARTESIAN_POINT('Ctrl Pts',(0.0505404794985263,1.78171253234494,
12.2834536902561));
#38526=CARTESIAN_POINT('Ctrl Pts',(0.0500651520789352,1.78163747387719,
12.2834237409152));
#38527=CARTESIAN_POINT('Ctrl Pts',(0.049863011192974,1.78160575129675,12.2834110173884));
#38528=CARTESIAN_POINT('Ctrl Pts',(0.0494392676495891,1.78153966537809,
12.2833843726261));
#38529=CARTESIAN_POINT('Ctrl Pts',(0.0492176593973558,1.78150534083437,
12.2833704536787));
#38530=CARTESIAN_POINT('Ctrl Pts',(0.0486859051418298,1.78142354652447,
12.2833370920217));
#38531=CARTESIAN_POINT('Ctrl Pts',(0.0483757241973754,1.78137629815266,
12.283317661956));
#38532=CARTESIAN_POINT('Ctrl Pts',(0.0477189829142257,1.78127724103635,
12.283276586237));
#38533=CARTESIAN_POINT('Ctrl Pts',(0.0473724057203805,1.7812255443252,12.2832549469167));
#38534=CARTESIAN_POINT('Ctrl Pts',(0.0444003026821778,1.78078716873952,
12.283069691129));
#38535=CARTESIAN_POINT('Ctrl Pts',(0.041770077282181,1.78043235417886,12.2829078458918));
#38536=CARTESIAN_POINT('Ctrl Pts',(0.0298089336753,1.77896901543558,12.2821801443013));
#38537=CARTESIAN_POINT('Ctrl Pts',(0.020435847663643,1.7782363056478,12.2816327291349));
#38538=CARTESIAN_POINT('Ctrl Pts',(-0.00712414928507726,1.77729135873321,
12.280055637314));
#38539=CARTESIAN_POINT('Ctrl Pts',(-0.0253123740940854,1.77820664955439,
12.2790546045622));
#38540=CARTESIAN_POINT('Ctrl Pts',(-0.0634717890011353,1.78338384563155,
12.2768876884808));
#38541=CARTESIAN_POINT('Ctrl Pts',(-0.0833095118123769,1.78801635332981,
12.2757197626134));
#38542=CARTESIAN_POINT('Ctrl Pts',(-0.103807366950076,1.79489855778915,
12.2744064894633));
#38543=CARTESIAN_POINT('Ctrl Pts',(-0.105034992433163,1.79531900328397,
12.274327434013));
#38544=CARTESIAN_POINT('Ctrl Pts',(-0.106742880670442,1.79591548110399,
12.2742168769918));
#38545=CARTESIAN_POINT('Ctrl Pts',(-0.107225325634724,1.79608526402327,
12.2741855827038));
#38546=CARTESIAN_POINT('Ctrl Pts',(-0.108057480004907,1.79638034543847,
12.274131492634));
#38547=CARTESIAN_POINT('Ctrl Pts',(-0.108407381708901,1.79650510183823,
12.2741087148992));
#38548=CARTESIAN_POINT('Ctrl Pts',(-0.109130919859783,1.79676448808675,
12.2740615433948));
#38549=CARTESIAN_POINT('Ctrl Pts',(-0.109504524570909,1.79689920413989,
12.2740371467862));
#38550=CARTESIAN_POINT('Ctrl Pts',(-0.110244172821911,1.79716745583784,
12.2739887691711));
#38551=CARTESIAN_POINT('Ctrl Pts',(-0.110610225120833,1.79730096541035,
12.2739647890702));
#38552=CARTESIAN_POINT('Ctrl Pts',(-0.11145779460694,1.79761184056866,12.2739091762592));
#38553=CARTESIAN_POINT('Ctrl Pts',(-0.111939131127701,1.79778969266352,
12.2738775273313));
#38554=CARTESIAN_POINT('Ctrl Pts',(-0.114568944040615,1.79876854373663,
12.2737042464412));
#38555=CARTESIAN_POINT('Ctrl Pts',(-0.11670920590725,1.79959128840738,12.2735618881268));
#38556=CARTESIAN_POINT('Ctrl Pts',(-0.122232166625808,1.80178231578794,
12.2731909846474));
#38557=CARTESIAN_POINT('Ctrl Pts',(-0.125600656724107,1.80318530526818,
12.2729612843199));
#38558=CARTESIAN_POINT('Ctrl Pts',(-0.139059090113749,1.80906091828334,
12.2720291402559));
#38559=CARTESIAN_POINT('Ctrl Pts',(-0.148939151080029,1.81399289355591,
12.271311505751));
#38560=CARTESIAN_POINT('Ctrl Pts',(-0.166247880318986,1.8237735026707,12.2699949973283));
#38561=CARTESIAN_POINT('Ctrl Pts',(-0.173766948893,1.8284406711377,12.2694014357622));
#38562=CARTESIAN_POINT('Ctrl Pts',(-0.201371345133162,1.84719132991211,
12.2671491173728));
#38563=CARTESIAN_POINT('Ctrl Pts',(-0.220020846834212,1.86324341739304,
12.265468116185));
#38564=CARTESIAN_POINT('Ctrl Pts',(-0.237601176571995,1.882264520404,12.2638318294844));
#38565=CARTESIAN_POINT('Ctrl Pts',(-0.238526035780492,1.88327808463892,
12.263745596696));
#38566=CARTESIAN_POINT('Ctrl Pts',(-0.239720194637914,1.88460368229058,
12.2636340925793));
#38567=CARTESIAN_POINT('Ctrl Pts',(-0.239995390756795,1.88491034934239,
12.2636083849277));
#38568=CARTESIAN_POINT('Ctrl Pts',(-0.240417286702995,1.88538231032765,
12.2635689569453));
#38569=CARTESIAN_POINT('Ctrl Pts',(-0.240564404610092,1.88554722734081,
12.2635552050967));
#38570=CARTESIAN_POINT('Ctrl Pts',(-0.240856286568796,1.88587510103593,
12.2635279155951));
#38571=CARTESIAN_POINT('Ctrl Pts',(-0.241001054010817,1.88603805220957,
12.2635143777422));
#38572=CARTESIAN_POINT('Ctrl Pts',(-0.241323580563573,1.88640183282966,
12.2634842104317));
#38573=CARTESIAN_POINT('Ctrl Pts',(-0.241501253893264,1.88660273684092,
12.2634675874784));
#38574=CARTESIAN_POINT('Ctrl Pts',(-0.242020126930007,1.88719093018711,
12.2634190285126));
#38575=CARTESIAN_POINT('Ctrl Pts',(-0.242360649297349,1.8875788199949,12.2633871432225));
#38576=CARTESIAN_POINT('Ctrl Pts',(-0.244797174068739,1.89036775674494,
12.2631588567562));
#38577=CARTESIAN_POINT('Ctrl Pts',(-0.246858481669566,1.89279906918405,
12.2629649846397));
#38578=CARTESIAN_POINT('Ctrl Pts',(-0.25804471650477,1.90639718441898,12.2619061468094));
#38579=CARTESIAN_POINT('Ctrl Pts',(-0.266449291991257,1.91813741883173,
12.2610848142352));
#38580=CARTESIAN_POINT('Ctrl Pts',(-0.276856558504016,1.93495373522362,
12.2599729298432));
#38581=CARTESIAN_POINT('Ctrl Pts',(-0.279559457379286,1.93957452076478,
12.2596736637416));
#38582=CARTESIAN_POINT('Ctrl Pts',(-0.284878868591628,1.94921145279089,
12.2590583792889));
#38583=CARTESIAN_POINT('Ctrl Pts',(-0.287480892726333,1.95423343546623,
12.2587424775959));
#38584=CARTESIAN_POINT('Ctrl Pts',(-0.2917277738155,1.96298657431101,12.2581965109031));
#38585=CARTESIAN_POINT('Ctrl Pts',(-0.293436447127396,1.96668524663971,
12.2579671965251));
#38586=CARTESIAN_POINT('Ctrl Pts',(-0.302247550410876,1.98674881454398,
12.2567271385163));
#38587=CARTESIAN_POINT('Ctrl Pts',(-0.308051008610819,2.00364727176851,
12.2556940009228));
#38588=CARTESIAN_POINT('Ctrl Pts',(-0.3127407994431,2.02217963188986,12.2545327916796));
#38589=CARTESIAN_POINT('Ctrl Pts',(-0.313047719423597,2.02342361578632,
12.2544547259284));
#38590=CARTESIAN_POINT('Ctrl Pts',(-0.313466110480629,2.02516396619935,
12.2543453332399));
#38591=CARTESIAN_POINT('Ctrl Pts',(-0.313583839660738,2.02565882786899,
12.254314207863));
#38592=CARTESIAN_POINT('Ctrl Pts',(-0.313785350715879,2.02651485347623,
12.2542603309783));
#38593=CARTESIAN_POINT('Ctrl Pts',(-0.313869682102774,2.02687588811926,
12.2542375971832));
#38594=CARTESIAN_POINT('Ctrl Pts',(-0.314043158577843,2.02762439459965,
12.2541904420627));
#38595=CARTESIAN_POINT('Ctrl Pts',(-0.314132209969285,2.0280118873409,12.2541660177685));
#38596=CARTESIAN_POINT('Ctrl Pts',(-0.314307294999275,2.02878025272953,
12.2541175609856));
#38597=CARTESIAN_POINT('Ctrl Pts',(-0.314393353965068,2.02916111892832,
12.2540935293596));
#38598=CARTESIAN_POINT('Ctrl Pts',(-0.314591414144997,2.03004513259632,
12.2540377213459));
#38599=CARTESIAN_POINT('Ctrl Pts',(-0.314702900589451,2.03054839323059,
12.2540059284872));
#38600=CARTESIAN_POINT('Ctrl Pts',(-0.314988697414981,2.03185332591277,
12.253923433308));
#38601=CARTESIAN_POINT('Ctrl Pts',(-0.315161154041282,2.03265539626854,
12.2538726716854));
#38602=CARTESIAN_POINT('Ctrl Pts',(-0.319969153789331,2.05543967834303,
12.252429054407));
#38603=CARTESIAN_POINT('Ctrl Pts',(-0.322295489667893,2.07784050634339,
12.2509596929231));
#38604=CARTESIAN_POINT('Ctrl Pts',(-0.322274864054643,2.10029601277207,
12.2494497673494));
#38605=CARTESIAN_POINT('',(-0.322274852789156,2.09973668262869,11.999512253058));
#38606=CARTESIAN_POINT('Ctrl Pts',(-0.322274864232108,2.10029581950008,
12.2494497803451));
#38607=CARTESIAN_POINT('Ctrl Pts',(-0.322250804242316,2.12650751258178,
12.2476872860856));
#38608=CARTESIAN_POINT('Ctrl Pts',(-0.319029134840591,2.15262041363499,
12.2458804051903));
#38609=CARTESIAN_POINT('Ctrl Pts',(-0.312335749251866,2.17943278422205,
12.2441234271947));
#38610=CARTESIAN_POINT('Ctrl Pts',(-0.311983118138568,2.18080669301348,
12.244033702601));
#38611=CARTESIAN_POINT('Ctrl Pts',(-0.311456902473738,2.18280211221575,
12.2439038798979));
#38612=CARTESIAN_POINT('Ctrl Pts',(-0.311290509892046,2.18342547784592,
12.2438633933506));
#38613=CARTESIAN_POINT('Ctrl Pts',(-0.310988428232003,2.18454369526298,
12.2437908977568));
#38614=CARTESIAN_POINT('Ctrl Pts',(-0.310853427789059,2.18503872849104,
12.2437588501594));
#38615=CARTESIAN_POINT('Ctrl Pts',(-0.310646233430755,2.18579140322462,
12.2437101957219));
#38616=CARTESIAN_POINT('Ctrl Pts',(-0.310574900793226,2.18604927780341,
12.2436935391326));
#38617=CARTESIAN_POINT('Ctrl Pts',(-0.310444881871579,2.18651704133597,
12.2436633493241));
#38618=CARTESIAN_POINT('Ctrl Pts',(-0.310386304035035,2.18672695884262,
12.2436498098575));
#38619=CARTESIAN_POINT('Ctrl Pts',(-0.310267791099378,2.18714999967907,
12.2436225418471));
#38620=CARTESIAN_POINT('Ctrl Pts',(-0.310207849597125,2.18736311971762,
12.2436088137578));
#38621=CARTESIAN_POINT('Ctrl Pts',(-0.310035195816046,2.18797456648244,
12.2435694529774));
#38622=CARTESIAN_POINT('Ctrl Pts',(-0.309921935076539,2.18837273988864,
12.2435438523035));
#38623=CARTESIAN_POINT('Ctrl Pts',(-0.309425415538343,2.19010558287245,
12.243432569365));
#38624=CARTESIAN_POINT('Ctrl Pts',(-0.309034292726241,2.19143801139799,
12.2433473389029));
#38625=CARTESIAN_POINT('Ctrl Pts',(-0.300978091751989,2.21824062416167,
12.2416389227375));
#38626=CARTESIAN_POINT('Ctrl Pts',(-0.290196131766033,2.24267227207735,
12.2401863497874));
#38627=CARTESIAN_POINT('Ctrl Pts',(-0.272379716501707,2.27244079019132,
12.2382417670585));
#38628=CARTESIAN_POINT('Ctrl Pts',(-0.267968456496069,2.27921895814117,
12.2377863219828));
#38629=CARTESIAN_POINT('Ctrl Pts',(-0.255609014495846,2.29673193404628,
12.2365620763112));
#38630=CARTESIAN_POINT('Ctrl Pts',(-0.247241377281068,2.30714984607449,
12.2357831466496));
#38631=CARTESIAN_POINT('Ctrl Pts',(-0.236703618400437,2.31871868643102,
12.2348384449069));
#38632=CARTESIAN_POINT('Ctrl Pts',(-0.235136515747221,2.32040255283496,
12.234698832962));
#38633=CARTESIAN_POINT('Ctrl Pts',(-0.233197724706082,2.32244158893129,
12.2345271102168));
#38634=CARTESIAN_POINT('Ctrl Pts',(-0.232843009565415,2.32281286360105,
12.2344957327835));
#38635=CARTESIAN_POINT('Ctrl Pts',(-0.232217490047426,2.32346445993949,
12.2344404706035));
#38636=CARTESIAN_POINT('Ctrl Pts',(-0.231947060957858,2.32374514173693,
12.2344166021647));
#38637=CARTESIAN_POINT('Ctrl Pts',(-0.231400004059731,2.32431088142892,
12.2343683639391));
#38638=CARTESIAN_POINT('Ctrl Pts',(-0.231123357125802,2.32459591980906,
12.2343439933396));
#38639=CARTESIAN_POINT('Ctrl Pts',(-0.230587046640819,2.32514645780451,
12.2342967932374));
#38640=CARTESIAN_POINT('Ctrl Pts',(-0.23032744961418,2.3254120216246,12.2342739666683));
#38641=CARTESIAN_POINT('Ctrl Pts',(-0.229709536040932,2.32604195591522,
12.2342196807777));
#38642=CARTESIAN_POINT('Ctrl Pts',(-0.229350811508963,2.32640592315021,
12.2341882035323));
#38643=CARTESIAN_POINT('Ctrl Pts',(-0.228079868694,2.32768932038622,12.2340768137432));
#38644=CARTESIAN_POINT('Ctrl Pts',(-0.22716298434059,2.32860409355114,12.2339966950039));
#38645=CARTESIAN_POINT('Ctrl Pts',(-0.212148286912016,2.34340469295182,
12.2326884795065));
#38646=CARTESIAN_POINT('Ctrl Pts',(-0.196809271708206,2.3559659932542,12.2314019909232));
#38647=CARTESIAN_POINT('Ctrl Pts',(-0.173047426057694,2.37202002073897,
12.2294834996321));
#38648=CARTESIAN_POINT('Ctrl Pts',(-0.16547382187034,2.37669244426367,12.2288823993777));
#38649=CARTESIAN_POINT('Ctrl Pts',(-0.150621434502374,2.38502729611989,
12.227729892546));
#38650=CARTESIAN_POINT('Ctrl Pts',(-0.143377607654854,2.38873905573101,
12.2271790412801));
#38651=CARTESIAN_POINT('Ctrl Pts',(-0.127034843866261,2.39634630763618,
12.2259696778447));
#38652=CARTESIAN_POINT('Ctrl Pts',(-0.117880532467543,2.40010531447949,
12.2253141148235));
#38653=CARTESIAN_POINT('Ctrl Pts',(-0.106203351810587,2.40428329927523,
12.2245163542929));
#38654=CARTESIAN_POINT('Ctrl Pts',(-0.103829724148162,2.40510140513925,
12.2243561447867));
#38655=CARTESIAN_POINT('Ctrl Pts',(-0.100040925568022,2.40635793181671,
12.2241037752353));
#38656=CARTESIAN_POINT('Ctrl Pts',(-0.0986319240098715,2.40681446012524,
12.2240106546567));
#38657=CARTESIAN_POINT('Ctrl Pts',(-0.0968297941768319,2.40738466765821,
12.223892529625));
#38658=CARTESIAN_POINT('Ctrl Pts',(-0.0964395577434483,2.40750732456046,
12.2238670089029));
#38659=CARTESIAN_POINT('Ctrl Pts',(-0.0958153736175292,2.40770220953033,
12.2238262827595));
#38660=CARTESIAN_POINT('Ctrl Pts',(-0.0955815769472646,2.40777491405335,
12.2238110493515));
#38661=CARTESIAN_POINT('Ctrl Pts',(-0.0951382946752794,2.40791220918779,
12.2237822068922));
#38662=CARTESIAN_POINT('Ctrl Pts',(-0.0949288277662168,2.40797685195456,
12.2237685948769));
#38663=CARTESIAN_POINT('Ctrl Pts',(-0.0944495052593821,2.40812423833353,
12.2237374854126));
#38664=CARTESIAN_POINT('Ctrl Pts',(-0.0941796072273278,2.40820684106023,
12.2237199963553));
#38665=CARTESIAN_POINT('Ctrl Pts',(-0.0933498478083672,2.40845959854538,
12.2236663144005));
#38666=CARTESIAN_POINT('Ctrl Pts',(-0.0927896272933311,2.40862858438597,
12.2236301899016));
#38667=CARTESIAN_POINT('Ctrl Pts',(-0.0885802610561344,2.40988580710984,
12.223359633033));
#38668=CARTESIAN_POINT('Ctrl Pts',(-0.0849123539528292,2.41091087362385,
12.2231288051788));
#38669=CARTESIAN_POINT('Ctrl Pts',(-0.0801491223111135,2.4121514605577,
12.2228343566469));
#38670=CARTESIAN_POINT('Ctrl Pts',(-0.0790698348165592,2.41242659525752,
12.2227679881324));
#38671=CARTESIAN_POINT('Ctrl Pts',(-0.0590812300213608,2.41741192670176,
12.2215449267224));
#38672=CARTESIAN_POINT('Ctrl Pts',(-0.0397823280552906,2.42040359528464,
12.2204630903205));
#38673=CARTESIAN_POINT('Ctrl Pts',(-0.00804815058294582,2.42240942696339,
12.2186855301368));
#38674=CARTESIAN_POINT('Ctrl Pts',(0.0042672199520332,2.42248159880663,
12.2179963541319));
#38675=CARTESIAN_POINT('Ctrl Pts',(0.0261215335935303,2.42135740472693,
12.2167425664218));
#38676=CARTESIAN_POINT('Ctrl Pts',(0.035659595430544,2.42043920724829,12.2161849462941));
#38677=CARTESIAN_POINT('Ctrl Pts',(0.0498771597140101,2.4184278795096,12.2153294109509));
#38678=CARTESIAN_POINT('Ctrl Pts',(0.0545965565166873,2.41765273148977,
12.2150413906576));
#38679=CARTESIAN_POINT('Ctrl Pts',(0.0601296352072875,2.41661699346929,
12.214698382625));
#38680=CARTESIAN_POINT('Ctrl Pts',(0.060961869112126,2.41645780773511,12.2146466482518));
#38681=CARTESIAN_POINT('Ctrl Pts',(0.0621766979386902,2.41622047108946,
12.2145709193467));
#38682=CARTESIAN_POINT('Ctrl Pts',(0.0625597987679584,2.4161449029774,12.2145470072282));
#38683=CARTESIAN_POINT('Ctrl Pts',(0.063332705772376,2.41599098419503,12.2144987020316));
#38684=CARTESIAN_POINT('Ctrl Pts',(0.0637225061250163,2.41591260804826,
12.2144743081783));
#38685=CARTESIAN_POINT('Ctrl Pts',(0.064475490071809,2.4157597571795,12.2144271237479));
#38686=CARTESIAN_POINT('Ctrl Pts',(0.0648386923591865,2.41568537667339,
12.214404336217));
#38687=CARTESIAN_POINT('Ctrl Pts',(0.0656998717638844,2.41550746611676,
12.2143502382763));
#38688=CARTESIAN_POINT('Ctrl Pts',(0.066197732608585,2.41540338380866,12.2143189102327));
#38689=CARTESIAN_POINT('Ctrl Pts',(0.0679486142395856,2.41503301798155,
12.2142085468187));
#38690=CARTESIAN_POINT('Ctrl Pts',(0.0692002792039081,2.41476044522338,
12.2141293102095));
#38691=CARTESIAN_POINT('Ctrl Pts',(0.087828832837606,2.41058725486211,12.212944868522));
#38692=CARTESIAN_POINT('Ctrl Pts',(0.104851695093844,2.40526099663527,12.2117928196736));
#38693=CARTESIAN_POINT('Ctrl Pts',(0.139086622981571,2.39134659077768,12.209332885756));
#38694=CARTESIAN_POINT('Ctrl Pts',(0.156149579701987,2.3825688798747,12.2080244026759));
#38695=CARTESIAN_POINT('Ctrl Pts',(0.180610036853933,2.36709021070331,12.2060829640449));
#38696=CARTESIAN_POINT('Ctrl Pts',(0.188646652213701,2.36147588809568,12.2054337561444));
#38697=CARTESIAN_POINT('Ctrl Pts',(0.199386534870449,2.35321972326171,12.2045624920863));
#38698=CARTESIAN_POINT('Ctrl Pts',(0.202317611698718,2.35088404803902,12.2043243265548));
#38699=CARTESIAN_POINT('Ctrl Pts',(0.205621469516025,2.34815574792004,12.2040560681335));
#38700=CARTESIAN_POINT('Ctrl Pts',(0.206034653917612,2.34781280303211,12.2040225230517));
#38701=CARTESIAN_POINT('Ctrl Pts',(0.206656251727172,2.34729424481476,12.2039720656141));
#38702=CARTESIAN_POINT('Ctrl Pts',(0.206865300057859,2.3471193993391,12.2039550977502));
#38703=CARTESIAN_POINT('Ctrl Pts',(0.207225435419358,2.34681740929815,12.2039258693378));
#38704=CARTESIAN_POINT('Ctrl Pts',(0.207376627210429,2.34669039118906,12.2039135995398));
#38705=CARTESIAN_POINT('Ctrl Pts',(0.207690843875046,2.34642592084633,12.2038881014997));
#38706=CARTESIAN_POINT('Ctrl Pts',(0.207853848592266,2.34628844617744,12.2038748750081));
#38707=CARTESIAN_POINT('Ctrl Pts',(0.20830198834681,2.34590973297768,12.2038385145462));
#38708=CARTESIAN_POINT('Ctrl Pts',(0.208586841799942,2.34566815942173,12.2038154052217));
#38709=CARTESIAN_POINT('Ctrl Pts',(0.209688630620329,2.34473047574918,12.2037260277778));
#38710=CARTESIAN_POINT('Ctrl Pts',(0.210502518383633,2.34403077142529,12.2036600208582));
#38711=CARTESIAN_POINT('Ctrl Pts',(0.225125678314963,2.33133155420441,12.2024740383108));
#38712=CARTESIAN_POINT('Ctrl Pts',(0.237894279003523,2.31817970358389,12.2014370338216));
#38713=CARTESIAN_POINT('Ctrl Pts',(0.259096788216579,2.29225206439306,12.1995588905049));
#38714=CARTESIAN_POINT('Ctrl Pts',(0.267870622983788,2.27982580697308,12.1987166418511));
#38715=CARTESIAN_POINT('Ctrl Pts',(0.280867591647279,2.25834416493337,12.1972895732924));
#38716=CARTESIAN_POINT('Ctrl Pts',(0.28560546553727,2.24962945234911,12.196718004842));
#38717=CARTESIAN_POINT('Ctrl Pts',(0.292792061107095,2.2348214985129,12.1957469240929));
#38718=CARTESIAN_POINT('Ctrl Pts',(0.295469947551666,2.22884691841445,12.1953552084476));
#38719=CARTESIAN_POINT('Ctrl Pts',(0.298388592006374,2.22176479766612,12.1948893996792));
#38720=CARTESIAN_POINT('Ctrl Pts',(0.298807902691788,2.22073216236912,12.1948214458469));
#38721=CARTESIAN_POINT('Ctrl Pts',(0.299419525000876,2.21920321703179,12.1947207729682));
#38722=CARTESIAN_POINT('Ctrl Pts',(0.2996159801839,2.21870856462594,12.1946881937081));
#38723=CARTESIAN_POINT('Ctrl Pts',(0.29995766127044,2.21784199794879,12.1946311023845));
#38724=CARTESIAN_POINT('Ctrl Pts',(0.300103423458345,2.217470295231,12.1946066084267));
#38725=CARTESIAN_POINT('Ctrl Pts',(0.300382326988072,2.21675516659423,12.1945594731608));
#38726=CARTESIAN_POINT('Ctrl Pts',(0.300515571129466,2.21641178119159,12.1945368353513));
#38727=CARTESIAN_POINT('Ctrl Pts',(0.300828033805284,2.21560241761011,12.1944834662569));
#38728=CARTESIAN_POINT('Ctrl Pts',(0.301006758400135,2.21513625090918,12.1944527184548));
#38729=CARTESIAN_POINT('Ctrl Pts',(0.301531338127078,2.21375842165901,12.1943618109359));
#38730=CARTESIAN_POINT('Ctrl Pts',(0.301874137554118,2.21284560874719,12.1943015490802));
#38731=CARTESIAN_POINT('Ctrl Pts',(0.304877158035974,2.20473749695399,12.193765932672));
#38732=CARTESIAN_POINT('Ctrl Pts',(0.307283622332338,2.19745144409209,12.1932821808523));
#38733=CARTESIAN_POINT('Ctrl Pts',(0.310853718739578,2.1851889937031,12.1924630099013));
#38734=CARTESIAN_POINT('Ctrl Pts',(0.312163153298217,2.18025808638123,12.1921323142605));
#38735=CARTESIAN_POINT('Ctrl Pts',(0.313439924575449,2.17494479002986,12.1917746960576));
#38736=CARTESIAN_POINT('Ctrl Pts',(0.313524292624309,2.17459105712778,12.1917508816788));
#38737=CARTESIAN_POINT('Ctrl Pts',(0.318895616440199,2.15190040026306,12.1902229019562));
#38738=CARTESIAN_POINT('Ctrl Pts',(0.321781203752501,2.12906404462975,12.1886549049665));
#38739=CARTESIAN_POINT('Ctrl Pts',(0.32242591360832,2.09511207005607,12.1863712952104));
#38740=CARTESIAN_POINT('Ctrl Pts',(0.322070845718145,2.08410105736389,12.1856393320636));
#38741=CARTESIAN_POINT('Ctrl Pts',(0.32089073715439,2.06999684966461,12.1847290903559));
#38742=CARTESIAN_POINT('Ctrl Pts',(0.320582857158575,2.0668686300036,12.1845289620307));
#38743=CARTESIAN_POINT('Ctrl Pts',(0.320123001118662,2.06280683191284,12.1842718267559));
#38744=CARTESIAN_POINT('Ctrl Pts',(0.3200126285265,2.06186884169009,12.1842126356778));
#38745=CARTESIAN_POINT('Ctrl Pts',(0.319856098208919,2.0605871557641,12.1841320272075));
#38746=CARTESIAN_POINT('Ctrl Pts',(0.319813508291047,2.06024304124477,12.1841104117294));
#38747=CARTESIAN_POINT('Ctrl Pts',(0.319741618123637,2.059669780189,12.1840744478115));
#38748=CARTESIAN_POINT('Ctrl Pts',(0.319712626839636,2.05944059627617,12.1840600818874));
#38749=CARTESIAN_POINT('Ctrl Pts',(0.31965524333122,2.05899084870637,12.184031914366));
#38750=CARTESIAN_POINT('Ctrl Pts',(0.319626869241094,2.05877028330721,12.1840181117807));
#38751=CARTESIAN_POINT('Ctrl Pts',(0.319563971740581,2.05828531806241,12.1839877881367));
#38752=CARTESIAN_POINT('Ctrl Pts',(0.319529348372247,2.0580209307658,12.183971272759));
#38753=CARTESIAN_POINT('Ctrl Pts',(0.319408122027109,2.0571040745269,12.1839140547224));
#38754=CARTESIAN_POINT('Ctrl Pts',(0.319319847631485,2.05645182247572,12.183873446173));
#38755=CARTESIAN_POINT('Ctrl Pts',(0.318432441939038,2.05004265714018,12.1834753257096));
#38756=CARTESIAN_POINT('Ctrl Pts',(0.317479650560253,2.04430764891223,12.1831262818762));
#38757=CARTESIAN_POINT('Ctrl Pts',(0.316309290210392,2.03827709090472,12.1827639166509));
#38758=CARTESIAN_POINT('Ctrl Pts',(0.316245905530741,2.03795314820902,12.1827444658467));
#38759=CARTESIAN_POINT('Ctrl Pts',(0.314836485356429,2.03080823339121,12.1823157616421));
#38760=CARTESIAN_POINT('Ctrl Pts',(0.313270491373051,2.02403209002309,12.1819152944566));
#38761=CARTESIAN_POINT('Ctrl Pts',(0.306311920104847,1.99781923183642,12.1803720175568));
#38762=CARTESIAN_POINT('Ctrl Pts',(0.299319123247003,1.97885541356391,12.1792656071151));
#38763=CARTESIAN_POINT('Ctrl Pts',(0.2838720343976,1.94663774137063,12.1772394782223));
#38764=CARTESIAN_POINT('Ctrl Pts',(0.276138037124895,1.93311379908045,12.176338122323));
#38765=CARTESIAN_POINT('Ctrl Pts',(0.266090193366134,1.91816711402503,12.1752518150215));
#38766=CARTESIAN_POINT('Ctrl Pts',(0.264698893619078,1.91614765535498,12.1751030522891));
#38767=CARTESIAN_POINT('Ctrl Pts',(0.262877421778093,1.91356734319342,12.1749103155457));
#38768=CARTESIAN_POINT('Ctrl Pts',(0.262468239007734,1.91299171701678,12.1748671465374));
#38769=CARTESIAN_POINT('Ctrl Pts',(0.261802911860804,1.91206223960147,12.1747971586335));
#38770=CARTESIAN_POINT('Ctrl Pts',(0.261547932810234,1.91170755383678,12.1747703846795));
#38771=CARTESIAN_POINT('Ctrl Pts',(0.261062328387458,1.9110349487793,12.1747194846121));
#38772=CARTESIAN_POINT('Ctrl Pts',(0.260831841235791,1.9107169302835,12.1746953638743));
#38773=CARTESIAN_POINT('Ctrl Pts',(0.260306970437709,1.90999551015389,12.1746405222584));
#38774=CARTESIAN_POINT('Ctrl Pts',(0.260012229837511,1.90959237055573,12.1746097875637));
#38775=CARTESIAN_POINT('Ctrl Pts',(0.259136874365433,1.90840090149541,12.1745186885712));
#38776=CARTESIAN_POINT('Ctrl Pts',(0.258553606675946,1.9076145362959,12.1744582210376));
#38777=CARTESIAN_POINT('Ctrl Pts',(0.254563678343172,1.90228620662541,12.1740461449688));
#38778=CARTESIAN_POINT('Ctrl Pts',(0.251041275456718,1.89783254016515,12.1736900014085));
#38779=CARTESIAN_POINT('Ctrl Pts',(0.227545942908155,1.86968676522925,12.1713601176505));
#38780=CARTESIAN_POINT('Ctrl Pts',(0.204364147588138,1.84889075130435,12.1692427519275));
#38781=CARTESIAN_POINT('Ctrl Pts',(0.170836805670864,1.82657268743745,12.1665364750497));
#38782=CARTESIAN_POINT('Ctrl Pts',(0.162873046236269,1.82175531227858,12.1659177552412));
#38783=CARTESIAN_POINT('Ctrl Pts',(0.150346199277729,1.81490009088923,12.1649921089536));
#38784=CARTESIAN_POINT('Ctrl Pts',(0.145925882047167,1.81261248882104,12.1646741610063));
#38785=CARTESIAN_POINT('Ctrl Pts',(0.140931396430074,1.81017271437321,12.1643259532111));
#38786=CARTESIAN_POINT('Ctrl Pts',(0.140408034509772,1.80991880817402,12.1642895987867));
#38787=CARTESIAN_POINT('Ctrl Pts',(0.139630318786893,1.80954410148359,12.1642357772598));
#38788=CARTESIAN_POINT('Ctrl Pts',(0.139376493185796,1.8094222168572,12.164218243068));
#38789=CARTESIAN_POINT('Ctrl Pts',(0.138943231789713,1.80921486718607,12.1641883679928));
#38790=CARTESIAN_POINT('Ctrl Pts',(0.138763876597136,1.80912923543541,12.1641760166591));
#38791=CARTESIAN_POINT('Ctrl Pts',(0.138395197330561,1.80895363098148,12.1641506602807));
#38792=CARTESIAN_POINT('Ctrl Pts',(0.13820586514329,1.80886367728561,12.1641376564394));
#38793=CARTESIAN_POINT('Ctrl Pts',(0.137749300413533,1.80864730436267,12.1641063407173));
#38794=CARTESIAN_POINT('Ctrl Pts',(0.137481980834658,1.80852106771337,12.1640880402419));
#38795=CARTESIAN_POINT('Ctrl Pts',(0.136658929270486,1.80813378123072,12.1640318011251));
#38796=CARTESIAN_POINT('Ctrl Pts',(0.136102620547022,1.80787394963331,12.1639939374812));
#38797=CARTESIAN_POINT('Ctrl Pts',(0.12948205741262,1.80480474240426,12.1635450549818));
#38798=CARTESIAN_POINT('Ctrl Pts',(0.123332048445309,1.80218283401148,12.1631452764038));
#38799=CARTESIAN_POINT('Ctrl Pts',(0.0917936320983183,1.78988196354108,
12.1611594158225));
#38800=CARTESIAN_POINT('Ctrl Pts',(0.0653340231711807,1.78324924108288,
12.1596921107348));
#38801=CARTESIAN_POINT('Ctrl Pts',(0.0234432435491287,1.77822818313575,
12.1572955251619));
#38802=CARTESIAN_POINT('Ctrl Pts',(0.0084280757097688,1.77748555327846,
12.1564240409192));
#38803=CARTESIAN_POINT('Ctrl Pts',(-0.0081725582554667,1.77782471727114,
12.1554222443731));
#38804=CARTESIAN_POINT('Ctrl Pts',(-0.00976187437105561,1.77786895651076,
12.1553259597712));
#38805=CARTESIAN_POINT('Ctrl Pts',(-0.0125458590993433,1.77796707149617,
12.1551566146936));
#38806=CARTESIAN_POINT('Ctrl Pts',(-0.0137406851767255,1.77801584024699,
12.1550837143999));
#38807=CARTESIAN_POINT('Ctrl Pts',(-0.0154692699800852,1.77809603426448,
12.1549779188142));
#38808=CARTESIAN_POINT('Ctrl Pts',(-0.0160032752173329,1.77812214017294,
12.1549451903418));
#38809=CARTESIAN_POINT('Ctrl Pts',(-0.0169345002865394,1.77816998806678,
12.1548880366442));
#38810=CARTESIAN_POINT('Ctrl Pts',(-0.0173317505223976,1.77819113700455,
12.1548636300678));
#38811=CARTESIAN_POINT('Ctrl Pts',(-0.0180988077204094,1.7782333982725,
12.1548164534638));
#38812=CARTESIAN_POINT('Ctrl Pts',(-0.0184686196537694,1.77825441275059,
12.1547936865428));
#38813=CARTESIAN_POINT('Ctrl Pts',(-0.0193448742813105,1.77830572142715,
12.1547396881524));
#38814=CARTESIAN_POINT('Ctrl Pts',(-0.0198512821545668,1.77833657401006,
12.1547084392025));
#38815=CARTESIAN_POINT('Ctrl Pts',(-0.0216285799493489,1.77844906782366,
12.1545986184576));
#38816=CARTESIAN_POINT('Ctrl Pts',(-0.022899044229911,1.77853704544257,
12.1545198480204));
#38817=CARTESIAN_POINT('Ctrl Pts',(-0.0411450457737177,1.77990926438546,
12.1533846502993));
#38818=CARTESIAN_POINT('Ctrl Pts',(-0.0579903969458637,1.78252883832415,
12.152285570243));
#38819=CARTESIAN_POINT('Ctrl Pts',(-0.0911875576247426,1.79042200291301,
12.1500191617782));
#38820=CARTESIAN_POINT('Ctrl Pts',(-0.10748522584018,1.79569657715043,12.1488551765193));
#38821=CARTESIAN_POINT('Ctrl Pts',(-0.130820924110811,1.805358579614,12.1471518794098));
#38822=CARTESIAN_POINT('Ctrl Pts',(-0.1382349412377,1.80876333489777,12.1466052785176));
#38823=CARTESIAN_POINT('Ctrl Pts',(-0.152033408991192,1.81574582668419,
12.1455865815941));
#38824=CARTESIAN_POINT('Ctrl Pts',(-0.158441140355762,1.81926700121857,
12.1451129415581));
#38825=CARTESIAN_POINT('Ctrl Pts',(-0.165761188492736,1.82362008047841,
12.1445758691809));
#38826=CARTESIAN_POINT('Ctrl Pts',(-0.166794819787399,1.82424264338602,
12.1445001279929));
#38827=CARTESIAN_POINT('Ctrl Pts',(-0.168146458673976,1.82506712475546,
12.1444012361979));
#38828=CARTESIAN_POINT('Ctrl Pts',(-0.168467625909909,1.82526380566341,
12.1443777495246));
#38829=CARTESIAN_POINT('Ctrl Pts',(-0.168990835316154,1.82558547843364,
12.1443395071253));
#38830=CARTESIAN_POINT('Ctrl Pts',(-0.169193084176494,1.82571013081948,
12.1443247291086));
#38831=CARTESIAN_POINT('Ctrl Pts',(-0.169583531184181,1.82595137185702,
12.1442962092028));
#38832=CARTESIAN_POINT('Ctrl Pts',(-0.169771746558197,1.82606793048867,
12.1442824654443));
#38833=CARTESIAN_POINT('Ctrl Pts',(-0.170208244731394,1.82633886916924,
12.1442506013793));
#38834=CARTESIAN_POINT('Ctrl Pts',(-0.170456438526596,1.82649339373872,
12.1442324906558));
#38835=CARTESIAN_POINT('Ctrl Pts',(-0.171259754222359,1.82699505339711,
12.1441738949846));
#38836=CARTESIAN_POINT('Ctrl Pts',(-0.171814033209855,1.82734354528852,
12.1441334992411));
#38837=CARTESIAN_POINT('Ctrl Pts',(-0.177179836772807,1.8307400473474,12.1437427378237));
#38838=CARTESIAN_POINT('Ctrl Pts',(-0.181911182404739,1.83391364538554,
12.1434005020155));
#38839=CARTESIAN_POINT('Ctrl Pts',(-0.195745284064745,1.84373460618117,
12.142398973718));
#38840=CARTESIAN_POINT('Ctrl Pts',(-0.204586613609977,1.85073602891783,
12.1417576053892));
#38841=CARTESIAN_POINT('Ctrl Pts',(-0.22128263679001,1.86544564942136,12.1405054370517));
#38842=CARTESIAN_POINT('Ctrl Pts',(-0.229145399952628,1.87312087174949,
12.1398950542117));
#38843=CARTESIAN_POINT('Ctrl Pts',(-0.251952900995127,1.89778197137217,
12.1380112652371));
#38844=CARTESIAN_POINT('Ctrl Pts',(-0.265512703365968,1.91594791907097,
12.1367206890951));
#38845=CARTESIAN_POINT('Ctrl Pts',(-0.277645959975347,1.936368660818,12.1352762218622));
#38846=CARTESIAN_POINT('Ctrl Pts',(-0.27822723456428,1.93735898381281,12.1352062020391));
#38847=CARTESIAN_POINT('Ctrl Pts',(-0.279066951837687,1.93880729381427,
12.1351038377163));
#38848=CARTESIAN_POINT('Ctrl Pts',(-0.279329590453365,1.93926284801754,
12.1350716451628));
#38849=CARTESIAN_POINT('Ctrl Pts',(-0.27978825219837,1.94006292899954,12.1350151144643));
#38850=CARTESIAN_POINT('Ctrl Pts',(-0.279984757338678,1.94040717934645,
12.1349907937725));
#38851=CARTESIAN_POINT('Ctrl Pts',(-0.280364853781442,1.94107591941838,
12.1349435533605));
#38852=CARTESIAN_POINT('Ctrl Pts',(-0.280548518191308,1.94140036707656,
12.13492063632));
#38853=CARTESIAN_POINT('Ctrl Pts',(-0.280985316710408,1.94217511518753,
12.1348659177072));
#38854=CARTESIAN_POINT('Ctrl Pts',(-0.281237931362542,1.94262570594003,
12.13483409754));
#38855=CARTESIAN_POINT('Ctrl Pts',(-0.28199748553383,1.94398819810244,12.1347378908009));
#38856=CARTESIAN_POINT('Ctrl Pts',(-0.28250107743314,1.94490194911993,12.1346733845903));
#38857=CARTESIAN_POINT('Ctrl Pts',(-0.287736591034372,1.95451171326688,
12.1339951036527));
#38858=CARTESIAN_POINT('Ctrl Pts',(-0.292069387199294,1.96341806184594,
12.133367244534));
#38859=CARTESIAN_POINT('Ctrl Pts',(-0.296869168429375,1.97456130509599,
12.132581496512));
#38860=CARTESIAN_POINT('Ctrl Pts',(-0.297731807523742,1.97662277450443,
12.1324361396497));
#38861=CARTESIAN_POINT('Ctrl Pts',(-0.298895556221969,1.97948710948933,
12.1322341931402));
#38862=CARTESIAN_POINT('Ctrl Pts',(-0.299215018163668,1.9802824858496,12.1321781184354));
#38863=CARTESIAN_POINT('Ctrl Pts',(-0.308750751162532,2.00430056038684,
12.1304849230833));
#38864=CARTESIAN_POINT('Ctrl Pts',(-0.315237930365231,2.02851427611628,
12.1287711660902));
#38865=CARTESIAN_POINT('Ctrl Pts',(-0.320147128974368,2.06198330959738,
12.1265069835472));
#38866=CARTESIAN_POINT('Ctrl Pts',(-0.321070208798186,2.07078699950152,
12.1259219516109));
#38867=CARTESIAN_POINT('Ctrl Pts',(-0.321876437882674,2.0835094746295,12.1251012450242));
#38868=CARTESIAN_POINT('Ctrl Pts',(-0.322052405675305,2.0874051564045,12.1248532804103));
#38869=CARTESIAN_POINT('Ctrl Pts',(-0.322172199007007,2.09184273151272,
12.1245753430664));
#38870=CARTESIAN_POINT('Ctrl Pts',(-0.32218540670297,2.09238222080429,12.1245416294158));
#38871=CARTESIAN_POINT('Ctrl Pts',(-0.322203257140202,2.09319476037057,
12.1244909694424));
#38872=CARTESIAN_POINT('Ctrl Pts',(-0.322208907938681,2.09346778410821,
12.1244739669452));
#38873=CARTESIAN_POINT('Ctrl Pts',(-0.322218412677592,2.09395707503039,
12.1244435325245));
#38874=CARTESIAN_POINT('Ctrl Pts',(-0.322222395911609,2.09417333847038,
12.1244300933561));
#38875=CARTESIAN_POINT('Ctrl Pts',(-0.322229951516671,2.09460728560368,
12.1244031522037));
#38876=CARTESIAN_POINT('Ctrl Pts',(-0.322233521017299,2.09482496797487,
12.1243896504294));
#38877=CARTESIAN_POINT('Ctrl Pts',(-0.322242957230069,2.09543833972952,
12.1243516416435));
#38878=CARTESIAN_POINT('Ctrl Pts',(-0.322248315737617,2.09583403828043,
12.1243271632287));
#38879=CARTESIAN_POINT('Ctrl Pts',(-0.322267433478843,2.0974680799195,12.1242262483593));
#38880=CARTESIAN_POINT('Ctrl Pts',(-0.322274783835762,2.09870650839261,
12.124150166534));
#38881=CARTESIAN_POINT('Ctrl Pts',(-0.322276342644679,2.10783575717569,
12.1235920718815));
#38882=CARTESIAN_POINT('Ctrl Pts',(-0.321987884382043,2.11572467674183,
12.1231249473739));
#38883=CARTESIAN_POINT('Ctrl Pts',(-0.320794431443524,2.13198133051904,
12.1221792048649));
#38884=CARTESIAN_POINT('Ctrl Pts',(-0.319850850105213,2.14034006637319,
12.121702180975));
#38885=CARTESIAN_POINT('Ctrl Pts',(-0.314846686075205,2.17310768393261,
12.1198374257963));
#38886=CARTESIAN_POINT('Ctrl Pts',(-0.30830907175252,2.19704965078469,12.1184794041006));
#38887=CARTESIAN_POINT('Ctrl Pts',(-0.298222415858701,2.22218873643454,
12.1168961651712));
#38888=CARTESIAN_POINT('Ctrl Pts',(-0.297323639458718,2.2243597590333,12.1167581572311));
#38889=CARTESIAN_POINT('Ctrl Pts',(-0.293834214327468,2.23253446624093,
12.1162333473793));
#38890=CARTESIAN_POINT('Ctrl Pts',(-0.291084937616096,2.23846833617486,
12.1158417462099));
#38891=CARTESIAN_POINT('Ctrl Pts',(-0.287693952721533,2.24523923553649,
12.1153808672837));
#38892=CARTESIAN_POINT('Ctrl Pts',(-0.28722622410126,2.24616204063013,12.1153177472294));
#38893=CARTESIAN_POINT('Ctrl Pts',(-0.28652410589395,2.24753089929728,12.1152236536467));
#38894=CARTESIAN_POINT('Ctrl Pts',(-0.286293097303326,2.24797868744418,
12.1151927991736));
#38895=CARTESIAN_POINT('Ctrl Pts',(-0.285879908224683,2.24877502604746,
12.1151377952781));
#38896=CARTESIAN_POINT('Ctrl Pts',(-0.285698137645992,2.24912378899897,
12.1151136603659));
#38897=CARTESIAN_POINT('Ctrl Pts',(-0.285314271613702,2.24985703422972,
12.1150628224405));
#38898=CARTESIAN_POINT('Ctrl Pts',(-0.285112036492967,2.25024144214723,
12.1150361145187));
#38899=CARTESIAN_POINT('Ctrl Pts',(-0.284577357507929,2.25125279102775,
12.1149657000253));
#38900=CARTESIAN_POINT('Ctrl Pts',(-0.284243620340959,2.25187904227533,
12.1149219476256));
#38901=CARTESIAN_POINT('Ctrl Pts',(-0.282738413854348,2.25468119422699,
12.1147254996966));
#38902=CARTESIAN_POINT('Ctrl Pts',(-0.281544033866004,2.25684463320035,
12.1145719896642));
#38903=CARTESIAN_POINT('Ctrl Pts',(-0.272595332374421,2.27262222748544,
12.1134386165789));
#38904=CARTESIAN_POINT('Ctrl Pts',(-0.263883444601653,2.28566649216866,
12.1124236805742));
#38905=CARTESIAN_POINT('Ctrl Pts',(-0.236605405955893,2.32069093170012,
12.1094737416403));
#38906=CARTESIAN_POINT('Ctrl Pts',(-0.216001620746892,2.34089377680088,
12.1074804842746));
#38907=CARTESIAN_POINT('Ctrl Pts',(-0.192765426186075,2.35826875051136,
12.105604309327));
#38908=CARTESIAN_POINT('Ctrl Pts',(-0.192536709343627,2.35843930153844,
12.1055858757837));
#38909=CARTESIAN_POINT('Ctrl Pts',(-0.188905269226977,2.36113972051574,
12.1052937389265));
#38910=CARTESIAN_POINT('Ctrl Pts',(-0.185452962391017,2.36360265062239,
12.1050235322111));
#38911=CARTESIAN_POINT('Ctrl Pts',(-0.181504106688871,2.366303831138,12.1047237410441));
#38912=CARTESIAN_POINT('Ctrl Pts',(-0.181054580133359,2.36660965895231,
12.1046897470741));
#38913=CARTESIAN_POINT('Ctrl Pts',(-0.180374006908891,2.36707016036639,
12.1046384848981));
#38914=CARTESIAN_POINT('Ctrl Pts',(-0.180143533298982,2.36722567305274,
12.1046211603767));
#38915=CARTESIAN_POINT('Ctrl Pts',(-0.179742795404267,2.367495317979,12.1045910987732));
#38916=CARTESIAN_POINT('Ctrl Pts',(-0.179572623437434,2.36760958606291,
12.1045783524571));
#38917=CARTESIAN_POINT('Ctrl Pts',(-0.179216320076034,2.36784834587156,
12.1045517048543));
#38918=CARTESIAN_POINT('Ctrl Pts',(-0.179030168039897,2.36797280589582,
12.1045378057822));
#38919=CARTESIAN_POINT('Ctrl Pts',(-0.178584310861066,2.36827023111519,
12.1045045705911));
#38920=CARTESIAN_POINT('Ctrl Pts',(-0.178324483040512,2.36844301395011,
12.1044852468717));
#38921=CARTESIAN_POINT('Ctrl Pts',(-0.177441278281839,2.36902848789052,
12.1044197110749));
#38922=CARTESIAN_POINT('Ctrl Pts',(-0.176816710423165,2.36943939109999,
12.1043736187561));
#38923=CARTESIAN_POINT('Ctrl Pts',(-0.175326403644068,2.37041245034939,
12.1042642203409));
#38924=CARTESIAN_POINT('Ctrl Pts',(-0.174459376618461,2.37097263163358,
12.1042010416293));
#38925=CARTESIAN_POINT('Ctrl Pts',(-0.163988764406526,2.37766654786409,
12.1034434792377));
#38926=CARTESIAN_POINT('Ctrl Pts',(-0.154067913270634,2.3832916613998,12.1027802092355));
#38927=CARTESIAN_POINT('Ctrl Pts',(-0.121248992365313,2.39966457572549,
12.1006890229254));
#38928=CARTESIAN_POINT('Ctrl Pts',(-0.0973802288642483,2.40824883565762,
12.0993143269129));
#38929=CARTESIAN_POINT('Ctrl Pts',(-0.0673866300508326,2.41519923857274,
12.0975427651838));
#38930=CARTESIAN_POINT('Ctrl Pts',(-0.0619896586598934,2.41630490929118,
12.0972226972234));
#38931=CARTESIAN_POINT('Ctrl Pts',(-0.0556434249638426,2.41743639576912,
12.0968434854783));
#38932=CARTESIAN_POINT('Ctrl Pts',(-0.0547189477608854,2.41759706048924,
12.0967881747857));
#38933=CARTESIAN_POINT('Ctrl Pts',(-0.0474315267750385,2.41883077705468,
12.0963515881348));
#38934=CARTESIAN_POINT('Ctrl Pts',(-0.0410387246194138,2.41971648117848,
12.0959650359531));
#38935=CARTESIAN_POINT('Ctrl Pts',(-0.0335993630445958,2.42052039014624,
12.0955096149025));
#38936=CARTESIAN_POINT('Ctrl Pts',(-0.0325742437269905,2.42062619403822,
12.0954467380287));
#38937=CARTESIAN_POINT('Ctrl Pts',(-0.0310479922440137,2.42077632531076,
12.095352937302));
#38938=CARTESIAN_POINT('Ctrl Pts',(-0.0305472283189572,2.420824399851,12.0953221314156));
#38939=CARTESIAN_POINT('Ctrl Pts',(-0.0296548761251554,2.4209079596199,
12.0952671820205));
#38940=CARTESIAN_POINT('Ctrl Pts',(-0.0292633307583247,2.42094390116679,
12.0952430529162));
#38941=CARTESIAN_POINT('Ctrl Pts',(-0.0284386802876307,2.42101807757636,
12.0951921942891));
#38942=CARTESIAN_POINT('Ctrl Pts',(-0.0280055619243542,2.42105615266753,
12.0951654597923));
#38943=CARTESIAN_POINT('Ctrl Pts',(-0.0268634325159719,2.42115422761673,
12.095094900364));
#38944=CARTESIAN_POINT('Ctrl Pts',(-0.0261543004354624,2.42121275578406,
12.0950510292621));
#38945=CARTESIAN_POINT('Ctrl Pts',(-0.0229629466071878,2.42146551582734,
12.0948533108662));
#38946=CARTESIAN_POINT('Ctrl Pts',(-0.0204787716737362,2.42163332248732,
12.0946986360709));
#38947=CARTESIAN_POINT('Ctrl Pts',(-0.00214820910588213,2.42265833610814,
12.0935513645042));
#38948=CARTESIAN_POINT('Ctrl Pts',(0.0137378763777866,2.42237269203914,
12.0925227540347));
#38949=CARTESIAN_POINT('Ctrl Pts',(0.0564403062377369,2.41844249300545,
12.0896714181599));
#38950=CARTESIAN_POINT('Ctrl Pts',(0.082924205436861,2.41259337476701,12.0878025395995));
#38951=CARTESIAN_POINT('Ctrl Pts',(0.108647696570679,2.40340887004453,12.086021597949));
#38952=CARTESIAN_POINT('Ctrl Pts',(0.108928147269132,2.40330829715905,12.0860021868571));
#38953=CARTESIAN_POINT('Ctrl Pts',(0.110229349414959,2.40283963342715,12.0859121530276));
#38954=CARTESIAN_POINT('Ctrl Pts',(0.111248389420634,2.40246677331318,12.0858417213046));
#38955=CARTESIAN_POINT('Ctrl Pts',(0.112389400507216,2.40204273826556,12.0857629623433));
#38956=CARTESIAN_POINT('Ctrl Pts',(0.112513233101716,2.40199663154147,12.0857544160885));
#38957=CARTESIAN_POINT('Ctrl Pts',(0.113001208460231,2.40181460134739,12.0857207441392));
#38958=CARTESIAN_POINT('Ctrl Pts',(0.113365135129699,2.40167809472999,12.0856956439717));
#38959=CARTESIAN_POINT('Ctrl Pts',(0.117575462687778,2.40009013263181,12.0854054020905));
#38960=CARTESIAN_POINT('Ctrl Pts',(0.121394225358391,2.39856577686673,12.0851435626341));
#38961=CARTESIAN_POINT('Ctrl Pts',(0.125679617542044,2.39675932980752,12.0848521719234));
#38962=CARTESIAN_POINT('Ctrl Pts',(0.126175726413537,2.39654873489412,12.0848184758354));
#38963=CARTESIAN_POINT('Ctrl Pts',(0.126925842305621,2.39622809253203,12.0847675867588));
#38964=CARTESIAN_POINT('Ctrl Pts',(0.127180236604031,2.39611896202188,12.084750338594));
#38965=CARTESIAN_POINT('Ctrl Pts',(0.127622478347012,2.39592857336603,12.0847203726292));
#38966=CARTESIAN_POINT('Ctrl Pts',(0.127810389052439,2.395847464016,12.0847076457372));
#38967=CARTESIAN_POINT('Ctrl Pts',(0.128203982621281,2.39567712919892,12.0846810006182));
#38968=CARTESIAN_POINT('Ctrl Pts',(0.128409649579512,2.39558786813145,12.0846670846682));
#38969=CARTESIAN_POINT('Ctrl Pts',(0.128902674474397,2.3953732797994,12.0846337419977));
#38970=CARTESIAN_POINT('Ctrl Pts',(0.129189944022693,2.39524774727593,12.0846143278844));
#38971=CARTESIAN_POINT('Ctrl Pts',(0.13016958531043,2.39481795507537,12.084548167074));
#38972=CARTESIAN_POINT('Ctrl Pts',(0.130861075784829,2.39451167455012,12.0845015432624));
#38973=CARTESIAN_POINT('Ctrl Pts',(0.142600617937084,2.38926239267484,12.0837112007433));
#38974=CARTESIAN_POINT('Ctrl Pts',(0.153364144754091,2.3837026318528,12.0830045167327));
#38975=CARTESIAN_POINT('Ctrl Pts',(0.191346715704932,2.36128795671964,12.0804868447398));
#38976=CARTESIAN_POINT('Ctrl Pts',(0.216326639293571,2.34101426935919,12.0787643842795));
#38977=CARTESIAN_POINT('Ctrl Pts',(0.242308366819171,2.31258014371959,12.0764899334645));
#38978=CARTESIAN_POINT('Ctrl Pts',(0.246557969961256,2.3076362695811,12.0760995388745));
#38979=CARTESIAN_POINT('Ctrl Pts',(0.25130423633888,2.30176328902512,12.0756399642001));
#38980=CARTESIAN_POINT('Ctrl Pts',(0.251950046323989,2.30095625921681,12.0755769019998));
#38981=CARTESIAN_POINT('Ctrl Pts',(0.252904760717497,2.2997513737652,12.0754828780808));
#38982=CARTESIAN_POINT('Ctrl Pts',(0.25321663718779,2.29935587265344,12.0754520351579));
#38983=CARTESIAN_POINT('Ctrl Pts',(0.253770370881625,2.29865026842742,12.0753970442252));
#38984=CARTESIAN_POINT('Ctrl Pts',(0.254012590589035,2.29834044999383,12.0753729107006));
#38985=CARTESIAN_POINT('Ctrl Pts',(0.254515789257966,2.2976943848864,12.0753226096125));
#38986=CARTESIAN_POINT('Ctrl Pts',(0.254776670233835,2.29735806317201,12.0752964382295));
#38987=CARTESIAN_POINT('Ctrl Pts',(0.255444997307883,2.29649293784218,12.0752291520355));
#38988=CARTESIAN_POINT('Ctrl Pts',(0.255851466518521,2.2959633852052,12.0751879987387));
#38989=CARTESIAN_POINT('Ctrl Pts',(0.256740117558838,2.29479816281396,12.0750975165));
#38990=CARTESIAN_POINT('Ctrl Pts',(0.257221588966973,2.29416195907221,12.0750481599284));
#38991=CARTESIAN_POINT('Ctrl Pts',(0.258615602521586,2.29230566065964,12.0749042785559));
#38992=CARTESIAN_POINT('Ctrl Pts',(0.259521851473747,2.29108088724055,12.074809508858));
#38993=CARTESIAN_POINT('Ctrl Pts',(0.268641970442819,2.27857070155952,12.0738430620765));
#38994=CARTESIAN_POINT('Ctrl Pts',(0.276122002535642,2.26677095102367,12.0729432997772));
#38995=CARTESIAN_POINT('Ctrl Pts',(0.292517403551519,2.23676392951125,12.0706840739576));
#38996=CARTESIAN_POINT('Ctrl Pts',(0.300526584624002,2.21812901149954,12.0693029557718));
#38997=CARTESIAN_POINT('Ctrl Pts',(0.311166577221818,2.18511888572013,12.0669694528979));
#38998=CARTESIAN_POINT('Ctrl Pts',(0.314669488683918,2.17108507123702,12.0660112204675));
#38999=CARTESIAN_POINT('Ctrl Pts',(0.317378876897357,2.1559700374265,12.0650455373233));
#39000=CARTESIAN_POINT('Ctrl Pts',(0.317534983662659,2.15507749801205,12.0649887586903));
#39001=CARTESIAN_POINT('Ctrl Pts',(0.317740022986055,2.15387533437661,12.0649126234802));
#39002=CARTESIAN_POINT('Ctrl Pts',(0.317792269155838,2.15356629096906,12.0648930814105));
#39003=CARTESIAN_POINT('Ctrl Pts',(0.317879516614113,2.15304558950056,12.0648602067882));
#39004=CARTESIAN_POINT('Ctrl Pts',(0.317914757412299,2.15283397267269,12.0648468606096));
#39005=CARTESIAN_POINT('Ctrl Pts',(0.317981975588801,2.15242783313206,12.0648212739914));
#39006=CARTESIAN_POINT('Ctrl Pts',(0.318013985555463,2.15223331769722,12.0648090317966));
#39007=CARTESIAN_POINT('Ctrl Pts',(0.318089377464563,2.15177254430247,12.0647800609023));
#39008=CARTESIAN_POINT('Ctrl Pts',(0.318132603531913,2.1515062614701,12.0647633412003));
#39009=CARTESIAN_POINT('Ctrl Pts',(0.318258753060684,2.15072293304063,12.0647142224976));
#39010=CARTESIAN_POINT('Ctrl Pts',(0.318340751250185,2.15020573611238,12.0646818760227));
#39011=CARTESIAN_POINT('Ctrl Pts',(0.31895192772459,2.14628908819037,12.0644375446238));
#39012=CARTESIAN_POINT('Ctrl Pts',(0.319427926279899,2.14288139592922,12.0642285151055));
#39013=CARTESIAN_POINT('Ctrl Pts',(0.32087536591281,2.13115089764422,12.0635191224879));
#39014=CARTESIAN_POINT('Ctrl Pts',(0.321576846406159,2.12279766927815,12.0630314413043));
#39015=CARTESIAN_POINT('Ctrl Pts',(0.323251811739511,2.0854165583293,12.0608899003674));
#39016=CARTESIAN_POINT('Ctrl Pts',(0.320625212844513,2.05636490487368,12.0593223774467));
#39017=CARTESIAN_POINT('Ctrl Pts',(0.311931257958311,2.01840243405245,12.0570572898398));
#39018=CARTESIAN_POINT('Ctrl Pts',(0.30927657115139,2.00885591194299,12.0564698452399));
#39019=CARTESIAN_POINT('Ctrl Pts',(0.30586122654522,1.99845604637467,12.0558042407609));
#39020=CARTESIAN_POINT('Ctrl Pts',(0.305530850052019,1.99746627848342,12.0557406356672));
#39021=CARTESIAN_POINT('Ctrl Pts',(0.305029731543204,1.99598891704386,12.0556453029613));
#39022=CARTESIAN_POINT('Ctrl Pts',(0.30486261210656,1.99550009455654,12.0556136950926));
#39023=CARTESIAN_POINT('Ctrl Pts',(0.304572859679391,1.9946591827585,12.0555592085317));
#39024=CARTESIAN_POINT('Ctrl Pts',(0.304450789345346,1.99430689948966,12.0555363485114));
#39025=CARTESIAN_POINT('Ctrl Pts',(0.30419767758189,1.99358052011555,12.0554891425613));
#39026=CARTESIAN_POINT('Ctrl Pts',(0.304066556779484,1.99320645248343,12.0554647940285));
#39027=CARTESIAN_POINT('Ctrl Pts',(0.303763412812162,1.99234671332916,12.0554087431974));
#39028=CARTESIAN_POINT('Ctrl Pts',(0.303590914737119,1.99186121149888,12.0553770251585));
#39029=CARTESIAN_POINT('Ctrl Pts',(0.303046059274321,1.99033927580699,12.0552773889728));
#39030=CARTESIAN_POINT('Ctrl Pts',(0.302669556041228,1.98930434394344,12.0552093329133));
#39031=CARTESIAN_POINT('Ctrl Pts',(0.301785139409619,1.98691150759013,12.0550512721788));
#39032=CARTESIAN_POINT('Ctrl Pts',(0.301273355848217,1.98555506813573,12.0549611390311));
#39033=CARTESIAN_POINT('Ctrl Pts',(0.299523426295115,1.98101011699842,12.0546573177753));
#39034=CARTESIAN_POINT('Ctrl Pts',(0.298243708771523,1.97783796053585,12.0544422438788));
#39035=CARTESIAN_POINT('Ctrl Pts',(0.295809896633002,1.9720713472433,12.0540455887641));
#39036=CARTESIAN_POINT('Ctrl Pts',(0.29467152676829,1.96947059471199,12.0538645463809));
#39037=CARTESIAN_POINT('Ctrl Pts',(0.289349290332363,1.957735821964,12.053037800909));
#39038=CARTESIAN_POINT('Ctrl Pts',(0.284774405934017,1.94878619648626,12.0523796310785));
#39039=CARTESIAN_POINT('Ctrl Pts',(0.272736844017015,1.92772768819283,12.0507664571177));
#39040=CARTESIAN_POINT('Ctrl Pts',(0.264876196253862,1.91587043053461,12.0498028038996));
#39041=CARTESIAN_POINT('Ctrl Pts',(0.24813767994117,1.89392176240011,12.0479363997521));
#39042=CARTESIAN_POINT('Ctrl Pts',(0.239359483924502,1.88378796914508,12.0470352881193));
#39043=CARTESIAN_POINT('Ctrl Pts',(0.229885608055355,1.87413765410015,12.0461568304018));
#39044=CARTESIAN_POINT('Ctrl Pts',(0.229795670977447,1.87404615142359,12.0461484991051));
#39045=CARTESIAN_POINT('Ctrl Pts',(0.229130367416071,1.87337007451341,12.0460869285154));
#39046=CARTESIAN_POINT('Ctrl Pts',(0.228552820111591,1.87278763932374,12.0460338087481));
#39047=CARTESIAN_POINT('Ctrl Pts',(0.224892119606804,1.86912403877662,12.0456992245402));
#39048=CARTESIAN_POINT('Ctrl Pts',(0.22174875870577,1.86610329715778,12.0454213116809));
#39049=CARTESIAN_POINT('Ctrl Pts',(0.21810335814314,1.86273967519813,12.0451104867994));
#39050=CARTESIAN_POINT('Ctrl Pts',(0.217660680020132,1.86233350058245,12.0450729298607));
#39051=CARTESIAN_POINT('Ctrl Pts',(0.217005210459183,1.86173544882039,12.0450176000678));
#39052=CARTESIAN_POINT('Ctrl Pts',(0.216793298041192,1.86154261671903,12.0449997550948));
#39053=CARTESIAN_POINT('Ctrl Pts',(0.216417884953318,1.86120191941071,12.0449682184425));
#39054=CARTESIAN_POINT('Ctrl Pts',(0.216254489534505,1.86105393918679,12.0449545179779));
#39055=CARTESIAN_POINT('Ctrl Pts',(0.215912759735543,1.86074508679979,12.0449259180504));
#39056=CARTESIAN_POINT('Ctrl Pts',(0.215734397737667,1.86058424667384,12.0449110210242));
#39057=CARTESIAN_POINT('Ctrl Pts',(0.215267257675232,1.86016394326313,12.0448720837695));
#39058=CARTESIAN_POINT('Ctrl Pts',(0.214978189188748,1.85990480114132,12.044848067914));
#39059=CARTESIAN_POINT('Ctrl Pts',(0.213711821596809,1.85877365726831,12.044743197888));
#39060=CARTESIAN_POINT('Ctrl Pts',(0.212729662234632,1.85790707969616,12.044662746984));
#39061=CARTESIAN_POINT('Ctrl Pts',(0.205424639930517,1.85154050472333,12.0440706370197));
#39062=CARTESIAN_POINT('Ctrl Pts',(0.19889407030068,1.84628248118893,12.0435757369528));
#39063=CARTESIAN_POINT('Ctrl Pts',(0.170912706136436,1.8254988411915,12.0415590738294));
#39064=CARTESIAN_POINT('Ctrl Pts',(0.147795140849095,1.81239117588283,12.0401266825216));
#39065=CARTESIAN_POINT('Ctrl Pts',(0.11788420284448,1.8000012067781,12.038277335202));
#39066=CARTESIAN_POINT('Ctrl Pts',(0.112374536890905,1.79789419130619,12.0379372667046));
#39067=CARTESIAN_POINT('Ctrl Pts',(0.0983432297810051,1.79296527299348,
12.0370688533339));
#39068=CARTESIAN_POINT('Ctrl Pts',(0.0897562555820195,1.7903461511095,12.0365351426031));
#39069=CARTESIAN_POINT('Ctrl Pts',(0.0800870385554768,1.78783293408209,
12.0359275320927));
#39070=CARTESIAN_POINT('Ctrl Pts',(0.0791011302280017,1.78758165555159,
12.0358655042935));
#39071=CARTESIAN_POINT('Ctrl Pts',(0.0776192087016818,1.78721142248327,
12.0357721539934));
#39072=CARTESIAN_POINT('Ctrl Pts',(0.0771240695528598,1.78708896843463,
12.035740944406));
#39073=CARTESIAN_POINT('Ctrl Pts',(0.07626817291972,1.78687944949197,12.035686961273));
#39074=CARTESIAN_POINT('Ctrl Pts',(0.0759075508650327,1.7867918310919,12.0356642056069));
#39075=CARTESIAN_POINT('Ctrl Pts',(0.0751604803441865,1.78661168540692,
12.0356170425145));
#39076=CARTESIAN_POINT('Ctrl Pts',(0.0747740106253885,1.78651924961515,
12.0355926321846));
#39077=CARTESIAN_POINT('Ctrl Pts',(0.0740078524348358,1.78633749738929,
12.0355442152473));
#39078=CARTESIAN_POINT('Ctrl Pts',(0.0736281707917203,1.78624815501775,
12.0355202095241));
#39079=CARTESIAN_POINT('Ctrl Pts',(0.0724221234276676,1.78596667141361,
12.0354439175581));
#39080=CARTESIAN_POINT('Ctrl Pts',(0.071595165802398,1.78577710516814,12.0353915486317));
#39081=CARTESIAN_POINT('Ctrl Pts',(0.0661184774266329,1.78454440771338,
12.0350443346611));
#39082=CARTESIAN_POINT('Ctrl Pts',(0.0614470571647858,1.78360129740196,
12.0347462998338));
#39083=CARTESIAN_POINT('Ctrl Pts',(0.0473622213240797,1.78108139661734,
12.0338414748463));
#39084=CARTESIAN_POINT('Ctrl Pts',(0.0378986335420009,1.7798189266956,12.0332250847503));
#39085=CARTESIAN_POINT('Ctrl Pts',(0.0177634636829779,1.77803801319208,
12.031896591862));
#39086=CARTESIAN_POINT('Ctrl Pts',(0.00709377815959828,1.77762643989674,
12.0311825477377));
#39087=CARTESIAN_POINT('Ctrl Pts',(-0.0285418148810626,1.77802188151593,
12.0287786998688));
#39088=CARTESIAN_POINT('Ctrl Pts',(-0.0533926499421487,1.78119916394683,
12.0270651365555));
#39089=CARTESIAN_POINT('Ctrl Pts',(-0.0790127093065122,1.78755768447728,
12.0253966855016));
#39090=CARTESIAN_POINT('Ctrl Pts',(-0.0803943417724939,1.78791033539869,
12.0253070424605));
#39091=CARTESIAN_POINT('Ctrl Pts',(-0.0821781723505735,1.78837827652663,
12.0251917758363));
#39092=CARTESIAN_POINT('Ctrl Pts',(-0.082582522253957,1.78848518883642,
12.0251656792093));
#39093=CARTESIAN_POINT('Ctrl Pts',(-0.0832014200565644,1.78865011848357,
12.0251257851231));
#39094=CARTESIAN_POINT('Ctrl Pts',(-0.083416116021289,1.78870757058941,
12.0251119549578));
#39095=CARTESIAN_POINT('Ctrl Pts',(-0.0838391513241743,1.78882124285904,
12.0250847223095));
#39096=CARTESIAN_POINT('Ctrl Pts',(-0.0840474924058254,1.7888774498507,
12.0250713192196));
#39097=CARTESIAN_POINT('Ctrl Pts',(-0.0845117840499707,1.78900320849143,
12.025041469623));
#39098=CARTESIAN_POINT('Ctrl Pts',(-0.0847677046050711,1.78907286668878,
12.0250250294524));
#39099=CARTESIAN_POINT('Ctrl Pts',(-0.0855078496417092,1.78927530613499,
12.024977520208));
#39100=CARTESIAN_POINT('Ctrl Pts',(-0.0859918529482133,1.78940890392279,
12.0249464985578));
#39101=CARTESIAN_POINT('Ctrl Pts',(-0.0892937978903761,1.79032863861711,
12.0247351664773));
#39102=CARTESIAN_POINT('Ctrl Pts',(-0.0921013497681738,1.79115201599534,
12.0245569813659));
#39103=CARTESIAN_POINT('Ctrl Pts',(-0.100876649826322,1.79385587943207,
12.0240036554662));
#39104=CARTESIAN_POINT('Ctrl Pts',(-0.106801380480692,1.79587207157472,
12.0236353465943));
#39105=CARTESIAN_POINT('Ctrl Pts',(-0.124372230523878,1.80242834231529,
12.0225486147373));
#39106=CARTESIAN_POINT('Ctrl Pts',(-0.135817159314458,1.80747464904349,
12.0218479521593));
#39107=CARTESIAN_POINT('Ctrl Pts',(-0.158129126622751,1.8189050158856,12.0204459340571));
#39108=CARTESIAN_POINT('Ctrl Pts',(-0.168972423408227,1.8252864791507,12.0197457025576));
#39109=CARTESIAN_POINT('Ctrl Pts',(-0.182305698061113,1.83422205232534,
12.0188335876833));
#39110=CARTESIAN_POINT('Ctrl Pts',(-0.185164806383448,1.83620599209155,
12.018634852377));
#39111=CARTESIAN_POINT('Ctrl Pts',(-0.188146863647378,1.83834761597694,
12.0184238482138));
#39112=CARTESIAN_POINT('Ctrl Pts',(-0.188302451619603,1.83845956511626,
12.0184128283133));
#39113=CARTESIAN_POINT('Ctrl Pts',(-0.190293104905162,1.83989458324062,
12.0182716960996));
#39114=CARTESIAN_POINT('Ctrl Pts',(-0.192114262601391,1.84123678117422,
12.0181410633676));
#39115=CARTESIAN_POINT('Ctrl Pts',(-0.196424308197925,1.84448387681834,
12.0178280509826));
#39116=CARTESIAN_POINT('Ctrl Pts',(-0.19889980335659,1.84640610138056,12.0176451471927));
#39117=CARTESIAN_POINT('Ctrl Pts',(-0.20725270393119,1.85308968599336,12.0170165166834));
#39118=CARTESIAN_POINT('Ctrl Pts',(-0.212989990671481,1.85802141359263,
12.0165648631693));
#39119=CARTESIAN_POINT('Ctrl Pts',(-0.219261865361007,1.86380865156669,
12.0160456431915));
#39120=CARTESIAN_POINT('Ctrl Pts',(-0.219972576534066,1.86447041753324,
12.0159864236756));
#39121=CARTESIAN_POINT('Ctrl Pts',(-0.221043380533475,1.86547655173177,
12.0158966128076));
#39122=CARTESIAN_POINT('Ctrl Pts',(-0.221405687971875,1.86581856351412,
12.0158661226934));
#39123=CARTESIAN_POINT('Ctrl Pts',(-0.22203426873031,1.86641469521266,12.0158130448627));
#39124=CARTESIAN_POINT('Ctrl Pts',(-0.222300903220632,1.86666843435003,
12.0157904736159));
#39125=CARTESIAN_POINT('Ctrl Pts',(-0.22285600012287,1.86719850000163,12.0157433651372));
#39126=CARTESIAN_POINT('Ctrl Pts',(-0.22314438450359,1.86747490704329,12.0157188244313));
#39127=CARTESIAN_POINT('Ctrl Pts',(-0.22371608023761,1.86802490180203,12.0156700412862));
#39128=CARTESIAN_POINT('Ctrl Pts',(-0.223999405455169,1.86829847412162,
12.0156457995407));
#39129=CARTESIAN_POINT('Ctrl Pts',(-0.224659066693588,1.86893776864342,
12.0155892045921));
#39130=CARTESIAN_POINT('Ctrl Pts',(-0.225035011544603,1.86930389127467,
12.0155568338936));
#39131=CARTESIAN_POINT('Ctrl Pts',(-0.22717827703285,1.87140138420925,12.0153716162313));
#39132=CARTESIAN_POINT('Ctrl Pts',(-0.228926468791885,1.87315210374666,
12.0152179192767));
#39133=CARTESIAN_POINT('Ctrl Pts',(-0.238144629100653,1.88259867437034,
12.0143931471996));
#39134=CARTESIAN_POINT('Ctrl Pts',(-0.245246334995195,1.89064290602669,
12.0137063221318));
#39135=CARTESIAN_POINT('Ctrl Pts',(-0.256415188918639,1.90464371245674,
12.0125350940816));
#39136=CARTESIAN_POINT('Ctrl Pts',(-0.260707645703019,1.91041006977626,
12.012059041826));
#39137=CARTESIAN_POINT('Ctrl Pts',(-0.280008198590011,1.93823406195168,
12.0097955623566));
#39138=CARTESIAN_POINT('Ctrl Pts',(-0.292432174307986,1.96195564328845,
12.007951472455));
#39139=CARTESIAN_POINT('Ctrl Pts',(-0.303300762439068,1.99096633662732,
12.0059507881019));
#39140=CARTESIAN_POINT('Ctrl Pts',(-0.304729646377609,1.99502600631241,
12.0056764943609));
#39141=CARTESIAN_POINT('Ctrl Pts',(-0.306247780501256,1.99963182463911,
12.0053726061509));
#39142=CARTESIAN_POINT('Ctrl Pts',(-0.306417371473822,2.00015077287905,
12.0053384700555));
#39143=CARTESIAN_POINT('Ctrl Pts',(-0.306671516496781,2.00093520191837,
12.0052870299657));
#39144=CARTESIAN_POINT('Ctrl Pts',(-0.306757045284716,2.00120036225258,
12.0052696691088));
#39145=CARTESIAN_POINT('Ctrl Pts',(-0.306904946481427,2.00166093590926,
12.0052395619487));
#39146=CARTESIAN_POINT('Ctrl Pts',(-0.306967476196906,2.0018562979155,12.0052268063435));
#39147=CARTESIAN_POINT('Ctrl Pts',(-0.307097837914521,2.00226493127482,
12.0052001573061));
#39148=CARTESIAN_POINT('Ctrl Pts',(-0.307165634245588,2.00247821346319,
12.0051862660588));
#39149=CARTESIAN_POINT('Ctrl Pts',(-0.307327216762531,2.00298838008869,
12.0051530810403));
#39150=CARTESIAN_POINT('Ctrl Pts',(-0.307420795324083,2.00328533117939,
12.0051337995716));
#39151=CARTESIAN_POINT('Ctrl Pts',(-0.307736404660327,2.00429193464956,
12.0050685544739));
#39152=CARTESIAN_POINT('Ctrl Pts',(-0.307956411812107,2.00500222646802,
12.0050227091639));
#39153=CARTESIAN_POINT('Ctrl Pts',(-0.308473906375646,2.00669364549663,
12.0049139839374));
#39154=CARTESIAN_POINT('Ctrl Pts',(-0.308769176331079,2.00767545008129,
12.0048512293244));
#39155=CARTESIAN_POINT('Ctrl Pts',(-0.312248405336297,2.01944766304421,
12.0041028513507));
#39156=CARTESIAN_POINT('Ctrl Pts',(-0.314870292802718,2.03039753573283,
12.0034475684549));
#39157=CARTESIAN_POINT('Ctrl Pts',(-0.320464631777269,2.06068495306943,
12.0016903915568));
#39158=CARTESIAN_POINT('Ctrl Pts',(-0.322258901590674,2.08018952259875,
12.0006170278004));
#39159=CARTESIAN_POINT('Ctrl Pts',(-0.322274892162095,2.09973635836811,
11.9995123401165));
#39160=CARTESIAN_POINT('',(-0.322274947886789,2.10018327456701,11.7491602604485));
#39161=CARTESIAN_POINT('Ctrl Pts',(-0.322274892430336,2.09973668646922,
11.9995123215739));
#39162=CARTESIAN_POINT('Ctrl Pts',(-0.322290032118282,2.11826646460107,
11.998465112534));
#39163=CARTESIAN_POINT('Ctrl Pts',(-0.320707131607427,2.13676088898733,
11.9973934805508));
#39164=CARTESIAN_POINT('Ctrl Pts',(-0.317403585914504,2.15582848056797,
11.9962171031456));
#39165=CARTESIAN_POINT('Ctrl Pts',(-0.317259700147515,2.15664042934577,
11.996166878222));
#39166=CARTESIAN_POINT('Ctrl Pts',(-0.317020494760566,2.15796075441193,
11.9960849888164));
#39167=CARTESIAN_POINT('Ctrl Pts',(-0.316927064028642,2.1584694726462,11.9960533843397));
#39168=CARTESIAN_POINT('Ctrl Pts',(-0.316760835545571,2.15936245995073,
11.9959978134875));
#39169=CARTESIAN_POINT('Ctrl Pts',(-0.316688562009118,2.15974682650481,
11.9959738638287));
#39170=CARTESIAN_POINT('Ctrl Pts',(-0.316541340729173,2.16052200912937,
11.9959255008523));
#39171=CARTESIAN_POINT('Ctrl Pts',(-0.316466368453675,2.16091281979292,
11.9959010867913));
#39172=CARTESIAN_POINT('Ctrl Pts',(-0.316320249528839,2.16166694758491,
11.995853914557));
#39173=CARTESIAN_POINT('Ctrl Pts',(-0.316249200246406,2.16203028315394,
11.9958311595252));
#39174=CARTESIAN_POINT('Ctrl Pts',(-0.316079443948475,2.16289051909309,
11.9957772186689));
#39175=CARTESIAN_POINT('Ctrl Pts',(-0.315980191234422,2.1633873096239,11.9957460154522));
#39176=CARTESIAN_POINT('Ctrl Pts',(-0.315628179142087,2.1651278665488,11.9956365076957));
#39177=CARTESIAN_POINT('Ctrl Pts',(-0.315369246679688,2.16637035968056,
11.995558006003));
#39178=CARTESIAN_POINT('Ctrl Pts',(-0.311603227944133,2.18392192505371,
11.994444337203));
#39179=CARTESIAN_POINT('Ctrl Pts',(-0.306842957685684,2.19993348265979,
11.9933682752765));
#39180=CARTESIAN_POINT('Ctrl Pts',(-0.300002591723112,2.21775153115264,
11.99210186751));
#39181=CARTESIAN_POINT('Ctrl Pts',(-0.29911409550308,2.2199905649123,11.9919414789931));
#39182=CARTESIAN_POINT('Ctrl Pts',(-0.291147692691763,2.23942762755785,
11.9905385877598));
#39183=CARTESIAN_POINT('Ctrl Pts',(-0.282618870641937,2.2559922311082,11.9892677428592));
#39184=CARTESIAN_POINT('Ctrl Pts',(-0.2665949560937,2.2814386367926,11.987254522305));
#39185=CARTESIAN_POINT('Ctrl Pts',(-0.259965399447129,2.29081640651409,
11.9864982388604));
#39186=CARTESIAN_POINT('Ctrl Pts',(-0.251875316259416,2.30105339186343,
11.9856727066131));
#39187=CARTESIAN_POINT('Ctrl Pts',(-0.250892691281396,2.30227827125091,
11.9855739349673));
#39188=CARTESIAN_POINT('Ctrl Pts',(-0.249639607953026,2.30381710748217,
11.9854499061954));
#39189=CARTESIAN_POINT('Ctrl Pts',(-0.249377465954066,2.30413776387588,
11.9854240648956));
#39190=CARTESIAN_POINT('Ctrl Pts',(-0.248958647495949,2.30464805879873,
11.985382947382));
#39191=CARTESIAN_POINT('Ctrl Pts',(-0.248802371927658,2.30483802346548,
11.9853676422378));
#39192=CARTESIAN_POINT('Ctrl Pts',(-0.24850656088635,2.30519676600037,11.985338741978));
#39193=CARTESIAN_POINT('Ctrl Pts',(-0.24836707203216,2.30536557917783,11.9853251437229));
#39194=CARTESIAN_POINT('Ctrl Pts',(-0.248048663944691,2.30575012634821,
11.9852941704474));
#39195=CARTESIAN_POINT('Ctrl Pts',(-0.247869635591606,2.30596576883105,
11.9852768035529));
#39196=CARTESIAN_POINT('Ctrl Pts',(-0.247334580884248,2.30660854270363,
11.9852250423686));
#39197=CARTESIAN_POINT('Ctrl Pts',(-0.246977727825137,2.30703498928574,
11.9851907081387));
#39198=CARTESIAN_POINT('Ctrl Pts',(-0.244462830659138,2.31002458643005,
11.9849500375422));
#39199=CARTESIAN_POINT('Ctrl Pts',(-0.24226593212391,2.31255498759519,11.9847464834603));
#39200=CARTESIAN_POINT('Ctrl Pts',(-0.223224836657174,2.3338077888887,11.9830335220682));
#39201=CARTESIAN_POINT('Ctrl Pts',(-0.204276648897697,2.35053310299692,
11.9816581951961));
#39202=CARTESIAN_POINT('Ctrl Pts',(-0.177410987497878,2.36915180801182,
11.9798239717321));
#39203=CARTESIAN_POINT('Ctrl Pts',(-0.171103661643706,2.3732048405163,11.9794010476863));
#39204=CARTESIAN_POINT('Ctrl Pts',(-0.157445147313083,2.38132305914348,
11.9784929139338));
#39205=CARTESIAN_POINT('Ctrl Pts',(-0.150064969971981,2.38532810505858,
11.9780066503481));
#39206=CARTESIAN_POINT('Ctrl Pts',(-0.138639245049303,2.39096258331196,
11.9772541433389));
#39207=CARTESIAN_POINT('Ctrl Pts',(-0.134702900288916,2.39280572252739,
11.9769949698291));
#39208=CARTESIAN_POINT('Ctrl Pts',(-0.129147863052701,2.39527106805049,
11.9766287446207));
#39209=CARTESIAN_POINT('Ctrl Pts',(-0.127559494214819,2.39596072275757,
11.976523976498));
#39210=CARTESIAN_POINT('Ctrl Pts',(-0.124795705033128,2.39713435222583,
11.9763415507626));
#39211=CARTESIAN_POINT('Ctrl Pts',(-0.123622826445872,2.39762423956485,
11.9762640947415));
#39212=CARTESIAN_POINT('Ctrl Pts',(-0.122050622481403,2.39827002009293,
11.9761602049899));
#39213=CARTESIAN_POINT('Ctrl Pts',(-0.121653828529178,2.39843207826192,
11.9761339799187));
#39214=CARTESIAN_POINT('Ctrl Pts',(-0.120916895736116,2.3987313416272,11.9760852639237));
#39215=CARTESIAN_POINT('Ctrl Pts',(-0.120576843290157,2.39886875883114,
11.9760627801999));
#39216=CARTESIAN_POINT('Ctrl Pts',(-0.119872197041766,2.39915211218997,
11.9760161813597));
#39217=CARTESIAN_POINT('Ctrl Pts',(-0.119507569749674,2.39929796294278,
11.9759920634093));
#39218=CARTESIAN_POINT('Ctrl Pts',(-0.118679023955847,2.39962762540449,
11.9759372485525));
#39219=CARTESIAN_POINT('Ctrl Pts',(-0.118214944108632,2.39981102651099,
11.9759065378809));
#39220=CARTESIAN_POINT('Ctrl Pts',(-0.11684074205851,2.40035041480111,11.9758155744021));
#39221=CARTESIAN_POINT('Ctrl Pts',(-0.115929430559339,2.4007033384791,11.9757552188162));
#39222=CARTESIAN_POINT('Ctrl Pts',(-0.109744237766218,2.40306638271131,
11.9753453398858));
#39223=CARTESIAN_POINT('Ctrl Pts',(-0.104420227298461,2.40494169881607,
11.9749913361187));
#39224=CARTESIAN_POINT('Ctrl Pts',(-0.0974708942640044,2.40718618789567,
11.9745273348628));
#39225=CARTESIAN_POINT('Ctrl Pts',(-0.095887912713916,2.40768398933973,
11.9744215150012));
#39226=CARTESIAN_POINT('Ctrl Pts',(-0.0914388700455854,2.40904541519539,
11.9741237455252));
#39227=CARTESIAN_POINT('Ctrl Pts',(-0.0885645721769404,2.40988135027313,
11.9739309561341));
#39228=CARTESIAN_POINT('Ctrl Pts',(-0.0820986371681164,2.41166453804147,
11.9734963474253));
#39229=CARTESIAN_POINT('Ctrl Pts',(-0.078501463073567,2.4125899697296,11.9732539345335));
#39230=CARTESIAN_POINT('Ctrl Pts',(-0.0721577895715706,2.41410558018112,
11.9728254524368));
#39231=CARTESIAN_POINT('Ctrl Pts',(-0.0694180200938113,2.41472241732074,
11.9726400777879));
#39232=CARTESIAN_POINT('Ctrl Pts',(-0.0497333249290104,2.41888472719661,
11.9713062976586));
#39233=CARTESIAN_POINT('Ctrl Pts',(-0.0325357846113654,2.42109535475346,
11.9701288366965));
#39234=CARTESIAN_POINT('Ctrl Pts',(-0.0129550453979711,2.42202266975356,
11.9688060154347));
#39235=CARTESIAN_POINT('Ctrl Pts',(-0.0106635950950383,2.42210669188842,
11.968651522797));
#39236=CARTESIAN_POINT('Ctrl Pts',(-0.00554141373540266,2.42223979072454,
11.9683070914584));
#39237=CARTESIAN_POINT('Ctrl Pts',(-0.00271051037756672,2.42227603640808,
11.9681173549484));
#39238=CARTESIAN_POINT('Ctrl Pts',(0.00803423608660622,2.4222720173494,
11.9674003142077));
#39239=CARTESIAN_POINT('Ctrl Pts',(0.0159457664539845,2.42197756729501,
11.9668786904721));
#39240=CARTESIAN_POINT('Ctrl Pts',(0.0276290591701246,2.42111096898884,
11.9661249527688));
#39241=CARTESIAN_POINT('Ctrl Pts',(0.0314140744901395,2.42076280706022,
11.9658833633901));
#39242=CARTESIAN_POINT('Ctrl Pts',(0.0357254596148987,2.42028917388723,
11.9656118155341));
#39243=CARTESIAN_POINT('Ctrl Pts',(0.0362585317030203,2.42022926515651,
11.9655783042387));
#39244=CARTESIAN_POINT('Ctrl Pts',(0.0370620921066239,2.42013692564997,
11.9655278874057));
#39245=CARTESIAN_POINT('Ctrl Pts',(0.0373326895944099,2.4201054828098,11.9655109264933));
#39246=CARTESIAN_POINT('Ctrl Pts',(0.0378200001968005,2.42004823205267,
11.9654804128906));
#39247=CARTESIAN_POINT('Ctrl Pts',(0.0380367264602394,2.42002254716826,
11.9654668532796));
#39248=CARTESIAN_POINT('Ctrl Pts',(0.0384704854097021,2.41997069422731,
11.9654397369456));
#39249=CARTESIAN_POINT('Ctrl Pts',(0.038687516599473,2.41994452561657,11.9654261803138));
#39250=CARTESIAN_POINT('Ctrl Pts',(0.0393017456622678,2.41986983060792,
11.9653878438923));
#39251=CARTESIAN_POINT('Ctrl Pts',(0.0396988817924841,2.41982078502464,
11.9653630935129));
#39252=CARTESIAN_POINT('Ctrl Pts',(0.0413596164800909,2.41961254632039,
11.9652597415022));
#39253=CARTESIAN_POINT('Ctrl Pts',(0.0426223791567534,2.41944660048657,
11.965181516215));
#39254=CARTESIAN_POINT('Ctrl Pts',(0.0656285555145804,2.41628439778233,
11.9637623600202));
#39255=CARTESIAN_POINT('Ctrl Pts',(0.0870146435547348,2.41108150852532,
11.9625391361374));
#39256=CARTESIAN_POINT('Ctrl Pts',(0.118644368864585,2.39986550952689,11.9606632941634));
#39257=CARTESIAN_POINT('Ctrl Pts',(0.129362706452983,2.39539987749009,11.9600154592711));
#39258=CARTESIAN_POINT('Ctrl Pts',(0.149846322273975,2.38553664431393,11.9587220616112));
#39259=CARTESIAN_POINT('Ctrl Pts',(0.159618264070581,2.38019113242853,11.9580783635133));
#39260=CARTESIAN_POINT('Ctrl Pts',(0.172112886572602,2.37249020127256,11.9572064947208));
#39261=CARTESIAN_POINT('Ctrl Pts',(0.175101251650892,2.37057957370505,11.9569941250499));
#39262=CARTESIAN_POINT('Ctrl Pts',(0.179298777869239,2.36779720318224,11.9566900088476));
#39263=CARTESIAN_POINT('Ctrl Pts',(0.180534430457346,2.36696575263963,11.9565997545202));
#39264=CARTESIAN_POINT('Ctrl Pts',(0.18269063448116,2.36549306242653,11.956440952947));
#39265=CARTESIAN_POINT('Ctrl Pts',(0.183613689926892,2.36485552088893,11.9563725457064));
#39266=CARTESIAN_POINT('Ctrl Pts',(0.184960819494214,2.36391465039563,11.9562720776961));
#39267=CARTESIAN_POINT('Ctrl Pts',(0.185387523140706,2.36361508625291,11.9562401607777));
#39268=CARTESIAN_POINT('Ctrl Pts',(0.186138175792319,2.36308537216911,11.9561838467203));
#39269=CARTESIAN_POINT('Ctrl Pts',(0.186462430353594,2.36285565544799,11.9561594662344));
#39270=CARTESIAN_POINT('Ctrl Pts',(0.187088670521513,2.36241025647235,11.9561122730182));
#39271=CARTESIAN_POINT('Ctrl Pts',(0.187390710258606,2.36219465106362,11.9560894632697));
#39272=CARTESIAN_POINT('Ctrl Pts',(0.188106955742959,2.36168150283269,11.9560352582659));
#39273=CARTESIAN_POINT('Ctrl Pts',(0.188520827984663,2.36138349820688,11.9560038452117));
#39274=CARTESIAN_POINT('Ctrl Pts',(0.189758048427826,2.36048818277634,11.9559096642018));
#39275=CARTESIAN_POINT('Ctrl Pts',(0.190579272037186,2.35988795920743,11.9558467834665));
#39276=CARTESIAN_POINT('Ctrl Pts',(0.198611418216968,2.35395880594021,11.9552281264419));
#39277=CARTESIAN_POINT('Ctrl Pts',(0.205599182870998,2.34833550035663,11.9546608298194));
#39278=CARTESIAN_POINT('Ctrl Pts',(0.215792649082532,2.33940705662627,11.9537867181084));
#39279=CARTESIAN_POINT('Ctrl Pts',(0.219177335534874,2.33631229050391,11.9534881547959));
#39280=CARTESIAN_POINT('Ctrl Pts',(0.240198806576647,2.31625122664893,11.9515807817846));
#39281=CARTESIAN_POINT('Ctrl Pts',(0.255919977060544,2.2973950444249,11.9499025030514));
#39282=CARTESIAN_POINT('Ctrl Pts',(0.274221513907964,2.26953564094756,11.9476714303976));
#39283=CARTESIAN_POINT('Ctrl Pts',(0.278781701335296,2.26192764082981,11.9470852370471));
#39284=CARTESIAN_POINT('Ctrl Pts',(0.284876502130722,2.2507367822357,11.9462649820303));
#39285=CARTESIAN_POINT('Ctrl Pts',(0.286668896460554,2.2472995116246,11.9460185119031));
#39286=CARTESIAN_POINT('Ctrl Pts',(0.288639446878408,2.24334830220079,11.945742071343));
#39287=CARTESIAN_POINT('Ctrl Pts',(0.288878748693808,2.24286544229179,11.9457084045001));
#39288=CARTESIAN_POINT('Ctrl Pts',(0.289237420356777,2.2421371337116,11.9456578007575));
#39289=CARTESIAN_POINT('Ctrl Pts',(0.289357689908607,2.24189213299711,11.9456408078689));
#39290=CARTESIAN_POINT('Ctrl Pts',(0.289573588557877,2.24145091050229,11.9456102597804));
#39291=CARTESIAN_POINT('Ctrl Pts',(0.289669329322274,2.24125474478102,11.9455966975893));
#39292=CARTESIAN_POINT('Ctrl Pts',(0.289874623182387,2.2408330264342,11.9455675831521));
#39293=CARTESIAN_POINT('Ctrl Pts',(0.28998411203079,2.24060744386585,11.9455520349794));
#39294=CARTESIAN_POINT('Ctrl Pts',(0.290278236130656,2.23999964796404,11.9455102109881));
#39295=CARTESIAN_POINT('Ctrl Pts',(0.290462380528173,2.23961719558844,11.9454839658433));
#39296=CARTESIAN_POINT('Ctrl Pts',(0.291305975726576,2.2378562269276,11.9453634499451));
#39297=CARTESIAN_POINT('Ctrl Pts',(0.291956386253598,2.23647336567625,11.9452697327507));
#39298=CARTESIAN_POINT('Ctrl Pts',(0.304726851911641,2.2088124524726,11.9434124367505));
#39299=CARTESIAN_POINT('Ctrl Pts',(0.313265033822044,2.18102005787011,11.9418480231226));
#39300=CARTESIAN_POINT('Ctrl Pts',(0.319877595125289,2.14093683388401,11.9395615871811));
#39301=CARTESIAN_POINT('Ctrl Pts',(0.321150507915636,2.12932269053951,11.9388969874046));
#39302=CARTESIAN_POINT('Ctrl Pts',(0.322233993380862,2.10958648611679,11.9377420710263));
#39303=CARTESIAN_POINT('Ctrl Pts',(0.322373073651035,2.10149394643532,11.9372613957773));
#39304=CARTESIAN_POINT('Ctrl Pts',(0.322173910703158,2.09176324702142,11.9366715175432));
#39305=CARTESIAN_POINT('Ctrl Pts',(0.32212775328657,2.09012157682071,11.9365715954554));
#39306=CARTESIAN_POINT('Ctrl Pts',(0.322047378265076,2.08787443243656,11.9364342451967));
#39307=CARTESIAN_POINT('Ctrl Pts',(0.322023996115217,2.08726857611234,11.9363971567013));
#39308=CARTESIAN_POINT('Ctrl Pts',(0.321983755255769,2.08629704494426,11.9363375897542));
#39309=CARTESIAN_POINT('Ctrl Pts',(0.321967982872494,2.08593132454236,11.9363151453895));
#39310=CARTESIAN_POINT('Ctrl Pts',(0.321933864762426,2.08517033656856,11.9362683989866));
#39311=CARTESIAN_POINT('Ctrl Pts',(0.321915414108091,2.08477507452373,11.9362440936967));
#39312=CARTESIAN_POINT('Ctrl Pts',(0.32187139489396,2.08386793737798,11.9361882547772));
#39313=CARTESIAN_POINT('Ctrl Pts',(0.321845333184344,2.08335608825896,11.9361567057334));
#39314=CARTESIAN_POINT('Ctrl Pts',(0.321772795567957,2.0819953788594,11.9360727220935));
#39315=CARTESIAN_POINT('Ctrl Pts',(0.321724181835174,2.0811466408737,11.9360202205443));
#39316=CARTESIAN_POINT('Ctrl Pts',(0.321374123720412,2.07543125128269,11.9356658759686));
#39317=CARTESIAN_POINT('Ctrl Pts',(0.320965637089675,2.07057201302788,11.9353606890644));
#39318=CARTESIAN_POINT('Ctrl Pts',(0.317382656091595,2.03707452902304,11.9332282390498));
#39319=CARTESIAN_POINT('Ctrl Pts',(0.310490344103112,2.00897009183596,11.9312768499659));
#39320=CARTESIAN_POINT('Ctrl Pts',(0.293935448393333,1.96682886709923,11.928219449767));
#39321=CARTESIAN_POINT('Ctrl Pts',(0.286743730421849,1.95197712001772,11.9271176273678));
#39322=CARTESIAN_POINT('Ctrl Pts',(0.277838680573019,1.93669567842793,11.9260022555656));
#39323=CARTESIAN_POINT('Ctrl Pts',(0.277224811596123,1.935655733864,11.9259264530588));
#39324=CARTESIAN_POINT('Ctrl Pts',(0.276411782096375,1.93429591357351,11.9258274934217));
#39325=CARTESIAN_POINT('Ctrl Pts',(0.27621789595906,1.93397291939105,11.9258039996525));
#39326=CARTESIAN_POINT('Ctrl Pts',(0.275900799351741,1.93344676227582,11.9257657485936));
#39327=CARTESIAN_POINT('Ctrl Pts',(0.275777930468778,1.93324339549339,11.9257509689941));
#39328=CARTESIAN_POINT('Ctrl Pts',(0.275540149903792,1.93285081387444,11.9257224481303));
#39329=CARTESIAN_POINT('Ctrl Pts',(0.275425268459795,1.93266158203951,11.9257087049925));
#39330=CARTESIAN_POINT('Ctrl Pts',(0.275158244064802,1.93222276140732,11.9256768452976));
#39331=CARTESIAN_POINT('Ctrl Pts',(0.275005955934355,1.93197326025641,11.9256587383154));
#39332=CARTESIAN_POINT('Ctrl Pts',(0.274511638028437,1.93116586708348,11.9256001668896));
#39333=CARTESIAN_POINT('Ctrl Pts',(0.274168245624862,1.93060880495312,11.925559791547));
#39334=CARTESIAN_POINT('Ctrl Pts',(0.270822938636907,1.92521876355081,11.9251694378927));
#39335=CARTESIAN_POINT('Ctrl Pts',(0.267695012077192,1.92046466943811,11.9248275714058));
#39336=CARTESIAN_POINT('Ctrl Pts',(0.263723836559744,1.91476367782538,11.9244174082025));
#39337=CARTESIAN_POINT('Ctrl Pts',(0.262999016781653,1.91373600917549,11.9243434634037));
#39338=CARTESIAN_POINT('Ctrl Pts',(0.259908487766431,1.90940818233584,11.9240319053703));
#39339=CARTESIAN_POINT('Ctrl Pts',(0.257486461069764,1.90614854232988,11.923796862455));
#39340=CARTESIAN_POINT('Ctrl Pts',(0.241403616829571,1.88533719064967,11.9222876757143));
#39341=CARTESIAN_POINT('Ctrl Pts',(0.226018265692793,1.86919343733556,11.9210727650098));
#39342=CARTESIAN_POINT('Ctrl Pts',(0.203039153480014,1.8496012106097,11.919360444021));
#39343=CARTESIAN_POINT('Ctrl Pts',(0.196797310161656,1.84466637698704,11.9189045709676));
#39344=CARTESIAN_POINT('Ctrl Pts',(0.18346821157641,1.834907634253,11.9179415332678));
#39345=CARTESIAN_POINT('Ctrl Pts',(0.176358382874251,1.8301254954577,11.9174334940673));
#39346=CARTESIAN_POINT('Ctrl Pts',(0.168091796792566,1.82503157355596,11.9168452059578));
#39347=CARTESIAN_POINT('Ctrl Pts',(0.167113432252009,1.82443587243894,11.9167756205313));
#39348=CARTESIAN_POINT('Ctrl Pts',(0.165352478042518,1.82337649948574,11.9166504341912));
#39349=CARTESIAN_POINT('Ctrl Pts',(0.164571058276077,1.8229108991988,11.9165949041077));
#39350=CARTESIAN_POINT('Ctrl Pts',(0.16337790477558,1.82220679948755,11.9165101429544));
#39351=CARTESIAN_POINT('Ctrl Pts',(0.162967592202825,1.82196589074799,11.916480999531));
#39352=CARTESIAN_POINT('Ctrl Pts',(0.1622509499628,1.82154725663906,11.9164301064376));
#39353=CARTESIAN_POINT('Ctrl Pts',(0.161944857281851,1.82136912545912,11.916408371524));
#39354=CARTESIAN_POINT('Ctrl Pts',(0.161310069617872,1.82100110903089,11.9163633018003));
#39355=CARTESIAN_POINT('Ctrl Pts',(0.160981331649354,1.82081129933216,11.9163399642999));
#39356=CARTESIAN_POINT('Ctrl Pts',(0.160182699637211,1.82035205747829,11.9162832748212));
#39357=CARTESIAN_POINT('Ctrl Pts',(0.159712461410356,1.8200832290051,11.9162499011231));
#39358=CARTESIAN_POINT('Ctrl Pts',(0.157950626792031,1.81908189822436,11.9161248785518));
#39359=CARTESIAN_POINT('Ctrl Pts',(0.156654666138279,1.81835714838134,11.9160329514677));
#39360=CARTESIAN_POINT('Ctrl Pts',(0.133439502823702,1.80558416115297,11.9143867113656));
#39361=CARTESIAN_POINT('Ctrl Pts',(0.110200969260311,1.79612169339898,11.9127363379));
#39362=CARTESIAN_POINT('Ctrl Pts',(0.0707623468615258,1.78518663572277,
11.9099726590372));
#39363=CARTESIAN_POINT('Ctrl Pts',(0.0551221973562432,1.78207494965335,
11.9088882984734));
#39364=CARTESIAN_POINT('Ctrl Pts',(0.0315516128561676,1.779177831656,11.9073169586769));
#39365=CARTESIAN_POINT('Ctrl Pts',(0.0237545825445637,1.77850643877727,
11.9068074961154));
#39366=CARTESIAN_POINT('Ctrl Pts',(0.0142754796270235,1.778037013981,11.9062065198696));
#39367=CARTESIAN_POINT('Ctrl Pts',(0.0126101110209586,1.77796748755945,
11.9061016240386));
#39368=CARTESIAN_POINT('Ctrl Pts',(0.0105217368608655,1.77789652688921,
11.9059710106224));
#39369=CARTESIAN_POINT('Ctrl Pts',(0.0100992070245002,1.77788300206456,
11.9059446317987));
#39370=CARTESIAN_POINT('Ctrl Pts',(0.00942886095272575,1.77786286513284,
11.9059028583119));
#39371=CARTESIAN_POINT('Ctrl Pts',(0.00918106346136307,1.77785570755638,
11.9058874331075));
#39372=CARTESIAN_POINT('Ctrl Pts',(0.00871468133577316,1.77784277477254,
11.9058584327669));
#39373=CARTESIAN_POINT('Ctrl Pts',(0.00849610084225586,1.7778369361521,
11.9058448542011));
#39374=CARTESIAN_POINT('Ctrl Pts',(0.00800045058094651,1.77782420135971,
11.9058140931454));
#39375=CARTESIAN_POINT('Ctrl Pts',(0.00772337830367184,1.77781744015548,
11.9057969183637));
#39376=CARTESIAN_POINT('Ctrl Pts',(0.00700960772429537,1.77780094378876,
11.9057527271239));
#39377=CARTESIAN_POINT('Ctrl Pts',(0.00657289594078645,1.77779173898219,
11.9057257403628));
#39378=CARTESIAN_POINT('Ctrl Pts',(0.00400707394892082,1.77774287649343,
11.9055674776781));
#39379=CARTESIAN_POINT('Ctrl Pts',(0.00187756722605931,1.77772343304744,
11.9054373134188));
#39380=CARTESIAN_POINT('Ctrl Pts',(-0.00065529111074268,1.77772541392767,
11.9052837398627));
#39381=CARTESIAN_POINT('Ctrl Pts',(-0.00105854100558473,1.77772648615029,
11.9052593273473));
#39382=CARTESIAN_POINT('Ctrl Pts',(-0.0366183193238867,1.77788778151695,
11.9031097860917));
#39383=CARTESIAN_POINT('Ctrl Pts',(-0.0715175642871153,1.78379852313034,
11.9012563065549));
#39384=CARTESIAN_POINT('Ctrl Pts',(-0.116042493295097,1.7991059675031,11.898551640593));
#39385=CARTESIAN_POINT('Ctrl Pts',(-0.127083108591905,1.80360007727022,
11.897853004082));
#39386=CARTESIAN_POINT('Ctrl Pts',(-0.139739951603399,1.80958943099496,
11.8970066206193));
#39387=CARTESIAN_POINT('Ctrl Pts',(-0.14162224708126,1.81050269176417,11.8968795397269));
#39388=CARTESIAN_POINT('Ctrl Pts',(-0.144093078184212,1.8117313650917,11.8967110762267));
#39389=CARTESIAN_POINT('Ctrl Pts',(-0.144689744782218,1.81203038563627,
11.8966702672072));
#39390=CARTESIAN_POINT('Ctrl Pts',(-0.145664783290114,1.81252282332818,
11.8966033683572));
#39391=CARTESIAN_POINT('Ctrl Pts',(-0.146043711151618,1.8127151402728,11.8965773171863));
#39392=CARTESIAN_POINT('Ctrl Pts',(-0.146775110598325,1.8130881678518,11.8965269319488));
#39393=CARTESIAN_POINT('Ctrl Pts',(-0.147127631751823,1.81326878005585,
11.8965026013804));
#39394=CARTESIAN_POINT('Ctrl Pts',(-0.147937782849754,1.81368574377397,
11.8964465798531));
#39395=CARTESIAN_POINT('Ctrl Pts',(-0.148395180061732,1.81392254293234,
11.8964148731453));
#39396=CARTESIAN_POINT('Ctrl Pts',(-0.149613656567506,1.81455706906073,
11.8963301993365));
#39397=CARTESIAN_POINT('Ctrl Pts',(-0.150373713274924,1.81495674119924,
11.8962771635227));
#39398=CARTESIAN_POINT('Ctrl Pts',(-0.155575117868523,1.81771846815806,
11.8959127037637));
#39399=CARTESIAN_POINT('Ctrl Pts',(-0.159962018908159,1.82018107924266,
11.8955977164679));
#39400=CARTESIAN_POINT('Ctrl Pts',(-0.174994238743154,1.82908852910586,
11.8944908398537));
#39401=CARTESIAN_POINT('Ctrl Pts',(-0.185321587955848,1.83604573378236,
11.8936806876661));
#39402=CARTESIAN_POINT('Ctrl Pts',(-0.200867946695899,1.84788170905821,
11.8923831625068));
#39403=CARTESIAN_POINT('Ctrl Pts',(-0.20637206961328,1.85236695200649,11.8919070608736));
#39404=CARTESIAN_POINT('Ctrl Pts',(-0.221380114951674,1.86544492897593,
11.8905648244737));
#39405=CARTESIAN_POINT('Ctrl Pts',(-0.230526544731307,1.8744279470857,11.8896938002725));
#39406=CARTESIAN_POINT('Ctrl Pts',(-0.245737109347077,1.89126085027975,
11.8881718151932));
#39407=CARTESIAN_POINT('Ctrl Pts',(-0.252020209061949,1.89889155219584,
11.8875170386819));
#39408=CARTESIAN_POINT('Ctrl Pts',(-0.260202234508694,1.90981542739261,
11.8866391297362));
#39409=CARTESIAN_POINT('Ctrl Pts',(-0.262408250939913,1.91287093380066,
11.8863996301579));
#39410=CARTESIAN_POINT('Ctrl Pts',(-0.264865990412456,1.91640405958182,
11.8861301793369));
#39411=CARTESIAN_POINT('Ctrl Pts',(-0.265170604581527,1.91684429386207,
11.8860967359273));
#39412=CARTESIAN_POINT('Ctrl Pts',(-0.265628443912795,1.91750950847004,
11.8860464006907));
#39413=CARTESIAN_POINT('Ctrl Pts',(-0.265782481415698,1.91773392447248,
11.8860294537558));
#39414=CARTESIAN_POINT('Ctrl Pts',(-0.266059503015643,1.91813861294209,
11.8859989552017));
#39415=CARTESIAN_POINT('Ctrl Pts',(-0.266182588033365,1.91831881474309,
11.8859853966925));
#39416=CARTESIAN_POINT('Ctrl Pts',(-0.266447006046569,1.91870677968211,
11.8859562533954));
#39417=CARTESIAN_POINT('Ctrl Pts',(-0.26658827868847,1.91891458249941,11.8859406727577));
#39418=CARTESIAN_POINT('Ctrl Pts',(-0.266968811070454,1.91947573116585,
11.8858986769967));
#39419=CARTESIAN_POINT('Ctrl Pts',(-0.267207613336945,1.91982938890535,
11.8858722929777));
#39420=CARTESIAN_POINT('Ctrl Pts',(-0.268310350832387,1.92146951900206,
11.8857503142456));
#39421=CARTESIAN_POINT('Ctrl Pts',(-0.269165721194187,1.92276176549964,
11.8856552895133));
#39422=CARTESIAN_POINT('Ctrl Pts',(-0.28737175625935,1.95070224543244,11.8836227082783));
#39423=CARTESIAN_POINT('Ctrl Pts',(-0.300696424273517,1.97977187474693,
11.8819234881039));
#39424=CARTESIAN_POINT('Ctrl Pts',(-0.313957892892305,2.02554999157407,
11.8792231192045));
#39425=CARTESIAN_POINT('Ctrl Pts',(-0.317238355945099,2.04107556579118,
11.8783059865185));
#39426=CARTESIAN_POINT('Ctrl Pts',(-0.319697177946093,2.05924365070786,
11.8772003247134));
#39427=CARTESIAN_POINT('Ctrl Pts',(-0.320002281765058,2.06171286477267,
11.877049409315));
#39428=CARTESIAN_POINT('Ctrl Pts',(-0.320357813053041,2.0648922619779,11.876854181309));
#39429=CARTESIAN_POINT('Ctrl Pts',(-0.320434525303831,2.06559946753773,
11.8768106984734));
#39430=CARTESIAN_POINT('Ctrl Pts',(-0.320554346822314,2.06673928197126,
11.8767405218595));
#39431=CARTESIAN_POINT('Ctrl Pts',(-0.320598923534733,2.06717173693439,
11.8767138743448));
#39432=CARTESIAN_POINT('Ctrl Pts',(-0.320682150337311,2.06799548956898,
11.8766630731254));
#39433=CARTESIAN_POINT('Ctrl Pts',(-0.320720959654002,2.06838677065958,
11.8766389244815));
#39434=CARTESIAN_POINT('Ctrl Pts',(-0.320807797281842,2.06927890001303,
11.8765838232452));
#39435=CARTESIAN_POINT('Ctrl Pts',(-0.320855368868727,2.06977979078873,
11.8765528563386));
#39436=CARTESIAN_POINT('Ctrl Pts',(-0.320996839248251,2.07130735806691,
11.8764583238351));
#39437=CARTESIAN_POINT('Ctrl Pts',(-0.321086983976121,2.07233436807111,
11.8763946403649));
#39438=CARTESIAN_POINT('Ctrl Pts',(-0.321706261765551,2.07980088929458,
11.8759307027241));
#39439=CARTESIAN_POINT('Ctrl Pts',(-0.322046527493159,2.08625418908253,
11.8755245499221));
#39440=CARTESIAN_POINT('Ctrl Pts',(-0.322248915265885,2.0952027048059,11.8749536251292));
#39441=CARTESIAN_POINT('Ctrl Pts',(-0.322276363226365,2.09769292396946,
11.8747939240554));
#39442=CARTESIAN_POINT('Ctrl Pts',(-0.322270555415569,2.10791201595138,
11.8741351782895));
#39443=CARTESIAN_POINT('Ctrl Pts',(-0.321988134303093,2.11563770899795,
11.8736291397252));
#39444=CARTESIAN_POINT('Ctrl Pts',(-0.319228571217128,2.15363251957197,
11.8711043324824));
#39445=CARTESIAN_POINT('Ctrl Pts',(-0.312759663303515,2.18345402603753,
11.8689914748367));
#39446=CARTESIAN_POINT('Ctrl Pts',(-0.300887051948024,2.21551082881476,
11.8667907638231));
#39447=CARTESIAN_POINT('Ctrl Pts',(-0.299496599585889,2.21906955794002,
11.8665477661154));
#39448=CARTESIAN_POINT('Ctrl Pts',(-0.297820304106974,2.22314457004338,
11.8662717236344));
#39449=CARTESIAN_POINT('Ctrl Pts',(-0.297596008258828,2.22368562790708,
11.8662351175877));
#39450=CARTESIAN_POINT('Ctrl Pts',(-0.297261395007878,2.22448661932958,
11.8661809959303));
#39451=CARTESIAN_POINT('Ctrl Pts',(-0.297152210597528,2.22474702037566,
11.8661634121434));
#39452=CARTESIAN_POINT('Ctrl Pts',(-0.296957647339344,2.22520934219326,
11.8661322136254));
#39453=CARTESIAN_POINT('Ctrl Pts',(-0.296872404712535,2.22541131929409,
11.8661185906067));
#39454=CARTESIAN_POINT('Ctrl Pts',(-0.296691548199762,2.22583862987168,
11.8660897838495));
#39455=CARTESIAN_POINT('Ctrl Pts',(-0.29659588393765,2.2260639408132,11.8660746032867));
#39456=CARTESIAN_POINT('Ctrl Pts',(-0.296339774721068,2.22666523060811,
11.8660341130841));
#39457=CARTESIAN_POINT('Ctrl Pts',(-0.296178870294943,2.22704101511689,
11.8660088315012));
#39458=CARTESIAN_POINT('Ctrl Pts',(-0.295419290077363,2.2288056912485,11.8658902148768));
#39459=CARTESIAN_POINT('Ctrl Pts',(-0.294811544391363,2.23019069303091,
11.8657974254289));
#39460=CARTESIAN_POINT('Ctrl Pts',(-0.289818244037389,2.24135572833373,
11.8650514974071));
#39461=CARTESIAN_POINT('Ctrl Pts',(-0.284956528384057,2.25091681558778,
11.8644256341339));
#39462=CARTESIAN_POINT('Ctrl Pts',(-0.265242888201808,2.28532265671748,
11.8621581376671));
#39463=CARTESIAN_POINT('Ctrl Pts',(-0.247544435414865,2.30837503945137,
11.8605954716918));
#39464=CARTESIAN_POINT('Ctrl Pts',(-0.220045814899674,2.33566324066035,
11.8583413584187));
#39465=CARTESIAN_POINT('Ctrl Pts',(-0.212774722407434,2.34224824413426,
11.857759612165));
#39466=CARTESIAN_POINT('Ctrl Pts',(-0.20441278130814,2.34915391581625,11.8571001647116));
#39467=CARTESIAN_POINT('Ctrl Pts',(-0.203607056224353,2.34981278098728,
11.8570367193307));
#39468=CARTESIAN_POINT('Ctrl Pts',(-0.202397177231539,2.35079239316756,
11.8569415871785));
#39469=CARTESIAN_POINT('Ctrl Pts',(-0.201995416286347,2.35111609589277,
11.8569100194504));
#39470=CARTESIAN_POINT('Ctrl Pts',(-0.201302132478617,2.35167194114552,
11.8568555836928));
#39471=CARTESIAN_POINT('Ctrl Pts',(-0.20101098023509,2.3519045460555,11.856832734255));
#39472=CARTESIAN_POINT('Ctrl Pts',(-0.200409235424575,2.35238357945124,
11.8567855329958));
#39473=CARTESIAN_POINT('Ctrl Pts',(-0.200098590349256,2.35262994073968,
11.8567611785416));
#39474=CARTESIAN_POINT('Ctrl Pts',(-0.199374434279252,2.35320206890304,
11.8567044341658));
#39475=CARTESIAN_POINT('Ctrl Pts',(-0.19896057903664,2.35352739639951,11.8566720268184));
#39476=CARTESIAN_POINT('Ctrl Pts',(-0.197638999398129,2.35456104814156,
11.8565686080163));
#39477=CARTESIAN_POINT('Ctrl Pts',(-0.196728283014751,2.3552655165136,11.8564974439261));
#39478=CARTESIAN_POINT('Ctrl Pts',(-0.176932844179349,2.37040906841153,
11.8549527444143));
#39479=CARTESIAN_POINT('Ctrl Pts',(-0.156515893223953,2.38271651318578,
11.8533929135579));
#39480=CARTESIAN_POINT('Ctrl Pts',(-0.113880288591816,2.40237402684906,
11.8502296219761));
#39481=CARTESIAN_POINT('Ctrl Pts',(-0.0918373759162351,2.40978183189838,
11.848638928633));
#39482=CARTESIAN_POINT('Ctrl Pts',(-0.0655494903571434,2.41556034238662,
11.846907275142));
#39483=CARTESIAN_POINT('Ctrl Pts',(-0.0618956947351822,2.41629731474561,
11.8466703110782));
#39484=CARTESIAN_POINT('Ctrl Pts',(-0.0576578814998444,2.41707583066751,
11.8464003970775));
#39485=CARTESIAN_POINT('Ctrl Pts',(-0.0570857268370138,2.41717933964332,
11.8463640589082));
#39486=CARTESIAN_POINT('Ctrl Pts',(-0.0562361318703206,2.41733066720835,
11.8463102567767));
#39487=CARTESIAN_POINT('Ctrl Pts',(-0.055958908008866,2.41737967089047,
11.8462927257952));
#39488=CARTESIAN_POINT('Ctrl Pts',(-0.055465785993254,2.41746617178284,
11.8462615863096));
#39489=CARTESIAN_POINT('Ctrl Pts',(-0.0552499138917325,2.41750381203751,
11.8462479696333));
#39490=CARTESIAN_POINT('Ctrl Pts',(-0.0547923474488468,2.41758311421874,
11.8462191396645));
#39491=CARTESIAN_POINT('Ctrl Pts',(-0.0545506445750195,2.41762472031194,
11.8462039296216));
#39492=CARTESIAN_POINT('Ctrl Pts',(-0.0539038505679594,2.41773529765177,
11.8461632779111));
#39493=CARTESIAN_POINT('Ctrl Pts',(-0.0534986729228843,2.41780377039904,
11.8461378646954));
#39494=CARTESIAN_POINT('Ctrl Pts',(-0.0515792134044037,2.41812437344344,
11.8460177184478));
#39495=CARTESIAN_POINT('Ctrl Pts',(-0.0500632410114724,2.41836646235672,
11.8459235482739));
#39496=CARTESIAN_POINT('Ctrl Pts',(-0.0376624745739469,2.42025599935117,
11.8451586826571));
#39497=CARTESIAN_POINT('Ctrl Pts',(-0.0267002706111915,2.4213557501579,
11.8445167428276));
#39498=CARTESIAN_POINT('Ctrl Pts',(0.0135194310577731,2.42331769512947,
11.842217052745));
#39499=CARTESIAN_POINT('Ctrl Pts',(0.0427983435519015,2.42075773510434,
11.8406367004223));
#39500=CARTESIAN_POINT('Ctrl Pts',(0.0802973369684861,2.4122467786152,11.8383934724666));
#39501=CARTESIAN_POINT('Ctrl Pts',(0.0891717756257766,2.40982911904033,
11.8378470192701));
#39502=CARTESIAN_POINT('Ctrl Pts',(0.0990138853554707,2.40668994128337,
11.83721875536));
#39503=CARTESIAN_POINT('Ctrl Pts',(0.100095767115053,2.40633854953513,11.8371493901617));
#39504=CARTESIAN_POINT('Ctrl Pts',(0.101667709352083,2.40581877146511,11.8370481535422));
#39505=CARTESIAN_POINT('Ctrl Pts',(0.10215926827498,2.40565491654134,11.8370164316362));
#39506=CARTESIAN_POINT('Ctrl Pts',(0.103026369990979,2.40536355382041,11.8369603601126));
#39507=CARTESIAN_POINT('Ctrl Pts',(0.10340207749022,2.40523653661353,11.8369360267526));
#39508=CARTESIAN_POINT('Ctrl Pts',(0.10417863280432,2.40497240460708,11.8368856525873));
#39509=CARTESIAN_POINT('Ctrl Pts',(0.104579446438932,2.40483519233284,11.8368596085937));
#39510=CARTESIAN_POINT('Ctrl Pts',(0.105605491691137,2.40448167999215,11.8367928257547));
#39511=CARTESIAN_POINT('Ctrl Pts',(0.106230327678378,2.40426424501917,11.8367520493369));
#39512=CARTESIAN_POINT('Ctrl Pts',(0.108783064134468,2.4033671033407,11.8365850164294));
#39513=CARTESIAN_POINT('Ctrl Pts',(0.11070511296696,2.40267099643893,11.8364582158546));
#39514=CARTESIAN_POINT('Ctrl Pts',(0.12337020740203,2.39794731305084,11.8356156708809));
#39515=CARTESIAN_POINT('Ctrl Pts',(0.133897036181778,2.39336724464954,11.8348814183693));
#39516=CARTESIAN_POINT('Ctrl Pts',(0.173384447266412,2.37361830053667,11.8319919691008));
#39517=CARTESIAN_POINT('Ctrl Pts',(0.20021401765059,2.35464295234354,11.8297132051395));
#39518=CARTESIAN_POINT('Ctrl Pts',(0.223820563282745,2.33187398884641,11.8275827498975));
#39519=CARTESIAN_POINT('Ctrl Pts',(0.223910487995763,2.33178715369351,11.8275746325986));
#39520=CARTESIAN_POINT('Ctrl Pts',(0.224587525771665,2.33113261535554,11.8275135050623));
#39521=CARTESIAN_POINT('Ctrl Pts',(0.225172535203309,2.33056272905623,11.8274606134425));
#39522=CARTESIAN_POINT('Ctrl Pts',(0.228868849438541,2.3269344818775,11.8271259945453));
#39523=CARTESIAN_POINT('Ctrl Pts',(0.231920137138423,2.32381524516,11.8268478256322));
#39524=CARTESIAN_POINT('Ctrl Pts',(0.235318729695183,2.32019680333319,11.826536743448));
#39525=CARTESIAN_POINT('Ctrl Pts',(0.235728915309947,2.31975762840941,11.8264991768293));
#39526=CARTESIAN_POINT('Ctrl Pts',(0.236332876158374,2.31910734670439,11.8264438354462));
#39527=CARTESIAN_POINT('Ctrl Pts',(0.236527599090586,2.31889712790053,11.8264259885201));
#39528=CARTESIAN_POINT('Ctrl Pts',(0.236871632926425,2.31852472111335,11.8263944496167));
#39529=CARTESIAN_POINT('Ctrl Pts',(0.237021057964513,2.31836263944517,11.8263807488501));
#39530=CARTESIAN_POINT('Ctrl Pts',(0.237329638806674,2.31802723119061,11.8263524503036));
#39531=CARTESIAN_POINT('Ctrl Pts',(0.237488770718182,2.31785388401488,11.8263378543486));
#39532=CARTESIAN_POINT('Ctrl Pts',(0.237901403974315,2.31740340079807,11.8262999991705));
#39533=CARTESIAN_POINT('Ctrl Pts',(0.238154611878585,2.31712599461115,11.8262767624031));
#39534=CARTESIAN_POINT('Ctrl Pts',(0.238706149547586,2.31651962268942,11.8262261303214));
#39535=CARTESIAN_POINT('Ctrl Pts',(0.239004286038416,2.31619048106282,11.8261987495092));
#39536=CARTESIAN_POINT('Ctrl Pts',(0.239872085081427,2.31522844488519,11.8261190140058));
#39537=CARTESIAN_POINT('Ctrl Pts',(0.2404399261004,2.31459390173835,11.8260667926926));
#39538=CARTESIAN_POINT('Ctrl Pts',(0.246385238683807,2.30789699140745,11.8255194472551));
#39539=CARTESIAN_POINT('Ctrl Pts',(0.251535254983926,2.30163552543278,11.8250402261378));
#39540=CARTESIAN_POINT('Ctrl Pts',(0.269277213457459,2.27832533865867,11.8233426880013));
#39541=CARTESIAN_POINT('Ctrl Pts',(0.280416999083914,2.26023913398309,11.8221814407824));
#39542=CARTESIAN_POINT('Ctrl Pts',(0.298542592863542,2.22304784971495,11.8198526846149));
#39543=CARTESIAN_POINT('Ctrl Pts',(0.305659081035013,2.20411914012657,11.8186927081922));
#39544=CARTESIAN_POINT('Ctrl Pts',(0.31129948776745,2.18339956135352,11.8173884658584));
#39545=CARTESIAN_POINT('Ctrl Pts',(0.311632613360392,2.18214604148449,11.8173094466799));
#39546=CARTESIAN_POINT('Ctrl Pts',(0.312086506964273,2.18039557993601,11.8171989323084));
#39547=CARTESIAN_POINT('Ctrl Pts',(0.312213675894898,2.17990029838397,11.8171676441869));
#39548=CARTESIAN_POINT('Ctrl Pts',(0.312431186227086,2.17904471819236,11.8171135619049));
#39549=CARTESIAN_POINT('Ctrl Pts',(0.312522084726933,2.17868456111227,11.8170907857792));
#39550=CARTESIAN_POINT('Ctrl Pts',(0.312708885920893,2.17793898917356,11.8170436149003));
#39551=CARTESIAN_POINT('Ctrl Pts',(0.312804699175932,2.17755355271382,11.8170192173035));
#39552=CARTESIAN_POINT('Ctrl Pts',(0.313026880080136,2.17665265579953,11.8169621637914));
#39553=CARTESIAN_POINT('Ctrl Pts',(0.313152687137656,2.1761370594843,11.8169294898667));
#39554=CARTESIAN_POINT('Ctrl Pts',(0.313552818524207,2.17447942750916,11.8168243737746));
#39555=CARTESIAN_POINT('Ctrl Pts',(0.313822171094595,2.17333621204769,11.8167517718033));
#39556=CARTESIAN_POINT('Ctrl Pts',(0.317929441702056,2.15546662800753,11.8156151982127));
#39557=CARTESIAN_POINT('Ctrl Pts',(0.320430964654827,2.13846426944246,11.814507810578));
#39558=CARTESIAN_POINT('Ctrl Pts',(0.32340940612798,2.09359540284013,11.8115214745401));
#39559=CARTESIAN_POINT('Ctrl Pts',(0.321651678455091,2.06572533584755,11.8095952147709));
#39560=CARTESIAN_POINT('Ctrl Pts',(0.316251564346348,2.03798120625939,11.8077558457193));
#39561=CARTESIAN_POINT('Ctrl Pts',(0.316163671503912,2.03753468519169,11.807726266824));
#39562=CARTESIAN_POINT('Ctrl Pts',(0.315918033270298,2.03630057254475,11.807644585584));
#39563=CARTESIAN_POINT('Ctrl Pts',(0.315758287728039,2.03551337689361,11.8075925630766));
#39564=CARTESIAN_POINT('Ctrl Pts',(0.31470885956459,2.03043939853587,11.8072577891008));
#39565=CARTESIAN_POINT('Ctrl Pts',(0.313734789617186,2.02617026301319,11.8069786223044));
#39566=CARTESIAN_POINT('Ctrl Pts',(0.312528233197793,2.02133844065882,11.8066665375241));
#39567=CARTESIAN_POINT('Ctrl Pts',(0.312380864642385,2.02075523435039,11.8066289332662));
#39568=CARTESIAN_POINT('Ctrl Pts',(0.312160855341345,2.01989470557334,11.8065735468188));
#39569=CARTESIAN_POINT('Ctrl Pts',(0.312089477168177,2.01961706620777,11.8065556923005));
#39570=CARTESIAN_POINT('Ctrl Pts',(0.311962548595352,2.01912607030098,11.8065241446454));
#39571=CARTESIAN_POINT('Ctrl Pts',(0.311907149646376,2.0189126752709,11.8065104427027));
#39572=CARTESIAN_POINT('Ctrl Pts',(0.311792190058654,2.01847171548664,11.806482148169));
#39573=CARTESIAN_POINT('Ctrl Pts',(0.311732599388707,2.01824415961858,11.8064675573899));
#39574=CARTESIAN_POINT('Ctrl Pts',(0.311577572073877,2.0176547984642,11.8064297946059));
#39575=CARTESIAN_POINT('Ctrl Pts',(0.311481754019993,2.01729309248063,11.8064066447906));
#39576=CARTESIAN_POINT('Ctrl Pts',(0.311271150555932,2.01650363721059,11.8063561737966));
#39577=CARTESIAN_POINT('Ctrl Pts',(0.311156112707261,2.01607595518661,11.8063288671162));
#39578=CARTESIAN_POINT('Ctrl Pts',(0.310818159188337,2.01482977534973,11.8062494012246));
#39579=CARTESIAN_POINT('Ctrl Pts',(0.310592890925302,2.01401191133708,11.8061973743052));
#39580=CARTESIAN_POINT('Ctrl Pts',(0.302752942807692,1.98598081934197,11.804418264597));
#39581=CARTESIAN_POINT('Ctrl Pts',(0.291593767699802,1.95988076927474,11.8028850860857));
#39582=CARTESIAN_POINT('Ctrl Pts',(0.266333502687802,1.9173015023525,11.8001038637217));
#39583=CARTESIAN_POINT('Ctrl Pts',(0.253719553825934,1.90015390823077,11.7988873460262));
#39584=CARTESIAN_POINT('Ctrl Pts',(0.238642380658758,1.88340664937096,11.7975187104103));
#39585=CARTESIAN_POINT('Ctrl Pts',(0.237766813883331,1.88244585151826,11.7974395171488));
#39586=CARTESIAN_POINT('Ctrl Pts',(0.236538432970812,1.88111416828081,11.7973287980994));
#39587=CARTESIAN_POINT('Ctrl Pts',(0.236190503537246,1.8807387776333,11.7972974803986));
#39588=CARTESIAN_POINT('Ctrl Pts',(0.23558844562702,1.88009229667204,11.7972433607571));
#39589=CARTESIAN_POINT('Ctrl Pts',(0.235334739117352,1.87982081329375,11.7972205769101));
#39590=CARTESIAN_POINT('Ctrl Pts',(0.234808935959189,1.87926011483875,11.7971734030118));
#39591=CARTESIAN_POINT('Ctrl Pts',(0.23453677325662,1.8789709627776,11.7971490101395));
#39592=CARTESIAN_POINT('Ctrl Pts',(0.233899929719419,1.87829686588267,11.7970919900868));
#39593=CARTESIAN_POINT('Ctrl Pts',(0.233534832652152,1.8779123174668,11.7970593449601));
#39594=CARTESIAN_POINT('Ctrl Pts',(0.232359734299669,1.87668071488045,11.7969544130597));
#39595=CARTESIAN_POINT('Ctrl Pts',(0.231546067791806,1.87583718492553,11.7968819672682));
#39596=CARTESIAN_POINT('Ctrl Pts',(0.219098745128709,1.86307309727659,11.7957768387381));
#39597=CARTESIAN_POINT('Ctrl Pts',(0.206564651470505,1.8520695603545,11.7947033443389));
#39598=CARTESIAN_POINT('Ctrl Pts',(0.170885980811952,1.82533793779371,11.791746987975));
#39599=CARTESIAN_POINT('Ctrl Pts',(0.146453590161215,1.81156893742319,11.7898124704495));
#39600=CARTESIAN_POINT('Ctrl Pts',(0.115038519631861,1.79889756380337,11.7876034564957));
#39601=CARTESIAN_POINT('Ctrl Pts',(0.109462644358897,1.79682599253988,11.7872217612272));
#39602=CARTESIAN_POINT('Ctrl Pts',(0.10326791928281,1.79471772442695,11.7868114405864));
#39603=CARTESIAN_POINT('Ctrl Pts',(0.102703090586885,1.79452724159198,11.786774152309));
#39604=CARTESIAN_POINT('Ctrl Pts',(0.101861516421708,1.7942460271544,11.7867187824942));
#39605=CARTESIAN_POINT('Ctrl Pts',(0.101585175188119,1.7941541031463,11.78670063131));
#39606=CARTESIAN_POINT('Ctrl Pts',(0.101110845955794,1.7939970328614,11.7866695277055));
#39607=CARTESIAN_POINT('Ctrl Pts',(0.100912919327229,1.79393170405783,11.7866565644709));
#39608=CARTESIAN_POINT('Ctrl Pts',(0.100516045488607,1.79380113641609,11.7866306025802));
#39609=CARTESIAN_POINT('Ctrl Pts',(0.100317098555393,1.7937358995926,11.7866176041135));
#39610=CARTESIAN_POINT('Ctrl Pts',(0.0998472197775074,1.79358232829294,
11.7865869410838));
#39611=CARTESIAN_POINT('Ctrl Pts',(0.0995762333188271,1.79349415896071,
11.7865692863477));
#39612=CARTESIAN_POINT('Ctrl Pts',(0.098733663440106,1.79322125210116,11.7865144824297));
#39613=CARTESIAN_POINT('Ctrl Pts',(0.0981616760392877,1.79303775178442,
11.7864774059885));
#39614=CARTESIAN_POINT('Ctrl Pts',(0.0968318748762844,1.79261523292338,
11.7863914970572));
#39615=CARTESIAN_POINT('Ctrl Pts',(0.0960736797804176,1.79237741450469,
11.7863427332254));
#39616=CARTESIAN_POINT('Ctrl Pts',(0.0935165471388722,1.79158571053427,
11.7861789778073));
#39617=CARTESIAN_POINT('Ctrl Pts',(0.0917136001434671,1.79104476948785,
11.7860646978029));
#39618=CARTESIAN_POINT('Ctrl Pts',(0.0840643965085473,1.78882262823844,
11.7855844197877));
#39619=CARTESIAN_POINT('Ctrl Pts',(0.0781755466227434,1.78729123246203,
11.7852259073712));
#39620=CARTESIAN_POINT('Ctrl Pts',(0.061770190224892,1.78351748904971,11.7842491674188));
#39621=CARTESIAN_POINT('Ctrl Pts',(0.051179219797018,1.78163315037415,11.7836431389335));
#39622=CARTESIAN_POINT('Ctrl Pts',(0.0168969983911632,1.77728905566019,
11.781706868318));
#39623=CARTESIAN_POINT('Ctrl Pts',(-0.00697599470007906,1.77692245346771,
11.7803910358026));
#39624=CARTESIAN_POINT('Ctrl Pts',(-0.038065382725545,1.77989474012361,
11.7785546517917));
#39625=CARTESIAN_POINT('Ctrl Pts',(-0.0454325132410477,1.78085704743446,
11.7781109326985));
#39626=CARTESIAN_POINT('Ctrl Pts',(-0.0537124806884222,1.78223109277357,
11.7776002559405));
#39627=CARTESIAN_POINT('Ctrl Pts',(-0.0546648261846304,1.78239353638826,
11.7775413398889));
#39628=CARTESIAN_POINT('Ctrl Pts',(-0.0561059094728479,1.78264601861147,
11.7774519122617));
#39629=CARTESIAN_POINT('Ctrl Pts',(-0.0565951989304509,1.78273291057127,
11.7774215006994));
#39630=CARTESIAN_POINT('Ctrl Pts',(-0.057446215786213,1.78288607227839,
11.7773685213464));
#39631=CARTESIAN_POINT('Ctrl Pts',(-0.0578080353158415,1.78295183029343,
11.7773459698734));
#39632=CARTESIAN_POINT('Ctrl Pts',(-0.0585628878815867,1.7830903542677,
11.7772988653871));
#39633=CARTESIAN_POINT('Ctrl Pts',(-0.0589558994954324,1.78316323239302,
11.7772743088354));
#39634=CARTESIAN_POINT('Ctrl Pts',(-0.0598850971739494,1.78333732695134,
11.7772161741735));
#39635=CARTESIAN_POINT('Ctrl Pts',(-0.0604211624921362,1.78343917411797,
11.7771825760081));
#39636=CARTESIAN_POINT('Ctrl Pts',(-0.0621912347783861,1.78378013046192,
11.7770714373212));
#39637=CARTESIAN_POINT('Ctrl Pts',(-0.063424089835754,1.78402509540998,
11.7769937101678));
#39638=CARTESIAN_POINT('Ctrl Pts',(-0.0785772970635241,1.78712825387335,
11.776034357707));
#39639=CARTESIAN_POINT('Ctrl Pts',(-0.0922933029898179,1.79089651047776,
11.7751233558813));
#39640=CARTESIAN_POINT('Ctrl Pts',(-0.11851376680257,1.80000126898148,11.773296165906));
#39641=CARTESIAN_POINT('Ctrl Pts',(-0.131019190881346,1.80524811571201,
11.772384093323));
#39642=CARTESIAN_POINT('Ctrl Pts',(-0.155959698262365,1.81761379658061,
11.7705008748386));
#39643=CARTESIAN_POINT('Ctrl Pts',(-0.168327112664878,1.82480658549107,
11.7695312717921));
#39644=CARTESIAN_POINT('Ctrl Pts',(-0.182065793034183,1.83407065982949,
11.768438366233));
#39645=CARTESIAN_POINT('Ctrl Pts',(-0.183941373147152,1.83536451734087,
11.7682888238722));
#39646=CARTESIAN_POINT('Ctrl Pts',(-0.186390828142627,1.83709288296392,
11.7680932274148));
#39647=CARTESIAN_POINT('Ctrl Pts',(-0.18697715500017,1.83750954964256,11.7680463846979));
#39648=CARTESIAN_POINT('Ctrl Pts',(-0.188428525437206,1.83854828042607,
11.7679303848923));
#39649=CARTESIAN_POINT('Ctrl Pts',(-0.189291894849796,1.83917268266337,
11.7678613388378));
#39650=CARTESIAN_POINT('Ctrl Pts',(-0.193657545165101,1.84236308311626,
11.767512055546));
#39651=CARTESIAN_POINT('Ctrl Pts',(-0.197111021480385,1.84499553816574,
11.7672352562673));
#39652=CARTESIAN_POINT('Ctrl Pts',(-0.20098033209129,1.84807056151212,11.7669255446263));
#39653=CARTESIAN_POINT('Ctrl Pts',(-0.201449177002585,1.84844530423166,
11.7668880240045));
#39654=CARTESIAN_POINT('Ctrl Pts',(-0.202140192272888,1.84900079618438,
11.7668327376979));
#39655=CARTESIAN_POINT('Ctrl Pts',(-0.202363169561291,1.84918053254417,
11.766814900055));
#39656=CARTESIAN_POINT('Ctrl Pts',(-0.202757338060085,1.84949912959089,
11.7667833718495));
#39657=CARTESIAN_POINT('Ctrl Pts',(-0.202928626597585,1.84963786883531,
11.7667696725172));
#39658=CARTESIAN_POINT('Ctrl Pts',(-0.203258333536368,1.84990548351178,
11.7667433061486));
#39659=CARTESIAN_POINT('Ctrl Pts',(-0.203416771180086,1.85003433329219,
11.766730637323));
#39660=CARTESIAN_POINT('Ctrl Pts',(-0.203844311905702,1.85038270745885,
11.7666964539154));
#39661=CARTESIAN_POINT('Ctrl Pts',(-0.204113183772749,1.85060251716441,
11.7666749600339));
#39662=CARTESIAN_POINT('Ctrl Pts',(-0.205134483944484,1.85144021433353,
11.7665933268893));
#39663=CARTESIAN_POINT('Ctrl Pts',(-0.205884476050621,1.85206108386853,
11.7665334014878));
#39664=CARTESIAN_POINT('Ctrl Pts',(-0.207750237339644,1.8536199294317,11.7663843463566));
#39665=CARTESIAN_POINT('Ctrl Pts',(-0.208862490711725,1.85456210471595,
11.7662955083583));
#39666=CARTESIAN_POINT('Ctrl Pts',(-0.213245148173981,1.85832596468861,
11.7659453578196));
#39667=CARTESIAN_POINT('Ctrl Pts',(-0.216465227154571,1.86120585867247,
11.7656878701537));
#39668=CARTESIAN_POINT('Ctrl Pts',(-0.224695530106086,1.8688700166897,11.7650261651648));
#39669=CARTESIAN_POINT('Ctrl Pts',(-0.229611266189895,1.87375272880925,
11.7646273251012));
#39670=CARTESIAN_POINT('Ctrl Pts',(-0.256251182606515,1.90197704973941,
11.7624192516564));
#39671=CARTESIAN_POINT('Ctrl Pts',(-0.274573409335034,1.92828140074248,
11.7606982614548));
#39672=CARTESIAN_POINT('Ctrl Pts',(-0.291305496533585,1.96202995618514,
11.7584660192234));
#39673=CARTESIAN_POINT('Ctrl Pts',(-0.293734421229658,1.96727958471352,
11.7581188801863));
#39674=CARTESIAN_POINT('Ctrl Pts',(-0.296409970276014,1.97349594964596,
11.7577068708082));
#39675=CARTESIAN_POINT('Ctrl Pts',(-0.296795106928273,1.97440219068517,
11.7576467845135));
#39676=CARTESIAN_POINT('Ctrl Pts',(-0.297369766324003,1.97577178942146,
11.7575559376356));
#39677=CARTESIAN_POINT('Ctrl Pts',(-0.29756237498149,1.97623385269775,11.7575252818974));
#39678=CARTESIAN_POINT('Ctrl Pts',(-0.297904230286483,1.97705936565765,
11.7574705004382));
#39679=CARTESIAN_POINT('Ctrl Pts',(-0.298053890669067,1.9774226438124,11.7574463887941));
#39680=CARTESIAN_POINT('Ctrl Pts',(-0.298368281932675,1.97818976157715,
11.7573954638254));
#39681=CARTESIAN_POINT('Ctrl Pts',(-0.298532857968454,1.97859366343433,
11.7573686453212));
#39682=CARTESIAN_POINT('Ctrl Pts',(-0.298966045346289,1.97966299693225,
11.7572976277554));
#39683=CARTESIAN_POINT('Ctrl Pts',(-0.299233253788373,1.98032899101605,
11.7572533814351));
#39684=CARTESIAN_POINT('Ctrl Pts',(-0.30043965629483,1.98336514961971,11.7570515934221));
#39685=CARTESIAN_POINT('Ctrl Pts',(-0.301352908470266,1.98574546243783,
11.7568931818498));
#39686=CARTESIAN_POINT('Ctrl Pts',(-0.305211968187628,1.99617202435961,
11.7561981954884));
#39687=CARTESIAN_POINT('Ctrl Pts',(-0.30786422930257,2.00432247852731,11.755651979041));
#39688=CARTESIAN_POINT('Ctrl Pts',(-0.318225927603125,2.04108352142416,
11.7531738206257));
#39689=CARTESIAN_POINT('Ctrl Pts',(-0.322291789681375,2.07056820816242,
11.7511303604084));
#39690=CARTESIAN_POINT('Ctrl Pts',(-0.322274947886789,2.10018327456701,
11.7491602604485));
#39691=CARTESIAN_POINT('',(-0.322274998490625,2.09996880917294,11.4996790403846));
#39692=CARTESIAN_POINT('Ctrl Pts',(-0.322274947619657,2.10018374369947,
11.7491602292402));
#39693=CARTESIAN_POINT('Ctrl Pts',(-0.322268950934441,2.11070155421152,
11.748460547305));
#39694=CARTESIAN_POINT('Ctrl Pts',(-0.321748061778375,2.12121429561999,
11.7477736286716));
#39695=CARTESIAN_POINT('Ctrl Pts',(-0.320667537867109,2.1321516176864,11.7470842989936));
#39696=CARTESIAN_POINT('Ctrl Pts',(-0.320620324781466,2.13261906965548,
11.7470548864868));
#39697=CARTESIAN_POINT('Ctrl Pts',(-0.320542098304985,2.13337700070024,
11.7470072778706));
#39698=CARTESIAN_POINT('Ctrl Pts',(-0.320511712109824,2.13366754169137,
11.7469890471902));
#39699=CARTESIAN_POINT('Ctrl Pts',(-0.32045782597811,2.13417609508444,11.7469571711405));
#39700=CARTESIAN_POINT('Ctrl Pts',(-0.320434498569135,2.13439412498187,
11.746943516111));
#39701=CARTESIAN_POINT('Ctrl Pts',(-0.320388722059018,2.13481788666074,
11.7469169979818));
#39702=CARTESIAN_POINT('Ctrl Pts',(-0.320366297251527,2.13502362117741,
11.7469041334929));
#39703=CARTESIAN_POINT('Ctrl Pts',(-0.320321291777004,2.13543286021143,
11.746878563936));
#39704=CARTESIAN_POINT('Ctrl Pts',(-0.320298715366229,2.13563636462625,
11.7468658586436));
#39705=CARTESIAN_POINT('Ctrl Pts',(-0.320245123767606,2.13611527569325,
11.7468359818308));
#39706=CARTESIAN_POINT('Ctrl Pts',(-0.320213947170666,2.13639066465521,
11.7468188194791));
#39707=CARTESIAN_POINT('Ctrl Pts',(-0.32012094981732,2.13720275502851,11.746768261156));
#39708=CARTESIAN_POINT('Ctrl Pts',(-0.320058134319823,2.13773934497758,
11.7467349209991));
#39709=CARTESIAN_POINT('Ctrl Pts',(-0.319501534579595,2.14239264178265,
11.7464463517458));
#39710=CARTESIAN_POINT('Ctrl Pts',(-0.318929669392683,2.14649985599115,
11.7461954222511));
#39711=CARTESIAN_POINT('Ctrl Pts',(-0.318222174302826,2.15095049448819,
11.7459265114914));
#39712=CARTESIAN_POINT('Ctrl Pts',(-0.318165087024727,2.15130577460117,
11.7459050660666));
#39713=CARTESIAN_POINT('Ctrl Pts',(-0.317946762045513,2.15265013197692,
11.7458239943743));
#39714=CARTESIAN_POINT('Ctrl Pts',(-0.317781504700217,2.15363856084549,
11.7457645436688));
#39715=CARTESIAN_POINT('Ctrl Pts',(-0.317405010814399,2.15582759849676,
11.7456331960615));
#39716=CARTESIAN_POINT('Ctrl Pts',(-0.317191566513112,2.15702781649517,
11.7455613909783));
#39717=CARTESIAN_POINT('Ctrl Pts',(-0.316441384880153,2.16111160639411,
11.7453177030334));
#39718=CARTESIAN_POINT('Ctrl Pts',(-0.315872083083141,2.16398911280353,
11.7451470707396));
#39719=CARTESIAN_POINT('Ctrl Pts',(-0.314939078590981,2.16838858669777,
11.7448872981295));
#39720=CARTESIAN_POINT('Ctrl Pts',(-0.31460345648086,2.16991628780983,11.7447972996535));
#39721=CARTESIAN_POINT('Ctrl Pts',(-0.310992465654227,2.1858003061269,11.7438631629755));
#39722=CARTESIAN_POINT('Ctrl Pts',(-0.306747789749089,2.19991917240016,
11.7430458268146));
#39723=CARTESIAN_POINT('Ctrl Pts',(-0.29284195021286,2.23680027423194,11.7408404606812));
#39724=CARTESIAN_POINT('Ctrl Pts',(-0.281507658437494,2.25882033261991,
11.739441533447));
#39725=CARTESIAN_POINT('Ctrl Pts',(-0.267130699610873,2.28028781170197,
11.7378704155822));
#39726=CARTESIAN_POINT('Ctrl Pts',(-0.266483815291574,2.28124260497022,
11.7378000935766));
#39727=CARTESIAN_POINT('Ctrl Pts',(-0.265534020539039,2.28262841250604,
11.7376973687041));
#39728=CARTESIAN_POINT('Ctrl Pts',(-0.265235151128824,2.28306219631199,
11.7376651193121));
#39729=CARTESIAN_POINT('Ctrl Pts',(-0.264709443973943,2.28382122602114,
11.7376085228084));
#39730=CARTESIAN_POINT('Ctrl Pts',(-0.264483066385325,2.28414679051792,
11.7375841932761));
#39731=CARTESIAN_POINT('Ctrl Pts',(-0.264042835826657,2.28477742089377,
11.7375369607276));
#39732=CARTESIAN_POINT('Ctrl Pts',(-0.263829053483098,2.28508253553466,
11.7375140604373));
#39733=CARTESIAN_POINT('Ctrl Pts',(-0.263318173917205,2.28580898983719,
11.7374594216567));
#39734=CARTESIAN_POINT('Ctrl Pts',(-0.263020594466208,2.28622998765269,
11.7374276646958));
#39735=CARTESIAN_POINT('Ctrl Pts',(-0.262120104481805,2.28749748402103,
11.7373317735963));
#39736=CARTESIAN_POINT('Ctrl Pts',(-0.261514112647027,2.28834177585879,
11.7372675209018));
#39737=CARTESIAN_POINT('Ctrl Pts',(-0.255181905203886,2.29707457739523,
11.7365989576935));
#39738=CARTESIAN_POINT('Ctrl Pts',(-0.249105237759864,2.30470159072167,
11.7359809991665));
#39739=CARTESIAN_POINT('Ctrl Pts',(-0.225254265144905,2.33200037509071,
11.733634866946));
#39740=CARTESIAN_POINT('Ctrl Pts',(-0.205421566774034,2.34973034338367,
11.7318229293518));
#39741=CARTESIAN_POINT('Ctrl Pts',(-0.176093504824484,2.37006806653454,
11.7294241289772));
#39742=CARTESIAN_POINT('Ctrl Pts',(-0.16831806673017,2.37498133766676,11.728812308266));
#39743=CARTESIAN_POINT('Ctrl Pts',(-0.158445115785468,2.38064409159899,
11.728073489801));
#39744=CARTESIAN_POINT('Ctrl Pts',(-0.156536478559515,2.38171313827169,
11.7279323641213));
#39745=CARTESIAN_POINT('Ctrl Pts',(-0.151857160786773,2.38427182910921,
11.7275907649438));
#39746=CARTESIAN_POINT('Ctrl Pts',(-0.149075193117343,2.38574054442383,
11.7273913794451));
#39747=CARTESIAN_POINT('Ctrl Pts',(-0.145817358688473,2.38739995460051,
11.7271625476154));
#39748=CARTESIAN_POINT('Ctrl Pts',(-0.145362122280678,2.38763047372248,
11.7271306763015));
#39749=CARTESIAN_POINT('Ctrl Pts',(-0.14471174805151,2.38795786681495,11.7270852946028));
#39750=CARTESIAN_POINT('Ctrl Pts',(-0.144517059551175,2.38805562411468,
11.7270717289667));
#39751=CARTESIAN_POINT('Ctrl Pts',(-0.144136419260573,2.38824626879369,
11.7270452443816));
#39752=CARTESIAN_POINT('Ctrl Pts',(-0.143950476235573,2.38833917393108,
11.7270323243075));
#39753=CARTESIAN_POINT('Ctrl Pts',(-0.143579924284762,2.38852386984925,
11.7270066121948));
#39754=CARTESIAN_POINT('Ctrl Pts',(-0.14339531745632,2.38861566323159,11.7269938199907));
#39755=CARTESIAN_POINT('Ctrl Pts',(-0.142957397485407,2.38883288945286,
11.7269635156129));
#39756=CARTESIAN_POINT('Ctrl Pts',(-0.14270400664981,2.38895816654491,11.7269460132635));
#39757=CARTESIAN_POINT('Ctrl Pts',(-0.141814477718846,2.38939649653379,
11.7268846839697));
#39758=CARTESIAN_POINT('Ctrl Pts',(-0.141177465730696,2.3897077863797,11.7268409666856));
#39759=CARTESIAN_POINT('Ctrl Pts',(-0.132776010820972,2.39377905027203,
11.72626697445));
#39760=CARTESIAN_POINT('Ctrl Pts',(-0.12486384559136,2.39722827971215,11.7257554464584));
#39761=CARTESIAN_POINT('Ctrl Pts',(-0.100692277647183,2.40662968978287,
11.7242509166264));
#39762=CARTESIAN_POINT('Ctrl Pts',(-0.0840822762275282,2.4115942188867,
11.7232924980548));
#39763=CARTESIAN_POINT('Ctrl Pts',(-0.0650240110179947,2.41565454490743,
11.7222020774622));
#39764=CARTESIAN_POINT('Ctrl Pts',(-0.0628905397562314,2.41608652876088,
11.7220801607051));
#39765=CARTESIAN_POINT('Ctrl Pts',(-0.0582041225921994,2.41698610566029,
11.7218124464915));
#39766=CARTESIAN_POINT('Ctrl Pts',(-0.055649583104193,2.4174445380996,11.7216665749756));
#39767=CARTESIAN_POINT('Ctrl Pts',(-0.0438989422912002,2.41940708623251,
11.7209950487034));
#39768=CARTESIAN_POINT('Ctrl Pts',(-0.03464628805122,2.42054270025812,11.7204646265548));
#39769=CARTESIAN_POINT('Ctrl Pts',(-0.0168046720244086,2.4219509146117,
11.7194257772018));
#39770=CARTESIAN_POINT('Ctrl Pts',(-0.00822857072006633,2.42228412916206,
11.7189193783453));
#39771=CARTESIAN_POINT('Ctrl Pts',(0.00290545431056951,2.42227203386079,
11.7182481671951));
#39772=CARTESIAN_POINT('Ctrl Pts',(0.00546062730743365,2.42223886550676,
11.7180931992389));
#39773=CARTESIAN_POINT('Ctrl Pts',(0.00873305095507294,2.42215745412284,
11.7178934545744));
#39774=CARTESIAN_POINT('Ctrl Pts',(0.00945095526919228,2.42213719260161,
11.7178495559387));
#39775=CARTESIAN_POINT('Ctrl Pts',(0.0106048421228915,2.42210076573501,
11.7177788692149));
#39776=CARTESIAN_POINT('Ctrl Pts',(0.0110408728203206,2.42208611439789,
11.7177521286204));
#39777=CARTESIAN_POINT('Ctrl Pts',(0.0118694936856635,2.42205658678744,
11.7177012549395));
#39778=CARTESIAN_POINT('Ctrl Pts',(0.012262089337997,2.42204187792339,11.717677127146));
#39779=CARTESIAN_POINT('Ctrl Pts',(0.0131546354110652,2.42200680358947,
11.7176222185132));
#39780=CARTESIAN_POINT('Ctrl Pts',(0.01365456638542,2.42198599162546,11.7175914237283));
#39781=CARTESIAN_POINT('Ctrl Pts',(0.0151370828808383,2.42192081602623,
11.7174999853565));
#39782=CARTESIAN_POINT('Ctrl Pts',(0.0161195093675584,2.42187311856155,
11.7174392373843));
#39783=CARTESIAN_POINT('Ctrl Pts',(0.0228562296136296,2.4215151265364,11.7170215999422));
#39784=CARTESIAN_POINT('Ctrl Pts',(0.0286012035467558,2.42105505455501,
11.7166600356854));
#39785=CARTESIAN_POINT('Ctrl Pts',(0.0346851291765129,2.42040325320505,
11.7162710444655));
#39786=CARTESIAN_POINT('Ctrl Pts',(0.0350397218225903,2.42036466837551,
11.7162483507436));
#39787=CARTESIAN_POINT('Ctrl Pts',(0.0581351308789641,2.41781274958896,
11.7147688263816));
#39788=CARTESIAN_POINT('Ctrl Pts',(0.0805401078380058,2.41288591071856,
11.7132359547607));
#39789=CARTESIAN_POINT('Ctrl Pts',(0.112884892985624,2.40206685704193,11.7109280549968));
#39790=CARTESIAN_POINT('Ctrl Pts',(0.12334569696915,2.39794838604962,11.7101671199623));
#39791=CARTESIAN_POINT('Ctrl Pts',(0.140384051959473,2.390188816883,11.7089216570347));
#39792=CARTESIAN_POINT('Ctrl Pts',(0.14708811074073,2.38684897848462,11.7084300481458));
#39793=CARTESIAN_POINT('Ctrl Pts',(0.155584474927382,2.38223995030405,11.7078103327022));
#39794=CARTESIAN_POINT('Ctrl Pts',(0.157488226382901,2.38118210740182,11.707671700506));
#39795=CARTESIAN_POINT('Ctrl Pts',(0.160149977319933,2.37966755769964,11.7074783438169));
#39796=CARTESIAN_POINT('Ctrl Pts',(0.160916994962477,2.37922693072113,11.7074226814974));
#39797=CARTESIAN_POINT('Ctrl Pts',(0.162249992586815,2.37845384959776,11.7073260567755));
#39798=CARTESIAN_POINT('Ctrl Pts',(0.162816784752807,2.3781228165235,11.7072850068874));
#39799=CARTESIAN_POINT('Ctrl Pts',(0.163636710600072,2.3776405761058,11.7072256791768));
#39800=CARTESIAN_POINT('Ctrl Pts',(0.163890649679756,2.37749075210822,11.7072073125257));
#39801=CARTESIAN_POINT('Ctrl Pts',(0.164322599988114,2.37723510175401,11.7071760844932));
#39802=CARTESIAN_POINT('Ctrl Pts',(0.164500715115238,2.37712945213184,11.707163211541));
#39803=CARTESIAN_POINT('Ctrl Pts',(0.164854920191167,2.37691889232597,11.7071376200604));
#39804=CARTESIAN_POINT('Ctrl Pts',(0.165031011709835,2.37681398594164,11.7071249013171));
#39805=CARTESIAN_POINT('Ctrl Pts',(0.165445707132117,2.37656639511478,11.7070949577055));
#39806=CARTESIAN_POINT('Ctrl Pts',(0.165684227181443,2.37642356950858,11.7070777421086));
#39807=CARTESIAN_POINT('Ctrl Pts',(0.166388590629643,2.37600055805358,11.7070269233886));
#39808=CARTESIAN_POINT('Ctrl Pts',(0.166853913217789,2.37571950020205,11.7069933768954));
#39809=CARTESIAN_POINT('Ctrl Pts',(0.170940563622235,2.37323700268524,11.7066989650441));
#39810=CARTESIAN_POINT('Ctrl Pts',(0.174519061167846,2.37096538048701,11.7064425934264));
#39811=CARTESIAN_POINT('Ctrl Pts',(0.178291119749714,2.36846514597378,11.7061727343928));
#39812=CARTESIAN_POINT('Ctrl Pts',(0.178530115806142,2.36830627226308,11.7061556378921));
#39813=CARTESIAN_POINT('Ctrl Pts',(0.179349488072056,2.36776001131051,11.7060970289044));
#39814=CARTESIAN_POINT('Ctrl Pts',(0.179928822076298,2.36737105589566,11.706055597448));
#39815=CARTESIAN_POINT('Ctrl Pts',(0.1809209483708,2.36670027348489,11.7059846499838));
#39816=CARTESIAN_POINT('Ctrl Pts',(0.181334354337716,2.36641936374597,11.7059550886397));
#39817=CARTESIAN_POINT('Ctrl Pts',(0.20432198646598,2.3507209530597,11.7043113027594));
#39818=CARTESIAN_POINT('Ctrl Pts',(0.224845996088185,2.33249324098366,11.7028347083803));
#39819=CARTESIAN_POINT('Ctrl Pts',(0.253235129311885,2.2999597358024,11.7003881792259));
#39820=CARTESIAN_POINT('Ctrl Pts',(0.262751652325356,2.28727892894038,11.6994717987528));
#39821=CARTESIAN_POINT('Ctrl Pts',(0.272639364276537,2.27185789585365,11.6983670340386));
#39822=CARTESIAN_POINT('Ctrl Pts',(0.2739572844014,2.26974912403018,11.6982161944951));
#39823=CARTESIAN_POINT('Ctrl Pts',(0.275620572735821,2.26701790728419,11.6980210511169));
#39824=CARTESIAN_POINT('Ctrl Pts',(0.275988490002778,2.26640923905249,11.6979775761631));
#39825=CARTESIAN_POINT('Ctrl Pts',(0.276578034813643,2.2654265857227,11.6979074092183));
#39826=CARTESIAN_POINT('Ctrl Pts',(0.276800927155291,2.26505335903363,11.6978807634678));
#39827=CARTESIAN_POINT('Ctrl Pts',(0.277223988937843,2.26434168733287,11.6978299636048));
#39828=CARTESIAN_POINT('Ctrl Pts',(0.277424295614608,2.26400332447419,11.6978058145487));
#39829=CARTESIAN_POINT('Ctrl Pts',(0.2778795276969,2.26323111505557,11.6977507095799));
#39830=CARTESIAN_POINT('Ctrl Pts',(0.278134056780807,2.26279703710267,11.6977197393458));
#39831=CARTESIAN_POINT('Ctrl Pts',(0.278907102504429,2.26147156789141,11.6976251868385));
#39832=CARTESIAN_POINT('Ctrl Pts',(0.279422354428512,2.26057828891466,11.6975614866189));
#39833=CARTESIAN_POINT('Ctrl Pts',(0.283137595973581,2.25406524301752,11.6970971748517));
#39834=CARTESIAN_POINT('Ctrl Pts',(0.286171876346258,2.24835310842052,11.6966906539616));
#39835=CARTESIAN_POINT('Ctrl Pts',(0.289295402289979,2.24202006941801,11.6962402302613));
#39836=CARTESIAN_POINT('Ctrl Pts',(0.28955720579601,2.24148552741459,11.6962022146931));
#39837=CARTESIAN_POINT('Ctrl Pts',(0.300755763059905,2.2184594044522,11.6945647492212));
#39838=CARTESIAN_POINT('Ctrl Pts',(0.30903713488611,2.19477500640232,11.6928747755306));
#39839=CARTESIAN_POINT('Ctrl Pts',(0.318245997667544,2.15362288023519,11.690023326279));
#39840=CARTESIAN_POINT('Ctrl Pts',(0.320650823101592,2.13659397024029,11.6888694836161));
#39841=CARTESIAN_POINT('Ctrl Pts',(0.321761238601345,2.11823125455351,11.6877027000368));
#39842=CARTESIAN_POINT('Ctrl Pts',(0.321828150896782,2.11700925363514,11.6876254247287));
#39843=CARTESIAN_POINT('Ctrl Pts',(0.321916456563464,2.11520873667219,11.6875121425098));
#39844=CARTESIAN_POINT('Ctrl Pts',(0.321943253939489,2.11463051374857,11.6874758502839));
#39845=CARTESIAN_POINT('Ctrl Pts',(0.321983193150699,2.1137154148654,11.6874185558428));
#39846=CARTESIAN_POINT('Ctrl Pts',(0.321997364350109,2.11337858850869,11.6873974975083));
#39847=CARTESIAN_POINT('Ctrl Pts',(0.322023170284944,2.11274141924462,11.6873577200725));
#39848=CARTESIAN_POINT('Ctrl Pts',(0.32203491341676,2.11244108143029,11.6873389949679));
#39849=CARTESIAN_POINT('Ctrl Pts',(0.322054481797711,2.11192200840681,11.6873066752643));
#39850=CARTESIAN_POINT('Ctrl Pts',(0.322062504400508,2.11170328119804,11.6872930695223));
#39851=CARTESIAN_POINT('Ctrl Pts',(0.322077625910719,2.11127921654863,11.6872667166317));
#39852=CARTESIAN_POINT('Ctrl Pts',(0.322084751272772,2.11107388081874,11.6872539679933));
#39853=CARTESIAN_POINT('Ctrl Pts',(0.322101120369138,2.11058877878363,11.6872238768023));
#39854=CARTESIAN_POINT('Ctrl Pts',(0.32211019599974,2.11030900642974,11.6872065437466));
#39855=CARTESIAN_POINT('Ctrl Pts',(0.322140476100427,2.10933646902387,11.6871463643265));
#39856=CARTESIAN_POINT('Ctrl Pts',(0.322159810468988,2.10864364134049,11.687103622272));
#39857=CARTESIAN_POINT('Ctrl Pts',(0.322369371893727,2.10015188148049,11.686581272501));
#39858=CARTESIAN_POINT('Ctrl Pts',(0.322278610382905,2.09234783307556,11.6861169808051));
#39859=CARTESIAN_POINT('Ctrl Pts',(0.32043795575391,2.05398724855068,11.683878934921));
#39860=CARTESIAN_POINT('Ctrl Pts',(0.31462527586319,2.02378356191423,11.682240403367));
#39861=CARTESIAN_POINT('Ctrl Pts',(0.301062831114946,1.98449037510482,11.6798431320755));
#39862=CARTESIAN_POINT('Ctrl Pts',(0.296960989024225,1.97432011298298,11.6791982728875));
#39863=CARTESIAN_POINT('Ctrl Pts',(0.291513079344913,1.9625763849461,11.6784152688151));
#39864=CARTESIAN_POINT('Ctrl Pts',(0.290660089526937,1.96078133212326,11.6782945035354));
#39865=CARTESIAN_POINT('Ctrl Pts',(0.28950418149779,1.95840574535073,11.678133197943));
#39866=CARTESIAN_POINT('Ctrl Pts',(0.28921600617323,1.95781805382669,11.6780931712929));
#39867=CARTESIAN_POINT('Ctrl Pts',(0.28873905529866,1.95685283190517,11.6780272298284));
#39868=CARTESIAN_POINT('Ctrl Pts',(0.288551323903355,1.95647478528402,11.678001351547));
#39869=CARTESIAN_POINT('Ctrl Pts',(0.288185470061826,1.95574166132243,11.6779510675016));
#39870=CARTESIAN_POINT('Ctrl Pts',(0.288007432640619,1.95538654220896,11.6779266647511));
#39871=CARTESIAN_POINT('Ctrl Pts',(0.287593904419605,1.95456549821941,11.6778701389721));
#39872=CARTESIAN_POINT('Ctrl Pts',(0.287357937644618,1.95409981550732,11.6778379992714));
#39873=CARTESIAN_POINT('Ctrl Pts',(0.286720033599365,1.95284845634464,11.6777514205894));
#39874=CARTESIAN_POINT('Ctrl Pts',(0.286316001005212,1.95206385833427,11.6776969079228));
#39875=CARTESIAN_POINT('Ctrl Pts',(0.283379961551483,1.94641939447648,11.6773030775343));
#39876=CARTESIAN_POINT('Ctrl Pts',(0.280727719342338,1.94162340249499,11.6769595180058));
#39877=CARTESIAN_POINT('Ctrl Pts',(0.277042167560516,1.93534258713933,11.6764971866976));
#39878=CARTESIAN_POINT('Ctrl Pts',(0.276116687236431,1.93379530380112,11.676382267651));
#39879=CARTESIAN_POINT('Ctrl Pts',(0.262420202890649,1.91132670479636,11.6746984319663));
#39880=CARTESIAN_POINT('Ctrl Pts',(0.24731789982308,1.89192441556278,11.6730434488863));
#39881=CARTESIAN_POINT('Ctrl Pts',(0.217081169941339,1.86107229301274,11.6701217793369));
#39882=CARTESIAN_POINT('Ctrl Pts',(0.20285671410034,1.8488824526282,11.6688643320497));
#39883=CARTESIAN_POINT('Ctrl Pts',(0.187161846662895,1.83764149556746,11.6676506485025));
#39884=CARTESIAN_POINT('Ctrl Pts',(0.186668962397552,1.83729057842244,11.6676127006088));
#39885=CARTESIAN_POINT('Ctrl Pts',(0.185780924304916,1.83666208595334,11.6675446329519));
#39886=CARTESIAN_POINT('Ctrl Pts',(0.185386130893913,1.83638400790271,11.6675144796184));
#39887=CARTESIAN_POINT('Ctrl Pts',(0.18477809496137,1.83595777105278,11.6674682061021));
#39888=CARTESIAN_POINT('Ctrl Pts',(0.184565298064352,1.83580898236971,11.6674520428669));
#39889=CARTESIAN_POINT('Ctrl Pts',(0.184175330853926,1.83553701640646,11.6674224800742));
#39890=CARTESIAN_POINT('Ctrl Pts',(0.183998217371865,1.83541376038978,11.6674090751256));
#39891=CARTESIAN_POINT('Ctrl Pts',(0.183638304127025,1.83516382734951,11.667381878982));
#39892=CARTESIAN_POINT('Ctrl Pts',(0.183455497818968,1.83503716221414,11.6673680886082));
#39893=CARTESIAN_POINT('Ctrl Pts',(0.182927915287885,1.83467241193609,11.6673283552339));
#39894=CARTESIAN_POINT('Ctrl Pts',(0.182582804056972,1.83443480866878,11.6673024452228));
#39895=CARTESIAN_POINT('Ctrl Pts',(0.181055744554309,1.83338783775543,11.667188150788));
#39896=CARTESIAN_POINT('Ctrl Pts',(0.179868847435537,1.83258566681254,11.6671002487598));
#39897=CARTESIAN_POINT('Ctrl Pts',(0.155924426925709,1.81663424572912,11.6653447127623));
#39898=CARTESIAN_POINT('Ctrl Pts',(0.131331797775004,1.80443091233002,11.6638565571037));
#39899=CARTESIAN_POINT('Ctrl Pts',(0.0845123520095106,1.78821209982904,
11.6610761676898));
#39900=CARTESIAN_POINT('Ctrl Pts',(0.0628439018776408,1.78313338422472,
11.6598071939064));
#39901=CARTESIAN_POINT('Ctrl Pts',(0.0396895936633786,1.78017625556617,
11.6583877067298));
#39902=CARTESIAN_POINT('Ctrl Pts',(0.0385510293995014,1.78003701866026,
11.6583177636331));
#39903=CARTESIAN_POINT('Ctrl Pts',(0.0368897058276257,1.77984284876052,
11.6582154908786));
#39904=CARTESIAN_POINT('Ctrl Pts',(0.0363675081555351,1.77978311064028,
11.65818331278));
#39905=CARTESIAN_POINT('Ctrl Pts',(0.0354512776032882,1.77968056625419,
11.6581267988061));
#39906=CARTESIAN_POINT('Ctrl Pts',(0.0350573065073592,1.779637208813,11.6581024803519));
#39907=CARTESIAN_POINT('Ctrl Pts',(0.0342925254220064,1.77955447050031,
11.6580552378965));
#39908=CARTESIAN_POINT('Ctrl Pts',(0.0339217249089475,1.77951500619601,
11.6580323165633));
#39909=CARTESIAN_POINT('Ctrl Pts',(0.033036831818815,1.77942237993539,11.6579775775109));
#39910=CARTESIAN_POINT('Ctrl Pts',(0.0325226794131003,1.77936981105682,
11.6579457411649));
#39911=CARTESIAN_POINT('Ctrl Pts',(0.0309691866045579,1.77921475121073,
11.6578494535648));
#39912=CARTESIAN_POINT('Ctrl Pts',(0.0299294799287948,1.77911607620548,
11.6577848823937));
#39913=CARTESIAN_POINT('Ctrl Pts',(0.0189897186077547,1.77813145191743,
11.6571040810206));
#39914=CARTESIAN_POINT('Ctrl Pts',(0.00905519104353847,1.77769899141529,
11.6564736520581));
#39915=CARTESIAN_POINT('Ctrl Pts',(-0.0291243773725897,1.77780355582412,
11.6540006821517));
#39916=CARTESIAN_POINT('Ctrl Pts',(-0.0572313375997836,1.781593186946,11.6520610039077));
#39917=CARTESIAN_POINT('Ctrl Pts',(-0.095309661136734,1.79193632518954,
11.6494213132625));
#39918=CARTESIAN_POINT('Ctrl Pts',(-0.105981618639087,1.79544275905365,
11.648682253378));
#39919=CARTESIAN_POINT('Ctrl Pts',(-0.117404642485375,1.79986940506027,
11.6479072777536));
#39920=CARTESIAN_POINT('Ctrl Pts',(-0.118357654597363,1.80024394958659,
11.6478427491901));
#39921=CARTESIAN_POINT('Ctrl Pts',(-0.119998940673424,1.80089804134049,
11.6477318569634));
#39922=CARTESIAN_POINT('Ctrl Pts',(-0.120688056501404,1.8011754352792,11.6476853705573));
#39923=CARTESIAN_POINT('Ctrl Pts',(-0.121664519046595,1.80157242538911,
11.6476196106227));
#39924=CARTESIAN_POINT('Ctrl Pts',(-0.121952654504553,1.80169005624313,
11.6476002197867));
#39925=CARTESIAN_POINT('Ctrl Pts',(-0.122447672051414,1.80189298346252,
11.6475669303474));
#39926=CARTESIAN_POINT('Ctrl Pts',(-0.122654636146046,1.80197807810044,
11.6475530194641));
#39927=CARTESIAN_POINT('Ctrl Pts',(-0.123051171011972,1.8021415990362,11.6475263808877));
#39928=CARTESIAN_POINT('Ctrl Pts',(-0.123240755231485,1.80221999065973,
11.6475136510959));
#39929=CARTESIAN_POINT('Ctrl Pts',(-0.123687730851597,1.80240531163081,
11.6474836528119));
#39930=CARTESIAN_POINT('Ctrl Pts',(-0.123945059139253,1.80251239416557,
11.6474663936746));
#39931=CARTESIAN_POINT('Ctrl Pts',(-0.1247064102858,1.8028303760903,11.6474153616381));
#39932=CARTESIAN_POINT('Ctrl Pts',(-0.125210039325594,1.80304222488139,
11.6473816460411));
#39933=CARTESIAN_POINT('Ctrl Pts',(-0.129686196226932,1.80493850746372,
11.6470823395953));
#39934=CARTESIAN_POINT('Ctrl Pts',(-0.133625294777522,1.80670138272974,
11.6468214085531));
#39935=CARTESIAN_POINT('Ctrl Pts',(-0.137735783309624,1.8086409733795,11.6465505269026));
#39936=CARTESIAN_POINT('Ctrl Pts',(-0.137943433484373,1.80873922757041,
11.646536846544));
#39937=CARTESIAN_POINT('Ctrl Pts',(-0.138269322529276,1.80889385573213,
11.6465153821158));
#39938=CARTESIAN_POINT('Ctrl Pts',(-0.138387632000905,1.80895007972428,
11.6465075909386));
#39939=CARTESIAN_POINT('Ctrl Pts',(-0.14978567381247,1.81437527118008,11.6457570929036));
#39940=CARTESIAN_POINT('Ctrl Pts',(-0.160744853738672,1.82039602086603,
11.6450457422108));
#39941=CARTESIAN_POINT('Ctrl Pts',(-0.1803598637424,1.83270762170132,11.6437428903569));
#39942=CARTESIAN_POINT('Ctrl Pts',(-0.189105176985062,1.83882164713838,
11.6431499147818));
#39943=CARTESIAN_POINT('Ctrl Pts',(-0.207285848164231,1.85292479024039,
11.641859869132));
#39944=CARTESIAN_POINT('Ctrl Pts',(-0.216596969026116,1.86104539360262,
11.6411620353827));
#39945=CARTESIAN_POINT('Ctrl Pts',(-0.231558581895466,1.87568860245673,
11.6399469375239));
#39946=CARTESIAN_POINT('Ctrl Pts',(-0.237455090466544,1.88194028174133,
11.6394399111003));
#39947=CARTESIAN_POINT('Ctrl Pts',(-0.244775943077742,1.89035154944457,
11.6387677002613));
#39948=CARTESIAN_POINT('Ctrl Pts',(-0.24643426610853,1.89230337741389,11.6386123838274));
#39949=CARTESIAN_POINT('Ctrl Pts',(-0.248527944533823,1.89482799156527,
11.6384122511904));
#39950=CARTESIAN_POINT('Ctrl Pts',(-0.24898492027092,1.89538279220981,11.6383683172778));
#39951=CARTESIAN_POINT('Ctrl Pts',(-0.249716361827222,1.89627689205044,
11.6382975872743));
#39952=CARTESIAN_POINT('Ctrl Pts',(-0.24999200290181,1.89661523026778,11.638270838782));
#39953=CARTESIAN_POINT('Ctrl Pts',(-0.250514462846134,1.89725919538126,
11.6382199588735));
#39954=CARTESIAN_POINT('Ctrl Pts',(-0.250761411971926,1.8975647159801,11.6381958327699));
#39955=CARTESIAN_POINT('Ctrl Pts',(-0.251321482938759,1.89826022213501,
11.638140940097));
#39956=CARTESIAN_POINT('Ctrl Pts',(-0.251634256268489,1.8986504859026,11.6381101596129));
#39957=CARTESIAN_POINT('Ctrl Pts',(-0.252558775573924,1.89980957606703,
11.6380188020629));
#39958=CARTESIAN_POINT('Ctrl Pts',(-0.253167911413419,1.90058046848366,
11.6379581208862));
#39959=CARTESIAN_POINT('Ctrl Pts',(-0.257312961672676,1.90587584124378,
11.6375418156726));
#39960=CARTESIAN_POINT('Ctrl Pts',(-0.260730734192278,1.91049109083251,
11.6371815505319));
#39961=CARTESIAN_POINT('Ctrl Pts',(-0.264222551135567,1.91547970325174,
11.6367944717464));
#39962=CARTESIAN_POINT('Ctrl Pts',(-0.264421408764202,1.91576478342534,
11.6367723596792));
#39963=CARTESIAN_POINT('Ctrl Pts',(-0.28272655300698,1.94209752888334,11.6347306119083));
#39964=CARTESIAN_POINT('Ctrl Pts',(-0.296885704238967,1.97067267719311,
11.6325556830131));
#39965=CARTESIAN_POINT('Ctrl Pts',(-0.310277277508958,2.01208645353341,
11.6296389571148));
#39966=CARTESIAN_POINT('Ctrl Pts',(-0.313292024768791,2.02352155528033,
11.6288592359749));
#39967=CARTESIAN_POINT('Ctrl Pts',(-0.315993252829298,2.0366597811229,11.6280104143363));
#39968=CARTESIAN_POINT('Ctrl Pts',(-0.316302843572848,2.03822435303421,
11.6279100823872));
#39969=CARTESIAN_POINT('Ctrl Pts',(-0.316678608463224,2.04020026790976,
11.6277843724921));
#39970=CARTESIAN_POINT('Ctrl Pts',(-0.316755610246725,2.04060949235659,
11.6277583911777));
#39971=CARTESIAN_POINT('Ctrl Pts',(-0.316876929331963,2.041261187991,11.6277171027624));
#39972=CARTESIAN_POINT('Ctrl Pts',(-0.316921761645495,2.04150356100089,
11.627701766315));
#39973=CARTESIAN_POINT('Ctrl Pts',(-0.317005883351596,2.04196127619565,
11.6276728403506));
#39974=CARTESIAN_POINT('Ctrl Pts',(-0.317045231087765,2.04217660520874,
11.6276592476182));
#39975=CARTESIAN_POINT('Ctrl Pts',(-0.31713430998197,2.04266691059038,11.6276283315031));
#39976=CARTESIAN_POINT('Ctrl Pts',(-0.317183902820995,2.04294191116372,
11.6276110161344));
#39977=CARTESIAN_POINT('Ctrl Pts',(-0.317333738537926,2.04377900739939,
11.6275583828218));
#39978=CARTESIAN_POINT('Ctrl Pts',(-0.317432846067931,2.04434130910205,
11.6275231294424));
#39979=CARTESIAN_POINT('Ctrl Pts',(-0.318130166857817,2.04836011434741,
11.6272718800847));
#39980=CARTESIAN_POINT('Ctrl Pts',(-0.318673433607352,2.05182608577884,
11.6270589358217));
#39981=CARTESIAN_POINT('Ctrl Pts',(-0.321220880109221,2.07001513449006,
11.625957721768));
#39982=CARTESIAN_POINT('Ctrl Pts',(-0.322261887838054,2.08485656652799,
11.6251144298139));
#39983=CARTESIAN_POINT('Ctrl Pts',(-0.322294982549349,2.12272268958028,
11.6229888485315));
#39984=CARTESIAN_POINT('Ctrl Pts',(-0.319852072557969,2.14566145757631,
11.6217211217113));
#39985=CARTESIAN_POINT('Ctrl Pts',(-0.313016431727294,2.17725826061194,
11.6198362669214));
#39986=CARTESIAN_POINT('Ctrl Pts',(-0.310650298176335,2.18628147024724,
11.6192822798217));
#39987=CARTESIAN_POINT('Ctrl Pts',(-0.307559310124833,2.19627953963459,
11.6186458637341));
#39988=CARTESIAN_POINT('Ctrl Pts',(-0.307216315599347,2.19736844649967,
11.6185762479169));
#39989=CARTESIAN_POINT('Ctrl Pts',(-0.306709015321908,2.19894960748956,
11.6184747126471));
#39990=CARTESIAN_POINT('Ctrl Pts',(-0.306549292307643,2.19944333201769,
11.6184429439665));
#39991=CARTESIAN_POINT('Ctrl Pts',(-0.306265354802826,2.20031383485516,
11.6183868179411));
#39992=CARTESIAN_POINT('Ctrl Pts',(-0.306141635424202,2.20069077451988,
11.6183624769552));
#39993=CARTESIAN_POINT('Ctrl Pts',(-0.30588445925753,2.20146946548055,11.6183121144855));
#39994=CARTESIAN_POINT('Ctrl Pts',(-0.305750906308165,2.20187118399819,
11.6182860898666));
#39995=CARTESIAN_POINT('Ctrl Pts',(-0.305407058006443,2.20289868988323,
11.6182194136248));
#39996=CARTESIAN_POINT('Ctrl Pts',(-0.305195631343805,2.20352409409471,
11.6181787246628));
#39997=CARTESIAN_POINT('Ctrl Pts',(-0.304325377490146,2.20607248549372,
11.6180124908964));
#39998=CARTESIAN_POINT('Ctrl Pts',(-0.303650296585401,2.20798983583043,
11.6178864085445));
#39999=CARTESIAN_POINT('Ctrl Pts',(-0.29502677676077,2.2317618259758,11.6163103068185));
#40000=CARTESIAN_POINT('Ctrl Pts',(-0.284755217455978,2.2526958973546,11.6147786317867));
#40001=CARTESIAN_POINT('Ctrl Pts',(-0.258910288675556,2.29353508859649,
11.611519191112));
#40002=CARTESIAN_POINT('Ctrl Pts',(-0.243066944424643,2.31309394962098,
11.6097970847404));
#40003=CARTESIAN_POINT('Ctrl Pts',(-0.224088639080887,2.33161932514816,
11.6081207007523));
#40004=CARTESIAN_POINT('Ctrl Pts',(-0.223056294069078,2.33261367071816,
11.6080305880336));
#40005=CARTESIAN_POINT('Ctrl Pts',(-0.221713556015596,2.33388982520161,
11.6079148042989));
#40006=CARTESIAN_POINT('Ctrl Pts',(-0.221409220103028,2.33417794198435,
11.607888655069));
#40007=CARTESIAN_POINT('Ctrl Pts',(-0.220942504697662,2.33461806135229,
11.6078486979615));
#40008=CARTESIAN_POINT('Ctrl Pts',(-0.220780529890952,2.33477048944992,
11.6078348572157));
#40009=CARTESIAN_POINT('Ctrl Pts',(-0.220461103724958,2.33507046588285,
11.6078076145963));
#40010=CARTESIAN_POINT('Ctrl Pts',(-0.220303662892221,2.33521802291246,
11.6077942120939));
#40011=CARTESIAN_POINT('Ctrl Pts',(-0.219952558918515,2.33554642357472,
11.6077643791886));
#40012=CARTESIAN_POINT('Ctrl Pts',(-0.219758821403285,2.33572718606536,
11.6077479550864));
#40013=CARTESIAN_POINT('Ctrl Pts',(-0.219198219044171,2.33624895188041,
11.6077005376548));
#40014=CARTESIAN_POINT('Ctrl Pts',(-0.218830779799195,2.3365893410896,11.6076695914653));
#40015=CARTESIAN_POINT('Ctrl Pts',(-0.216331132347251,2.33889416503876,
11.6074599561811));
#40016=CARTESIAN_POINT('Ctrl Pts',(-0.214173206739673,2.34083068708095,
11.6072833535722));
#40017=CARTESIAN_POINT('Ctrl Pts',(-0.207319556266128,2.3468161590465,11.6067349178555));
#40018=CARTESIAN_POINT('Ctrl Pts',(-0.202532722904973,2.35075909029097,
11.6063698025944));
#40019=CARTESIAN_POINT('Ctrl Pts',(-0.186347204485524,2.36332508720379,
11.6051819168795));
#40020=CARTESIAN_POINT('Ctrl Pts',(-0.174488478988628,2.37132859515005,
11.6043843633477));
#40021=CARTESIAN_POINT('Ctrl Pts',(-0.139037686017919,2.39196591710504,
11.6020915844994));
#40022=CARTESIAN_POINT('Ctrl Pts',(-0.114359331173322,2.40248513261884,
11.6005929856368));
#40023=CARTESIAN_POINT('Ctrl Pts',(-0.0871190585330053,2.41028058063091,
11.5988756565194));
#40024=CARTESIAN_POINT('Ctrl Pts',(-0.0855675125816673,2.41071203665191,
11.5987776775778));
#40025=CARTESIAN_POINT('Ctrl Pts',(-0.0834116565349521,2.41129416783258,
11.5986412886999));
#40026=CARTESIAN_POINT('Ctrl Pts',(-0.0828100275586342,2.41145475225085,
11.5986032003335));
#40027=CARTESIAN_POINT('Ctrl Pts',(-0.0818466672458766,2.41170889991738,
11.5985421672329));
#40028=CARTESIAN_POINT('Ctrl Pts',(-0.0814852299654972,2.4118035800348,
11.5985192587074));
#40029=CARTESIAN_POINT('Ctrl Pts',(-0.0807404149639149,2.41199730416301,
11.5984720303252));
#40030=CARTESIAN_POINT('Ctrl Pts',(-0.0803570178420062,2.41209627055588,
11.5984477080009));
#40031=CARTESIAN_POINT('Ctrl Pts',(-0.0794666862001406,2.41232434272856,
11.59839119963));
#40032=CARTESIAN_POINT('Ctrl Pts',(-0.0789596188527971,2.41245292103281,
11.5983589966031));
#40033=CARTESIAN_POINT('Ctrl Pts',(-0.0773525119523605,2.41285627708525,
11.5982568671196));
#40034=CARTESIAN_POINT('Ctrl Pts',(-0.0762513433221206,2.41312648212169,
11.5981867933586));
#40035=CARTESIAN_POINT('Ctrl Pts',(-0.0566201591266331,2.41783389305874,
11.5969357698892));
#40036=CARTESIAN_POINT('Ctrl Pts',(-0.0377375416710892,2.42062418627174,
11.5957008039333));
#40037=CARTESIAN_POINT('Ctrl Pts',(0.00944724371809469,2.4233699406826,
11.5925464508341));
#40038=CARTESIAN_POINT('Ctrl Pts',(0.0377087274903272,2.42130269127191,
11.5905907828801));
#40039=CARTESIAN_POINT('Ctrl Pts',(0.0687343848253874,2.41487899055468,
11.5885559794927));
#40040=CARTESIAN_POINT('Ctrl Pts',(0.0721177987617064,2.41412134575814,
11.5883358096784));
#40041=CARTESIAN_POINT('Ctrl Pts',(0.0760415652003278,2.4131759563471,11.5880830174059));
#40042=CARTESIAN_POINT('Ctrl Pts',(0.0765942892986817,2.41304123391435,
11.5880474666515));
#40043=CARTESIAN_POINT('Ctrl Pts',(0.0774175684257859,2.41283825465783,
11.5879946050238));
#40044=CARTESIAN_POINT('Ctrl Pts',(0.077688392470774,2.41277110984718,11.5879772304781));
#40045=CARTESIAN_POINT('Ctrl Pts',(0.0781714807961838,2.41265067265336,
11.5879462649079));
#40046=CARTESIAN_POINT('Ctrl Pts',(0.078383777808129,2.41259751582194,11.5879326660541));
#40047=CARTESIAN_POINT('Ctrl Pts',(0.0788353064461566,2.4124839691251,11.5879037627345));
#40048=CARTESIAN_POINT('Ctrl Pts',(0.0790745222186617,2.41242352094474,
11.5878884617445));
#40049=CARTESIAN_POINT('Ctrl Pts',(0.0797183508833321,2.41226004304615,
11.5878473114441));
#40050=CARTESIAN_POINT('Ctrl Pts',(0.0801228351073641,2.41215650121335,
11.5878214918196));
#40051=CARTESIAN_POINT('Ctrl Pts',(0.0820834626654473,2.41165054835129,
11.5876964931322));
#40052=CARTESIAN_POINT('Ctrl Pts',(0.0836368171896738,2.41123727635507,
11.5875979336032));
#40053=CARTESIAN_POINT('Ctrl Pts',(0.0967538331240418,2.40764218182421,
11.5867691762146));
#40054=CARTESIAN_POINT('Ctrl Pts',(0.108136080432116,2.40382836196836,11.5860730393524));
#40055=CARTESIAN_POINT('Ctrl Pts',(0.148902322741741,2.38758653384137,11.5835769229432));
#40056=CARTESIAN_POINT('Ctrl Pts',(0.176607206007824,2.37145512475177,11.5818555216293));
#40057=CARTESIAN_POINT('Ctrl Pts',(0.205965880738581,2.34793561198496,11.5796257127626));
#40058=CARTESIAN_POINT('Ctrl Pts',(0.210341472724196,2.34423445762416,11.5792817185573));
#40059=CARTESIAN_POINT('Ctrl Pts',(0.215348367164173,2.33976492752099,11.578873115035));
#40060=CARTESIAN_POINT('Ctrl Pts',(0.216077854672554,2.33910771714033,11.5788131992865));
#40061=CARTESIAN_POINT('Ctrl Pts',(0.217174263682004,2.33811082465448,11.5787225604055));
#40062=CARTESIAN_POINT('Ctrl Pts',(0.217543421257456,2.33777360132404,11.5786919414006));
#40063=CARTESIAN_POINT('Ctrl Pts',(0.218195274434962,2.33717534840772,11.5786376946601));
#40064=CARTESIAN_POINT('Ctrl Pts',(0.218478290782697,2.33691466846252,11.5786140818322));
#40065=CARTESIAN_POINT('Ctrl Pts',(0.219073065837619,2.3363648625266,11.5785643303538));
#40066=CARTESIAN_POINT('Ctrl Pts',(0.219384720351546,2.33607562535388,11.5785381869753));
#40067=CARTESIAN_POINT('Ctrl Pts',(0.220020489162074,2.33548324127708,11.5784847025341));
#40068=CARTESIAN_POINT('Ctrl Pts',(0.220344551396197,2.33518004005514,11.578457359168));
#40069=CARTESIAN_POINT('Ctrl Pts',(0.221141664138062,2.3344311464515,11.5783898995624));
#40070=CARTESIAN_POINT('Ctrl Pts',(0.221613993117354,2.33398469199712,11.5783497505026));
#40071=CARTESIAN_POINT('Ctrl Pts',(0.222915662144452,2.33274685237931,11.5782386160428));
#40072=CARTESIAN_POINT('Ctrl Pts',(0.223742129140374,2.33195247210348,11.5781675009021));
#40073=CARTESIAN_POINT('Ctrl Pts',(0.230716527319223,2.32517688937974,11.5775626303178));
#40074=CARTESIAN_POINT('Ctrl Pts',(0.236627135946422,2.31895735543262,11.5770184066137));
#40075=CARTESIAN_POINT('Ctrl Pts',(0.247531626405735,2.30652516356812,11.5759498409434));
#40076=CARTESIAN_POINT('Ctrl Pts',(0.252557095316357,2.30034831564823,11.5754272606583));
#40077=CARTESIAN_POINT('Ctrl Pts',(0.276693574097054,2.26832904843085,11.5727633715538));
#40078=CARTESIAN_POINT('Ctrl Pts',(0.292090245387561,2.23991862778065,11.570519664294));
#40079=CARTESIAN_POINT('Ctrl Pts',(0.303541696016864,2.20828609953411,11.5683918240097));
#40080=CARTESIAN_POINT('Ctrl Pts',(0.304044076873539,2.2068673949384,11.5682971658994));
#40081=CARTESIAN_POINT('Ctrl Pts',(0.304676227865976,2.20504167811461,11.5681763906884));
#40082=CARTESIAN_POINT('Ctrl Pts',(0.30481514215586,2.20463788551612,11.5681497439328));
#40083=CARTESIAN_POINT('Ctrl Pts',(0.305033741165144,2.20399833798408,11.5681076436178));
#40084=CARTESIAN_POINT('Ctrl Pts',(0.305113955461257,2.20376276661909,11.5680921587004));
#40085=CARTESIAN_POINT('Ctrl Pts',(0.305257069817226,2.20334087102509,11.568064466332));
#40086=CARTESIAN_POINT('Ctrl Pts',(0.305320071738619,2.20315458347293,11.5680522528696));
#40087=CARTESIAN_POINT('Ctrl Pts',(0.305467628496894,2.202716960059,11.568023594162));
#40088=CARTESIAN_POINT('Ctrl Pts',(0.305552043537183,2.20246557780416,11.5680071573199));
#40089=CARTESIAN_POINT('Ctrl Pts',(0.305795315547532,2.20173815637049,11.5679596671004));
#40090=CARTESIAN_POINT('Ctrl Pts',(0.305953371893711,2.20126184724465,11.5679286610876));
#40091=CARTESIAN_POINT('Ctrl Pts',(0.30702350579876,2.19801157701477,11.5677176820938));
#40092=CARTESIAN_POINT('Ctrl Pts',(0.307898995649087,2.19522558617688,11.5675398263198));
#40093=CARTESIAN_POINT('Ctrl Pts',(0.310527683880753,2.18644499578954,11.5669874879647));
#40094=CARTESIAN_POINT('Ctrl Pts',(0.312144665352545,2.18041080946064,11.5666198148879));
#40095=CARTESIAN_POINT('Ctrl Pts',(0.31708200760208,2.15958187472932,11.5653793042261));
#40096=CARTESIAN_POINT('Ctrl Pts',(0.319533689838805,2.14460136218606,11.5645352961534));
#40097=CARTESIAN_POINT('Ctrl Pts',(0.323292097284807,2.10371903122009,11.5622403722068));
#40098=CARTESIAN_POINT('Ctrl Pts',(0.322546407736126,2.07774769941953,11.5607834369839));
#40099=CARTESIAN_POINT('Ctrl Pts',(0.318474713637766,2.05063012017575,11.5591205728399));
#40100=CARTESIAN_POINT('Ctrl Pts',(0.318236139905476,2.04911495905617,11.5590272239508));
#40101=CARTESIAN_POINT('Ctrl Pts',(0.317897486116887,2.04705979366299,11.5588999911668));
#40102=CARTESIAN_POINT('Ctrl Pts',(0.317806825743077,2.04651824019661,11.5588664062252));
#40103=CARTESIAN_POINT('Ctrl Pts',(0.317650805832134,2.0456006724566,11.5588094030532));
#40104=CARTESIAN_POINT('Ctrl Pts',(0.317586161337876,2.04522453644538,11.5587860075707));
#40105=CARTESIAN_POINT('Ctrl Pts',(0.317455010129089,2.04446946620519,11.5587389852895));
#40106=CARTESIAN_POINT('Ctrl Pts',(0.317388492704829,2.04409053446726,11.558715358184));
#40107=CARTESIAN_POINT('Ctrl Pts',(0.31723637356626,2.04323297325173,11.5586618215789));
#40108=CARTESIAN_POINT('Ctrl Pts',(0.317150367029671,2.04275441739204,11.5586318992426));
#40109=CARTESIAN_POINT('Ctrl Pts',(0.31696853166609,2.04175564086098,11.558569351326));
#40110=CARTESIAN_POINT('Ctrl Pts',(0.316872504423855,2.04123545820077,11.5585367194967));
#40111=CARTESIAN_POINT('Ctrl Pts',(0.316618362073062,2.03987749758475,11.5584513861567));
#40112=CARTESIAN_POINT('Ctrl Pts',(0.316458203175623,2.03904011057298,11.5583986195659));
#40113=CARTESIAN_POINT('Ctrl Pts',(0.315974804409917,2.03656592237408,11.5582422765026));
#40114=CARTESIAN_POINT('Ctrl Pts',(0.315642178415896,2.03493100383112,11.5581384012001));
#40115=CARTESIAN_POINT('Ctrl Pts',(0.313530248452106,2.02494790629779,11.5575005943022));
#40116=CARTESIAN_POINT('Ctrl Pts',(0.311432701718048,2.01667123090506,11.5569565562979));
#40117=CARTESIAN_POINT('Ctrl Pts',(0.304929189452833,1.9947107353093,11.5554707995222));
#40118=CARTESIAN_POINT('Ctrl Pts',(0.299932643241671,1.98122301314241,11.5545124166085));
#40119=CARTESIAN_POINT('Ctrl Pts',(0.283893636129505,1.9454621464165,11.5518682411617));
#40120=CARTESIAN_POINT('Ctrl Pts',(0.271149457431684,1.92405761597038,11.5501650061831));
#40121=CARTESIAN_POINT('Ctrl Pts',(0.255214831423693,1.90320425899285,11.5485063981178));
#40122=CARTESIAN_POINT('Ctrl Pts',(0.254349157280599,1.90208668508119,11.548417534166));
#40123=CARTESIAN_POINT('Ctrl Pts',(0.253218712646049,1.90064696403551,11.5483031258811));
#40124=CARTESIAN_POINT('Ctrl Pts',(0.252960648693245,1.90031960637124,11.5482771170198));
#40125=CARTESIAN_POINT('Ctrl Pts',(0.252564193232096,1.89981869919597,11.5482373280888));
#40126=CARTESIAN_POINT('Ctrl Pts',(0.252426257595767,1.89964479200313,11.5482235155826));
#40127=CARTESIAN_POINT('Ctrl Pts',(0.252153858988122,1.89930208372765,11.5481962995014));
#40128=CARTESIAN_POINT('Ctrl Pts',(0.252019406935512,1.89913327620762,11.5481828953562));
#40129=CARTESIAN_POINT('Ctrl Pts',(0.251719059114187,1.89875695916607,11.5481530175509));
#40130=CARTESIAN_POINT('Ctrl Pts',(0.251553076701583,1.89854952020756,11.5481365502864));
#40131=CARTESIAN_POINT('Ctrl Pts',(0.251071361494426,1.89794901324016,11.548088886064));
#40132=CARTESIAN_POINT('Ctrl Pts',(0.250754960778373,1.89755647832917,11.54805773701));
#40133=CARTESIAN_POINT('Ctrl Pts',(0.248567924711413,1.89485617860846,11.5478434992577));
#40134=CARTESIAN_POINT('Ctrl Pts',(0.246666301272548,1.89257353596184,11.5476626032494));
#40135=CARTESIAN_POINT('Ctrl Pts',(0.240611127960411,1.88550617459855,11.5471019945483));
#40136=CARTESIAN_POINT('Ctrl Pts',(0.236347680480554,1.88081719731685,11.5467292597696));
#40137=CARTESIAN_POINT('Ctrl Pts',(0.219573710074085,1.86342808979586,11.5453301450097));
#40138=CARTESIAN_POINT('Ctrl Pts',(0.206155180735637,1.85164740602974,11.5443449852298));
#40139=CARTESIAN_POINT('Ctrl Pts',(0.17311150715471,1.82716991228453,11.5420418936996));
#40140=CARTESIAN_POINT('Ctrl Pts',(0.15294755859425,1.81537628546624,11.5407175853775));
#40141=CARTESIAN_POINT('Ctrl Pts',(0.130432206526646,1.80529588454672,11.5392201027296));
#40142=CARTESIAN_POINT('Ctrl Pts',(0.129170369982013,1.80474063674281,11.5391361449978));
#40143=CARTESIAN_POINT('Ctrl Pts',(0.127423279541293,1.80398520488836,11.5390198405335));
#40144=CARTESIAN_POINT('Ctrl Pts',(0.126941028366662,1.80377807912628,11.5389877306425));
#40145=CARTESIAN_POINT('Ctrl Pts',(0.126113320886006,1.80342497311812,11.5389326075727));
#40146=CARTESIAN_POINT('Ctrl Pts',(0.125768110707689,1.80327841567898,11.5389096140782));
#40147=CARTESIAN_POINT('Ctrl Pts',(0.125065802000194,1.80298169944869,11.5388628279137));
#40148=CARTESIAN_POINT('Ctrl Pts',(0.124708687029687,1.80283158130509,11.5388390339072));
#40149=CARTESIAN_POINT('Ctrl Pts',(0.123886507433871,1.80248770995678,11.5387842441287));
#40150=CARTESIAN_POINT('Ctrl Pts',(0.12342125830539,1.802294403068,11.5387532332825));
#40151=CARTESIAN_POINT('Ctrl Pts',(0.122444131166048,1.80189109961964,11.5386880885259));
#40152=CARTESIAN_POINT('Ctrl Pts',(0.121932162256249,1.80168132887061,11.5386539470785));
#40153=CARTESIAN_POINT('Ctrl Pts',(0.120576076219173,1.80112976925892,11.5385634902513));
#40154=CARTESIAN_POINT('Ctrl Pts',(0.119731050689025,1.80079024004354,11.5385070987075));
#40155=CARTESIAN_POINT('Ctrl Pts',(0.117188031169288,1.79978095875797,11.5383373141451));
#40156=CARTESIAN_POINT('Ctrl Pts',(0.115485796994084,1.79912205490355,11.5382235577248));
#40157=CARTESIAN_POINT('Ctrl Pts',(0.109411809852674,1.79683006346992,11.5378172217022));
#40158=CARTESIAN_POINT('Ctrl Pts',(0.105010457466901,1.7952775775871,11.5375219911797));
#40159=CARTESIAN_POINT('Ctrl Pts',(0.09047246689367,1.79050197058509,11.5365438819269));
#40160=CARTESIAN_POINT('Ctrl Pts',(0.0802106378386884,1.78768523418066,
11.5358485710002));
#40161=CARTESIAN_POINT('Ctrl Pts',(0.0385498039188777,1.77843867658274,
11.5330128265004));
#40162=CARTESIAN_POINT('Ctrl Pts',(0.00641209109946308,1.77619976194548,
11.5307763411033));
#40163=CARTESIAN_POINT('Ctrl Pts',(-0.0270412416340491,1.7788578899055,
11.5286534656157));
#40164=CARTESIAN_POINT('Ctrl Pts',(-0.0285548445712876,1.77898893369204,
11.5285579044613));
#40165=CARTESIAN_POINT('Ctrl Pts',(-0.0304891801006262,1.77917019325197,
11.5284364544719));
#40166=CARTESIAN_POINT('Ctrl Pts',(-0.030910785612659,1.77921053892174,
11.5284100243671));
#40167=CARTESIAN_POINT('Ctrl Pts',(-0.0315816542997596,1.77927607276519,
11.5283680347349));
#40168=CARTESIAN_POINT('Ctrl Pts',(-0.0318309679062435,1.77930072049908,
11.5283524448505));
#40169=CARTESIAN_POINT('Ctrl Pts',(-0.0322974772923847,1.77934739008711,
11.5283233011713));
#40170=CARTESIAN_POINT('Ctrl Pts',(-0.0325146777762391,1.77936934174519,
11.5283097435552));
#40171=CARTESIAN_POINT('Ctrl Pts',(-0.0330036834853458,1.77941926576802,
11.5282792451786));
#40172=CARTESIAN_POINT('Ctrl Pts',(-0.0332754749191719,1.77944736305164,
11.5282623116014));
#40173=CARTESIAN_POINT('Ctrl Pts',(-0.0340847077635674,1.77953206031344,
11.5282119448954));
#40174=CARTESIAN_POINT('Ctrl Pts',(-0.034622046298193,1.77958966684823,
11.5281785684253));
#40175=CARTESIAN_POINT('Ctrl Pts',(-0.0390589036127109,1.78007662133725,
11.5279035146523));
#40176=CARTESIAN_POINT('Ctrl Pts',(-0.0429506406741204,1.78057581178246,
11.527665694334));
#40177=CARTESIAN_POINT('Ctrl Pts',(-0.0555676082576323,1.78242896119883,
11.5269030683628));
#40178=CARTESIAN_POINT('Ctrl Pts',(-0.0642470442662829,1.78407047211645,
11.5263914977357));
#40179=CARTESIAN_POINT('Ctrl Pts',(-0.0874190444930373,1.78944757111988,
11.5250352567948));
#40180=CARTESIAN_POINT('Ctrl Pts',(-0.101736753244368,1.79383898697891,
11.5242068343924));
#40181=CARTESIAN_POINT('Ctrl Pts',(-0.123807947510714,1.80232858946436,
11.5228814082342));
#40182=CARTESIAN_POINT('Ctrl Pts',(-0.131788075182596,1.80577462666305,
11.5223917619239));
#40183=CARTESIAN_POINT('Ctrl Pts',(-0.152379927611386,1.81567272188714,
11.5210844163471));
#40184=CARTESIAN_POINT('Ctrl Pts',(-0.164721228471299,1.82264016020916,
11.5202550805417));
#40185=CARTESIAN_POINT('Ctrl Pts',(-0.177594807922572,1.83107105123723,
11.5193200036892));
#40186=CARTESIAN_POINT('Ctrl Pts',(-0.178622185018869,1.83175233414479,
11.519244878741));
#40187=CARTESIAN_POINT('Ctrl Pts',(-0.180060992451828,1.83271837897171,
11.5191389520845));
#40188=CARTESIAN_POINT('Ctrl Pts',(-0.180475715992405,1.8329982361953,11.5191083353731));
#40189=CARTESIAN_POINT('Ctrl Pts',(-0.18119484628816,1.83348594939298,11.5190550986719));
#40190=CARTESIAN_POINT('Ctrl Pts',(-0.181499552062431,1.83369336453694,
11.5190324953979));
#40191=CARTESIAN_POINT('Ctrl Pts',(-0.182126812189448,1.83412192107684,
11.5189858693268));
#40192=CARTESIAN_POINT('Ctrl Pts',(-0.182449321087705,1.83434312769534,
11.5189618440763));
#40193=CARTESIAN_POINT('Ctrl Pts',(-0.183204797520332,1.83486332835797,
11.5189054418962));
#40194=CARTESIAN_POINT('Ctrl Pts',(-0.183637436077162,1.83516279613761,
11.5188730469564));
#40195=CARTESIAN_POINT('Ctrl Pts',(-0.184548922504466,1.83579702464247,
11.5188045950571));
#40196=CARTESIAN_POINT('Ctrl Pts',(-0.185027596833968,1.83613203038645,
11.5187685287924));
#40197=CARTESIAN_POINT('Ctrl Pts',(-0.18631111447421,1.83703552482912,11.518671501027));
#40198=CARTESIAN_POINT('Ctrl Pts',(-0.187114261084638,1.83760640281702,
11.5186104478904));
#40199=CARTESIAN_POINT('Ctrl Pts',(-0.189565136793502,1.83936546406545,
11.518423089598));
#40200=CARTESIAN_POINT('Ctrl Pts',(-0.191204235688836,1.84056553359353,
11.5182963264613));
#40201=CARTESIAN_POINT('Ctrl Pts',(-0.19715353969909,1.84500833325495,11.5178307830151));
#40202=CARTESIAN_POINT('Ctrl Pts',(-0.201393303248048,1.84834348781353,
11.5174884248549));
#40203=CARTESIAN_POINT('Ctrl Pts',(-0.210134151579303,1.85558174706168,
11.5167596100325));
#40204=CARTESIAN_POINT('Ctrl Pts',(-0.214614703007654,1.85950641088499,
11.5163724123246));
#40205=CARTESIAN_POINT('Ctrl Pts',(-0.2310119738557,1.87469261431733,11.5149038770566));
#40206=CARTESIAN_POINT('Ctrl Pts',(-0.242171708430901,1.88673319717696,
11.5137961238617));
#40207=CARTESIAN_POINT('Ctrl Pts',(-0.264590190256713,1.91496072656484,
11.5113568924354));
#40208=CARTESIAN_POINT('Ctrl Pts',(-0.275382114609853,1.93144026323942,
11.510029418704));
#40209=CARTESIAN_POINT('Ctrl Pts',(-0.285139433592585,1.94980688134202,
11.5087184598918));
#40210=CARTESIAN_POINT('Ctrl Pts',(-0.285667777237769,1.95081424122439,
11.5086470714868));
#40211=CARTESIAN_POINT('Ctrl Pts',(-0.286366672148987,1.95216410771361,
11.5085521173304));
#40212=CARTESIAN_POINT('Ctrl Pts',(-0.286541954849484,1.9525041353785,11.508528258278));
#40213=CARTESIAN_POINT('Ctrl Pts',(-0.286814829203746,1.9530358015649,11.508491046378));
#40214=CARTESIAN_POINT('Ctrl Pts',(-0.286912834453933,1.9532272256203,11.5084776674048));
#40215=CARTESIAN_POINT('Ctrl Pts',(-0.28710025662649,1.95359420406155,11.5084520552274));
#40216=CARTESIAN_POINT('Ctrl Pts',(-0.287189703530052,1.95376974107267,
11.5084398201949));
#40217=CARTESIAN_POINT('Ctrl Pts',(-0.287400769416072,1.95418489252018,
11.5084109217064));
#40218=CARTESIAN_POINT('Ctrl Pts',(-0.287522249568002,1.95442457681697,
11.5083942671111));
#40219=CARTESIAN_POINT('Ctrl Pts',(-0.287877300741607,1.9551272824667,11.5083455254019));
#40220=CARTESIAN_POINT('Ctrl Pts',(-0.288110055483813,1.95559071876869,
11.5083134895959));
#40221=CARTESIAN_POINT('Ctrl Pts',(-0.289820138716054,1.9590162446977,11.5080774869168));
#40222=CARTESIAN_POINT('Ctrl Pts',(-0.291252941172031,1.96200051305261,
11.5078762524734));
#40223=CARTESIAN_POINT('Ctrl Pts',(-0.295849678470874,1.97196534042078,
11.5072169495189));
#40224=CARTESIAN_POINT('Ctrl Pts',(-0.298810795011803,1.97903705817536,
11.5067693345922));
#40225=CARTESIAN_POINT('Ctrl Pts',(-0.307023728810907,2.0007990766942,11.5054332065256));
#40226=CARTESIAN_POINT('Ctrl Pts',(-0.311464204206702,2.01577118909666,
11.5045687718015));
#40227=CARTESIAN_POINT('Ctrl Pts',(-0.31976848465604,2.0536619885797,11.5023974765617));
#40228=CARTESIAN_POINT('Ctrl Pts',(-0.322272754439886,2.07678245867823,
11.5010822755746));
#40229=CARTESIAN_POINT('Ctrl Pts',(-0.322274998490625,2.09996880917294,
11.4996790403846));
#40230=CARTESIAN_POINT('',(-0.322274977094782,2.09987849461815,11.2490951747016));
#40231=CARTESIAN_POINT('Ctrl Pts',(-0.322274998502865,2.0999689359024,11.499679032715));
#40232=CARTESIAN_POINT('Ctrl Pts',(-0.322275099486767,2.1010165950739,11.4996156284931));
#40233=CARTESIAN_POINT('Ctrl Pts',(-0.322270091837628,2.10206424137144,
11.4995520677508));
#40234=CARTESIAN_POINT('Ctrl Pts',(-0.322250763173066,2.10406590582397,
11.4994303174676));
#40235=CARTESIAN_POINT('Ctrl Pts',(-0.322237313678586,2.10501992015537,
11.4993721557721));
#40236=CARTESIAN_POINT('Ctrl Pts',(-0.322211300242446,2.10642304140411,
11.4992864120943));
#40237=CARTESIAN_POINT('Ctrl Pts',(-0.322202033181655,2.1068722103572,11.499258933258));
#40238=CARTESIAN_POINT('Ctrl Pts',(-0.322183414761047,2.10769155343982,
11.4992087521226));
#40239=CARTESIAN_POINT('Ctrl Pts',(-0.322174364562626,2.108061734197,11.4991860592853));
#40240=CARTESIAN_POINT('Ctrl Pts',(-0.322155452750297,2.10878431390489,
11.4991417225374));
#40241=CARTESIAN_POINT('Ctrl Pts',(-0.322145650852467,2.10913671400454,
11.4991200805285));
#40242=CARTESIAN_POINT('Ctrl Pts',(-0.322121913947223,2.10994253304504,
11.4990705486242));
#40243=CARTESIAN_POINT('Ctrl Pts',(-0.322107599802702,2.11039593932095,
11.4990426468884));
#40244=CARTESIAN_POINT('Ctrl Pts',(-0.322066224517841,2.11162428097165,
11.4989669700515));
#40245=CARTESIAN_POINT('Ctrl Pts',(-0.322037323927901,2.11239914770598,
11.4989191373895));
#40246=CARTESIAN_POINT('Ctrl Pts',(-0.321900227497391,2.11575015473037,
11.4987118670454));
#40247=CARTESIAN_POINT('Ctrl Pts',(-0.321763916376092,2.11832499204841,
11.4985515505396));
#40248=CARTESIAN_POINT('Ctrl Pts',(-0.319263892784774,2.15679780651772,
11.4961397562275));
#40249=CARTESIAN_POINT('Ctrl Pts',(-0.310935952237075,2.19204820152477,
11.4936741023558));
#40250=CARTESIAN_POINT('Ctrl Pts',(-0.292507500731267,2.23576630667989,
11.4904977398617));
#40251=CARTESIAN_POINT('Ctrl Pts',(-0.287482295100116,2.2461065314714,11.4897406225045));
#40252=CARTESIAN_POINT('Ctrl Pts',(-0.281153711068542,2.25753169482296,
11.4889142598651));
#40253=CARTESIAN_POINT('Ctrl Pts',(-0.280382358983871,2.25890052589766,
11.4888154316593));
#40254=CARTESIAN_POINT('Ctrl Pts',(-0.279395006402081,2.26062309182209,
11.4886913419045));
#40255=CARTESIAN_POINT('Ctrl Pts',(-0.279188309941846,2.26098209473509,
11.4886654954915));
#40256=CARTESIAN_POINT('Ctrl Pts',(-0.278857764268774,2.26155365501622,
11.4886243717364));
#40257=CARTESIAN_POINT('Ctrl Pts',(-0.278734363776928,2.26176646930969,
11.4886090654487));
#40258=CARTESIAN_POINT('Ctrl Pts',(-0.278500655260794,2.26216845747054,
11.4885801642548));
#40259=CARTESIAN_POINT('Ctrl Pts',(-0.278390399007472,2.26235765864237,
11.4885665662065));
#40260=CARTESIAN_POINT('Ctrl Pts',(-0.278138603285059,2.262788732787,11.4885355950427));
#40261=CARTESIAN_POINT('Ctrl Pts',(-0.277996941361132,2.26303053319867,
11.488518230049));
#40262=CARTESIAN_POINT('Ctrl Pts',(-0.277573327529032,2.2637514351171,11.4884664796885));
#40263=CARTESIAN_POINT('Ctrl Pts',(-0.27729044935753,2.26422999532499,11.4884321543444));
#40264=CARTESIAN_POINT('Ctrl Pts',(-0.275295345043811,2.26758537037305,
11.4881916679761));
#40265=CARTESIAN_POINT('Ctrl Pts',(-0.273539542368667,2.27043621757659,
11.4879882844259));
#40266=CARTESIAN_POINT('Ctrl Pts',(-0.263757127463278,2.28577893642419,
11.4868959496517));
#40267=CARTESIAN_POINT('Ctrl Pts',(-0.25491804438629,2.29773348066788,11.4860525721841));
#40268=CARTESIAN_POINT('Ctrl Pts',(-0.225675311325338,2.33204705575656,
11.483521013414));
#40269=CARTESIAN_POINT('Ctrl Pts',(-0.202928302829027,2.35218072922635,
11.481859864261));
#40270=CARTESIAN_POINT('Ctrl Pts',(-0.176096250597378,2.36991670446061,
11.4799250680259));
#40271=CARTESIAN_POINT('Ctrl Pts',(-0.174473134938694,2.37096870992292,
11.4798081929933));
#40272=CARTESIAN_POINT('Ctrl Pts',(-0.172038542058987,2.37251572226197,
11.4796330839575));
#40273=CARTESIAN_POINT('Ctrl Pts',(-0.171234165914402,2.37302186584085,
11.4795752607826));
#40274=CARTESIAN_POINT('Ctrl Pts',(-0.169943980107026,2.37382575463158,
11.4794825605243));
#40275=CARTESIAN_POINT('Ctrl Pts',(-0.169459595047152,2.37412578483988,
11.4794477675519));
#40276=CARTESIAN_POINT('Ctrl Pts',(-0.168535344675143,2.3746948836423,11.479381397671));
#40277=CARTESIAN_POINT('Ctrl Pts',(-0.168095623858632,2.37496418446539,
11.479349829408));
#40278=CARTESIAN_POINT('Ctrl Pts',(-0.167322805386222,2.37543493961424,
11.4792943604496));
#40279=CARTESIAN_POINT('Ctrl Pts',(-0.166989984642264,2.37563684838867,
11.4792704764686));
#40280=CARTESIAN_POINT('Ctrl Pts',(-0.166338962227335,2.37603018524685,
11.479223765414));
#40281=CARTESIAN_POINT('Ctrl Pts',(-0.166020793780224,2.37622166742142,
11.4792009403648));
#40282=CARTESIAN_POINT('Ctrl Pts',(-0.16526406560645,2.37667530664248,11.4791466617775));
#40283=CARTESIAN_POINT('Ctrl Pts',(-0.16482521298458,2.37693697089098,11.4791151903267));
#40284=CARTESIAN_POINT('Ctrl Pts',(-0.163272195535001,2.37785795265877,
11.4790038405145));
#40285=CARTESIAN_POINT('Ctrl Pts',(-0.162154693317995,2.3785115923028,11.4789237561517));
#40286=CARTESIAN_POINT('Ctrl Pts',(-0.144001112821963,2.38898353272403,
11.4776233458485));
#40287=CARTESIAN_POINT('Ctrl Pts',(-0.126108816074974,2.39722737567277,
11.4763454014616));
#40288=CARTESIAN_POINT('Ctrl Pts',(-0.0982467335899388,2.40709410472849,
11.4743685632446));
#40289=CARTESIAN_POINT('Ctrl Pts',(-0.088766373968394,2.4099673030876,11.4736988387156));
#40290=CARTESIAN_POINT('Ctrl Pts',(-0.0714363988427003,2.41435911294969,
11.4724890071636));
#40291=CARTESIAN_POINT('Ctrl Pts',(-0.0636334050071042,2.41603102103039,
11.4719494526071));
#40292=CARTESIAN_POINT('Ctrl Pts',(-0.0443777946816995,2.419414658434,11.470640203911));
#40293=CARTESIAN_POINT('Ctrl Pts',(-0.0328783151121363,2.42080241689272,
11.469877166965));
#40294=CARTESIAN_POINT('Ctrl Pts',(-0.020289506899484,2.42163736500157,
11.4690788757297));
#40295=CARTESIAN_POINT('Ctrl Pts',(-0.019250756896274,2.42170120777318,
11.4690132811013));
#40296=CARTESIAN_POINT('Ctrl Pts',(-0.0174604423789802,2.4218025400341,
11.4689007223165));
#40297=CARTESIAN_POINT('Ctrl Pts',(-0.0167090295677126,2.4218424306681,
11.4688536305295));
#40298=CARTESIAN_POINT('Ctrl Pts',(-0.0156450045574491,2.42189518066471,
11.468787166297));
#40299=CARTESIAN_POINT('Ctrl Pts',(-0.0153325101002077,2.42191021673564,
11.4687676731249));
#40300=CARTESIAN_POINT('Ctrl Pts',(-0.0147961569684847,2.42193524127602,
11.4687342623279));
#40301=CARTESIAN_POINT('Ctrl Pts',(-0.0145723092897989,2.42194545134163,
11.4687203321926));
#40302=CARTESIAN_POINT('Ctrl Pts',(-0.0141438508557647,2.42196454626536,
11.4686936958779));
#40303=CARTESIAN_POINT('Ctrl Pts',(-0.0139392425620056,2.42197346953789,
11.4686809875242));
#40304=CARTESIAN_POINT('Ctrl Pts',(-0.0134575333082109,2.42199401755607,
11.4686510954841));
#40305=CARTESIAN_POINT('Ctrl Pts',(-0.0131804250432202,2.42200547967644,
11.46863392099));
#40306=CARTESIAN_POINT('Ctrl Pts',(-0.0123627202737596,2.42203824535184,
11.468583303329));
#40307=CARTESIAN_POINT('Ctrl Pts',(-0.0118220811168599,2.42205854550056,
11.4685499161619));
#40308=CARTESIAN_POINT('Ctrl Pts',(-0.00711694632201651,2.42222335197574,
11.4682600229133));
#40309=CARTESIAN_POINT('Ctrl Pts',(-0.00294982476750907,2.42228844537827,
11.4680078600452));
#40310=CARTESIAN_POINT('Ctrl Pts',(0.0348191690993515,2.42214574517247,
11.4657544547342));
#40311=CARTESIAN_POINT('Ctrl Pts',(0.0681982705008702,2.41676484451376,
11.4639737192927));
#40312=CARTESIAN_POINT('Ctrl Pts',(0.109349437952026,2.40331109514354,11.4614842261548));
#40313=CARTESIAN_POINT('Ctrl Pts',(0.118411268170538,2.39988942290897,11.4609179314254));
#40314=CARTESIAN_POINT('Ctrl Pts',(0.129566858940363,2.39509264252856,11.4601906293601));
#40315=CARTESIAN_POINT('Ctrl Pts',(0.131817648449671,2.39409411020995,11.4600423146492));
#40316=CARTESIAN_POINT('Ctrl Pts',(0.135089797935967,2.39259735585401,11.4598242933062));
#40317=CARTESIAN_POINT('Ctrl Pts',(0.13612035074755,2.39211935269724,11.4597552762567));
#40318=CARTESIAN_POINT('Ctrl Pts',(0.137732722919111,2.39136109844096,11.4596467320565));
#40319=CARTESIAN_POINT('Ctrl Pts',(0.138316270542451,2.39108452714142,11.4596073317756));
#40320=CARTESIAN_POINT('Ctrl Pts',(0.139413540868271,2.3905604333434,11.4595330249397));
#40321=CARTESIAN_POINT('Ctrl Pts',(0.139927446235233,2.39031329729384,11.4594981318693));
#40322=CARTESIAN_POINT('Ctrl Pts',(0.140800361237079,2.38989065798852,11.459438705858));
#40323=CARTESIAN_POINT('Ctrl Pts',(0.141159706592269,2.38971584793727,11.4594141970884));
#40324=CARTESIAN_POINT('Ctrl Pts',(0.141875440732306,2.38936601836966,11.4593652902418));
#40325=CARTESIAN_POINT('Ctrl Pts',(0.14223183307106,2.38919100769059,11.4593408925058));
#40326=CARTESIAN_POINT('Ctrl Pts',(0.14302225731945,2.38880104591987,11.459286681423));
#40327=CARTESIAN_POINT('Ctrl Pts',(0.143456129273519,2.38858577439461,11.4592568569069));
#40328=CARTESIAN_POINT('Ctrl Pts',(0.144934102996692,2.38784830077549,11.459155028864));
#40329=CARTESIAN_POINT('Ctrl Pts',(0.14597584252845,2.38732140855043,11.4590828610627));
#40330=CARTESIAN_POINT('Ctrl Pts',(0.156555869938985,2.38189783899782,11.4583458390003));
#40331=CARTESIAN_POINT('Ctrl Pts',(0.165845996589991,2.37653425400956,11.4576644588148));
#40332=CARTESIAN_POINT('Ctrl Pts',(0.191418932790986,2.3600172712934,11.4556862858127));
#40333=CARTESIAN_POINT('Ctrl Pts',(0.206967948304152,2.34781905697087,11.4543547210414));
#40334=CARTESIAN_POINT('Ctrl Pts',(0.224239975295333,2.33150363854518,11.4527470631791));
#40335=CARTESIAN_POINT('Ctrl Pts',(0.227124799251591,2.3286740633799,11.4524738420395));
#40336=CARTESIAN_POINT('Ctrl Pts',(0.232897783138565,2.32279459709926,11.4519183112049));
#40337=CARTESIAN_POINT('Ctrl Pts',(0.235781107814682,2.31974093962852,11.4516361155775));
#40338=CARTESIAN_POINT('Ctrl Pts',(0.245801185449163,2.30870455873079,11.4506405023665));
#40339=CARTESIAN_POINT('Ctrl Pts',(0.252599707040138,2.30042269000668,11.4499368973252));
#40340=CARTESIAN_POINT('Ctrl Pts',(0.259873551972031,2.29060219656546,11.4491640796824));
#40341=CARTESIAN_POINT('Ctrl Pts',(0.260764673861288,2.28938121720207,11.4490690322456));
#40342=CARTESIAN_POINT('Ctrl Pts',(0.261885802040222,2.28782217480185,11.4489490262113));
#40343=CARTESIAN_POINT('Ctrl Pts',(0.262123781509663,2.28748990860582,11.4489235280372));
#40344=CARTESIAN_POINT('Ctrl Pts',(0.262503270459444,2.28695793251417,11.4488828294243));
#40345=CARTESIAN_POINT('Ctrl Pts',(0.262645184616516,2.28675851394405,11.4488676010649));
#40346=CARTESIAN_POINT('Ctrl Pts',(0.26291378186107,2.28638016792461,11.4488387626131));
#40347=CARTESIAN_POINT('Ctrl Pts',(0.263040508499757,2.28620127436881,11.4488251495694));
#40348=CARTESIAN_POINT('Ctrl Pts',(0.263330057784839,2.28579164685265,11.4487940302376));
#40349=CARTESIAN_POINT('Ctrl Pts',(0.263492759516144,2.28556082845583,11.4487765323604));
#40350=CARTESIAN_POINT('Ctrl Pts',(0.263992073592508,2.28485049080302,11.4487227968521));
#40351=CARTESIAN_POINT('Ctrl Pts',(0.264327684286568,2.28437026387744,11.4486866278184));
#40352=CARTESIAN_POINT('Ctrl Pts',(0.266843949689678,2.28074873476982,11.4484150402188));
#40353=CARTESIAN_POINT('Ctrl Pts',(0.268969963243728,2.27756959371364,11.4481832570298));
#40354=CARTESIAN_POINT('Ctrl Pts',(0.271353787627852,2.27386384363646,11.4479197001052));
#40355=CARTESIAN_POINT('Ctrl Pts',(0.271667253712895,2.27337363540563,11.4478849674402));
#40356=CARTESIAN_POINT('Ctrl Pts',(0.288269994341243,2.24725415373155,11.4460411581386));
#40357=CARTESIAN_POINT('Ctrl Pts',(0.30085862087886,2.21944874733956,11.4444151023456));
#40358=CARTESIAN_POINT('Ctrl Pts',(0.31146520517992,2.18310588371104,11.4422597171165));
#40359=CARTESIAN_POINT('Ctrl Pts',(0.313310588607304,2.17585266633669,11.4418289820176));
#40360=CARTESIAN_POINT('Ctrl Pts',(0.316128907222517,2.16290451368283,11.4410535042307));
#40361=CARTESIAN_POINT('Ctrl Pts',(0.31720432306609,2.15723526241841,11.4407118033176));
#40362=CARTESIAN_POINT('Ctrl Pts',(0.318468392006984,2.14943295465982,11.4402371406345));
#40363=CARTESIAN_POINT('Ctrl Pts',(0.318788873850223,2.14732216489365,11.4401082940329));
#40364=CARTESIAN_POINT('Ctrl Pts',(0.319231747721815,2.14419628688937,11.4399167817488));
#40365=CARTESIAN_POINT('Ctrl Pts',(0.319370324105763,2.14318352199022,11.4398546242671));
#40366=CARTESIAN_POINT('Ctrl Pts',(0.319582514386165,2.14157585158959,11.4397557762692));
#40367=CARTESIAN_POINT('Ctrl Pts',(0.319659291547239,2.14098136474885,11.439719185386));
#40368=CARTESIAN_POINT('Ctrl Pts',(0.319801633734589,2.13985446582775,11.4396497495591));
#40369=CARTESIAN_POINT('Ctrl Pts',(0.319867528948603,2.13932209689917,11.4396169151304));
#40370=CARTESIAN_POINT('Ctrl Pts',(0.31996140237849,2.13854783917416,11.4395691152713));
#40371=CARTESIAN_POINT('Ctrl Pts',(0.319990436357057,2.13830607727909,11.4395541831574));
#40372=CARTESIAN_POINT('Ctrl Pts',(0.320064618999412,2.13768239892331,11.4395156452872));
#40373=CARTESIAN_POINT('Ctrl Pts',(0.320109357994325,2.13730043493417,11.4394920266442));
#40374=CARTESIAN_POINT('Ctrl Pts',(0.320210661597778,2.13642193802021,11.4394376664272));
#40375=CARTESIAN_POINT('Ctrl Pts',(0.320266755062864,2.13592535270603,11.4394069100561));
#40376=CARTESIAN_POINT('Ctrl Pts',(0.32042950410366,2.13445388649695,11.4393156887068));
#40377=CARTESIAN_POINT('Ctrl Pts',(0.320532864331179,2.13347865356412,11.4392551200791));
#40378=CARTESIAN_POINT('Ctrl Pts',(0.321207458607547,2.12682398969673,11.4388410488103));
#40379=CARTESIAN_POINT('Ctrl Pts',(0.321632135590966,2.12113103200114,11.4384829612592));
#40380=CARTESIAN_POINT('Ctrl Pts',(0.323401327081103,2.08422180573654,11.4361344265199));
#40381=CARTESIAN_POINT('Ctrl Pts',(0.320350390423041,2.05296599248663,11.4339977024744));
#40382=CARTESIAN_POINT('Ctrl Pts',(0.309558844462763,2.00931922038741,11.4309785531798));
#40383=CARTESIAN_POINT('Ctrl Pts',(0.305414583016254,1.99621312605224,11.4300710101978));
#40384=CARTESIAN_POINT('Ctrl Pts',(0.300171775123826,1.98270270036126,11.4291612766139));
#40385=CARTESIAN_POINT('Ctrl Pts',(0.299894839063215,1.98199645507691,11.429113798996));
#40386=CARTESIAN_POINT('Ctrl Pts',(0.299499789011998,1.98099936751194,11.429046886384));
#40387=CARTESIAN_POINT('Ctrl Pts',(0.299383742588535,1.98070771681925,11.4290273284594));
#40388=CARTESIAN_POINT('Ctrl Pts',(0.299184050149406,1.98020797163346,11.4289938407599));
#40389=CARTESIAN_POINT('Ctrl Pts',(0.29910061282879,1.97999979445627,11.4289798983277));
#40390=CARTESIAN_POINT('Ctrl Pts',(0.298940646929157,1.97960188085142,11.4289532629432));
#40391=CARTESIAN_POINT('Ctrl Pts',(0.298864155086619,1.97941213043648,11.4289405677695));
#40392=CARTESIAN_POINT('Ctrl Pts',(0.298683862137945,1.97896610982035,11.4289107413907));
#40393=CARTESIAN_POINT('Ctrl Pts',(0.2985799116175,1.97870989960647,11.428893619277));
#40394=CARTESIAN_POINT('Ctrl Pts',(0.298272832111733,1.97795581789813,11.4288432573979));
#40395=CARTESIAN_POINT('Ctrl Pts',(0.298068785393743,1.97745831752176,11.4288100728361));
#40396=CARTESIAN_POINT('Ctrl Pts',(0.296306614940954,1.97319229100682,11.4285258539455));
#40397=CARTESIAN_POINT('Ctrl Pts',(0.294678251095913,1.96945293103433,11.4282789774995));
#40398=CARTESIAN_POINT('Ctrl Pts',(0.292524022787654,1.96475183592434,11.4279702517209));
#40399=CARTESIAN_POINT('Ctrl Pts',(0.292063731776089,1.96376070157079,11.4279052569048));
#40400=CARTESIAN_POINT('Ctrl Pts',(0.291549097490608,1.96266714601046,11.4278336293091));
#40401=CARTESIAN_POINT('Ctrl Pts',(0.291499736042787,1.96256240354417,11.4278267695566));
#40402=CARTESIAN_POINT('Ctrl Pts',(0.291262961256112,1.96206068094208,11.4277939149084));
#40403=CARTESIAN_POINT('Ctrl Pts',(0.291074792508294,1.96166405560422,11.4277679543356));
#40404=CARTESIAN_POINT('Ctrl Pts',(0.280057161954155,1.93856291004629,11.4262565256465));
#40405=CARTESIAN_POINT('Ctrl Pts',(0.26660633350777,1.91720146391741,11.4248884855704));
#40406=CARTESIAN_POINT('Ctrl Pts',(0.239618237195677,1.88375551133249,11.4224661705895));
#40407=CARTESIAN_POINT('Ctrl Pts',(0.227301585258933,1.87084407132313,11.4214422151618));
#40408=CARTESIAN_POINT('Ctrl Pts',(0.212675172725801,1.85785644170849,11.4202636956892));
#40409=CARTESIAN_POINT('Ctrl Pts',(0.211358525140154,1.85670633879562,11.4201579346938));
#40410=CARTESIAN_POINT('Ctrl Pts',(0.209363430169687,1.85499202431341,11.4199981328109));
#40411=CARTESIAN_POINT('Ctrl Pts',(0.20869190239758,1.85441978114678,11.4199444219011));
#40412=CARTESIAN_POINT('Ctrl Pts',(0.2076045101523,1.8535008395092,11.4198575680532));
#40413=CARTESIAN_POINT('Ctrl Pts',(0.207190103872449,1.85315241623636,11.419824495693));
#40414=CARTESIAN_POINT('Ctrl Pts',(0.206394984843502,1.85248731126307,11.4197610918534));
#40415=CARTESIAN_POINT('Ctrl Pts',(0.206014416009136,1.85217045929425,11.419730767429));
#40416=CARTESIAN_POINT('Ctrl Pts',(0.205335787486942,1.85160809369365,11.4196767325492));
#40417=CARTESIAN_POINT('Ctrl Pts',(0.205038013334749,1.85136223571826,11.4196530361506));
#40418=CARTESIAN_POINT('Ctrl Pts',(0.20444782292304,1.85087672475632,11.4196060959728));
#40419=CARTESIAN_POINT('Ctrl Pts',(0.204155425333689,1.85063704992314,11.4195828531303));
#40420=CARTESIAN_POINT('Ctrl Pts',(0.203447407510393,1.85005877612463,11.4195266026581));
#40421=CARTESIAN_POINT('Ctrl Pts',(0.203031363903342,1.84972069945555,11.419493574015));
#40422=CARTESIAN_POINT('Ctrl Pts',(0.201487768961774,1.848472757312,11.41937112307));
#40423=CARTESIAN_POINT('Ctrl Pts',(0.200354942296662,1.84756947125457,11.4192814370363));
#40424=CARTESIAN_POINT('Ctrl Pts',(0.181275877559256,1.83256566414207,11.4177737993979));
#40425=CARTESIAN_POINT('Ctrl Pts',(0.161891611982213,1.82040604046788,11.4162769405174));
#40426=CARTESIAN_POINT('Ctrl Pts',(0.125092269501113,1.80243987375647,11.41351982038));
#40427=CARTESIAN_POINT('Ctrl Pts',(0.108151860438058,1.79587288790738,11.4122808171936));
#40428=CARTESIAN_POINT('Ctrl Pts',(0.0846397711225724,1.7889729609589,11.4106593261453));
#40429=CARTESIAN_POINT('Ctrl Pts',(0.078478514648324,1.7873614803117,11.4102433906528));
#40430=CARTESIAN_POINT('Ctrl Pts',(0.06934940390309,1.78526068437766,11.4096440118448));
#40431=CARTESIAN_POINT('Ctrl Pts',(0.0664162700588182,1.78462869933861,
11.4094539725711));
#40432=CARTESIAN_POINT('Ctrl Pts',(0.062979010804003,1.78393817795183,11.4092345664235));
#40433=CARTESIAN_POINT('Ctrl Pts',(0.0624831720564446,1.78383978052845,
11.4092029960339));
#40434=CARTESIAN_POINT('Ctrl Pts',(0.0617261136775131,1.78369139555529,
11.4091549175691));
#40435=CARTESIAN_POINT('Ctrl Pts',(0.0614650631572211,1.78364056459812,
11.4091383615193));
#40436=CARTESIAN_POINT('Ctrl Pts',(0.0609920549182021,1.78354906945807,
11.4091084039986));
#40437=CARTESIAN_POINT('Ctrl Pts',(0.0607801200964875,1.78350829520217,
11.4090949962657));
#40438=CARTESIAN_POINT('Ctrl Pts',(0.0603503060075456,1.78342605069282,
11.4090678350604));
#40439=CARTESIAN_POINT('Ctrl Pts',(0.0601324258355243,1.78338459263799,
11.409054082332));
#40440=CARTESIAN_POINT('Ctrl Pts',(0.0595058004750214,1.78326602905287,
11.4090145742024));
#40441=CARTESIAN_POINT('Ctrl Pts',(0.0590969466601207,1.7831894895333,11.4089888512012));
#40442=CARTESIAN_POINT('Ctrl Pts',(0.0573056209852522,1.78285773258151,
11.4088763856765));
#40443=CARTESIAN_POINT('Ctrl Pts',(0.0559216089114385,1.78261076608365,
11.4087901068411));
#40444=CARTESIAN_POINT('Ctrl Pts',(0.0290012912009832,1.77798859707933,
11.4071230451104));
#40445=CARTESIAN_POINT('Ctrl Pts',(0.0030263258399031,1.77669868232371,
11.4057041329939));
#40446=CARTESIAN_POINT('Ctrl Pts',(-0.0464229641918105,1.78020991766549,
11.4029276692986));
#40447=CARTESIAN_POINT('Ctrl Pts',(-0.0697593588392407,1.78447793757808,
11.4015823151899));
#40448=CARTESIAN_POINT('Ctrl Pts',(-0.0935197057024527,1.79159026387387,
11.4000741097969));
#40449=CARTESIAN_POINT('Ctrl Pts',(-0.0946206878970762,1.79192626522192,
11.4000039201711));
#40450=CARTESIAN_POINT('Ctrl Pts',(-0.0962224496205946,1.79242449239783,
11.399901353231));
#40451=CARTESIAN_POINT('Ctrl Pts',(-0.0967246778120061,1.79258206073052,
11.3998691287208));
#40452=CARTESIAN_POINT('Ctrl Pts',(-0.0976045129501196,1.79286046840959,
11.3998125610325));
#40453=CARTESIAN_POINT('Ctrl Pts',(-0.0979822881245507,1.79298077580482,
11.3997882353785));
#40454=CARTESIAN_POINT('Ctrl Pts',(-0.0987147319342856,1.79321552156216,
11.3997409994211));
#40455=CARTESIAN_POINT('Ctrl Pts',(-0.099069426142199,1.79332987867535,
11.3997180918234));
#40456=CARTESIAN_POINT('Ctrl Pts',(-0.100011515011491,1.79363542294212,
11.3996571595791));
#40457=CARTESIAN_POINT('Ctrl Pts',(-0.100598557546721,1.7938276834497,11.399619099606));
#40458=CARTESIAN_POINT('Ctrl Pts',(-0.102685099663265,1.7945176892436,11.3994834942132));
#40459=CARTESIAN_POINT('Ctrl Pts',(-0.104181468755356,1.79502476608227,
11.3993856410926));
#40460=CARTESIAN_POINT('Ctrl Pts',(-0.12899374249744,1.80363685690961,11.3977528514854));
#40461=CARTESIAN_POINT('Ctrl Pts',(-0.15130124512736,1.81438147232735,11.3961246305909));
#40462=CARTESIAN_POINT('Ctrl Pts',(-0.181975728002518,1.83376545720852,
11.393674846602));
#40463=CARTESIAN_POINT('Ctrl Pts',(-0.191449045639193,1.84049419208442,
11.3928860442356));
#40464=CARTESIAN_POINT('Ctrl Pts',(-0.208370023553719,1.85394473579229,
11.3914354188375));
#40465=CARTESIAN_POINT('Ctrl Pts',(-0.215908032359701,1.86053180516414,
11.3907719916862));
#40466=CARTESIAN_POINT('Ctrl Pts',(-0.225865789374535,1.87008649868474,
11.3898841502351));
#40467=CARTESIAN_POINT('Ctrl Pts',(-0.228557198741824,1.87276183652576,
11.3896429557711));
#40468=CARTESIAN_POINT('Ctrl Pts',(-0.231574433270721,1.87586891110053,
11.3893718040988));
#40469=CARTESIAN_POINT('Ctrl Pts',(-0.231947037657232,1.87625453102284,
11.389338305572));
#40470=CARTESIAN_POINT('Ctrl Pts',(-0.232507455706521,1.87683742954081,
11.3892879040854));
#40471=CARTESIAN_POINT('Ctrl Pts',(-0.232695982221152,1.87703401678166,
11.389270945801));
#40472=CARTESIAN_POINT('Ctrl Pts',(-0.233035115930447,1.87738854926842,
11.389240435029));
#40473=CARTESIAN_POINT('Ctrl Pts',(-0.233185811563569,1.87754640812089,
11.3892268756263));
#40474=CARTESIAN_POINT('Ctrl Pts',(-0.233509580011898,1.87788625719874,
11.3891977395314));
#40475=CARTESIAN_POINT('Ctrl Pts',(-0.233682599952229,1.87806829613795,
11.3891821669704));
#40476=CARTESIAN_POINT('Ctrl Pts',(-0.234148642674469,1.87855978148246,
11.3891402139529));
#40477=CARTESIAN_POINT('Ctrl Pts',(-0.234441266027767,1.87886960853007,
11.3891138644934));
#40478=CARTESIAN_POINT('Ctrl Pts',(-0.235791390892575,1.88030480125339,
11.3889922512655));
#40479=CARTESIAN_POINT('Ctrl Pts',(-0.236841432429995,1.88143720243551,
11.3888975533506));
#40480=CARTESIAN_POINT('Ctrl Pts',(-0.259372643302606,1.9060886997761,11.3868619276317));
#40481=CARTESIAN_POINT('Ctrl Pts',(-0.277261718287582,1.9326605253831,11.3851601879815));
#40482=CARTESIAN_POINT('Ctrl Pts',(-0.298528101470506,1.97731458201701,
11.3823575257023));
#40483=CARTESIAN_POINT('Ctrl Pts',(-0.304778660268125,1.99378997435736,
11.3813365373181));
#40484=CARTESIAN_POINT('Ctrl Pts',(-0.30996516036343,2.01177278597578,11.3801982217841));
#40485=CARTESIAN_POINT('Ctrl Pts',(-0.310271334769157,2.01285563297686,
11.3801295974769));
#40486=CARTESIAN_POINT('Ctrl Pts',(-0.310711089494955,2.01444261310416,
11.3800289000181));
#40487=CARTESIAN_POINT('Ctrl Pts',(-0.310849129633137,2.01494551047207,
11.3799969718492));
#40488=CARTESIAN_POINT('Ctrl Pts',(-0.31108976779386,2.0158305958635,11.3799407463367));
#40489=CARTESIAN_POINT('Ctrl Pts',(-0.311192883929079,2.01621264290853,
11.3799164658603));
#40490=CARTESIAN_POINT('Ctrl Pts',(-0.311392120010616,2.01695625736643,
11.3798691851972));
#40491=CARTESIAN_POINT('Ctrl Pts',(-0.311488314563644,2.01731780431216,
11.3798461874716));
#40492=CARTESIAN_POINT('Ctrl Pts',(-0.311743586295423,2.01828401045264,
11.3797847013309));
#40493=CARTESIAN_POINT('Ctrl Pts',(-0.311901533189148,2.01888896419416,
11.3797461763876));
#40494=CARTESIAN_POINT('Ctrl Pts',(-0.312463938284782,2.02106897137341,
11.3796072459193));
#40495=CARTESIAN_POINT('Ctrl Pts',(-0.312858229029909,2.0226466007139,11.3795065125137));
#40496=CARTESIAN_POINT('Ctrl Pts',(-0.319266889452423,2.04913962117935,
11.3778115051525));
#40497=CARTESIAN_POINT('Ctrl Pts',(-0.322298473416595,2.07467656809684,
11.3761160603101));
#40498=CARTESIAN_POINT('Ctrl Pts',(-0.322253346302143,2.12364577356137,
11.3728067123969));
#40499=CARTESIAN_POINT('Ctrl Pts',(-0.319694501316975,2.14692529899204,
11.3712117409314));
#40500=CARTESIAN_POINT('Ctrl Pts',(-0.314359649194358,2.17099921377188,
11.3696549685826));
#40501=CARTESIAN_POINT('Ctrl Pts',(-0.314069674331122,2.17227113670679,
11.3695730133649));
#40502=CARTESIAN_POINT('Ctrl Pts',(-0.313679796577574,2.17393459291369,
11.3694662490481));
#40503=CARTESIAN_POINT('Ctrl Pts',(-0.313586874787494,2.1743277254833,11.3694410476469));
#40504=CARTESIAN_POINT('Ctrl Pts',(-0.313442351362779,2.17493407850222,
11.369402226484));
#40505=CARTESIAN_POINT('Ctrl Pts',(-0.313391271220161,2.17514742093047,
11.3693885767228));
#40506=CARTESIAN_POINT('Ctrl Pts',(-0.313288962954833,2.17557280530305,
11.3693613791507));
#40507=CARTESIAN_POINT('Ctrl Pts',(-0.313237737731742,2.17578484592476,
11.3693478313569));
#40508=CARTESIAN_POINT('Ctrl Pts',(-0.31312238908277,2.17626020276741,11.3693174804528));
#40509=CARTESIAN_POINT('Ctrl Pts',(-0.313058148939225,2.1765234895641,11.3693006842261));
#40510=CARTESIAN_POINT('Ctrl Pts',(-0.312867386664942,2.17730106392869,
11.3692511206979));
#40511=CARTESIAN_POINT('Ctrl Pts',(-0.312739928028976,2.17781512416576,
11.3692184073775));
#40512=CARTESIAN_POINT('Ctrl Pts',(-0.311735517035027,2.18182373706968,
11.3689637117584));
#40513=CARTESIAN_POINT('Ctrl Pts',(-0.310801242347256,2.18530385064392,
11.3687449750859));
#40514=CARTESIAN_POINT('Ctrl Pts',(-0.307295983124388,2.1975375743701,11.367982111548));
#40515=CARTESIAN_POINT('Ctrl Pts',(-0.304411744969148,2.20619754121014,
11.3674531122003));
#40516=CARTESIAN_POINT('Ctrl Pts',(-0.291928334298789,2.23896789179042,
11.3654534256326));
#40517=CARTESIAN_POINT('Ctrl Pts',(-0.279799623035608,2.26200765349055,
11.3640441005038));
#40518=CARTESIAN_POINT('Ctrl Pts',(-0.261908755108897,2.28787033300837,
11.3622303962566));
#40519=CARTESIAN_POINT('Ctrl Pts',(-0.258662816353377,2.29231484830051,
11.3619098155108));
#40520=CARTESIAN_POINT('Ctrl Pts',(-0.254253890372147,2.29803812845045,
11.3614836535988));
#40521=CARTESIAN_POINT('Ctrl Pts',(-0.253192075065908,2.29939386663975,
11.3613816908475));
#40522=CARTESIAN_POINT('Ctrl Pts',(-0.248909954603756,2.30477196992698,
11.3609730305071));
#40523=CARTESIAN_POINT('Ctrl Pts',(-0.245604389998335,2.30872518817796,
11.3606631854897));
#40524=CARTESIAN_POINT('Ctrl Pts',(-0.241634750866392,2.31324767682501,
11.3602967438195));
#40525=CARTESIAN_POINT('Ctrl Pts',(-0.241061270838694,2.31389574137006,
11.3602439384914));
#40526=CARTESIAN_POINT('Ctrl Pts',(-0.240141007125877,2.31492728917213,
11.360159409913));
#40527=CARTESIAN_POINT('Ctrl Pts',(-0.239795895994813,2.3153122643823,11.36012775688));
#40528=CARTESIAN_POINT('Ctrl Pts',(-0.239184544853084,2.31599094025439,
11.3600717655193));
#40529=CARTESIAN_POINT('Ctrl Pts',(-0.23891868589476,2.31628498398328,11.3600474432997));
#40530=CARTESIAN_POINT('Ctrl Pts',(-0.23836726707907,2.31689260357345,11.3599970514745));
#40531=CARTESIAN_POINT('Ctrl Pts',(-0.238081629523655,2.31720610760345,
11.3599709786015));
#40532=CARTESIAN_POINT('Ctrl Pts',(-0.237347416437861,2.31800876134596,
11.3599040369711));
#40533=CARTESIAN_POINT('Ctrl Pts',(-0.23689794883459,2.31849708908991,11.3598631302928));
#40534=CARTESIAN_POINT('Ctrl Pts',(-0.235046242546941,2.32049646033625,
11.3596949006925));
#40535=CARTESIAN_POINT('Ctrl Pts',(-0.233631054122086,2.32199539497185,
11.3595670238161));
#40536=CARTESIAN_POINT('Ctrl Pts',(-0.22413656197855,2.3318603950268,11.3587135207124));
#40537=CARTESIAN_POINT('Ctrl Pts',(-0.215624758982773,2.33979647510923,
11.357968864963));
#40538=CARTESIAN_POINT('Ctrl Pts',(-0.181055528946665,2.36869617858792,
11.3550181370014));
#40539=CARTESIAN_POINT('Ctrl Pts',(-0.152232497679068,2.38601319419522,
11.3526824613742));
#40540=CARTESIAN_POINT('Ctrl Pts',(-0.117208616749167,2.40023739173137,
11.3502400099718));
#40541=CARTESIAN_POINT('Ctrl Pts',(-0.113118033792052,2.40180236311669,
11.3499607862732));
#40542=CARTESIAN_POINT('Ctrl Pts',(-0.108430467011868,2.40348702003269,
11.3496486443292));
#40543=CARTESIAN_POINT('Ctrl Pts',(-0.107863778379305,2.4036888915195,11.3496110379291));
#40544=CARTESIAN_POINT('Ctrl Pts',(-0.107026203868007,2.40398462048627,
11.3495556489169));
#40545=CARTESIAN_POINT('Ctrl Pts',(-0.106755756827718,2.40407970368351,
11.3495377939667));
#40546=CARTESIAN_POINT('Ctrl Pts',(-0.106277095754183,2.40424727303559,
11.3495062458134));
#40547=CARTESIAN_POINT('Ctrl Pts',(-0.106068933964605,2.40431990648054,
11.3494925438038));
#40548=CARTESIAN_POINT('Ctrl Pts',(-0.105633923129305,2.40447119330934,
11.3494639469764));
#40549=CARTESIAN_POINT('Ctrl Pts',(-0.105407061199591,2.40454980663443,
11.3494490545828));
#40550=CARTESIAN_POINT('Ctrl Pts',(-0.104813468497689,2.40475475861509,
11.3494101427263));
#40551=CARTESIAN_POINT('Ctrl Pts',(-0.104446595726837,2.40488068932269,
11.3493861475778));
#40552=CARTESIAN_POINT('Ctrl Pts',(-0.102842839134792,2.40542795133668,
11.3492814889179));
#40553=CARTESIAN_POINT('Ctrl Pts',(-0.101603604243687,2.4058424279928,11.3492012266636));
#40554=CARTESIAN_POINT('Ctrl Pts',(-0.0924298191168617,2.40884879544283,
11.3486113104357));
#40555=CARTESIAN_POINT('Ctrl Pts',(-0.0843990020981954,2.41113933395943,
11.348118284486));
#40556=CARTESIAN_POINT('Ctrl Pts',(-0.0608749879572826,2.41687073066331,
11.3467171688794));
#40557=CARTESIAN_POINT('Ctrl Pts',(-0.0452051845918544,2.41948298976214,
11.3458361389578));
#40558=CARTESIAN_POINT('Ctrl Pts',(-0.00452228508986718,2.42321063729027,
11.3435515659846));
#40559=CARTESIAN_POINT('Ctrl Pts',(0.02053775698261,2.42258876656911,11.3421403900052));
#40560=CARTESIAN_POINT('Ctrl Pts',(0.0467323080080221,2.41887213776658,
11.3405353959467));
#40561=CARTESIAN_POINT('Ctrl Pts',(0.0481904201930731,2.41865503627687,
11.340445654233));
#40562=CARTESIAN_POINT('Ctrl Pts',(0.050180546179098,2.41834475028077,11.3403226053533));
#40563=CARTESIAN_POINT('Ctrl Pts',(0.0507139069303691,2.41826021882167,
11.3402895724247));
#40564=CARTESIAN_POINT('Ctrl Pts',(0.0516213770467913,2.418114056295,11.3402332743332));
#40565=CARTESIAN_POINT('Ctrl Pts',(0.0519955959776072,2.41805310465016,
11.3402100307555));
#40566=CARTESIAN_POINT('Ctrl Pts',(0.0527192841295516,2.41793392116256,
11.340165027124));
#40567=CARTESIAN_POINT('Ctrl Pts',(0.0530687667862062,2.41787577311767,
11.3401432697593));
#40568=CARTESIAN_POINT('Ctrl Pts',(0.053898022902754,2.41773639315297,11.3400915857229));
#40569=CARTESIAN_POINT('Ctrl Pts',(0.0543777086429537,2.4176546508479,11.3400616428753));
#40570=CARTESIAN_POINT('Ctrl Pts',(0.0557929840800038,2.41741017684335,
11.339973161816));
#40571=CARTESIAN_POINT('Ctrl Pts',(0.0567280356482728,2.41724439691957,
11.3399145267954));
#40572=CARTESIAN_POINT('Ctrl Pts',(0.0640509930196899,2.41591266314197,
11.3394539141401));
#40573=CARTESIAN_POINT('Ctrl Pts',(0.0704026703108798,2.41455809409364,
11.3390459532616));
#40574=CARTESIAN_POINT('Ctrl Pts',(0.0829432737469404,2.41148481926685,
11.3382227377634));
#40575=CARTESIAN_POINT('Ctrl Pts',(0.0891303931241315,2.40977111455441,
11.3378078056179));
#40576=CARTESIAN_POINT('Ctrl Pts',(0.12618682374267,2.39830516734182,11.3352699337926));
#40577=CARTESIAN_POINT('Ctrl Pts',(0.155488028036088,2.38413396138863,11.3330145199447));
#40578=CARTESIAN_POINT('Ctrl Pts',(0.18246282617565,2.36564752262211,11.3308858038243));
#40579=CARTESIAN_POINT('Ctrl Pts',(0.182740533754245,2.3654565624283,11.3308638849336));
#40580=CARTESIAN_POINT('Ctrl Pts',(0.183379332606582,2.36501582739628,11.3308134584491));
#40581=CARTESIAN_POINT('Ctrl Pts',(0.183740214838645,2.36476574901755,11.3307849651146));
#40582=CARTESIAN_POINT('Ctrl Pts',(0.18811028475716,2.36172421019724,11.3304398719187));
#40583=CARTESIAN_POINT('Ctrl Pts',(0.192056286464393,2.35884248242849,11.3301276894277));
#40584=CARTESIAN_POINT('Ctrl Pts',(0.196384680129769,2.35552798891617,11.3297859787899));
#40585=CARTESIAN_POINT('Ctrl Pts',(0.196832965692875,2.35518283511489,11.3297505972382));
#40586=CARTESIAN_POINT('Ctrl Pts',(0.197504640355259,2.35466286168595,11.3296976007998));
#40587=CARTESIAN_POINT('Ctrl Pts',(0.197728708399935,2.35448892698888,11.3296799241469));
#40588=CARTESIAN_POINT('Ctrl Pts',(0.198115442409466,2.35418790237786,11.3296494200222));
#40589=CARTESIAN_POINT('Ctrl Pts',(0.198278215942483,2.35406095197721,11.3296365826508));
#40590=CARTESIAN_POINT('Ctrl Pts',(0.19861284832173,2.35379944788421,11.3296101948599));
#40591=CARTESIAN_POINT('Ctrl Pts',(0.198784692216103,2.35366487617642,11.3295966458465));
#40592=CARTESIAN_POINT('Ctrl Pts',(0.199189694368833,2.35334705292501,11.3295647177061));
#40593=CARTESIAN_POINT('Ctrl Pts',(0.199422737410001,2.3531636533433,11.3295463491652));
#40594=CARTESIAN_POINT('Ctrl Pts',(0.19991584763242,2.35277448341472,11.3295074882116));
#40595=CARTESIAN_POINT('Ctrl Pts',(0.200175851280654,2.35256863258638,11.3294870015374));
#40596=CARTESIAN_POINT('Ctrl Pts',(0.200878252913607,2.35201075922419,11.3294316651193));
#40597=CARTESIAN_POINT('Ctrl Pts',(0.201320045589448,2.35165797128934,11.3293968690411));
#40598=CARTESIAN_POINT('Ctrl Pts',(0.213573677646391,2.34182007065545,11.3284319410117));
#40599=CARTESIAN_POINT('Ctrl Pts',(0.224704873299075,2.33151353625263,11.327559757136));
#40600=CARTESIAN_POINT('Ctrl Pts',(0.255400806295196,2.29878333129684,11.3250249098442));
#40601=CARTESIAN_POINT('Ctrl Pts',(0.272633249537323,2.27440028916025,11.3234068039666));
#40602=CARTESIAN_POINT('Ctrl Pts',(0.288898485470596,2.24293818888046,11.3213070850102));
#40603=CARTESIAN_POINT('Ctrl Pts',(0.291381042673278,2.23780690307811,11.3209649033049));
#40604=CARTESIAN_POINT('Ctrl Pts',(0.294129493499249,2.23171931354814,11.320558263061));
#40605=CARTESIAN_POINT('Ctrl Pts',(0.29452877257205,2.23082407500769,11.3204984463579));
#40606=CARTESIAN_POINT('Ctrl Pts',(0.295125393567224,2.22946979317445,11.3204079282924));
#40607=CARTESIAN_POINT('Ctrl Pts',(0.2953257649204,2.22901208409517,11.3203773306423));
#40608=CARTESIAN_POINT('Ctrl Pts',(0.295681751970442,2.22819372629069,11.3203226139489));
#40609=CARTESIAN_POINT('Ctrl Pts',(0.295837774596875,2.22783325478138,11.3202985088563));
#40610=CARTESIAN_POINT('Ctrl Pts',(0.296165862624206,2.22707142925538,11.320247557236));
#40611=CARTESIAN_POINT('Ctrl Pts',(0.296337771929277,2.22667000924429,11.320220705448));
#40612=CARTESIAN_POINT('Ctrl Pts',(0.296790962609327,2.22560580615584,11.3201495063654));
#40613=CARTESIAN_POINT('Ctrl Pts',(0.297070838473189,2.22494243051109,11.3201051113781));
#40614=CARTESIAN_POINT('Ctrl Pts',(0.29834088854247,2.22190370216548,11.3199016879763));
#40615=CARTESIAN_POINT('Ctrl Pts',(0.299304789493341,2.21951753321753,11.3197417723334));
#40616=CARTESIAN_POINT('Ctrl Pts',(0.303269873599306,2.20935295435963,11.3190596490866));
#40617=CARTESIAN_POINT('Ctrl Pts',(0.305996968363029,2.20147176797048,11.3185283850568));
#40618=CARTESIAN_POINT('Ctrl Pts',(0.312511922447542,2.17998048936091,11.3170724314153));
#40619=CARTESIAN_POINT('Ctrl Pts',(0.315715518841181,2.16621342556584,11.3161314727547));
#40620=CARTESIAN_POINT('Ctrl Pts',(0.321555727886701,2.13069027157465,11.3137039684498));
#40621=CARTESIAN_POINT('Ctrl Pts',(0.32289747059995,2.10879225398944,11.3122056014617));
#40622=CARTESIAN_POINT('Ctrl Pts',(0.321981298021614,2.08622647382615,11.3107459870959));
#40623=CARTESIAN_POINT('Ctrl Pts',(0.321950599739869,2.08552665748753,11.3107008095637));
#40624=CARTESIAN_POINT('Ctrl Pts',(0.321740343714891,2.08106578262378,11.3104134188027));
#40625=CARTESIAN_POINT('Ctrl Pts',(0.321497155651959,2.07730781352421,11.3101739698107));
#40626=CARTESIAN_POINT('Ctrl Pts',(0.321140290116267,2.07297353486125,11.3099015304684));
#40627=CARTESIAN_POINT('Ctrl Pts',(0.32109085533509,2.07239242157138,11.3098650811168));
#40628=CARTESIAN_POINT('Ctrl Pts',(0.321015188402491,2.07153064997296,11.3098111463397));
#40629=CARTESIAN_POINT('Ctrl Pts',(0.320990165425847,2.07124989082816,11.3097935934159));
#40630=CARTESIAN_POINT('Ctrl Pts',(0.320945481107521,2.07075586124075,11.3097627401829));
#40631=CARTESIAN_POINT('Ctrl Pts',(0.320925975516493,2.07054257759177,11.3097494310759));
#40632=CARTESIAN_POINT('Ctrl Pts',(0.320885628894405,2.07010620471909,11.3097222234596));
#40633=CARTESIAN_POINT('Ctrl Pts',(0.320864767894126,2.06988311848417,11.309708326134));
#40634=CARTESIAN_POINT('Ctrl Pts',(0.320808399800986,2.0692870282428,11.3096712238331));
#40635=CARTESIAN_POINT('Ctrl Pts',(0.320772474693204,2.06891406267128,11.3096480424899));
#40636=CARTESIAN_POINT('Ctrl Pts',(0.320692650090385,2.06810021783746,11.3095975292078));
#40637=CARTESIAN_POINT('Ctrl Pts',(0.320648491632602,2.06765936390213,11.3095702117091));
#40638=CARTESIAN_POINT('Ctrl Pts',(0.320517087765459,2.06637422876746,11.3094907064822));
#40639=CARTESIAN_POINT('Ctrl Pts',(0.320427415167719,2.06553019166484,11.3094386512038));
#40640=CARTESIAN_POINT('Ctrl Pts',(0.317235386036507,2.03657477832187,11.3076580867215));
#40641=CARTESIAN_POINT('Ctrl Pts',(0.310448791682766,2.00898789033902,11.3061237860713));
#40642=CARTESIAN_POINT('Ctrl Pts',(0.292419750605674,1.96287986451402,11.3033424926663));
#40643=CARTESIAN_POINT('Ctrl Pts',(0.282763374647675,1.94393618872499,11.3021272706346));
#40644=CARTESIAN_POINT('Ctrl Pts',(0.27061562193278,1.92498557071362,11.3007601152078));
#40645=CARTESIAN_POINT('Ctrl Pts',(0.269907521962876,1.92389550033283,11.3006809240588));
#40646=CARTESIAN_POINT('Ctrl Pts',(0.26891144580463,1.92238223087507,11.300570207493));
#40647=CARTESIAN_POINT('Ctrl Pts',(0.268629020101468,1.92195537877203,11.3005388901509));
#40648=CARTESIAN_POINT('Ctrl Pts',(0.268139806322849,1.92121980545952,11.3004847709626));
#40649=CARTESIAN_POINT('Ctrl Pts',(0.267933498366403,1.92091076485157,11.3004619872092));
#40650=CARTESIAN_POINT('Ctrl Pts',(0.267505610792991,1.92027220164292,11.3004148133478));
#40651=CARTESIAN_POINT('Ctrl Pts',(0.267283955767604,1.91994273051322,11.3003904204184));
#40652=CARTESIAN_POINT('Ctrl Pts',(0.26676488889663,1.91917425277872,11.3003333999611));
#40653=CARTESIAN_POINT('Ctrl Pts',(0.266467002007438,1.91873556983795,11.300300754486));
#40654=CARTESIAN_POINT('Ctrl Pts',(0.265507225842488,1.91732963478781,11.3001958203587));
#40655=CARTESIAN_POINT('Ctrl Pts',(0.264841147969225,1.91636526585228,11.3001233726792));
#40656=CARTESIAN_POINT('Ctrl Pts',(0.254625774337976,1.90174630475253,11.2990178787223));
#40657=CARTESIAN_POINT('Ctrl Pts',(0.244038487195102,1.88885107144398,11.2979439910343));
#40658=CARTESIAN_POINT('Ctrl Pts',(0.229809403740695,1.87402666052507,11.2965813541071));
#40659=CARTESIAN_POINT('Ctrl Pts',(0.227064745038438,1.87126890808962,11.2963218932464));
#40660=CARTESIAN_POINT('Ctrl Pts',(0.203516933220354,1.84845035945618,11.2941254875298));
#40661=CARTESIAN_POINT('Ctrl Pts',(0.180152157028259,1.83122188011563,11.2921222987019));
#40662=CARTESIAN_POINT('Ctrl Pts',(0.153511652218545,1.81663183568528,11.2902016840408));
#40663=CARTESIAN_POINT('Ctrl Pts',(0.152215280648293,1.81593336618361,11.2901090847738));
#40664=CARTESIAN_POINT('Ctrl Pts',(0.150539974389725,1.81504549300565,11.2899905675948));
#40665=CARTESIAN_POINT('Ctrl Pts',(0.150165417586754,1.81484793125153,11.2899641436437));
#40666=CARTESIAN_POINT('Ctrl Pts',(0.149570832201879,1.81453581080391,11.2899223151025));
#40667=CARTESIAN_POINT('Ctrl Pts',(0.14935106053848,1.81442076777894,11.289906879834));
#40668=CARTESIAN_POINT('Ctrl Pts',(0.148941164310051,1.81420680356039,11.2898781392636));
#40669=CARTESIAN_POINT('Ctrl Pts',(0.148751075399112,1.81410781905559,11.2898648300061));
#40670=CARTESIAN_POINT('Ctrl Pts',(0.148322240818617,1.8138850566243,11.2898348477393));
#40671=CARTESIAN_POINT('Ctrl Pts',(0.148083439378098,1.813761388126,11.2898181817485));
#40672=CARTESIAN_POINT('Ctrl Pts',(0.147583922668493,1.81350349499057,11.2897833824373));
#40673=CARTESIAN_POINT('Ctrl Pts',(0.147323178253634,1.81336932689661,11.2897652526915));
#40674=CARTESIAN_POINT('Ctrl Pts',(0.146641821407566,1.81301990472017,11.2897179685363));
#40675=CARTESIAN_POINT('Ctrl Pts',(0.146220916192554,1.8128052184545,11.289688849441));
#40676=CARTESIAN_POINT('Ctrl Pts',(0.144972528190746,1.81217192345535,11.2896027466521));
#40677=CARTESIAN_POINT('Ctrl Pts',(0.144143700632759,1.81175595549363,11.2895459233637));
#40678=CARTESIAN_POINT('Ctrl Pts',(0.141232883023147,1.81031078338081,11.2893475171262));
#40679=CARTESIAN_POINT('Ctrl Pts',(0.139141518589621,1.80930048509612,11.2892070296331));
#40680=CARTESIAN_POINT('Ctrl Pts',(0.132667334532932,1.80625880850857,11.2887778936299));
#40681=CARTESIAN_POINT('Ctrl Pts',(0.128249455929038,1.80430321065738,11.2884931142327));
#40682=CARTESIAN_POINT('Ctrl Pts',(0.116223922539828,1.7993002958613,11.2877351292652));
#40683=CARTESIAN_POINT('Ctrl Pts',(0.108541091946679,1.79644249644365,11.2872689956764));
#40684=CARTESIAN_POINT('Ctrl Pts',(0.077182039404477,1.78612086063972,11.2854084415905));
#40685=CARTESIAN_POINT('Ctrl Pts',(0.0527907366784927,1.7811108512324,11.2840486745648));
#40686=CARTESIAN_POINT('Ctrl Pts',(0.0186781773322447,1.77812873778148,
11.2820530226371));
#40687=CARTESIAN_POINT('Ctrl Pts',(0.00925949832198398,1.77772027806431,
11.2814933064693));
#40688=CARTESIAN_POINT('Ctrl Pts',(-0.00130767159243636,1.77772561986267,
11.2808506894171));
#40689=CARTESIAN_POINT('Ctrl Pts',(-0.00245240735778875,1.77773229801436,
11.2807808852584));
#40690=CARTESIAN_POINT('Ctrl Pts',(-0.00411653486913456,1.77775087332754,
11.2806791256132));
#40691=CARTESIAN_POINT('Ctrl Pts',(-0.0046359807307583,1.77775792767212,
11.2806473218467));
#40692=CARTESIAN_POINT('Ctrl Pts',(-0.00555217478502938,1.77777258582359,
11.2805911549076));
#40693=CARTESIAN_POINT('Ctrl Pts',(-0.00594893121706805,1.77777966652181,
11.2805668081702));
#40694=CARTESIAN_POINT('Ctrl Pts',(-0.0067686959336765,1.77779581101593,
11.2805164543174));
#40695=CARTESIAN_POINT('Ctrl Pts',(-0.00719170127821379,1.77780497509501,
11.2804904441068));
#40696=CARTESIAN_POINT('Ctrl Pts',(-0.00827362898359217,1.77783054592782,
11.2804238471732));
#40697=CARTESIAN_POINT('Ctrl Pts',(-0.00893251893961792,1.77784814113712,
11.2803832232845));
#40698=CARTESIAN_POINT('Ctrl Pts',(-0.0116146488198333,1.77792800037926,
11.2802175819054));
#40699=CARTESIAN_POINT('Ctrl Pts',(-0.0136373005621482,1.77800730328181,
11.2800920316862));
#40700=CARTESIAN_POINT('Ctrl Pts',(-0.0466842568565628,1.77961492217671,
11.2780299958882));
#40701=CARTESIAN_POINT('Ctrl Pts',(-0.0773217963492715,1.78560148169534,
11.2759393477898));
#40702=CARTESIAN_POINT('Ctrl Pts',(-0.111101254718751,1.79744383609631,
11.2735195361634));
#40703=CARTESIAN_POINT('Ctrl Pts',(-0.115546893373469,1.79911357955727,
11.2731991765968));
#40704=CARTESIAN_POINT('Ctrl Pts',(-0.127451296333696,1.80388753756222,
11.2723384685707));
#40705=CARTESIAN_POINT('Ctrl Pts',(-0.134833341961031,1.80717511998225,
11.271801601766));
#40706=CARTESIAN_POINT('Ctrl Pts',(-0.1470422208551,1.81317205438604,11.2709166706874));
#40707=CARTESIAN_POINT('Ctrl Pts',(-0.151936917833623,1.81573451278306,
11.2705627521864));
#40708=CARTESIAN_POINT('Ctrl Pts',(-0.157274657684916,1.81870620391343,
11.2701797304175));
#40709=CARTESIAN_POINT('Ctrl Pts',(-0.15778487669942,1.8189920813138,11.2701431487217));
#40710=CARTESIAN_POINT('Ctrl Pts',(-0.158545568256638,1.81942102429236,
11.270088657122));
#40711=CARTESIAN_POINT('Ctrl Pts',(-0.158796628013536,1.81956303782116,
11.2700706805443));
#40712=CARTESIAN_POINT('Ctrl Pts',(-0.159228129668902,1.8198078846927,11.2700397978916));
#40713=CARTESIAN_POINT('Ctrl Pts',(-0.159408662858292,1.81991055542109,
11.2700268813413));
#40714=CARTESIAN_POINT('Ctrl Pts',(-0.159778028335868,1.82012108943712,
11.2700004633603));
#40715=CARTESIAN_POINT('Ctrl Pts',(-0.159966850332798,1.82022896913444,
11.2699869631153));
#40716=CARTESIAN_POINT('Ctrl Pts',(-0.16041277516867,1.82048433846677,11.2699550917747));
#40717=CARTESIAN_POINT('Ctrl Pts',(-0.160669784799948,1.8206319922867,11.269936731338));
#40718=CARTESIAN_POINT('Ctrl Pts',(-0.161210346190913,1.82094354125368,
11.2698981318075));
#40719=CARTESIAN_POINT('Ctrl Pts',(-0.161493852808435,1.8211075146327,11.2698778977728));
#40720=CARTESIAN_POINT('Ctrl Pts',(-0.162257378338485,1.8215506739812,11.2698234305137));
#40721=CARTESIAN_POINT('Ctrl Pts',(-0.162736929102377,1.82183067044949,
11.2697892487911));
#40722=CARTESIAN_POINT('Ctrl Pts',(-0.164212992263351,1.82269762651548,
11.2696841151418));
#40723=CARTESIAN_POINT('Ctrl Pts',(-0.165207083623808,1.82328871945569,
11.2696134203523));
#40724=CARTESIAN_POINT('Ctrl Pts',(-0.1688890343888,1.82550494518646,11.2693519060697));
#40725=CARTESIAN_POINT('Ctrl Pts',(-0.171556367827907,1.82716405051337,
11.2691631080574));
#40726=CARTESIAN_POINT('Ctrl Pts',(-0.18077973775653,1.83308982525626,11.268511008555));
#40727=CARTESIAN_POINT('Ctrl Pts',(-0.187204730967481,1.83755617556832,
11.2680580651307));
#40728=CARTESIAN_POINT('Ctrl Pts',(-0.216191211510735,1.85931294985773,
11.2659899158481));
#40729=CARTESIAN_POINT('Ctrl Pts',(-0.236564245898053,1.87930483769415,
11.2644522131718));
#40730=CARTESIAN_POINT('Ctrl Pts',(-0.260074077646783,1.90942600154758,
11.2622288005819));
#40731=CARTESIAN_POINT('Ctrl Pts',(-0.265741114708693,1.91741137636493,
11.2616480809618));
#40732=CARTESIAN_POINT('Ctrl Pts',(-0.271598532797114,1.92651658605029,
11.2609897426253));
#40733=CARTESIAN_POINT('Ctrl Pts',(-0.272157136290327,1.9273942322524,11.2609263262336));
#40734=CARTESIAN_POINT('Ctrl Pts',(-0.272986333648588,1.92871105307256,
11.2608312304881));
#40735=CARTESIAN_POINT('Ctrl Pts',(-0.273260142264864,1.9291482035713,11.2607996700504));
#40736=CARTESIAN_POINT('Ctrl Pts',(-0.273729938942078,1.92990227807647,
11.2607452435183));
#40737=CARTESIAN_POINT('Ctrl Pts',(-0.273926429608413,1.93021888904562,
11.260722396001));
#40738=CARTESIAN_POINT('Ctrl Pts',(-0.274330862200261,1.93087309238842,
11.2606751955851));
#40739=CARTESIAN_POINT('Ctrl Pts',(-0.274538731037759,1.9312107290383,11.2606508400483));
#40740=CARTESIAN_POINT('Ctrl Pts',(-0.275021188533818,1.93199762289192,
11.2605940878111));
#40741=CARTESIAN_POINT('Ctrl Pts',(-0.275295299750861,1.93244717016309,
11.2605616736701));
#40742=CARTESIAN_POINT('Ctrl Pts',(-0.276165615009344,1.93388240384989,
11.2604582118271));
#40743=CARTESIAN_POINT('Ctrl Pts',(-0.276757631206685,1.9348706077713,11.26038701131));
#40744=CARTESIAN_POINT('Ctrl Pts',(-0.289584037343805,1.95654340768279,
11.2588261757985));
#40745=CARTESIAN_POINT('Ctrl Pts',(-0.299469411161466,1.97852439614754,
11.2572482081739));
#40746=CARTESIAN_POINT('Ctrl Pts',(-0.313383815465663,2.02182035364275,
11.2541829465012));
#40747=CARTESIAN_POINT('Ctrl Pts',(-0.317892374598418,2.04285112077207,
11.2527138231252));
#40748=CARTESIAN_POINT('Ctrl Pts',(-0.320430100751893,2.06553829594953,
11.2512321995997));
#40749=CARTESIAN_POINT('Ctrl Pts',(-0.320573929873987,2.06690295894055,
11.251143486109));
#40750=CARTESIAN_POINT('Ctrl Pts',(-0.321084753464039,2.0720658367076,11.2508095024859));
#40751=CARTESIAN_POINT('Ctrl Pts',(-0.321393014763523,2.0758697363302,11.2505667861608));
#40752=CARTESIAN_POINT('Ctrl Pts',(-0.321670576091457,2.08026275306692,
11.2502910292397));
#40753=CARTESIAN_POINT('Ctrl Pts',(-0.321705903848731,2.08084719651897,
11.2502544355313));
#40754=CARTESIAN_POINT('Ctrl Pts',(-0.321755905452735,2.0817135941602,11.2502003285863));
#40755=CARTESIAN_POINT('Ctrl Pts',(-0.321771801624668,2.08199547243258,
11.250182747227));
#40756=CARTESIAN_POINT('Ctrl Pts',(-0.32179894351493,2.08248828402835,11.250152048515));
#40757=CARTESIAN_POINT('Ctrl Pts',(-0.321810352264769,2.0826992075374,11.2501389219625));
#40758=CARTESIAN_POINT('Ctrl Pts',(-0.321832392049017,2.08311424190376,
11.2501131175547));
#40759=CARTESIAN_POINT('Ctrl Pts',(-0.321843036248721,2.0833183508837,11.2501004389825));
#40760=CARTESIAN_POINT('Ctrl Pts',(-0.321865672053124,2.08376049317069,
11.2500729997118));
#40761=CARTESIAN_POINT('Ctrl Pts',(-0.321877593802975,2.08399853016888,
11.2500582429597));
#40762=CARTESIAN_POINT('Ctrl Pts',(-0.321905926134909,2.08457707681381,
11.2500224146935));
#40763=CARTESIAN_POINT('Ctrl Pts',(-0.321922060554809,2.08491760062065,
11.2500013586024));
#40764=CARTESIAN_POINT('Ctrl Pts',(-0.321964557838471,2.08584567117974,
11.2499440572337));
#40765=CARTESIAN_POINT('Ctrl Pts',(-0.321989852871072,2.08643326903229,
11.2499078706804));
#40766=CARTESIAN_POINT('Ctrl Pts',(-0.322186188854554,2.09130441040243,
11.2496086350079));
#40767=CARTESIAN_POINT('Ctrl Pts',(-0.322273360650711,2.09559111682564,
11.249350095042));
#40768=CARTESIAN_POINT('Ctrl Pts',(-0.322274977094782,2.09987849461815,
11.2490951747016));
#40769=CARTESIAN_POINT('',(-0.32227491802331,2.10022986532739,10.9995935809957));
#40770=CARTESIAN_POINT('Ctrl Pts',(-0.322274976960673,2.09987813943263,
11.2490951958204));
#40771=CARTESIAN_POINT('Ctrl Pts',(-0.322285613871733,2.12800873443155,
11.2474225961834));
#40772=CARTESIAN_POINT('Ctrl Pts',(-0.318613164737115,2.15602501186304,
11.245905465835));
#40773=CARTESIAN_POINT('Ctrl Pts',(-0.308097884298559,2.19536871258844,
11.243599559658));
#40774=CARTESIAN_POINT('Ctrl Pts',(-0.304140198034284,2.20732283407027,
11.2428754933141));
#40775=CARTESIAN_POINT('Ctrl Pts',(-0.297415342162845,2.22424563838345,
11.2417949778934));
#40776=CARTESIAN_POINT('Ctrl Pts',(-0.295199879667812,2.22942136407662,
11.2414567578009));
#40777=CARTESIAN_POINT('Ctrl Pts',(-0.292467475953579,2.23536909277436,
11.2410580357785));
#40778=CARTESIAN_POINT('Ctrl Pts',(-0.292081288333471,2.23620035516626,
11.2410020785454));
#40779=CARTESIAN_POINT('Ctrl Pts',(-0.291487600522268,2.23746412066347,
11.2409166497411));
#40780=CARTESIAN_POINT('Ctrl Pts',(-0.291282669932361,2.23789783145908,
11.2408872671398));
#40781=CARTESIAN_POINT('Ctrl Pts',(-0.290925065218167,2.23865030462103,
11.240836176833));
#40782=CARTESIAN_POINT('Ctrl Pts',(-0.290772833214783,2.23896927720312,
11.240814484499));
#40783=CARTESIAN_POINT('Ctrl Pts',(-0.290454859202993,2.23963272009415,
11.2407692921755));
#40784=CARTESIAN_POINT('Ctrl Pts',(-0.290289028477201,2.23997714706095,
11.2407457891262));
#40785=CARTESIAN_POINT('Ctrl Pts',(-0.289882535188768,2.24081759611114,
11.2406883368147));
#40786=CARTESIAN_POINT('Ctrl Pts',(-0.289641212488931,2.24131329592043,
11.24065436459));
#40787=CARTESIAN_POINT('Ctrl Pts',(-0.288717148140621,2.24319910099912,
11.2405247907533));
#40788=CARTESIAN_POINT('Ctrl Pts',(-0.288025669814612,2.24458488009068,
11.240428884289));
#40789=CARTESIAN_POINT('Ctrl Pts',(-0.287063662926605,2.24647853101494,
11.2402968671713));
#40790=CARTESIAN_POINT('Ctrl Pts',(-0.286801714679353,2.24699075845509,
11.2402610597552));
#40791=CARTESIAN_POINT('Ctrl Pts',(-0.270637040716542,2.27839230563341,
11.238059927211));
#40792=CARTESIAN_POINT('Ctrl Pts',(-0.249847768579935,2.30650188632565,
11.2356952319962));
#40793=CARTESIAN_POINT('Ctrl Pts',(-0.218019421384603,2.33753606109702,
11.2327050717952));
#40794=CARTESIAN_POINT('Ctrl Pts',(-0.210748303738176,2.34401030651234,
11.2320569718964));
#40795=CARTESIAN_POINT('Ctrl Pts',(-0.200532469710946,2.3523086792004,11.2312033860424));
#40796=CARTESIAN_POINT('Ctrl Pts',(-0.197835609615366,2.35442880086486,
11.2309831051006));
#40797=CARTESIAN_POINT('Ctrl Pts',(-0.194123838752605,2.35725207755928,
11.2306872882039));
#40798=CARTESIAN_POINT('Ctrl Pts',(-0.193138086907931,2.35799297602575,
11.230609418173));
#40799=CARTESIAN_POINT('Ctrl Pts',(-0.191680793684819,2.35907525501481,
11.2304953416608));
#40800=CARTESIAN_POINT('Ctrl Pts',(-0.191212554997324,2.35942103471458,
11.2304588452868));
#40801=CARTESIAN_POINT('Ctrl Pts',(-0.190470584742774,2.35996585643628,
11.2304012647322));
#40802=CARTESIAN_POINT('Ctrl Pts',(-0.190197474824839,2.36016573705552,
11.2303801237182));
#40803=CARTESIAN_POINT('Ctrl Pts',(-0.189680464266221,2.36054287172317,
11.230340204892));
#40804=CARTESIAN_POINT('Ctrl Pts',(-0.189436629036298,2.36072021423578,
11.230321420994));
#40805=CARTESIAN_POINT('Ctrl Pts',(-0.18901509188959,2.36102589662939,11.2302890222007));
#40806=CARTESIAN_POINT('Ctrl Pts',(-0.188837507538888,2.36115439766695,
11.2302753960522));
#40807=CARTESIAN_POINT('Ctrl Pts',(-0.188493372383148,2.36140288125228,
11.2302490345981));
#40808=CARTESIAN_POINT('Ctrl Pts',(-0.188326838302245,2.36152288568124,
11.2302362977434));
#40809=CARTESIAN_POINT('Ctrl Pts',(-0.187933542788105,2.36180572387793,
11.2302062645911));
#40810=CARTESIAN_POINT('Ctrl Pts',(-0.187706683766943,2.36196842258318,
11.2301889777015));
#40811=CARTESIAN_POINT('Ctrl Pts',(-0.186919367530656,2.36253152210366,
11.2301291094583));
#40812=CARTESIAN_POINT('Ctrl Pts',(-0.186357833207874,2.36293042440687,
11.230086630991));
#40813=CARTESIAN_POINT('Ctrl Pts',(-0.179585403879764,2.36770882202297,
11.2295769141881));
#40814=CARTESIAN_POINT('Ctrl Pts',(-0.173222161193793,2.37186951886729,
11.2291242070256));
#40815=CARTESIAN_POINT('Ctrl Pts',(-0.159017811271356,2.38045579372389,
11.2281558457846));
#40816=CARTESIAN_POINT('Ctrl Pts',(-0.151126467388971,2.3847857556229,11.2276442947439));
#40817=CARTESIAN_POINT('Ctrl Pts',(-0.133822548380917,2.39335824994293,
11.2265568819979));
#40818=CARTESIAN_POINT('Ctrl Pts',(-0.124366724062661,2.39749026890407,
11.2259831164714));
#40819=CARTESIAN_POINT('Ctrl Pts',(-0.0927006455418031,2.40955360643537,
11.2240850941368));
#40820=CARTESIAN_POINT('Ctrl Pts',(-0.0698220287320776,2.41550195275426,
11.2227440935401));
#40821=CARTESIAN_POINT('Ctrl Pts',(-0.0453623845872847,2.41906857302622,
11.2212409750878));
#40822=CARTESIAN_POINT('Ctrl Pts',(-0.044222644669577,2.41922853549308,
11.2211707976746));
#40823=CARTESIAN_POINT('Ctrl Pts',(-0.0425604781814816,2.41945274821947,
11.2210682453056));
#40824=CARTESIAN_POINT('Ctrl Pts',(-0.042038703434711,2.4195218303283,11.2210360230923));
#40825=CARTESIAN_POINT('Ctrl Pts',(-0.0411236032885894,2.4196407077668,
11.2209794580633));
#40826=CARTESIAN_POINT('Ctrl Pts',(-0.0407303498345634,2.41969105619203,
11.2209551327666));
#40827=CARTESIAN_POINT('Ctrl Pts',(-0.0399672512741995,2.41978732517869,
11.2209078964919));
#40828=CARTESIAN_POINT('Ctrl Pts',(-0.039597417263531,2.41983333013243,
11.2208849882177));
#40829=CARTESIAN_POINT('Ctrl Pts',(-0.0387153032508349,2.41994150592843,
11.2208303113702));
#40830=CARTESIAN_POINT('Ctrl Pts',(-0.0382029532823698,2.42000308791809,
11.220798524267));
#40831=CARTESIAN_POINT('Ctrl Pts',(-0.0366564009198007,2.42018520890683,
11.2207024826953));
#40832=CARTESIAN_POINT('Ctrl Pts',(-0.0356217676849437,2.42030196589673,
11.2206381091554));
#40833=CARTESIAN_POINT('Ctrl Pts',(-0.0248233406750721,2.4214675865628,
11.2199649375776));
#40834=CARTESIAN_POINT('Ctrl Pts',(-0.0150179880984472,2.42207457782395,
11.2193422854927));
#40835=CARTESIAN_POINT('Ctrl Pts',(0.010961889585408,2.42249390725853,11.2176601383133));
#40836=CARTESIAN_POINT('Ctrl Pts',(0.0271197255087503,2.42153832634082,
11.216579705673));
#40837=CARTESIAN_POINT('Ctrl Pts',(0.0585276572852727,2.41729625747436,
11.214438504025));
#40838=CARTESIAN_POINT('Ctrl Pts',(0.0737493797053583,2.41410740569524,
11.2133816388565));
#40839=CARTESIAN_POINT('Ctrl Pts',(0.0946027756135815,2.40813863009649,
11.2119469449604));
#40840=CARTESIAN_POINT('Ctrl Pts',(0.100473973942773,2.40627453598039,11.2115446908144));
#40841=CARTESIAN_POINT('Ctrl Pts',(0.108216262023889,2.4035697383151,11.2110196280893));
#40842=CARTESIAN_POINT('Ctrl Pts',(0.110137620995487,2.40287794623495,11.2108897771829));
#40843=CARTESIAN_POINT('Ctrl Pts',(0.112843366527661,2.40187457998704,11.2107076830228));
#40844=CARTESIAN_POINT('Ctrl Pts',(0.113633258633955,2.40157813246455,11.2106546171051));
#40845=CARTESIAN_POINT('Ctrl Pts',(0.114834374047575,2.40112196325454,11.2105740765876));
#40846=CARTESIAN_POINT('Ctrl Pts',(0.115246441315336,2.40096449622298,11.2105464728183));
#40847=CARTESIAN_POINT('Ctrl Pts',(0.116006850408579,2.40067212345244,11.2104955863505));
#40848=CARTESIAN_POINT('Ctrl Pts',(0.116355282739889,2.40053745747411,11.210472289592));
#40849=CARTESIAN_POINT('Ctrl Pts',(0.116922409217856,2.40031713406066,11.2104344045713));
#40850=CARTESIAN_POINT('Ctrl Pts',(0.11714124400075,2.40023184331866,11.2104197942876));
#40851=CARTESIAN_POINT('Ctrl Pts',(0.117560109263007,2.40006806312464,11.2103918452568));
#40852=CARTESIAN_POINT('Ctrl Pts',(0.117760153850822,2.39998961309109,11.2103785042327));
#40853=CARTESIAN_POINT('Ctrl Pts',(0.118224723989199,2.39980688969554,11.2103475381091));
#40854=CARTESIAN_POINT('Ctrl Pts',(0.118489190888015,2.39970246598156,11.2103299221318));
#40855=CARTESIAN_POINT('Ctrl Pts',(0.119322112804953,2.39937231520747,11.2102744790684));
#40856=CARTESIAN_POINT('Ctrl Pts',(0.119890067899432,2.39914531811557,11.2102367282776));
#40857=CARTESIAN_POINT('Ctrl Pts',(0.124574211061576,2.3972577032683,11.2099258094942));
#40858=CARTESIAN_POINT('Ctrl Pts',(0.128656583540053,2.3955137298424,11.2096575566237));
#40859=CARTESIAN_POINT('Ctrl Pts',(0.133385808904091,2.39337683086763,11.209348540669));
#40860=CARTESIAN_POINT('Ctrl Pts',(0.134068675389736,2.39306540090211,11.209303963966));
#40861=CARTESIAN_POINT('Ctrl Pts',(0.147305370410249,2.38697269040325,11.2084406076175));
#40862=CARTESIAN_POINT('Ctrl Pts',(0.159476800673317,2.38039154855982,11.2076589334872));
#40863=CARTESIAN_POINT('Ctrl Pts',(0.183658203039899,2.36523091259455,11.206058624942));
#40864=CARTESIAN_POINT('Ctrl Pts',(0.195577010718693,2.35656850234787,11.2052424318784));
#40865=CARTESIAN_POINT('Ctrl Pts',(0.219781571794237,2.33630723684455,11.2034504378983));
#40866=CARTESIAN_POINT('Ctrl Pts',(0.231831313928422,2.32449758894549,11.2024708155577));
#40867=CARTESIAN_POINT('Ctrl Pts',(0.243672787482944,2.31091733967566,11.2013753224514));
#40868=CARTESIAN_POINT('Ctrl Pts',(0.244438845653017,2.31002905088213,11.2013038063654));
#40869=CARTESIAN_POINT('Ctrl Pts',(0.245544253451992,2.30873302707068,11.2011996581206));
#40870=CARTESIAN_POINT('Ctrl Pts',(0.245887478845685,2.30832859797681,11.2011671855499));
#40871=CARTESIAN_POINT('Ctrl Pts',(0.2464859151481,2.30761990984583,11.2011103300268));
#40872=CARTESIAN_POINT('Ctrl Pts',(0.246741565746916,2.30731602220104,11.2010859651509));
#40873=CARTESIAN_POINT('Ctrl Pts',(0.247235302823283,2.3067269181715,11.2010387609057));
#40874=CARTESIAN_POINT('Ctrl Pts',(0.247473459189251,2.30644176092525,11.2010159244417));
#40875=CARTESIAN_POINT('Ctrl Pts',(0.248038414911546,2.30576292701271,11.2009615910351));
#40876=CARTESIAN_POINT('Ctrl Pts',(0.248364770165664,2.30536888357394,11.2009300760952));
#40877=CARTESIAN_POINT('Ctrl Pts',(0.249516236996881,2.30397183611664,11.2008184260229));
#40878=CARTESIAN_POINT('Ctrl Pts',(0.250336213842704,2.30296463340585,11.2007380834278));
#40879=CARTESIAN_POINT('Ctrl Pts',(0.264110365233951,2.28583496744804,11.1993741383148));
#40880=CARTESIAN_POINT('Ctrl Pts',(0.275486518072593,2.26851054009212,11.1980264471711));
#40881=CARTESIAN_POINT('Ctrl Pts',(0.298206251272945,2.22538733023949,11.1947590847124));
#40882=CARTESIAN_POINT('Ctrl Pts',(0.307989310832357,2.19895275257214,11.1928164904636));
#40883=CARTESIAN_POINT('Ctrl Pts',(0.31450507181521,2.17035150983895,11.1909550176108));
#40884=CARTESIAN_POINT('Ctrl Pts',(0.314778738451621,2.1691167206544,11.1908751275911));
#40885=CARTESIAN_POINT('Ctrl Pts',(0.315170035809796,2.16730063740992,11.190758356452));
#40886=CARTESIAN_POINT('Ctrl Pts',(0.31529333847217,2.16672059649205,11.1907211696297));
#40887=CARTESIAN_POINT('Ctrl Pts',(0.315485408764238,2.16580463544437,11.1906626220033));
#40888=CARTESIAN_POINT('Ctrl Pts',(0.315555241745524,2.16546894377188,11.1906412019184));
#40889=CARTESIAN_POINT('Ctrl Pts',(0.315686078668222,2.16483492944696,11.1906008170881));
#40890=CARTESIAN_POINT('Ctrl Pts',(0.315747195736611,2.16453663089756,11.1905818459469));
#40891=CARTESIAN_POINT('Ctrl Pts',(0.315851708661636,2.16402282472951,11.1905492204608));
#40892=CARTESIAN_POINT('Ctrl Pts',(0.315895306875682,2.16380735886874,11.1905355544618));
#40893=CARTESIAN_POINT('Ctrl Pts',(0.315979044848403,2.16339132967506,11.1905091979407));
#40894=CARTESIAN_POINT('Ctrl Pts',(0.316019214090229,2.16319077296282,11.1904965057144));
#40895=CARTESIAN_POINT('Ctrl Pts',(0.316113197175031,2.1627192039169,11.1904666940577));
#40896=CARTESIAN_POINT('Ctrl Pts',(0.316166853583983,2.16244815981532,11.1904495836958));
#40897=CARTESIAN_POINT('Ctrl Pts',(0.316323760870393,2.16165016038049,11.1903992791347));
#40898=CARTESIAN_POINT('Ctrl Pts',(0.316426044030888,2.16112301231846,11.1903661399613));
#40899=CARTESIAN_POINT('Ctrl Pts',(0.317291007385889,2.15660479260114,11.1900828652619));
#40900=CARTESIAN_POINT('Ctrl Pts',(0.317979504687194,2.15259966007758,11.1898368576505));
#40901=CARTESIAN_POINT('Ctrl Pts',(0.321896462525297,2.12691313595252,11.1882854398066));
#40902=CARTESIAN_POINT('Ctrl Pts',(0.322981878540907,2.10496044507895,11.1870762052888));
#40903=CARTESIAN_POINT('Ctrl Pts',(0.321076436946661,2.06874910247598,11.1850472913117));
#40904=CARTESIAN_POINT('Ctrl Pts',(0.319368744020788,2.05449989656714,11.1842405294662));
#40905=CARTESIAN_POINT('Ctrl Pts',(0.315142780545402,2.03203812379401,11.1829133508353));
#40906=CARTESIAN_POINT('Ctrl Pts',(0.313235813604235,2.02373011712177,11.1824102444439));
#40907=CARTESIAN_POINT('Ctrl Pts',(0.310565814597484,2.0139022717199,11.181796198236));
#40908=CARTESIAN_POINT('Ctrl Pts',(0.310117175908395,2.01230005097512,11.1816954866114));
#40909=CARTESIAN_POINT('Ctrl Pts',(0.309312491112667,2.00950968698331,11.1815190010501));
#40910=CARTESIAN_POINT('Ctrl Pts',(0.308961952652534,2.00831998225319,11.181443406533));
#40911=CARTESIAN_POINT('Ctrl Pts',(0.308448177452069,2.00661267773816,11.1813344126332));
#40912=CARTESIAN_POINT('Ctrl Pts',(0.30829048404227,2.00609341036949,11.1813011945935));
#40913=CARTESIAN_POINT('Ctrl Pts',(0.308014519554895,2.00519287621554,11.181243467265));
#40914=CARTESIAN_POINT('Ctrl Pts',(0.307896849927373,2.00481142516353,11.1812189777286));
#40915=CARTESIAN_POINT('Ctrl Pts',(0.307669215582214,2.00407833848334,11.1811718408395));
#40916=CARTESIAN_POINT('Ctrl Pts',(0.307559355927551,2.00372667064669,11.1811491969664));
#40917=CARTESIAN_POINT('Ctrl Pts',(0.307299091623264,2.00289853991067,11.1810957980815));
#40918=CARTESIAN_POINT('Ctrl Pts',(0.307148181830025,2.0024222378921,11.1810650265071));
#40919=CARTESIAN_POINT('Ctrl Pts',(0.306699044088186,2.0010160334167,11.180974002785));
#40920=CARTESIAN_POINT('Ctrl Pts',(0.306397698388591,2.00008713959804,11.1809136481302));
#40921=CARTESIAN_POINT('Ctrl Pts',(0.303679116966014,1.99183512242224,11.1803754276997));
#40922=CARTESIAN_POINT('Ctrl Pts',(0.301004157866724,1.98460014184695,11.1798890747005));
#40923=CARTESIAN_POINT('Ctrl Pts',(0.296756684033871,1.97426765330199,11.1791724056787));
#40924=CARTESIAN_POINT('Ctrl Pts',(0.2953894403431,1.97108828732678,11.1789487811933));
#40925=CARTESIAN_POINT('Ctrl Pts',(0.282900253255653,1.94328857258051,11.1769661304825));
#40926=CARTESIAN_POINT('Ctrl Pts',(0.268774979054459,1.92013708425124,11.1751115548118));
#40927=CARTESIAN_POINT('Ctrl Pts',(0.247787912721925,1.89382900540209,11.1728595445137));
#40928=CARTESIAN_POINT('Ctrl Pts',(0.243484203653094,1.88876368386816,11.1724189725811));
#40929=CARTESIAN_POINT('Ctrl Pts',(0.235436107571636,1.87986442529763,11.1716370361573));
#40930=CARTESIAN_POINT('Ctrl Pts',(0.231746855031262,1.87598385035512,11.1712931624396));
#40931=CARTESIAN_POINT('Ctrl Pts',(0.227487563396585,1.87172158370865,11.1709139301591));
#40932=CARTESIAN_POINT('Ctrl Pts',(0.227011255874286,1.87124791461094,11.1708717639116));
#40933=CARTESIAN_POINT('Ctrl Pts',(0.226267118919601,1.87051251287593,11.1708062690723));
#40934=CARTESIAN_POINT('Ctrl Pts',(0.226000311769296,1.87024975531191,11.1707828620879));
#40935=CARTESIAN_POINT('Ctrl Pts',(0.225553056226599,1.86981082117102,11.1707437521506));
#40936=CARTESIAN_POINT('Ctrl Pts',(0.22537285879264,1.86963439114361,11.1707280294873));
#40937=CARTESIAN_POINT('Ctrl Pts',(0.225020911832249,1.86929061057975,11.1706973889708));
#40938=CARTESIAN_POINT('Ctrl Pts',(0.224849182308022,1.86912323992053,11.1706824695363));
#40939=CARTESIAN_POINT('Ctrl Pts',(0.224524020966735,1.86880703876358,11.1706542798342));
#40940=CARTESIAN_POINT('Ctrl Pts',(0.224370629137461,1.86865817045535,11.1706410066135));
#40941=CARTESIAN_POINT('Ctrl Pts',(0.224016326330692,1.8683149998818,11.1706104057283));
#40942=CARTESIAN_POINT('Ctrl Pts',(0.223815310910442,1.86812080656957,11.1705930866693));
#40943=CARTESIAN_POINT('Ctrl Pts',(0.223202671170461,1.86753049759624,11.1705404311935));
#40944=CARTESIAN_POINT('Ctrl Pts',(0.22279024321544,1.86713521196774,11.1705051594211));
#40945=CARTESIAN_POINT('Ctrl Pts',(0.219833462812496,1.86431637404737,11.1702535236381));
#40946=CARTESIAN_POINT('Ctrl Pts',(0.217250551001605,1.86193336340606,11.1700402219281));
#40947=CARTESIAN_POINT('Ctrl Pts',(0.196989426977284,1.8438447673167,11.1684118011165));
#40948=CARTESIAN_POINT('Ctrl Pts',(0.177667599327041,1.83008357075567,11.1671135651346));
#40949=CARTESIAN_POINT('Ctrl Pts',(0.145559128197653,1.81217072971679,11.1650540867161));
#40950=CARTESIAN_POINT('Ctrl Pts',(0.133728251883271,1.8064870230169,11.1643141049457));
#40951=CARTESIAN_POINT('Ctrl Pts',(0.113642965582844,1.79830480511951,11.1630551781468));
#40952=CARTESIAN_POINT('Ctrl Pts',(0.105575822666422,1.79538804882416,11.1625490226636));
#40953=CARTESIAN_POINT('Ctrl Pts',(0.0949687400073146,1.79202494829385,
11.1618781984801));
#40954=CARTESIAN_POINT('Ctrl Pts',(0.0925259912391918,1.791282273883,11.1617233649469));
#40955=CARTESIAN_POINT('Ctrl Pts',(0.0893853738948245,1.79036804745345,
11.1615237699575));
#40956=CARTESIAN_POINT('Ctrl Pts',(0.0886953543514017,1.79016968320151,
11.1614798849497));
#40957=CARTESIAN_POINT('Ctrl Pts',(0.0875850338067536,1.78985450547714,
11.1614092149451));
#40958=CARTESIAN_POINT('Ctrl Pts',(0.0871651457482567,1.78973623594837,
11.1613824774016));
#40959=CARTESIAN_POINT('Ctrl Pts',(0.0863666376024173,1.78951306969385,
11.1613316061232));
#40960=CARTESIAN_POINT('Ctrl Pts',(0.085988062998148,1.78940801201361,11.1613074776737));
#40961=CARTESIAN_POINT('Ctrl Pts',(0.0851268238044925,1.78917070609547,
11.1612525628597));
#40962=CARTESIAN_POINT('Ctrl Pts',(0.0846440422280816,1.78903888958421,
11.1612217625379));
#40963=CARTESIAN_POINT('Ctrl Pts',(0.0832110993756456,1.78865122959978,
11.1611302928646));
#40964=CARTESIAN_POINT('Ctrl Pts',(0.0822600776489263,1.78839861444494,
11.1610695190216));
#40965=CARTESIAN_POINT('Ctrl Pts',(0.0757240228596573,1.78669448217,11.1606513642812));
#40966=CARTESIAN_POINT('Ctrl Pts',(0.0701023438682621,1.78538892331602,
11.1602892954836));
#40967=CARTESIAN_POINT('Ctrl Pts',(0.0633030533443531,1.78400116014501,
11.1598481107241));
#40968=CARTESIAN_POINT('Ctrl Pts',(0.0621559262149118,1.78377352398619,
11.1597735672833));
#40969=CARTESIAN_POINT('Ctrl Pts',(0.0305142368402735,1.77767336127625,
11.1577143530949));
#40970=CARTESIAN_POINT('Ctrl Pts',(-0.000665465190473068,1.77623402889956,
11.1555837734216));
#40971=CARTESIAN_POINT('Ctrl Pts',(-0.0431443463476149,1.7804139342069,
11.1527247989634));
#40972=CARTESIAN_POINT('Ctrl Pts',(-0.0546605162650784,1.78218090287316,
11.1519570922089));
#40973=CARTESIAN_POINT('Ctrl Pts',(-0.0670786734378294,1.78478147759472,
11.1511542696831));
#40974=CARTESIAN_POINT('Ctrl Pts',(-0.0680993544880657,1.78500040748456,
11.1510884720872));
#40975=CARTESIAN_POINT('Ctrl Pts',(-0.0698557039191077,1.78538606959842,
11.1509755963115));
#40976=CARTESIAN_POINT('Ctrl Pts',(-0.0705918766489096,1.78555043083012,
11.1509283895594));
#40977=CARTESIAN_POINT('Ctrl Pts',(-0.0716328708023237,1.78578668787489,
11.1508617916843));
#40978=CARTESIAN_POINT('Ctrl Pts',(-0.0719381676920451,1.78585644407832,
11.15084227918));
#40979=CARTESIAN_POINT('Ctrl Pts',(-0.0724617971480981,1.78597688967753,
11.1508088454324));
#40980=CARTESIAN_POINT('Ctrl Pts',(-0.0726801789829622,1.78602736194589,
11.150794911635));
#40981=CARTESIAN_POINT('Ctrl Pts',(-0.0730979400746548,1.78612437383693,
11.1507682756381));
#40982=CARTESIAN_POINT('Ctrl Pts',(-0.0732973273698071,1.78617087556532,
11.1507555712502));
#40983=CARTESIAN_POINT('Ctrl Pts',(-0.0737664575355801,1.78628075904453,
11.1507256989386));
#40984=CARTESIAN_POINT('Ctrl Pts',(-0.0740361637636604,1.78634429885698,
11.150708540177));
#40985=CARTESIAN_POINT('Ctrl Pts',(-0.0748312611590856,1.78653269771403,
11.1506579993924));
#40986=CARTESIAN_POINT('Ctrl Pts',(-0.0753564241334326,1.78665853035246,
11.1506246731293));
#40987=CARTESIAN_POINT('Ctrl Pts',(-0.0799049534559692,1.78776048571096,
11.1503364944292));
#40988=CARTESIAN_POINT('Ctrl Pts',(-0.0839097086400566,1.7888127885025,
11.1500859287721));
#40989=CARTESIAN_POINT('Ctrl Pts',(-0.0882443117006682,1.79004153473639,
11.1498170730391));
#40990=CARTESIAN_POINT('Ctrl Pts',(-0.0885951571941766,1.79014163419365,
11.1497953285321));
#40991=CARTESIAN_POINT('Ctrl Pts',(-0.089197947030021,1.79031472319032,
11.1497579969354));
#40992=CARTESIAN_POINT('Ctrl Pts',(-0.0894499728793633,1.79038742470663,
11.1497423969871));
#40993=CARTESIAN_POINT('Ctrl Pts',(-0.117807831053197,1.7986052887049,11.1479880083282));
#40994=CARTESIAN_POINT('Ctrl Pts',(-0.144676856635989,1.81054096151597,
11.1464158822174));
#40995=CARTESIAN_POINT('Ctrl Pts',(-0.182302251693312,1.83382091072605,
11.143902255676));
#40996=CARTESIAN_POINT('Ctrl Pts',(-0.194470363975291,1.84257698301877,
11.1430331014031));
#40997=CARTESIAN_POINT('Ctrl Pts',(-0.20720562916949,1.85316093801789,11.1420339906839));
#40998=CARTESIAN_POINT('Ctrl Pts',(-0.208418884574288,1.85418449256799,
11.1419378612906));
#40999=CARTESIAN_POINT('Ctrl Pts',(-0.210531607811743,1.85599376239595,
11.1417687670302));
#41000=CARTESIAN_POINT('Ctrl Pts',(-0.211434368456021,1.8567755981547,11.1416959616922));
#41001=CARTESIAN_POINT('Ctrl Pts',(-0.212734734273322,1.85791449031987,
11.1415902790221));
#41002=CARTESIAN_POINT('Ctrl Pts',(-0.213135837161863,1.85826755270484,
11.1415575680086));
#41003=CARTESIAN_POINT('Ctrl Pts',(-0.213833978093957,1.85888516500358,
11.1415004346921));
#41004=CARTESIAN_POINT('Ctrl Pts',(-0.214131408721481,1.85914927104221,
11.1414760309989));
#41005=CARTESIAN_POINT('Ctrl Pts',(-0.214704923779828,1.85966043066521,
11.1414288526659));
#41006=CARTESIAN_POINT('Ctrl Pts',(-0.214981072798249,1.85990741115131,
11.1414060811192));
#41007=CARTESIAN_POINT('Ctrl Pts',(-0.215634589475266,1.86049393088982,
11.1413520603655));
#41008=CARTESIAN_POINT('Ctrl Pts',(-0.216011581135442,1.8608338859089,11.1413207936436));
#41009=CARTESIAN_POINT('Ctrl Pts',(-0.217332760792655,1.86203094145216,
11.1412108510957));
#41010=CARTESIAN_POINT('Ctrl Pts',(-0.218272654015633,1.86289274542222,
11.1411319760462));
#41011=CARTESIAN_POINT('Ctrl Pts',(-0.231831284114687,1.87547382062437,
11.1399844216267));
#41012=CARTESIAN_POINT('Ctrl Pts',(-0.243493797013867,1.88817850576825,
11.1388720569459));
#41013=CARTESIAN_POINT('Ctrl Pts',(-0.266656452250681,1.91786489637708,
11.1363697114697));
#41014=CARTESIAN_POINT('Ctrl Pts',(-0.27766703046908,1.93513702317913,11.1349713234374));
#41015=CARTESIAN_POINT('Ctrl Pts',(-0.290871241177242,1.96097234106822,
11.1330287542691));
#41016=CARTESIAN_POINT('Ctrl Pts',(-0.294469114255374,1.96876459170062,
11.1324610320473));
#41017=CARTESIAN_POINT('Ctrl Pts',(-0.299380234701648,1.98062345002478,
11.131632784031));
#41018=CARTESIAN_POINT('Ctrl Pts',(-0.30093056188646,1.98458731913911,11.1313617357899));
#41019=CARTESIAN_POINT('Ctrl Pts',(-0.302592309191356,1.98909746158374,
11.1310607566978));
#41020=CARTESIAN_POINT('Ctrl Pts',(-0.302781288963815,1.98961444989041,
11.1310263652634));
#41021=CARTESIAN_POINT('Ctrl Pts',(-0.303062795549528,1.99039072409714,
11.1309748918061));
#41022=CARTESIAN_POINT('Ctrl Pts',(-0.30315631496482,1.99064964513751,11.1309577508931));
#41023=CARTESIAN_POINT('Ctrl Pts',(-0.303316468447645,1.99109483607576,
11.1309283266668));
#41024=CARTESIAN_POINT('Ctrl Pts',(-0.303383262730744,1.99128104739011,
11.1309160337373));
#41025=CARTESIAN_POINT('Ctrl Pts',(-0.303521293162504,1.99166697096075,
11.1308905865732));
#41026=CARTESIAN_POINT('Ctrl Pts',(-0.303592503478052,1.99186669145726,
11.1308774339137));
#41027=CARTESIAN_POINT('Ctrl Pts',(-0.303786591998069,1.99241274614059,
11.1308415182288));
#41028=CARTESIAN_POINT('Ctrl Pts',(-0.303909075496294,1.99275922181843,
11.1308187788229));
#41029=CARTESIAN_POINT('Ctrl Pts',(-0.304372682610936,1.99407782527937,
11.1307324229937));
#41030=CARTESIAN_POINT('Ctrl Pts',(-0.304709741401117,1.99505139076526,
11.1306690456774));
#41031=CARTESIAN_POINT('Ctrl Pts',(-0.310970101904116,2.0134183306045,11.1294802755612));
#41032=CARTESIAN_POINT('Ctrl Pts',(-0.315400836322276,2.03128815683696,
11.1284388282697));
#41033=CARTESIAN_POINT('Ctrl Pts',(-0.320928806882402,2.06608821077844,
11.1264630025729));
#41034=CARTESIAN_POINT('Ctrl Pts',(-0.32226302998602,2.08291697756033,11.1255295197136));
#41035=CARTESIAN_POINT('Ctrl Pts',(-0.322279117997924,2.10572423217828,
11.1242264343365));
#41036=CARTESIAN_POINT('Ctrl Pts',(-0.322118451696256,2.11167452734151,
11.1238831533318));
#41037=CARTESIAN_POINT('Ctrl Pts',(-0.321647698777409,2.12027344737234,
11.1233800252546));
#41038=CARTESIAN_POINT('Ctrl Pts',(-0.32146936504506,2.12292818301118,11.1232237255624));
#41039=CARTESIAN_POINT('Ctrl Pts',(-0.32075409603904,2.1319110928246,11.1226911743545));
#41040=CARTESIAN_POINT('Ctrl Pts',(-0.320063017265102,2.1382251811988,11.1223106207509));
#41041=CARTESIAN_POINT('Ctrl Pts',(-0.319044223611113,2.14553033222982,
11.1218616849225));
#41042=CARTESIAN_POINT('Ctrl Pts',(-0.318897694264697,2.14654555109881,
11.121799100939));
#41043=CARTESIAN_POINT('Ctrl Pts',(-0.318672223507138,2.14805665093449,
11.1217056530564));
#41044=CARTESIAN_POINT('Ctrl Pts',(-0.31859696480177,2.14855308176226,11.1216749058185));
#41045=CARTESIAN_POINT('Ctrl Pts',(-0.318460721454884,2.149437829895,11.1216200221086));
#41046=CARTESIAN_POINT('Ctrl Pts',(-0.318400185796314,2.1498262161617,11.1215958999131));
#41047=CARTESIAN_POINT('Ctrl Pts',(-0.318271112559775,2.15064448670135,
11.1215450158031));
#41048=CARTESIAN_POINT('Ctrl Pts',(-0.318202414281175,2.15107434449849,
11.121518248835));
#41049=CARTESIAN_POINT('Ctrl Pts',(-0.318018756444221,2.15220877137954,
11.1214475123212));
#41050=CARTESIAN_POINT('Ctrl Pts',(-0.317902326837207,2.15291309703346,
11.1214034961857));
#41051=CARTESIAN_POINT('Ctrl Pts',(-0.317365517759242,2.15609471886882,
11.1212042144911));
#41052=CARTESIAN_POINT('Ctrl Pts',(-0.316918523890522,2.15856737989268,
11.1210481052854));
#41053=CARTESIAN_POINT('Ctrl Pts',(-0.314833793246507,2.16937598269823,
11.1203601355605));
#41054=CARTESIAN_POINT('Ctrl Pts',(-0.312895858390997,2.17764988373085,
11.1198187847556));
#41055=CARTESIAN_POINT('Ctrl Pts',(-0.306831272443274,2.19959687304708,
11.118342079836));
#41056=CARTESIAN_POINT('Ctrl Pts',(-0.302119352988017,2.21308752254531,
11.1173902852623));
#41057=CARTESIAN_POINT('Ctrl Pts',(-0.286749788100479,2.24919526734346,
11.1147432845072));
#41058=CARTESIAN_POINT('Ctrl Pts',(-0.274332596453154,2.27095759539256,
11.113029537657));
#41059=CARTESIAN_POINT('Ctrl Pts',(-0.258680684119955,2.29221735861426,
11.1113609142009));
#41060=CARTESIAN_POINT('Ctrl Pts',(-0.257827572545595,2.29336016214196,
11.1112712594194));
#41061=CARTESIAN_POINT('Ctrl Pts',(-0.256714457306904,2.29483079319912,
11.1111559798661));
#41062=CARTESIAN_POINT('Ctrl Pts',(-0.256461379224928,2.29516380694108,
11.1111298819214));
#41063=CARTESIAN_POINT('Ctrl Pts',(-0.256072829916008,2.29567302011369,
11.1110899862565));
#41064=CARTESIAN_POINT('Ctrl Pts',(-0.255937824764592,2.29584957206252,
11.1110761558261));
#41065=CARTESIAN_POINT('Ctrl Pts',(-0.255671380674219,2.29619726627702,
11.1110489229284));
#41066=CARTESIAN_POINT('Ctrl Pts',(-0.25553995325328,2.2963684151851,11.1110355198537));
#41067=CARTESIAN_POINT('Ctrl Pts',(-0.25524660623941,2.29674962762791,11.1110056706771));
#41068=CARTESIAN_POINT('Ctrl Pts',(-0.255084599612639,2.2969596227914,11.1109892309105));
#41069=CARTESIAN_POINT('Ctrl Pts',(-0.254615165849222,2.29756655844655,
11.1109417239758));
#41070=CARTESIAN_POINT('Ctrl Pts',(-0.254307068377375,2.2979629831009,11.1109107042241));
#41071=CARTESIAN_POINT('Ctrl Pts',(-0.252197798673163,2.30066390020984,
11.1106994150509));
#41072=CARTESIAN_POINT('Ctrl Pts',(-0.250366178895085,2.3029445944537,11.1105212699617));
#41073=CARTESIAN_POINT('Ctrl Pts',(-0.244520805746983,2.31002352155858,
11.1099680631264));
#41074=CARTESIAN_POINT('Ctrl Pts',(-0.240398061280094,2.31473026535673,
11.1095998306152));
#41075=CARTESIAN_POINT('Ctrl Pts',(-0.225764312132883,2.33048675150322,
11.1083537559461));
#41076=CARTESIAN_POINT('Ctrl Pts',(-0.214607462332204,2.3409094563838,11.1075050890333));
#41077=CARTESIAN_POINT('Ctrl Pts',(-0.182738411805528,2.36670379927038,
11.1052131722153));
#41078=CARTESIAN_POINT('Ctrl Pts',(-0.160857040059098,2.38044428517751,
11.1037637547439));
#41079=CARTESIAN_POINT('Ctrl Pts',(-0.136162617065269,2.39210162444621,
11.1021081069975));
#41080=CARTESIAN_POINT('Ctrl Pts',(-0.134744754261485,2.39275837879598,
11.1020130196591));
#41081=CARTESIAN_POINT('Ctrl Pts',(-0.132818375103367,2.39363371928278,
11.1018837746176));
#41082=CARTESIAN_POINT('Ctrl Pts',(-0.132313973312393,2.39386135221428,
11.101849928158));
#41083=CARTESIAN_POINT('Ctrl Pts',(-0.131459630790511,2.39424426530894,
11.1017925904391));
#41084=CARTESIAN_POINT('Ctrl Pts',(-0.131109993854174,2.39440022368247,
11.1017691224852));
#41085=CARTESIAN_POINT('Ctrl Pts',(-0.130437166088818,2.39469890761734,
11.1017239561701));
#41086=CARTESIAN_POINT('Ctrl Pts',(-0.130114016632863,2.39484172554479,
11.1017022610099));
#41087=CARTESIAN_POINT('Ctrl Pts',(-0.129352654250365,2.39517671897671,
11.1016511396702));
#41088=CARTESIAN_POINT('Ctrl Pts',(-0.128914247759272,2.39536845008942,
11.1016216983517));
#41089=CARTESIAN_POINT('Ctrl Pts',(-0.127639979228913,2.39592235665005,
11.101536109849));
#41090=CARTESIAN_POINT('Ctrl Pts',(-0.126803011665821,2.39628196311635,
11.1014798751963));
#41091=CARTESIAN_POINT('Ctrl Pts',(-0.120904922981518,2.39878653090654,
11.1010834480923));
#41092=CARTESIAN_POINT('Ctrl Pts',(-0.115791439402396,2.40080513293414,
11.100738994105));
#41093=CARTESIAN_POINT('Ctrl Pts',(-0.0994712558807518,2.40676990086376,
11.0996363197452));
#41094=CARTESIAN_POINT('Ctrl Pts',(-0.0880977061581307,2.41022740422566,
11.0988625954484));
#41095=CARTESIAN_POINT('Ctrl Pts',(-0.0449963585995469,2.42076841611452,
11.095917465657));
#41096=CARTESIAN_POINT('Ctrl Pts',(-0.0124488653819679,2.42366955683189,
11.0936472027799));
#41097=CARTESIAN_POINT('Ctrl Pts',(0.0214561711553594,2.42156335563747,
11.0914990887251));
#41098=CARTESIAN_POINT('Ctrl Pts',(0.0229303290677825,2.4214615982928,11.0914061658428));
#41099=CARTESIAN_POINT('Ctrl Pts',(0.0248265762976301,2.42131759449503,
11.0912872934295));
#41100=CARTESIAN_POINT('Ctrl Pts',(0.0252493235984321,2.4212846511825,11.0912608341821));
#41101=CARTESIAN_POINT('Ctrl Pts',(0.0259194047849398,2.42123110322143,
11.091218962582));
#41102=CARTESIAN_POINT('Ctrl Pts',(0.026166780128673,2.42121104719477,11.0912035194437));
#41103=CARTESIAN_POINT('Ctrl Pts',(0.0266102105352606,2.42117458029343,
11.0911758636298));
#41104=CARTESIAN_POINT('Ctrl Pts',(0.0268062723042598,2.42115827577202,
11.0911636450406));
#41105=CARTESIAN_POINT('Ctrl Pts',(0.0272674612588645,2.42111949797235,
11.0911349256308));
#41106=CARTESIAN_POINT('Ctrl Pts',(0.0275325752427082,2.42109687591636,
11.0911184333299));
#41107=CARTESIAN_POINT('Ctrl Pts',(0.0283018649697433,2.4210302730123,11.0910706257092));
#41108=CARTESIAN_POINT('Ctrl Pts',(0.0288059684242431,2.42098543260172,
11.0910393587396));
#41109=CARTESIAN_POINT('Ctrl Pts',(0.0323107292670041,2.42066535838381,
11.0908223848903));
#41110=CARTESIAN_POINT('Ctrl Pts',(0.0353076301967922,2.42034922837953,
11.0906389351467));
#41111=CARTESIAN_POINT('Ctrl Pts',(0.0446266766786995,2.41923383023239,
11.0900737592643));
#41112=CARTESIAN_POINT('Ctrl Pts',(0.0509301623547187,2.41828903274906,
11.0896990414985));
#41113=CARTESIAN_POINT('Ctrl Pts',(0.0727402495397434,2.41435541333712,
11.0884162132588));
#41114=CARTESIAN_POINT('Ctrl Pts',(0.0880526634141122,2.41041466362918,
11.087539050788));
#41115=CARTESIAN_POINT('Ctrl Pts',(0.126801261285647,2.39734285721421,11.0852523562657));
#41116=CARTESIAN_POINT('Ctrl Pts',(0.149564247831897,2.38656869013924,11.0838353556271));
#41117=CARTESIAN_POINT('Ctrl Pts',(0.172103804205766,2.37247689678683,11.0822228713464));
#41118=CARTESIAN_POINT('Ctrl Pts',(0.173356886600899,2.3716813730417,11.082132519326));
#41119=CARTESIAN_POINT('Ctrl Pts',(0.175059611923363,2.37058381547612,11.0820087616163));
#41120=CARTESIAN_POINT('Ctrl Pts',(0.175514068538771,2.37028925369628,11.0819756342714));
#41121=CARTESIAN_POINT('Ctrl Pts',(0.176285778108725,2.36978629346281,11.0819192156953));
#41122=CARTESIAN_POINT('Ctrl Pts',(0.176603410390046,2.36957847677515,11.0818959462469));
#41123=CARTESIAN_POINT('Ctrl Pts',(0.177243009337119,2.36915839200497,11.0818489929649));
#41124=CARTESIAN_POINT('Ctrl Pts',(0.177564963603618,2.3689461062072,11.0818253084913));
#41125=CARTESIAN_POINT('Ctrl Pts',(0.178295694490519,2.36846240280061,11.0817714391224));
#41126=CARTESIAN_POINT('Ctrl Pts',(0.178704233102021,2.36819062895356,11.0817412408593));
#41127=CARTESIAN_POINT('Ctrl Pts',(0.179557545754608,2.36762016073199,11.081677995748));
#41128=CARTESIAN_POINT('Ctrl Pts',(0.1800021984696,2.36732128835576,11.0816449422332));
#41129=CARTESIAN_POINT('Ctrl Pts',(0.181165921206137,2.36653487460004,11.0815581800709));
#41130=CARTESIAN_POINT('Ctrl Pts',(0.181883765084588,2.36604553437236,11.0815044033373));
#41131=CARTESIAN_POINT('Ctrl Pts',(0.18401015692187,2.36458338597921,11.0813443345965));
#41132=CARTESIAN_POINT('Ctrl Pts',(0.185412925159595,2.36360226286643,11.0812377265307));
#41133=CARTESIAN_POINT('Ctrl Pts',(0.200764104832932,2.35268219260395,11.0800597461879));
#41134=CARTESIAN_POINT('Ctrl Pts',(0.213904514039949,2.34165928001635,11.0789456286619));
#41135=CARTESIAN_POINT('Ctrl Pts',(0.246240300319671,2.30982207801136,11.075917236271));
#41136=CARTESIAN_POINT('Ctrl Pts',(0.263679868442746,2.2874366970557,11.0739587115042));
#41137=CARTESIAN_POINT('Ctrl Pts',(0.279718055797393,2.26009630305539,11.0719233937438));
#41138=CARTESIAN_POINT('Ctrl Pts',(0.281411632792724,2.25710032551796,11.0717048798757));
#41139=CARTESIAN_POINT('Ctrl Pts',(0.283328344537239,2.25357912285398,11.0714537815786));
#41140=CARTESIAN_POINT('Ctrl Pts',(0.283598395506784,2.25307987415876,11.0714183124619));
#41141=CARTESIAN_POINT('Ctrl Pts',(0.28399910708349,2.25233437073984,11.0713655484525));
#41142=CARTESIAN_POINT('Ctrl Pts',(0.284130767607277,2.25208865912102,11.0713481902297));
#41143=CARTESIAN_POINT('Ctrl Pts',(0.284365210050861,2.25164976366982,11.0713172427194));
#41144=CARTESIAN_POINT('Ctrl Pts',(0.284468113929106,2.25145664616336,11.0713036456383));
#41145=CARTESIAN_POINT('Ctrl Pts',(0.284686704167322,2.25104541387169,11.0712747342533));
#41146=CARTESIAN_POINT('Ctrl Pts',(0.284802336260141,2.25082727154951,11.0712594234496));
#41147=CARTESIAN_POINT('Ctrl Pts',(0.285113172787784,2.25023924004627,11.0712182193114));
#41148=CARTESIAN_POINT('Ctrl Pts',(0.285307908893267,2.24986910180032,11.0711923557973));
#41149=CARTESIAN_POINT('Ctrl Pts',(0.286251249457965,2.24806757604753,11.071066820996));
#41150=CARTESIAN_POINT('Ctrl Pts',(0.286989822621137,2.24663092054597,11.0709677756827));
#41151=CARTESIAN_POINT('Ctrl Pts',(0.291186723640849,2.23831400680171,11.0704001595333));
#41152=CARTESIAN_POINT('Ctrl Pts',(0.294408667973479,2.23131652476751,11.0699452060125));
#41153=CARTESIAN_POINT('Ctrl Pts',(0.303225123611616,2.21020858436422,11.0686195744459));
#41154=CARTESIAN_POINT('Ctrl Pts',(0.308077472363713,2.19581095917314,11.0677748511331));
#41155=CARTESIAN_POINT('Ctrl Pts',(0.314869487164515,2.16969776225745,11.0662665723314));
#41156=CARTESIAN_POINT('Ctrl Pts',(0.317211239260883,2.1581169896719,11.0656057025822));
#41157=CARTESIAN_POINT('Ctrl Pts',(0.320996684282201,2.13211842079167,11.0641039172204));
#41158=CARTESIAN_POINT('Ctrl Pts',(0.322114557332758,2.11768027433914,11.0632573188632));
#41159=CARTESIAN_POINT('Ctrl Pts',(0.322271302044505,2.10197901312523,11.0623032319578));
#41160=CARTESIAN_POINT('Ctrl Pts',(0.322276526654214,2.10074088812983,11.0622277801365));
#41161=CARTESIAN_POINT('Ctrl Pts',(0.322273843065144,2.0990015220015,11.0621214676756));
#41162=CARTESIAN_POINT('Ctrl Pts',(0.322271900252881,2.09850027162237,11.0620907938385));
#41163=CARTESIAN_POINT('Ctrl Pts',(0.322266497944401,2.0976301958884,11.062037485386));
#41164=CARTESIAN_POINT('Ctrl Pts',(0.322263574667099,2.09726136716151,11.0620148675977));
#41165=CARTESIAN_POINT('Ctrl Pts',(0.32225624989628,2.09650174838609,11.0619682435209));
#41166=CARTESIAN_POINT('Ctrl Pts',(0.322251770710347,2.09611095982051,11.0619442348352));
#41167=CARTESIAN_POINT('Ctrl Pts',(0.32223959754566,2.09519438803488,11.0618878700318));
#41168=CARTESIAN_POINT('Ctrl Pts',(0.322231327556487,2.0946686147481,11.0618554959246));
#41169=CARTESIAN_POINT('Ctrl Pts',(0.322211171522466,2.09355975953625,11.0617871304216));
#41170=CARTESIAN_POINT('Ctrl Pts',(0.322198989441538,2.09297668548288,11.0617511298493));
#41171=CARTESIAN_POINT('Ctrl Pts',(0.322162028490324,2.0914111154573,11.0616543271295));
#41172=CARTESIAN_POINT('Ctrl Pts',(0.322134338011105,2.09042870027305,11.0615934338998));
#41173=CARTESIAN_POINT('Ctrl Pts',(0.322035864637907,2.08742322411333,11.0614066837301));
#41174=CARTESIAN_POINT('Ctrl Pts',(0.321950515038195,2.08540072021513,11.0612803722761));
#41175=CARTESIAN_POINT('Ctrl Pts',(0.32029236528087,2.05329223099935,11.0592646618716));
#41176=CARTESIAN_POINT('Ctrl Pts',(0.314527605761694,2.02357761218143,11.0572323069601));
#41177=CARTESIAN_POINT('Ctrl Pts',(0.299903426465526,1.9810939538075,11.0541958279302));
#41178=CARTESIAN_POINT('Ctrl Pts',(0.294119812161654,1.96743176257577,11.0532013403303));
#41179=CARTESIAN_POINT('Ctrl Pts',(0.285910411790693,1.95124688877837,11.0520369663987));
#41180=CARTESIAN_POINT('Ctrl Pts',(0.2843589592489,1.94830215524334,11.0518257401204));
#41181=CARTESIAN_POINT('Ctrl Pts',(0.282495867423631,1.9448949761208,11.05158253724));
#41182=CARTESIAN_POINT('Ctrl Pts',(0.282228381032615,1.9444087904327,11.051547862261));
#41183=CARTESIAN_POINT('Ctrl Pts',(0.281824021988285,1.94367829750742,11.0514958092828));
#41184=CARTESIAN_POINT('Ctrl Pts',(0.281688086219814,1.94343347700394,11.0514783718401));
#41185=CARTESIAN_POINT('Ctrl Pts',(0.281445290663683,1.942997541639,11.0514473365238));
#41186=CARTESIAN_POINT('Ctrl Pts',(0.281338555273559,1.94280635863426,11.051433730683));
#41187=CARTESIAN_POINT('Ctrl Pts',(0.281111425655288,1.94240049945948,11.0514048577014));
#41188=CARTESIAN_POINT('Ctrl Pts',(0.280990980664248,1.94218585300777,11.0513895939443));
#41189=CARTESIAN_POINT('Ctrl Pts',(0.280666881642268,1.94160981959497,11.0513486478316));
#41190=CARTESIAN_POINT('Ctrl Pts',(0.280462774706148,1.94124868596375,11.0513229946538));
#41191=CARTESIAN_POINT('Ctrl Pts',(0.279479200947461,1.93951623153267,11.0512000074647));
#41192=CARTESIAN_POINT('Ctrl Pts',(0.278690353321097,1.93815022116898,11.0511032691406));
#41193=CARTESIAN_POINT('Ctrl Pts',(0.27203104218852,1.92681166241834,11.0503017892195));
#41194=CARTESIAN_POINT('Ctrl Pts',(0.26563667952492,1.91715496782149,11.0496287843113));
#41195=CARTESIAN_POINT('Ctrl Pts',(0.240250574813183,1.88296961864961,11.047202714715));
#41196=CARTESIAN_POINT('Ctrl Pts',(0.218270933963974,1.86087572183108,11.0455293532236));
#41197=CARTESIAN_POINT('Ctrl Pts',(0.192520298191899,1.84154588523502,11.0436320462348));
#41198=CARTESIAN_POINT('Ctrl Pts',(0.191563664544495,1.84083604218772,11.0435616702048));
#41199=CARTESIAN_POINT('Ctrl Pts',(0.185877920286694,1.83666577631576,11.0431439745677));
#41200=CARTESIAN_POINT('Ctrl Pts',(0.181059318987063,1.83332973372031,11.0427923298735));
#41201=CARTESIAN_POINT('Ctrl Pts',(0.175324772006733,1.82958665453525,11.0423754421814));
#41202=CARTESIAN_POINT('Ctrl Pts',(0.174494388865769,1.82905007601985,11.0423151144478));
#41203=CARTESIAN_POINT('Ctrl Pts',(0.17323913449647,1.82824711710714,11.0422239731899));
#41204=CARTESIAN_POINT('Ctrl Pts',(0.172816083772021,1.82797789011392,11.0421932655301));
#41205=CARTESIAN_POINT('Ctrl Pts',(0.172060362746374,1.82749942817451,11.042138426083));
#41206=CARTESIAN_POINT('Ctrl Pts',(0.171727934110242,1.82728981185572,11.0421143084859));
#41207=CARTESIAN_POINT('Ctrl Pts',(0.171033590667704,1.82685375941754,11.0420639447801));
#41208=CARTESIAN_POINT('Ctrl Pts',(0.170671607888851,1.82662743345599,11.0420376946634));
#41209=CARTESIAN_POINT('Ctrl Pts',(0.169722914018998,1.82603689123126,11.0419689128574));
#41210=CARTESIAN_POINT('Ctrl Pts',(0.169135482410123,1.8256738417734,11.0419263382903));
#41211=CARTESIAN_POINT('Ctrl Pts',(0.16784948556733,1.82488475993528,11.0418331656254));
#41212=CARTESIAN_POINT('Ctrl Pts',(0.167150457094497,1.82445949518378,11.0417825396755));
#41213=CARTESIAN_POINT('Ctrl Pts',(0.165099279114955,1.82322230727891,11.041634040344));
#41214=CARTESIAN_POINT('Ctrl Pts',(0.16374279454102,1.82241765141529,11.0415359027395));
#41215=CARTESIAN_POINT('Ctrl Pts',(0.159070777691876,1.81969241076672,11.0411980978001));
#41216=CARTESIAN_POINT('Ctrl Pts',(0.155727032314647,1.81782107401212,11.0409566725901));
#41217=CARTESIAN_POINT('Ctrl Pts',(0.145708991078284,1.81244674342985,11.0402341163603));
#41218=CARTESIAN_POINT('Ctrl Pts',(0.138944662149605,1.80911797607926,11.0397471622313));
#41219=CARTESIAN_POINT('Ctrl Pts',(0.100930842397006,1.79203974173737,11.0370166351006));
#41220=CARTESIAN_POINT('Ctrl Pts',(0.0677721683802175,1.78308830305369,
11.0346271685664));
#41221=CARTESIAN_POINT('Ctrl Pts',(0.0302654281520986,1.77912926837845,
11.0322030515938));
#41222=CARTESIAN_POINT('Ctrl Pts',(0.0266947533513148,1.77881249191683,
11.031975301615));
#41223=CARTESIAN_POINT('Ctrl Pts',(0.0225460814464715,1.7785141057799,11.0317147648449));
#41224=CARTESIAN_POINT('Ctrl Pts',(0.0219726903407202,1.77847440714246,
11.0316788461748));
#41225=CARTESIAN_POINT('Ctrl Pts',(0.0211196163049158,1.77841763739252,
11.0316255448654));
#41226=CARTESIAN_POINT('Ctrl Pts',(0.0208400163266329,1.7783993969937,11.0316080969997));
#41227=CARTESIAN_POINT('Ctrl Pts',(0.0203418600286957,1.77836755091128,
11.0315770501018));
#41228=CARTESIAN_POINT('Ctrl Pts',(0.0201233137717307,1.77835380334885,
11.0315634430796));
#41229=CARTESIAN_POINT('Ctrl Pts',(0.0196591910234741,1.7783250827866,11.0315345750139));
#41230=CARTESIAN_POINT('Ctrl Pts',(0.0194136120554594,1.77831016829269,
11.031519317339));
#41231=CARTESIAN_POINT('Ctrl Pts',(0.0187543718336034,1.77827088899131,
11.0314784045715));
#41232=CARTESIAN_POINT('Ctrl Pts',(0.0183406785079819,1.77824704065116,
11.0314527785743));
#41233=CARTESIAN_POINT('Ctrl Pts',(0.0163568486976606,1.77813651658437,
11.0313301166423));
#41234=CARTESIAN_POINT('Ctrl Pts',(0.0147861031163011,1.77806053387875,
11.0312336725858));
#41235=CARTESIAN_POINT('Ctrl Pts',(0.00171869788088448,1.77752425629725,
11.0304364904961));
#41236=CARTESIAN_POINT('Ctrl Pts',(-0.00979585634195999,1.77766839654384,
11.0297671310321));
#41237=CARTESIAN_POINT('Ctrl Pts',(-0.0245016404735278,1.77864151713911,
11.0289271936185));
#41238=CARTESIAN_POINT('Ctrl Pts',(-0.0277206975157908,1.77890317892308,
11.0287442636428));
#41239=CARTESIAN_POINT('Ctrl Pts',(-0.0335646388919616,1.7794667439872,
11.0284130544401));
#41240=CARTESIAN_POINT('Ctrl Pts',(-0.0361907565463395,1.7797526228393,
11.0282645440845));
#41241=CARTESIAN_POINT('Ctrl Pts',(-0.0410439982808445,1.78034140703195,
11.0279902596633));
#41242=CARTESIAN_POINT('Ctrl Pts',(-0.0432720300804582,1.78063538493908,
11.0278644086016));
#41243=CARTESIAN_POINT('Ctrl Pts',(-0.0648293316889683,1.78370950079021,
11.0266460526296));
#41244=CARTESIAN_POINT('Ctrl Pts',(-0.0838698940767816,1.78821754088196,
11.025561537711));
#41245=CARTESIAN_POINT('Ctrl Pts',(-0.104098591739613,1.79499520404949,
11.0243222163564));
#41246=CARTESIAN_POINT('Ctrl Pts',(-0.105807482652546,1.79558380659809,
11.0242168449933));
#41247=CARTESIAN_POINT('Ctrl Pts',(-0.109291999942323,1.79681688321899,
11.0240005220917));
#41248=CARTESIAN_POINT('Ctrl Pts',(-0.111067088979279,1.79746265503595,
11.0238895375877));
#41249=CARTESIAN_POINT('Ctrl Pts',(-0.119097215571865,1.80046418653697,
11.0233837073748));
#41250=CARTESIAN_POINT('Ctrl Pts',(-0.125283358621095,1.80299845029202,
11.0229835779295));
#41251=CARTESIAN_POINT('Ctrl Pts',(-0.132336707711849,1.80614756152015,
11.0225134808532));
#41252=CARTESIAN_POINT('Ctrl Pts',(-0.133285418125911,1.80657665893172,
11.0224499562903));
#41253=CARTESIAN_POINT('Ctrl Pts',(-0.134691306536387,1.80722076100732,
11.0223553757741));
#41254=CARTESIAN_POINT('Ctrl Pts',(-0.135150091809499,1.80743225823597,
11.0223244406983));
#41255=CARTESIAN_POINT('Ctrl Pts',(-0.135965301887799,1.80781039184513,
11.0222693462241));
#41256=CARTESIAN_POINT('Ctrl Pts',(-0.136321923188993,1.80797660421292,
11.0222452015121));
#41257=CARTESIAN_POINT('Ctrl Pts',(-0.137010098445047,1.80829888098698,
11.0221985255289));
#41258=CARTESIAN_POINT('Ctrl Pts',(-0.13734169251422,1.80845485871835,11.0221759972878));
#41259=CARTESIAN_POINT('Ctrl Pts',(-0.138241775466249,1.80888012291063,
11.0221147436299));
#41260=CARTESIAN_POINT('Ctrl Pts',(-0.138809740948873,1.80915050777191,
11.0220759801544));
#41261=CARTESIAN_POINT('Ctrl Pts',(-0.141003111879503,1.81020256897181,
11.0219258485607));
#41262=CARTESIAN_POINT('Ctrl Pts',(-0.142622711880395,1.81099621034718,
11.021814064774));
#41263=CARTESIAN_POINT('Ctrl Pts',(-0.146634782764315,1.81300415627534,
11.0215348055511));
#41264=CARTESIAN_POINT('Ctrl Pts',(-0.149018877871526,1.81423480413325,
11.0213667623699));
#41265=CARTESIAN_POINT('Ctrl Pts',(-0.158327768679603,1.8191881364948,11.0207021861747));
#41266=CARTESIAN_POINT('Ctrl Pts',(-0.165130277988696,1.82313367952103,
11.0201978958739));
#41267=CARTESIAN_POINT('Ctrl Pts',(-0.177771575930151,1.83109747659912,
11.0192244968837));
#41268=CARTESIAN_POINT('Ctrl Pts',(-0.183635541835949,1.83506740854312,
11.0187571505113));
#41269=CARTESIAN_POINT('Ctrl Pts',(-0.211803155702295,1.85552169293917,
11.0164367826161));
#41270=CARTESIAN_POINT('Ctrl Pts',(-0.232044528409271,1.87464356862274,
11.0145160745419));
#41271=CARTESIAN_POINT('Ctrl Pts',(-0.252350114430097,1.8995014730939,11.0124423923362));
#41272=CARTESIAN_POINT('Ctrl Pts',(-0.255043477133289,1.9029389206495,11.0121639983922));
#41273=CARTESIAN_POINT('Ctrl Pts',(-0.258027329705992,1.90691081327303,
11.011852690093));
#41274=CARTESIAN_POINT('Ctrl Pts',(-0.258387009880774,1.9073923935957,11.0118151149746));
#41275=CARTESIAN_POINT('Ctrl Pts',(-0.258916184969184,1.90810506283431,
11.0117597634147));
#41276=CARTESIAN_POINT('Ctrl Pts',(-0.259086719712887,1.9083353725416,11.0117419147737));
#41277=CARTESIAN_POINT('Ctrl Pts',(-0.259387899072206,1.90874325622439,
11.0117103738938));
#41278=CARTESIAN_POINT('Ctrl Pts',(-0.25951866883508,1.90892073699119,11.0116966728617));
#41279=CARTESIAN_POINT('Ctrl Pts',(-0.259791507792974,1.90929183087134,
11.0116680740764));
#41280=CARTESIAN_POINT('Ctrl Pts',(-0.259933542396538,1.90948546818722,
11.0116531787552));
#41281=CARTESIAN_POINT('Ctrl Pts',(-0.260304551421007,1.90999245606685,
11.0116142508483));
#41282=CARTESIAN_POINT('Ctrl Pts',(-0.260533177362328,1.91030606298766,
11.011590242614));
#41283=CARTESIAN_POINT('Ctrl Pts',(-0.26153023281012,1.91167892985865,11.0114854504282));
#41284=CARTESIAN_POINT('Ctrl Pts',(-0.262292786927755,1.9127424709231,11.0114050690028));
#41285=CARTESIAN_POINT('Ctrl Pts',(-0.267883344341346,1.92064082668769,
11.0108137674166));
#41286=CARTESIAN_POINT('Ctrl Pts',(-0.272450451507057,1.92765738291489,
11.0103195579266));
#41287=CARTESIAN_POINT('Ctrl Pts',(-0.2912016926338,1.95907752358079,11.0082024002778));
#41288=CARTESIAN_POINT('Ctrl Pts',(-0.302418854024023,1.985105968262,11.0066814454124));
#41289=CARTESIAN_POINT('Ctrl Pts',(-0.310711320300946,2.01441583205885,
11.0049312656844));
#41290=CARTESIAN_POINT('Ctrl Pts',(-0.311297573753096,2.01657341751796,
11.0048022975496));
#41291=CARTESIAN_POINT('Ctrl Pts',(-0.312508079197259,2.02121894326585,
11.0045241528572));
#41292=CARTESIAN_POINT('Ctrl Pts',(-0.313125170536016,2.02370857468679,
11.0043748069752));
#41293=CARTESIAN_POINT('Ctrl Pts',(-0.314135560411626,2.02800389326498,
11.0041164630363));
#41294=CARTESIAN_POINT('Ctrl Pts',(-0.314543170787361,2.02980610266152,
11.0040078640121));
#41295=CARTESIAN_POINT('Ctrl Pts',(-0.316343626074911,2.03809738625001,
11.0035071287701));
#41296=CARTESIAN_POINT('Ctrl Pts',(-0.317551230152649,2.04462464494493,
11.0031097627783));
#41297=CARTESIAN_POINT('Ctrl Pts',(-0.31871381437623,2.0522112997722,11.0026426526187));
#41298=CARTESIAN_POINT('Ctrl Pts',(-0.318866238879339,2.05323915091653,
11.002579258297));
#41299=CARTESIAN_POINT('Ctrl Pts',(-0.319085316794538,2.05476736777779,
11.0024848345324));
#41300=CARTESIAN_POINT('Ctrl Pts',(-0.319155770787228,2.05526718899678,
11.0024539253791));
#41301=CARTESIAN_POINT('Ctrl Pts',(-0.319279044924097,2.05615684931865,
11.0023988600579));
#41302=CARTESIAN_POINT('Ctrl Pts',(-0.319332326163335,2.05654662436303,
11.0023747185198));
#41303=CARTESIAN_POINT('Ctrl Pts',(-0.319433861995732,2.057299675252,11.0023280444873));
#41304=CARTESIAN_POINT('Ctrl Pts',(-0.319482210925086,2.05766293794149,
11.0023055150149));
#41305=CARTESIAN_POINT('Ctrl Pts',(-0.319585361997866,2.05844818778289,
11.0022567823775));
#41306=CARTESIAN_POINT('Ctrl Pts',(-0.319639948113751,2.05887020217776,
11.0022305724271));
#41307=CARTESIAN_POINT('Ctrl Pts',(-0.319770202014971,2.05989313822431,
11.0021669928502));
#41308=CARTESIAN_POINT('Ctrl Pts',(-0.319845011704316,2.06049416577215,
11.0021295961878));
#41309=CARTESIAN_POINT('Ctrl Pts',(-0.320043362362268,2.06212523167554,
11.0020279980808));
#41310=CARTESIAN_POINT('Ctrl Pts',(-0.320163623885117,2.06315565486961,
11.0019636933928));
#41311=CARTESIAN_POINT('Ctrl Pts',(-0.321617301848811,2.07615589485294,
11.0011508482936));
#41312=CARTESIAN_POINT('Ctrl Pts',(-0.322283506226235,2.08818906550373,
11.0003813438037));
#41313=CARTESIAN_POINT('Ctrl Pts',(-0.32227491802331,2.10022986532739,10.9995935809957));
#41314=CARTESIAN_POINT('',(-0.322274874088783,2.09970506445917,10.749346402247));
#41315=CARTESIAN_POINT('Ctrl Pts',(-0.322274918312996,2.1002294588239,10.9995936075909));
#41316=CARTESIAN_POINT('Ctrl Pts',(-0.322254316620498,2.12916453594962,
10.9977005467693));
#41317=CARTESIAN_POINT('Ctrl Pts',(-0.318337387949409,2.15796166008248,
10.9957002776856));
#41318=CARTESIAN_POINT('Ctrl Pts',(-0.3089462136507,2.19194228602188,10.9933681639819));
#41319=CARTESIAN_POINT('Ctrl Pts',(-0.307082988721927,2.19798569347298,
10.9929552751647));
#41320=CARTESIAN_POINT('Ctrl Pts',(-0.3040875609404,2.20677407166114,10.9923613634342));
#41321=CARTESIAN_POINT('Ctrl Pts',(-0.303093442514989,2.20956419913827,
10.9921737956288));
#41322=CARTESIAN_POINT('Ctrl Pts',(-0.301885355354942,2.21281250649253,
10.9919569134209));
#41323=CARTESIAN_POINT('Ctrl Pts',(-0.301708643818288,2.2132842603914,10.9919254524363));
#41324=CARTESIAN_POINT('Ctrl Pts',(-0.301437080941571,2.21400408936757,
10.9918775061136));
#41325=CARTESIAN_POINT('Ctrl Pts',(-0.301343028918333,2.21425246204196,
10.9918609732035));
#41326=CARTESIAN_POINT('Ctrl Pts',(-0.301178787374538,2.21468457763812,
10.9918322284167));
#41327=CARTESIAN_POINT('Ctrl Pts',(-0.301108736863945,2.21486837204954,
10.9918200082126));
#41328=CARTESIAN_POINT('Ctrl Pts',(-0.300949785464969,2.21528427486162,
10.9917923690978));
#41329=CARTESIAN_POINT('Ctrl Pts',(-0.300860784485301,2.2155163441322,10.9917769563335));
#41330=CARTESIAN_POINT('Ctrl Pts',(-0.300618636409769,2.21614556491955,
10.9917351923026));
#41331=CARTESIAN_POINT('Ctrl Pts',(-0.300464970138649,2.21654251812908,
10.991708872271));
#41332=CARTESIAN_POINT('Ctrl Pts',(-0.299768965779487,2.21832992120043,
10.9915904769586));
#41333=CARTESIAN_POINT('Ctrl Pts',(-0.299217748024084,2.21971692681167,
10.991498927462));
#41334=CARTESIAN_POINT('Ctrl Pts',(-0.286543749729241,2.25097352823701,
10.9894420916439));
#41335=CARTESIAN_POINT('Ctrl Pts',(-0.270014895549163,2.27886618433466,
10.9877223439953));
#41336=CARTESIAN_POINT('Ctrl Pts',(-0.24636705480681,2.30782408624367,10.9856019524841));
#41337=CARTESIAN_POINT('Ctrl Pts',(-0.243022451321976,2.31172543971965,
10.9853085200821));
#41338=CARTESIAN_POINT('Ctrl Pts',(-0.234031854218152,2.32171881209846,
10.984533264499));
#41339=CARTESIAN_POINT('Ctrl Pts',(-0.228241429859492,2.32767514960056,
10.9840470198535));
#41340=CARTESIAN_POINT('Ctrl Pts',(-0.220203271341155,2.33532851329367,
10.9833839950791));
#41341=CARTESIAN_POINT('Ctrl Pts',(-0.218153818122197,2.33722963723058,
10.9832159359588));
#41342=CARTESIAN_POINT('Ctrl Pts',(-0.214699020833591,2.34035176385765,
10.9829340984594));
#41343=CARTESIAN_POINT('Ctrl Pts',(-0.213307339321934,2.34158770395463,
10.9828209521063));
#41344=CARTESIAN_POINT('Ctrl Pts',(-0.211424555353486,2.34323083632394,
10.9826683581312));
#41345=CARTESIAN_POINT('Ctrl Pts',(-0.210942817587459,2.34364874316177,
10.9826293564194));
#41346=CARTESIAN_POINT('Ctrl Pts',(-0.210182117332645,2.34430470250415,
10.9825678338617));
#41347=CARTESIAN_POINT('Ctrl Pts',(-0.209903981748576,2.34454371502128,
10.9825453527292));
#41348=CARTESIAN_POINT('Ctrl Pts',(-0.209327089228582,2.34503775144521,
10.9824987511044));
#41349=CARTESIAN_POINT('Ctrl Pts',(-0.209028272924962,2.34529270481218,
10.9824746277635));
#41350=CARTESIAN_POINT('Ctrl Pts',(-0.20834822011093,2.34587078833507,10.9824197613047));
#41351=CARTESIAN_POINT('Ctrl Pts',(-0.2079666972623,2.34619357872461,10.9823890043224));
#41352=CARTESIAN_POINT('Ctrl Pts',(-0.206834232999903,2.34714719813158,
10.9822977795223));
#41353=CARTESIAN_POINT('Ctrl Pts',(-0.206081166134593,2.34777548388713,
10.9822372080432));
#41354=CARTESIAN_POINT('Ctrl Pts',(-0.200924954385384,2.35203755761678,
10.9818230803444));
#41355=CARTESIAN_POINT('Ctrl Pts',(-0.196429034515186,2.35555702966356,
10.9814649377996));
#41356=CARTESIAN_POINT('Ctrl Pts',(-0.190873433857037,2.35967279716054,
10.981025498682));
#41357=CARTESIAN_POINT('Ctrl Pts',(-0.189900617704411,2.36038506998423,
10.9809486642239));
#41358=CARTESIAN_POINT('Ctrl Pts',(-0.186218527130038,2.36304939925105,
10.9806582703352));
#41359=CARTESIAN_POINT('Ctrl Pts',(-0.183483036271274,2.36496471541736,
10.9804433860462));
#41360=CARTESIAN_POINT('Ctrl Pts',(-0.167480955484765,2.3758022991545,10.9791912758487));
#41361=CARTESIAN_POINT('Ctrl Pts',(-0.153596232881644,2.38376904641042,
10.9781225019774));
#41362=CARTESIAN_POINT('Ctrl Pts',(-0.127084837253748,2.39646320816438,
10.976136632348));
#41363=CARTESIAN_POINT('Ctrl Pts',(-0.114640459262448,2.40149389703811,
10.9752251475055));
#41364=CARTESIAN_POINT('Ctrl Pts',(-0.0923493499580106,2.40892478214824,
10.9736590598583));
#41365=CARTESIAN_POINT('Ctrl Pts',(-0.0826344512289054,2.41166410603651,
10.9729978027781));
#41366=CARTESIAN_POINT('Ctrl Pts',(-0.0713828064349738,2.41427345614789,
10.9722677230855));
#41367=CARTESIAN_POINT('Ctrl Pts',(-0.0699572672683585,2.41459385124713,
10.9721758755418));
#41368=CARTESIAN_POINT('Ctrl Pts',(-0.0681349771411878,2.41499041825054,
10.9720593378102));
#41369=CARTESIAN_POINT('Ctrl Pts',(-0.0677402239639423,2.41507554770442,
10.9720341449901));
#41370=CARTESIAN_POINT('Ctrl Pts',(-0.0671070212604436,2.41521085434428,
10.9719938192418));
#41371=CARTESIAN_POINT('Ctrl Pts',(-0.0668686746399742,2.41526150312358,
10.9719786592792));
#41372=CARTESIAN_POINT('Ctrl Pts',(-0.0664155347493087,2.41535725858015,
10.9719498743019));
#41373=CARTESIAN_POINT('Ctrl Pts',(-0.0662007546369079,2.4154024157818,
10.9719362465048));
#41374=CARTESIAN_POINT('Ctrl Pts',(-0.0657121539662772,2.41550462227561,
10.9719052804098));
#41375=CARTESIAN_POINT('Ctrl Pts',(-0.0654383055761518,2.4155615344444,
10.9718879500929));
#41376=CARTESIAN_POINT('Ctrl Pts',(-0.0645890026122627,2.41573688656978,
10.9718342802672));
#41377=CARTESIAN_POINT('Ctrl Pts',(-0.064013293893507,2.41585411033732,
10.9717980102496));
#41378=CARTESIAN_POINT('Ctrl Pts',(-0.0596521447409737,2.41672969844215,
10.9715240700566));
#41379=CARTESIAN_POINT('Ctrl Pts',(-0.0558534718073047,2.41742160158631,
10.9712901062092));
#41380=CARTESIAN_POINT('Ctrl Pts',(-0.022133890849511,2.4229392807607,10.9692469362343));
#41381=CARTESIAN_POINT('Ctrl Pts',(0.00832014880910999,2.42359083319733,
10.9676232160316));
#41382=CARTESIAN_POINT('Ctrl Pts',(0.0497949703326796,2.41861087059711,
10.9652492598846));
#41383=CARTESIAN_POINT('Ctrl Pts',(0.0610878232946712,2.41663964773347,
10.9645874688396));
#41384=CARTESIAN_POINT('Ctrl Pts',(0.0757319884901491,2.41327080868357,
10.9636950022801));
#41385=CARTESIAN_POINT('Ctrl Pts',(0.0791992448934196,2.41241224648511,
10.9634811622914));
#41386=CARTESIAN_POINT('Ctrl Pts',(0.0840984811542229,2.41111229888031,
10.9631750862183));
#41387=CARTESIAN_POINT('Ctrl Pts',(0.0855428338205187,2.41071826549557,
10.9630843645337));
#41388=CARTESIAN_POINT('Ctrl Pts',(0.0877428747093789,2.41010157061525,
10.9629454121138));
#41389=CARTESIAN_POINT('Ctrl Pts',(0.0885005919638206,2.4098861748532,10.9628974164195));
#41390=CARTESIAN_POINT('Ctrl Pts',(0.0898781615628398,2.40948910952578,
10.9628099012137));
#41391=CARTESIAN_POINT('Ctrl Pts',(0.0904982736319636,2.40930834987281,
10.9627704114327));
#41392=CARTESIAN_POINT('Ctrl Pts',(0.0915278360996699,2.40900487625663,
10.9627046878403));
#41393=CARTESIAN_POINT('Ctrl Pts',(0.0919375952288033,2.4088832091782,10.962678488258));
#41394=CARTESIAN_POINT('Ctrl Pts',(0.0927235219460625,2.40864814670382,
10.9626281557183));
#41395=CARTESIAN_POINT('Ctrl Pts',(0.0930997268350522,2.40853487784504,
10.9626040269384));
#41396=CARTESIAN_POINT('Ctrl Pts',(0.0939547066874318,2.40827575191144,
10.9625491090141));
#41397=CARTESIAN_POINT('Ctrl Pts',(0.0944333500400041,2.40812946714165,
10.9625183059064));
#41398=CARTESIAN_POINT('Ctrl Pts',(0.0958522123211437,2.40769221260033,
10.9624268204824));
#41399=CARTESIAN_POINT('Ctrl Pts',(0.0967914348802043,2.40739805204516,
10.9623660336209));
#41400=CARTESIAN_POINT('Ctrl Pts',(0.103231934263653,2.40534847132313,10.9619476182942));
#41401=CARTESIAN_POINT('Ctrl Pts',(0.108686211086973,2.40344986693634,10.9615852953156));
#41402=CARTESIAN_POINT('Ctrl Pts',(0.115180196672241,2.40099180393797,10.9611438379382));
#41403=CARTESIAN_POINT('Ctrl Pts',(0.116271846229873,2.40057179086019,10.9610692824062));
#41404=CARTESIAN_POINT('Ctrl Pts',(0.143171311263054,2.39005372836305,10.9592235711181));
#41405=CARTESIAN_POINT('Ctrl Pts',(0.16756828748977,2.37667583573062,10.9573390505891));
#41406=CARTESIAN_POINT('Ctrl Pts',(0.202882739244931,2.35091059781883,10.9543912104484));
#41407=CARTESIAN_POINT('Ctrl Pts',(0.215097910206543,2.34052144286568,10.9533245559022));
#41408=CARTESIAN_POINT('Ctrl Pts',(0.227027262906564,2.32873645301858,10.9522719553081));
#41409=CARTESIAN_POINT('Ctrl Pts',(0.227561287297254,2.32820517871654,10.9522248124474));
#41410=CARTESIAN_POINT('Ctrl Pts',(0.228314563999211,2.3274505077033,10.9521582888395));
#41411=CARTESIAN_POINT('Ctrl Pts',(0.228535355924007,2.32722866166774,10.952138787075));
#41412=CARTESIAN_POINT('Ctrl Pts',(0.228913682197164,2.32684741997869,10.9521053660784));
#41413=CARTESIAN_POINT('Ctrl Pts',(0.229071373813674,2.32668818131585,10.9520914343164));
#41414=CARTESIAN_POINT('Ctrl Pts',(0.229372836325212,2.32638312550459,10.9520647981472));
#41415=CARTESIAN_POINT('Ctrl Pts',(0.22951663414784,2.32623733601492,10.9520520915594));
#41416=CARTESIAN_POINT('Ctrl Pts',(0.22985478371803,2.32589384870671,10.9520222083011));
#41417=CARTESIAN_POINT('Ctrl Pts',(0.230049019887142,2.3256960365888,10.9520050408094));
#41418=CARTESIAN_POINT('Ctrl Pts',(0.230621243873135,2.32511177161235,10.9519544573711));
#41419=CARTESIAN_POINT('Ctrl Pts',(0.230998517266899,2.32472461563995,10.9519210973174));
#41420=CARTESIAN_POINT('Ctrl Pts',(0.234267124511223,2.32135345947039,10.9516319681619));
#41421=CARTESIAN_POINT('Ctrl Pts',(0.23710163858998,2.31831458173548,10.9513805170775));
#41422=CARTESIAN_POINT('Ctrl Pts',(0.240112276858187,2.31495905310643,10.9511115257517));
#41423=CARTESIAN_POINT('Ctrl Pts',(0.240347375534513,2.31469615526651,10.9510905074132));
#41424=CARTESIAN_POINT('Ctrl Pts',(0.240667576049242,2.31433690766734,10.9510618621699));
#41425=CARTESIAN_POINT('Ctrl Pts',(0.240753051632117,2.31424089310806,10.9510542136806));
#41426=CARTESIAN_POINT('Ctrl Pts',(0.26291036367739,2.28932162143064,10.949071063481));
#41427=CARTESIAN_POINT('Ctrl Pts',(0.281014620332351,2.26123268985443,10.94730844595));
#41428=CARTESIAN_POINT('Ctrl Pts',(0.298453417663256,2.22198838381815,10.9448383265381));
#41429=CARTESIAN_POINT('Ctrl Pts',(0.301995551289514,2.21293480116184,10.9442697073108));
#41430=CARTESIAN_POINT('Ctrl Pts',(0.305893015935163,2.20147097981928,10.9435440885228));
#41431=CARTESIAN_POINT('Ctrl Pts',(0.306637690292235,2.19919790002815,10.9433999543898));
#41432=CARTESIAN_POINT('Ctrl Pts',(0.307691347324556,2.19585638559832,10.943187609609));
#41433=CARTESIAN_POINT('Ctrl Pts',(0.308020223203044,2.19479427160036,10.943120047172));
#41434=CARTESIAN_POINT('Ctrl Pts',(0.308601785342841,2.19288111649883,10.9429982177161));
#41435=CARTESIAN_POINT('Ctrl Pts',(0.308856464905853,2.19203068933758,10.942944016205));
#41436=CARTESIAN_POINT('Ctrl Pts',(0.309240909085793,2.19072738121578,10.9428608758231));
#41437=CARTESIAN_POINT('Ctrl Pts',(0.309373201238093,2.19027524525831,10.9428320195204));
#41438=CARTESIAN_POINT('Ctrl Pts',(0.309612821181782,2.18944958148121,10.9427792981806));
#41439=CARTESIAN_POINT('Ctrl Pts',(0.309720465742506,2.18907614588346,10.9427554435234));
#41440=CARTESIAN_POINT('Ctrl Pts',(0.309950777308237,2.18827169474433,10.9427040350708));
#41441=CARTESIAN_POINT('Ctrl Pts',(0.310073221206371,2.18784061665591,10.9426764740658));
#41442=CARTESIAN_POINT('Ctrl Pts',(0.310398684274769,2.18668562564395,10.94260259423));
#41443=CARTESIAN_POINT('Ctrl Pts',(0.310600069066699,2.18596125856009,10.9425562223569));
#41444=CARTESIAN_POINT('Ctrl Pts',(0.311499074570377,2.18268319194556,10.9423461965308));
#41445=CARTESIAN_POINT('Ctrl Pts',(0.312167732363441,2.18012171919535,10.9421816062565));
#41446=CARTESIAN_POINT('Ctrl Pts',(0.312960646702323,2.17692352681353,10.94197545816));
#41447=CARTESIAN_POINT('Ctrl Pts',(0.313114653077911,2.17629422900715,10.9419348642213));
#41448=CARTESIAN_POINT('Ctrl Pts',(0.313504607476084,2.17467973619252,10.9418306382932));
#41449=CARTESIAN_POINT('Ctrl Pts',(0.313737808262352,2.17369389076172,10.9417669190733));
#41450=CARTESIAN_POINT('Ctrl Pts',(0.31405875518752,2.17230796401215,10.9416772313852));
#41451=CARTESIAN_POINT('Ctrl Pts',(0.314150394484256,2.17190878258199,10.9416513863601));
#41452=CARTESIAN_POINT('Ctrl Pts',(0.314280578138682,2.17133670309884,10.9416143286759));
#41453=CARTESIAN_POINT('Ctrl Pts',(0.3143197415451,2.17116394507767,10.9416031355049));
#41454=CARTESIAN_POINT('Ctrl Pts',(0.321651449884091,2.13869811527477,10.9394991892384));
#41455=CARTESIAN_POINT('Ctrl Pts',(0.323923122566275,2.10547854432306,10.9372318975712));
#41456=CARTESIAN_POINT('Ctrl Pts',(0.320074875582644,2.06053197107727,10.9342072271989));
#41457=CARTESIAN_POINT('Ctrl Pts',(0.318380185112872,2.04862124594854,10.9334134189066));
#41458=CARTESIAN_POINT('Ctrl Pts',(0.315708264437853,2.03525390527992,10.932550648803));
#41459=CARTESIAN_POINT('Ctrl Pts',(0.31538103641162,2.03367830563291,10.9324494087023));
#41460=CARTESIAN_POINT('Ctrl Pts',(0.314954016971755,2.0316968721015,10.9323227214565));
#41461=CARTESIAN_POINT('Ctrl Pts',(0.314865227085134,2.03128872825598,10.9322966596325));
#41462=CARTESIAN_POINT('Ctrl Pts',(0.314722717788588,2.03063972730411,10.9322552729572));
#41463=CARTESIAN_POINT('Ctrl Pts',(0.314669515175312,2.03039875905561,10.932239918519));
#41464=CARTESIAN_POINT('Ctrl Pts',(0.314568608398194,2.02994420703047,10.9322109776543));
#41465=CARTESIAN_POINT('Ctrl Pts',(0.314520963842863,2.02973061248421,10.9321973879688));
#41466=CARTESIAN_POINT('Ctrl Pts',(0.314412091095358,2.0292448558908,10.9321665041076));
#41467=CARTESIAN_POINT('Ctrl Pts',(0.314350727184671,2.0289727252054,10.9321492178825));
#41468=CARTESIAN_POINT('Ctrl Pts',(0.314163213885511,2.0281461624335,10.9320967594241));
#41469=CARTESIAN_POINT('Ctrl Pts',(0.314035949611341,2.02759198044919,10.9320616511268));
#41470=CARTESIAN_POINT('Ctrl Pts',(0.313123686387054,2.02366710813565,10.9318134344212));
#41471=CARTESIAN_POINT('Ctrl Pts',(0.312285865082099,2.02030875721253,10.9316032953075));
#41472=CARTESIAN_POINT('Ctrl Pts',(0.30412240492641,1.98969474568462,10.9297029302322));
#41473=CARTESIAN_POINT('Ctrl Pts',(0.293299188776839,1.96349445808206,10.9281790672865));
#41474=CARTESIAN_POINT('Ctrl Pts',(0.27064135323254,1.92419331536507,10.9256178589639));
#41475=CARTESIAN_POINT('Ctrl Pts',(0.26091500242289,1.91005796651308,10.9246307799976));
#41476=CARTESIAN_POINT('Ctrl Pts',(0.249032498569792,1.89543479785534,10.9234951732656));
#41477=CARTESIAN_POINT('Ctrl Pts',(0.247942173707335,1.89411462996041,10.9233915672007));
#41478=CARTESIAN_POINT('Ctrl Pts',(0.246282758382411,1.89213770531581,10.9232347427594));
#41479=CARTESIAN_POINT('Ctrl Pts',(0.24572143520289,1.89147444548307,10.9231818397407));
#41480=CARTESIAN_POINT('Ctrl Pts',(0.24480964222259,1.89040586409597,10.9230961358285));
#41481=CARTESIAN_POINT('Ctrl Pts',(0.244460829260343,1.88999912932942,10.9230634029898));
#41482=CARTESIAN_POINT('Ctrl Pts',(0.243790300620451,1.88922119119517,10.923000581946));
#41483=CARTESIAN_POINT('Ctrl Pts',(0.243468747166803,1.88884984947532,10.9229705004899));
#41484=CARTESIAN_POINT('Ctrl Pts',(0.242893253357124,1.88818831052414,10.9229167413469));
#41485=CARTESIAN_POINT('Ctrl Pts',(0.242639638238097,1.88789783056598,10.9228930772035));
#41486=CARTESIAN_POINT('Ctrl Pts',(0.242135290452497,1.88732226048309,10.9228460710658));
#41487=CARTESIAN_POINT('Ctrl Pts',(0.241884574095973,1.88703715680657,10.9228227297723));
#41488=CARTESIAN_POINT('Ctrl Pts',(0.241274795363934,1.88634620906036,10.9227660227479));
#41489=CARTESIAN_POINT('Ctrl Pts',(0.240915212987752,1.88594082732541,10.9227326352689));
#41490=CARTESIAN_POINT('Ctrl Pts',(0.23956552476436,1.88442694030493,10.9226075090879));
#41491=CARTESIAN_POINT('Ctrl Pts',(0.238568788506461,1.88332439511175,10.9225154915827));
#41492=CARTESIAN_POINT('Ctrl Pts',(0.220630299820272,1.86375547317653,10.9208661447417));
#41493=CARTESIAN_POINT('Ctrl Pts',(0.201602972975033,1.84732444533936,10.9192123540315));
#41494=CARTESIAN_POINT('Ctrl Pts',(0.16777896148828,1.82438874823419,10.916452550539));
#41495=CARTESIAN_POINT('Ctrl Pts',(0.15405209957324,1.81648752694927,10.9153756496069));
#41496=CARTESIAN_POINT('Ctrl Pts',(0.134071172587125,1.80686773202247,10.9139079826725));
#41497=CARTESIAN_POINT('Ctrl Pts',(0.128261309521345,1.80427943318373,10.9134925004579));
#41498=CARTESIAN_POINT('Ctrl Pts',(0.119566489977303,1.80071039373603,10.9128909615369));
#41499=CARTESIAN_POINT('Ctrl Pts',(0.116738381563927,1.79959599559338,10.912698398922));
#41500=CARTESIAN_POINT('Ctrl Pts',(0.113420286245595,1.79834245973328,10.9124764183916));
#41501=CARTESIAN_POINT('Ctrl Pts',(0.112945339238842,1.79816431078419,10.9124447380932));
#41502=CARTESIAN_POINT('Ctrl Pts',(0.112220391474482,1.79789433919556,10.9123965269131));
#41503=CARTESIAN_POINT('Ctrl Pts',(0.111970696998275,1.79780170488944,10.9123799476507));
#41504=CARTESIAN_POINT('Ctrl Pts',(0.111536325250548,1.79764116931983,10.9123511519816));
#41505=CARTESIAN_POINT('Ctrl Pts',(0.111351701107732,1.79757312784446,10.9123389271494));
#41506=CARTESIAN_POINT('Ctrl Pts',(0.110934228695462,1.79741970646472,10.9123113169187));
#41507=CARTESIAN_POINT('Ctrl Pts',(0.110701344600727,1.79733442640971,10.9122959375879));
#41508=CARTESIAN_POINT('Ctrl Pts',(0.110070780717832,1.79710434474412,10.9122543572663));
#41509=CARTESIAN_POINT('Ctrl Pts',(0.109672912008038,1.79696005689472,10.9122281870433));
#41510=CARTESIAN_POINT('Ctrl Pts',(0.107891537478405,1.79631800578265,10.9121113047588));
#41511=CARTESIAN_POINT('Ctrl Pts',(0.106504890900473,1.79582892004842,10.9120211022404));
#41512=CARTESIAN_POINT('Ctrl Pts',(0.0743400643474861,1.78473095328814,
10.9099457077039));
#41513=CARTESIAN_POINT('Ctrl Pts',(0.0421281686983365,1.77883479836709,
10.9082110626206));
#41514=CARTESIAN_POINT('Ctrl Pts',(-0.00711923318000085,1.77737109440469,
10.9054145130027));
#41515=CARTESIAN_POINT('Ctrl Pts',(-0.0238236530241909,1.77817332683375,
10.9044439802448));
#41516=CARTESIAN_POINT('Ctrl Pts',(-0.0416961499783715,1.7804310060269,
10.9033497841008));
#41517=CARTESIAN_POINT('Ctrl Pts',(-0.043001996829613,1.78060410300044,
10.9032695245635));
#41518=CARTESIAN_POINT('Ctrl Pts',(-0.044857634027944,1.78086166379507,
10.9031550172557));
#41519=CARTESIAN_POINT('Ctrl Pts',(-0.0454083356291735,1.78093955429183,
10.9031209773756));
#41520=CARTESIAN_POINT('Ctrl Pts',(-0.046356353356507,1.78107614477175,
10.9030622789614));
#41521=CARTESIAN_POINT('Ctrl Pts',(-0.0467537677345155,1.78113416280443,
10.9030376420575));
#41522=CARTESIAN_POINT('Ctrl Pts',(-0.0475126636617733,1.78124640233266,
10.9029905377392));
#41523=CARTESIAN_POINT('Ctrl Pts',(-0.0478741637130052,1.78130049626462,
10.9029680743997));
#41524=CARTESIAN_POINT('Ctrl Pts',(-0.04871808646623,1.78142824696226,10.9029155744689));
#41525=CARTESIAN_POINT('Ctrl Pts',(-0.0492004344679933,1.78150238458278,
10.9028855226772));
#41526=CARTESIAN_POINT('Ctrl Pts',(-0.0508566626605956,1.78176080152828,
10.9027821779457));
#41527=CARTESIAN_POINT('Ctrl Pts',(-0.0520296802832212,1.78195047572764,
10.9027087141035));
#41528=CARTESIAN_POINT('Ctrl Pts',(-0.0646036709469267,1.78405508309663,
10.9019182780645));
#41529=CARTESIAN_POINT('Ctrl Pts',(-0.0758934435529317,1.78657543915536,
10.9011820395239));
#41530=CARTESIAN_POINT('Ctrl Pts',(-0.106434539356613,1.79514047041579,
10.8991140943432));
#41531=CARTESIAN_POINT('Ctrl Pts',(-0.12529113690889,1.80239354146713,10.8977487760819));
#41532=CARTESIAN_POINT('Ctrl Pts',(-0.159478555645247,1.81937163159771,
10.8951675838473));
#41533=CARTESIAN_POINT('Ctrl Pts',(-0.174914761135057,1.82872397092471,
10.893956884432));
#41534=CARTESIAN_POINT('Ctrl Pts',(-0.190466743979409,1.84002874482821,
10.8927444072567));
#41535=CARTESIAN_POINT('Ctrl Pts',(-0.191439617028282,1.84074432075764,
10.8926685992253));
#41536=CARTESIAN_POINT('Ctrl Pts',(-0.192710679276106,1.84169027962395,
10.8925696334761));
#41537=CARTESIAN_POINT('Ctrl Pts',(-0.193012503042593,1.84191572845193,
10.8925461390678));
#41538=CARTESIAN_POINT('Ctrl Pts',(-0.193504043646303,1.84228423181158,
10.8925078872289));
#41539=CARTESIAN_POINT('Ctrl Pts',(-0.193693997730832,1.84242696700869,
10.8924931074868));
#41540=CARTESIAN_POINT('Ctrl Pts',(-0.194060625142903,1.84270309290592,
10.8924645865368));
#41541=CARTESIAN_POINT('Ctrl Pts',(-0.194237318433028,1.84283645522895,
10.8924508434548));
#41542=CARTESIAN_POINT('Ctrl Pts',(-0.194646996931876,1.84314633027963,
10.8924189841531));
#41543=CARTESIAN_POINT('Ctrl Pts',(-0.194879880320359,1.84332297860666,
10.8924008775076));
#41544=CARTESIAN_POINT('Ctrl Pts',(-0.195633331826957,1.84389610840547,
10.8923423082637));
#41545=CARTESIAN_POINT('Ctrl Pts',(-0.196152937086307,1.84429386182243,
10.8923019347568));
#41546=CARTESIAN_POINT('Ctrl Pts',(-0.201177682031358,1.8481645902218,10.8919116441347));
#41547=CARTESIAN_POINT('Ctrl Pts',(-0.205591674108126,1.85175494646884,
10.8915698359808));
#41548=CARTESIAN_POINT('Ctrl Pts',(-0.210099706711998,1.855624566939,10.8912191013189));
#41549=CARTESIAN_POINT('Ctrl Pts',(-0.210290602584344,1.855788817804,10.8912042460605));
#41550=CARTESIAN_POINT('Ctrl Pts',(-0.234795515099827,1.87692340327459,
10.8892968729428));
#41551=CARTESIAN_POINT('Ctrl Pts',(-0.255841720139801,1.90141089006542,
10.8875866634696));
#41552=CARTESIAN_POINT('Ctrl Pts',(-0.278955740211868,1.93821740473511,
10.8850841948291));
#41553=CARTESIAN_POINT('Ctrl Pts',(-0.284477639338235,1.94813709026265,
10.8844174875965));
#41554=CARTESIAN_POINT('Ctrl Pts',(-0.29035718954039,1.96015008023005,10.8836087549886));
#41555=CARTESIAN_POINT('Ctrl Pts',(-0.291232431988367,1.96198200174203,
10.883485405026));
#41556=CARTESIAN_POINT('Ctrl Pts',(-0.292369123367405,1.96442010930197,
10.8833211663119));
#41557=CARTESIAN_POINT('Ctrl Pts',(-0.292646115816498,1.96501903116504,
10.8832808153461));
#41558=CARTESIAN_POINT('Ctrl Pts',(-0.293097759542932,1.96600351446988,
10.8832144771566));
#41559=CARTESIAN_POINT('Ctrl Pts',(-0.293273495054448,1.96638857878403,
10.8831885273421));
#41560=CARTESIAN_POINT('Ctrl Pts',(-0.293612485267293,1.9671352509777,10.8831382026958));
#41561=CARTESIAN_POINT('Ctrl Pts',(-0.293775831879298,1.96749681649491,
10.8831138310801));
#41562=CARTESIAN_POINT('Ctrl Pts',(-0.294151348364753,1.96833212491591,
10.8830575199645));
#41563=CARTESIAN_POINT('Ctrl Pts',(-0.294363041740745,1.9688060796909,10.8830255641853));
#41564=CARTESIAN_POINT('Ctrl Pts',(-0.295037021186503,1.97032487839287,
10.8829231444916));
#41565=CARTESIAN_POINT('Ctrl Pts',(-0.295494892439676,1.9713716612771,10.8828525297723));
#41566=CARTESIAN_POINT('Ctrl Pts',(-0.299649797587623,1.98100985401166,
10.8822020801297));
#41567=CARTESIAN_POINT('Ctrl Pts',(-0.302976406617867,1.98975516428787,
10.88160973112));
#41568=CARTESIAN_POINT('Ctrl Pts',(-0.315418084558816,2.02730284350263,
10.8790539498074));
#41569=CARTESIAN_POINT('Ctrl Pts',(-0.32083960404873,2.05716510600591,10.876972307672));
#41570=CARTESIAN_POINT('Ctrl Pts',(-0.322193647604366,2.0915969622432,10.8746763502237));
#41571=CARTESIAN_POINT('Ctrl Pts',(-0.322276631350591,2.09586077190173,
10.8743942202839));
#41572=CARTESIAN_POINT('Ctrl Pts',(-0.322274825622189,2.10051169824796,
10.8740896644046));
#41573=CARTESIAN_POINT('Ctrl Pts',(-0.322273979979023,2.10089827381881,
10.8740643744063));
#41574=CARTESIAN_POINT('Ctrl Pts',(-0.322268744481638,2.10221146871072,
10.8739785481545));
#41575=CARTESIAN_POINT('Ctrl Pts',(-0.322261053749342,2.10313807832468,
10.8739181294848));
#41576=CARTESIAN_POINT('Ctrl Pts',(-0.32223793987718,2.1049705677535,10.8737989397274));
#41577=CARTESIAN_POINT('Ctrl Pts',(-0.322222693036883,2.10587644173465,
10.8737401624225));
#41578=CARTESIAN_POINT('Ctrl Pts',(-0.322200901706047,2.10691168030863,
10.873673163529));
#41579=CARTESIAN_POINT('Ctrl Pts',(-0.322198099238625,2.10704111013993,
10.8736647901252));
#41580=CARTESIAN_POINT('Ctrl Pts',(-0.322187161584062,2.10753257392999,
10.8736330068673));
#41581=CARTESIAN_POINT('Ctrl Pts',(-0.32217849415639,2.10789459720923,10.8736096188517));
#41582=CARTESIAN_POINT('Ctrl Pts',(-0.322063063684964,2.11239864417594,
10.8733189489061));
#41583=CARTESIAN_POINT('Ctrl Pts',(-0.321877034748086,2.11653849738668,
10.8730550180787));
#41584=CARTESIAN_POINT('Ctrl Pts',(-0.321576555715706,2.12121287806403,
10.8727615263765));
#41585=CARTESIAN_POINT('Ctrl Pts',(-0.321540550165263,2.12175182730689,
10.8727277552361));
#41586=CARTESIAN_POINT('Ctrl Pts',(-0.321484022016173,2.12256714445417,
10.8726767721292));
#41587=CARTESIAN_POINT('Ctrl Pts',(-0.321464497884594,2.12284357725347,
10.8726595047004));
#41588=CARTESIAN_POINT('Ctrl Pts',(-0.321429928709937,2.12332420363556,
10.8726295146196));
#41589=CARTESIAN_POINT('Ctrl Pts',(-0.32141504563002,2.12352840812515,10.8726167828399));
#41590=CARTESIAN_POINT('Ctrl Pts',(-0.321383462720451,2.1239561213365,10.8725901371635));
#41591=CARTESIAN_POINT('Ctrl Pts',(-0.321366724336315,2.12417962674193,
10.872576225528));
#41592=CARTESIAN_POINT('Ctrl Pts',(-0.321326042531581,2.12471534064146,
10.872542910239));
#41593=CARTESIAN_POINT('Ctrl Pts',(-0.321301877147555,2.12502753314797,
10.8725235191398));
#41594=CARTESIAN_POINT('Ctrl Pts',(-0.321217966831608,2.12609141650644,
10.8724575178563));
#41595=CARTESIAN_POINT('Ctrl Pts',(-0.321156038134715,2.12684293998963,
10.8724110297553));
#41596=CARTESIAN_POINT('Ctrl Pts',(-0.319379622969743,2.14751361592085,
10.8711359180619));
#41597=CARTESIAN_POINT('Ctrl Pts',(-0.315817567634234,2.16723409805002,
10.8700087077598));
#41598=CARTESIAN_POINT('Ctrl Pts',(-0.304441948982124,2.20806140802929,
10.8676358545664));
#41599=CARTESIAN_POINT('Ctrl Pts',(-0.296205064151348,2.2289365695121,10.8663957408124));
#41600=CARTESIAN_POINT('Ctrl Pts',(-0.28505537167474,2.25035870644512,10.8649801648288));
#41601=CARTESIAN_POINT('Ctrl Pts',(-0.284225684101026,2.25192124886153,
10.8648760763473));
#41602=CARTESIAN_POINT('Ctrl Pts',(-0.280309857622231,2.259151520405,10.8643903783157));
#41603=CARTESIAN_POINT('Ctrl Pts',(-0.277066956436572,2.26473225398132,
10.8640037869734));
#41604=CARTESIAN_POINT('Ctrl Pts',(-0.273114567388822,2.27108673484803,
10.8635483235887));
#41605=CARTESIAN_POINT('Ctrl Pts',(-0.272566059816848,2.27195924156083,
10.8634854448175));
#41606=CARTESIAN_POINT('Ctrl Pts',(-0.271743593836216,2.27325370967893,
10.8633916418055));
#41607=CARTESIAN_POINT('Ctrl Pts',(-0.271472813460144,2.27367769072633,
10.8633608355396));
#41608=CARTESIAN_POINT('Ctrl Pts',(-0.270988629768869,2.27443191440212,
10.8633058857192));
#41609=CARTESIAN_POINT('Ctrl Pts',(-0.270775612263447,2.27476240450159,
10.8632817565698));
#41610=CARTESIAN_POINT('Ctrl Pts',(-0.270325770988583,2.27545752250566,
10.8632308981058));
#41611=CARTESIAN_POINT('Ctrl Pts',(-0.270088813242093,2.27582206238958,
10.8632041638177));
#41612=CARTESIAN_POINT('Ctrl Pts',(-0.269462129081457,2.27678190770583,
10.8631336055275));
#41613=CARTESIAN_POINT('Ctrl Pts',(-0.26907116920142,2.27737640145416,10.8630897353578));
#41614=CARTESIAN_POINT('Ctrl Pts',(-0.267303381510711,2.28004520622942,
10.86289202697));
#41615=CARTESIAN_POINT('Ctrl Pts',(-0.265904543063711,2.28210477059075,
10.8627373613536));
#41616=CARTESIAN_POINT('Ctrl Pts',(-0.255415098375652,2.29717021427896,
10.861590199882));
#41617=CARTESIAN_POINT('Ctrl Pts',(-0.24540022877856,2.30950312357756,10.8605616978375));
#41618=CARTESIAN_POINT('Ctrl Pts',(-0.21267000601413,2.34422817888678,10.8573888244243));
#41619=CARTESIAN_POINT('Ctrl Pts',(-0.187505946093624,2.36404054256763,
10.8551661494065));
#41620=CARTESIAN_POINT('Ctrl Pts',(-0.158550648780054,2.38057992092367,
10.8530572512341));
#41621=CARTESIAN_POINT('Ctrl Pts',(-0.157250372257713,2.38131071946006,
10.8529634465478));
#41622=CARTESIAN_POINT('Ctrl Pts',(-0.155572626892992,2.38223840008126,
10.8528436067625));
#41623=CARTESIAN_POINT('Ctrl Pts',(-0.155199804278868,2.3824435828189,10.852817051861));
#41624=CARTESIAN_POINT('Ctrl Pts',(-0.154608606444273,2.38276742422637,
10.8527750635793));
#41625=CARTESIAN_POINT('Ctrl Pts',(-0.154390500164541,2.38288656887558,
10.852759599122));
#41626=CARTESIAN_POINT('Ctrl Pts',(-0.153999528060085,2.3830995578787,10.8527319247046));
#41627=CARTESIAN_POINT('Ctrl Pts',(-0.15382671539677,2.38319349558986,10.8527197087809));
#41628=CARTESIAN_POINT('Ctrl Pts',(-0.153420334544091,2.38341391483853,
10.8526910205767));
#41629=CARTESIAN_POINT('Ctrl Pts',(-0.153186696262187,2.38354026568587,
10.852674556756));
#41630=CARTESIAN_POINT('Ctrl Pts',(-0.152509362044669,2.38390548433638,
10.8526269122443));
#41631=CARTESIAN_POINT('Ctrl Pts',(-0.152065259194466,2.38414360190195,
10.8525957793959));
#41632=CARTESIAN_POINT('Ctrl Pts',(-0.149004317073925,2.38577557588487,
10.8523819141305));
#41633=CARTESIAN_POINT('Ctrl Pts',(-0.146368800705609,2.38713436221885,
10.8522013657055));
#41634=CARTESIAN_POINT('Ctrl Pts',(-0.138051505692683,2.39127820287519,
10.8516415861598));
#41635=CARTESIAN_POINT('Ctrl Pts',(-0.132305952769972,2.3939325697275,10.8512693190619));
#41636=CARTESIAN_POINT('Ctrl Pts',(-0.112118376941293,2.40254693496245,
10.8499982120266));
#41637=CARTESIAN_POINT('Ctrl Pts',(-0.0973234851078491,2.40762539220445,
10.8491298564629));
#41638=CARTESIAN_POINT('Ctrl Pts',(-0.0668949738773259,2.41565387959206,
10.8473703637616));
#41639=CARTESIAN_POINT('Ctrl Pts',(-0.0512956472830773,2.4185608467032,
10.8464811473232));
#41640=CARTESIAN_POINT('Ctrl Pts',(-0.0322804170163812,2.42067109467057,
10.8453688679589));
#41641=CARTESIAN_POINT('Ctrl Pts',(-0.0290087619299157,2.42098359302477,
10.8451765541134));
#41642=CARTESIAN_POINT('Ctrl Pts',(-0.0245484507849553,2.42134088020315,
10.8449127816755));
#41643=CARTESIAN_POINT('Ctrl Pts',(-0.023363421891669,2.42142921178927,
10.8448425499225));
#41644=CARTESIAN_POINT('Ctrl Pts',(-0.0164123305417085,2.42190870054511,
10.8444296412595));
#41645=CARTESIAN_POINT('Ctrl Pts',(-0.0106373668911117,2.42215123167219,
10.8440827533912));
#41646=CARTESIAN_POINT('Ctrl Pts',(-0.00387491567942501,2.42225320762339,
10.8436710160015));
#41647=CARTESIAN_POINT('Ctrl Pts',(-0.0028905090694996,2.42226354078405,
10.8436109432667));
#41648=CARTESIAN_POINT('Ctrl Pts',(-0.00140553397426754,2.42227232374715,
10.8435201129249));
#41649=CARTESIAN_POINT('Ctrl Pts',(-0.000904984925018192,2.4222741180687,
10.8434894601056));
#41650=CARTESIAN_POINT('Ctrl Pts',(-1.1542251554175E-5,2.42227523928697,
10.8434346819036));
#41651=CARTESIAN_POINT('Ctrl Pts',(0.000381350629554541,2.42227501386274,
10.8434105705915));
#41652=CARTESIAN_POINT('Ctrl Pts',(0.00121041202159171,2.42227302210117,
10.8433596442969));
#41653=CARTESIAN_POINT('Ctrl Pts',(0.00164657900812938,2.42227108875305,
10.8433328241308));
#41654=CARTESIAN_POINT('Ctrl Pts',(0.00280044562657512,2.42226363160241,
10.8432617975017));
#41655=CARTESIAN_POINT('Ctrl Pts',(0.0035181300406506,2.42225659573851,
10.8432175437585));
#41656=CARTESIAN_POINT('Ctrl Pts',(0.00678621880943238,2.42221363832007,
10.8430156744027));
#41657=CARTESIAN_POINT('Ctrl Pts',(0.00933610820792382,2.42214983775739,
10.842857188052));
#41658=CARTESIAN_POINT('Ctrl Pts',(0.0204498601225729,2.42173970387509,
10.8421619773793));
#41659=CARTESIAN_POINT('Ctrl Pts',(0.0289980645457899,2.42108211381585,
10.8416156066078));
#41660=CARTESIAN_POINT('Ctrl Pts',(0.0518506750052404,2.41840411832439,
10.840122660526));
#41661=CARTESIAN_POINT('Ctrl Pts',(0.0660614457994081,2.41576175021939,
10.8391592651973));
#41662=CARTESIAN_POINT('Ctrl Pts',(0.100061661172676,2.40704366481283,10.8367908423604));
#41663=CARTESIAN_POINT('Ctrl Pts',(0.11953833727544,2.39999803835101,10.8353782450734));
#41664=CARTESIAN_POINT('Ctrl Pts',(0.142793934344817,2.38895821323529,10.8337078052743));
#41665=CARTESIAN_POINT('Ctrl Pts',(0.147329061408764,2.38667248130582,10.8333830738473));
#41666=CARTESIAN_POINT('Ctrl Pts',(0.152368685614037,2.38398127130485,10.8330249437837));
#41667=CARTESIAN_POINT('Ctrl Pts',(0.152927913338762,2.38368051069083,10.8329852419164));
#41668=CARTESIAN_POINT('Ctrl Pts',(0.153740130145165,2.38324058919787,10.8329276394043));
#41669=CARTESIAN_POINT('Ctrl Pts',(0.153993822444982,2.38310274042573,10.83290965607));
#41670=CARTESIAN_POINT('Ctrl Pts',(0.154441187509682,2.38285887642632,10.8328779595415));
#41671=CARTESIAN_POINT('Ctrl Pts',(0.15463493685416,2.38275300295109,10.8328642372649));
#41672=CARTESIAN_POINT('Ctrl Pts',(0.155038322735569,2.3825320358852,10.8328356784643));
#41673=CARTESIAN_POINT('Ctrl Pts',(0.155247939552821,2.38241690828205,10.8328208442059));
#41674=CARTESIAN_POINT('Ctrl Pts',(0.155786759878913,2.38212019144365,10.832782728005));
#41675=CARTESIAN_POINT('Ctrl Pts',(0.156115775298288,2.38193825863157,10.8327594681153));
#41676=CARTESIAN_POINT('Ctrl Pts',(0.157500660487726,2.38116930312701,10.8326616217875));
#41677=CARTESIAN_POINT('Ctrl Pts',(0.158553561158957,2.38057691178591,10.8325873752561));
#41678=CARTESIAN_POINT('Ctrl Pts',(0.166009405698405,2.37632667238095,10.8320624640645));
#41679=CARTESIAN_POINT('Ctrl Pts',(0.172289033519813,2.37245561244307,10.8316248037739));
#41680=CARTESIAN_POINT('Ctrl Pts',(0.187890154103074,2.36208299841643,10.8305344728968));
#41681=CARTESIAN_POINT('Ctrl Pts',(0.197010994941928,2.35529768771181,10.8298939995265));
#41682=CARTESIAN_POINT('Ctrl Pts',(0.227028489085056,2.33039792720633,10.8277088209117));
#41683=CARTESIAN_POINT('Ctrl Pts',(0.245940977411665,2.31009047109807,10.8261815815243));
#41684=CARTESIAN_POINT('Ctrl Pts',(0.263275708302855,2.28588074828818,10.8244000716234));
#41685=CARTESIAN_POINT('Ctrl Pts',(0.264503637797201,2.28412923838518,10.8242714611924));
#41686=CARTESIAN_POINT('Ctrl Pts',(0.266893076745795,2.28064773092194,10.824016275425));
#41687=CARTESIAN_POINT('Ctrl Pts',(0.268055424469995,2.27891843448501,10.8238897397952));
#41688=CARTESIAN_POINT('Ctrl Pts',(0.269581618897993,2.27659956379977,10.8237203050365));
#41689=CARTESIAN_POINT('Ctrl Pts',(0.269960468991074,2.2760198862409,10.8236779691838));
#41690=CARTESIAN_POINT('Ctrl Pts',(0.270548379797402,2.27511396276046,10.8236118356599));
#41691=CARTESIAN_POINT('Ctrl Pts',(0.270758727020435,2.27478855084024,10.8235880860411));
#41692=CARTESIAN_POINT('Ctrl Pts',(0.271159266944028,2.27416644847412,10.8235426937839));
#41693=CARTESIAN_POINT('Ctrl Pts',(0.271349560984522,2.27386982364876,10.8235210549582));
#41694=CARTESIAN_POINT('Ctrl Pts',(0.271792334550795,2.27317714372988,10.8234705344156));
#41695=CARTESIAN_POINT('Ctrl Pts',(0.2720444350845,2.27278084837991,10.823441638686));
#41696=CARTESIAN_POINT('Ctrl Pts',(0.272751531107803,2.27166392814386,10.8233602205534));
#41697=CARTESIAN_POINT('Ctrl Pts',(0.273204533208145,2.27094205146664,10.8233076245379));
#41698=CARTESIAN_POINT('Ctrl Pts',(0.275961294149326,2.26651009509438,10.8229848557913));
#41699=CARTESIAN_POINT('Ctrl Pts',(0.278192213177379,2.26275545196488,10.8227120211129));
#41700=CARTESIAN_POINT('Ctrl Pts',(0.284577792356043,2.2514934472642,10.8218949441144));
#41701=CARTESIAN_POINT('Ctrl Pts',(0.288509454058563,2.24386471994284,10.8213430165293));
#41702=CARTESIAN_POINT('Ctrl Pts',(0.302868305213806,2.21304162077153,10.819119239426));
#41703=CARTESIAN_POINT('Ctrl Pts',(0.3108389087555,2.1888060638396,10.8173752510299));
#41704=CARTESIAN_POINT('Ctrl Pts',(0.31716280067314,2.15754049933757,10.8152396653128));
#41705=CARTESIAN_POINT('Ctrl Pts',(0.318255514282371,2.15115259386374,10.8148097021576));
#41706=CARTESIAN_POINT('Ctrl Pts',(0.319219968588202,2.14427196206787,10.8143561049554));
#41707=CARTESIAN_POINT('Ctrl Pts',(0.319283969726922,2.14380800898004,10.8143255657953));
#41708=CARTESIAN_POINT('Ctrl Pts',(0.320114209472132,2.13769101344285,10.8139235465938));
#41709=CARTESIAN_POINT('Ctrl Pts',(0.320731287520682,2.13201828848829,10.8135577436096));
#41710=CARTESIAN_POINT('Ctrl Pts',(0.321250974254636,2.12567909643771,10.8131589439058));
#41711=CARTESIAN_POINT('Ctrl Pts',(0.321302490496047,2.12502626764627,10.8131179921234));
#41712=CARTESIAN_POINT('Ctrl Pts',(0.321374130021455,2.1240817289397,10.8130589162377));
#41713=CARTESIAN_POINT('Ctrl Pts',(0.321395846311586,2.1237901469322,10.8130407034126));
#41714=CARTESIAN_POINT('Ctrl Pts',(0.321433308186684,2.12327773668905,10.8130087399866));
#41715=CARTESIAN_POINT('Ctrl Pts',(0.321449223072885,2.12305692139539,10.8129949798098));
#41716=CARTESIAN_POINT('Ctrl Pts',(0.32148174423954,2.12259911908549,10.8129664808602));
#41717=CARTESIAN_POINT('Ctrl Pts',(0.321498315987564,2.12236213050614,10.8129517440802));
#41718=CARTESIAN_POINT('Ctrl Pts',(0.321539958544361,2.12175699528843,10.8129141553932));
#41719=CARTESIAN_POINT('Ctrl Pts',(0.321564659237252,2.12138882225719,10.8128913243839));
#41720=CARTESIAN_POINT('Ctrl Pts',(0.321663347109478,2.11987902239117,10.8127978540849));
#41721=CARTESIAN_POINT('Ctrl Pts',(0.321731888698102,2.11873702996835,10.8127275173552));
#41722=CARTESIAN_POINT('Ctrl Pts',(0.322162733150101,2.11085718583566,10.812244542223));
#41723=CARTESIAN_POINT('Ctrl Pts',(0.322319460272764,2.10410922070286,10.811842803961));
#41724=CARTESIAN_POINT('Ctrl Pts',(0.322170215683179,2.08588560106358,10.8107780117959));
#41725=CARTESIAN_POINT('Ctrl Pts',(0.321463384350314,2.07442279251201,10.8101296455797));
#41726=CARTESIAN_POINT('Ctrl Pts',(0.318151064318214,2.04574598094925,10.8085108981325));
#41727=CARTESIAN_POINT('Ctrl Pts',(0.314760745307126,2.02866101804574,10.807548186357));
#41728=CARTESIAN_POINT('Ctrl Pts',(0.308293931901818,2.00589683634375,10.8061938089964));
#41729=CARTESIAN_POINT('Ctrl Pts',(0.306403266848392,1.99991211037764,10.8058309528896));
#41730=CARTESIAN_POINT('Ctrl Pts',(0.303769500211715,1.99235119368304,10.8053615327717));
#41731=CARTESIAN_POINT('Ctrl Pts',(0.303186653246037,1.99072041408497,10.8052596251761));
#41732=CARTESIAN_POINT('Ctrl Pts',(0.300375677576086,1.98305105078815,10.8047770948787));
#41733=CARTESIAN_POINT('Ctrl Pts',(0.297980236284294,1.97707573723689,10.8043914992427));
#41734=CARTESIAN_POINT('Ctrl Pts',(0.294995983397775,1.97023249289481,10.8039371122638));
#41735=CARTESIAN_POINT('Ctrl Pts',(0.294579819742053,1.96929052871632,10.8038742817928));
#41736=CARTESIAN_POINT('Ctrl Pts',(0.293953711182385,1.96789154368097,10.8037805369586));
#41737=CARTESIAN_POINT('Ctrl Pts',(0.293747196819757,1.96743298711633,10.8037497403544));
#41738=CARTESIAN_POINT('Ctrl Pts',(0.293377320838695,1.96661680080161,10.8036948013628));
#41739=CARTESIAN_POINT('Ctrl Pts',(0.293214376166809,1.96625898229106,10.8036706733594));
#41740=CARTESIAN_POINT('Ctrl Pts',(0.292869827375283,1.96550602633493,10.8036198107353));
#41741=CARTESIAN_POINT('Ctrl Pts',(0.292688077572445,1.96511095677171,10.8035930711282));
#41742=CARTESIAN_POINT('Ctrl Pts',(0.292206683881702,1.96407010504709,10.8035224838292));
#41743=CARTESIAN_POINT('Ctrl Pts',(0.291905700070021,1.96342494846904,10.8034785899013));
#41744=CARTESIAN_POINT('Ctrl Pts',(0.290563828504156,1.96057335619494,10.8032839470755));
#41745=CARTESIAN_POINT('Ctrl Pts',(0.289500065727184,1.95837783063611,10.803132406664));
#41746=CARTESIAN_POINT('Ctrl Pts',(0.285336166523421,1.95002684542292,10.802549412836));
#41747=CARTESIAN_POINT('Ctrl Pts',(0.282063980205399,1.94395970263495,10.8021119786927));
#41748=CARTESIAN_POINT('Ctrl Pts',(0.274779318427399,1.9314316915685,10.8011784549952));
#41749=CARTESIAN_POINT('Ctrl Pts',(0.270727600632003,1.92499856860512,10.8006812427713));
#41750=CARTESIAN_POINT('Ctrl Pts',(0.256201855459062,1.90364863809213,10.7989713365855));
#41751=CARTESIAN_POINT('Ctrl Pts',(0.244692238546218,1.88947951314088,10.7977307628302));
#41752=CARTESIAN_POINT('Ctrl Pts',(0.221115940790994,1.86501680838258,10.7954398317263));
#41753=CARTESIAN_POINT('Ctrl Pts',(0.209365082551467,1.85448878692668,10.7943902494897));
#41754=CARTESIAN_POINT('Ctrl Pts',(0.196176144150561,1.84431091437637,10.7933426458307));
#41755=CARTESIAN_POINT('Ctrl Pts',(0.195460253945488,1.84376323992363,10.7932861654675));
#41756=CARTESIAN_POINT('Ctrl Pts',(0.194492881862838,1.84302958859923,10.79321036955));
#41757=CARTESIAN_POINT('Ctrl Pts',(0.194243422120287,1.84284097061193,10.7931908705696));
#41758=CARTESIAN_POINT('Ctrl Pts',(0.193822531167957,1.84252369433805,10.7931580510286));
#41759=CARTESIAN_POINT('Ctrl Pts',(0.193651246138516,1.8423948439272,10.7931447169323));
#41760=CARTESIAN_POINT('Ctrl Pts',(0.193322141882042,1.84214778658587,10.7931191395962));
#41761=CARTESIAN_POINT('Ctrl Pts',(0.193164343881372,1.84202955448821,10.7931068946283));
#41762=CARTESIAN_POINT('Ctrl Pts',(0.192790079310927,1.8417496680869,10.7930778964225));
#41763=CARTESIAN_POINT('Ctrl Pts',(0.192573518154887,1.84158814129249,10.7930611522335));
#41764=CARTESIAN_POINT('Ctrl Pts',(0.191943536556329,1.84111948771465,10.7930125440126));
#41765=CARTESIAN_POINT('Ctrl Pts',(0.191529580269318,1.84081307757253,10.7929807301094));
#41766=CARTESIAN_POINT('Ctrl Pts',(0.188488287307231,1.83857317962341,10.7927479062483));
#41767=CARTESIAN_POINT('Ctrl Pts',(0.185832343635391,1.83667860149329,10.792549548796));
#41768=CARTESIAN_POINT('Ctrl Pts',(0.177133834337808,1.83067082608023,10.7919142072025));
#41769=CARTESIAN_POINT('Ctrl Pts',(0.170979667262602,1.82672254280494,10.7914866064025));
#41770=CARTESIAN_POINT('Ctrl Pts',(0.150500920550196,1.81454706264683,10.7901155524729));
#41771=CARTESIAN_POINT('Ctrl Pts',(0.135677266190528,1.80721057699218,10.7892015917685));
#41772=CARTESIAN_POINT('Ctrl Pts',(0.098848311992101,1.79238378771678,10.7869781129733));
#41773=CARTESIAN_POINT('Ctrl Pts',(0.0764728904200744,1.78607263948,10.785660325576));
#41774=CARTESIAN_POINT('Ctrl Pts',(0.0521666338831035,1.78197173393901,
10.7841649158761));
#41775=CARTESIAN_POINT('Ctrl Pts',(0.0507157585877637,1.78173714099231,
10.7840754443978));
#41776=CARTESIAN_POINT('Ctrl Pts',(0.0487303563231147,1.78143004084754,
10.7839527095283));
#41777=CARTESIAN_POINT('Ctrl Pts',(0.0481971612349797,1.78134893669549,
10.7839197185659));
#41778=CARTESIAN_POINT('Ctrl Pts',(0.0472889729973594,1.78121312406217,
10.7838634740113));
#41779=CARTESIAN_POINT('Ctrl Pts',(0.0469140810878628,1.78115773769614,
10.783840241917));
#41780=CARTESIAN_POINT('Ctrl Pts',(0.0461884616525597,1.78105184246282,
10.7837952461277));
#41781=CARTESIAN_POINT('Ctrl Pts',(0.0458377466165753,1.7810012505201,10.783773485095));
#41782=CARTESIAN_POINT('Ctrl Pts',(0.0450047784740421,1.78088249381383,
10.7837217699005));
#41783=CARTESIAN_POINT('Ctrl Pts',(0.0445224539117189,1.78081484380767,
10.7836917995057));
#41784=CARTESIAN_POINT('Ctrl Pts',(0.0435239257859611,1.7806770993354,10.7836297009935));
#41785=CARTESIAN_POINT('Ctrl Pts',(0.0430077022223628,1.78060716265214,
10.7835975679744));
#41786=CARTESIAN_POINT('Ctrl Pts',(0.0400986429325167,1.78022023107301,
10.7834163238579));
#41787=CARTESIAN_POINT('Ctrl Pts',(0.0377025264427915,1.77992888169953,
10.7832664050089));
#41788=CARTESIAN_POINT('Ctrl Pts',(0.0243791632026217,1.77846054556863,
10.7824291016603));
#41789=CARTESIAN_POINT('Ctrl Pts',(0.0134016727939297,1.77781633631662,
10.7817250760602));
#41790=CARTESIAN_POINT('Ctrl Pts',(-0.0153453844068379,1.7776010274237,
10.77984378476));
#41791=CARTESIAN_POINT('Ctrl Pts',(-0.0330835211050536,1.7789362295998,
10.7786438881372));
#41792=CARTESIAN_POINT('Ctrl Pts',(-0.0648422002494271,1.7839872358441,
10.7764679307087));
#41793=CARTESIAN_POINT('Ctrl Pts',(-0.0788983628367126,1.7872002450973,
10.775495491016));
#41794=CARTESIAN_POINT('Ctrl Pts',(-0.0981707844038029,1.79298797823714,
10.7741848989983));
#41795=CARTESIAN_POINT('Ctrl Pts',(-0.103603952139945,1.7947785794191,10.7738181481725));
#41796=CARTESIAN_POINT('Ctrl Pts',(-0.109603861005411,1.79693466221395,
10.7734183992851));
#41797=CARTESIAN_POINT('Ctrl Pts',(-0.110220075302332,1.79715822558155,
10.7733774061805));
#41798=CARTESIAN_POINT('Ctrl Pts',(-0.111110274720616,1.79748426811576,
10.773318281662));
#41799=CARTESIAN_POINT('Ctrl Pts',(-0.111384804077562,1.79758524075671,
10.7733000613232));
#41800=CARTESIAN_POINT('Ctrl Pts',(-0.11186689015307,1.79776329883086,10.7732680891249));
#41801=CARTESIAN_POINT('Ctrl Pts',(-0.112074505271714,1.79784022452448,
10.7732543276733));
#41802=CARTESIAN_POINT('Ctrl Pts',(-0.112504677296678,1.79800011651413,
10.7732258305171));
#41803=CARTESIAN_POINT('Ctrl Pts',(-0.112727221386195,1.79808311475088,
10.7732110967968));
#41804=CARTESIAN_POINT('Ctrl Pts',(-0.113177731384221,1.79825170085499,
10.7731812880924));
#41805=CARTESIAN_POINT('Ctrl Pts',(-0.113405692488535,1.79833730122814,
10.7731662138721));
#41806=CARTESIAN_POINT('Ctrl Pts',(-0.113964366481706,1.79854780848473,
10.7731292928594));
#41807=CARTESIAN_POINT('Ctrl Pts',(-0.114294972239522,1.79867300167344,
10.7731074631));
#41808=CARTESIAN_POINT('Ctrl Pts',(-0.117197162756775,1.79977746143001,
10.7729159935531));
#41809=CARTESIAN_POINT('Ctrl Pts',(-0.119756414988149,1.80078912134339,
10.7727482593783));
#41810=CARTESIAN_POINT('Ctrl Pts',(-0.127698422202196,1.80404678858108,
10.7722302834361));
#41811=CARTESIAN_POINT('Ctrl Pts',(-0.133033630854286,1.80640631422611,
10.7718860012415));
#41812=CARTESIAN_POINT('Ctrl Pts',(-0.145807976095883,1.81247562911149,
10.7710638616066));
#41813=CARTESIAN_POINT('Ctrl Pts',(-0.153173438418639,1.81633092851107,
10.7705916484649));
#41814=CARTESIAN_POINT('Ctrl Pts',(-0.167248980172034,1.82440676164033,
10.7696778047332));
#41815=CARTESIAN_POINT('Ctrl Pts',(-0.173968550279033,1.82859845044054,
10.7692360983364));
#41816=CARTESIAN_POINT('Ctrl Pts',(-0.193904732327327,1.84207960883757,
10.7678905955094));
#41817=CARTESIAN_POINT('Ctrl Pts',(-0.206582853771419,1.85211808789723,
10.7669846279726));
#41818=CARTESIAN_POINT('Ctrl Pts',(-0.22567209497134,1.86971830563562,10.7654739439579));
#41819=CARTESIAN_POINT('Ctrl Pts',(-0.232581221058186,1.87669863558606,
10.7648915233247));
#41820=CARTESIAN_POINT('Ctrl Pts',(-0.239858432389519,1.88475550647357,
10.7642313472801));
#41821=CARTESIAN_POINT('Ctrl Pts',(-0.240552536525814,1.88553150181668,
10.764167882888));
#41822=CARTESIAN_POINT('Ctrl Pts',(-0.24158501751995,1.88669711391323,10.7640727268612));
#41823=CARTESIAN_POINT('Ctrl Pts',(-0.241926243234808,1.88708420741413,
10.7640411543528));
#41824=CARTESIAN_POINT('Ctrl Pts',(-0.242512304681486,1.88775227540928,
10.7639867125459));
#41825=CARTESIAN_POINT('Ctrl Pts',(-0.24275758616245,1.88803285897444,10.7639638618486));
#41826=CARTESIAN_POINT('Ctrl Pts',(-0.243262798702852,1.88861281122461,
10.763916660035));
#41827=CARTESIAN_POINT('Ctrl Pts',(-0.243522665041562,1.88891223526701,
10.7638923062895));
#41828=CARTESIAN_POINT('Ctrl Pts',(-0.244126240357445,1.88961028676714,
10.7638355670627));
#41829=CARTESIAN_POINT('Ctrl Pts',(-0.244469525864673,1.89000927738701,
10.7638031641654));
#41830=CARTESIAN_POINT('Ctrl Pts',(-0.245185987935276,1.89084613812682,
10.7637352584002));
#41831=CARTESIAN_POINT('Ctrl Pts',(-0.245558972192081,1.89128416977776,
10.7636997477658));
#41832=CARTESIAN_POINT('Ctrl Pts',(-0.246553615560689,1.89245863286658,
10.763604621645));
#41833=CARTESIAN_POINT('Ctrl Pts',(-0.247173143968474,1.89319685378121,
10.7635449191471));
#41834=CARTESIAN_POINT('Ctrl Pts',(-0.251699643887626,1.89863996102266,
10.7631053579098));
#41835=CARTESIAN_POINT('Ctrl Pts',(-0.255475071885383,1.90345215488008,
10.7627202152829));
#41836=CARTESIAN_POINT('Ctrl Pts',(-0.266748429169294,1.91869523109058,
10.7615097313423));
#41837=CARTESIAN_POINT('Ctrl Pts',(-0.273760717666368,1.92946804588284,
10.7606669029885));
#41838=CARTESIAN_POINT('Ctrl Pts',(-0.282428943559775,1.94470338840907,
10.7594961165116));
#41839=CARTESIAN_POINT('Ctrl Pts',(-0.284657654187898,1.94882737080095,
10.7591812800396));
#41840=CARTESIAN_POINT('Ctrl Pts',(-0.288995875197006,1.95729110644638,
10.7585402058681));
#41841=CARTESIAN_POINT('Ctrl Pts',(-0.291099489825572,1.96163262545429,
10.7582139804731));
#41842=CARTESIAN_POINT('Ctrl Pts',(-0.301787756297035,1.98501503467603,
10.7564742353186));
#41843=CARTESIAN_POINT('Ctrl Pts',(-0.308604591443418,2.00481175290639,
10.7550579039448));
#41844=CARTESIAN_POINT('Ctrl Pts',(-0.313744243975711,2.02633016006292,
10.7536620709368));
#41845=CARTESIAN_POINT('Ctrl Pts',(-0.314023811025219,2.02753109515205,
10.753584641336));
#41846=CARTESIAN_POINT('Ctrl Pts',(-0.314383842334844,2.0291188927553,10.7534829174762));
#41847=CARTESIAN_POINT('Ctrl Pts',(-0.314470492790375,2.02950432031956,
10.7534582750149));
#41848=CARTESIAN_POINT('Ctrl Pts',(-0.314603767138215,2.03010226995748,
10.7534201239611));
#41849=CARTESIAN_POINT('Ctrl Pts',(-0.314650884507248,2.03031467986631,
10.7534065870088));
#41850=CARTESIAN_POINT('Ctrl Pts',(-0.314744419923687,2.03073837608001,
10.7533796157682));
#41851=CARTESIAN_POINT('Ctrl Pts',(-0.314790840000343,2.03094965986041,
10.7533661814998));
#41852=CARTESIAN_POINT('Ctrl Pts',(-0.314895436098572,2.03142803291989,
10.7533357993947));
#41853=CARTESIAN_POINT('Ctrl Pts',(-0.314953484940393,2.03169514899971,
10.7533188589836));
#41854=CARTESIAN_POINT('Ctrl Pts',(-0.315073269849817,2.03224974754472,
10.7532837367297));
#41855=CARTESIAN_POINT('Ctrl Pts',(-0.315134952510768,2.0325372414641,10.7532655579586));
#41856=CARTESIAN_POINT('Ctrl Pts',(-0.315295126749975,2.03328880355613,
10.7532181074321));
#41857=CARTESIAN_POINT('Ctrl Pts',(-0.315392987693711,2.03375300758843,
10.7531888713319));
#41858=CARTESIAN_POINT('Ctrl Pts',(-0.315680163968844,2.03513029022962,
10.7531023368503));
#41859=CARTESIAN_POINT('Ctrl Pts',(-0.315866543726185,2.03604398564295,
10.7530452008022));
#41860=CARTESIAN_POINT('Ctrl Pts',(-0.320169775754063,2.05761758049861,
10.7517022603504));
#41861=CARTESIAN_POINT('Ctrl Pts',(-0.322255586913252,2.07863376685202,
10.7505244445363));
#41862=CARTESIAN_POINT('Ctrl Pts',(-0.322274865121244,2.09970515074319,
10.7493463817436));
#41863=CARTESIAN_POINT('',(-0.322378175270278,2.10028753889625,10.4993773449273));
#41864=CARTESIAN_POINT('Ctrl Pts',(-0.322274865041499,2.09970506359358,
10.749346386616));
#41865=CARTESIAN_POINT('Ctrl Pts',(-0.322298947962674,2.12602029631154,
10.747875149744));
#41866=CARTESIAN_POINT('Ctrl Pts',(-0.319100146337298,2.15223683286578,
10.7464067880084));
#41867=CARTESIAN_POINT('Ctrl Pts',(-0.312294610467603,2.17960409921395,
10.7447097168287));
#41868=CARTESIAN_POINT('Ctrl Pts',(-0.311823167679749,2.18143124833739,
10.7445956620758));
#41869=CARTESIAN_POINT('Ctrl Pts',(-0.311094630812034,2.18415567252314,
10.744424429838));
#41870=CARTESIAN_POINT('Ctrl Pts',(-0.310849635013528,2.18505616333527,
10.7443676417984));
#41871=CARTESIAN_POINT('Ctrl Pts',(-0.310450663350225,2.18649784874588,
10.7442764120228));
#41872=CARTESIAN_POINT('Ctrl Pts',(-0.31029917412897,2.18703973081777,10.7442420508823));
#41873=CARTESIAN_POINT('Ctrl Pts',(-0.310005712233462,2.18807895042629,
10.7441760158872));
#41874=CARTESIAN_POINT('Ctrl Pts',(-0.309863959764702,2.18857634875961,
10.7441443492701));
#41875=CARTESIAN_POINT('Ctrl Pts',(-0.309611814493428,2.18945309408581,
10.7440884241138));
#41876=CARTESIAN_POINT('Ctrl Pts',(-0.309501920051702,2.18983258427484,
10.7440641818648));
#41877=CARTESIAN_POINT('Ctrl Pts',(-0.309286221045972,2.19057234725597,
10.7440168550992));
#41878=CARTESIAN_POINT('Ctrl Pts',(-0.30918048407323,2.19093263925974,10.7439937728217));
#41879=CARTESIAN_POINT('Ctrl Pts',(-0.308895022809321,2.19189907628478,
10.7439317701755));
#41880=CARTESIAN_POINT('Ctrl Pts',(-0.308714144787251,2.19250487629064,
10.7438928121462));
#41881=CARTESIAN_POINT('Ctrl Pts',(-0.308048997736904,2.19470891996789,
10.7437507342567));
#41882=CARTESIAN_POINT('Ctrl Pts',(-0.307554096759057,2.19630390400352,
10.7436472667847));
#41883=CARTESIAN_POINT('Ctrl Pts',(-0.298907164508607,2.22342494795731,
10.7418765848048));
#41884=CARTESIAN_POINT('Ctrl Pts',(-0.287617053967074,2.24783445387442,
10.7400979402577));
#41885=CARTESIAN_POINT('Ctrl Pts',(-0.271109525969361,2.27429921569771,
10.7379882550481));
#41886=CARTESIAN_POINT('Ctrl Pts',(-0.268701074259604,2.27798967495513,
10.7376898907732));
#41887=CARTESIAN_POINT('Ctrl Pts',(-0.263954048790093,2.28494747437011,
10.7371203814653));
#41888=CARTESIAN_POINT('Ctrl Pts',(-0.261628532548203,2.28822279319848,
10.7368492118639));
#41889=CARTESIAN_POINT('Ctrl Pts',(-0.253165820068518,2.29968192028348,
10.7358912199109));
#41890=CARTESIAN_POINT('Ctrl Pts',(-0.246700451731211,2.30761677042343,
10.735210522179));
#41891=CARTESIAN_POINT('Ctrl Pts',(-0.237627904264332,2.31772782629353,
10.7343326017391));
#41892=CARTESIAN_POINT('Ctrl Pts',(-0.235348762854026,2.32018943914594,
10.7341179940958));
#41893=CARTESIAN_POINT('Ctrl Pts',(-0.232056064482261,2.32363620601565,
10.7338168096945));
#41894=CARTESIAN_POINT('Ctrl Pts',(-0.231073905433615,2.32465088494316,
10.7337280582832));
#41895=CARTESIAN_POINT('Ctrl Pts',(-0.229878412548336,2.32586982576314,
10.7336213716394));
#41896=CARTESIAN_POINT('Ctrl Pts',(-0.229671447282492,2.32608027125522,
10.7336029500902));
#41897=CARTESIAN_POINT('Ctrl Pts',(-0.22930944242504,2.32644735328804,10.7335708133176));
#41898=CARTESIAN_POINT('Ctrl Pts',(-0.229154531159029,2.32660411524599,
10.7335570881019));
#41899=CARTESIAN_POINT('Ctrl Pts',(-0.22884277404062,2.32691895024804,10.7335295206109));
#41900=CARTESIAN_POINT('Ctrl Pts',(-0.228685924671178,2.32707702012919,
10.7335156785938));
#41901=CARTESIAN_POINT('Ctrl Pts',(-0.228383273736942,2.32738139449964,
10.7334890228318));
#41902=CARTESIAN_POINT('Ctrl Pts',(-0.228237495679712,2.32752772106683,
10.7334762072742));
#41903=CARTESIAN_POINT('Ctrl Pts',(-0.227890852872223,2.32787499979183,
10.7334457894489));
#41904=CARTESIAN_POINT('Ctrl Pts',(-0.227689862447762,2.32807582706836,
10.7334281971804));
#41905=CARTESIAN_POINT('Ctrl Pts',(-0.227086533149923,2.32867707427269,
10.7333755215595));
#41906=CARTESIAN_POINT('Ctrl Pts',(-0.226683398982979,2.32907669997849,
10.7333405008279));
#41907=CARTESIAN_POINT('Ctrl Pts',(-0.222759111821345,2.33294633098297,
10.733001274239));
#41908=CARTESIAN_POINT('Ctrl Pts',(-0.219159377203399,2.33633617777352,
10.7327031976152));
#41909=CARTESIAN_POINT('Ctrl Pts',(-0.204157909887012,2.34982528945459,
10.7315061892919));
#41910=CARTESIAN_POINT('Ctrl Pts',(-0.192124151046473,2.35919400674232,
10.7306483123578));
#41911=CARTESIAN_POINT('Ctrl Pts',(-0.170176457118849,2.3739094618392,10.7291689120569));
#41912=CARTESIAN_POINT('Ctrl Pts',(-0.160562881928018,2.37965331498035,
10.7285461873567));
#41913=CARTESIAN_POINT('Ctrl Pts',(-0.138568829296287,2.39128552974201,
10.7271421017815));
#41914=CARTESIAN_POINT('Ctrl Pts',(-0.126073159891165,2.39690753071808,
10.7263574913742));
#41915=CARTESIAN_POINT('Ctrl Pts',(-0.109638873987785,2.40307662867029,
10.7253171200076));
#41916=CARTESIAN_POINT('Ctrl Pts',(-0.105994959828447,2.40437015643307,
10.7250859917346));
#41917=CARTESIAN_POINT('Ctrl Pts',(-0.100055025677356,2.40635913080523,
10.7247080451412));
#41918=CARTESIAN_POINT('Ctrl Pts',(-0.0977729069876538,2.40709507220141,
10.7245625600458));
#41919=CARTESIAN_POINT('Ctrl Pts',(-0.0948072288030243,2.40801504079811,
10.7243730687199));
#41920=CARTESIAN_POINT('Ctrl Pts',(-0.0941309386358112,2.40822239109148,
10.7243298286319));
#41921=CARTESIAN_POINT('Ctrl Pts',(-0.0930387630393945,2.4085533218532,
10.7242599498034));
#41922=CARTESIAN_POINT('Ctrl Pts',(-0.0926232985535299,2.40867829275266,
10.7242333566144));
#41923=CARTESIAN_POINT('Ctrl Pts',(-0.0918306228589753,2.40891498361228,
10.7241825968639));
#41924=CARTESIAN_POINT('Ctrl Pts',(-0.0914534566807141,2.40902685264199,
10.7241584352265));
#41925=CARTESIAN_POINT('Ctrl Pts',(-0.0905918456461861,2.40928069446871,
10.7241032175996));
#41926=CARTESIAN_POINT('Ctrl Pts',(-0.0901072710311573,2.40942221990563,
10.7240721470738));
#41927=CARTESIAN_POINT('Ctrl Pts',(-0.0886239874656251,2.40985164963416,
10.7239769905544));
#41928=CARTESIAN_POINT('Ctrl Pts',(-0.0876242238987311,2.41013585939218,
10.7239127843964));
#41929=CARTESIAN_POINT('Ctrl Pts',(-0.0802244784532333,2.41220079992454,
10.7234370328298));
#41930=CARTESIAN_POINT('Ctrl Pts',(-0.0737725856011363,2.41378798805052,
10.7230192456786));
#41931=CARTESIAN_POINT('Ctrl Pts',(-0.0654651764833456,2.41556127321382,
10.7224769617545));
#41932=CARTESIAN_POINT('Ctrl Pts',(-0.0636504578355044,2.41593231154828,
10.7223582434674));
#41933=CARTESIAN_POINT('Ctrl Pts',(-0.0599144870418084,2.41666267528131,
10.722113304814));
#41934=CARTESIAN_POINT('Ctrl Pts',(-0.0579929644795718,2.41702020675858,
10.7219870373087));
#41935=CARTESIAN_POINT('Ctrl Pts',(-0.0407613136134358,2.42006453921861,
10.7208521619613));
#41936=CARTESIAN_POINT('Ctrl Pts',(-0.0252803082319925,2.42165758931989,
10.7198131369327));
#41937=CARTESIAN_POINT('Ctrl Pts',(0.00553072171022078,2.422589818381,10.7177309124917));
#41938=CARTESIAN_POINT('Ctrl Pts',(0.02082175660266,2.42196469037408,10.716690841117));
#41939=CARTESIAN_POINT('Ctrl Pts',(0.0451900359692089,2.41922461576825,
10.715066236458));
#41940=CARTESIAN_POINT('Ctrl Pts',(0.0543214520439307,2.41779822476334,
10.7144653013709));
#41941=CARTESIAN_POINT('Ctrl Pts',(0.0641483601666872,2.41582713286592,
10.7138359049116));
#41942=CARTESIAN_POINT('Ctrl Pts',(0.0649162972986963,2.41567018285206,
10.7137868362696));
#41943=CARTESIAN_POINT('Ctrl Pts',(0.0659257224586744,2.41546003847582,
10.7137224974864));
#41944=CARTESIAN_POINT('Ctrl Pts',(0.066167724158927,2.41540936739016,10.7137070848949));
#41945=CARTESIAN_POINT('Ctrl Pts',(0.0666446111939686,2.41530894226107,
10.7136767371661));
#41946=CARTESIAN_POINT('Ctrl Pts',(0.0668794996752409,2.41525920414016,
10.7136618011274));
#41947=CARTESIAN_POINT('Ctrl Pts',(0.0673299694455499,2.4151632901314,10.7136331792871));
#41948=CARTESIAN_POINT('Ctrl Pts',(0.0675455582484216,2.41511715566297,
10.7136194912026));
#41949=CARTESIAN_POINT('Ctrl Pts',(0.0680413648033316,2.41501052439887,
10.7135880342486));
#41950=CARTESIAN_POINT('Ctrl Pts',(0.0683215501142049,2.41494987473862,
10.7135702742098));
#41951=CARTESIAN_POINT('Ctrl Pts',(0.069189430855253,2.41476079832211,10.7135153124763));
#41952=CARTESIAN_POINT('Ctrl Pts',(0.0697768521861863,2.41463109893208,
10.7134781835308));
#41953=CARTESIAN_POINT('Ctrl Pts',(0.0746372189181442,2.41354367544523,
10.7131715437163));
#41954=CARTESIAN_POINT('Ctrl Pts',(0.0788908541853553,2.41250054176492,
10.7129068178719));
#41955=CARTESIAN_POINT('Ctrl Pts',(0.083301800030047,2.41132301602692,10.7126348525201));
#41956=CARTESIAN_POINT('Ctrl Pts',(0.0834814016268824,2.41127490386966,
10.7126237832735));
#41957=CARTESIAN_POINT('Ctrl Pts',(0.0961816200177723,2.40786095286697,
10.7118413478027));
#41958=CARTESIAN_POINT('Ctrl Pts',(0.108489056587662,2.40374242506058,10.7111039683175));
#41959=CARTESIAN_POINT('Ctrl Pts',(0.136685402817694,2.39237345193751,10.7093949101415));
#41960=CARTESIAN_POINT('Ctrl Pts',(0.152298840695882,2.38455261435712,10.7084317662239));
#41961=CARTESIAN_POINT('Ctrl Pts',(0.173493095747547,2.37169000430709,10.7070191853711));
#41962=CARTESIAN_POINT('Ctrl Pts',(0.179650255244757,2.36765853034723,10.7065952825656));
#41963=CARTESIAN_POINT('Ctrl Pts',(0.192441241305427,2.35864318358707,10.7056789730607));
#41964=CARTESIAN_POINT('Ctrl Pts',(0.19903128990327,2.35360689100153,10.705185030678));
#41965=CARTESIAN_POINT('Ctrl Pts',(0.206293111102138,2.34759970432696,10.7046119130088));
#41966=CARTESIAN_POINT('Ctrl Pts',(0.20716295721725,2.34687237669808,10.7045427759468));
#41967=CARTESIAN_POINT('Ctrl Pts',(0.208433989094991,2.34579814701021,10.7044410261721));
#41968=CARTESIAN_POINT('Ctrl Pts',(0.208838192253594,2.34545481526066,10.7044085598966));
#41969=CARTESIAN_POINT('Ctrl Pts',(0.209543567714831,2.3448526629359,10.7043517116932));
#41970=CARTESIAN_POINT('Ctrl Pts',(0.209845113349675,2.34459427981546,10.7043273478277));
#41971=CARTESIAN_POINT('Ctrl Pts',(0.210427878719988,2.34409305917469,10.704280142839));
#41972=CARTESIAN_POINT('Ctrl Pts',(0.210709157720643,2.3438502912254,10.7042573046161));
#41973=CARTESIAN_POINT('Ctrl Pts',(0.211376847838965,2.34327199944299,10.7042029627682));
#41974=CARTESIAN_POINT('Ctrl Pts',(0.211762879955846,2.3429360413428,10.7041714411327));
#41975=CARTESIAN_POINT('Ctrl Pts',(0.213126273336623,2.34174378116023,10.7040597447862));
#41976=CARTESIAN_POINT('Ctrl Pts',(0.214099244157049,2.34088249767896,10.7039793623865));
#41977=CARTESIAN_POINT('Ctrl Pts',(0.230671677884107,2.3260326854551,10.7025985633957));
#41978=CARTESIAN_POINT('Ctrl Pts',(0.244872459941179,2.31056440479508,10.7012322714636));
#41979=CARTESIAN_POINT('Ctrl Pts',(0.267782336255844,2.28013266425698,10.698677420583));
#41980=CARTESIAN_POINT('Ctrl Pts',(0.276984782086083,2.26563385157707,10.69750693796));
#41981=CARTESIAN_POINT('Ctrl Pts',(0.290155500838176,2.2406888498499,10.6956207521332));
#41982=CARTESIAN_POINT('Ctrl Pts',(0.294814341998062,2.2306450388883,10.6948927521361));
#41983=CARTESIAN_POINT('Ctrl Pts',(0.299520623389033,2.21895765766375,10.6940958083928));
#41984=CARTESIAN_POINT('Ctrl Pts',(0.300083396109276,2.21753077790015,10.6939993442869));
#41985=CARTESIAN_POINT('Ctrl Pts',(0.300783776247607,2.21571717201296,10.6938778374951));
#41986=CARTESIAN_POINT('Ctrl Pts',(0.300930849044591,2.2153341582108,10.6938522386131));
#41987=CARTESIAN_POINT('Ctrl Pts',(0.301165289484826,2.21472011610684,10.6938112993711));
#41988=CARTESIAN_POINT('Ctrl Pts',(0.301253123042089,2.21448926800543,10.6937959310524));
#41989=CARTESIAN_POINT('Ctrl Pts',(0.301418266577142,2.21405372451225,10.6937669786296));
#41990=CARTESIAN_POINT('Ctrl Pts',(0.301495632846599,2.21384905303181,10.6937533912328));
#41991=CARTESIAN_POINT('Ctrl Pts',(0.301671034769556,2.21338359680543,10.6937225319647));
#41992=CARTESIAN_POINT('Ctrl Pts',(0.301768940556282,2.21312276411232,10.6937052679955));
#41993=CARTESIAN_POINT('Ctrl Pts',(0.302065003905849,2.21233089647643,10.6936529428578));
#41994=CARTESIAN_POINT('Ctrl Pts',(0.302262100223842,2.21179946183977,10.6936179451481));
#41995=CARTESIAN_POINT('Ctrl Pts',(0.303640443295218,2.20805272009653,10.6933720182825));
#41996=CARTESIAN_POINT('Ctrl Pts',(0.304771819561358,2.20481912710627,10.6931639969605));
#41997=CARTESIAN_POINT('Ctrl Pts',(0.308988971208575,2.19212002273206,10.6923611950681));
#41998=CARTESIAN_POINT('Ctrl Pts',(0.311687299820541,2.1825308818715,10.6917853491847));
#41999=CARTESIAN_POINT('Ctrl Pts',(0.318786142613836,2.15193153154589,10.6899988111078));
#42000=CARTESIAN_POINT('Ctrl Pts',(0.32153568657827,2.13059965247486,10.6888241535609));
#42001=CARTESIAN_POINT('Ctrl Pts',(0.322550512340565,2.09487949536509,10.6867893455161));
#42002=CARTESIAN_POINT('Ctrl Pts',(0.322007000756692,2.08059723941255,10.6859586247012));
#42003=CARTESIAN_POINT('Ctrl Pts',(0.320357601281125,2.06486359599118,10.6850037512694));
#42004=CARTESIAN_POINT('Ctrl Pts',(0.320185589843294,2.06332920079406,10.6849102190718));
#42005=CARTESIAN_POINT('Ctrl Pts',(0.319865379692897,2.06064706297677,10.6847459802128));
#42006=CARTESIAN_POINT('Ctrl Pts',(0.319722011447954,2.05949876397645,10.6846754259583));
#42007=CARTESIAN_POINT('Ctrl Pts',(0.319503506014869,2.05782216241935,10.684572053971));
#42008=CARTESIAN_POINT('Ctrl Pts',(0.319433235232706,2.05729322580515,10.6845393899724));
#42009=CARTESIAN_POINT('Ctrl Pts',(0.319308305521555,2.05637042556133,10.6844823115127));
#42010=CARTESIAN_POINT('Ctrl Pts',(0.319254230489449,2.05597648295462,10.6844579155562));
#42011=CARTESIAN_POINT('Ctrl Pts',(0.319148337154954,2.05521549459697,10.6844107324549));
#42012=CARTESIAN_POINT('Ctrl Pts',(0.319096614363009,2.05484843598226,10.6843879483665));
#42013=CARTESIAN_POINT('Ctrl Pts',(0.318972449709663,2.05397815263709,10.6843338670379));
#42014=CARTESIAN_POINT('Ctrl Pts',(0.31889945025578,2.05347500961513,10.6843025521895));
#42015=CARTESIAN_POINT('Ctrl Pts',(0.318638513152496,2.05170599078855,10.6841922794232));
#42016=CARTESIAN_POINT('Ctrl Pts',(0.318444228085861,2.05044107636091,10.6841131207015));
#42017=CARTESIAN_POINT('Ctrl Pts',(0.315454607189546,2.03172059443509,10.682936914757));
#42018=CARTESIAN_POINT('Ctrl Pts',(0.311235719264727,2.01452588216347,10.6817937398494));
#42019=CARTESIAN_POINT('Ctrl Pts',(0.297965061485477,1.97485311257546,10.6790100413986));
#42020=CARTESIAN_POINT('Ctrl Pts',(0.287748941994135,1.95287628132012,10.6773465842651));
#42021=CARTESIAN_POINT('Ctrl Pts',(0.271159156558394,1.92566307328497,10.6752430291027));
#42022=CARTESIAN_POINT('Ctrl Pts',(0.266909354062832,1.91922369921736,10.6747423755288));
#42023=CARTESIAN_POINT('Ctrl Pts',(0.261712726710623,1.91193309486013,10.6741775670027));
#42024=CARTESIAN_POINT('Ctrl Pts',(0.260987420186091,1.91092784775599,10.6740997371059));
#42025=CARTESIAN_POINT('Ctrl Pts',(0.260031860263166,1.90961945448595,10.6739985257031));
#42026=CARTESIAN_POINT('Ctrl Pts',(0.259806857078832,1.90931251357122,10.6739747885978));
#42027=CARTESIAN_POINT('Ctrl Pts',(0.259438954608668,1.90881249477511,10.6739361314559));
#42028=CARTESIAN_POINT('Ctrl Pts',(0.259296383063203,1.90861917793623,10.6739211886853));
#42029=CARTESIAN_POINT('Ctrl Pts',(0.259022558868092,1.90824875954998,10.6738925622388));
#42030=CARTESIAN_POINT('Ctrl Pts',(0.258891341066005,1.90807163383708,10.6738788762628));
#42031=CARTESIAN_POINT('Ctrl Pts',(0.258589193275903,1.90766465016238,10.6738474354345));
#42032=CARTESIAN_POINT('Ctrl Pts',(0.258418137997655,1.90743488469717,10.6738296893832));
#42033=CARTESIAN_POINT('Ctrl Pts',(0.257887573750776,1.90672419846363,10.6737748107936));
#42034=CARTESIAN_POINT('Ctrl Pts',(0.25752702431116,1.90624405062624,10.6737377506899));
#42035=CARTESIAN_POINT('Ctrl Pts',(0.254545119754088,1.90229604168079,10.6734331351089));
#42036=CARTESIAN_POINT('Ctrl Pts',(0.251855031601444,1.89888033237553,10.6731702945455));
#42037=CARTESIAN_POINT('Ctrl Pts',(0.248965139386178,1.895359882096,10.6728989071326));
#42038=CARTESIAN_POINT('Ctrl Pts',(0.248833628196177,1.89519999032107,10.6728865801924));
#42039=CARTESIAN_POINT('Ctrl Pts',(0.247035462461752,1.89301806292881,10.6727183470089));
#42040=CARTESIAN_POINT('Ctrl Pts',(0.245344313343016,1.89101624302113,10.6725638084742));
#42041=CARTESIAN_POINT('Ctrl Pts',(0.225994854707848,1.86867086841682,10.6708336974255));
#42042=CARTESIAN_POINT('Ctrl Pts',(0.205875823633146,1.85059615837575,10.6693780503921));
#42043=CARTESIAN_POINT('Ctrl Pts',(0.171515019078687,1.82675064351744,10.6670012313608));
#42044=CARTESIAN_POINT('Ctrl Pts',(0.158718311161655,1.8191245379348,10.6661372540693));
#42045=CARTESIAN_POINT('Ctrl Pts',(0.143310313993249,1.81133231217202,10.6650954261186));
#42046=CARTESIAN_POINT('Ctrl Pts',(0.141167095034946,1.81027818360029,10.6649505077027));
#42047=CARTESIAN_POINT('Ctrl Pts',(0.138375351502392,1.80894341388019,10.6647616653035));
#42048=CARTESIAN_POINT('Ctrl Pts',(0.137737306751037,1.80864092850298,10.6647185011272));
#42049=CARTESIAN_POINT('Ctrl Pts',(0.136705890871401,1.80815609820774,10.6646487154176));
#42050=CARTESIAN_POINT('Ctrl Pts',(0.136313134433313,1.80797244480987,10.6646221392139));
#42051=CARTESIAN_POINT('Ctrl Pts',(0.135563242327533,1.80762363676797,10.6645713922998));
#42052=CARTESIAN_POINT('Ctrl Pts',(0.135206172209959,1.80745834238302,10.6645472264705));
#42053=CARTESIAN_POINT('Ctrl Pts',(0.134389815687101,1.80708224969276,10.6644919718286));
#42054=CARTESIAN_POINT('Ctrl Pts',(0.13393033521952,1.80687187731503,10.664460868409));
#42055=CARTESIAN_POINT('Ctrl Pts',(0.132521872648275,1.80623101800445,10.6643655133251));
#42056=CARTESIAN_POINT('Ctrl Pts',(0.131571302829227,1.80580405552783,10.6643011407628));
#42057=CARTESIAN_POINT('Ctrl Pts',(0.124491868373924,1.80266539616593,10.6638215685955));
#42058=CARTESIAN_POINT('Ctrl Pts',(0.118282214609934,1.80014103520548,10.6634000141291));
#42059=CARTESIAN_POINT('Ctrl Pts',(0.110169026472496,1.79713407427764,10.6628474968132));
#42060=CARTESIAN_POINT('Ctrl Pts',(0.108333221760304,1.79647257757789,10.6627223678306));
#42061=CARTESIAN_POINT('Ctrl Pts',(0.0784607091494834,1.78601412567791,
10.660684477829));
#42062=CARTESIAN_POINT('Ctrl Pts',(0.0492102102441535,1.78012347961877,
10.6586444317073));
#42063=CARTESIAN_POINT('Ctrl Pts',(0.00835778947718865,1.77763742442317,
10.6559062865581));
#42064=CARTESIAN_POINT('Ctrl Pts',(-0.00288948366096541,1.77754195451658,
10.6551662377923));
#42065=CARTESIAN_POINT('Ctrl Pts',(-0.0151435571886671,1.77807936038324,
10.6543902989268));
#42066=CARTESIAN_POINT('Ctrl Pts',(-0.016167020799385,1.77812913608182,
10.6543257256139));
#42067=CARTESIAN_POINT('Ctrl Pts',(-0.0179324322385133,1.77822343790756,
10.6542147633768));
#42068=CARTESIAN_POINT('Ctrl Pts',(-0.018674488473154,1.77826565066146,
10.6541682515068));
#42069=CARTESIAN_POINT('Ctrl Pts',(-0.0197271244150919,1.77832918520907,
10.6541024619283));
#42070=CARTESIAN_POINT('Ctrl Pts',(-0.0200378223479627,1.77834839001886,
10.6540830667695));
#42071=CARTESIAN_POINT('Ctrl Pts',(-0.0205718335789742,1.77838217498306,
10.6540497722085));
#42072=CARTESIAN_POINT('Ctrl Pts',(-0.0207951599992192,1.77839653760077,
10.6540358605166));
#42073=CARTESIAN_POINT('Ctrl Pts',(-0.0212231723529629,1.77842451172198,
10.6540092220555));
#42074=CARTESIAN_POINT('Ctrl Pts',(-0.0214278599319772,1.77843808601562,
10.6539964931844));
#42075=CARTESIAN_POINT('Ctrl Pts',(-0.0219105658856927,1.7784705606347,
10.6539664994505));
#42076=CARTESIAN_POINT('Ctrl Pts',(-0.0221885735159514,1.77848962616631,
10.6539492439355));
#42077=CARTESIAN_POINT('Ctrl Pts',(-0.0230113653269691,1.77854712482837,
10.6538982296592));
#42078=CARTESIAN_POINT('Ctrl Pts',(-0.0235560804115875,1.77858658245765,
10.653864528144));
#42079=CARTESIAN_POINT('Ctrl Pts',(-0.0283969981610894,1.77894961745865,
10.6535656363785));
#42080=CARTESIAN_POINT('Ctrl Pts',(-0.0326866629084256,1.77935795018307,
10.6533050917391));
#42081=CARTESIAN_POINT('Ctrl Pts',(-0.0371999536787768,1.77987909469105,
10.6530343071208));
#42082=CARTESIAN_POINT('Ctrl Pts',(-0.0374327802155412,1.77990623633773,
10.6530203475944));
#42083=CARTESIAN_POINT('Ctrl Pts',(-0.0377932934974776,1.77994866172931,
10.6529987466642));
#42084=CARTESIAN_POINT('Ctrl Pts',(-0.0379210005963382,1.77996376786914,
10.6529910975941));
#42085=CARTESIAN_POINT('Ctrl Pts',(-0.0394341395470693,1.78014367156438,
10.6529005000365));
#42086=CARTESIAN_POINT('Ctrl Pts',(-0.0408185170970988,1.78031739023526,
10.6528179351177));
#42087=CARTESIAN_POINT('Ctrl Pts',(-0.0739911911105266,1.78469906512859,
10.6508463323331));
#42088=CARTESIAN_POINT('Ctrl Pts',(-0.104978714780698,1.79361893231556,
10.6491381366845));
#42089=CARTESIAN_POINT('Ctrl Pts',(-0.144449100312507,1.81168743387289,
10.6466386064222));
#42090=CARTESIAN_POINT('Ctrl Pts',(-0.154499215229547,1.81694589126024,
10.6459724841665));
#42091=CARTESIAN_POINT('Ctrl Pts',(-0.165996547881922,1.82375655838926,
10.645164440796));
#42092=CARTESIAN_POINT('Ctrl Pts',(-0.1677325133804,1.82480716469213,10.6450411597027));
#42093=CARTESIAN_POINT('Ctrl Pts',(-0.170019579463829,1.82622097692943,
10.644876999074));
#42094=CARTESIAN_POINT('Ctrl Pts',(-0.170579677278318,1.82656959831804,
10.6448366566744));
#42095=CARTESIAN_POINT('Ctrl Pts',(-0.17149733033233,1.82714468954034,10.6447703289663));
#42096=CARTESIAN_POINT('Ctrl Pts',(-0.17185551879193,1.82737014944213,10.6447443810438));
#42097=CARTESIAN_POINT('Ctrl Pts',(-0.172548627551553,1.82780833190964,
10.644694057495));
#42098=CARTESIAN_POINT('Ctrl Pts',(-0.172883601350699,1.82802096876871,
10.6446696850796));
#42099=CARTESIAN_POINT('Ctrl Pts',(-0.173655975585981,1.82851326496984,
10.6446133683992));
#42100=CARTESIAN_POINT('Ctrl Pts',(-0.174093093761888,1.82879336318327,
10.6445814078448));
#42101=CARTESIAN_POINT('Ctrl Pts',(-0.175490378955381,1.8296934908691,10.6444789576728));
#42102=CARTESIAN_POINT('Ctrl Pts',(-0.17644791700731,1.83031756728649,10.6444083171237));
#42103=CARTESIAN_POINT('Ctrl Pts',(-0.185221654035153,1.83610259026258,
10.643757018908));
#42104=CARTESIAN_POINT('Ctrl Pts',(-0.192811980867188,1.84159641133959,
10.6431638111054));
#42105=CARTESIAN_POINT('Ctrl Pts',(-0.206178374068528,1.85218801574152,
10.6420618352222));
#42106=CARTESIAN_POINT('Ctrl Pts',(-0.212031769976707,1.8571773977429,10.641557348302));
#42107=CARTESIAN_POINT('Ctrl Pts',(-0.23299369306225,1.87638140299186,10.6396701529999));
#42108=CARTESIAN_POINT('Ctrl Pts',(-0.246898036763436,1.89183513913508,
10.6382508834874));
#42109=CARTESIAN_POINT('Ctrl Pts',(-0.266099788641974,1.9178293326402,10.636086655363));
#42110=CARTESIAN_POINT('Ctrl Pts',(-0.272473526524003,1.92750800428579,
10.6353232116672));
#42111=CARTESIAN_POINT('Ctrl Pts',(-0.279108542127127,1.93887245111991,
10.6344905536046));
#42112=CARTESIAN_POINT('Ctrl Pts',(-0.279894101009923,1.94024093841722,
10.6343912988104));
#42113=CARTESIAN_POINT('Ctrl Pts',(-0.280873484909639,1.94197647892662,
10.6342667492149));
#42114=CARTESIAN_POINT('Ctrl Pts',(-0.281076677249562,1.94233818075179,
10.6342408643287));
#42115=CARTESIAN_POINT('Ctrl Pts',(-0.281399310538288,1.94291510499665,
10.6341996936114));
#42116=CARTESIAN_POINT('Ctrl Pts',(-0.281519203475698,1.94313007208193,
10.6341843787205));
#42117=CARTESIAN_POINT('Ctrl Pts',(-0.281745284159368,1.94353652687675,
10.6341554704877));
#42118=CARTESIAN_POINT('Ctrl Pts',(-0.281851522159065,1.94372798387184,
10.6341418739827));
#42119=CARTESIAN_POINT('Ctrl Pts',(-0.282093176684477,1.94416453003825,
10.6341109186484));
#42120=CARTESIAN_POINT('Ctrl Pts',(-0.282228468728226,1.94440968709176,
10.6340935679099));
#42121=CARTESIAN_POINT('Ctrl Pts',(-0.282640045704719,1.94515779168168,
10.6340407219673));
#42122=CARTESIAN_POINT('Ctrl Pts',(-0.282915308897297,1.94566130453969,
10.634005292096));
#42123=CARTESIAN_POINT('Ctrl Pts',(-0.284891237555549,1.94929873249034,
10.6337503187314));
#42124=CARTESIAN_POINT('Ctrl Pts',(-0.286541217937032,1.95246009946763,
10.6335339297426));
#42125=CARTESIAN_POINT('Ctrl Pts',(-0.295789101613459,1.97091968191431,
10.6322965619018));
#42126=CARTESIAN_POINT('Ctrl Pts',(-0.302214540346773,1.98677705091995,
10.6313355261449));
#42127=CARTESIAN_POINT('Ctrl Pts',(-0.312263334152678,2.01864078124881,
10.629465696369));
#42128=CARTESIAN_POINT('Ctrl Pts',(-0.31598328516405,2.03456111486351,10.6285587985491));
#42129=CARTESIAN_POINT('Ctrl Pts',(-0.32037303737777,2.06291573048987,10.6269135315642));
#42130=CARTESIAN_POINT('Ctrl Pts',(-0.321559891740573,2.07523492808655,
10.6261893231636));
#42131=CARTESIAN_POINT('Ctrl Pts',(-0.322118447795861,2.08973037114639,
10.6253127410583));
#42132=CARTESIAN_POINT('Ctrl Pts',(-0.322179563960661,2.09187055286401,
10.6251827124183));
#42133=CARTESIAN_POINT('Ctrl Pts',(-0.32223186003238,2.09468424722614,10.6250109183032));
#42134=CARTESIAN_POINT('Ctrl Pts',(-0.322242261255481,2.09535738246266,
10.6249697555244));
#42135=CARTESIAN_POINT('Ctrl Pts',(-0.322255803055986,2.09645673960136,
10.6249024234368));
#42136=CARTESIAN_POINT('Ctrl Pts',(-0.322260207395294,2.09688294621664,
10.6248762937635));
#42137=CARTESIAN_POINT('Ctrl Pts',(-0.322267069478345,2.09770477124514,
10.624825859299));
#42138=CARTESIAN_POINT('Ctrl Pts',(-0.32226964426969,2.09810038812739,10.6248015582207));
#42139=CARTESIAN_POINT('Ctrl Pts',(-0.322273880357315,2.0990080855648,10.6247457500752));
#42140=CARTESIAN_POINT('Ctrl Pts',(-0.322275049623255,2.09952016637256,
10.6247142276505));
#42141=CARTESIAN_POINT('Ctrl Pts',(-0.322274887805991,2.10113743837012,
10.6246145509417));
#42142=CARTESIAN_POINT('Ctrl Pts',(-0.322269092092557,2.10224261220303,
10.624546257021));
#42143=CARTESIAN_POINT('Ctrl Pts',(-0.322101872276328,2.11833947907641,
10.6235488922284));
#42144=CARTESIAN_POINT('Ctrl Pts',(-0.320900231448132,2.13329980047741,
10.62258695804));
#42145=CARTESIAN_POINT('Ctrl Pts',(-0.316133179799011,2.16486808434016,
10.6204814041765));
#42146=CARTESIAN_POINT('Ctrl Pts',(-0.312287957371054,2.18138922386094,
10.6193332870512));
#42147=CARTESIAN_POINT('Ctrl Pts',(-0.303289733818903,2.2097283377801,10.617322755468));
#42148=CARTESIAN_POINT('Ctrl Pts',(-0.298693116954973,2.22168582585911,
10.6164613590884));
#42149=CARTESIAN_POINT('Ctrl Pts',(-0.293053731852387,2.23409464896252,
10.6155728443954));
#42150=CARTESIAN_POINT('Ctrl Pts',(-0.292707376819011,2.23484901265895,
10.6155188532204));
#42151=CARTESIAN_POINT('Ctrl Pts',(-0.29021861512046,2.24021478501449,10.6151350270138));
#42152=CARTESIAN_POINT('Ctrl Pts',(-0.287970100311195,2.24477658321316,
10.6148098210626));
#42153=CARTESIAN_POINT('Ctrl Pts',(-0.285320173614871,2.24984651363281,
10.6144512190946));
#42154=CARTESIAN_POINT('Ctrl Pts',(-0.285024265203572,2.25040860141961,
10.6144115017946));
#42155=CARTESIAN_POINT('Ctrl Pts',(-0.284591419897391,2.25122494084432,
10.6143538810633));
#42156=CARTESIAN_POINT('Ctrl Pts',(-0.284455802464262,2.25147988466644,
10.6143358948691));
#42157=CARTESIAN_POINT('Ctrl Pts',(-0.284215886085028,2.25192943912444,
10.6143041950273));
#42158=CARTESIAN_POINT('Ctrl Pts',(-0.284111729658993,2.25212412513184,
10.6142904722913));
#42159=CARTESIAN_POINT('Ctrl Pts',(-0.283894350902737,2.25252944087545,
10.6142619142993));
#42160=CARTESIAN_POINT('Ctrl Pts',(-0.283781094439752,2.25274005122342,
10.6142470813055));
#42161=CARTESIAN_POINT('Ctrl Pts',(-0.283485564342004,2.25328815204493,
10.6142084952888));
#42162=CARTESIAN_POINT('Ctrl Pts',(-0.283302921747109,2.25362544477016,
10.614184765834));
#42163=CARTESIAN_POINT('Ctrl Pts',(-0.282514127177264,2.25507594986013,
10.6140827833769));
#42164=CARTESIAN_POINT('Ctrl Pts',(-0.28190200207261,2.25618592648598,10.6140049066545));
#42165=CARTESIAN_POINT('Ctrl Pts',(-0.270885211488913,2.27588708081191,
10.6126250639713));
#42166=CARTESIAN_POINT('Ctrl Pts',(-0.258666983423515,2.2934082683905,10.6114342541627));
#42167=CARTESIAN_POINT('Ctrl Pts',(-0.230280174730862,2.32656366791077,
10.6089940764318));
#42168=CARTESIAN_POINT('Ctrl Pts',(-0.214031094273961,2.3419723542264,10.6077488458138));
#42169=CARTESIAN_POINT('Ctrl Pts',(-0.195078654313094,2.3565305939115,10.6063361835187));
#42170=CARTESIAN_POINT('Ctrl Pts',(-0.193830089353779,2.35747528681586,
10.6062433144724));
#42171=CARTESIAN_POINT('Ctrl Pts',(-0.188672568959996,2.36131880978429,
10.6058604076998));
#42172=CARTESIAN_POINT('Ctrl Pts',(-0.184705237869046,2.36413789928119,
10.6055675176712));
#42173=CARTESIAN_POINT('Ctrl Pts',(-0.179972230122461,2.36734227841042,
10.6052194089959));
#42174=CARTESIAN_POINT('Ctrl Pts',(-0.179266829279648,2.36781579740422,
10.6051675612142));
#42175=CARTESIAN_POINT('Ctrl Pts',(-0.178133045596116,2.36857039337862,
10.6050842774087));
#42176=CARTESIAN_POINT('Ctrl Pts',(-0.177705847259194,2.36885324989294,
10.6050529083604));
#42177=CARTESIAN_POINT('Ctrl Pts',(-0.176947551250084,2.36935273580443,
10.6049972463795));
#42178=CARTESIAN_POINT('Ctrl Pts',(-0.176616724968369,2.36956977693718,
10.6049729689409));
#42179=CARTESIAN_POINT('Ctrl Pts',(-0.175928790754885,2.37001929149389,
10.6049224985648));
#42180=CARTESIAN_POINT('Ctrl Pts',(-0.175571619964615,2.37025166688767,
10.604896302027));
#42181=CARTESIAN_POINT('Ctrl Pts',(-0.174649415671359,2.37084905339973,
10.60482868164));
#42182=CARTESIAN_POINT('Ctrl Pts',(-0.174083700411648,2.37121300367405,
10.604787218368));
#42183=CARTESIAN_POINT('Ctrl Pts',(-0.171716491882821,2.37272547833394,
10.6046137871584));
#42184=CARTESIAN_POINT('Ctrl Pts',(-0.169904772413769,2.37385782456362,
10.6044812212612));
#42185=CARTESIAN_POINT('Ctrl Pts',(-0.157566280887133,2.38139996513841,
10.6035793654261));
#42186=CARTESIAN_POINT('Ctrl Pts',(-0.146691831263112,2.38721858357531,
10.6027886524027));
#42187=CARTESIAN_POINT('Ctrl Pts',(-0.120714326350644,2.39925780171569,
10.6009084360497));
#42188=CARTESIAN_POINT('Ctrl Pts',(-0.105418495876552,2.40498202632303,
10.5998069942132));
#42189=CARTESIAN_POINT('Ctrl Pts',(-0.0706824252419293,2.41505490133353,
10.5973595269109));
#42190=CARTESIAN_POINT('Ctrl Pts',(-0.0511353081470509,2.41881181000973,
10.5960171592826));
#42191=CARTESIAN_POINT('Ctrl Pts',(-0.0301904195768933,2.42085994815445,
10.594690072508));
#42192=CARTESIAN_POINT('Ctrl Pts',(-0.0290154878773678,2.42096833072649,
10.5946160029913));
#42193=CARTESIAN_POINT('Ctrl Pts',(-0.0274533135494249,2.42110378668643,
10.594518043206));
#42194=CARTESIAN_POINT('Ctrl Pts',(-0.0270665983569622,2.42113661501977,
10.5944938358132));
#42195=CARTESIAN_POINT('Ctrl Pts',(-0.0264643920446245,2.42118664092582,
10.594456206358));
#42196=CARTESIAN_POINT('Ctrl Pts',(-0.0262489429777537,2.42120432025226,
10.5944427571859));
#42197=CARTESIAN_POINT('Ctrl Pts',(-0.0258373323102506,2.42123767931074,
10.5944170886015));
#42198=CARTESIAN_POINT('Ctrl Pts',(-0.0256411754988713,2.42125339604306,
10.5944048672057));
#42199=CARTESIAN_POINT('Ctrl Pts',(-0.0251792841491755,2.42128997856143,
10.5943761156927));
#42200=CARTESIAN_POINT('Ctrl Pts',(-0.0249135384118099,2.42131069431207,
10.5943595941566));
#42201=CARTESIAN_POINT('Ctrl Pts',(-0.0241409223233759,2.42136995798687,
10.5943116188553));
#42202=CARTESIAN_POINT('Ctrl Pts',(-0.0236339831433821,2.42140763661781,
10.5942802139651));
#42203=CARTESIAN_POINT('Ctrl Pts',(-0.0200708746813913,2.42166399172676,
10.5940599811173));
#42204=CARTESIAN_POINT('Ctrl Pts',(-0.017011680900007,2.4218402833017,10.5938734883344));
#42205=CARTESIAN_POINT('Ctrl Pts',(-0.00765904737650977,2.42224551019416,
10.5933099911903));
#42206=CARTESIAN_POINT('Ctrl Pts',(-0.00136071564873546,2.42233366108226,
10.5929396977314));
#42207=CARTESIAN_POINT('Ctrl Pts',(0.0336364142372838,2.42179751739353,
10.5909134702201));
#42208=CARTESIAN_POINT('Ctrl Pts',(0.0621499220440724,2.41752587772587,
10.5893682522793));
#42209=CARTESIAN_POINT('Ctrl Pts',(0.095190739864799,2.40794855632652,10.5873889479673));
#42210=CARTESIAN_POINT('Ctrl Pts',(0.100615844160285,2.40621893677704,10.5870580450734));
#42211=CARTESIAN_POINT('Ctrl Pts',(0.112766068418738,2.4019874858033,10.5863006353681));
#42212=CARTESIAN_POINT('Ctrl Pts',(0.119458951637307,2.39940303035856,10.5858718325772));
#42213=CARTESIAN_POINT('Ctrl Pts',(0.127037746239446,2.39618189693642,10.5853707473604));
#42214=CARTESIAN_POINT('Ctrl Pts',(0.12801374092245,2.39576136856441,10.5853059182461));
#42215=CARTESIAN_POINT('Ctrl Pts',(0.12945447431168,2.39513213011022,10.5852097691087));
#42216=CARTESIAN_POINT('Ctrl Pts',(0.129920833710825,2.3949271301625,10.5851785759291));
#42217=CARTESIAN_POINT('Ctrl Pts',(0.130747017803886,2.39456162037406,10.5851231900771));
#42218=CARTESIAN_POINT('Ctrl Pts',(0.131107038721515,2.39440155444136,10.5850990126554));
#42219=CARTESIAN_POINT('Ctrl Pts',(0.131860726772466,2.39406480671901,10.5850483092035));
#42220=CARTESIAN_POINT('Ctrl Pts',(0.132254334155832,2.39388799381697,10.5850217787077));
#42221=CARTESIAN_POINT('Ctrl Pts',(0.133282653787309,2.3934235767643,10.5849523322017));
#42222=CARTESIAN_POINT('Ctrl Pts',(0.133916787902301,2.39313470471352,10.5849093726236));
#42223=CARTESIAN_POINT('Ctrl Pts',(0.136641973021836,2.39188259140979,10.5847241725702));
#42224=CARTESIAN_POINT('Ctrl Pts',(0.138723564965764,2.39089903410002,10.5845812320817));
#42225=CARTESIAN_POINT('Ctrl Pts',(0.153393941048295,2.38377397492711,10.5835631032709));
#42226=CARTESIAN_POINT('Ctrl Pts',(0.165579396523631,2.37684063854556,10.5826600642274));
#42227=CARTESIAN_POINT('Ctrl Pts',(0.201385022007874,2.35325639864308,10.5798267934464));
#42228=CARTESIAN_POINT('Ctrl Pts',(0.223250001140489,2.33420923502168,10.5778247748898));
#42229=CARTESIAN_POINT('Ctrl Pts',(0.242545427619116,2.31220991204856,10.5759144852643));
#42230=CARTESIAN_POINT('Ctrl Pts',(0.242804994717016,2.31191287307241,10.5758887599422));
#42231=CARTESIAN_POINT('Ctrl Pts',(0.246848734076133,2.30726818401922,10.5754875684628));
#42232=CARTESIAN_POINT('Ctrl Pts',(0.250516448660152,2.30281991238011,10.5751178834493));
#42233=CARTESIAN_POINT('Ctrl Pts',(0.25446721754494,2.29775753388324,10.5747152442235));
#42234=CARTESIAN_POINT('Ctrl Pts',(0.25486972589158,2.29723851006993,10.5746741697713));
#42235=CARTESIAN_POINT('Ctrl Pts',(0.255449341274268,2.29648637450622,10.5746149495273));
#42236=CARTESIAN_POINT('Ctrl Pts',(0.255627718487173,2.29625425056984,10.5745967144107));
#42237=CARTESIAN_POINT('Ctrl Pts',(0.255940473772509,2.29584610935328,10.5745647249529));
#42238=CARTESIAN_POINT('Ctrl Pts',(0.256074986949946,2.29567019630872,10.5745509609879));
#42239=CARTESIAN_POINT('Ctrl Pts',(0.256353339706178,2.29530539473941,10.5745224673296));
#42240=CARTESIAN_POINT('Ctrl Pts',(0.256497151634962,2.29511648622516,10.5745077396035));
#42241=CARTESIAN_POINT('Ctrl Pts',(0.256863539178482,2.29463410167027,10.5744702012048));
#42242=CARTESIAN_POINT('Ctrl Pts',(0.257085821427088,2.29434040165818,10.5744474113197));
#42243=CARTESIAN_POINT('Ctrl Pts',(0.257991893972917,2.29313893927685,10.5743544467344));
#42244=CARTESIAN_POINT('Ctrl Pts',(0.258671394440155,2.29222792983773,10.5742845703029));
#42245=CARTESIAN_POINT('Ctrl Pts',(0.263310484633149,2.28593913735411,10.5738062662536));
#42246=CARTESIAN_POINT('Ctrl Pts',(0.267107221845943,2.28044256921731,10.5734085171922));
#42247=CARTESIAN_POINT('Ctrl Pts',(0.274541894537162,2.2689298065942,10.5726074331073));
#42248=CARTESIAN_POINT('Ctrl Pts',(0.278159303437135,2.26290470701461,10.5722050891743));
#42249=CARTESIAN_POINT('Ctrl Pts',(0.291810712716592,2.23838455480655,10.5706148842395));
#42250=CARTESIAN_POINT('Ctrl Pts',(0.300219878349783,2.21904548873031,10.569461277327));
#42251=CARTESIAN_POINT('Ctrl Pts',(0.311284802758755,2.18477681716413,10.5674062770849));
#42252=CARTESIAN_POINT('Ctrl Pts',(0.314886195136794,2.17022769700975,10.5665314504221));
#42253=CARTESIAN_POINT('Ctrl Pts',(0.317677709120912,2.15425496251369,10.565546258926));
#42254=CARTESIAN_POINT('Ctrl Pts',(0.317885075620312,2.15302646942378,10.5654703384502));
#42255=CARTESIAN_POINT('Ctrl Pts',(0.318166089919634,2.15130075490805,10.5653634730838));
#42256=CARTESIAN_POINT('Ctrl Pts',(0.318245707636989,2.15080450565649,10.5653327176017));
#42257=CARTESIAN_POINT('Ctrl Pts',(0.318381794601162,2.14994341586929,10.565279306535));
#42258=CARTESIAN_POINT('Ctrl Pts',(0.318438798537131,2.14957865978964,10.5652566679368));
#42259=CARTESIAN_POINT('Ctrl Pts',(0.318556050739551,2.14881984305812,10.5652095429882));
#42260=CARTESIAN_POINT('Ctrl Pts',(0.318616194840782,2.14842576712818,10.5651850533784));
#42261=CARTESIAN_POINT('Ctrl Pts',(0.318756017143791,2.14749808672523,10.5651273645859));
#42262=CARTESIAN_POINT('Ctrl Pts',(0.318835086673455,2.14696439298249,10.565094146193));
#42263=CARTESIAN_POINT('Ctrl Pts',(0.319084133879111,2.14525378604073,10.5649875760334));
#42264=CARTESIAN_POINT('Ctrl Pts',(0.319248936517816,2.144076139984,10.5649140608115));
#42265=CARTESIAN_POINT('Ctrl Pts',(0.319619739695642,2.14131521275585,10.5647413505592));
#42266=CARTESIAN_POINT('Ctrl Pts',(0.319820497828673,2.13973127016687,10.5646419915434));
#42267=CARTESIAN_POINT('Ctrl Pts',(0.321799984932654,2.12312518055891,10.5635973333809));
#42268=CARTESIAN_POINT('Ctrl Pts',(0.322530461533653,2.10799925431078,10.562618927519));
#42269=CARTESIAN_POINT('Ctrl Pts',(0.321708972110891,2.07082628030248,10.5601524719535));
#42270=CARTESIAN_POINT('Ctrl Pts',(0.318958807320579,2.04888302401824,10.5586401747953));
#42271=CARTESIAN_POINT('Ctrl Pts',(0.313075447295526,2.02344018879822,10.5568965820186));
#42272=CARTESIAN_POINT('Ctrl Pts',(0.312086665109935,2.01950431042533,10.5566273229405));
#42273=CARTESIAN_POINT('Ctrl Pts',(0.310772070619766,2.0146605641952,10.5562973093378));
#42274=CARTESIAN_POINT('Ctrl Pts',(0.310516205919494,2.01373421838026,10.5562342575917));
#42275=CARTESIAN_POINT('Ctrl Pts',(0.31007843366465,2.01217647056235,10.5561283486323));
#42276=CARTESIAN_POINT('Ctrl Pts',(0.309898733082624,2.01154445979593,10.5560854122902));
#42277=CARTESIAN_POINT('Ctrl Pts',(0.309582155672909,2.01044385661525,10.5560107043556));
#42278=CARTESIAN_POINT('Ctrl Pts',(0.309446145197896,2.00997501926407,10.5559788999947));
#42279=CARTESIAN_POINT('Ctrl Pts',(0.309213486176365,2.00917978493676,10.5559249897273));
#42280=CARTESIAN_POINT('Ctrl Pts',(0.309117385196703,2.0088532300715,10.5559028622814));
#42281=CARTESIAN_POINT('Ctrl Pts',(0.308986956979781,2.00841260878144,10.555873020056));
#42282=CARTESIAN_POINT('Ctrl Pts',(0.308953083959704,2.00829840936104,10.5558652869088));
#42283=CARTESIAN_POINT('Ctrl Pts',(0.308563903481817,2.00698899051464,10.5557766332601));
#42284=CARTESIAN_POINT('Ctrl Pts',(0.308201720128999,2.00579580570652,10.5556959942204));
#42285=CARTESIAN_POINT('Ctrl Pts',(0.306670808935692,2.00085568214609,10.5553628113027));
#42286=CARTESIAN_POINT('Ctrl Pts',(0.305440544302357,1.99712795249222,10.5551130357275));
#42287=CARTESIAN_POINT('Ctrl Pts',(0.303947183381552,1.99286628043021,10.554830121659));
#42288=CARTESIAN_POINT('Ctrl Pts',(0.303750417245472,1.99230966528624,10.5547932226244));
#42289=CARTESIAN_POINT('Ctrl Pts',(0.303456971511172,1.99148676433291,10.5547387517394));
#42290=CARTESIAN_POINT('Ctrl Pts',(0.30336146995417,1.99122006424714,10.554721110437));
#42291=CARTESIAN_POINT('Ctrl Pts',(0.303191399953817,1.99074708823794,10.5546898474431));
#42292=CARTESIAN_POINT('Ctrl Pts',(0.303116972585147,1.99054076253522,10.5546762173379));
#42293=CARTESIAN_POINT('Ctrl Pts',(0.302959213473314,1.99010482147521,10.5546474350154));
#42294=CARTESIAN_POINT('Ctrl Pts',(0.302875831530322,1.98987522546161,10.5546322858942));
#42295=CARTESIAN_POINT('Ctrl Pts',(0.302655786487334,1.98927146163625,10.5545924732672));
#42296=CARTESIAN_POINT('Ctrl Pts',(0.302518690019417,1.98889745054488,10.5545678356814));
#42297=CARTESIAN_POINT('Ctrl Pts',(0.301892668864792,1.98719936021826,10.5544560852029));
#42298=CARTESIAN_POINT('Ctrl Pts',(0.30139573267332,1.98587822141475,10.5543694443169));
#42299=CARTESIAN_POINT('Ctrl Pts',(0.300046290324357,1.98236093844937,10.5541394808833));
#42300=CARTESIAN_POINT('Ctrl Pts',(0.299178340854831,1.98017076224843,10.5539970189566));
#42301=CARTESIAN_POINT('Ctrl Pts',(0.294929597163461,1.96978354019558,10.5533239896147));
#42302=CARTESIAN_POINT('Ctrl Pts',(0.291235219924701,1.96171816118037,10.5528091740582));
#42303=CARTESIAN_POINT('Ctrl Pts',(0.279803782528578,1.93925861825843,10.5513703368679));
#42304=CARTESIAN_POINT('Ctrl Pts',(0.27129888416226,1.92528621808786,10.5504678513984));
#42305=CARTESIAN_POINT('Ctrl Pts',(0.24911055958682,1.89438818792162,10.5483326841923));
#42306=CARTESIAN_POINT('Ctrl Pts',(0.234703613114626,1.87808494617109,10.5470916570029));
#42307=CARTESIAN_POINT('Ctrl Pts',(0.217792534424859,1.86245135971162,10.5456931832354));
#42308=CARTESIAN_POINT('Ctrl Pts',(0.216810342469333,1.86155457674852,10.5456121670436));
#42309=CARTESIAN_POINT('Ctrl Pts',(0.215438789395028,1.86031777120266,10.5454993079632));
#42310=CARTESIAN_POINT('Ctrl Pts',(0.215054109500165,1.85997255832002,10.5454676839457));
#42311=CARTESIAN_POINT('Ctrl Pts',(0.214390468380293,1.85937988082783,10.5454131769422));
#42312=CARTESIAN_POINT('Ctrl Pts',(0.214111904214357,1.85913197149775,10.5453903126606));
#42313=CARTESIAN_POINT('Ctrl Pts',(0.21353637839345,1.85862156720664,10.5453431048006));
#42314=CARTESIAN_POINT('Ctrl Pts',(0.213239361619447,1.85835913555627,10.5453187586313));
#42315=CARTESIAN_POINT('Ctrl Pts',(0.212547360771013,1.85774998187117,10.5452620746047));
#42316=CARTESIAN_POINT('Ctrl Pts',(0.212152011984379,1.85740367756311,10.5452297194353));
#42317=CARTESIAN_POINT('Ctrl Pts',(0.21091961347521,1.85632947908972,10.5451289495501));
#42318=CARTESIAN_POINT('Ctrl Pts',(0.210079658207441,1.85560494426572,10.5450603959269));
#42319=CARTESIAN_POINT('Ctrl Pts',(0.202601837551441,1.84922170495013,10.5444511773602));
#42320=CARTESIAN_POINT('Ctrl Pts',(0.19574109711567,1.84383080405913,10.5438996492481));
#42321=CARTESIAN_POINT('Ctrl Pts',(0.182445252792877,1.834229665401,10.5428428548966));
#42322=CARTESIAN_POINT('Ctrl Pts',(0.17606154320618,1.82995841072312,10.5423403043375));
#42323=CARTESIAN_POINT('Ctrl Pts',(0.154077303472251,1.81636012076571,10.5406277681789));
#42324=CARTESIAN_POINT('Ctrl Pts',(0.137842674218888,1.8081255148071,10.5393904728125));
#42325=CARTESIAN_POINT('Ctrl Pts',(0.106504061008595,1.79543021926908,10.5371108478022));
#42326=CARTESIAN_POINT('Ctrl Pts',(0.0915954623321869,1.79061953914345,
10.5360690606917));
#42327=CARTESIAN_POINT('Ctrl Pts',(0.075517958927093,1.78669658828385,10.5350283790326));
#42328=CARTESIAN_POINT('Ctrl Pts',(0.0746403921908587,1.78648636104104,
10.5349718332031));
#42329=CARTESIAN_POINT('Ctrl Pts',(0.0734573570829739,1.78620820562718,
10.5348959628036));
#42330=CARTESIAN_POINT('Ctrl Pts',(0.0731526667984573,1.78613703489003,
10.5348764543548));
#42331=CARTESIAN_POINT('Ctrl Pts',(0.0726390404861891,1.78601784862661,
10.5348436227112));
#42332=CARTESIAN_POINT('Ctrl Pts',(0.0724301601614801,1.78596959783579,
10.5348302859608));
#42333=CARTESIAN_POINT('Ctrl Pts',(0.0720290773354552,1.7858773702539,10.534804706592));
#42334=CARTESIAN_POINT('Ctrl Pts',(0.0718368840411786,1.78583336174587,
10.5347924622396));
#42335=CARTESIAN_POINT('Ctrl Pts',(0.071439914866234,1.78574284688465,10.534767198483));
#42336=CARTESIAN_POINT('Ctrl Pts',(0.0712351345868771,1.78569636444793,
10.5347541805086));
#42337=CARTESIAN_POINT('Ctrl Pts',(0.0707724429555244,1.78559181494002,
10.5347247996032));
#42338=CARTESIAN_POINT('Ctrl Pts',(0.0705145048948518,1.78553386491512,
10.5347084434182));
#42339=CARTESIAN_POINT('Ctrl Pts',(0.0693220148394745,1.78526749340417,
10.5346329305535));
#42340=CARTESIAN_POINT('Ctrl Pts',(0.068386595416225,1.78506291728116,10.5345739927676));
#42341=CARTESIAN_POINT('Ctrl Pts',(0.0591054079231446,1.78307642386444,
10.533992025009));
#42342=CARTESIAN_POINT('Ctrl Pts',(0.0506920417893542,1.78162231783749,
10.5334869485133));
#42343=CARTESIAN_POINT('Ctrl Pts',(0.0278578942360343,1.77860416692022,
10.5321524706262));
#42344=CARTESIAN_POINT('Ctrl Pts',(0.013372957283202,1.77767630779857,10.531344018866));
#42345=CARTESIAN_POINT('Ctrl Pts',(-0.0275380678385514,1.77781925070106,
10.5290573279285));
#42346=CARTESIAN_POINT('Ctrl Pts',(-0.0538341553457881,1.78115771537185,
10.5275746766322));
#42347=CARTESIAN_POINT('Ctrl Pts',(-0.0809851227926357,1.78806223254299,
10.5258766317182));
#42348=CARTESIAN_POINT('Ctrl Pts',(-0.0825403888697342,1.78847015401542,
10.5257788067047));
#42349=CARTESIAN_POINT('Ctrl Pts',(-0.0846932386512311,1.78905206515365,
10.5256425980039));
#42350=CARTESIAN_POINT('Ctrl Pts',(-0.0852934866823589,1.7892161780603,
10.5256045347661));
#42351=CARTESIAN_POINT('Ctrl Pts',(-0.0862532940489387,1.7894815876104,
10.5255435317106));
#42352=CARTESIAN_POINT('Ctrl Pts',(-0.0866131611832705,1.78958177328774,
10.5255206280355));
#42353=CARTESIAN_POINT('Ctrl Pts',(-0.087354164912857,1.78978945485657,
10.5254734019636));
#42354=CARTESIAN_POINT('Ctrl Pts',(-0.08773527906754,1.78989702798817,10.5254490770859));
#42355=CARTESIAN_POINT('Ctrl Pts',(-0.0886196317688793,1.79014840581414,
10.5253925497597));
#42356=CARTESIAN_POINT('Ctrl Pts',(-0.0891227191391028,1.79029273421104,
10.525360330295));
#42357=CARTESIAN_POINT('Ctrl Pts',(-0.0901741305228367,1.79059714271747,
10.5252928627609));
#42358=CARTESIAN_POINT('Ctrl Pts',(-0.0907223845407319,1.7907574562796,
10.5252576071557));
#42359=CARTESIAN_POINT('Ctrl Pts',(-0.0944597070016526,1.79186107132695,
10.5250167625057));
#42360=CARTESIAN_POINT('Ctrl Pts',(-0.0976343366093973,1.79285220073833,
10.5248096142726));
#42361=CARTESIAN_POINT('Ctrl Pts',(-0.106445393299578,1.79575344237772,
10.5242272700972));
#42362=CARTESIAN_POINT('Ctrl Pts',(-0.112044860295305,1.79777073045438,
10.523848611848));
#42363=CARTESIAN_POINT('Ctrl Pts',(-0.129604033082161,1.80465171211856,
10.5226332916566));
#42364=CARTESIAN_POINT('Ctrl Pts',(-0.141327994616978,1.81007905776409,
10.5217793971582));
#42365=CARTESIAN_POINT('Ctrl Pts',(-0.161938767634362,1.82116811827667,
10.5202083379808));
#42366=CARTESIAN_POINT('Ctrl Pts',(-0.170934887300376,1.82659071321151,
10.5194964845861));
#42367=CARTESIAN_POINT('Ctrl Pts',(-0.191661696099379,1.84050762106991,
10.5178086440866));
#42368=CARTESIAN_POINT('Ctrl Pts',(-0.203117712482278,1.84937324099307,
10.5168361074261));
#42369=CARTESIAN_POINT('Ctrl Pts',(-0.216977054017489,1.86167537853919,
10.5156411938572));
#42370=CARTESIAN_POINT('Ctrl Pts',(-0.219963097604545,1.86442855296617,
10.515382606792));
#42371=CARTESIAN_POINT('Ctrl Pts',(-0.223284232364362,1.86760891701959,
10.5150944976478));
#42372=CARTESIAN_POINT('Ctrl Pts',(-0.22367107175575,1.86798121726714,10.5150609313825));
#42373=CARTESIAN_POINT('Ctrl Pts',(-0.224255567306875,1.86854656518548,
10.5150102049987));
#42374=CARTESIAN_POINT('Ctrl Pts',(-0.224453906178619,1.86873890089742,
10.514992990197));
#42375=CARTESIAN_POINT('Ctrl Pts',(-0.22479864712963,1.86907406878476,10.5149630659779));
#42376=CARTESIAN_POINT('Ctrl Pts',(-0.224945160625977,1.86921678533643,
10.5149503475301));
#42377=CARTESIAN_POINT('Ctrl Pts',(-0.225252079722071,1.86951632047462,
10.514923703264));
#42378=CARTESIAN_POINT('Ctrl Pts',(-0.2254124574173,1.86967316702536,10.5149097797504));
#42379=CARTESIAN_POINT('Ctrl Pts',(-0.225732110340787,1.86998643556904,
10.5148820265226));
#42380=CARTESIAN_POINT('Ctrl Pts',(-0.225891387297782,1.87014285608982,
10.5148681966655));
#42381=CARTESIAN_POINT('Ctrl Pts',(-0.226266301135242,1.87051181236128,
10.5148356406512));
#42382=CARTESIAN_POINT('Ctrl Pts',(-0.226481801758825,1.87072448720158,
10.51481692539));
#42383=CARTESIAN_POINT('Ctrl Pts',(-0.227791668892591,1.87202082732957,
10.5147031543778));
#42384=CARTESIAN_POINT('Ctrl Pts',(-0.228878580045845,1.87311204658134,
10.5146086850561));
#42385=CARTESIAN_POINT('Ctrl Pts',(-0.238322141041879,1.88272996201918,
10.5137868732515));
#42386=CARTESIAN_POINT('Ctrl Pts',(-0.246207834619344,1.89170817784276,
10.5130934479709));
#42387=CARTESIAN_POINT('Ctrl Pts',(-0.258428329101278,1.90728844259288,
10.5119666122913));
#42388=CARTESIAN_POINT('Ctrl Pts',(-0.263051139700552,1.91364804661381,
10.5115257644934));
#42389=CARTESIAN_POINT('Ctrl Pts',(-0.272793876415334,1.92813714314506,
10.5105489647993));
#42390=CARTESIAN_POINT('Ctrl Pts',(-0.277792130959398,1.93633916329057,
10.5100140008736));
#42391=CARTESIAN_POINT('Ctrl Pts',(-0.29193191614421,1.9620613018615,10.5083603983596));
#42392=CARTESIAN_POINT('Ctrl Pts',(-0.299834191301724,1.98020596888851,
10.507223475659));
#42393=CARTESIAN_POINT('Ctrl Pts',(-0.30643168634884,2.00018780500769,10.5059453785795));
#42394=CARTESIAN_POINT('Ctrl Pts',(-0.306830285453337,2.0014199385275,10.5058664820753));
#42395=CARTESIAN_POINT('Ctrl Pts',(-0.307375796135252,2.00314156359891,
10.5057561119614));
#42396=CARTESIAN_POINT('Ctrl Pts',(-0.307528989687556,2.003629064294,10.5057248447093));
#42397=CARTESIAN_POINT('Ctrl Pts',(-0.30779150984991,2.00447147023506,10.5056707887805));
#42398=CARTESIAN_POINT('Ctrl Pts',(-0.307901383990714,2.00482620492242,
10.5056480180975));
#42399=CARTESIAN_POINT('Ctrl Pts',(-0.308127513809282,2.00556076745532,
10.5056008493205));
#42400=CARTESIAN_POINT('Ctrl Pts',(-0.308243680835297,2.00594062177102,
10.5055764483671));
#42401=CARTESIAN_POINT('Ctrl Pts',(-0.308513512481653,2.00682881207109,
10.5055193711379));
#42402=CARTESIAN_POINT('Ctrl Pts',(-0.308666623148082,2.00733731391317,
10.505486676808));
#42403=CARTESIAN_POINT('Ctrl Pts',(-0.308984852165373,2.00840373753051,
10.5054180745856));
#42404=CARTESIAN_POINT('Ctrl Pts',(-0.309149717700978,2.00896173219829,
10.5053821585542));
#42405=CARTESIAN_POINT('Ctrl Pts',(-0.309588072645398,2.01046028618344,
10.5052856453655));
#42406=CARTESIAN_POINT('Ctrl Pts',(-0.309858784942062,2.01140164541683,
10.5052249578356));
#42407=CARTESIAN_POINT('Ctrl Pts',(-0.310673289159565,2.01428335237103,
10.5050389893905));
#42408=CARTESIAN_POINT('Ctrl Pts',(-0.31120316940756,2.0162275502832,10.5049132583973));
#42409=CARTESIAN_POINT('Ctrl Pts',(-0.313069312008367,2.02333681113125,
10.5044524816794));
#42410=CARTESIAN_POINT('Ctrl Pts',(-0.314295436241986,2.02852964265951,
10.5041139380964));
#42411=CARTESIAN_POINT('Ctrl Pts',(-0.319988664784006,2.0556331378746,10.5023360342051));
#42412=CARTESIAN_POINT('Ctrl Pts',(-0.32229453126736,2.07793112920496,10.500830560742));
#42413=CARTESIAN_POINT('Ctrl Pts',(-0.322274875394328,2.10028339825448,
10.4993179956939));
#42414=CARTESIAN_POINT('',(-0.322700899340442,2.0998332352938,10.3743773449273));
#42415=CARTESIAN_POINT('Ctrl Pts',(-0.322700899340442,2.0998332352938,10.3743773449273));
#42416=CARTESIAN_POINT('Ctrl Pts',(-0.322760860387383,2.0903049967056,10.3749677204787));
#42417=CARTESIAN_POINT('Ctrl Pts',(-0.318052407360913,1.97393915136881,
10.3821815438711));
#42418=CARTESIAN_POINT('Ctrl Pts',(-0.176976240170584,1.76251740973093,
10.3960188151044));
#42419=CARTESIAN_POINT('Ctrl Pts',(0.187960967754062,1.7685097845779,10.4158891586272));
#42420=CARTESIAN_POINT('Ctrl Pts',(0.38046957633948,2.07859930375687,10.43575950215));
#42421=CARTESIAN_POINT('Ctrl Pts',(0.223949144889084,2.4083210482972,10.4556298456727));
#42422=CARTESIAN_POINT('Ctrl Pts',(-0.138014139074013,2.45520020514535,
10.4755001891955));
#42423=CARTESIAN_POINT('Ctrl Pts',(-0.310736422666012,2.2504699430552,10.4900826889471));
#42424=CARTESIAN_POINT('Ctrl Pts',(-0.322577931129815,2.12189942032013,
10.4980417408576));
#42425=CARTESIAN_POINT('Ctrl Pts',(-0.322378175270278,2.10028753889625,
10.4993773449273));
#42426=CARTESIAN_POINT('',(-0.322274890758155,2.1002653522546,10.1245441658164));
#42427=CARTESIAN_POINT('Ctrl Pts',(-0.322274949351636,2.09981931961724,
10.3741325730749));
#42428=CARTESIAN_POINT('Ctrl Pts',(-0.32228888357138,2.12467342881166,10.3726881081679));
#42429=CARTESIAN_POINT('Ctrl Pts',(-0.319427720275429,2.14944844835512,
10.3713381024607));
#42430=CARTESIAN_POINT('Ctrl Pts',(-0.310180543568759,2.18884054883889,
10.3690438376053));
#42431=CARTESIAN_POINT('Ctrl Pts',(-0.305516975523145,2.203749193326,10.3681401976533));
#42432=CARTESIAN_POINT('Ctrl Pts',(-0.298888071275734,2.22055361361139,
10.3670506232369));
#42433=CARTESIAN_POINT('Ctrl Pts',(-0.297957186028004,2.22283634510533,
10.366901076289));
#42434=CARTESIAN_POINT('Ctrl Pts',(-0.29672498390221,2.22576152928336,10.3667073754916));
#42435=CARTESIAN_POINT('Ctrl Pts',(-0.296447590535905,2.22641401968239,
10.3666640354162));
#42436=CARTESIAN_POINT('Ctrl Pts',(-0.29599684421038,2.22746463192364,10.3665940339328));
#42437=CARTESIAN_POINT('Ctrl Pts',(-0.295824834774944,2.22786333055801,
10.366567418369));
#42438=CARTESIAN_POINT('Ctrl Pts',(-0.295495483213476,2.22862250863517,
10.3665166416145));
#42439=CARTESIAN_POINT('Ctrl Pts',(-0.295338285794573,2.22898305031636,
10.3664924854043));
#42440=CARTESIAN_POINT('Ctrl Pts',(-0.29497810100415,2.22980504495677,10.36643731608));
#42441=CARTESIAN_POINT('Ctrl Pts',(-0.294774690477397,2.2302663103707,10.3664062885217));
#42442=CARTESIAN_POINT('Ctrl Pts',(-0.294150004752996,2.23167392827167,
10.3663113910337));
#42443=CARTESIAN_POINT('Ctrl Pts',(-0.293725251432721,2.23261872157932,
10.3662474018934));
#42444=CARTESIAN_POINT('Ctrl Pts',(-0.290574359519416,2.23953796292447,
10.3657765898293));
#42445=CARTESIAN_POINT('Ctrl Pts',(-0.287670902185649,2.24542951321801,
10.3653636698464));
#42446=CARTESIAN_POINT('Ctrl Pts',(-0.269898940067852,2.27887384299062,
10.3629467531254));
#42447=CARTESIAN_POINT('Ctrl Pts',(-0.251259525838447,2.30422824573741,
10.360799342436));
#42448=CARTESIAN_POINT('Ctrl Pts',(-0.225064991562881,2.33074370695163,
10.3583024557819));
#42449=CARTESIAN_POINT('Ctrl Pts',(-0.22074620877351,2.33487874920317,10.3579051320033));
#42450=CARTESIAN_POINT('Ctrl Pts',(-0.212752015246372,2.34211744153673,
10.3571984501881));
#42451=CARTESIAN_POINT('Ctrl Pts',(-0.209117384443732,2.34526353261613,
10.35688720574));
#42452=CARTESIAN_POINT('Ctrl Pts',(-0.204199881916846,2.34933123481119,
10.3564807132202));
#42453=CARTESIAN_POINT('Ctrl Pts',(-0.202978858835254,2.35032626614653,
10.3563809404691));
#42454=CARTESIAN_POINT('Ctrl Pts',(-0.200943097520943,2.35196055122853,
10.3562165741361));
#42455=CARTESIAN_POINT('Ctrl Pts',(-0.200132500537109,2.35260488933306,
10.3561516403509));
#42456=CARTESIAN_POINT('Ctrl Pts',(-0.199039747335734,2.35346494967293,
10.356064807213));
#42457=CARTESIAN_POINT('Ctrl Pts',(-0.198760331187157,2.35368411949004,
10.3560426653862));
#42458=CARTESIAN_POINT('Ctrl Pts',(-0.198319477644181,2.35402874288414,
10.3560078280483));
#42459=CARTESIAN_POINT('Ctrl Pts',(-0.198158283219286,2.3541545046158,10.3559951105071));
#42460=CARTESIAN_POINT('Ctrl Pts',(-0.197823646432666,2.35441507186388,
10.3559687516828));
#42461=CARTESIAN_POINT('Ctrl Pts',(-0.197650187280385,2.35454985238201,
10.355955112282));
#42462=CARTESIAN_POINT('Ctrl Pts',(-0.197254415426059,2.3548567249601,10.3559240458154));
#42463=CARTESIAN_POINT('Ctrl Pts',(-0.197032015560026,2.3550287033027,10.355906626919));
#42464=CARTESIAN_POINT('Ctrl Pts',(-0.196338277321527,2.35556371110128,
10.3558524107671));
#42465=CARTESIAN_POINT('Ctrl Pts',(-0.195866155124501,2.35592572919409,
10.3558156850643));
#42466=CARTESIAN_POINT('Ctrl Pts',(-0.19218798343589,2.35872997081875,10.355530868397));
#42467=CARTESIAN_POINT('Ctrl Pts',(-0.188937202371077,2.36111330103821,
10.3552868210233));
#42468=CARTESIAN_POINT('Ctrl Pts',(-0.176407953253459,2.36994264559564,
10.354371411469));
#42469=CARTESIAN_POINT('Ctrl Pts',(-0.166836817887374,2.37596072621874,
10.353723361673));
#42470=CARTESIAN_POINT('Ctrl Pts',(-0.150673855232,2.38497457981584,10.3526774425168));
#42471=CARTESIAN_POINT('Ctrl Pts',(-0.144263074596166,2.38827294512693,
10.3522742943601));
#42472=CARTESIAN_POINT('Ctrl Pts',(-0.123884236810992,2.3979077095669,10.3510142095415));
#42473=CARTESIAN_POINT('Ctrl Pts',(-0.109571847785605,2.40346380995871,
10.3501588139026));
#42474=CARTESIAN_POINT('Ctrl Pts',(-0.0838887909432318,2.41137930242907,
10.3486126514736));
#42475=CARTESIAN_POINT('Ctrl Pts',(-0.0726849642575297,2.41418346665747,
10.3479348745162));
#42476=CARTESIAN_POINT('Ctrl Pts',(-0.0593414268293379,2.4167711802308,
10.3471130954248));
#42477=CARTESIAN_POINT('Ctrl Pts',(-0.0573234940589404,2.41714255830781,
10.3469884457075));
#42478=CARTESIAN_POINT('Ctrl Pts',(-0.0546494956259246,2.41760832354531,
10.3468227339911));
#42479=CARTESIAN_POINT('Ctrl Pts',(-0.0539964580017836,2.41771999790753,
10.3467822221186));
#42480=CARTESIAN_POINT('Ctrl Pts',(-0.0529250745727525,2.41789981403068,
10.3467156870208));
#42481=CARTESIAN_POINT('Ctrl Pts',(-0.0525069282532875,2.41796914592765,
10.3466897016421));
#42482=CARTESIAN_POINT('Ctrl Pts',(-0.0516973453375493,2.41810174054077,
10.3466393561319));
#42483=CARTESIAN_POINT('Ctrl Pts',(-0.051305926177642,2.4181651061742,10.3466149993161));
#42484=CARTESIAN_POINT('Ctrl Pts',(-0.0504032445082699,2.41830952943369,
10.346558791696));
#42485=CARTESIAN_POINT('Ctrl Pts',(-0.0498919026602835,2.41839007778071,
10.3465269248019));
#42486=CARTESIAN_POINT('Ctrl Pts',(-0.0482589475640513,2.41864327614353,
10.3464250714086));
#42487=CARTESIAN_POINT('Ctrl Pts',(-0.0471366248648717,2.41881123254212,
10.3463549364466));
#42488=CARTESIAN_POINT('Ctrl Pts',(-0.036996373656594,2.42027401329828,
10.3457200401463));
#42489=CARTESIAN_POINT('Ctrl Pts',(-0.027929024218799,2.42119171500596,
10.3451434158459));
#42490=CARTESIAN_POINT('Ctrl Pts',(0.00616481034600214,2.4231877736036,
10.3429390215637));
#42491=CARTESIAN_POINT('Ctrl Pts',(0.0312478486247287,2.42173211827196,
10.3412357634632));
#42492=CARTESIAN_POINT('Ctrl Pts',(0.0640096514840762,2.4159615054665,10.3389915977708));
#42493=CARTESIAN_POINT('Ctrl Pts',(0.0720576291801567,2.41422383712596,
10.3384396590112));
#42494=CARTESIAN_POINT('Ctrl Pts',(0.0851627889161504,2.41086419116731,
10.3375478688154));
#42495=CARTESIAN_POINT('Ctrl Pts',(0.0902620665210687,2.40942206140203,
10.3372026676597));
#42496=CARTESIAN_POINT('Ctrl Pts',(0.0972998478321883,2.40724289181015,
10.3367308506347));
#42497=CARTESIAN_POINT('Ctrl Pts',(0.0992700618918268,2.40661198651308,
10.336599277179));
#42498=CARTESIAN_POINT('Ctrl Pts',(0.102042765033955,2.40569457833011,10.3364149692848));
#42499=CARTESIAN_POINT('Ctrl Pts',(0.102850355345233,2.40542381301977,10.3363613901504));
#42500=CARTESIAN_POINT('Ctrl Pts',(0.104077455316809,2.40500697733076,10.3362801463517));
#42501=CARTESIAN_POINT('Ctrl Pts',(0.104497744595358,2.40486323869189,10.3362523498254));
#42502=CARTESIAN_POINT('Ctrl Pts',(0.10527292751445,2.40459633529156,10.3362011389486));
#42503=CARTESIAN_POINT('Ctrl Pts',(0.105627904785272,2.40447341833829,10.3361777102524));
#42504=CARTESIAN_POINT('Ctrl Pts',(0.106204906794605,2.40427249099568,10.3361396647962));
#42505=CARTESIAN_POINT('Ctrl Pts',(0.106427061142112,2.40419485804575,10.336125025662));
#42506=CARTESIAN_POINT('Ctrl Pts',(0.106857155987072,2.40404403042252,10.3360967016149));
#42507=CARTESIAN_POINT('Ctrl Pts',(0.107065105764317,2.40397086595448,10.3360830150157));
#42508=CARTESIAN_POINT('Ctrl Pts',(0.107543155856651,2.4038021187272,10.3360515694152));
#42509=CARTESIAN_POINT('Ctrl Pts',(0.107813204678027,2.40370638882533,10.3360338192235));
#42510=CARTESIAN_POINT('Ctrl Pts',(0.108533359442728,2.40345001880399,10.3359865184103));
#42511=CARTESIAN_POINT('Ctrl Pts',(0.108983238487022,2.40328873661888,10.3359570058469));
#42512=CARTESIAN_POINT('Ctrl Pts',(0.112049193641018,2.40218188522832,10.3357561118189));
#42513=CARTESIAN_POINT('Ctrl Pts',(0.114653393363298,2.4012034431985,10.3355866471551));
#42514=CARTESIAN_POINT('Ctrl Pts',(0.146073802186834,2.38893168298727,10.3335525475035));
#42515=CARTESIAN_POINT('Ctrl Pts',(0.173135203120958,2.37357619847468,10.3318963168215));
#42516=CARTESIAN_POINT('Ctrl Pts',(0.209717493048685,2.34518415853004,10.329268612545));
#42517=CARTESIAN_POINT('Ctrl Pts',(0.221152153919479,2.33492196932802,10.3283790017032));
#42518=CARTESIAN_POINT('Ctrl Pts',(0.233507469593503,2.32212923514616,10.3273061448079));
#42519=CARTESIAN_POINT('Ctrl Pts',(0.235183386320996,2.32035405545381,10.3271580378102));
#42520=CARTESIAN_POINT('Ctrl Pts',(0.237318084299341,2.31804082566691,10.3269659451595));
#42521=CARTESIAN_POINT('Ctrl Pts',(0.237795518183092,2.31752003657717,10.3269227566169));
#42522=CARTESIAN_POINT('Ctrl Pts',(0.238563232468572,2.31667705878603,10.326852941018));
#42523=CARTESIAN_POINT('Ctrl Pts',(0.238854583624589,2.31635584477576,10.3268263593625));
#42524=CARTESIAN_POINT('Ctrl Pts',(0.239409031984174,2.31574208174269,10.326775608335));
#42525=CARTESIAN_POINT('Ctrl Pts',(0.239672243716308,2.31544963685297,10.326751443858));
#42526=CARTESIAN_POINT('Ctrl Pts',(0.240272186324793,2.31478060273538,10.3266962011299));
#42527=CARTESIAN_POINT('Ctrl Pts',(0.240608567968258,2.31440370297245,10.3266651082944));
#42528=CARTESIAN_POINT('Ctrl Pts',(0.241635529617899,2.31324758038979,10.3265698171269));
#42529=CARTESIAN_POINT('Ctrl Pts',(0.242323215649973,2.31246580626568,10.3265054981333));
#42530=CARTESIAN_POINT('Ctrl Pts',(0.247396682743893,2.30664152290583,10.3260271590527));
#42531=CARTESIAN_POINT('Ctrl Pts',(0.251628174194777,2.30146733928063,10.3256068207285));
#42532=CARTESIAN_POINT('Ctrl Pts',(0.256946929484487,2.29453451538598,10.3250488904696));
#42533=CARTESIAN_POINT('Ctrl Pts',(0.258182660862609,2.29289146060889,10.3249170402512));
#42534=CARTESIAN_POINT('Ctrl Pts',(0.274202255765956,2.27116172203337,10.3231781984959));
#42535=CARTESIAN_POINT('Ctrl Pts',(0.286619670091613,2.24943898557834,10.3214847050039));
#42536=CARTESIAN_POINT('Ctrl Pts',(0.299703202609065,2.21878414318467,10.3192344285879));
#42537=CARTESIAN_POINT('Ctrl Pts',(0.302696397552957,2.21093505487075,10.318670453852));
#42538=CARTESIAN_POINT('Ctrl Pts',(0.307887253472908,2.19554160296507,10.3175975708367));
#42539=CARTESIAN_POINT('Ctrl Pts',(0.310122591076253,2.18801568214007,10.3170878336785));
#42540=CARTESIAN_POINT('Ctrl Pts',(0.312289642975818,2.1796056098065,10.3165398846622));
#42541=CARTESIAN_POINT('Ctrl Pts',(0.312495052782837,2.17879540751088,10.3164873172727));
#42542=CARTESIAN_POINT('Ctrl Pts',(0.312803334240926,2.17755927853038,10.3164074603327));
#42543=CARTESIAN_POINT('Ctrl Pts',(0.312908491284998,2.17713393342408,10.3163800442021));
#42544=CARTESIAN_POINT('Ctrl Pts',(0.313101115162584,2.17634792097324,10.3163294973434));
#42545=CARTESIAN_POINT('Ctrl Pts',(0.313188826877085,2.17598731522856,10.3163063527586));
#42546=CARTESIAN_POINT('Ctrl Pts',(0.313330929731969,2.17539866748338,10.3162686465582));
#42547=CARTESIAN_POINT('Ctrl Pts',(0.313385694975512,2.17517071750707,10.3162540633385));
#42548=CARTESIAN_POINT('Ctrl Pts',(0.313491543304857,2.17472801768963,10.316225777102));
#42549=CARTESIAN_POINT('Ctrl Pts',(0.313542654336369,2.17451327575281,10.3162120725404));
#42550=CARTESIAN_POINT('Ctrl Pts',(0.313660037091126,2.17401783528397,10.3161804915533));
#42551=CARTESIAN_POINT('Ctrl Pts',(0.313726152871029,2.17373709930849,10.316162624188));
#42552=CARTESIAN_POINT('Ctrl Pts',(0.313936242456229,2.17283963466513,10.3161055925557));
#42553=CARTESIAN_POINT('Ctrl Pts',(0.314078776384394,2.17222256535615,10.3160665109579));
#42554=CARTESIAN_POINT('Ctrl Pts',(0.315336291067836,2.16670430241477,10.3157181588576));
#42555=CARTESIAN_POINT('Ctrl Pts',(0.316338360191054,2.16177773979604,10.3154152068479));
#42556=CARTESIAN_POINT('Ctrl Pts',(0.323019288146932,2.12448445034314,10.3131685268737));
#42557=CARTESIAN_POINT('Ctrl Pts',(0.323833741487077,2.09144019812893,10.3114227468492));
#42558=CARTESIAN_POINT('Ctrl Pts',(0.318164550493345,2.04741487200693,10.3088687628231));
#42559=CARTESIAN_POINT('Ctrl Pts',(0.316081937562729,2.03607784908025,10.3081922643318));
#42560=CARTESIAN_POINT('Ctrl Pts',(0.312919456651998,2.02288457336635,10.3073719923769));
#42561=CARTESIAN_POINT('Ctrl Pts',(0.312422767184617,2.02089633623996,10.3072474924329));
#42562=CARTESIAN_POINT('Ctrl Pts',(0.311740538841501,2.01827209412849,10.3070819503873));
#42563=CARTESIAN_POINT('Ctrl Pts',(0.31157194583778,2.01763170080743,10.307041456983));
#42564=CARTESIAN_POINT('Ctrl Pts',(0.311292226117584,2.01658234490789,10.306974944488));
#42565=CARTESIAN_POINT('Ctrl Pts',(0.311182263805687,2.01617307167528,10.3069489631936));
#42566=CARTESIAN_POINT('Ctrl Pts',(0.310967846889535,2.01538126051426,10.3068986201016));
#42567=CARTESIAN_POINT('Ctrl Pts',(0.310863492837383,2.01499869595132,10.3068742616084));
#42568=CARTESIAN_POINT('Ctrl Pts',(0.310621243925306,2.0141170181182,10.3068180422084));
#42569=CARTESIAN_POINT('Ctrl Pts',(0.310482851962785,2.01361804362786,10.3067861651902));
#42570=CARTESIAN_POINT('Ctrl Pts',(0.310037090084867,2.01202575253903,10.3066842473918));
#42571=CARTESIAN_POINT('Ctrl Pts',(0.309725145734263,2.01093373538995,10.3066140578834));
#42572=CARTESIAN_POINT('Ctrl Pts',(0.306851162286687,2.00107054325669,10.3059774121687));
#42573=CARTESIAN_POINT('Ctrl Pts',(0.303923167713101,1.99241118079135,10.3053990206713));
#42574=CARTESIAN_POINT('Ctrl Pts',(0.289621201534053,1.95538105461509,10.3028364944962));
#42575=CARTESIAN_POINT('Ctrl Pts',(0.274612318745951,1.92858657832475,10.3007294914701));
#42576=CARTESIAN_POINT('Ctrl Pts',(0.250061221206791,1.89646073636747,10.2980365885471));
#42577=CARTESIAN_POINT('Ctrl Pts',(0.243701609858709,1.88888767586324,10.2973892404031));
#42578=CARTESIAN_POINT('Ctrl Pts',(0.23635656803126,1.88091631897174,10.2967041988586));
#42579=CARTESIAN_POINT('Ctrl Pts',(0.235706703685719,1.88021729723407,10.2966440952859));
#42580=CARTESIAN_POINT('Ctrl Pts',(0.234723635409272,1.87916924259015,10.2965539481341));
#42581=CARTESIAN_POINT('Ctrl Pts',(0.234392744231831,1.87881806154996,10.2965237361173));
#42582=CARTESIAN_POINT('Ctrl Pts',(0.233784848633584,1.87817578663082,10.2964684733158));
#42583=CARTESIAN_POINT('Ctrl Pts',(0.233508086819422,1.8778844659156,10.296443404363));
#42584=CARTESIAN_POINT('Ctrl Pts',(0.233064229844219,1.87741900657247,10.2964033465404));
#42585=CARTESIAN_POINT('Ctrl Pts',(0.232897483811156,1.87724453788197,10.2963883307694));
#42586=CARTESIAN_POINT('Ctrl Pts',(0.232579100267325,1.87691215704683,10.2963597228517));
#42587=CARTESIAN_POINT('Ctrl Pts',(0.232427499064008,1.87675421340187,10.2963461281565));
#42588=CARTESIAN_POINT('Ctrl Pts',(0.232081820906305,1.87639480712275,10.2963151915413));
#42589=CARTESIAN_POINT('Ctrl Pts',(0.231887642858669,1.87619344297423,10.2962978576754));
#42590=CARTESIAN_POINT('Ctrl Pts',(0.23129529204231,1.87558076905126,10.2962451132226));
#42591=CARTESIAN_POINT('Ctrl Pts',(0.230896282584455,1.87517026433067,10.2962097676011));
#42592=CARTESIAN_POINT('Ctrl Pts',(0.228023468230252,1.8722303995527,10.2959565764503));
#42593=CARTESIAN_POINT('Ctrl Pts',(0.225509133083264,1.86974074100718,10.2957418360165));
#42594=CARTESIAN_POINT('Ctrl Pts',(0.200808359003068,1.84607519642265,10.2936912834566));
#42595=CARTESIAN_POINT('Ctrl Pts',(0.175744145554674,1.82812429515202,10.2920497191915));
#42596=CARTESIAN_POINT('Ctrl Pts',(0.138360804401912,1.80871248818975,10.2896557637877));
#42597=CARTESIAN_POINT('Ctrl Pts',(0.127932185399244,1.80398404516596,10.2889946999428));
#42598=CARTESIAN_POINT('Ctrl Pts',(0.112213942916123,1.79784320445093,10.2879924354602));
#42599=CARTESIAN_POINT('Ctrl Pts',(0.107104065019908,1.79599438829222,10.2876657978369));
#42600=CARTESIAN_POINT('Ctrl Pts',(0.101088566561202,1.79398839540164,10.287279488529));
#42601=CARTESIAN_POINT('Ctrl Pts',(0.100225811631146,1.79370473870034,10.2872240415869));
#42602=CARTESIAN_POINT('Ctrl Pts',(0.0989072417658184,1.7932773866257,10.2871392330804));
#42603=CARTESIAN_POINT('Ctrl Pts',(0.0984522821738875,1.79313105051226,
10.2871099584991));
#42604=CARTESIAN_POINT('Ctrl Pts',(0.0976604894913164,1.79287831533009,
10.2870589883422));
#42605=CARTESIAN_POINT('Ctrl Pts',(0.0973238029757818,1.79277145677051,
10.2870373079109));
#42606=CARTESIAN_POINT('Ctrl Pts',(0.0966215736010932,1.79254985131148,
10.2869920742734));
#42607=CARTESIAN_POINT('Ctrl Pts',(0.0962560006242379,1.79243520234657,
10.286968517891));
#42608=CARTESIAN_POINT('Ctrl Pts',(0.0953609181330605,1.79215624369425,
10.2869108209865));
#42609=CARTESIAN_POINT('Ctrl Pts',(0.0948311888292194,1.79199264842748,
10.2868766570994));
#42610=CARTESIAN_POINT('Ctrl Pts',(0.0928002307785471,1.79137116767388,
10.2867456050262));
#42611=CARTESIAN_POINT('Ctrl Pts',(0.0912961058345109,1.79092289004995,
10.2866484030595));
#42612=CARTESIAN_POINT('Ctrl Pts',(0.0892799708107033,1.79033801796338,
10.2865179063589));
#42613=CARTESIAN_POINT('Ctrl Pts',(0.0887707933898943,1.79019166805533,
10.2864849316899));
#42614=CARTESIAN_POINT('Ctrl Pts',(0.0551558524363579,1.78061959431953,
10.284306825811));
#42615=CARTESIAN_POINT('Ctrl Pts',(0.020760017249443,1.77655946288935,10.2819664939808));
#42616=CARTESIAN_POINT('Ctrl Pts',(-0.0250630580282221,1.77849670661605,
10.2788795165502));
#42617=CARTESIAN_POINT('Ctrl Pts',(-0.036480735185802,1.77959130892716,
10.2781164839686));
#42618=CARTESIAN_POINT('Ctrl Pts',(-0.0515216636897675,1.78184794640111,
10.2771383104572));
#42619=CARTESIAN_POINT('Ctrl Pts',(-0.0552168129024151,1.78246839899426,
10.2769002159862));
#42620=CARTESIAN_POINT('Ctrl Pts',(-0.0594260976411399,1.78325088737467,
10.2766321758607));
#42621=CARTESIAN_POINT('Ctrl Pts',(-0.0599514607852521,1.78334990322238,
10.2765987785384));
#42622=CARTESIAN_POINT('Ctrl Pts',(-0.0607437887374191,1.78350127684038,
10.2765484987052));
#42623=CARTESIAN_POINT('Ctrl Pts',(-0.061010934330028,1.78355266547918,
10.2765315612672));
#42624=CARTESIAN_POINT('Ctrl Pts',(-0.0614922493452293,1.78364588431146,
10.2765010729285));
#42625=CARTESIAN_POINT('Ctrl Pts',(-0.0617064408349523,1.78368759366248,
10.2764875151588));
#42626=CARTESIAN_POINT('Ctrl Pts',(-0.0621672939050994,1.78377782116313,
10.2764583657971));
#42627=CARTESIAN_POINT('Ctrl Pts',(-0.0624139403753086,1.78382641023058,
10.2764427783713));
#42628=CARTESIAN_POINT('Ctrl Pts',(-0.0630795790524016,1.78395834952927,
10.2764007466804));
#42629=CARTESIAN_POINT('Ctrl Pts',(-0.0634984646465469,1.78404224472533,
10.2763743336099));
#42630=CARTESIAN_POINT('Ctrl Pts',(-0.0654404843702239,1.78443521412597,
10.2762520468699));
#42631=CARTESIAN_POINT('Ctrl Pts',(-0.0669615699209405,1.78475447749471,
10.2761567466713));
#42632=CARTESIAN_POINT('Ctrl Pts',(-0.0994897466986224,1.79182793597579,
10.2741279229893));
#42633=CARTESIAN_POINT('Ctrl Pts',(-0.129338973517293,1.80311542309378,
10.2724317403689));
#42634=CARTESIAN_POINT('Ctrl Pts',(-0.17094618758953,1.82633696985537,10.2697324499497));
#42635=CARTESIAN_POINT('Ctrl Pts',(-0.184237619829957,1.83510293895639,
10.2688124043368));
#42636=CARTESIAN_POINT('Ctrl Pts',(-0.198800815478983,1.84633560430254,
10.2677032683209));
#42637=CARTESIAN_POINT('Ctrl Pts',(-0.200756944743664,1.84788090417787,
10.2675520596688));
#42638=CARTESIAN_POINT('Ctrl Pts',(-0.203248338926103,1.84989643127474,
10.2673565045241));
#42639=CARTESIAN_POINT('Ctrl Pts',(-0.203800280530339,1.85034598339245,
10.267312991252));
#42640=CARTESIAN_POINT('Ctrl Pts',(-0.204686984609724,1.85107309695564,
10.2672427772997));
#42641=CARTESIAN_POINT('Ctrl Pts',(-0.205022684764122,1.8513495154699,10.2672161229725));
#42642=CARTESIAN_POINT('Ctrl Pts',(-0.205660839807665,1.85187714901132,
10.2671653165093));
#42643=CARTESIAN_POINT('Ctrl Pts',(-0.205963396675659,1.85212823992881,
10.2671411694511));
#42644=CARTESIAN_POINT('Ctrl Pts',(-0.206651925693984,1.85270177885855,
10.2670860825993));
#42645=CARTESIAN_POINT('Ctrl Pts',(-0.207037603344304,1.85302457739761,
10.2670551285189));
#42646=CARTESIAN_POINT('Ctrl Pts',(-0.208210768992602,1.85401115463935,
10.2669606731019));
#42647=CARTESIAN_POINT('Ctrl Pts',(-0.208995826325596,1.8546778018495,10.2668970541735));
#42648=CARTESIAN_POINT('Ctrl Pts',(-0.214665828100839,1.8595395675113,10.2664345553281));
#42649=CARTESIAN_POINT('Ctrl Pts',(-0.21942696528653,1.86387623032181,10.2660298178779));
#42650=CARTESIAN_POINT('Ctrl Pts',(-0.225299385120587,1.86955616526625,
10.2655087580452));
#42651=CARTESIAN_POINT('Ctrl Pts',(-0.226534264798849,1.87076998322098,
10.265397908653));
#42652=CARTESIAN_POINT('Ctrl Pts',(-0.229836476142383,1.87406861668662,
10.265098007707));
#42653=CARTESIAN_POINT('Ctrl Pts',(-0.231885162902036,1.87617179331546,
10.264908210074));
#42654=CARTESIAN_POINT('Ctrl Pts',(-0.253919368813548,1.89941927591674,
10.2628256590534));
#42655=CARTESIAN_POINT('Ctrl Pts',(-0.270981027425314,1.92314833595424,
10.2608192281397));
#42656=CARTESIAN_POINT('Ctrl Pts',(-0.287089866249677,1.95347963865494,
10.2585345788915));
#42657=CARTESIAN_POINT('Ctrl Pts',(-0.289441649321907,1.95818200128935,
10.258188066369));
#42658=CARTESIAN_POINT('Ctrl Pts',(-0.293981129700156,1.96784247263212,
10.257494468844));
#42659=CARTESIAN_POINT('Ctrl Pts',(-0.296161017229568,1.97280260529715,
10.2571477893164));
#42660=CARTESIAN_POINT('Ctrl Pts',(-0.298434240647232,1.97835085647988,
10.2567722005812));
#42661=CARTESIAN_POINT('Ctrl Pts',(-0.298652070592939,1.9788866198442,10.2567360564568));
#42662=CARTESIAN_POINT('Ctrl Pts',(-0.298973558686569,1.97968347686127,
10.2566824859202));
#42663=CARTESIAN_POINT('Ctrl Pts',(-0.299078318099037,1.97994412060046,
10.256664993321));
#42664=CARTESIAN_POINT('Ctrl Pts',(-0.299256576842517,1.98038931359871,
10.2566351662712));
#42665=CARTESIAN_POINT('Ctrl Pts',(-0.299330246356087,1.98057379390534,
10.2566228214587));
#42666=CARTESIAN_POINT('Ctrl Pts',(-0.299481390866339,1.98095330249226,
10.256597456956));
#42667=CARTESIAN_POINT('Ctrl Pts',(-0.299558845753334,1.98114833785637,
10.2565844385071));
#42668=CARTESIAN_POINT('Ctrl Pts',(-0.299745277471662,1.9816191224415,10.2565530541385));
#42669=CARTESIAN_POINT('Ctrl Pts',(-0.299854064609073,1.98189494728363,
10.2565346997336));
#42670=CARTESIAN_POINT('Ctrl Pts',(-0.300252222039868,1.98290855351865,
10.2564673710249));
#42671=CARTESIAN_POINT('Ctrl Pts',(-0.300539254413513,1.98364725930728,
10.2564185366112));
#42672=CARTESIAN_POINT('Ctrl Pts',(-0.305770102730545,1.99725786341734,
10.2555229342964));
#42673=CARTESIAN_POINT('Ctrl Pts',(-0.309886240042588,2.01043478888042,
10.2547241392142));
#42674=CARTESIAN_POINT('Ctrl Pts',(-0.315669846875002,2.03421408591075,
10.2533358784551));
#42675=CARTESIAN_POINT('Ctrl Pts',(-0.317676512083658,2.04471090220126,
10.252740725704));
#42676=CARTESIAN_POINT('Ctrl Pts',(-0.321225274298717,2.07004240427519,
10.2513105902921));
#42677=CARTESIAN_POINT('Ctrl Pts',(-0.322266549859838,2.08492145256059,
10.2504748489422));
#42678=CARTESIAN_POINT('Ctrl Pts',(-0.322276716835356,2.10295423647165,
10.2494303352084));
#42679=CARTESIAN_POINT('Ctrl Pts',(-0.322232712885111,2.10608996056174,
10.2492475951044));
#42680=CARTESIAN_POINT('Ctrl Pts',(-0.321916774282351,2.1171233663404,10.2485999739315));
#42681=CARTESIAN_POINT('Ctrl Pts',(-0.321400168572899,2.1250106968606,10.2481285768766));
#42682=CARTESIAN_POINT('Ctrl Pts',(-0.320484300312303,2.13394336119121,
10.2475823036084));
#42683=CARTESIAN_POINT('Ctrl Pts',(-0.320368928388166,2.13501554218857,
10.2475165327137));
#42684=CARTESIAN_POINT('Ctrl Pts',(-0.3201905497065,2.13659852962666,10.2474191219767));
#42685=CARTESIAN_POINT('Ctrl Pts',(-0.32013169620365,2.13710980427196,10.247387613064));
#42686=CARTESIAN_POINT('Ctrl Pts',(-0.320025387588235,2.13801425739179,
10.2473317890992));
#42687=CARTESIAN_POINT('Ctrl Pts',(-0.31997843183043,2.13840749441407,10.2473074898431));
#42688=CARTESIAN_POINT('Ctrl Pts',(-0.319879569557385,2.13922266342354,
10.2472570593305));
#42689=CARTESIAN_POINT('Ctrl Pts',(-0.319827552811289,2.13964458104508,
10.2472309246392));
#42690=CARTESIAN_POINT('Ctrl Pts',(-0.319691629977039,2.14072939753612,
10.2471636434788));
#42691=CARTESIAN_POINT('Ctrl Pts',(-0.319606497098098,2.14139213817831,
10.24712245834));
#42692=CARTESIAN_POINT('Ctrl Pts',(-0.319245440845404,2.1441353441082,10.2469516444635));
#42693=CARTESIAN_POINT('Ctrl Pts',(-0.318951264403229,2.14621331735357,
10.246821440134));
#42694=CARTESIAN_POINT('Ctrl Pts',(-0.316842833626621,2.16012610043917,
10.2459440636011));
#42695=CARTESIAN_POINT('Ctrl Pts',(-0.314390777516254,2.1718533805654,10.2451766990906));
#42696=CARTESIAN_POINT('Ctrl Pts',(-0.302037930123091,2.21795183181976,
10.2420470090228));
#42697=CARTESIAN_POINT('Ctrl Pts',(-0.287103176946999,2.25070114578868,
10.239534197368));
#42698=CARTESIAN_POINT('Ctrl Pts',(-0.266030208539513,2.28191416455311,
10.2371437585563));
#42699=CARTESIAN_POINT('Ctrl Pts',(-0.264945674874943,2.28349012210745,
10.237023172216));
#42700=CARTESIAN_POINT('Ctrl Pts',(-0.263605782795067,2.28540049507824,
10.2368772223337));
#42701=CARTESIAN_POINT('Ctrl Pts',(-0.263363749535825,2.28574414589281,
10.2368509768337));
#42702=CARTESIAN_POINT('Ctrl Pts',(-0.262963952131915,2.28630944559922,
10.2368078195395));
#42703=CARTESIAN_POINT('Ctrl Pts',(-0.262806579345573,2.28653136866038,
10.2367908811256));
#42704=CARTESIAN_POINT('Ctrl Pts',(-0.262522472564793,2.28693093548578,
10.2367603917376));
#42705=CARTESIAN_POINT('Ctrl Pts',(-0.262395839468559,2.28710864938224,
10.2367468338922));
#42706=CARTESIAN_POINT('Ctrl Pts',(-0.262122941521863,2.28749080602003,
10.2367176851553));
#42707=CARTESIAN_POINT('Ctrl Pts',(-0.261976618393266,2.287695205667,10.2367020984283));
#42708=CARTESIAN_POINT('Ctrl Pts',(-0.261574473839645,2.28825557739459,
10.2366593762261));
#42709=CARTESIAN_POINT('Ctrl Pts',(-0.261318163849062,2.28861120070823,
10.236632274472));
#42710=CARTESIAN_POINT('Ctrl Pts',(-0.2599716316571,2.29047146472033,10.2364905547087));
#42711=CARTESIAN_POINT('Ctrl Pts',(-0.258869108857966,2.2919672185651,10.2363767739299));
#42712=CARTESIAN_POINT('Ctrl Pts',(-0.247465091304613,2.30716171801238,
10.2352217418688));
#42713=CARTESIAN_POINT('Ctrl Pts',(-0.236097727779618,2.32002949904546,
10.2342495618533));
#42714=CARTESIAN_POINT('Ctrl Pts',(-0.208483600994742,2.34667040192605,
10.2320971245937));
#42715=CARTESIAN_POINT('Ctrl Pts',(-0.191790570564711,2.35986155516685,
10.2309252112259));
#42716=CARTESIAN_POINT('Ctrl Pts',(-0.172080245809586,2.37249651712578,
10.2295676575219));
#42717=CARTESIAN_POINT('Ctrl Pts',(-0.170226295930851,2.37365849288642,
10.2294402483126));
#42718=CARTESIAN_POINT('Ctrl Pts',(-0.16669107266537,2.37582439317333,10.2291976941318));
#42719=CARTESIAN_POINT('Ctrl Pts',(-0.165012197320453,2.37683205032779,
10.229082672291));
#42720=CARTESIAN_POINT('Ctrl Pts',(-0.157549501012761,2.38121913695622,
10.228571924948));
#42721=CARTESIAN_POINT('Ctrl Pts',(-0.151670646041347,2.38443286290163,
10.2281709271541));
#42722=CARTESIAN_POINT('Ctrl Pts',(-0.144766875374731,2.38793195898004,
10.2276998915251));
#42723=CARTESIAN_POINT('Ctrl Pts',(-0.143835245869158,2.38839847990868,
10.2276363262004));
#42724=CARTESIAN_POINT('Ctrl Pts',(-0.14244844965183,2.38908453809908,10.2275416966308));
#42725=CARTESIAN_POINT('Ctrl Pts',(-0.141994996024861,2.38930753891918,
10.2275107534478));
#42726=CARTESIAN_POINT('Ctrl Pts',(-0.14118753056389,2.38970228107067,10.2274556498518));
#42727=CARTESIAN_POINT('Ctrl Pts',(-0.140833724373961,2.38987444268348,
10.2274315041428));
#42728=CARTESIAN_POINT('Ctrl Pts',(-0.140089375947592,2.39023495718478,
10.2273807030773));
#42729=CARTESIAN_POINT('Ctrl Pts',(-0.139698767369983,2.39042317059391,
10.2273540429306));
#42730=CARTESIAN_POINT('Ctrl Pts',(-0.138670980821531,2.39091585278389,
10.2272838890154));
#42731=CARTESIAN_POINT('Ctrl Pts',(-0.138033182441832,2.39121901527077,
10.2272403500317));
#42732=CARTESIAN_POINT('Ctrl Pts',(-0.135188967272487,2.39255950348518,
10.2270461661523));
#42733=CARTESIAN_POINT('Ctrl Pts',(-0.132971863918247,2.39357384562058,
10.2268947296445));
#42734=CARTESIAN_POINT('Ctrl Pts',(-0.116746815116286,2.40077543070837,
10.2257857568515));
#42735=CARTESIAN_POINT('Ctrl Pts',(-0.102327240609211,2.40598152330111,
10.2247947645774));
#42736=CARTESIAN_POINT('Ctrl Pts',(-0.0563260178287632,2.41897372077274,
10.2216220048773));
#42737=CARTESIAN_POINT('Ctrl Pts',(-0.0239046922849002,2.42302527443662,
10.2193519646799));
#42738=CARTESIAN_POINT('Ctrl Pts',(0.0100509583545428,2.4221216198764,10.2172040174813));
#42739=CARTESIAN_POINT('Ctrl Pts',(0.0115280616561617,2.42207214059716,
10.2171110777308));
#42740=CARTESIAN_POINT('Ctrl Pts',(0.013428515059428,2.42199538883481,10.2169921868044));
#42741=CARTESIAN_POINT('Ctrl Pts',(0.01385219329443,2.42197744050387,10.21696572572));
#42742=CARTESIAN_POINT('Ctrl Pts',(0.0145237866074252,2.42194766165806,
10.216923851879));
#42743=CARTESIAN_POINT('Ctrl Pts',(0.0147717236872081,2.42193638098981,
10.2169084083311));
#42744=CARTESIAN_POINT('Ctrl Pts',(0.0152161732483076,2.42191564485549,
10.2168807521608));
#42745=CARTESIAN_POINT('Ctrl Pts',(0.0154126886648717,2.42190629593017,
10.2168685336239));
#42746=CARTESIAN_POINT('Ctrl Pts',(0.0158749520332594,2.42188388017218,
10.2168398148181));
#42747=CARTESIAN_POINT('Ctrl Pts',(0.0161406920627803,2.42187066420803,
10.2168233230679));
#42748=CARTESIAN_POINT('Ctrl Pts',(0.0169118072180625,2.42183135721213,
10.2167755186033));
#42749=CARTESIAN_POINT('Ctrl Pts',(0.0174171405580597,2.42180440477317,
10.2167442542293));
#42750=CARTESIAN_POINT('Ctrl Pts',(0.0209300547234772,2.42160874119018,
10.2165273411002));
#42751=CARTESIAN_POINT('Ctrl Pts',(0.0239353317044781,2.42139905269883,
10.2163439480406));
#42752=CARTESIAN_POINT('Ctrl Pts',(0.0332869399459402,2.42061465364066,
10.2157788349526));
#42753=CARTESIAN_POINT('Ctrl Pts',(0.0396197786009589,2.41989382740721,
10.2154041244397));
#42754=CARTESIAN_POINT('Ctrl Pts',(0.0615536735255772,2.41673578941638,
10.2141213986409));
#42755=CARTESIAN_POINT('Ctrl Pts',(0.0769944377059781,2.41334060814226,
10.2132443265186));
#42756=CARTESIAN_POINT('Ctrl Pts',(0.116177662349037,2.40165201901112,10.2109578937159));
#42757=CARTESIAN_POINT('Ctrl Pts',(0.139305755559593,2.39169305825259,10.2095410773283));
#42758=CARTESIAN_POINT('Ctrl Pts',(0.162332192302773,2.37840914221612,10.2079285586656));
#42759=CARTESIAN_POINT('Ctrl Pts',(0.163616299877506,2.37765643775332,10.2078379538772));
#42760=CARTESIAN_POINT('Ctrl Pts',(0.165360992359369,2.37661744670995,10.2077139027223));
#42761=CARTESIAN_POINT('Ctrl Pts',(0.165826151011712,2.37633884499538,10.2076807364101));
#42762=CARTESIAN_POINT('Ctrl Pts',(0.166615896668097,2.37586312333279,10.2076242680939));
#42763=CARTESIAN_POINT('Ctrl Pts',(0.166940843494051,2.37566660045956,10.2076009879542));
#42764=CARTESIAN_POINT('Ctrl Pts',(0.167568120305008,2.37528571716469,10.2075559590203));
#42765=CARTESIAN_POINT('Ctrl Pts',(0.167870495444122,2.37510143179418,10.2075342130002));
#42766=CARTESIAN_POINT('Ctrl Pts',(0.168578162750681,2.37466853612653,10.2074832251134));
#42767=CARTESIAN_POINT('Ctrl Pts',(0.168983208882309,2.37441952701345,10.2074539686122));
#42768=CARTESIAN_POINT('Ctrl Pts',(0.170160508556535,2.37369216676697,10.2073687194778));
#42769=CARTESIAN_POINT('Ctrl Pts',(0.170931287748707,2.37321144863153,10.2073126396266));
#42770=CARTESIAN_POINT('Ctrl Pts',(0.172667580331227,2.37211833742271,10.2071857018617));
#42771=CARTESIAN_POINT('Ctrl Pts',(0.173631884057074,2.3715040545623,10.2071147742441));
#42772=CARTESIAN_POINT('Ctrl Pts',(0.181769531307242,2.3662591088262,10.2065125499472));
#42773=CARTESIAN_POINT('Ctrl Pts',(0.188758910962429,2.36135058227448,10.2059708815105));
#42774=CARTESIAN_POINT('Ctrl Pts',(0.201861163279412,2.35134914339914,10.2049059746637));
#42775=CARTESIAN_POINT('Ctrl Pts',(0.207996722431496,2.34629589797771,10.204384435751));
#42776=CARTESIAN_POINT('Ctrl Pts',(0.238026839225436,2.31964012652625,10.2017172461518));
#42777=CARTESIAN_POINT('Ctrl Pts',(0.258772052938662,2.29477041105743,10.1994682660753));
#42778=CARTESIAN_POINT('Ctrl Pts',(0.276261903006829,2.26596016100563,10.1973366749835));
#42779=CARTESIAN_POINT('Ctrl Pts',(0.277029407627232,2.26467580760319,10.1972425764988));
#42780=CARTESIAN_POINT('Ctrl Pts',(0.278003958552199,2.26301888288995,10.1971224145955));
#42781=CARTESIAN_POINT('Ctrl Pts',(0.278219232702047,2.2626512087537,10.197095827993));
#42782=CARTESIAN_POINT('Ctrl Pts',(0.278558981842014,2.26206829141269,10.1970538010444));
#42783=CARTESIAN_POINT('Ctrl Pts',(0.278683936995338,2.26185333085257,10.1970383295244));
#42784=CARTESIAN_POINT('Ctrl Pts',(0.27890728954147,2.261468071608,10.1970106489211));
#42785=CARTESIAN_POINT('Ctrl Pts',(0.279005779096378,2.26129782868756,10.1969984338577));
#42786=CARTESIAN_POINT('Ctrl Pts',(0.27923683638241,2.26089759259308,10.196969755885));
#42787=CARTESIAN_POINT('Ctrl Pts',(0.279369275633034,2.26066752605488,10.196953301416));
#42788=CARTESIAN_POINT('Ctrl Pts',(0.279751933616068,2.2600008889506,10.1969057104104));
#42789=CARTESIAN_POINT('Ctrl Pts',(0.280001415769493,2.25956389316541,10.1968746215505));
#42790=CARTESIAN_POINT('Ctrl Pts',(0.281706097630932,2.25656164372482,10.1966617631));
#42791=CARTESIAN_POINT('Ctrl Pts',(0.28312710826658,2.2539769975604,10.1964821540814));
#42792=CARTESIAN_POINT('Ctrl Pts',(0.287472416019746,2.24580979767593,10.1959247874246));
#42793=CARTESIAN_POINT('Ctrl Pts',(0.290268730264669,2.24016048723107,10.1955539482835));
#42794=CARTESIAN_POINT('Ctrl Pts',(0.299371105407499,2.22032847871433,10.1942899559377));
#42795=CARTESIAN_POINT('Ctrl Pts',(0.304817709053173,2.20577442773385,10.1934269641108));
#42796=CARTESIAN_POINT('Ctrl Pts',(0.309985007400795,2.18819481770798,10.1924025607434));
#42797=CARTESIAN_POINT('Ctrl Pts',(0.310740271305906,2.18549569791799,10.192245790965));
#42798=CARTESIAN_POINT('Ctrl Pts',(0.317335580343344,2.16068293176026,10.1908071293027));
#42799=CARTESIAN_POINT('Ctrl Pts',(0.320840369902876,2.13801994083312,10.1895048771523));
#42800=CARTESIAN_POINT('Ctrl Pts',(0.321981601457013,2.11381610238357,10.1880338495369));
#42801=CARTESIAN_POINT('Ctrl Pts',(0.322037195550189,2.11245315039475,10.1879507702548));
#42802=CARTESIAN_POINT('Ctrl Pts',(0.322102113908958,2.11056772596927,10.1878354936258));
#42803=CARTESIAN_POINT('Ctrl Pts',(0.322118823364463,2.11004550874783,10.1878035276797));
#42804=CARTESIAN_POINT('Ctrl Pts',(0.322145326270901,2.10914901971396,10.1877485873219));
#42805=CARTESIAN_POINT('Ctrl Pts',(0.322155737615082,2.10877476607529,10.1877256323026));
#42806=CARTESIAN_POINT('Ctrl Pts',(0.32217580818246,2.10800504438436,10.1876783810458));
#42807=CARTESIAN_POINT('Ctrl Pts',(0.322185391472247,2.1076095751076,10.1876540824681));
#42808=CARTESIAN_POINT('Ctrl Pts',(0.322205665476916,2.1067041016306,10.1875983978331));
#42809=CARTESIAN_POINT('Ctrl Pts',(0.32221587345273,2.1061940886673,10.1875669967084));
#42810=CARTESIAN_POINT('Ctrl Pts',(0.322243841858294,2.10460858072232,10.1874692636264));
#42811=CARTESIAN_POINT('Ctrl Pts',(0.322257428620327,2.10353302787113,10.1874028011198));
#42812=CARTESIAN_POINT('Ctrl Pts',(0.322276367159658,2.10104944880743,10.1872489452351));
#42813=CARTESIAN_POINT('Ctrl Pts',(0.322277876209116,2.09964142322781,10.1871614325446));
#42814=CARTESIAN_POINT('Ctrl Pts',(0.322203230711669,2.08602390545062,10.1863122317901));
#42815=CARTESIAN_POINT('Ctrl Pts',(0.321442523306059,2.07382952204161,10.1855291560603));
#42816=CARTESIAN_POINT('Ctrl Pts',(0.317925889171002,2.04444164648694,10.1835863912151));
#42817=CARTESIAN_POINT('Ctrl Pts',(0.314465551617781,2.02737136985831,10.1824099858604));
#42818=CARTESIAN_POINT('Ctrl Pts',(0.304390135563161,1.99244868612957,10.1799509659343));
#42819=CARTESIAN_POINT('Ctrl Pts',(0.29753656184219,1.97472902765568,10.1786732057549));
#42820=CARTESIAN_POINT('Ctrl Pts',(0.289049496588848,1.9574811205319,10.1774614717579));
#42821=CARTESIAN_POINT('Ctrl Pts',(0.288935056620201,1.95724925380214,10.1774451886932));
#42822=CARTESIAN_POINT('Ctrl Pts',(0.288402527519514,1.95617356089962,10.1773696781551));
#42823=CARTESIAN_POINT('Ctrl Pts',(0.287981014348883,1.95533142051241,10.1773106510515));
#42824=CARTESIAN_POINT('Ctrl Pts',(0.287396055339469,1.95417541979105,10.1772297597578));
#42825=CARTESIAN_POINT('Ctrl Pts',(0.287235780315555,1.95385997356241,10.1772077002351));
#42826=CARTESIAN_POINT('Ctrl Pts',(0.286979856702142,1.95335832348388,10.1771726421203));
#42827=CARTESIAN_POINT('Ctrl Pts',(0.28688454621999,1.95317194891642,10.1771596222539));
#42828=CARTESIAN_POINT('Ctrl Pts',(0.286698331466266,1.95280868941753,10.1771342554664));
#42829=CARTESIAN_POINT('Ctrl Pts',(0.286607445316277,1.95263179628577,10.1771219074995));
#42830=CARTESIAN_POINT('Ctrl Pts',(0.286387115623111,1.95220393994474,10.1770920522105));
#42831=CARTESIAN_POINT('Ctrl Pts',(0.286257505534049,1.95195306187,10.1770745554682));
#42832=CARTESIAN_POINT('Ctrl Pts',(0.285858014603468,1.95118227844976,10.1770208268521));
#42833=CARTESIAN_POINT('Ctrl Pts',(0.285587043966299,1.9506629346352,10.1769846635502));
#42834=CARTESIAN_POINT('Ctrl Pts',(0.282616016091493,1.94500630660084,10.1765911645923));
#42835=CARTESIAN_POINT('Ctrl Pts',(0.279778868587143,1.93994172134119,10.1762423376253));
#42836=CARTESIAN_POINT('Ctrl Pts',(0.273367816919066,1.92918931030657,10.1755033435574));
#42837=CARTESIAN_POINT('Ctrl Pts',(0.269749793022916,1.92353098117248,10.1751154440138));
#42838=CARTESIAN_POINT('Ctrl Pts',(0.250806165353673,1.89585016570161,10.1732018665211));
#42839=CARTESIAN_POINT('Ctrl Pts',(0.23295011912224,1.87568945784308,10.1717467469305));
#42840=CARTESIAN_POINT('Ctrl Pts',(0.209949120621521,1.85546581051673,10.1699752498973));
#42841=CARTESIAN_POINT('Ctrl Pts',(0.207052551073976,1.85300841581856,10.1697539697653));
#42842=CARTESIAN_POINT('Ctrl Pts',(0.198211181805984,1.84577240263181,10.1690827987541));
#42843=CARTESIAN_POINT('Ctrl Pts',(0.192139863679668,1.84115332287285,10.1686274646284));
#42844=CARTESIAN_POINT('Ctrl Pts',(0.185115652869838,1.8361926493763,10.1681042798604));
#42845=CARTESIAN_POINT('Ctrl Pts',(0.184317991449631,1.83563472017691,10.1680449198895));
#42846=CARTESIAN_POINT('Ctrl Pts',(0.183107765355365,1.83479635989196,10.1679549316943));
#42847=CARTESIAN_POINT('Ctrl Pts',(0.18269705222233,1.83451325538768,10.167924405277));
#42848=CARTESIAN_POINT('Ctrl Pts',(0.181982023188761,1.83402283095983,10.1678712819083));
#42849=CARTESIAN_POINT('Ctrl Pts',(0.181678005380304,1.83381507635911,10.1678487014972));
#42850=CARTESIAN_POINT('Ctrl Pts',(0.181043536555791,1.83338309698869,10.1678015910343));
#42851=CARTESIAN_POINT('Ctrl Pts',(0.180713023645052,1.83315896458229,10.1677770575382));
#42852=CARTESIAN_POINT('Ctrl Pts',(0.179940682784765,1.83263730619594,10.1677197452475));
#42853=CARTESIAN_POINT('Ctrl Pts',(0.179498533056314,1.83234026080785,10.1676869483947));
#42854=CARTESIAN_POINT('Ctrl Pts',(0.178062439832272,1.83138062225204,10.167580466456));
#42855=CARTESIAN_POINT('Ctrl Pts',(0.17706555713016,1.830722464737,10.1675066149567));
#42856=CARTESIAN_POINT('Ctrl Pts',(0.174723142355374,1.82919459760054,10.1673332224154));
#42857=CARTESIAN_POINT('Ctrl Pts',(0.173374747444346,1.8283293552063,10.1672335167237));
#42858=CARTESIAN_POINT('Ctrl Pts',(0.168710575844485,1.82538530097995,10.1668889623726));
#42859=CARTESIAN_POINT('Ctrl Pts',(0.165363523589845,1.82335691907918,10.1666422763839));
#42860=CARTESIAN_POINT('Ctrl Pts',(0.15533981381169,1.81752925441043,10.1659049287698));
#42861=CARTESIAN_POINT('Ctrl Pts',(0.148563710120675,1.81390737749328,10.1654082401108));
#42862=CARTESIAN_POINT('Ctrl Pts',(0.130514708312829,1.80507425221755,10.1640903474292));
#42863=CARTESIAN_POINT('Ctrl Pts',(0.119059145155823,1.80026651421094,10.1632585227543));
#42864=CARTESIAN_POINT('Ctrl Pts',(0.0973078349957262,1.79258184458971,
10.1617004316635));
#42865=CARTESIAN_POINT('Ctrl Pts',(0.0870900312954191,1.7895325031056,10.1609769460985));
#42866=CARTESIAN_POINT('Ctrl Pts',(0.0632446307792649,1.78368629242499,
10.1593271839626));
#42867=CARTESIAN_POINT('Ctrl Pts',(0.0495476097231807,1.78125342099902,
10.1584075849549));
#42868=CARTESIAN_POINT('Ctrl Pts',(0.0348937968962166,1.7796184860574,10.1574809326854));
#42869=CARTESIAN_POINT('Ctrl Pts',(0.0340525205807042,1.77952797716765,
10.1574279335444));
#42870=CARTESIAN_POINT('Ctrl Pts',(0.0329079980250895,1.7794094012341,10.1573561112264));
#42871=CARTESIAN_POINT('Ctrl Pts',(0.0326050637718685,1.77937845024172,
10.1573371279083));
#42872=CARTESIAN_POINT('Ctrl Pts',(0.0320911049542223,1.77932667467969,
10.1573049666544));
#42873=CARTESIAN_POINT('Ctrl Pts',(0.0318801036735994,1.77930562901804,
10.1572917762466));
#42874=CARTESIAN_POINT('Ctrl Pts',(0.0314722135044432,1.77926535182979,
10.1572663031904));
#42875=CARTESIAN_POINT('Ctrl Pts',(0.0312753291881682,1.77924609348583,
10.1572540191428));
#42876=CARTESIAN_POINT('Ctrl Pts',(0.0308044471122331,1.7792004715839,10.1572246671725));
#42877=CARTESIAN_POINT('Ctrl Pts',(0.0305304334143919,1.77917427779125,
10.1572076089586));
#42878=CARTESIAN_POINT('Ctrl Pts',(0.0297085218762604,1.77909677132138,
10.1571565079363));
#42879=CARTESIAN_POINT('Ctrl Pts',(0.0291605222703362,1.77904651053473,
10.1571225242911));
#42880=CARTESIAN_POINT('Ctrl Pts',(0.024378692687874,1.77862028442435,10.1568267248375));
#42881=CARTESIAN_POINT('Ctrl Pts',(0.0201376909896521,1.77832668760928,
10.1565694454976));
#42882=CARTESIAN_POINT('Ctrl Pts',(0.00731995009551853,1.77769385517253,
10.1558037977783));
#42883=CARTESIAN_POINT('Ctrl Pts',(-0.00126615595632977,1.77761319421737,
10.1553069807815));
#42884=CARTESIAN_POINT('Ctrl Pts',(-0.0126959361606186,1.77796254975445,
10.1546552530361));
#42885=CARTESIAN_POINT('Ctrl Pts',(-0.0155447750850952,1.77808748610062,
10.154493614807));
#42886=CARTESIAN_POINT('Ctrl Pts',(-0.0207295372943453,1.77838385360752,
10.1542003455146));
#42887=CARTESIAN_POINT('Ctrl Pts',(-0.0230659477176856,1.77854297086814,
10.1540685251049));
#42888=CARTESIAN_POINT('Ctrl Pts',(-0.043670795470961,1.78017203082368,
10.1529075143096));
#42889=CARTESIAN_POINT('Ctrl Pts',(-0.0617840496531189,1.78317231238318,
10.1518952230683));
#42890=CARTESIAN_POINT('Ctrl Pts',(-0.0855973286917739,1.78923756164319,
10.1504892536515));
#42891=CARTESIAN_POINT('Ctrl Pts',(-0.0916043077933855,1.79095495408075,
10.150128191693));
#42892=CARTESIAN_POINT('Ctrl Pts',(-0.0992687234499406,1.79338930160738,
10.1496569403565));
#42893=CARTESIAN_POINT('Ctrl Pts',(-0.100975485081835,1.79394714335067,
10.1495513175315));
#42894=CARTESIAN_POINT('Ctrl Pts',(-0.108824841347796,1.79658545023754,
10.1490622486057));
#42895=CARTESIAN_POINT('Ctrl Pts',(-0.114908076181694,1.79883665540829,
10.1486737839291));
#42896=CARTESIAN_POINT('Ctrl Pts',(-0.121875645928436,1.80165696292966,
10.1482162954444));
#42897=CARTESIAN_POINT('Ctrl Pts',(-0.122830460859628,1.80204879814811,
10.1481533261168));
#42898=CARTESIAN_POINT('Ctrl Pts',(-0.124248128650533,1.80263855069187,
10.1480594140394));
#42899=CARTESIAN_POINT('Ctrl Pts',(-0.124712433090793,1.8028329795623,10.1480285896695));
#42900=CARTESIAN_POINT('Ctrl Pts',(-0.125538633007392,1.80318123058497,
10.1479736195501));
#42901=CARTESIAN_POINT('Ctrl Pts',(-0.125900706848187,1.80333462914022,
10.1479494882453));
#42902=CARTESIAN_POINT('Ctrl Pts',(-0.126599727730764,1.80363229104882,
10.1479028202342));
#42903=CARTESIAN_POINT('Ctrl Pts',(-0.126936711359007,1.80377646737967,
10.1478802865232));
#42904=CARTESIAN_POINT('Ctrl Pts',(-0.127665055410159,1.80408955586728,
10.1478315046946));
#42905=CARTESIAN_POINT('Ctrl Pts',(-0.128056327755394,1.80425867005318,
10.1478052497084));
#42906=CARTESIAN_POINT('Ctrl Pts',(-0.129591659113807,1.80492588305837,
10.1477020331109));
#42907=CARTESIAN_POINT('Ctrl Pts',(-0.130733145177707,1.805429843191,10.1476248712256));
#42908=CARTESIAN_POINT('Ctrl Pts',(-0.133415914618493,1.80663293700132,
10.1474425116309));
#42909=CARTESIAN_POINT('Ctrl Pts',(-0.134954662744456,1.8073376027681,10.1473371251291));
#42910=CARTESIAN_POINT('Ctrl Pts',(-0.140305131230139,1.8098390049233,10.1469678719691));
#42911=CARTESIAN_POINT('Ctrl Pts',(-0.144086972472864,1.81169829244366,
10.146701861441));
#42912=CARTESIAN_POINT('Ctrl Pts',(-0.159119056548183,1.81945824904999,
10.1456238283261));
#42913=CARTESIAN_POINT('Ctrl Pts',(-0.170051302617941,1.82594701594472,
10.1447918851835));
#42914=CARTESIAN_POINT('Ctrl Pts',(-0.202157140040345,1.84766522436195,
10.1422066529196));
#42915=CARTESIAN_POINT('Ctrl Pts',(-0.221891288400186,1.86483077169538,
10.1404065459565));
#42916=CARTESIAN_POINT('Ctrl Pts',(-0.243181659338713,1.88844216379355,
10.1383357323394));
#42917=CARTESIAN_POINT('Ctrl Pts',(-0.246906541402382,1.89280152645085,
10.1379681039967));
#42918=CARTESIAN_POINT('Ctrl Pts',(-0.250926024741231,1.89776811346674,
10.1375674905578));
#42919=CARTESIAN_POINT('Ctrl Pts',(-0.251337092179029,1.89827922284463,
10.1375264730715));
#42920=CARTESIAN_POINT('Ctrl Pts',(-0.251929268592681,1.89902013818866,
10.1374673198599));
#42921=CARTESIAN_POINT('Ctrl Pts',(-0.252111626093049,1.89924893719411,
10.13744909509));
#42922=CARTESIAN_POINT('Ctrl Pts',(-0.252431441275568,1.89965132367063,
10.1374171177172));
#42923=CARTESIAN_POINT('Ctrl Pts',(-0.252569031887072,1.89982480477289,
10.1374033555128));
#42924=CARTESIAN_POINT('Ctrl Pts',(-0.252853827547614,1.90018465044015,
10.1373748594096));
#42925=CARTESIAN_POINT('Ctrl Pts',(-0.253001005139948,1.90037103560792,
10.1373601274899));
#42926=CARTESIAN_POINT('Ctrl Pts',(-0.25338079451323,1.90085309410642,10.1373220969849));
#42927=CARTESIAN_POINT('Ctrl Pts',(-0.253613095671186,1.90114901342301,
10.1372988207149));
#42928=CARTESIAN_POINT('Ctrl Pts',(-0.254586176694237,1.90239306196783,
10.1372012545747));
#42929=CARTESIAN_POINT('Ctrl Pts',(-0.255322174348429,1.90334494485143,
10.1371273016437));
#42930=CARTESIAN_POINT('Ctrl Pts',(-0.26047015059009,1.91008056205998,10.1366087357031));
#42931=CARTESIAN_POINT('Ctrl Pts',(-0.264690904509269,1.9160085985615,10.136176777103));
#42932=CARTESIAN_POINT('Ctrl Pts',(-0.282832977836315,1.94340729504158,
10.1342631611438));
#42933=CARTESIAN_POINT('Ctrl Pts',(-0.294368688616418,1.96634720330998,
10.1328759772448));
#42934=CARTESIAN_POINT('Ctrl Pts',(-0.303860509652376,1.99259717453918,
10.1312917150564));
#42935=CARTESIAN_POINT('Ctrl Pts',(-0.304627078778883,1.99479107038169,
10.1311593926873));
#42936=CARTESIAN_POINT('Ctrl Pts',(-0.307026183798727,2.00190335025002,
10.1307303534473));
#42937=CARTESIAN_POINT('Ctrl Pts',(-0.308563790076345,2.0068527279617,10.130431667043));
#42938=CARTESIAN_POINT('Ctrl Pts',(-0.312570459064317,2.02094016733407,
10.1295782427468));
#42939=CARTESIAN_POINT('Ctrl Pts',(-0.314757085133555,2.03015231006502,
10.1290161858076));
#42940=CARTESIAN_POINT('Ctrl Pts',(-0.316750433080215,2.04057229495527,
10.1283710347541));
#42941=CARTESIAN_POINT('Ctrl Pts',(-0.316959754494367,2.04169903121609,
10.1283011542116));
#42942=CARTESIAN_POINT('Ctrl Pts',(-0.317255262062329,2.04333833362079,
10.1281993035841));
#42943=CARTESIAN_POINT('Ctrl Pts',(-0.317346226628274,2.04385003844255,
10.1281674856041));
#42944=CARTESIAN_POINT('Ctrl Pts',(-0.317504466997128,2.04475285926548,
10.1281113020831));
#42945=CARTESIAN_POINT('Ctrl Pts',(-0.317572259066667,2.04514388464785,
10.1280869530082));
#42946=CARTESIAN_POINT('Ctrl Pts',(-0.317701194322453,2.04589583420773,
10.128040099773));
#42947=CARTESIAN_POINT('Ctrl Pts',(-0.317762445199514,2.04625673950106,
10.128017599076));
#42948=CARTESIAN_POINT('Ctrl Pts',(-0.31789177382186,2.04702672613575,10.1279695660028));
#42949=CARTESIAN_POINT('Ctrl Pts',(-0.317959677070191,2.04743583575896,
10.1279440281244));
#42950=CARTESIAN_POINT('Ctrl Pts',(-0.318120470596281,2.04841631167379,
10.1278827827648));
#42951=CARTESIAN_POINT('Ctrl Pts',(-0.318212611229245,2.04898779791655,
10.127847051547));
#42952=CARTESIAN_POINT('Ctrl Pts',(-0.318455392460631,2.05051986214893,
10.127751170967));
#42953=CARTESIAN_POINT('Ctrl Pts',(-0.318603225545463,2.05148087317603,
10.1276909327731));
#42954=CARTESIAN_POINT('Ctrl Pts',(-0.321109153307386,2.06827647272606,
10.1266364395165));
#42955=CARTESIAN_POINT('Ctrl Pts',(-0.322288067930669,2.08426144891936,
10.1256045749165));
#42956=CARTESIAN_POINT('Ctrl Pts',(-0.322274890758155,2.1002653522546,10.1245441658164));
#42957=CARTESIAN_POINT('',(-0.322274855599701,2.09970609858236,9.87441280121724));
#42958=CARTESIAN_POINT('Ctrl Pts',(-0.32227489106725,2.10026497658775,10.1245441907079));
#42959=CARTESIAN_POINT('Ctrl Pts',(-0.322257938840951,2.12088293733043,
10.1231780574279));
#42960=CARTESIAN_POINT('Ctrl Pts',(-0.320262365543633,2.14145188343667,
10.1217683869481));
#42961=CARTESIAN_POINT('Ctrl Pts',(-0.314416419040088,2.17142809675683,
10.1197192579556));
#42962=CARTESIAN_POINT('Ctrl Pts',(-0.312067804907137,2.1810763657603,10.1190613622444));
#42963=CARTESIAN_POINT('Ctrl Pts',(-0.308215404461165,2.19422691146406,
10.1181798669604));
#42964=CARTESIAN_POINT('Ctrl Pts',(-0.307089664032326,2.19783346940103,
10.117939751909));
#42965=CARTESIAN_POINT('Ctrl Pts',(-0.30573213545481,2.20192803298355,10.117669683351));
#42966=CARTESIAN_POINT('Ctrl Pts',(-0.305562294710364,2.20243606112507,
10.1176362198667));
#42967=CARTESIAN_POINT('Ctrl Pts',(-0.30530421929072,2.20320166390911,10.1175858604995));
#42968=CARTESIAN_POINT('Ctrl Pts',(-0.30521692463703,2.20345955087256,10.1175689094299));
#42969=CARTESIAN_POINT('Ctrl Pts',(-0.305059069943524,2.20392394861108,
10.1175384064259));
#42970=CARTESIAN_POINT('Ctrl Pts',(-0.304988627112674,2.2041304978505,10.1175248475924));
#42971=CARTESIAN_POINT('Ctrl Pts',(-0.304836638538316,2.2045746744916,10.1174957069249));
#42972=CARTESIAN_POINT('Ctrl Pts',(-0.304755024970108,2.20481227741475,
10.1174801292341));
#42973=CARTESIAN_POINT('Ctrl Pts',(-0.304534102242949,2.20545301379606,
10.1174381490695));
#42974=CARTESIAN_POINT('Ctrl Pts',(-0.304394269865006,2.20585596830555,
10.1174117776608));
#42975=CARTESIAN_POINT('Ctrl Pts',(-0.303743346225721,2.20771977789344,
10.1172899324101));
#42976=CARTESIAN_POINT('Ctrl Pts',(-0.303222524836559,2.2091772484648,10.1171950270397));
#42977=CARTESIAN_POINT('Ctrl Pts',(-0.291885997197875,2.24019449508783,
10.1151821921667));
#42978=CARTESIAN_POINT('Ctrl Pts',(-0.276806062846409,2.26802116132223,
10.1134980411939));
#42979=CARTESIAN_POINT('Ctrl Pts',(-0.253686308562861,2.29888302171432,
10.1113150609373));
#42980=CARTESIAN_POINT('Ctrl Pts',(-0.249260761820422,2.30440221290151,
10.110911066259));
#42981=CARTESIAN_POINT('Ctrl Pts',(-0.237701694976071,2.31788362479289,
10.1098820233748));
#42982=CARTESIAN_POINT('Ctrl Pts',(-0.230347476959078,2.32564434936758,
10.1092499782684));
#42983=CARTESIAN_POINT('Ctrl Pts',(-0.221719771297361,2.33388688615347,
10.1085249330278));
#42984=CARTESIAN_POINT('Ctrl Pts',(-0.22081258398833,2.33474355195118,10.1084488915513));
#42985=CARTESIAN_POINT('Ctrl Pts',(-0.219588472391922,2.3358861177505,10.1083465367667));
#42986=CARTESIAN_POINT('Ctrl Pts',(-0.219275913257072,2.33617669575412,
10.1083204237822));
#42987=CARTESIAN_POINT('Ctrl Pts',(-0.218693804263142,2.33671571553767,
10.1082718310615));
#42988=CARTESIAN_POINT('Ctrl Pts',(-0.218424405603673,2.33696432018454,
10.1082493583156));
#42989=CARTESIAN_POINT('Ctrl Pts',(-0.217865231186964,2.33747856998585,
10.108202745465));
#42990=CARTESIAN_POINT('Ctrl Pts',(-0.217575392501089,2.3377441455399,10.1081786024608));
#42991=CARTESIAN_POINT('Ctrl Pts',(-0.216914028386872,2.33834792284827,
10.1081235525712));
#42992=CARTESIAN_POINT('Ctrl Pts',(-0.216542197232684,2.33868578686254,
10.1080926314698));
#42993=CARTESIAN_POINT('Ctrl Pts',(-0.215407693083005,2.33971181997201,
10.1079983741018));
#42994=CARTESIAN_POINT('Ctrl Pts',(-0.214642523986204,2.34039720824363,
10.107934920965));
#42995=CARTESIAN_POINT('Ctrl Pts',(-0.209099607407693,2.34531462816244,
10.1074760967494));
#42996=CARTESIAN_POINT('Ctrl Pts',(-0.204200641510692,2.34940729985432,
10.1070749724205));
#42997=CARTESIAN_POINT('Ctrl Pts',(-0.197848672282886,2.35440118381033,
10.1065597818018));
#42998=CARTESIAN_POINT('Ctrl Pts',(-0.196505417293216,2.3554401696114,10.1064511048776));
#42999=CARTESIAN_POINT('Ctrl Pts',(-0.190261421843346,2.36019140031748,
10.1059471673028));
#43000=CARTESIAN_POINT('Ctrl Pts',(-0.185263543514597,2.36377335980565,
10.105547253633));
#43001=CARTESIAN_POINT('Ctrl Pts',(-0.169603270706567,2.37433230840627,
10.1043052506307));
#43002=CARTESIAN_POINT('Ctrl Pts',(-0.158627726238927,2.3808214479617,10.1034494648409));
#43003=CARTESIAN_POINT('Ctrl Pts',(-0.137297717399238,2.39178231562937,
10.1018281959589));
#43004=CARTESIAN_POINT('Ctrl Pts',(-0.127035467839363,2.39639430087592,
10.1010651243515));
#43005=CARTESIAN_POINT('Ctrl Pts',(-0.105972115751367,2.40456508181908,
10.0995531464768));
#43006=CARTESIAN_POINT('Ctrl Pts',(-0.0951804873906182,2.40810827966795,
10.0988055092198));
#43007=CARTESIAN_POINT('Ctrl Pts',(-0.0827165842986341,2.41148287085239,
10.0979885942502));
#43008=CARTESIAN_POINT('Ctrl Pts',(-0.081206913461176,2.4118798640383,10.0978904135174));
#43009=CARTESIAN_POINT('Ctrl Pts',(-0.0792939039620157,2.41236808935681,
10.0977670220605));
#43010=CARTESIAN_POINT('Ctrl Pts',(-0.0788932270376829,2.41246952681196,
10.0977412343538));
#43011=CARTESIAN_POINT('Ctrl Pts',(-0.0782539623965361,2.41263005838896,
10.0977001822613));
#43012=CARTESIAN_POINT('Ctrl Pts',(-0.0780155020060391,2.41268965043116,
10.0976848891038));
#43013=CARTESIAN_POINT('Ctrl Pts',(-0.0775644227889487,2.41280182850157,
10.0976559986108));
#43014=CARTESIAN_POINT('Ctrl Pts',(-0.0773518202869763,2.41285447015362,
10.097642398165));
#43015=CARTESIAN_POINT('Ctrl Pts',(-0.076866722751274,2.41297405849796,
10.0976114026443));
#43016=CARTESIAN_POINT('Ctrl Pts',(-0.0765941943045591,2.41304086595759,
10.0975940157387));
#43017=CARTESIAN_POINT('Ctrl Pts',(-0.0757612032789912,2.41324391196034,
10.0975409518931));
#43018=CARTESIAN_POINT('Ctrl Pts',(-0.0752004580343544,2.41337900284813,
10.097505341078));
#43019=CARTESIAN_POINT('Ctrl Pts',(-0.0711124136956874,2.41435226189732,
10.0972465071859));
#43020=CARTESIAN_POINT('Ctrl Pts',(-0.0675713803009467,2.41513240263841,
10.0970265470143));
#43021=CARTESIAN_POINT('Ctrl Pts',(-0.0398524872201292,2.42075053288999,
10.0953323217932));
#43022=CARTESIAN_POINT('Ctrl Pts',(-0.01520152465871,2.42285969969594,10.0939840630197));
#43023=CARTESIAN_POINT('Ctrl Pts',(0.0222284425364871,2.42176149852903,
10.0918834827467));
#43024=CARTESIAN_POINT('Ctrl Pts',(0.0349709647895566,2.42062682508333,
10.091159828552));
#43025=CARTESIAN_POINT('Ctrl Pts',(0.0541172346379056,2.41776684339642,
10.0900325041495));
#43026=CARTESIAN_POINT('Ctrl Pts',(0.060591126940391,2.41659619159425,10.089644391292));
#43027=CARTESIAN_POINT('Ctrl Pts',(0.070529094835069,2.41448316461107,10.0890353207473));
#43028=CARTESIAN_POINT('Ctrl Pts',(0.0740210384586993,2.41367961095249,
10.0888187505667));
#43029=CARTESIAN_POINT('Ctrl Pts',(0.0782778912461906,2.41262500168678,
10.0885513625044));
#43030=CARTESIAN_POINT('Ctrl Pts',(0.079056298122792,2.41242906658376,10.0885023291108));
#43031=CARTESIAN_POINT('Ctrl Pts',(0.0802011898678842,2.41213632990032,
10.0884300027874));
#43032=CARTESIAN_POINT('Ctrl Pts',(0.0805682531630738,2.41204178547141,
10.0884067828422));
#43033=CARTESIAN_POINT('Ctrl Pts',(0.0812791306576516,2.41185734692955,
10.0883617523849));
#43034=CARTESIAN_POINT('Ctrl Pts',(0.0816229647808132,2.41176753123623,
10.0883399444388));
#43035=CARTESIAN_POINT('Ctrl Pts',(0.082330285709921,2.41158151591081,10.0882950245047));
#43036=CARTESIAN_POINT('Ctrl Pts',(0.0826937540325095,2.41148524851829,
10.0882719103474));
#43037=CARTESIAN_POINT('Ctrl Pts',(0.0835676497070665,2.41125215309455,
10.0882162606517));
#43038=CARTESIAN_POINT('Ctrl Pts',(0.0840779093554974,2.4111147055937,10.0881837050567));
#43039=CARTESIAN_POINT('Ctrl Pts',(0.0856408400567726,2.41068957661684,
10.0880837946781));
#43040=CARTESIAN_POINT('Ctrl Pts',(0.0866923817143451,2.41039780509801,
10.0880163071685));
#43041=CARTESIAN_POINT('Ctrl Pts',(0.0991974009266791,2.40685953340229,
10.0872105065631));
#43042=CARTESIAN_POINT('Ctrl Pts',(0.11046261599593,2.40298654826912,10.0864517047593));
#43043=CARTESIAN_POINT('Ctrl Pts',(0.145614598909193,2.38868000602228,10.083974147244));
#43044=CARTESIAN_POINT('Ctrl Pts',(0.168461385669334,2.37597139833511,10.0821865246162));
#43045=CARTESIAN_POINT('Ctrl Pts',(0.198709220412049,2.35397785761062,10.079683643709));
#43046=CARTESIAN_POINT('Ctrl Pts',(0.207534718826404,2.34681877113475,10.0789356189322));
#43047=CARTESIAN_POINT('Ctrl Pts',(0.217123610877008,2.33816160703279,10.0781183174426));
#43048=CARTESIAN_POINT('Ctrl Pts',(0.218274934662435,2.33710686746058,10.0780201100507));
#43049=CARTESIAN_POINT('Ctrl Pts',(0.21972132695564,2.33576234849268,10.0778966898337));
#43050=CARTESIAN_POINT('Ctrl Pts',(0.220023539461164,2.33548033585304,10.0778708997022));
#43051=CARTESIAN_POINT('Ctrl Pts',(0.220504597472854,2.33502969713769,10.0778298446499));
#43052=CARTESIAN_POINT('Ctrl Pts',(0.220683792803222,2.33486144774793,10.0778145509501));
#43053=CARTESIAN_POINT('Ctrl Pts',(0.221022296633268,2.33454289157154,10.0777856600161));
#43054=CARTESIAN_POINT('Ctrl Pts',(0.221181643081175,2.33439262863835,10.0777720596704));
#43055=CARTESIAN_POINT('Ctrl Pts',(0.221544775322975,2.33404949664125,10.0777410651604));
#43056=CARTESIAN_POINT('Ctrl Pts',(0.221748462158523,2.33385652413968,10.0777236791637));
#43057=CARTESIAN_POINT('Ctrl Pts',(0.222370035760419,2.33326610429487,10.0776706207997));
#43058=CARTESIAN_POINT('Ctrl Pts',(0.222787110817126,2.33286779829533,10.0776350145374));
#43059=CARTESIAN_POINT('Ctrl Pts',(0.225817231897343,2.32995844563729,10.0773762784198));
#43060=CARTESIAN_POINT('Ctrl Pts',(0.228388957410542,2.32740447611739,10.0771564087011));
#43061=CARTESIAN_POINT('Ctrl Pts',(0.252283850739779,2.30286018615077,10.0751044007694));
#43062=CARTESIAN_POINT('Ctrl Pts',(0.270415585602447,2.27797584412988,10.0734648398319));
#43063=CARTESIAN_POINT('Ctrl Pts',(0.290098639794037,2.24083261814496,10.07107543535));
#43064=CARTESIAN_POINT('Ctrl Pts',(0.294896447858766,2.23048791291838,10.0704170032287));
#43065=CARTESIAN_POINT('Ctrl Pts',(0.300463205362311,2.21660085570194,10.069528388724));
#43066=CARTESIAN_POINT('Ctrl Pts',(0.301735221928695,2.21326849373299,10.0693148477026));
#43067=CARTESIAN_POINT('Ctrl Pts',(0.303461710412642,2.20850991946455,10.0690091700895));
#43068=CARTESIAN_POINT('Ctrl Pts',(0.303961988309701,2.2071005222001,10.0689185433705));
#43069=CARTESIAN_POINT('Ctrl Pts',(0.304710566600814,2.20494410801539,10.0687797231434));
#43070=CARTESIAN_POINT('Ctrl Pts',(0.304965974502683,2.20419956614008,10.0687317641293));
#43071=CARTESIAN_POINT('Ctrl Pts',(0.305426453901111,2.20284102260284,10.0686441991254));
#43072=CARTESIAN_POINT('Ctrl Pts',(0.305632408491317,2.20222732287784,10.0686046224626));
#43073=CARTESIAN_POINT('Ctrl Pts',(0.305971105406613,2.20120790732546,10.068538846021));
#43074=CARTESIAN_POINT('Ctrl Pts',(0.306104893788574,2.20080253888099,10.0685126808088));
#43075=CARTESIAN_POINT('Ctrl Pts',(0.306360305359024,2.20002346411796,10.0684623756392));
#43076=CARTESIAN_POINT('Ctrl Pts',(0.306482051215201,2.19964979856769,10.068438239776));
#43077=CARTESIAN_POINT('Ctrl Pts',(0.306757585183341,2.19879884116886,10.0683832556798));
#43078=CARTESIAN_POINT('Ctrl Pts',(0.306910943129306,2.19832141204627,10.0683523933568));
#43079=CARTESIAN_POINT('Ctrl Pts',(0.307363350304337,2.1969016201845,10.0682605728334));
#43080=CARTESIAN_POINT('Ctrl Pts',(0.307659175984739,2.19595824353433,10.0681995089459));
#43081=CARTESIAN_POINT('Ctrl Pts',(0.309678354745062,2.18941383427287,10.0677755034296));
#43082=CARTESIAN_POINT('Ctrl Pts',(0.311252901154919,2.1837683794723,10.0674077242376));
#43083=CARTESIAN_POINT('Ctrl Pts',(0.312961178244143,2.17692785680348,10.0669592815705));
#43084=CARTESIAN_POINT('Ctrl Pts',(0.313243345746615,2.17577071021195,10.0668833282047));
#43085=CARTESIAN_POINT('Ctrl Pts',(0.320891644032214,2.14363263204022,10.0647711886882));
#43086=CARTESIAN_POINT('Ctrl Pts',(0.3236306162865,2.11173451208725,10.0625809613985));
#43087=CARTESIAN_POINT('Ctrl Pts',(0.321114975689018,2.07134975382454,10.0598775156433));
#43088=CARTESIAN_POINT('Ctrl Pts',(0.320232533196219,2.06276005330485,10.059308253438));
#43089=CARTESIAN_POINT('Ctrl Pts',(0.318509799473951,2.05075680522363,10.05852968785));
#43090=CARTESIAN_POINT('Ctrl Pts',(0.317957157957463,2.04730623594852,10.0583078698918));
#43091=CARTESIAN_POINT('Ctrl Pts',(0.317256915639011,2.04334753819743,10.0580562149974));
#43092=CARTESIAN_POINT('Ctrl Pts',(0.317164086560611,2.04283012896168,10.0580233790373));
#43093=CARTESIAN_POINT('Ctrl Pts',(0.317021627833639,2.04204712162714,10.0579737745547));
#43094=CARTESIAN_POINT('Ctrl Pts',(0.316972930028647,2.04178135817173,10.0579569532872));
#43095=CARTESIAN_POINT('Ctrl Pts',(0.316888114847453,2.04132174871779,10.0579278893369));
#43096=CARTESIAN_POINT('Ctrl Pts',(0.31685215384638,2.04112787494252,10.0579156377147));
#43097=CARTESIAN_POINT('Ctrl Pts',(0.316776733186256,2.04072333618625,10.0578900905857));
#43098=CARTESIAN_POINT('Ctrl Pts',(0.316737241427864,2.04051267820464,10.0578767969841));
#43099=CARTESIAN_POINT('Ctrl Pts',(0.31663961497295,2.03999476992276,10.0578441378509));
#43100=CARTESIAN_POINT('Ctrl Pts',(0.316581243038617,2.03968756376258,10.05782478591));
#43101=CARTESIAN_POINT('Ctrl Pts',(0.316352932096357,2.03849544797276,10.0577497679926));
#43102=CARTESIAN_POINT('Ctrl Pts',(0.316179727128979,2.03761115673253,10.0576942866655));
#43103=CARTESIAN_POINT('Ctrl Pts',(0.312891692424119,2.02118965111645,10.0566668710805));
#43104=CARTESIAN_POINT('Ctrl Pts',(0.308638297132342,2.00589987146619,10.0557578937949));
#43105=CARTESIAN_POINT('Ctrl Pts',(0.296240964791316,1.97141144097039,10.0536919400521));
#43106=CARTESIAN_POINT('Ctrl Pts',(0.287327840234406,1.95256718710399,10.0525485720161));
#43107=CARTESIAN_POINT('Ctrl Pts',(0.270390434237204,1.92421695238188,10.050653856929));
#43108=CARTESIAN_POINT('Ctrl Pts',(0.263528127440062,1.91408727580639,10.0499375451591));
#43109=CARTESIAN_POINT('Ctrl Pts',(0.255252176139032,1.90325273054783,10.049113611773));
#43110=CARTESIAN_POINT('Ctrl Pts',(0.254389440072215,1.90213849757197,10.0490281673853));
#43111=CARTESIAN_POINT('Ctrl Pts',(0.252855227652787,1.9001836671427,10.0488769834624));
#43112=CARTESIAN_POINT('Ctrl Pts',(0.252186793683828,1.89934070149784,10.0488113648431));
#43113=CARTESIAN_POINT('Ctrl Pts',(0.251194974773575,1.89810269719179,10.0487143599643));
#43114=CARTESIAN_POINT('Ctrl Pts',(0.250874847083431,1.89770504868175,10.0486831044575));
#43115=CARTESIAN_POINT('Ctrl Pts',(0.250318364242457,1.89701716267315,10.0486288660998));
#43116=CARTESIAN_POINT('Ctrl Pts',(0.250082445113057,1.89672657239415,10.048605900858));
#43117=CARTESIAN_POINT('Ctrl Pts',(0.24961213210839,1.89614932857523,10.0485601759538));
#43118=CARTESIAN_POINT('Ctrl Pts',(0.24937774934492,1.89586266665327,10.0485374167606));
#43119=CARTESIAN_POINT('Ctrl Pts',(0.248821359932251,1.89518456263703,10.0484834557578));
#43120=CARTESIAN_POINT('Ctrl Pts',(0.248498923536025,1.8947934758896,10.0484522365249));
#43121=CARTESIAN_POINT('Ctrl Pts',(0.247364916840373,1.89342461853874,10.0483426192306));
#43122=CARTESIAN_POINT('Ctrl Pts',(0.246548495519373,1.89245089835831,10.0482640234958));
#43123=CARTESIAN_POINT('Ctrl Pts',(0.234871704821368,1.87869047620885,10.0471443863688));
#43124=CARTESIAN_POINT('Ctrl Pts',(0.223036685775311,1.86676814607881,10.0460619688402));
#43125=CARTESIAN_POINT('Ctrl Pts',(0.194469139846209,1.84216067223422,10.0435594611397));
#43126=CARTESIAN_POINT('Ctrl Pts',(0.177315769270858,1.83007706165624,10.0421266493883));
#43127=CARTESIAN_POINT('Ctrl Pts',(0.148177984968654,1.81353428856733,10.039883571533));
#43128=CARTESIAN_POINT('Ctrl Pts',(0.136886513768707,1.80797006349781,10.0390560840142));
#43129=CARTESIAN_POINT('Ctrl Pts',(0.124659281116331,1.80281029815124,10.0382236044869));
#43130=CARTESIAN_POINT('Ctrl Pts',(0.12402034133007,1.80254309520393,10.0381802818811));
#43131=CARTESIAN_POINT('Ctrl Pts',(0.123101140871952,1.80216216457543,10.0381182185526));
#43132=CARTESIAN_POINT('Ctrl Pts',(0.122821579338308,1.80204677087669,10.038099377624));
#43133=CARTESIAN_POINT('Ctrl Pts',(0.122336342135631,1.80184728008658,10.0380667360205));
#43134=CARTESIAN_POINT('Ctrl Pts',(0.122130741510867,1.80176300199657,10.0380529242923));
#43135=CARTESIAN_POINT('Ctrl Pts',(0.121733206233193,1.80160052768474,10.0380262555862));
#43136=CARTESIAN_POINT('Ctrl Pts',(0.121541283793706,1.80152230416289,10.0380133969313));
#43137=CARTESIAN_POINT('Ctrl Pts',(0.121083594931224,1.80133627452097,10.0379827711138));
#43138=CARTESIAN_POINT('Ctrl Pts',(0.12081775924943,1.80122863770115,10.0379650142728));
#43139=CARTESIAN_POINT('Ctrl Pts',(0.119871906633108,1.800847130967,10.0379019448621));
#43140=CARTESIAN_POINT('Ctrl Pts',(0.119191092694471,1.80057522397447,10.0378567503022));
#43141=CARTESIAN_POINT('Ctrl Pts',(0.109104809388386,1.79658676431529,10.0371900931612));
#43142=CARTESIAN_POINT('Ctrl Pts',(0.0995293102140311,1.79331218692966,
10.0365944258341));
#43143=CARTESIAN_POINT('Ctrl Pts',(0.0640982872391286,1.78303059544257,
10.0344702615992));
#43144=CARTESIAN_POINT('Ctrl Pts',(0.0375515841675513,1.77880186724202,
10.0330215100762));
#43145=CARTESIAN_POINT('Ctrl Pts',(0.00305160629579006,1.77764653690111,
10.0310410290353));
#43146=CARTESIAN_POINT('Ctrl Pts',(-0.00468940555814354,1.7776662218976,
10.030591126381));
#43147=CARTESIAN_POINT('Ctrl Pts',(-0.0185481650303265,1.77820079400813,
10.0297701632972));
#43148=CARTESIAN_POINT('Ctrl Pts',(-0.0246661630684275,1.77861186061775,
10.0294023306781));
#43149=CARTESIAN_POINT('Ctrl Pts',(-0.0317006599856948,1.77928654402572,
10.0289719121467));
#43150=CARTESIAN_POINT('Ctrl Pts',(-0.0326324956545053,1.77938001795773,
10.0289147450226));
#43151=CARTESIAN_POINT('Ctrl Pts',(-0.0340451421202877,1.77952794497241,
10.0288278470609));
#43152=CARTESIAN_POINT('Ctrl Pts',(-0.0345262650427791,1.77957942205013,
10.0287982099866));
#43153=CARTESIAN_POINT('Ctrl Pts',(-0.0353591133794374,1.77967042909022,
10.0287468348102));
#43154=CARTESIAN_POINT('Ctrl Pts',(-0.0357108939321741,1.77970945541402,
10.0287251126152));
#43155=CARTESIAN_POINT('Ctrl Pts',(-0.0364405615694661,1.77979162135027,
10.0286800097669));
#43156=CARTESIAN_POINT('Ctrl Pts',(-0.0368184378454589,1.77983485055728,
10.0286566263195));
#43157=CARTESIAN_POINT('Ctrl Pts',(-0.0377369484826849,1.77994157617379,
10.0285997245305));
#43158=CARTESIAN_POINT('Ctrl Pts',(-0.0382774987910083,1.78000577345302,
10.0285661841251));
#43159=CARTESIAN_POINT('Ctrl Pts',(-0.0403094183755431,1.78025231220636,
10.0284399041278));
#43160=CARTESIAN_POINT('Ctrl Pts',(-0.041799651003758,1.78044371057293,
10.0283468790925));
#43161=CARTESIAN_POINT('Ctrl Pts',(-0.0682995418918661,1.78403576837955,
10.026685214084));
#43162=CARTESIAN_POINT('Ctrl Pts',(-0.0928202254584118,1.7903516388729,
10.0250186242543));
#43163=CARTESIAN_POINT('Ctrl Pts',(-0.130982357759135,1.80512535971778,
10.0222545370275));
#43164=CARTESIAN_POINT('Ctrl Pts',(-0.145183608765201,1.8118521525183,10.0211863666889));
#43165=CARTESIAN_POINT('Ctrl Pts',(-0.164360709565477,1.8227149293279,10.0197281524638));
#43166=CARTESIAN_POINT('Ctrl Pts',(-0.169789601093856,1.82600555492843,
10.0193136117893));
#43167=CARTESIAN_POINT('Ctrl Pts',(-0.177618913456452,1.83107329735673,
10.0187169725749));
#43168=CARTESIAN_POINT('Ctrl Pts',(-0.180097254258496,1.832726674774,10.0185282949015));
#43169=CARTESIAN_POINT('Ctrl Pts',(-0.182968213115632,1.83470005054465,
10.018310278956));
#43170=CARTESIAN_POINT('Ctrl Pts',(-0.183383339477102,1.83498682862508,
10.0182787686229));
#43171=CARTESIAN_POINT('Ctrl Pts',(-0.184016087661491,1.83542614314818,
10.0182307626915));
#43172=CARTESIAN_POINT('Ctrl Pts',(-0.184234194730501,1.83557797417591,
10.0182142193399));
#43173=CARTESIAN_POINT('Ctrl Pts',(-0.184629083903442,1.83585359442723,
10.0181842751113));
#43174=CARTESIAN_POINT('Ctrl Pts',(-0.184805928771692,1.83597729095465,
10.0181708680005));
#43175=CARTESIAN_POINT('Ctrl Pts',(-0.18516437036028,1.83622854433962,10.0181436994989));
#43176=CARTESIAN_POINT('Ctrl Pts',(-0.185345958793273,1.83635611057367,
10.0181299388684));
#43177=CARTESIAN_POINT('Ctrl Pts',(-0.185868051887956,1.83672368799987,
10.0180903834698));
#43178=CARTESIAN_POINT('Ctrl Pts',(-0.186208224727613,1.83696417312192,
10.018064621225));
#43179=CARTESIAN_POINT('Ctrl Pts',(-0.187698832711067,1.83802229894201,
10.0179517740247));
#43180=CARTESIAN_POINT('Ctrl Pts',(-0.188844378291509,1.83884684835942,
10.0178651566286));
#43181=CARTESIAN_POINT('Ctrl Pts',(-0.210017328042146,1.85429904328435,
10.0162654589097));
#43182=CARTESIAN_POINT('Ctrl Pts',(-0.228299263844469,1.87118540841104,
10.0149008792548));
#43183=CARTESIAN_POINT('Ctrl Pts',(-0.260594661000986,1.90878193117505,
10.0121278900786));
#43184=CARTESIAN_POINT('Ctrl Pts',(-0.274504581900125,1.92935153722198,
10.0107256188471));
#43185=CARTESIAN_POINT('Ctrl Pts',(-0.28645522827859,1.95233176310571,10.009150554318));
#43186=CARTESIAN_POINT('Ctrl Pts',(-0.286981889916914,1.95335791599553,
10.009080225143));
#43187=CARTESIAN_POINT('Ctrl Pts',(-0.287741048973956,1.95485682283767,
10.0089774917182));
#43188=CARTESIAN_POINT('Ctrl Pts',(-0.287977917823889,1.95532736270456,
10.0089452409794));
#43189=CARTESIAN_POINT('Ctrl Pts',(-0.288391061362612,1.95615310711098,
10.0088886429157));
#43190=CARTESIAN_POINT('Ctrl Pts',(-0.288567836625784,1.95650806109568,
10.0088643131732));
#43191=CARTESIAN_POINT('Ctrl Pts',(-0.288909421908162,1.9571971276497,10.0088170808077));
#43192=CARTESIAN_POINT('Ctrl Pts',(-0.289074308655236,1.95753120168791,
10.0087941809118));
#43193=CARTESIAN_POINT('Ctrl Pts',(-0.28951076963833,1.95841938452501,10.0087332961776));
#43194=CARTESIAN_POINT('Ctrl Pts',(-0.289781331302907,1.95897398667369,
10.0086952761154));
#43195=CARTESIAN_POINT('Ctrl Pts',(-0.290737243225128,1.9609477979679,10.0085599536462));
#43196=CARTESIAN_POINT('Ctrl Pts',(-0.291413765317225,1.96237123581862,
10.008462345224));
#43197=CARTESIAN_POINT('Ctrl Pts',(-0.302478602737599,1.98609961421407,
10.006834753535));
#43198=CARTESIAN_POINT('Ctrl Pts',(-0.310287119609825,2.0095123061569,10.0052121268332));
#43199=CARTESIAN_POINT('Ctrl Pts',(-0.318653451112574,2.04923482588306,
10.0024717411476));
#43200=CARTESIAN_POINT('Ctrl Pts',(-0.320780473736779,2.06511389630568,
10.001382024296));
#43201=CARTESIAN_POINT('Ctrl Pts',(-0.322090856425951,2.08740249954927,
9.99990349791909));
#43202=CARTESIAN_POINT('Ctrl Pts',(-0.322276135752653,2.09372942164882,
9.99948967543666));
#43203=CARTESIAN_POINT('Ctrl Pts',(-0.322274427660535,2.1032036216054,9.99888259274212));
#43204=CARTESIAN_POINT('Ctrl Pts',(-0.3222278084343,2.10634911052634,9.99868311965728));
#43205=CARTESIAN_POINT('Ctrl Pts',(-0.322119078848428,2.11003852156452,
9.99845198836603));
#43206=CARTESIAN_POINT('Ctrl Pts',(-0.322101635213386,2.110583452961,9.99841792256334));
#43207=CARTESIAN_POINT('Ctrl Pts',(-0.322073210953433,2.11140612405797,
9.99836660649659));
#43208=CARTESIAN_POINT('Ctrl Pts',(-0.32206325386039,2.11168389464756,9.99834929923402));
#43209=CARTESIAN_POINT('Ctrl Pts',(-0.322044818626816,2.11218024084605,
9.9983184079959));
#43210=CARTESIAN_POINT('Ctrl Pts',(-0.322036477318266,2.11239882046523,
9.99830481633854));
#43211=CARTESIAN_POINT('Ctrl Pts',(-0.322018227529482,2.11286460140716,
9.99827587925237));
#43212=CARTESIAN_POINT('Ctrl Pts',(-0.322008256967211,2.11311179913358,
9.99826053739987));
#43213=CARTESIAN_POINT('Ctrl Pts',(-0.321980571357155,2.11377911857146,
9.99821916287334));
#43214=CARTESIAN_POINT('Ctrl Pts',(-0.321962318626598,2.11419921932475,
9.99819316044732));
#43215=CARTESIAN_POINT('Ctrl Pts',(-0.321868808545783,2.11625848123244,
9.99806591283297));
#43216=CARTESIAN_POINT('Ctrl Pts',(-0.321781853616707,2.11789712482943,
9.99796531443234));
#43217=CARTESIAN_POINT('Ctrl Pts',(-0.321211848651136,2.12728334796018,
9.9973924903088));
#43218=CARTESIAN_POINT('Ctrl Pts',(-0.32046147700495,2.13501279660081,9.99693407346861));
#43219=CARTESIAN_POINT('Ctrl Pts',(-0.317373799432371,2.15810681107936,
9.99558448835812));
#43220=CARTESIAN_POINT('Ctrl Pts',(-0.314204109480535,2.17333738151107,
9.99472060000492));
#43221=CARTESIAN_POINT('Ctrl Pts',(-0.303005055353753,2.2126565419427,9.99243493162794));
#43222=CARTESIAN_POINT('Ctrl Pts',(-0.293212390040804,2.23612420541474,
9.99100641944024));
#43223=CARTESIAN_POINT('Ctrl Pts',(-0.2799927778458,2.25958617438035,9.98937395786617));
#43224=CARTESIAN_POINT('Ctrl Pts',(-0.279202197387143,2.26096532400603,
9.98927723262625));
#43225=CARTESIAN_POINT('Ctrl Pts',(-0.278089489355844,2.26287355552748,
9.98914231194009));
#43226=CARTESIAN_POINT('Ctrl Pts',(-0.277775982250721,2.26340765850033,
9.98910442899438));
#43227=CARTESIAN_POINT('Ctrl Pts',(-0.277271204202263,2.26426196778395,
9.98904364143787));
#43228=CARTESIAN_POINT('Ctrl Pts',(-0.277080912458586,2.26458275331653,
9.98902077249597));
#43229=CARTESIAN_POINT('Ctrl Pts',(-0.276687281689178,2.26524370134464,
9.98897356253363));
#43230=CARTESIAN_POINT('Ctrl Pts',(-0.27648387129758,2.26558382044372,9.98894921893539));
#43231=CARTESIAN_POINT('Ctrl Pts',(-0.276009377259191,2.26637390192887,
9.98889255370635));
#43232=CARTESIAN_POINT('Ctrl Pts',(-0.275737820354292,2.26682357746763,
9.98886021479901));
#43233=CARTESIAN_POINT('Ctrl Pts',(-0.274870614785753,2.26825169509022,
9.98875722898129));
#43234=CARTESIAN_POINT('Ctrl Pts',(-0.274270853349249,2.26922761808348,
9.98868643123666));
#43235=CARTESIAN_POINT('Ctrl Pts',(-0.262187115022523,2.28865711950061,
9.98726841125085));
#43236=CARTESIAN_POINT('Ctrl Pts',(-0.248873077788396,2.30590152937929,
9.98584990813407));
#43237=CARTESIAN_POINT('Ctrl Pts',(-0.214830239536102,2.3418265075295,9.98252691750616));
#43238=CARTESIAN_POINT('Ctrl Pts',(-0.1932073726006,2.35942851485318,9.9806075647171));
#43239=CARTESIAN_POINT('Ctrl Pts',(-0.168344444614696,2.37481536929332,
9.97875874962293));
#43240=CARTESIAN_POINT('Ctrl Pts',(-0.167088357873659,2.37558087758689,
9.97866625120993));
#43241=CARTESIAN_POINT('Ctrl Pts',(-0.16546409441007,2.37655557896717,9.97854784476274));
#43242=CARTESIAN_POINT('Ctrl Pts',(-0.165100711778827,2.37677266803609,
9.97852143183302));
#43243=CARTESIAN_POINT('Ctrl Pts',(-0.164523730722105,2.37711582266043,
9.97847961673739));
#43244=CARTESIAN_POINT('Ctrl Pts',(-0.164310414269465,2.37724235770004,
9.9784641839265));
#43245=CARTESIAN_POINT('Ctrl Pts',(-0.163927606569691,2.37746883454628,
9.97843653708687));
#43246=CARTESIAN_POINT('Ctrl Pts',(-0.163758171114338,2.37756886665066,
9.97842431716883));
#43247=CARTESIAN_POINT('Ctrl Pts',(-0.163359199415934,2.37780392097325,
9.97839558246649));
#43248=CARTESIAN_POINT('Ctrl Pts',(-0.163129587683745,2.37793881370778,
9.97837907623125));
#43249=CARTESIAN_POINT('Ctrl Pts',(-0.162462209276824,2.37832977453201,
9.97833118872053));
#43250=CARTESIAN_POINT('Ctrl Pts',(-0.16202400248376,2.37858509554819,9.97829985604492));
#43251=CARTESIAN_POINT('Ctrl Pts',(-0.158957264853038,2.38036224546542,
9.97808133759348));
#43252=CARTESIAN_POINT('Ctrl Pts',(-0.156307825888829,2.38184794821856,
9.97789644576719));
#43253=CARTESIAN_POINT('Ctrl Pts',(-0.148045826866276,2.38632861178732,
9.97733058097489));
#43254=CARTESIAN_POINT('Ctrl Pts',(-0.14236503606082,2.38919517351615,9.97695654454989));
#43255=CARTESIAN_POINT('Ctrl Pts',(-0.12228275084459,2.39859350017305,9.97567319543483));
#43256=CARTESIAN_POINT('Ctrl Pts',(-0.10748807371349,2.40423268843545,9.97479491325108));
#43257=CARTESIAN_POINT('Ctrl Pts',(-0.0683187311445838,2.41594662720813,
9.97250877154913));
#43258=CARTESIAN_POINT('Ctrl Pts',(-0.0435470809002119,2.42030160167511,
9.97109339465884));
#43259=CARTESIAN_POINT('Ctrl Pts',(-0.0170441859333898,2.42182738383034,
9.96948302173576));
#43260=CARTESIAN_POINT('Ctrl Pts',(-0.0155649931259492,2.42190231458012,
9.96939286242818));
#43261=CARTESIAN_POINT('Ctrl Pts',(-0.0135447902681954,2.4219906940448,
9.9692693284925));
#43262=CARTESIAN_POINT('Ctrl Pts',(-0.0130041691089597,2.422012981066,9.96923623090867));
#43263=CARTESIAN_POINT('Ctrl Pts',(-0.0120843380306304,2.42204858077036,
9.96917985031591));
#43264=CARTESIAN_POINT('Ctrl Pts',(-0.0117051547589277,2.42206258545804,
9.96915658902747));
#43265=CARTESIAN_POINT('Ctrl Pts',(-0.0109719679962917,2.42208836831021,
9.96911157320205));
#43266=CARTESIAN_POINT('Ctrl Pts',(-0.0106179678933904,2.42210023259645,
9.96908982139554));
#43267=CARTESIAN_POINT('Ctrl Pts',(-0.00977827451479799,2.42212698907843,
9.96903818493204));
#43268=CARTESIAN_POINT('Ctrl Pts',(-0.0092925667307152,2.42214136639785,
9.9690082841862));
#43269=CARTESIAN_POINT('Ctrl Pts',(-0.00786082108146649,2.42218050642356,
9.96892004764882));
#43270=CARTESIAN_POINT('Ctrl Pts',(-0.0069147106419934,2.42220220044805,
9.96886161585609));
#43271=CARTESIAN_POINT('Ctrl Pts',(0.000430746176232562,2.42233826149321,
9.96840697726688));
#43272=CARTESIAN_POINT('Ctrl Pts',(0.00683172553678939,2.42226612979754,
9.9680049603652));
#43273=CARTESIAN_POINT('Ctrl Pts',(0.0164802454951995,2.42186982671293,
9.9673895424762));
#43274=CARTESIAN_POINT('Ctrl Pts',(0.0197322176373569,2.42168683875623,
9.9671805066665));
#43275=CARTESIAN_POINT('Ctrl Pts',(0.0309153723111586,2.42088735575775,
9.9664560929486));
#43276=CARTESIAN_POINT('Ctrl Pts',(0.0388257315951886,2.42002656552045,
9.9659339414994));
#43277=CARTESIAN_POINT('Ctrl Pts',(0.0743421798614234,2.41482556262928,
9.96354939349386));
#43278=CARTESIAN_POINT('Ctrl Pts',(0.101342683735276,2.40719937007033,9.96161364461138));
#43279=CARTESIAN_POINT('Ctrl Pts',(0.127994942158417,2.3957694955005,9.95972886991709));
#43280=CARTESIAN_POINT('Ctrl Pts',(0.128967281588405,2.39534681312629,9.95966016489659));
#43281=CARTESIAN_POINT('Ctrl Pts',(0.130431308069238,2.39470178256397,9.95955682089262));
#43282=CARTESIAN_POINT('Ctrl Pts',(0.130924542684925,2.39448298915511,9.95952202179467));
#43283=CARTESIAN_POINT('Ctrl Pts',(0.134921117966737,2.39269812688596,9.95924020977094));
#43284=CARTESIAN_POINT('Ctrl Pts',(0.138396974080169,2.39107075145244,9.95899609736042));
#43285=CARTESIAN_POINT('Ctrl Pts',(0.142369733439022,2.38912346597851,9.95871892385743));
#43286=CARTESIAN_POINT('Ctrl Pts',(0.142895649236577,2.38886390051554,9.95868226907393));
#43287=CARTESIAN_POINT('Ctrl Pts',(0.143673856950674,2.38847717114101,9.95862808930645));
#43288=CARTESIAN_POINT('Ctrl Pts',(0.143926691189009,2.38835111063675,9.9586104959348));
#43289=CARTESIAN_POINT('Ctrl Pts',(0.144375441830021,2.38812663099788,9.95857928668488));
#43290=CARTESIAN_POINT('Ctrl Pts',(0.144571423523204,2.38802834443051,9.95856566249799));
#43291=CARTESIAN_POINT('Ctrl Pts',(0.144985921345089,2.38781994043295,9.95853685987343));
#43292=CARTESIAN_POINT('Ctrl Pts',(0.145204411796217,2.38770977441683,9.95852168459812));
#43293=CARTESIAN_POINT('Ctrl Pts',(0.145787232609275,2.38741507479854,9.95848122335879));
#43294=CARTESIAN_POINT('Ctrl Pts',(0.146151339539563,2.38723009655759,9.95845596538122));
#43295=CARTESIAN_POINT('Ctrl Pts',(0.147829914123303,2.38637330752127,9.9583396085866));
#43296=CARTESIAN_POINT('Ctrl Pts',(0.149140134923043,2.38569314853776,9.9582490275766));
#43297=CARTESIAN_POINT('Ctrl Pts',(0.159581464332736,2.38018146177653,9.95752874655522));
#43298=CARTESIAN_POINT('Ctrl Pts',(0.168481143155382,2.37492189206595,9.95692440920953));
#43299=CARTESIAN_POINT('Ctrl Pts',(0.201372335738656,2.35328540411384,9.9546691702936));
#43300=CARTESIAN_POINT('Ctrl Pts',(0.223363077614642,2.33412261094557,9.95310233313227));
#43301=CARTESIAN_POINT('Ctrl Pts',(0.243895946659408,2.31066678998633,9.95129085454785));
#43302=CARTESIAN_POINT('Ctrl Pts',(0.245285482959955,2.30904726923819,9.95116632754694));
#43303=CARTESIAN_POINT('Ctrl Pts',(0.247781625529479,2.3060788327349,9.95093895117049));
#43304=CARTESIAN_POINT('Ctrl Pts',(0.248893562213517,2.30473449582485,9.95083629517814));
#43305=CARTESIAN_POINT('Ctrl Pts',(0.254058750345577,2.29838548908786,9.95035280385406));
#43306=CARTESIAN_POINT('Ctrl Pts',(0.257972088933788,2.29326935456872,9.94996699589042));
#43307=CARTESIAN_POINT('Ctrl Pts',(0.262330314866976,2.28720321143833,9.94951237937307));
#43308=CARTESIAN_POINT('Ctrl Pts',(0.262927260730678,2.28636386988115,9.94944953859246));
#43309=CARTESIAN_POINT('Ctrl Pts',(0.263809696536688,2.28511043351522,9.94935578133985));
#43310=CARTESIAN_POINT('Ctrl Pts',(0.264098261236531,2.28469850294542,9.94932498267308));
#43311=CARTESIAN_POINT('Ctrl Pts',(0.26461068953753,2.2839633474271,9.94927004136994));
#43312=CARTESIAN_POINT('Ctrl Pts',(0.264834928629913,2.28364038441891,9.94924591312216));
#43313=CARTESIAN_POINT('Ctrl Pts',(0.265305929811726,2.28295936250936,9.94919505138741));
#43314=CARTESIAN_POINT('Ctrl Pts',(0.265552559159887,2.2826012131498,9.94916831291676));
#43315=CARTESIAN_POINT('Ctrl Pts',(0.266192951426772,2.28166720918872,9.94909860728448));
#43316=CARTESIAN_POINT('Ctrl Pts',(0.266585569229281,2.28109057554214,9.94905559682116));
#43317=CARTESIAN_POINT('Ctrl Pts',(0.268303054001373,2.27855043399833,9.94886623262979));
#43318=CARTESIAN_POINT('Ctrl Pts',(0.269608095662722,2.27657366887186,9.94871913397827));
#43319=CARTESIAN_POINT('Ctrl Pts',(0.278847560161128,2.26223725939757,9.94765398310607));
#43320=CARTESIAN_POINT('Ctrl Pts',(0.285949539159132,2.24936412936613,9.94670522712979));
#43321=CARTESIAN_POINT('Ctrl Pts',(0.301082257611119,2.21686949364581,9.94433090147214));
#43322=CARTESIAN_POINT('Ctrl Pts',(0.308104539559079,2.19685293314543,9.94288294783857));
#43323=CARTESIAN_POINT('Ctrl Pts',(0.315430119668036,2.16678882704539,9.94080898680035));
#43324=CARTESIAN_POINT('Ctrl Pts',(0.317312540636782,2.15718123311942,9.94016140148789));
#43325=CARTESIAN_POINT('Ctrl Pts',(0.319260964792439,2.14410665541701,9.93931264677654));
#43326=CARTESIAN_POINT('Ctrl Pts',(0.319712706564265,2.14070317303685,9.93909466106959));
#43327=CARTESIAN_POINT('Ctrl Pts',(0.320175631422935,2.13672958433276,9.93884410324045));
#43328=CARTESIAN_POINT('Ctrl Pts',(0.320239777906501,2.13616603351734,9.93880866027399));
#43329=CARTESIAN_POINT('Ctrl Pts',(0.320333222918022,2.13532533908251,9.93875592753803));
#43330=CARTESIAN_POINT('Ctrl Pts',(0.320363649842978,2.13504832588064,9.93873857454801));
#43331=CARTESIAN_POINT('Ctrl Pts',(0.320417326081064,2.13455373571113,9.9387076328236));
#43332=CARTESIAN_POINT('Ctrl Pts',(0.320440713096714,2.13433617473823,9.93869403630715));
#43333=CARTESIAN_POINT('Ctrl Pts',(0.320490022249684,2.13387303123522,9.93866512231968));
#43334=CARTESIAN_POINT('Ctrl Pts',(0.320515883628373,2.13362744339926,9.93864980835655));
#43335=CARTESIAN_POINT('Ctrl Pts',(0.320584808286457,2.13296560988164,9.9386085868841));
#43336=CARTESIAN_POINT('Ctrl Pts',(0.320627343347362,2.13254930785193,9.93858270923863));
#43337=CARTESIAN_POINT('Ctrl Pts',(0.320826191888578,2.13056490762895,9.93845959640086));
#43338=CARTESIAN_POINT('Ctrl Pts',(0.320971816750039,2.12899572502474,9.93836295471556));
#43339=CARTESIAN_POINT('Ctrl Pts',(0.322096081983343,2.11583249258218,9.93755775061893));
#43340=CARTESIAN_POINT('Ctrl Pts',(0.32245780670679,2.10419293988358,9.93688127269676));
#43341=CARTESIAN_POINT('Ctrl Pts',(0.321679383321662,2.07049203399388,9.93496109997406));
#43342=CARTESIAN_POINT('Ctrl Pts',(0.318904246982666,2.04853656503831,9.93375421829145));
#43343=CARTESIAN_POINT('Ctrl Pts',(0.3129719385023,2.02301433285571,9.93226130685605));
#43344=CARTESIAN_POINT('Ctrl Pts',(0.311959850441387,2.01901063427327,9.93202455944491));
#43345=CARTESIAN_POINT('Ctrl Pts',(0.307852385798196,2.00398349729733,9.93112419992008));
#43346=CARTESIAN_POINT('Ctrl Pts',(0.304247572103815,1.99310926153087,9.93044816898485));
#43347=CARTESIAN_POINT('Ctrl Pts',(0.299634031006727,1.98133211799154,9.92967928593688));
#43348=CARTESIAN_POINT('Ctrl Pts',(0.299189610870233,1.98021604680129,9.92960605344678));
#43349=CARTESIAN_POINT('Ctrl Pts',(0.298558116737004,1.97865561832781,9.92950313737762));
#43350=CARTESIAN_POINT('Ctrl Pts',(0.298376265985279,1.97820914678989,9.92947363027879));
#43351=CARTESIAN_POINT('Ctrl Pts',(0.298041504438547,1.97739250567677,9.9294195470382));
#43352=CARTESIAN_POINT('Ctrl Pts',(0.29788890383604,1.97702220931696,9.9293949814364));
#43353=CARTESIAN_POINT('Ctrl Pts',(0.297578944887952,1.97627403369104,9.92934526138899));
#43354=CARTESIAN_POINT('Ctrl Pts',(0.297421556106704,1.97589616790638,9.92932010594664));
#43355=CARTESIAN_POINT('Ctrl Pts',(0.297105031377695,1.9751403020841,9.92926969683701));
#43356=CARTESIAN_POINT('Ctrl Pts',(0.296945892911048,1.97476230394019,9.92924444312115));
#43357=CARTESIAN_POINT('Ctrl Pts',(0.29636080066708,1.97337993184939,9.92915192319876));
#43358=CARTESIAN_POINT('Ctrl Pts',(0.295930472863308,1.97237742748832,9.92908450814562));
#43359=CARTESIAN_POINT('Ctrl Pts',(0.292615373881578,1.96476139892518,9.92856989439813));
#43360=CARTESIAN_POINT('Ctrl Pts',(0.289514524806766,1.95824470859934,9.92811531981475));
#43361=CARTESIAN_POINT('Ctrl Pts',(0.280801322774155,1.94141381685969,9.92690191945861));
#43362=CARTESIAN_POINT('Ctrl Pts',(0.274839909389009,1.93129334741991,9.92613164837258));
#43363=CARTESIAN_POINT('Ctrl Pts',(0.260209445633106,1.90929662481274,9.92436918699135));
#43364=CARTESIAN_POINT('Ctrl Pts',(0.251252856615057,1.89764214254737,9.923371464577));
#43365=CARTESIAN_POINT('Ctrl Pts',(0.233272338496599,1.8772874060257,9.92153798110756));
#43366=CARTESIAN_POINT('Ctrl Pts',(0.224474209971092,1.86842222459683,9.92070216614003));
#43367=CARTESIAN_POINT('Ctrl Pts',(0.215048630320779,1.85996813753457,9.91988317028396));
#43368=CARTESIAN_POINT('Ctrl Pts',(0.214913754662031,1.85984736841161,9.91987146593201));
#43369=CARTESIAN_POINT('Ctrl Pts',(0.211508350184048,1.8568032988135,9.91957633107998));
#43370=CARTESIAN_POINT('Ctrl Pts',(0.208178370920202,1.85394677753,9.91929661495904));
#43371=CARTESIAN_POINT('Ctrl Pts',(0.204326190093038,1.85077651414553,9.91898397836417));
#43372=CARTESIAN_POINT('Ctrl Pts',(0.203860396397636,1.85039535931021,9.91894635344377));
#43373=CARTESIAN_POINT('Ctrl Pts',(0.20317111825768,1.8498345456569,9.91889094225948));
#43374=CARTESIAN_POINT('Ctrl Pts',(0.202948460844892,1.84965387943292,9.91887308357512));
#43375=CARTESIAN_POINT('Ctrl Pts',(0.202554168861857,1.84933481910675,9.91884153111645));
#43376=CARTESIAN_POINT('Ctrl Pts',(0.202382633184889,1.84919630381134,9.91882782852744));
#43377=CARTESIAN_POINT('Ctrl Pts',(0.202024023594359,1.84890733354367,9.91879923285478));
#43378=CARTESIAN_POINT('Ctrl Pts',(0.201836924106067,1.8487569118847,9.91878434219066));
#43379=CARTESIAN_POINT('Ctrl Pts',(0.201347183744103,1.84836407733003,9.91874543981633));
#43380=CARTESIAN_POINT('Ctrl Pts',(0.201044271995156,1.84812200040232,9.91872145239876));
#43381=CARTESIAN_POINT('Ctrl Pts',(0.199743205868219,1.84708607425493,9.9186187362274));
#43382=CARTESIAN_POINT('Ctrl Pts',(0.198740763297477,1.84629759311834,9.9185403878987));
#43383=CARTESIAN_POINT('Ctrl Pts',(0.196105743028156,1.84425019422551,9.91833642652194));
#43384=CARTESIAN_POINT('Ctrl Pts',(0.19446569281328,1.84300093305569,9.91821145293172));
#43385=CARTESIAN_POINT('Ctrl Pts',(0.188257270686234,1.8383653090094,9.91774525227942));
#43386=CARTESIAN_POINT('Ctrl Pts',(0.183611283871766,1.83508413412942,9.91741021433531));
#43387=CARTESIAN_POINT('Ctrl Pts',(0.161238713334929,1.82015526854867,9.91584871759364));
#43388=CARTESIAN_POINT('Ctrl Pts',(0.142476617277192,1.81015254588702,9.91468602094042));
#43389=CARTESIAN_POINT('Ctrl Pts',(0.103897293103256,1.79424265276844,9.9123386514134));
#43390=CARTESIAN_POINT('Ctrl Pts',(0.0842274701162847,1.78825050759077,
9.91116056863902));
#43391=CARTESIAN_POINT('Ctrl Pts',(0.0628509912032709,1.783910433408,9.90983574671813));
#43392=CARTESIAN_POINT('Ctrl Pts',(0.061577117259003,1.78365980376095,9.909756650878));
#43393=CARTESIAN_POINT('Ctrl Pts',(0.059799250334402,1.78332116114134,9.90964604636691));
#43394=CARTESIAN_POINT('Ctrl Pts',(0.0592964977090335,1.78322663831044,
9.90961474521436));
#43395=CARTESIAN_POINT('Ctrl Pts',(0.0584282511968487,1.78306553815482,
9.90956064647477));
#43396=CARTESIAN_POINT('Ctrl Pts',(0.058062862257227,1.78299839485006,9.90953786694847));
#43397=CARTESIAN_POINT('Ctrl Pts',(0.0573066411346103,1.7828607841615,9.90949069474523));
#43398=CARTESIAN_POINT('Ctrl Pts',(0.0569157933064921,1.78279040712664,
9.90946629923456));
#43399=CARTESIAN_POINT('Ctrl Pts',(0.0561412495934787,1.78265241845381,
9.90941792477365));
#43400=CARTESIAN_POINT('Ctrl Pts',(0.0557575591850463,1.78258477980611,
9.90939394673067));
#43401=CARTESIAN_POINT('Ctrl Pts',(0.0545391516424456,1.7823722708823,9.90931775798246));
#43402=CARTESIAN_POINT('Ctrl Pts',(0.053703990584452,1.78222999710527,9.90926546484314));
#43403=CARTESIAN_POINT('Ctrl Pts',(0.0482173738705924,1.78131757238235,
9.90892145735028));
#43404=CARTESIAN_POINT('Ctrl Pts',(0.0435502627541095,1.78064631577146,
9.9086266223099));
#43405=CARTESIAN_POINT('Ctrl Pts',(0.029503215702636,1.77893961102169,9.90773201748767));
#43406=CARTESIAN_POINT('Ctrl Pts',(0.0200915086086435,1.77821355551467,
9.90712286250005));
#43407=CARTESIAN_POINT('Ctrl Pts',(-0.00320482895261495,1.77744239212582,
9.90559179177143));
#43408=CARTESIAN_POINT('Ctrl Pts',(-0.0170859994902055,1.77787937975245,
9.90465868507315));
#43409=CARTESIAN_POINT('Ctrl Pts',(-0.0528572907629566,1.78132444348676,
9.90222793680644));
#43410=CARTESIAN_POINT('Ctrl Pts',(-0.0745469458705863,1.78568969554585,
9.90072617269828));
#43411=CARTESIAN_POINT('Ctrl Pts',(-0.0968715275370533,1.79262596959161,
9.89925019946796));
#43412=CARTESIAN_POINT('Ctrl Pts',(-0.098118613909208,1.7930217838997,9.89916800148322));
#43413=CARTESIAN_POINT('Ctrl Pts',(-0.0997480071222414,1.79354988291193,
9.89906096753402));
#43414=CARTESIAN_POINT('Ctrl Pts',(-0.100132501498861,1.79367530080649,
9.89903573683006));
#43415=CARTESIAN_POINT('Ctrl Pts',(-0.100725279075145,1.79386989376178,
9.89899688053894));
#43416=CARTESIAN_POINT('Ctrl Pts',(-0.100933727654732,1.79393855778194,
9.89898322486533));
#43417=CARTESIAN_POINT('Ctrl Pts',(-0.101349215904362,1.79407589235037,
9.89895602207031));
#43418=CARTESIAN_POINT('Ctrl Pts',(-0.101556254570495,1.79414455969573,
9.89894247495338));
#43419=CARTESIAN_POINT('Ctrl Pts',(-0.102020208771163,1.79429895979606,
9.89891213515838));
#43420=CARTESIAN_POINT('Ctrl Pts',(-0.102277085407242,1.79438480603646,
9.89889534934122));
#43421=CARTESIAN_POINT('Ctrl Pts',(-0.102809300702446,1.79456341455317,
9.89886059632654));
#43422=CARTESIAN_POINT('Ctrl Pts',(-0.103084622906925,1.79465622560456,
9.8988426320253));
#43423=CARTESIAN_POINT('Ctrl Pts',(-0.104626507929913,1.79517831782669,
9.89874210264318));
#43424=CARTESIAN_POINT('Ctrl Pts',(-0.105890539280028,1.79561511548371,
9.89865997643893));
#43425=CARTESIAN_POINT('Ctrl Pts',(-0.109220987549227,1.79678923998765,
9.89844426130085));
#43426=CARTESIAN_POINT('Ctrl Pts',(-0.111282694445221,1.79753983467174,
9.89831140718745));
#43427=CARTESIAN_POINT('Ctrl Pts',(-0.120509233626228,1.80100600837233,
9.89771926082861));
#43428=CARTESIAN_POINT('Ctrl Pts',(-0.127584026453293,1.8039557181631,9.89727173367249));
#43429=CARTESIAN_POINT('Ctrl Pts',(-0.142415278774063,1.81076992881478,
9.89633416192085));
#43430=CARTESIAN_POINT('Ctrl Pts',(-0.150134572369021,1.81470056383909,
9.89584650502563));
#43431=CARTESIAN_POINT('Ctrl Pts',(-0.165343665065552,1.82323342688669,
9.89486932217386));
#43432=CARTESIAN_POINT('Ctrl Pts',(-0.172822088431143,1.82784050751257,
9.89438026524213));
#43433=CARTESIAN_POINT('Ctrl Pts',(-0.189464822290432,1.8390561320578,9.89325437129716));
#43434=CARTESIAN_POINT('Ctrl Pts',(-0.198488147396845,1.84585230217753,
9.89261587677547));
#43435=CARTESIAN_POINT('Ctrl Pts',(-0.209774029586698,1.85532084110524,
9.89176288373902));
#43436=CARTESIAN_POINT('Ctrl Pts',(-0.212376465921326,1.85757625966877,
9.89156217395371));
#43437=CARTESIAN_POINT('Ctrl Pts',(-0.220680320827547,1.86500919335534,
9.89090769484742));
#43438=CARTESIAN_POINT('Ctrl Pts',(-0.226232090747193,1.87034915733732,
9.89044802174623));
#43439=CARTESIAN_POINT('Ctrl Pts',(-0.232265822520867,1.87658398398682,
9.88992016073117));
#43440=CARTESIAN_POINT('Ctrl Pts',(-0.232941473464575,1.87728853098725,
9.88986063461622));
#43441=CARTESIAN_POINT('Ctrl Pts',(-0.233958021673845,1.87835824116803,
9.88977043670227));
#43442=CARTESIAN_POINT('Ctrl Pts',(-0.234301292147323,1.87872114954807,
9.88973986738567));
#43443=CARTESIAN_POINT('Ctrl Pts',(-0.234896251734726,1.87935308235259,
9.88968669018425));
#43444=CARTESIAN_POINT('Ctrl Pts',(-0.235148326565042,1.8796217436811,9.88966409892309));
#43445=CARTESIAN_POINT('Ctrl Pts',(-0.235672592724414,1.88018243011378,
9.88961698600386));
#43446=CARTESIAN_POINT('Ctrl Pts',(-0.235944703100051,1.88047452979455,
9.8895924609364));
#43447=CARTESIAN_POINT('Ctrl Pts',(-0.236483887368894,1.88105548327224,
9.88954372109935));
#43448=CARTESIAN_POINT('Ctrl Pts',(-0.236750976490736,1.88134432200661,
9.88951950704539));
#43449=CARTESIAN_POINT('Ctrl Pts',(-0.237372284102953,1.88201869696176,
9.88946301503901));
#43450=CARTESIAN_POINT('Ctrl Pts',(-0.237726092559501,1.8824046079401,9.88943071972559));
#43451=CARTESIAN_POINT('Ctrl Pts',(-0.238644874247811,1.88341167010896,
9.88934652547109));
#43452=CARTESIAN_POINT('Ctrl Pts',(-0.239208360415563,1.88403416720314,
9.8892945637996));
#43453=CARTESIAN_POINT('Ctrl Pts',(-0.24378790951703,1.88913321946703,9.88886958074356));
#43454=CARTESIAN_POINT('Ctrl Pts',(-0.247680147097211,1.89371892759231,
9.8884914187218));
#43455=CARTESIAN_POINT('Ctrl Pts',(-0.258288162271286,1.90695026083382,
9.88741045229816));
#43456=CARTESIAN_POINT('Ctrl Pts',(-0.264694543023223,1.91583232275206,
9.88669621031294));
#43457=CARTESIAN_POINT('Ctrl Pts',(-0.272807188855462,1.92838006764074,
9.88570425678538));
#43458=CARTESIAN_POINT('Ctrl Pts',(-0.274915416618389,1.93177789754889,
9.88543730002398));
#43459=CARTESIAN_POINT('Ctrl Pts',(-0.27920181128111,1.93898214507799,9.88487518992631));
#43460=CARTESIAN_POINT('Ctrl Pts',(-0.281366618228485,1.94279559185344,
9.88457985994763));
#43461=CARTESIAN_POINT('Ctrl Pts',(-0.294976223507685,1.96795197570047,
9.88264855050122));
#43462=CARTESIAN_POINT('Ctrl Pts',(-0.304062964015647,1.99048478518868,
9.88099028826353));
#43463=CARTESIAN_POINT('Ctrl Pts',(-0.31088806913972,2.01507956364011,9.879378855255));
#43464=CARTESIAN_POINT('Ctrl Pts',(-0.311228740860092,2.01633672822256,
9.8792970300292));
#43465=CARTESIAN_POINT('Ctrl Pts',(-0.311665015206745,2.01798623954543,
9.87919041012149));
#43466=CARTESIAN_POINT('Ctrl Pts',(-0.311767509279796,2.01837672654547,
9.87916522443983));
#43467=CARTESIAN_POINT('Ctrl Pts',(-0.311924551957967,2.01897964692479,
9.87912642212161));
#43468=CARTESIAN_POINT('Ctrl Pts',(-0.311979617453781,2.01919194334296,
9.87911277553228));
#43469=CARTESIAN_POINT('Ctrl Pts',(-0.31208902156242,2.01961551248133,9.87908558075673));
#43470=CARTESIAN_POINT('Ctrl Pts',(-0.312143362001146,2.01982678269834,
9.8790720325945));
#43471=CARTESIAN_POINT('Ctrl Pts',(-0.312264752969119,2.02030073291758,
9.87904167570545));
#43472=CARTESIAN_POINT('Ctrl Pts',(-0.312331686422183,2.02056344180222,
9.87902487387452));
#43473=CARTESIAN_POINT('Ctrl Pts',(-0.312469755638817,2.02110822563968,
9.87899008260698));
#43474=CARTESIAN_POINT('Ctrl Pts',(-0.312540841170675,2.02139031323937,
9.8789720960847));
#43475=CARTESIAN_POINT('Ctrl Pts',(-0.312725024878638,2.02212540566602,
9.87892529776407));
#43476=CARTESIAN_POINT('Ctrl Pts',(-0.312837521218514,2.02257856270861,
9.87889652029228));
#43477=CARTESIAN_POINT('Ctrl Pts',(-0.313166919160517,2.02391788193043,
9.87881167569745));
#43478=CARTESIAN_POINT('Ctrl Pts',(-0.313381045314108,2.02480473133156,
9.87875576342964));
#43479=CARTESIAN_POINT('Ctrl Pts',(-0.319337393109999,2.04994161834231,
9.87717827828858));
#43480=CARTESIAN_POINT('Ctrl Pts',(-0.32225212581812,2.07477878869423,9.87580752190471));
#43481=CARTESIAN_POINT('Ctrl Pts',(-0.322274865898728,2.09970600177385,
9.87441282464039));
#43482=CARTESIAN_POINT('',(-0.322274934653358,2.10025575292171,9.62425292903915));
#43483=CARTESIAN_POINT('Ctrl Pts',(-0.322274865987935,2.09970609957732,
9.87441281916821));
#43484=CARTESIAN_POINT('Ctrl Pts',(-0.322297305845905,2.12431240042638,
9.87303607716149));
#43485=CARTESIAN_POINT('Ctrl Pts',(-0.319501846540933,2.14883719023601,
9.87164199941798));
#43486=CARTESIAN_POINT('Ctrl Pts',(-0.313754231368156,2.17362174744587,
9.87009562371563));
#43487=CARTESIAN_POINT('Ctrl Pts',(-0.313561525540082,2.17443822323641,
9.87004453368211));
#43488=CARTESIAN_POINT('Ctrl Pts',(-0.313243454059054,2.17576270781824,
9.86996141168674));
#43489=CARTESIAN_POINT('Ctrl Pts',(-0.313120034411434,2.17627118362734,
9.86992944227753));
#43490=CARTESIAN_POINT('Ctrl Pts',(-0.312878946613936,2.17725399166109,
9.86986753602526));
#43491=CARTESIAN_POINT('Ctrl Pts',(-0.312761436680213,2.17772836151223,
9.86983760434906));
#43492=CARTESIAN_POINT('Ctrl Pts',(-0.31255681030874,2.17854643004297,9.86978589644286));
#43493=CARTESIAN_POINT('Ctrl Pts',(-0.312470204590151,2.1788902565887,9.86976413674167));
#43494=CARTESIAN_POINT('Ctrl Pts',(-0.312290031664546,2.17960059569219,
9.86971912476365));
#43495=CARTESIAN_POINT('Ctrl Pts',(-0.312196386258506,2.17996708771004,
9.86969586998628));
#43496=CARTESIAN_POINT('Ctrl Pts',(-0.311968290064461,2.1808532606959,9.86963956403524));
#43497=CARTESIAN_POINT('Ctrl Pts',(-0.311833186037185,2.1813727709448,9.86960649175923));
#43498=CARTESIAN_POINT('Ctrl Pts',(-0.311327472885493,2.18329761441702,
9.8694837181674));
#43499=CARTESIAN_POINT('Ctrl Pts',(-0.310948660734578,2.18470075688653,
9.8693937513264));
#43500=CARTESIAN_POINT('Ctrl Pts',(-0.304231966502203,2.20892733406003,
9.86783211893535));
#43501=CARTESIAN_POINT('Ctrl Pts',(-0.295407752386047,2.23098121234592,
9.86627500938244));
#43502=CARTESIAN_POINT('Ctrl Pts',(-0.281907377722443,2.25625018624662,
9.86434362167931));
#43503=CARTESIAN_POINT('Ctrl Pts',(-0.279463590524266,2.26058016997776,
9.86400734931183));
#43504=CARTESIAN_POINT('Ctrl Pts',(-0.274526895559133,2.2688729054334,9.8633542530397));
#43505=CARTESIAN_POINT('Ctrl Pts',(-0.272045833207488,2.27284137153076,
9.86303752074926));
#43506=CARTESIAN_POINT('Ctrl Pts',(-0.26305180116042,2.28655364383423,9.86193078240501));
#43507=CARTESIAN_POINT('Ctrl Pts',(-0.256094118617026,2.2959958126746,9.86114603027968));
#43508=CARTESIAN_POINT('Ctrl Pts',(-0.245460969945522,2.30888994205179,
9.86006169507488));
#43509=CARTESIAN_POINT('Ctrl Pts',(-0.242195669241725,2.31266725250173,
9.8597424072951));
#43510=CARTESIAN_POINT('Ctrl Pts',(-0.238531092191241,2.31671250655774,
9.85940008782886));
#43511=CARTESIAN_POINT('Ctrl Pts',(-0.238217726939383,2.31705692114904,
9.85937093955482));
#43512=CARTESIAN_POINT('Ctrl Pts',(-0.237707734013839,2.31761501127303,
9.85932370444822));
#43513=CARTESIAN_POINT('Ctrl Pts',(-0.237511563464139,2.31782910081931,
9.85930558377508));
#43514=CARTESIAN_POINT('Ctrl Pts',(-0.237131942192299,2.3182422757059,9.85927061143396));
#43515=CARTESIAN_POINT('Ctrl Pts',(-0.236948529544064,2.31844139548487,
9.85925375691608));
#43516=CARTESIAN_POINT('Ctrl Pts',(-0.236616886121135,2.31880053108729,
9.85922335745016));
#43517=CARTESIAN_POINT('Ctrl Pts',(-0.236468744204284,2.31896062709332,
9.85920980581612));
#43518=CARTESIAN_POINT('Ctrl Pts',(-0.236171173121815,2.31928155601092,
9.85918263998217));
#43519=CARTESIAN_POINT('Ctrl Pts',(-0.236021742819249,2.3194423859184,9.859169025997));
#43520=CARTESIAN_POINT('Ctrl Pts',(-0.235596331700964,2.31989931321491,
9.85913034704425));
#43521=CARTESIAN_POINT('Ctrl Pts',(-0.23531995597679,2.32019504487311,9.85910531234822));
#43522=CARTESIAN_POINT('Ctrl Pts',(-0.234145974951239,2.32144651081927,
9.85899936329186));
#43523=CARTESIAN_POINT('Ctrl Pts',(-0.233243082558528,2.32239730060512,
9.85891884917301));
#43524=CARTESIAN_POINT('Ctrl Pts',(-0.216653209305993,2.33965508587502,
9.85745647204684));
#43525=CARTESIAN_POINT('Ctrl Pts',(-0.199294803930529,2.35427367903028,
9.85619933181208));
#43526=CARTESIAN_POINT('Ctrl Pts',(-0.172947693847635,2.37209262161914,
9.85442150969516));
#43527=CARTESIAN_POINT('Ctrl Pts',(-0.16513445194697,2.3769041462864,9.85390879256252));
#43528=CARTESIAN_POINT('Ctrl Pts',(-0.146695956796233,2.38720063285064,
9.85271304547522));
#43529=CARTESIAN_POINT('Ctrl Pts',(-0.135950164127302,2.3924404561668,9.85202616048031));
#43530=CARTESIAN_POINT('Ctrl Pts',(-0.121149094371218,2.39866532500085,
9.85107616240516));
#43531=CARTESIAN_POINT('Ctrl Pts',(-0.117329187001707,2.40018650708016,
9.85083070045081));
#43532=CARTESIAN_POINT('Ctrl Pts',(-0.111128590942264,2.40251930660861,
9.850431246539));
#43533=CARTESIAN_POINT('Ctrl Pts',(-0.108765611497405,2.40337688738464,
9.85027878759168));
#43534=CARTESIAN_POINT('Ctrl Pts',(-0.105895087750046,2.40438082090678,
9.85009322709453));
#43535=CARTESIAN_POINT('Ctrl Pts',(-0.10539685915934,2.40455369940232,9.85006100707462));
#43536=CARTESIAN_POINT('Ctrl Pts',(-0.104433292487991,2.40488539618656,
9.84999866830571));
#43537=CARTESIAN_POINT('Ctrl Pts',(-0.103968010586591,2.40504437408048,
9.84996855493053));
#43538=CARTESIAN_POINT('Ctrl Pts',(-0.103166196521292,2.405316290966,9.84991664037546));
#43539=CARTESIAN_POINT('Ctrl Pts',(-0.102829837268975,2.40542974020141,
9.84989485610887));
#43540=CARTESIAN_POINT('Ctrl Pts',(-0.102135802974879,2.40566255177041,
9.84984989393903));
#43541=CARTESIAN_POINT('Ctrl Pts',(-0.101778104623577,2.40578184253071,
9.84982671370945));
#43542=CARTESIAN_POINT('Ctrl Pts',(-0.100914867664108,2.40606804560246,
9.84977075493809));
#43543=CARTESIAN_POINT('Ctrl Pts',(-0.100409124472092,2.4062343331044,9.84973795584884));
#43544=CARTESIAN_POINT('Ctrl Pts',(-0.098547393548133,2.40684135934776,
9.84961716120124));
#43545=CARTESIAN_POINT('Ctrl Pts',(-0.0971889126785451,2.4072743460314,
9.84952891097501));
#43546=CARTESIAN_POINT('Ctrl Pts',(-0.0746653382698697,2.41428894622515,
9.84806381705592));
#43547=CARTESIAN_POINT('Ctrl Pts',(-0.0528840396137501,2.41867753686474,
9.84661282817544));
#43548=CARTESIAN_POINT('Ctrl Pts',(-0.0136957691263339,2.42244357503113,
9.8439652832459));
#43549=CARTESIAN_POINT('Ctrl Pts',(0.00354165867539437,2.42271488028246,
9.84279015883714));
#43550=CARTESIAN_POINT('Ctrl Pts',(0.0305861848955652,2.4209726468715,9.84098619256883));
#43551=CARTESIAN_POINT('Ctrl Pts',(0.0404207035808147,2.41988304722363,
9.84033903892978));
#43552=CARTESIAN_POINT('Ctrl Pts',(0.0514736619476156,2.41814041739219,
9.83963276640123));
#43553=CARTESIAN_POINT('Ctrl Pts',(0.0527556133379823,2.41793035157104,
9.83955117641875));
#43554=CARTESIAN_POINT('Ctrl Pts',(0.0543201203553452,2.41766426151279,
9.83945203012769));
#43555=CARTESIAN_POINT('Ctrl Pts',(0.0546038921248988,2.4176156064872,9.83943406406591));
#43556=CARTESIAN_POINT('Ctrl Pts',(0.0551526201268768,2.41752076538734,
9.83939935693965));
#43557=CARTESIAN_POINT('Ctrl Pts',(0.0554175843488946,2.41747462781335,
9.83938261314604));
#43558=CARTESIAN_POINT('Ctrl Pts',(0.0558765676366583,2.41739411405798,
9.83935363553895));
#43559=CARTESIAN_POINT('Ctrl Pts',(0.056070612556328,2.4173598916968,9.8393413929505));
#43560=CARTESIAN_POINT('Ctrl Pts',(0.0564762599574232,2.4172879668102,9.83931581747479));
#43561=CARTESIAN_POINT('Ctrl Pts',(0.056687855455908,2.41725023067884,9.83930248657712));
#43562=CARTESIAN_POINT('Ctrl Pts',(0.0572753631028552,2.41714484749377,
9.83926549960808));
#43563=CARTESIAN_POINT('Ctrl Pts',(0.0576511945525295,2.41707674351907,
9.8392418696566));
#43564=CARTESIAN_POINT('Ctrl Pts',(0.0591417272083596,2.41680390811209,
9.83914827321261));
#43565=CARTESIAN_POINT('Ctrl Pts',(0.0602554833517576,2.4165939622104,9.83907860025547));
#43566=CARTESIAN_POINT('Ctrl Pts',(0.0798942418021805,2.41278461609167,
9.83785436160617));
#43567=CARTESIAN_POINT('Ctrl Pts',(0.0980720670802945,2.40757015995193,
9.83678772290392));
#43568=CARTESIAN_POINT('Ctrl Pts',(0.127938775151546,2.39608282335079,9.83499494080691));
#43569=CARTESIAN_POINT('Ctrl Pts',(0.13988712130818,2.39062855134709,9.8342659770238));
#43570=CARTESIAN_POINT('Ctrl Pts',(0.162598744044753,2.3785351045183,9.83280917768137));
#43571=CARTESIAN_POINT('Ctrl Pts',(0.173369665320538,2.37196151943526,9.83208367517406));
#43572=CARTESIAN_POINT('Ctrl Pts',(0.188351024389268,2.36156594038538,9.83100171622776));
#43573=CARTESIAN_POINT('Ctrl Pts',(0.192889763408983,2.35823706697396,9.83066358574443));
#43574=CARTESIAN_POINT('Ctrl Pts',(0.198061036653866,2.35423185455756,9.83026514598197));
#43575=CARTESIAN_POINT('Ctrl Pts',(0.198780866103344,2.35366942534805,9.83020937977084));
#43576=CARTESIAN_POINT('Ctrl Pts',(0.199804897234676,2.35286227690106,9.83012960699683));
#43577=CARTESIAN_POINT('Ctrl Pts',(0.200111065197759,2.35262004992052,9.83010569984734));
#43578=CARTESIAN_POINT('Ctrl Pts',(0.200728123989581,2.35213003374753,9.83005740228364));
#43579=CARTESIAN_POINT('Ctrl Pts',(0.201038997914169,2.35188222444881,9.83003301108998));
#43580=CARTESIAN_POINT('Ctrl Pts',(0.201638942873929,2.35140216753829,9.82998582495835));
#43581=CARTESIAN_POINT('Ctrl Pts',(0.201928073334578,2.35116999487173,9.82996303305393));
#43582=CARTESIAN_POINT('Ctrl Pts',(0.202613050362183,2.35061800897674,9.82990891401737));
#43583=CARTESIAN_POINT('Ctrl Pts',(0.203008540493409,2.35029775684678,9.82987756921893));
#43584=CARTESIAN_POINT('Ctrl Pts',(0.204398126183931,2.34916706579596,9.82976709084794));
#43585=CARTESIAN_POINT('Ctrl Pts',(0.20538813062054,2.34835163858689,9.82968775548488));
#43586=CARTESIAN_POINT('Ctrl Pts',(0.220184281651923,2.33601565760847,9.82849252063869));
#43587=CARTESIAN_POINT('Ctrl Pts',(0.233004963278584,2.32336740463764,9.82732882929094));
#43588=CARTESIAN_POINT('Ctrl Pts',(0.256627144583543,2.29580466365642,9.82491131665182));
#43589=CARTESIAN_POINT('Ctrl Pts',(0.267342925314749,2.28089959298636,9.82366061887386));
#43590=CARTESIAN_POINT('Ctrl Pts',(0.280263660576456,2.25925107628006,9.8219671747482));
#43591=CARTESIAN_POINT('Ctrl Pts',(0.283603572256919,2.25322417628279,9.82150802947032));
#43592=CARTESIAN_POINT('Ctrl Pts',(0.289488578222333,2.24175187647036,9.82066226873715));
#43593=CARTESIAN_POINT('Ctrl Pts',(0.292079610990846,2.23633320594882,9.82027407308481));
#43594=CARTESIAN_POINT('Ctrl Pts',(0.295128831444165,2.22946973712254,9.81979908925867));
#43595=CARTESIAN_POINT('Ctrl Pts',(0.295730152220973,2.22809026995562,9.81970445331327));
#43596=CARTESIAN_POINT('Ctrl Pts',(0.296486919263441,2.22632046036078,9.81958414378047));
#43597=CARTESIAN_POINT('Ctrl Pts',(0.296651282214774,2.22593398574326,9.81955793879455));
#43598=CARTESIAN_POINT('Ctrl Pts',(0.296911222348168,2.22531944309033,9.81951637741319));
#43599=CARTESIAN_POINT('Ctrl Pts',(0.297007292593845,2.22509158612718,9.81950099100123));
#43600=CARTESIAN_POINT('Ctrl Pts',(0.297187857639902,2.22466194588452,9.81947202343226));
#43601=CARTESIAN_POINT('Ctrl Pts',(0.297272408554982,2.22446018878566,9.81945843893898));
#43602=CARTESIAN_POINT('Ctrl Pts',(0.297463994149048,2.22400171437883,9.81942761135309));
#43603=CARTESIAN_POINT('Ctrl Pts',(0.297570901761335,2.22374494498902,9.81941037610029));
#43604=CARTESIAN_POINT('Ctrl Pts',(0.297893773244277,2.22296663826904,9.81935822271649));
#43605=CARTESIAN_POINT('Ctrl Pts',(0.298108700852122,2.22244466812636,9.81932336743259));
#43606=CARTESIAN_POINT('Ctrl Pts',(0.29960031731831,2.21879494196711,9.81908048013223));
#43607=CARTESIAN_POINT('Ctrl Pts',(0.300829187814022,2.21564769917812,9.81887527519133));
#43608=CARTESIAN_POINT('Ctrl Pts',(0.30239082270291,2.21145477342877,9.8186067395954));
#43609=CARTESIAN_POINT('Ctrl Pts',(0.302768012732389,2.21042602368287,9.81854123625238));
#43610=CARTESIAN_POINT('Ctrl Pts',(0.306011596891683,2.2014378912329,9.81797210545464));
#43611=CARTESIAN_POINT('Ctrl Pts',(0.308569024512462,2.1933698134325,9.81748281031494));
#43612=CARTESIAN_POINT('Ctrl Pts',(0.315262583000933,2.16895481292754,9.81604063135334));
#43613=CARTESIAN_POINT('Ctrl Pts',(0.318437097088449,2.15237476589654,9.81511055965198));
#43614=CARTESIAN_POINT('Ctrl Pts',(0.321787789347033,2.12224657356128,9.81340581455307));
#43615=CARTESIAN_POINT('Ctrl Pts',(0.322435947403746,2.10879221106583,9.81263954639161));
#43616=CARTESIAN_POINT('Ctrl Pts',(0.322133748893646,2.08790630496455,9.81141197503266));
#43617=CARTESIAN_POINT('Ctrl Pts',(0.321769214110453,2.08048156844214,9.81096826794861));
#43618=CARTESIAN_POINT('Ctrl Pts',(0.321053213688853,2.07194099058388,9.81044709169071));
#43619=CARTESIAN_POINT('Ctrl Pts',(0.320951999024646,2.07080602289462,9.81037761328371));
#43620=CARTESIAN_POINT('Ctrl Pts',(0.320794868993983,2.06914373957591,9.81027552622825));
#43621=CARTESIAN_POINT('Ctrl Pts',(0.320743667074442,2.06861597848335,9.81024306589319));
#43622=CARTESIAN_POINT('Ctrl Pts',(0.320651843407382,2.06769321086289,9.8101862245961));
#43623=CARTESIAN_POINT('Ctrl Pts',(0.320611793523599,2.06729814751118,9.81016186168329));
#43624=CARTESIAN_POINT('Ctrl Pts',(0.320532852972805,2.06653354119646,9.81011465599012));
#43625=CARTESIAN_POINT('Ctrl Pts',(0.320494053107751,2.06616398929387,9.81009181610536));
#43626=CARTESIAN_POINT('Ctrl Pts',(0.320400287332385,2.06528554339751,9.81003746628292));
#43627=CARTESIAN_POINT('Ctrl Pts',(0.320344748127649,2.06477671278701,9.8100059383226));
#43628=CARTESIAN_POINT('Ctrl Pts',(0.320143858098891,2.06297601035928,9.8098941982516));
#43629=CARTESIAN_POINT('Ctrl Pts',(0.319991904291529,2.06168490120324,9.80981377823887));
#43630=CARTESIAN_POINT('Ctrl Pts',(0.317213236251432,2.03924576441126,9.80841074147783));
#43631=CARTESIAN_POINT('Ctrl Pts',(0.312503683243919,2.01841299505657,9.80701984634121));
#43632=CARTESIAN_POINT('Ctrl Pts',(0.296868475033331,1.97144949488446,9.80369754655943));
#43633=CARTESIAN_POINT('Ctrl Pts',(0.284490267505094,1.94598192489157,9.80174706064239));
#43634=CARTESIAN_POINT('Ctrl Pts',(0.268255980660065,1.92139004441731,9.79988758999824));
#43635=CARTESIAN_POINT('Ctrl Pts',(0.267550278724164,1.92033465588822,9.79980786236898));
#43636=CARTESIAN_POINT('Ctrl Pts',(0.266620717420602,1.91896210538215,9.79970430083597));
#43637=CARTESIAN_POINT('Ctrl Pts',(0.266402508452238,1.9186411575366,9.79968009373914));
#43638=CARTESIAN_POINT('Ctrl Pts',(0.26604833992763,1.91812225502829,9.79964097181865));
#43639=CARTESIAN_POINT('Ctrl Pts',(0.265912738776006,1.91792405800933,9.79962603274411));
#43640=CARTESIAN_POINT('Ctrl Pts',(0.265652230018293,1.91754420559659,9.79959740882915));
#43641=CARTESIAN_POINT('Ctrl Pts',(0.265527357951223,1.91736252738076,9.79958372169801));
#43642=CARTESIAN_POINT('Ctrl Pts',(0.265239734521849,1.91694497827603,9.79955227202741));
#43643=CARTESIAN_POINT('Ctrl Pts',(0.26507685442797,1.91670919555067,9.79953451830532));
#43644=CARTESIAN_POINT('Ctrl Pts',(0.264571375157276,1.915979554558,9.79947959412768));
#43645=CARTESIAN_POINT('Ctrl Pts',(0.264227706227595,1.91548643364585,9.79944249627908));
#43646=CARTESIAN_POINT('Ctrl Pts',(0.261376327266272,1.91141937331919,9.79913668576985));
#43647=CARTESIAN_POINT('Ctrl Pts',(0.258797459936304,1.90789555829201,9.798872729477));
#43648=CARTESIAN_POINT('Ctrl Pts',(0.255529827265504,1.90361588813574,9.79855193963046));
#43649=CARTESIAN_POINT('Ctrl Pts',(0.254908188881738,1.90280966731294,9.79849149841036));
#43650=CARTESIAN_POINT('Ctrl Pts',(0.253633684977315,1.90117282485844,9.79836873641439));
#43651=CARTESIAN_POINT('Ctrl Pts',(0.252980534255685,1.90034244049195,9.7983064315288));
#43652=CARTESIAN_POINT('Ctrl Pts',(0.252068397777214,1.89919445633103,9.79822023632875));
#43653=CARTESIAN_POINT('Ctrl Pts',(0.251812878213565,1.8988741242535,9.7981961779597));
#43654=CARTESIAN_POINT('Ctrl Pts',(0.248949098441692,1.8952979593143,9.7979275075971));
#43655=CARTESIAN_POINT('Ctrl Pts',(0.246278371066991,1.89209245915756,9.79768589830229));
#43656=CARTESIAN_POINT('Ctrl Pts',(0.226995911383314,1.86984211116259,9.79599605017308));
#43657=CARTESIAN_POINT('Ctrl Pts',(0.208256714985489,1.85275707254662,9.79462396134834));
#43658=CARTESIAN_POINT('Ctrl Pts',(0.177201069282904,1.83050381469792,9.79243793321324));
#43659=CARTESIAN_POINT('Ctrl Pts',(0.166246492520114,1.82361176460769,9.79168210148426));
#43660=CARTESIAN_POINT('Ctrl Pts',(0.153631087115734,1.81669665282146,9.79081306423907));
#43661=CARTESIAN_POINT('Ctrl Pts',(0.152349034829988,1.81600516038142,9.79072477163155));
#43662=CARTESIAN_POINT('Ctrl Pts',(0.150085494271084,1.81480402703968,9.79056890617822));
#43663=CARTESIAN_POINT('Ctrl Pts',(0.14910598185343,1.81429069894181,9.79050146450662));
#43664=CARTESIAN_POINT('Ctrl Pts',(0.147659742344713,1.81354223835232,9.79040189028089));
#43665=CARTESIAN_POINT('Ctrl Pts',(0.147195047098176,1.81330317960921,9.79036989622024));
#43666=CARTESIAN_POINT('Ctrl Pts',(0.146377303071823,1.81288500997988,9.79031359479054));
#43667=CARTESIAN_POINT('Ctrl Pts',(0.146024500974872,1.81270541692957,9.79028930443455));
#43668=CARTESIAN_POINT('Ctrl Pts',(0.145337939969498,1.81235751608429,9.79024203438235));
#43669=CARTESIAN_POINT('Ctrl Pts',(0.145004217232303,1.81218913792076,9.79021905720225));
#43670=CARTESIAN_POINT('Ctrl Pts',(0.144113030328574,1.81174143741682,9.79015769700574));
#43671=CARTESIAN_POINT('Ctrl Pts',(0.143555049261279,1.81146315272417,9.79011927773544));
#43672=CARTESIAN_POINT('Ctrl Pts',(0.141548432629224,1.81046964418382,9.78998110774663));
#43673=CARTESIAN_POINT('Ctrl Pts',(0.140095249812797,1.80976370567053,9.7898810338229));
#43674=CARTESIAN_POINT('Ctrl Pts',(0.136621955895356,1.80810858450049,9.78964179041358));
#43675=CARTESIAN_POINT('Ctrl Pts',(0.134597192394109,1.80716941302022,9.78950227967538));
#43676=CARTESIAN_POINT('Ctrl Pts',(0.131862739252417,1.80593540906021,9.78931378259872));
#43677=CARTESIAN_POINT('Ctrl Pts',(0.131161478861849,1.80562195718072,9.789265434269));
#43678=CARTESIAN_POINT('Ctrl Pts',(0.129710176596205,1.80497946420575,9.7891653573722));
#43679=CARTESIAN_POINT('Ctrl Pts',(0.128959988174738,1.80465076962471,9.78911361757299));
#43680=CARTESIAN_POINT('Ctrl Pts',(0.0979021320076369,1.79118367829456,
9.78697117288976));
#43681=CARTESIAN_POINT('Ctrl Pts',(0.0657592857931973,1.78278227175213,
9.78470741414048));
#43682=CARTESIAN_POINT('Ctrl Pts',(0.0211334842549709,1.77820069796031,
9.78170098806605));
#43683=CARTESIAN_POINT('Ctrl Pts',(0.00929398069462249,1.77764134582955,
9.78091941939964));
#43684=CARTESIAN_POINT('Ctrl Pts',(-0.00414735685355448,1.77774773135416,
9.78006876629563));
#43685=CARTESIAN_POINT('Ctrl Pts',(-0.00574397429082147,1.77777223548279,
9.77996831396354));
#43686=CARTESIAN_POINT('Ctrl Pts',(-0.00775684790823911,1.77781809413138,
9.77984247446533));
#43687=CARTESIAN_POINT('Ctrl Pts',(-0.00817329750369071,1.777828389874,
9.77981648243746));
#43688=CARTESIAN_POINT('Ctrl Pts',(-0.00883616280807769,1.7778460637758,
9.77977518094625));
#43689=CARTESIAN_POINT('Ctrl Pts',(-0.00908259024036353,1.77785291720485,
9.77975984210432));
#43690=CARTESIAN_POINT('Ctrl Pts',(-0.00954780777627352,1.77786638967031,
9.77973091416207));
#43691=CARTESIAN_POINT('Ctrl Pts',(-0.00976659720525034,1.77787294879703,
9.77971732184053));
#43692=CARTESIAN_POINT('Ctrl Pts',(-0.010264619509705,1.77788838695266,
9.77968641004311));
#43693=CARTESIAN_POINT('Ctrl Pts',(-0.010543847128047,1.77789740615327,
9.77966909857274));
#43694=CARTESIAN_POINT('Ctrl Pts',(-0.0112668465988965,1.77792170057866,
9.77962432508355));
#43695=CARTESIAN_POINT('Ctrl Pts',(-0.0117106011090723,1.77793752994541,
9.77959689408986));
#43696=CARTESIAN_POINT('Ctrl Pts',(-0.014387501042807,1.7780385588006,9.7794317111711));
#43697=CARTESIAN_POINT('Ctrl Pts',(-0.0166198142580742,1.77814607002657,
9.77929518628514));
#43698=CARTESIAN_POINT('Ctrl Pts',(-0.0189881557188142,1.7782848395385,
9.77915147160512));
#43699=CARTESIAN_POINT('Ctrl Pts',(-0.0191254049468808,1.77829296959169,
9.77914314713557));
#43700=CARTESIAN_POINT('Ctrl Pts',(-0.0530559000650971,1.78032465637091,
9.77708617441784));
#43701=CARTESIAN_POINT('Ctrl Pts',(-0.0863249158435276,1.78766022651808,
9.7752929580443));
#43702=CARTESIAN_POINT('Ctrl Pts',(-0.13138131169467,1.80536190709868,9.77252575341611));
#43703=CARTESIAN_POINT('Ctrl Pts',(-0.144539335843734,1.81158892235489,
9.77167459192762));
#43704=CARTESIAN_POINT('Ctrl Pts',(-0.158283573633327,1.8192706995653,9.7707174952245));
#43705=CARTESIAN_POINT('Ctrl Pts',(-0.159332890610663,1.81986492595089,
9.7706439845545));
#43706=CARTESIAN_POINT('Ctrl Pts',(-0.160844171122918,1.82073199958781,
9.7705374634627));
#43707=CARTESIAN_POINT('Ctrl Pts',(-0.161308835825522,1.82100013814061,
9.77050462309901));
#43708=CARTESIAN_POINT('Ctrl Pts',(-0.162117156461919,1.8214692804964,9.77044733865349));
#43709=CARTESIAN_POINT('Ctrl Pts',(-0.162461114451169,1.82166976374192,
9.77042291347187));
#43710=CARTESIAN_POINT('Ctrl Pts',(-0.163123962618023,1.82205776625446,
9.77037574742084));
#43711=CARTESIAN_POINT('Ctrl Pts',(-0.163442903330892,1.82224519836975,
9.77035300974457));
#43712=CARTESIAN_POINT('Ctrl Pts',(-0.164196918533735,1.82269005944786,
9.77029915301651));
#43713=CARTESIAN_POINT('Ctrl Pts',(-0.164631710461629,1.82294796320757,
9.77026801670179));
#43714=CARTESIAN_POINT('Ctrl Pts',(-0.166150550320656,1.82385372510966,
9.77015896583892));
#43715=CARTESIAN_POINT('Ctrl Pts',(-0.167231384753808,1.82450692497236,
9.77008085630155));
#43716=CARTESIAN_POINT('Ctrl Pts',(-0.182106017075454,1.83361616473498,
9.76899879903645));
#43717=CARTESIAN_POINT('Ctrl Pts',(-0.195245558213547,1.84309150434982,
9.76795646474507));
#43718=CARTESIAN_POINT('Ctrl Pts',(-0.214244502983612,1.85909429095789,
9.76631072098358));
#43719=CARTESIAN_POINT('Ctrl Pts',(-0.2206441005582,1.86494163359599,9.76572923614095));
#43720=CARTESIAN_POINT('Ctrl Pts',(-0.238646699960941,1.88277435840428,
9.76401898430969));
#43721=CARTESIAN_POINT('Ctrl Pts',(-0.2495650155238,1.89541123703916,9.76288251820967));
#43722=CARTESIAN_POINT('Ctrl Pts',(-0.263119839030976,1.91380852466656,
9.7613722471434));
#43723=CARTESIAN_POINT('Ctrl Pts',(-0.2666396745088,1.91888509251695,9.76096928698511));
#43724=CARTESIAN_POINT('Ctrl Pts',(-0.271588654478606,1.9264801954585,9.76038973025778));
#43725=CARTESIAN_POINT('Ctrl Pts',(-0.273133105823263,1.92892157431099,
9.76020684904137));
#43726=CARTESIAN_POINT('Ctrl Pts',(-0.274906385955153,1.93180991419906,
9.75999475982114));
#43727=CARTESIAN_POINT('Ctrl Pts',(-0.275167194512037,1.93223694961925,
9.7599635112288));
#43728=CARTESIAN_POINT('Ctrl Pts',(-0.275564535202329,1.93289095561116,
9.75991582153778));
#43729=CARTESIAN_POINT('Ctrl Pts',(-0.275701782372438,1.93311748750783,
9.75989933364467));
#43730=CARTESIAN_POINT('Ctrl Pts',(-0.275940429603432,1.93351248216052,
9.75987063810736));
#43731=CARTESIAN_POINT('Ctrl Pts',(-0.276041954461068,1.93368086801554,
9.75985842223128));
#43732=CARTESIAN_POINT('Ctrl Pts',(-0.276255251691661,1.93403536922291,
9.75983274005259));
#43733=CARTESIAN_POINT('Ctrl Pts',(-0.276366989752446,1.93422150401203,
9.75981927603268));
#43734=CARTESIAN_POINT('Ctrl Pts',(-0.27668031325391,1.93474463975906,9.75978149279504));
#43735=CARTESIAN_POINT('Ctrl Pts',(-0.276881471829862,1.93508189792549,
9.75975720161944));
#43736=CARTESIAN_POINT('Ctrl Pts',(-0.277702491903747,1.93646413902228,
9.75965791607218));
#43737=CARTESIAN_POINT('Ctrl Pts',(-0.278317068317699,1.93751227299109,
9.75958326223036));
#43738=CARTESIAN_POINT('Ctrl Pts',(-0.288969533244621,1.95591736306462,
9.75828294139061));
#43739=CARTESIAN_POINT('Ctrl Pts',(-0.297373684356233,1.9741733270885,9.75715597044031));
#43740=CARTESIAN_POINT('Ctrl Pts',(-0.30940996989391,2.0084032019257,9.75512584973383));
#43741=CARTESIAN_POINT('Ctrl Pts',(-0.313628873807836,2.02409609566827,
9.75422387174479));
#43742=CARTESIAN_POINT('Ctrl Pts',(-0.318091344003069,2.04766202799877,
9.75284758579285));
#43743=CARTESIAN_POINT('Ctrl Pts',(-0.31925899291133,2.05533402496134,9.75239646562233));
#43744=CARTESIAN_POINT('Ctrl Pts',(-0.320844999060878,2.06907217242906,
9.75157762129026));
#43745=CARTESIAN_POINT('Ctrl Pts',(-0.321370705784315,2.07512217954957,
9.75121326509177));
#43746=CARTESIAN_POINT('Ctrl Pts',(-0.321779745936544,2.08211582770399,
9.75078656525539));
#43747=CARTESIAN_POINT('Ctrl Pts',(-0.321830240036878,2.08304874392122,
9.75072953358463));
#43748=CARTESIAN_POINT('Ctrl Pts',(-0.321900703160517,2.08446466577264,
9.75064279999281));
#43749=CARTESIAN_POINT('Ctrl Pts',(-0.321923643536548,2.084947524027,9.75061319129254));
#43750=CARTESIAN_POINT('Ctrl Pts',(-0.321963022232995,2.08581767970143,
9.75055977752707));
#43751=CARTESIAN_POINT('Ctrl Pts',(-0.321979848354056,2.08620495935959,
9.75053598466833));
#43752=CARTESIAN_POINT('Ctrl Pts',(-0.322014522698576,2.08703768771663,
9.75048478183374));
#43753=CARTESIAN_POINT('Ctrl Pts',(-0.322032145437325,2.08748314454919,
9.75045736483829));
#43754=CARTESIAN_POINT('Ctrl Pts',(-0.322077341531188,2.08868891949312,
9.75038307868663));
#43755=CARTESIAN_POINT('Ctrl Pts',(-0.322103146726464,2.08944929750828,
9.75033615420771));
#43756=CARTESIAN_POINT('Ctrl Pts',(-0.322206688439654,2.09285610738308,
9.75012555520162));
#43757=CARTESIAN_POINT('Ctrl Pts',(-0.322254502150832,2.09550328480943,
9.74996094611242));
#43758=CARTESIAN_POINT('Ctrl Pts',(-0.322273411130203,2.09879845286177,
9.74975478492523));
#43759=CARTESIAN_POINT('Ctrl Pts',(-0.322275175211994,2.0994462227569,9.74971419696014));
#43760=CARTESIAN_POINT('Ctrl Pts',(-0.322273302805116,2.10586638760011,
9.74931131846836));
#43761=CARTESIAN_POINT('Ctrl Pts',(-0.322116532944669,2.11163737770104,
9.74894430989695));
#43762=CARTESIAN_POINT('Ctrl Pts',(-0.321400676334139,2.12487623154211,
9.74809086439356));
#43763=CARTESIAN_POINT('Ctrl Pts',(-0.320736129714393,2.13233486589216,
9.74760156373966));
#43764=CARTESIAN_POINT('Ctrl Pts',(-0.316059594151767,2.16994792426403,
9.74509395513849));
#43765=CARTESIAN_POINT('Ctrl Pts',(-0.308052987212269,2.19944621280876,
9.74297782292642));
#43766=CARTESIAN_POINT('Ctrl Pts',(-0.294323019277409,2.23135378497443,
9.74073427392886));
#43767=CARTESIAN_POINT('Ctrl Pts',(-0.29253483335679,2.23528943906034,9.74045874355568));
#43768=CARTESIAN_POINT('Ctrl Pts',(-0.290431825866982,2.2396811688905,9.74015361694825));
#43769=CARTESIAN_POINT('Ctrl Pts',(-0.290194488546534,2.24017358255626,
9.74011943874484));
#43770=CARTESIAN_POINT('Ctrl Pts',(-0.289834215223509,2.24091621989981,
9.74006794595621));
#43771=CARTESIAN_POINT('Ctrl Pts',(-0.289712206985829,2.24116688871659,
9.74005057434575));
#43772=CARTESIAN_POINT('Ctrl Pts',(-0.289499843316978,2.24160176001176,
9.74002045369831));
#43773=CARTESIAN_POINT('Ctrl Pts',(-0.289409637228505,2.24178603456894,
9.74000769533899));
#43774=CARTESIAN_POINT('Ctrl Pts',(-0.2892206828405,2.24217110223605,9.73998104584695));
#43775=CARTESIAN_POINT('Ctrl Pts',(-0.28912190145218,2.24237187852504,9.7399671568904));
#43776=CARTESIAN_POINT('Ctrl Pts',(-0.288885262682978,2.24285159236075,
9.73993398660289));
#43777=CARTESIAN_POINT('Ctrl Pts',(-0.288747209818941,2.24313043442657,
9.73991471754587));
#43778=CARTESIAN_POINT('Ctrl Pts',(-0.288278395582984,2.24407391648643,
9.73984955767201));
#43779=CARTESIAN_POINT('Ctrl Pts',(-0.287945738362077,2.24473761970016,
9.73980378475377));
#43780=CARTESIAN_POINT('Ctrl Pts',(-0.287149164594124,2.24631329323574,
9.73969525668464));
#43781=CARTESIAN_POINT('Ctrl Pts',(-0.286683189442699,2.24722422171532,
9.7396326262312));
#43782=CARTESIAN_POINT('Ctrl Pts',(-0.28106100386613,2.25808704548987,9.73888691337876));
#43783=CARTESIAN_POINT('Ctrl Pts',(-0.275392728065583,2.26776681825872,
9.73823394896948));
#43784=CARTESIAN_POINT('Ctrl Pts',(-0.253634613879629,2.30083785970426,
9.73597506091713));
#43785=CARTESIAN_POINT('Ctrl Pts',(-0.234976438492165,2.32237926423071,
9.73443965479729));
#43786=CARTESIAN_POINT('Ctrl Pts',(-0.206384737560527,2.34771564530996,
9.73221703103888));
#43787=CARTESIAN_POINT('Ctrl Pts',(-0.198738179819942,2.35389132946558,
9.73163417717737));
#43788=CARTESIAN_POINT('Ctrl Pts',(-0.189982896015386,2.36032433467239,
9.73097353306597));
#43789=CARTESIAN_POINT('Ctrl Pts',(-0.189140753605194,2.36093684156681,
9.73091005647415));
#43790=CARTESIAN_POINT('Ctrl Pts',(-0.187876842277496,2.36184677597961,
9.73081488512686));
#43791=CARTESIAN_POINT('Ctrl Pts',(-0.187457297738772,2.36214729347195,
9.73078330955119));
#43792=CARTESIAN_POINT('Ctrl Pts',(-0.186733529275324,2.36266309898837,
9.73072886386259));
#43793=CARTESIAN_POINT('Ctrl Pts',(-0.186429649492779,2.36287887004074,
9.730706012357));
#43794=CARTESIAN_POINT('Ctrl Pts',(-0.185801741133313,2.36332308253775,
9.73065881018705));
#43795=CARTESIAN_POINT('Ctrl Pts',(-0.185477664043718,2.36355145407311,
9.73063445689574));
#43796=CARTESIAN_POINT('Ctrl Pts',(-0.184722395585458,2.36408159569706,
9.73057772097054));
#43797=CARTESIAN_POINT('Ctrl Pts',(-0.184290885682848,2.36438290804386,
9.73054532092668));
#43798=CARTESIAN_POINT('Ctrl Pts',(-0.182913530616396,2.36533966944501,
9.73044194838399));
#43799=CARTESIAN_POINT('Ctrl Pts',(-0.181964920019094,2.36599110453385,
9.73037082344262));
#43800=CARTESIAN_POINT('Ctrl Pts',(-0.16156198415252,2.37984209861582,9.72884245102156));
#43801=CARTESIAN_POINT('Ctrl Pts',(-0.140728943060134,2.3908759347482,9.72730094024204));
#43802=CARTESIAN_POINT('Ctrl Pts',(-0.0971380128821049,2.40817667079334,
9.72414230148877));
#43803=CARTESIAN_POINT('Ctrl Pts',(-0.0745139122299928,2.414414442158,9.7225362033182));
#43804=CARTESIAN_POINT('Ctrl Pts',(-0.0476865638607515,2.41874977041065,
9.72078726636761));
#43805=CARTESIAN_POINT('Ctrl Pts',(-0.0439496405399965,2.41928648058782,
9.72054720724879));
#43806=CARTESIAN_POINT('Ctrl Pts',(-0.0396248762496681,2.41983024472311,
9.72027414815069));
#43807=CARTESIAN_POINT('Ctrl Pts',(-0.0390455961610972,2.41990148122594,
9.72023767168754));
#43808=CARTESIAN_POINT('Ctrl Pts',(-0.0381861800249611,2.42000479805665,
9.72018370457097));
#43809=CARTESIAN_POINT('Ctrl Pts',(-0.0379061943391096,2.42003808454051,
9.72016614630204));
#43810=CARTESIAN_POINT('Ctrl Pts',(-0.0374084835451638,2.42009659327066,
9.72013497633107));
#43811=CARTESIAN_POINT('Ctrl Pts',(-0.0371907764593803,2.42012196084004,
9.7201213563972));
#43812=CARTESIAN_POINT('Ctrl Pts',(-0.0367296514535556,2.42017521509013,
9.72009253851741));
#43813=CARTESIAN_POINT('Ctrl Pts',(-0.0364862282470712,2.42020304621158,
9.72007734378288));
#43814=CARTESIAN_POINT('Ctrl Pts',(-0.0358355633737592,2.42027668657897,
9.72003677594483));
#43815=CARTESIAN_POINT('Ctrl Pts',(-0.0354282639708158,2.4203219968793,
9.72001143108791));
#43816=CARTESIAN_POINT('Ctrl Pts',(-0.0335066025968067,2.42053206334819,
9.71989208170253));
#43817=CARTESIAN_POINT('Ctrl Pts',(-0.0319911389339923,2.42068686174598,
9.71979863100221));
#43818=CARTESIAN_POINT('Ctrl Pts',(-0.0196668766053605,2.42185750006908,
9.71904369244579));
#43819=CARTESIAN_POINT('Ctrl Pts',(-0.00881290768415047,2.42233743589281,
9.71841017903219));
#43820=CARTESIAN_POINT('Ctrl Pts',(0.0297640250337196,2.42209255575652,
9.71620553632143));
#43821=CARTESIAN_POINT('Ctrl Pts',(0.0573435442426511,2.41834154859798,
9.71470519896699));
#43822=CARTESIAN_POINT('Ctrl Pts',(0.0865115727784765,2.41045634845394,
9.71295451375038));
#43823=CARTESIAN_POINT('Ctrl Pts',(0.0889116345882098,2.40977752876617,
9.71280930240391));
#43824=CARTESIAN_POINT('Ctrl Pts',(0.0930996700890285,2.4085403291196,9.71255369594664));
#43825=CARTESIAN_POINT('Ctrl Pts',(0.0948911200014029,2.40799408827722,
9.71244364299952));
#43826=CARTESIAN_POINT('Ctrl Pts',(0.103042272576261,2.40543080974689,9.71193944017563));
#43827=CARTESIAN_POINT('Ctrl Pts',(0.109342789235478,2.40323231052469,9.71154001766711));
#43828=CARTESIAN_POINT('Ctrl Pts',(0.116541694706376,2.40046679028313,9.71107068468672));
#43829=CARTESIAN_POINT('Ctrl Pts',(0.117511347641383,2.40008888983726,9.71100719336631));
#43830=CARTESIAN_POINT('Ctrl Pts',(0.11894885492292,2.39952061806226,9.71091265285657));
#43831=CARTESIAN_POINT('Ctrl Pts',(0.119418126202741,2.39933383013203,9.7108817243945));
#43832=CARTESIAN_POINT('Ctrl Pts',(0.120252158387223,2.39899957997237,9.71082663736028));
#43833=CARTESIAN_POINT('Ctrl Pts',(0.120617092814937,2.39885255116719,9.71080249345997));
#43834=CARTESIAN_POINT('Ctrl Pts',(0.121383752197806,2.39854203797431,9.7107516863605));
#43835=CARTESIAN_POINT('Ctrl Pts',(0.121785417924807,2.39837841026694,9.71072501835167));
#43836=CARTESIAN_POINT('Ctrl Pts',(0.122840736899737,2.3979460160531,9.71065482155169));
#43837=CARTESIAN_POINT('Ctrl Pts',(0.12349383581315,2.39767591039152,9.71061124744473));
#43838=CARTESIAN_POINT('Ctrl Pts',(0.126400980172652,2.39646237303852,9.71041669272082));
#43839=CARTESIAN_POINT('Ctrl Pts',(0.12864509346945,2.39549549203602,9.71026491676627));
#43840=CARTESIAN_POINT('Ctrl Pts',(0.144924368008203,2.38826094255759,9.70915197812451));
#43841=CARTESIAN_POINT('Ctrl Pts',(0.158504091427189,2.3810227274615,9.70815709961872));
#43842=CARTESIAN_POINT('Ctrl Pts',(0.193873218945202,2.35878916428168,9.70538365929412));
#43843=CARTESIAN_POINT('Ctrl Pts',(0.214418115340905,2.34204010927256,9.70355912743421));
#43844=CARTESIAN_POINT('Ctrl Pts',(0.234449587056449,2.32113580206036,9.70166030311343));
#43845=CARTESIAN_POINT('Ctrl Pts',(0.236188516074258,2.3192775351903,9.70149442044739));
#43846=CARTESIAN_POINT('Ctrl Pts',(0.237995550803001,2.31730004906291,9.70132110110298));
#43847=CARTESIAN_POINT('Ctrl Pts',(0.238085740899935,2.31720122813882,9.70131244814136));
#43848=CARTESIAN_POINT('Ctrl Pts',(0.238448427285877,2.31680333679867,9.70127764155284));
#43849=CARTESIAN_POINT('Ctrl Pts',(0.238720423042076,2.31650380816066,9.70125151578924));
#43850=CARTESIAN_POINT('Ctrl Pts',(0.241737083712688,2.31316918850029,9.70096151457338));
#43851=CARTESIAN_POINT('Ctrl Pts',(0.244424428647334,2.31008241985739,9.70070091239005));
#43852=CARTESIAN_POINT('Ctrl Pts',(0.247398026389371,2.30653252012041,9.70041076509293));
#43853=CARTESIAN_POINT('Ctrl Pts',(0.24774262048269,2.30611904166025,9.70037711362685));
#43854=CARTESIAN_POINT('Ctrl Pts',(0.248262749695936,2.30549174986433,9.70032628046412));
#43855=CARTESIAN_POINT('Ctrl Pts',(0.248439045929106,2.30527857318321,9.70030904376083));
#43856=CARTESIAN_POINT('Ctrl Pts',(0.24874526993362,2.30490731607397,9.70027909214027));
#43857=CARTESIAN_POINT('Ctrl Pts',(0.24887532167581,2.30474933884215,9.70026636815217));
#43858=CARTESIAN_POINT('Ctrl Pts',(0.249147580844303,2.30441797589654,9.70023972334232));
#43859=CARTESIAN_POINT('Ctrl Pts',(0.249289757723291,2.30424456566779,9.70022580480711));
#43860=CARTESIAN_POINT('Ctrl Pts',(0.249626410401491,2.3038330820903,9.7001928372904));
#43861=CARTESIAN_POINT('Ctrl Pts',(0.249820727446279,2.30359487779523,9.70017379991667));
#43862=CARTESIAN_POINT('Ctrl Pts',(0.250469294822435,2.30279750242345,9.70011022974829));
#43863=CARTESIAN_POINT('Ctrl Pts',(0.250922015132587,2.30223708112844,9.70006580711069));
#43864=CARTESIAN_POINT('Ctrl Pts',(0.251996452292413,2.30089787621244,9.69996024993827));
#43865=CARTESIAN_POINT('Ctrl Pts',(0.252616448016272,2.30011771257346,9.69989923473677));
#43866=CARTESIAN_POINT('Ctrl Pts',(0.259836386610023,2.29094557305619,9.69918730882531));
#43867=CARTESIAN_POINT('Ctrl Pts',(0.266019766997821,2.28223252866871,9.69856376919799));
#43868=CARTESIAN_POINT('Ctrl Pts',(0.282935060744857,2.25569579448488,9.69676391775409));
#43869=CARTESIAN_POINT('Ctrl Pts',(0.292387961617191,2.23712323255697,9.69562488934197));
#43870=CARTESIAN_POINT('Ctrl Pts',(0.306474581017473,2.20124115123914,9.69344298233561));
#43871=CARTESIAN_POINT('Ctrl Pts',(0.311585156899191,2.18420801882584,9.69241441053767));
#43872=CARTESIAN_POINT('Ctrl Pts',(0.315532591716083,2.1655896247659,9.69125831523383));
#43873=CARTESIAN_POINT('Ctrl Pts',(0.315790706479602,2.16433540968771,9.69118029717301));
#43874=CARTESIAN_POINT('Ctrl Pts',(0.316140874837186,2.16258099947833,9.69107096060646));
#43875=CARTESIAN_POINT('Ctrl Pts',(0.316239231772965,2.16208206279994,9.69103984338694));
#43876=CARTESIAN_POINT('Ctrl Pts',(0.316407246904658,2.16121900982434,9.69098597679048));
#43877=CARTESIAN_POINT('Ctrl Pts',(0.316477458722706,2.1608550012424,9.69096324511032));
#43878=CARTESIAN_POINT('Ctrl Pts',(0.316621674550341,2.16010032386752,9.69091609074094));
#43879=CARTESIAN_POINT('Ctrl Pts',(0.316695583922795,2.1597096377952,9.69089166507675));
#43880=CARTESIAN_POINT('Ctrl Pts',(0.316866959808635,2.1587944724058,9.69083441460974));
#43881=CARTESIAN_POINT('Ctrl Pts',(0.31696384724667,2.15826988705133,9.69080157142553));
#43882=CARTESIAN_POINT('Ctrl Pts',(0.317272539779687,2.15657495645995,9.69069536861242));
#43883=CARTESIAN_POINT('Ctrl Pts',(0.317479166862667,2.15540368890333,9.69062184449973));
#43884=CARTESIAN_POINT('Ctrl Pts',(0.320347110052166,2.13860368757796,9.68956527917788));
#43885=CARTESIAN_POINT('Ctrl Pts',(0.321857732102564,2.12280302647857,9.68854539866703));
#43886=CARTESIAN_POINT('Ctrl Pts',(0.322765895945265,2.08074538670313,9.6857623188952));
#43887=CARTESIAN_POINT('Ctrl Pts',(0.320131327700838,2.0545650565599,9.68395303870373));
#43888=CARTESIAN_POINT('Ctrl Pts',(0.313751729094932,2.0263213945268,9.68204242564132));
#43889=CARTESIAN_POINT('Ctrl Pts',(0.313113903708506,2.02365624738803,9.68186266548118));
#43890=CARTESIAN_POINT('Ctrl Pts',(0.311045257683612,2.01547488020574,9.68131310887575));
#43891=CARTESIAN_POINT('Ctrl Pts',(0.309501974975,2.00998785831035,9.68094771684389));
#43892=CARTESIAN_POINT('Ctrl Pts',(0.307619959387924,2.00391896756355,9.68054932246434));
#43893=CARTESIAN_POINT('Ctrl Pts',(0.307424145800625,2.00329426695134,9.68050838246976));
#43894=CARTESIAN_POINT('Ctrl Pts',(0.307138134588658,2.00239145848262,9.68044932045833));
#43895=CARTESIAN_POINT('Ctrl Pts',(0.30704946158886,2.00211287502759,9.68043110977744));
#43896=CARTESIAN_POINT('Ctrl Pts',(0.306892976049632,2.00162355014508,9.68039914885447));
#43897=CARTESIAN_POINT('Ctrl Pts',(0.306825325329854,2.0014127575592,9.6803853890412));
#43898=CARTESIAN_POINT('Ctrl Pts',(0.306694890901151,2.00100777216361,9.68035896930418));
#43899=CARTESIAN_POINT('Ctrl Pts',(0.306632140132289,2.0008135699033,9.68034630745979));
#43900=CARTESIAN_POINT('Ctrl Pts',(0.306464553154103,2.00029659757223,9.6803126200624));
#43901=CARTESIAN_POINT('Ctrl Pts',(0.306359391154507,1.99997393214978,9.68029161380569));
#43902=CARTESIAN_POINT('Ctrl Pts',(0.305965644879077,1.9987722581922,9.68021345285742));
#43903=CARTESIAN_POINT('Ctrl Pts',(0.305673782034734,1.99789431659462,9.68015648978955));
#43904=CARTESIAN_POINT('Ctrl Pts',(0.304942640766353,1.99572623129545,9.68001614052509));
#43905=CARTESIAN_POINT('Ctrl Pts',(0.30449894716187,1.99443758091691,9.67993300333779));
#43906=CARTESIAN_POINT('Ctrl Pts',(0.29459374035864,1.96625134973172,9.67811997973813));
#43907=CARTESIAN_POINT('Ctrl Pts',(0.281610634958944,1.94071974251957,9.67657783164741));
#43908=CARTESIAN_POINT('Ctrl Pts',(0.254054139738275,1.90070045060612,9.67384227256632));
#43909=CARTESIAN_POINT('Ctrl Pts',(0.241157391568482,1.88527518302982,9.67268848181439));
#43910=CARTESIAN_POINT('Ctrl Pts',(0.225990983968544,1.87023722719579,9.67139126148756));
#43911=CARTESIAN_POINT('Ctrl Pts',(0.225064822218721,1.86932992754876,9.67131227304987));
#43912=CARTESIAN_POINT('Ctrl Pts',(0.223765851833434,1.86807268257528,9.67120179482591));
#43913=CARTESIAN_POINT('Ctrl Pts',(0.223397638424758,1.86771799002923,9.67117051193214));
#43914=CARTESIAN_POINT('Ctrl Pts',(0.22276046617002,1.8671071312891,9.6711164362519));
#43915=CARTESIAN_POINT('Ctrl Pts',(0.22249190483519,1.86685055036391,9.67109366148995));
#43916=CARTESIAN_POINT('Ctrl Pts',(0.221935245502373,1.86632056106337,9.67104649113982));
#43917=CARTESIAN_POINT('Ctrl Pts',(0.221647084541177,1.86604721995639,9.67102209270401));
#43918=CARTESIAN_POINT('Ctrl Pts',(0.220972635679982,1.86540982189782,9.6709650332595));
#43919=CARTESIAN_POINT('Ctrl Pts',(0.220585953031272,1.86504618602526,9.67093235423016));
#43920=CARTESIAN_POINT('Ctrl Pts',(0.219340446031754,1.86388069772156,9.67082720546776));
#43921=CARTESIAN_POINT('Ctrl Pts',(0.218478141739201,1.86308259308897,9.67075457579111));
#43922=CARTESIAN_POINT('Ctrl Pts',(0.204884015400362,1.85063789719057,9.66961213293194));
#43923=CARTESIAN_POINT('Ctrl Pts',(0.191243584381455,1.84002955330688,9.66849840762894));
#43924=CARTESIAN_POINT('Ctrl Pts',(0.159422390758528,1.81914629676992,9.66597001102608));
#43925=CARTESIAN_POINT('Ctrl Pts',(0.140958016660451,1.80944010063729,9.66454536184561));
#43926=CARTESIAN_POINT('Ctrl Pts',(0.117050947254558,1.79969126141603,9.66281779162803));
#43927=CARTESIAN_POINT('Ctrl Pts',(0.112369380547921,1.79790831022279,9.66248496547189));
#43928=CARTESIAN_POINT('Ctrl Pts',(0.10569537890864,1.79554318209087,9.66201981266193));
#43929=CARTESIAN_POINT('Ctrl Pts',(0.103736105362701,1.79487004748534,9.66188437853778));
#43930=CARTESIAN_POINT('Ctrl Pts',(0.1008447564537,1.79390775489137,9.661686287607));
#43931=CARTESIAN_POINT('Ctrl Pts',(0.0999176731577746,1.79360387395548,
9.6616230380762));
#43932=CARTESIAN_POINT('Ctrl Pts',(0.0985425931815952,1.79316005279076,
9.6615296324339));
#43933=CARTESIAN_POINT('Ctrl Pts',(0.098095655878483,1.79301687639666,9.66149933680355));
#43934=CARTESIAN_POINT('Ctrl Pts',(0.0938207827218467,1.79165770959473,
9.66121018305601));
#43935=CARTESIAN_POINT('Ctrl Pts',(0.0899705219735288,1.79051233274813,
9.66095448269854));
#43936=CARTESIAN_POINT('Ctrl Pts',(0.0855269045845084,1.78928038771488,
9.66066557237252));
#43937=CARTESIAN_POINT('Ctrl Pts',(0.0849537231626,1.78912318548882,9.66062842346025));
#43938=CARTESIAN_POINT('Ctrl Pts',(0.0841088869527132,1.78889398955743,
9.6605738445402));
#43939=CARTESIAN_POINT('Ctrl Pts',(0.0838375718119742,1.78882076523002,
9.66055634353805));
#43940=CARTESIAN_POINT('Ctrl Pts',(0.0833540208688621,1.7886909396163,9.66052520049876));
#43941=CARTESIAN_POINT('Ctrl Pts',(0.0831418228972066,1.78863420040336,
9.66051155041395));
#43942=CARTESIAN_POINT('Ctrl Pts',(0.0827319949474164,1.78852506611443,
9.66048521933963));
#43943=CARTESIAN_POINT('Ctrl Pts',(0.0825343739693234,1.78847264238746,
9.66047253668263));
#43944=CARTESIAN_POINT('Ctrl Pts',(0.0819932171208717,1.78832963857264,
9.66043784587077));
#43945=CARTESIAN_POINT('Ctrl Pts',(0.0816495798421923,1.788239438093,9.66041585985452));
#43946=CARTESIAN_POINT('Ctrl Pts',(0.0803081056948663,1.78788968805235,
9.66033019643814));
#43947=CARTESIAN_POINT('Ctrl Pts',(0.0793091607788174,1.78763435568414,
9.66026676103446));
#43948=CARTESIAN_POINT('Ctrl Pts',(0.0767871373355638,1.78700259979855,
9.6601074605342));
#43949=CARTESIAN_POINT('Ctrl Pts',(0.0752624850015386,1.78663249120714,
9.66001194094924));
#43950=CARTESIAN_POINT('Ctrl Pts',(0.0690816467831274,1.78517980835601,
9.65962765012849));
#43951=CARTESIAN_POINT('Ctrl Pts',(0.064404110413597,1.78418970449458,9.6593435547836));
#43952=CARTESIAN_POINT('Ctrl Pts',(0.0461472220217545,1.78074777255789,
9.65825466628726));
#43953=CARTESIAN_POINT('Ctrl Pts',(0.0324371090219725,1.77906473163229,
9.65747915312179));
#43954=CARTESIAN_POINT('Ctrl Pts',(-0.00459485485672079,1.77691690260174,
9.65540346189885));
#43955=CARTESIAN_POINT('Ctrl Pts',(-0.0279253700752546,1.77809339996285,
9.65411083291383));
#43956=CARTESIAN_POINT('Ctrl Pts',(-0.0525708204126776,1.78203732300837,
9.65263860172436));
#43957=CARTESIAN_POINT('Ctrl Pts',(-0.0542149651854748,1.78231353109772,
9.65253990278948));
#43958=CARTESIAN_POINT('Ctrl Pts',(-0.0609871603706854,1.78350532880924,
9.65213126043745));
#43959=CARTESIAN_POINT('Ctrl Pts',(-0.0660945622508937,1.78453238722273,
9.65181807030848));
#43960=CARTESIAN_POINT('Ctrl Pts',(-0.0720215679705755,1.78587450998456,
9.65144801434797));
#43961=CARTESIAN_POINT('Ctrl Pts',(-0.0728677325276198,1.78606971591847,
9.6513950258484));
#43962=CARTESIAN_POINT('Ctrl Pts',(-0.0742172705369502,1.7863867977772,
9.65131025934326));
#43963=CARTESIAN_POINT('Ctrl Pts',(-0.0747211611001894,1.78650647226252,
9.65127855218297));
#43964=CARTESIAN_POINT('Ctrl Pts',(-0.0756103630484235,1.78671992421559,
9.65122249783128));
#43965=CARTESIAN_POINT('Ctrl Pts',(-0.0759957948580573,1.78681319943928,
9.6511981668653));
#43966=CARTESIAN_POINT('Ctrl Pts',(-0.0767927284878099,1.78700761664186,
9.65114778896317));
#43967=CARTESIAN_POINT('Ctrl Pts',(-0.0772042047549721,1.78710885925895,
9.65112173882189));
#43968=CARTESIAN_POINT('Ctrl Pts',(-0.0782580297563936,1.7873703553762,
9.65105492217032));
#43969=CARTESIAN_POINT('Ctrl Pts',(-0.0789000842249391,1.78753177662712,
9.65101411801351));
#43970=CARTESIAN_POINT('Ctrl Pts',(-0.0815261491698611,1.78820061513566,
9.65084683091554));
#43971=CARTESIAN_POINT('Ctrl Pts',(-0.083505764720183,1.78872495065035,
9.65071980180084));
#43972=CARTESIAN_POINT('Ctrl Pts',(-0.0965745684920587,1.79232008894459,
9.64987493425429));
#43973=CARTESIAN_POINT('Ctrl Pts',(-0.107496235180663,1.79596368469782,
9.64913847784199));
#43974=CARTESIAN_POINT('Ctrl Pts',(-0.129395424622546,1.80459713889712,
9.64759771418822));
#43975=CARTESIAN_POINT('Ctrl Pts',(-0.140335201254751,1.80963468491326,
9.64679301073633));
#43976=CARTESIAN_POINT('Ctrl Pts',(-0.160825555686133,1.82049895660885,
9.64522823538065));
#43977=CARTESIAN_POINT('Ctrl Pts',(-0.17040606698088,1.82623465177606,9.64447028875704));
#43978=CARTESIAN_POINT('Ctrl Pts',(-0.19150560710119,1.84040408036623,9.64276092390233));
#43979=CARTESIAN_POINT('Ctrl Pts',(-0.202802618122204,1.84913022313688,
9.64181587047063));
#43980=CARTESIAN_POINT('Ctrl Pts',(-0.214160064984539,1.85917339731651,
9.64086250368771));
#43981=CARTESIAN_POINT('Ctrl Pts',(-0.214831935488261,1.85977255457693,
9.64080609495576));
#43982=CARTESIAN_POINT('Ctrl Pts',(-0.215733708240548,1.86058354180188,
9.64073038054132));
#43983=CARTESIAN_POINT('Ctrl Pts',(-0.215965817402716,1.86079289508265,
9.64071089192738));
#43984=CARTESIAN_POINT('Ctrl Pts',(-0.216356540145974,1.86114634379626,
9.6406780856364));
#43985=CARTESIAN_POINT('Ctrl Pts',(-0.216515314616055,1.86129025976481,
9.64066475444523));
#43986=CARTESIAN_POINT('Ctrl Pts',(-0.216819916785194,1.86156691044629,
9.64063917932997));
#43987=CARTESIAN_POINT('Ctrl Pts',(-0.216965765125472,1.86169961965489,
9.64062693368429));
#43988=CARTESIAN_POINT('Ctrl Pts',(-0.217266714589235,1.86197396261683,
9.64060166565402));
#43989=CARTESIAN_POINT('Ctrl Pts',(-0.217421798549298,1.86211561367562,
9.64058864470244));
#43990=CARTESIAN_POINT('Ctrl Pts',(-0.217771890320768,1.86243600990774,
9.64055925059881));
#43991=CARTESIAN_POINT('Ctrl Pts',(-0.217966817056536,1.86261484404903,
9.64054288421044));
#43992=CARTESIAN_POINT('Ctrl Pts',(-0.218879440232389,1.86345419547722,
9.64046625697669));
#43993=CARTESIAN_POINT('Ctrl Pts',(-0.219594365894017,1.86411773801526,
9.64040622392944));
#43994=CARTESIAN_POINT('Ctrl Pts',(-0.227868223018751,1.87186715451755,
9.63971124320402));
#43995=CARTESIAN_POINT('Ctrl Pts',(-0.235085117380544,1.87931117101581,
9.63910287960286));
#43996=CARTESIAN_POINT('Ctrl Pts',(-0.246446218813147,1.89222094044135,
9.63811526922609));
#43997=CARTESIAN_POINT('Ctrl Pts',(-0.250796775581789,1.89749355473368,
9.63772882436611));
#43998=CARTESIAN_POINT('Ctrl Pts',(-0.267409485491206,1.91898450258699,
9.63620240134716));
#43999=CARTESIAN_POINT('Ctrl Pts',(-0.278292231497932,1.93620789944952,
9.63508166515518));
#44000=CARTESIAN_POINT('Ctrl Pts',(-0.289465650486568,1.95826040287656,
9.63365841333895));
#44001=CARTESIAN_POINT('Ctrl Pts',(-0.291370859629078,1.96221939135869,
9.63340349084786));
#44002=CARTESIAN_POINT('Ctrl Pts',(-0.293948058140469,1.96786745300775,
9.6330397951582));
#44003=CARTESIAN_POINT('Ctrl Pts',(-0.294687645890394,1.9695252436679,9.63293304483894));
#44004=CARTESIAN_POINT('Ctrl Pts',(-0.298025339558335,1.97717986953488,
9.63243997253386));
#44005=CARTESIAN_POINT('Ctrl Pts',(-0.300454513442979,1.9832482821958,9.63204856364141));
#44006=CARTESIAN_POINT('Ctrl Pts',(-0.303052461128865,1.99035762013918,
9.63158789255539));
#44007=CARTESIAN_POINT('Ctrl Pts',(-0.303402821716402,1.99133089954722,
9.6315247817099));
#44008=CARTESIAN_POINT('Ctrl Pts',(-0.303916853318795,1.99278071188368,
9.63143069921532));
#44009=CARTESIAN_POINT('Ctrl Pts',(-0.304084104740397,1.99325597574082,
9.63139984658037));
#44010=CARTESIAN_POINT('Ctrl Pts',(-0.304379924156572,1.99410291755908,
9.63134484474805));
#44011=CARTESIAN_POINT('Ctrl Pts',(-0.304508927864861,1.99447444315486,
9.631320710057));
#44012=CARTESIAN_POINT('Ctrl Pts',(-0.304778981913126,1.99525680693905,
9.63126987135502));
#44013=CARTESIAN_POINT('Ctrl Pts',(-0.304919882252861,1.99566769573825,
9.63124316243321));
#44014=CARTESIAN_POINT('Ctrl Pts',(-0.305288802220212,1.99675065839842,
9.63117274248554));
#44015=CARTESIAN_POINT('Ctrl Pts',(-0.305515432337938,1.99742320002702,
9.63112898561881));
#44016=CARTESIAN_POINT('Ctrl Pts',(-0.306521456895406,2.00044156275256,
9.63093249002478));
#44017=CARTESIAN_POINT('Ctrl Pts',(-0.307276051298396,2.00279550568328,
9.63077893630882));
#44018=CARTESIAN_POINT('Ctrl Pts',(-0.312616496928581,2.02013880424848,
9.62964504455104));
#44019=CARTESIAN_POINT('Ctrl Pts',(-0.316129707743057,2.03543404583506,
9.62862959870862));
#44020=CARTESIAN_POINT('Ctrl Pts',(-0.321031559363108,2.06724720442419,
9.62649063397092));
#44021=CARTESIAN_POINT('Ctrl Pts',(-0.322287987666894,2.08374034465902,
9.62536730016875));
#44022=CARTESIAN_POINT('Ctrl Pts',(-0.322274898786015,2.10025541625633,
9.62425288911819));
#44023=CARTESIAN_POINT('',(-0.322274974372014,2.0998714756124,9.37464719300612));
#44024=CARTESIAN_POINT('Ctrl Pts',(-0.32227489852238,2.1002557486849,9.62425286668644));
#44025=CARTESIAN_POINT('Ctrl Pts',(-0.322262200382935,2.11625697114477,
9.62317312952553));
#44026=CARTESIAN_POINT('Ctrl Pts',(-0.32105779650295,2.13223770964696,9.62210508086643));
#44027=CARTESIAN_POINT('Ctrl Pts',(-0.318559698462321,2.14880006876696,
9.62104974482184));
#44028=CARTESIAN_POINT('Ctrl Pts',(-0.318446288819205,2.14953472881498,
9.62100304252109));
#44029=CARTESIAN_POINT('Ctrl Pts',(-0.318267537075045,2.15066668100986,
9.62093126009712));
#44030=CARTESIAN_POINT('Ctrl Pts',(-0.318203991608626,2.15106424824529,
9.6209060819385));
#44031=CARTESIAN_POINT('Ctrl Pts',(-0.318097551833309,2.15172226614342,
9.62086446587441));
#44032=CARTESIAN_POINT('Ctrl Pts',(-0.318055082501554,2.15198278362567,
9.62084800425017));
#44033=CARTESIAN_POINT('Ctrl Pts',(-0.317978271682708,2.15245034230063,
9.62081848681461));
#44034=CARTESIAN_POINT('Ctrl Pts',(-0.317944047994441,2.15265740228388,
9.62080542433574));
#44035=CARTESIAN_POINT('Ctrl Pts',(-0.317877288140574,2.15305887450531,
9.62078011573428));
#44036=CARTESIAN_POINT('Ctrl Pts',(-0.317844775902008,2.15325329015126,
9.62076786828978));
#44037=CARTESIAN_POINT('Ctrl Pts',(-0.317776494501317,2.15365930693899,
9.62074230842603));
#44038=CARTESIAN_POINT('Ctrl Pts',(-0.317740692463515,2.15387090153504,
9.62072899795028));
#44039=CARTESIAN_POINT('Ctrl Pts',(-0.317652038852291,2.15439169268582,
9.62069626151754));
#44040=CARTESIAN_POINT('Ctrl Pts',(-0.31759894702101,2.15470084892705,9.62067684928027));
#44041=CARTESIAN_POINT('Ctrl Pts',(-0.317390446015414,2.15590442321913,
9.62060135579262));
#44042=CARTESIAN_POINT('Ctrl Pts',(-0.31723170734028,2.15679827164526,9.62054546216686));
#44043=CARTESIAN_POINT('Ctrl Pts',(-0.314185992258422,2.17353736242995,
9.6195017760887));
#44044=CARTESIAN_POINT('Ctrl Pts',(-0.310118498624611,2.1891473767991,9.61857899885584));
#44045=CARTESIAN_POINT('Ctrl Pts',(-0.303523922562006,2.20840871653887,
9.61743207485421));
#44046=CARTESIAN_POINT('Ctrl Pts',(-0.302068576776011,2.21240016502262,
9.61719397365354));
#44047=CARTESIAN_POINT('Ctrl Pts',(-0.299115915760111,2.22002618872931,
9.61673639628704));
#44048=CARTESIAN_POINT('Ctrl Pts',(-0.297630190971355,2.22366441101369,
9.61651690271767));
#44049=CARTESIAN_POINT('Ctrl Pts',(-0.29278406786216,2.23493792828201,9.6158308302073));
#44050=CARTESIAN_POINT('Ctrl Pts',(-0.289193613252246,2.24247036002145,
9.61536370601801));
#44051=CARTESIAN_POINT('Ctrl Pts',(-0.277972408313161,2.26383489276387,
9.61399617820118));
#44052=CARTESIAN_POINT('Ctrl Pts',(-0.269613145963772,2.27725457793182,
9.61308221121115));
#44053=CARTESIAN_POINT('Ctrl Pts',(-0.258841199852033,2.29201190703257,
9.61198032464317));
#44054=CARTESIAN_POINT('Ctrl Pts',(-0.257354390451935,2.29400014527333,
9.6118297288318));
#44055=CARTESIAN_POINT('Ctrl Pts',(-0.255412555826358,2.29653525689399,
9.61163485739529));
#44056=CARTESIAN_POINT('Ctrl Pts',(-0.254978459021187,2.29709811338156,
9.61159140779182));
#44057=CARTESIAN_POINT('Ctrl Pts',(-0.254275939551286,2.29800280576156,
9.6115212719459));
#44058=CARTESIAN_POINT('Ctrl Pts',(-0.2540086795961,2.29834554497405,9.61149463186924));
#44059=CARTESIAN_POINT('Ctrl Pts',(-0.253498295711054,2.29899734753555,
9.61144383636427));
#44060=CARTESIAN_POINT('Ctrl Pts',(-0.253255297658299,2.29930650882603,
9.61141968597809));
#44061=CARTESIAN_POINT('Ctrl Pts',(-0.252699948816612,2.3000104119233,9.61136456898333));
#44062=CARTESIAN_POINT('Ctrl Pts',(-0.252387238360407,2.30040486750044,
9.61133358803049));
#44063=CARTESIAN_POINT('Ctrl Pts',(-0.251430539233022,2.30160586499184,
9.61123897106904));
#44064=CARTESIAN_POINT('Ctrl Pts',(-0.250783603796875,2.30241004146305,
9.61117521687842));
#44065=CARTESIAN_POINT('Ctrl Pts',(-0.246043343329121,2.30824483490925,
9.61070969752524));
#44066=CARTESIAN_POINT('Ctrl Pts',(-0.241803108043954,2.31315366557734,
9.61030198837819));
#44067=CARTESIAN_POINT('Ctrl Pts',(-0.23702695959817,2.31835688745248,9.60985142922304));
#44068=CARTESIAN_POINT('Ctrl Pts',(-0.236634860480233,2.31878174666313,
9.60981450207376));
#44069=CARTESIAN_POINT('Ctrl Pts',(-0.219260692004582,2.33750618960886,
9.6081809467608));
#44070=CARTESIAN_POINT('Ctrl Pts',(-0.200213234783425,2.35376898319434,
9.60649414298764));
#44071=CARTESIAN_POINT('Ctrl Pts',(-0.169107449288632,2.37462694249824,
9.60396166265019));
#44072=CARTESIAN_POINT('Ctrl Pts',(-0.158333428910285,2.38097661047446,
9.60312056227439));
#44073=CARTESIAN_POINT('Ctrl Pts',(-0.143380544254812,2.38865515258379,
9.60202291003595));
#44074=CARTESIAN_POINT('Ctrl Pts',(-0.139504468742105,2.3905482486897,9.60174440643881));
#44075=CARTESIAN_POINT('Ctrl Pts',(-0.134270435620357,2.39297567453766,
9.60137742851918));
#44076=CARTESIAN_POINT('Ctrl Pts',(-0.132945349283149,2.39357934198294,
9.60128528981925));
#44077=CARTESIAN_POINT('Ctrl Pts',(-0.130726949434735,2.39457187467758,
9.60113236892195));
#44078=CARTESIAN_POINT('Ctrl Pts',(-0.129835896943699,2.39496570068809,
9.60107130256961));
#44079=CARTESIAN_POINT('Ctrl Pts',(-0.128701317121672,2.39546102310331,
9.60099401158509));
#44080=CARTESIAN_POINT('Ctrl Pts',(-0.128459444896338,2.39556626367063,
9.60097756129436));
#44081=CARTESIAN_POINT('Ctrl Pts',(-0.128024947095562,2.3957546830887,9.60094805849397));
#44082=CARTESIAN_POINT('Ctrl Pts',(-0.127832369349131,2.39583797084706,
9.60093499933557));
#44083=CARTESIAN_POINT('Ctrl Pts',(-0.12745873450257,2.39599913085923,9.60090969550594));
#44084=CARTESIAN_POINT('Ctrl Pts',(-0.127277687473913,2.39607702501623,
9.60089744951695));
#44085=CARTESIAN_POINT('Ctrl Pts',(-0.126899269591281,2.39623942529309,
9.60087188506872));
#44086=CARTESIAN_POINT('Ctrl Pts',(-0.126701886352943,2.39632390000818,
9.60085856856663));
#44087=CARTESIAN_POINT('Ctrl Pts',(-0.126215593575093,2.39653144551308,
9.60082580454638));
#44088=CARTESIAN_POINT('Ctrl Pts',(-0.125926587550521,2.39665429170909,
9.60080637079407));
#44089=CARTESIAN_POINT('Ctrl Pts',(-0.12479918848569,2.39713156462441,9.60073070716098));
#44090=CARTESIAN_POINT('Ctrl Pts',(-0.123959464514552,2.39748286563609,
9.60067466597537));
#44091=CARTESIAN_POINT('Ctrl Pts',(-0.109602727176092,2.40341770357699,
9.59972172271853));
#44092=CARTESIAN_POINT('Ctrl Pts',(-0.0957205202169412,2.4080791540464,
9.59887836496327));
#44093=CARTESIAN_POINT('Ctrl Pts',(-0.0647724982464628,2.41617572595831,
9.59706923663539));
#44094=CARTESIAN_POINT('Ctrl Pts',(-0.047649535788878,2.41920542803547,
9.5961120391964));
#44095=CARTESIAN_POINT('Ctrl Pts',(-0.0277172395205832,2.42109189847781,
9.59497935859231));
#44096=CARTESIAN_POINT('Ctrl Pts',(-0.0250658405173782,2.42130975075981,
9.59482835755838));
#44097=CARTESIAN_POINT('Ctrl Pts',(-0.0120856330054162,2.42221462852288,
9.59408668449346));
#44098=CARTESIAN_POINT('Ctrl Pts',(-0.0017313098922815,2.42243651090348,
9.5934872682096));
#44099=CARTESIAN_POINT('Ctrl Pts',(0.0141499249286719,2.42201181827835,
9.59254417541785));
#44100=CARTESIAN_POINT('Ctrl Pts',(0.0196797071634084,2.42172120682249,
9.59221142530428));
#44101=CARTESIAN_POINT('Ctrl Pts',(0.0261088941127144,2.42121695821156,
9.59181856411351));
#44102=CARTESIAN_POINT('Ctrl Pts',(0.027018456789112,2.42114173126566,9.59176284510302));
#44103=CARTESIAN_POINT('Ctrl Pts',(0.0284047419802902,2.42102114504787,
9.5916777058286));
#44104=CARTESIAN_POINT('Ctrl Pts',(0.0288817084638099,2.42097858471723,
9.59164837360437));
#44105=CARTESIAN_POINT('Ctrl Pts',(0.0297104511044625,2.42090277277109,
9.59159733939132));
#44106=CARTESIAN_POINT('Ctrl Pts',(0.0300622716399671,2.42087000529694,
9.59157565266798));
#44107=CARTESIAN_POINT('Ctrl Pts',(0.0307949967019486,2.4208005458817,9.59153044133358));
#44108=CARTESIAN_POINT('Ctrl Pts',(0.0311758910053264,2.4207637539965,9.59150691360876));
#44109=CARTESIAN_POINT('Ctrl Pts',(0.0321068169729162,2.42067215885965,
9.59144934806742));
#44110=CARTESIAN_POINT('Ctrl Pts',(0.0326567734245254,2.42061661888814,
9.59141528710243));
#44111=CARTESIAN_POINT('Ctrl Pts',(0.0347566106547962,2.42039909802098,
9.59128503011621));
#44112=CARTESIAN_POINT('Ctrl Pts',(0.0363054324183795,2.42022729339774,
9.59118852513341));
#44113=CARTESIAN_POINT('Ctrl Pts',(0.0639137852114066,2.41696194218873,
9.58946046070311));
#44114=CARTESIAN_POINT('Ctrl Pts',(0.0894947956353229,2.41070877779957,
9.58772234137034));
#44115=CARTESIAN_POINT('Ctrl Pts',(0.125759547124205,2.39698990098813,9.58510099455854));
#44116=CARTESIAN_POINT('Ctrl Pts',(0.137220981084427,2.39187134585129,9.58424942537694));
#44117=CARTESIAN_POINT('Ctrl Pts',(0.154585295669267,2.38286713023584,9.5829456135246));
#44118=CARTESIAN_POINT('Ctrl Pts',(0.16070867663877,2.37943364438964,9.5824831341886));
#44119=CARTESIAN_POINT('Ctrl Pts',(0.170394335078156,2.37357892060517,9.58175261457821));
#44120=CARTESIAN_POINT('Ctrl Pts',(0.174028602965502,2.37128159736772,9.58147875662744));
#44121=CARTESIAN_POINT('Ctrl Pts',(0.17807485841601,2.36860905195801,9.58117509203288));
#44122=CARTESIAN_POINT('Ctrl Pts',(0.178532916415187,2.36830481874274,9.58114073380981));
#44123=CARTESIAN_POINT('Ctrl Pts',(0.179174893619348,2.36787605800137,9.58109260830749));
#44124=CARTESIAN_POINT('Ctrl Pts',(0.179359462830936,2.36775251268208,9.58107877545264));
#44125=CARTESIAN_POINT('Ctrl Pts',(0.179729637470673,2.3675041739151,9.58105103891933));
#44126=CARTESIAN_POINT('Ctrl Pts',(0.179915241297113,2.36737937765932,9.58103713541177));
#44127=CARTESIAN_POINT('Ctrl Pts',(0.180270957688532,2.36713966306584,9.58101049569891));
#44128=CARTESIAN_POINT('Ctrl Pts',(0.180441090084959,2.36702477558911,9.5809977574241));
#44129=CARTESIAN_POINT('Ctrl Pts',(0.180842396925008,2.3667532213209,9.58096771726819));
#44130=CARTESIAN_POINT('Ctrl Pts',(0.181073478187405,2.3665964161596,9.58095042480586));
#44131=CARTESIAN_POINT('Ctrl Pts',(0.181874238109931,2.36605152185603,9.58089051905368));
#44132=CARTESIAN_POINT('Ctrl Pts',(0.182442880431044,2.36566190199324,9.58084800882122));
#44133=CARTESIAN_POINT('Ctrl Pts',(0.189277482867107,2.36094670496566,9.58033738346792));
#44134=CARTESIAN_POINT('Ctrl Pts',(0.19539009704611,2.35640179442417,9.5798838542713));
#44135=CARTESIAN_POINT('Ctrl Pts',(0.204583388007249,2.34904638882819,9.57919700659558));
#44136=CARTESIAN_POINT('Ctrl Pts',(0.207779810020162,2.34638591538527,9.57895725704352));
#44137=CARTESIAN_POINT('Ctrl Pts',(0.227227294108857,2.32955152005743,9.57748654493841));
#44138=CARTESIAN_POINT('Ctrl Pts',(0.242073486590309,2.31383789687348,9.57630693256959));
#44139=CARTESIAN_POINT('Ctrl Pts',(0.264664552003215,2.28453229202876,9.5742078271869));
#44140=CARTESIAN_POINT('Ctrl Pts',(0.273197779444786,2.27164606688306,9.57331323507061));
#44141=CARTESIAN_POINT('Ctrl Pts',(0.281976865919095,2.25606480793316,9.57223444345279));
#44142=CARTESIAN_POINT('Ctrl Pts',(0.283155031914784,2.25391687554846,9.57208582322332));
#44143=CARTESIAN_POINT('Ctrl Pts',(0.284641681938783,2.25113169407895,9.57189315725605));
#44144=CARTESIAN_POINT('Ctrl Pts',(0.28497273514287,2.25050653229922,9.57184991454794));
#44145=CARTESIAN_POINT('Ctrl Pts',(0.285503502177493,2.24949620097949,9.57178003250549));
#44146=CARTESIAN_POINT('Ctrl Pts',(0.285704502469419,2.24911170688011,9.57175343873018));
#44147=CARTESIAN_POINT('Ctrl Pts',(0.286086277894366,2.24837780155266,9.5717026785355));
#44148=CARTESIAN_POINT('Ctrl Pts',(0.286267190987562,2.24802846265149,9.57167851704167));
#44149=CARTESIAN_POINT('Ctrl Pts',(0.28667878307703,2.2472301116744,9.57162330068709));
#44150=CARTESIAN_POINT('Ctrl Pts',(0.286909047234248,2.24678088792719,9.5715922312924));
#44151=CARTESIAN_POINT('Ctrl Pts',(0.287610149502256,2.24540515000235,9.57149708159677));
#44152=CARTESIAN_POINT('Ctrl Pts',(0.288077558600378,2.24447690450115,9.57143288115675));
#44153=CARTESIAN_POINT('Ctrl Pts',(0.291498511127966,2.2376005002462,9.57095726035912));
#44154=CARTESIAN_POINT('Ctrl Pts',(0.294271866965297,2.2315649550397,9.57053960211202));
#44155=CARTESIAN_POINT('Ctrl Pts',(0.29769817705045,2.22345705565405,9.56997768814089));
#44156=CARTESIAN_POINT('Ctrl Pts',(0.298519620662459,2.22145733793528,9.56983903659537));
#44157=CARTESIAN_POINT('Ctrl Pts',(0.30461196548733,2.20619092602549,9.56878005247665));
#44158=CARTESIAN_POINT('Ctrl Pts',(0.309015694559345,2.19259687341035,9.56783327375727));
#44159=CARTESIAN_POINT('Ctrl Pts',(0.317052240468025,2.16070832568831,9.56562049512444));
#44160=CARTESIAN_POINT('Ctrl Pts',(0.320028753029072,2.14229940775301,9.56434813988974));
#44161=CARTESIAN_POINT('Ctrl Pts',(0.322002352563823,2.11557606543788,9.56257572151944));
#44162=CARTESIAN_POINT('Ctrl Pts',(0.322294072033266,2.10739498105171,9.56204346907199));
#44163=CARTESIAN_POINT('Ctrl Pts',(0.322271937457032,2.09835464559558,9.56147291617144));
#44164=CARTESIAN_POINT('Ctrl Pts',(0.322266428092087,2.09749835518705,9.56141904902585));
#44165=CARTESIAN_POINT('Ctrl Pts',(0.32225085192922,2.09600351792167,9.56132532983165));
#44166=CARTESIAN_POINT('Ctrl Pts',(0.322242299990887,2.09536496480488,9.56128539669779));
#44167=CARTESIAN_POINT('Ctrl Pts',(0.32222707184162,2.09443447573501,9.56122735829162));
#44168=CARTESIAN_POINT('Ctrl Pts',(0.322221896895899,2.09414252184006,9.56120916966992));
#44169=CARTESIAN_POINT('Ctrl Pts',(0.322212099423005,2.09362915592398,9.56117722586175));
#44170=CARTESIAN_POINT('Ctrl Pts',(0.322207645462111,2.09340774122246,9.56116346116637));
#44171=CARTESIAN_POINT('Ctrl Pts',(0.322198555549368,2.09297789993895,9.561136763985));
#44172=CARTESIAN_POINT('Ctrl Pts',(0.322193945597875,2.09276947387359,9.56112383004818));
#44173=CARTESIAN_POINT('Ctrl Pts',(0.322182406982745,2.09226972360657,9.56109284464231));
#44174=CARTESIAN_POINT('Ctrl Pts',(0.322175285414927,2.09197840342102,9.56107480405686));
#44175=CARTESIAN_POINT('Ctrl Pts',(0.322152374648972,2.09109049388134,9.56101988379818));
#44176=CARTESIAN_POINT('Ctrl Pts',(0.322135323297227,2.09049393410301,9.56098307440614));
#44177=CARTESIAN_POINT('Ctrl Pts',(0.321929495049367,2.08393118524587,9.5605790899159));
#44178=CARTESIAN_POINT('Ctrl Pts',(0.321576636889494,2.07797083062628,9.56022087105718));
#44179=CARTESIAN_POINT('Ctrl Pts',(0.320849482351277,2.06962607213052,9.55972727286096));
#44180=CARTESIAN_POINT('Ctrl Pts',(0.320613746052935,2.06723123117278,9.55958653631537));
#44181=CARTESIAN_POINT('Ctrl Pts',(0.317112316144761,2.03532958863653,9.55772145355924));
#44182=CARTESIAN_POINT('Ctrl Pts',(0.309811651127446,2.00640765961136,9.55612782221892));
#44183=CARTESIAN_POINT('Ctrl Pts',(0.294402274104891,1.96840795179206,9.55376650848369));
#44184=CARTESIAN_POINT('Ctrl Pts',(0.289602167492814,1.95815604146774,9.55310166458326));
#44185=CARTESIAN_POINT('Ctrl Pts',(0.283318703559918,1.94639077166714,9.55229512733951));
#44186=CARTESIAN_POINT('Ctrl Pts',(0.282347152558168,1.94461220135647,9.55217199681078));
#44187=CARTESIAN_POINT('Ctrl Pts',(0.281037339644572,1.9422672380458,9.55200800690835));
#44188=CARTESIAN_POINT('Ctrl Pts',(0.28071400674343,1.94169252425718,9.55196768325072));
#44189=CARTESIAN_POINT('Ctrl Pts',(0.280180290848348,1.9407506379302,9.55190137847451));
#44190=CARTESIAN_POINT('Ctrl Pts',(0.279970943418237,1.94038287830468,9.55187543469108));
#44191=CARTESIAN_POINT('Ctrl Pts',(0.279563896009068,1.93967108458481,9.55182511353908));
#44192=CARTESIAN_POINT('Ctrl Pts',(0.279366283698531,1.93932700102315,9.55180073936971));
#44193=CARTESIAN_POINT('Ctrl Pts',(0.278908566316841,1.93853341842758,9.55174441049451));
#44194=CARTESIAN_POINT('Ctrl Pts',(0.278648009691453,1.93808418230589,9.55171243947689));
#44195=CARTESIAN_POINT('Ctrl Pts',(0.277810078809478,1.9366474849296,9.55160992250343));
#44196=CARTESIAN_POINT('Ctrl Pts',(0.277228537538048,1.93566247540991,9.55153922533839));
#44197=CARTESIAN_POINT('Ctrl Pts',(0.271822131594927,1.92661551753557,9.55088606290102));
#44198=CARTESIAN_POINT('Ctrl Pts',(0.266652572284206,1.91876582547396,9.55029096810441));
#44199=CARTESIAN_POINT('Ctrl Pts',(0.2575564174807,1.90618711625269,9.54928780248056));
#44200=CARTESIAN_POINT('Ctrl Pts',(0.253824097440571,1.90132422772779,9.54888686715949));
#44201=CARTESIAN_POINT('Ctrl Pts',(0.23546340181205,1.878764235516,9.54696487238793));
#44202=CARTESIAN_POINT('Ctrl Pts',(0.219110156697215,1.86255764209322,9.5453904925347));
#44203=CARTESIAN_POINT('Ctrl Pts',(0.196200223475837,1.84425164395871,9.5434303131087));
#44204=CARTESIAN_POINT('Ctrl Pts',(0.191106881836289,1.84042357958275,9.54300847770785));
#44205=CARTESIAN_POINT('Ctrl Pts',(0.181618528278885,1.83372307855538,9.54225199652814));
#44206=CARTESIAN_POINT('Ctrl Pts',(0.177260359660562,1.83080218932308,9.54191522249682));
#44207=CARTESIAN_POINT('Ctrl Pts',(0.172272005362578,1.82763265094092,9.54154330565076));
#44208=CARTESIAN_POINT('Ctrl Pts',(0.171710369556634,1.82727822663,9.54150162166511));
#44209=CARTESIAN_POINT('Ctrl Pts',(0.170706536442728,1.82664908078055,9.54142746208543));
#44210=CARTESIAN_POINT('Ctrl Pts',(0.170264763597251,1.82637369112494,9.54139494368331));
#44211=CARTESIAN_POINT('Ctrl Pts',(0.169594624499057,1.82595819526466,9.54134579657827));
#44212=CARTESIAN_POINT('Ctrl Pts',(0.169366750303672,1.82581730307256,9.54132911620578));
#44213=CARTESIAN_POINT('Ctrl Pts',(0.168970518307262,1.825572999496,9.54130016731315));
#44214=CARTESIAN_POINT('Ctrl Pts',(0.168802241245001,1.8254694588682,9.54128789020965));
#44215=CARTESIAN_POINT('Ctrl Pts',(0.168452494093744,1.8252547031193,9.54126240946086));
#44216=CARTESIAN_POINT('Ctrl Pts',(0.168271009577188,1.82514351333658,9.54124920750826));
#44217=CARTESIAN_POINT('Ctrl Pts',(0.167772447948109,1.82483873937888,9.54121299468463));
#44218=CARTESIAN_POINT('Ctrl Pts',(0.167455144778372,1.82464552277536,9.54119000811692));
#44219=CARTESIAN_POINT('Ctrl Pts',(0.166232521407313,1.82390392111312,9.54110166719506));
#44220=CARTESIAN_POINT('Ctrl Pts',(0.165324822862846,1.82335944084633,9.54103656630801));
#44221=CARTESIAN_POINT('Ctrl Pts',(0.148991893445009,1.81367128148101,9.53987352616547));
#44222=CARTESIAN_POINT('Ctrl Pts',(0.132830145442655,1.80582475657567,9.53885537707198));
#44223=CARTESIAN_POINT('Ctrl Pts',(0.0872678167512609,1.788229920304,9.53611492919086));
#44224=CARTESIAN_POINT('Ctrl Pts',(0.0569913055994698,1.78130258358455,
9.53441383211136));
#44225=CARTESIAN_POINT('Ctrl Pts',(0.0241819768845004,1.77862720009411,
9.53242319043524));
#44226=CARTESIAN_POINT('Ctrl Pts',(0.0221700400539088,1.77848214114527,
9.53230063097016));
#44227=CARTESIAN_POINT('Ctrl Pts',(0.0194999424237518,1.77831481045842,
9.53213728876131));
#44228=CARTESIAN_POINT('Ctrl Pts',(0.0188428552820707,1.77827565258498,
9.53209703636636));
#44229=CARTESIAN_POINT('Ctrl Pts',(0.0177634174025764,1.77821464377222,
9.53203081877783));
#44230=CARTESIAN_POINT('Ctrl Pts',(0.0173411332415027,1.77819161046415,
9.53200489072639));
#44231=CARTESIAN_POINT('Ctrl Pts',(0.0165224530627962,1.7781485720087,9.53195457862853));
#44232=CARTESIAN_POINT('Ctrl Pts',(0.0161260628354912,1.77812846778499,
9.53193019773693));
#44233=CARTESIAN_POINT('Ctrl Pts',(0.0152102808405446,1.77808371684926,
9.53187382224672));
#44234=CARTESIAN_POINT('Ctrl Pts',(0.0146908655803926,1.778059594856,9.53184181125095));
#44235=CARTESIAN_POINT('Ctrl Pts',(0.0130251493995336,1.77798627740993,
9.53173903879166));
#44236=CARTESIAN_POINT('Ctrl Pts',(0.0118786529883231,1.77794194684527,
9.53166812505455));
#44237=CARTESIAN_POINT('Ctrl Pts',(0.0012295803227088,1.77758712937605,
9.53100777644001));
#44238=CARTESIAN_POINT('Ctrl Pts',(-0.00828123938175379,1.77769120185321,
9.53040540354889));
#44239=CARTESIAN_POINT('Ctrl Pts',(-0.0484849893704627,1.77991173552702,
9.52780206738453));
#44240=CARTESIAN_POINT('Ctrl Pts',(-0.0787944586706913,1.78599659003403,
9.52567840086594));
#44241=CARTESIAN_POINT('Ctrl Pts',(-0.116587095282174,1.79940711355527,
9.52301290550568));
#44242=CARTESIAN_POINT('Ctrl Pts',(-0.125261250160921,1.80291703217472,
9.52240163803254));
#44243=CARTESIAN_POINT('Ctrl Pts',(-0.134612679942308,1.8071835772769,9.52175229565125));
#44244=CARTESIAN_POINT('Ctrl Pts',(-0.135452470403925,1.80757110380903,
9.52169407098286));
#44245=CARTESIAN_POINT('Ctrl Pts',(-0.136911382833796,1.80825196111897,
9.52159309039891));
#44246=CARTESIAN_POINT('Ctrl Pts',(-0.137531254346956,1.80854365843481,
9.52155023862078));
#44247=CARTESIAN_POINT('Ctrl Pts',(-0.138422226582637,1.80896640490814,
9.52148872774822));
#44248=CARTESIAN_POINT('Ctrl Pts',(-0.138694075758991,1.80909585833935,
9.52146997088275));
#44249=CARTESIAN_POINT('Ctrl Pts',(-0.139166021526329,1.80932140885519,
9.52143742759432));
#44250=CARTESIAN_POINT('Ctrl Pts',(-0.13936620065474,1.80941733187669,9.5214236303044));
#44251=CARTESIAN_POINT('Ctrl Pts',(-0.139753411835051,1.80960337018746,
9.52139695403305));
#44252=CARTESIAN_POINT('Ctrl Pts',(-0.139940455423047,1.80969345914598,
9.52138407344192));
#44253=CARTESIAN_POINT('Ctrl Pts',(-0.140386897085345,1.80990901809716,
9.52135334238382));
#44254=CARTESIAN_POINT('Ctrl Pts',(-0.140646214732792,1.81003465562684,
9.52133550240228));
#44255=CARTESIAN_POINT('Ctrl Pts',(-0.141571868939122,1.81048466229307,
9.52127185677726));
#44256=CARTESIAN_POINT('Ctrl Pts',(-0.142237261285626,1.81081098504613,
9.52122617198096));
#44257=CARTESIAN_POINT('Ctrl Pts',(-0.1524949885873,1.81588556412855,9.52052282116987));
#44258=CARTESIAN_POINT('Ctrl Pts',(-0.161847251649668,1.82110708807086,
9.51989406040356));
#44259=CARTESIAN_POINT('Ctrl Pts',(-0.180688775895657,1.83289434623079,
9.51861791437396));
#44260=CARTESIAN_POINT('Ctrl Pts',(-0.190120169967184,1.83952311101595,
9.51797355961805));
#44261=CARTESIAN_POINT('Ctrl Pts',(-0.20757322411916,1.85324383430506,9.51673251120817));
#44262=CARTESIAN_POINT('Ctrl Pts',(-0.215636241772114,1.86025794772687,
9.5161365362948));
#44263=CARTESIAN_POINT('Ctrl Pts',(-0.232194561016728,1.87617451830043,
9.5148348278502));
#44264=CARTESIAN_POINT('Ctrl Pts',(-0.240558125970735,1.88518867777577,
9.51412700060318));
#44265=CARTESIAN_POINT('Ctrl Pts',(-0.251935142187424,1.89895054453304,
9.51306720596917));
#44266=CARTESIAN_POINT('Ctrl Pts',(-0.255372020243777,1.90333448473139,
9.51273249672363));
#44267=CARTESIAN_POINT('Ctrl Pts',(-0.259238560149989,1.90853882871748,
9.51233753616644));
#44268=CARTESIAN_POINT('Ctrl Pts',(-0.259780564072263,1.90927488450449,
9.51228173127294));
#44269=CARTESIAN_POINT('Ctrl Pts',(-0.260601899006011,1.91040027569842,
9.51219648760874));
#44270=CARTESIAN_POINT('Ctrl Pts',(-0.260883508380502,1.91078794892528,
9.51216713721252));
#44271=CARTESIAN_POINT('Ctrl Pts',(-0.261371298139543,1.91146261641315,
9.51211608277731));
#44272=CARTESIAN_POINT('Ctrl Pts',(-0.2615778735475,1.91174932518128,9.51209439404199));
#44273=CARTESIAN_POINT('Ctrl Pts',(-0.262007079546186,1.91234709643269,
9.51204918961638));
#44274=CARTESIAN_POINT('Ctrl Pts',(-0.262229628604596,1.91265821654128,
9.51202567083189));
#44275=CARTESIAN_POINT('Ctrl Pts',(-0.262772109619359,1.91341945707909,
9.51196814630246));
#44276=CARTESIAN_POINT('Ctrl Pts',(-0.263091438682812,1.91387000382471,
9.51193411747648));
#44277=CARTESIAN_POINT('Ctrl Pts',(-0.264305427773408,1.91559220730796,
9.51180410815769));
#44278=CARTESIAN_POINT('Ctrl Pts',(-0.265192027464228,1.91686949574299,
9.51170782019642));
#44279=CARTESIAN_POINT('Ctrl Pts',(-0.280043615311895,1.9385996040674,9.51007180700548));
#44280=CARTESIAN_POINT('Ctrl Pts',(-0.291611482455007,1.96058420260175,
9.50843811227095));
#44281=CARTESIAN_POINT('Ctrl Pts',(-0.306297162876582,1.99852606400774,
9.50569119760377));
#44282=CARTESIAN_POINT('Ctrl Pts',(-0.31093782209877,2.01378740786188,9.50460637168407));
#44283=CARTESIAN_POINT('Ctrl Pts',(-0.316270759515971,2.03751506230766,
9.50299628840218));
#44284=CARTESIAN_POINT('Ctrl Pts',(-0.317790333033185,2.04577000387048,
9.50245009064185));
#44285=CARTESIAN_POINT('Ctrl Pts',(-0.319172855946122,2.05537286202421,
9.50183767905432));
#44286=CARTESIAN_POINT('Ctrl Pts',(-0.319351712198856,2.05667128582541,
9.50175535679495));
#44287=CARTESIAN_POINT('Ctrl Pts',(-0.319573287332469,2.05835578749012,
9.50164921420182));
#44288=CARTESIAN_POINT('Ctrl Pts',(-0.319623233285,2.05874087785389,9.50162499366399));
#44289=CARTESIAN_POINT('Ctrl Pts',(-0.31970294684166,2.05936431250664,9.5015858553297));
#44290=CARTESIAN_POINT('Ctrl Pts',(-0.319733144027407,2.05960259997779,
9.5015709132452));
#44291=CARTESIAN_POINT('Ctrl Pts',(-0.319790544045989,2.06005964250263,
9.50154228726918));
#44292=CARTESIAN_POINT('Ctrl Pts',(-0.319817788744533,2.06027839100649,
9.50152860107921));
#44293=CARTESIAN_POINT('Ctrl Pts',(-0.319879922981636,2.06078147679054,
9.50149715861155));
#44294=CARTESIAN_POINT('Ctrl Pts',(-0.319914657957807,2.06106583358114,
9.50147941113791));
#44295=CARTESIAN_POINT('Ctrl Pts',(-0.320021037209972,2.06194645831825,
9.50142452409698));
#44296=CARTESIAN_POINT('Ctrl Pts',(-0.320091394492724,2.06254288482971,
9.50138745699609));
#44297=CARTESIAN_POINT('Ctrl Pts',(-0.320657979770469,2.06746408884773,
9.50108246417541));
#44298=CARTESIAN_POINT('Ctrl Pts',(-0.321068231883772,2.07179857236548,
9.50081926665511));
#44299=CARTESIAN_POINT('Ctrl Pts',(-0.321451662752336,2.07696339077266,
9.50051069023453));
#44300=CARTESIAN_POINT('Ctrl Pts',(-0.321509607149703,2.07778672946825,
9.50046165123315));
#44301=CARTESIAN_POINT('Ctrl Pts',(-0.321573059917299,2.07874065310821,
9.5004050012432));
#44302=CARTESIAN_POINT('Ctrl Pts',(-0.321581652130227,2.07887102207547,
9.50039726272073));
#44303=CARTESIAN_POINT('Ctrl Pts',(-0.321736937581211,2.08124919325417,
9.5002561629741));
#44304=CARTESIAN_POINT('Ctrl Pts',(-0.321860142625702,2.08349852052804,
9.50012377032853));
#44305=CARTESIAN_POINT('Ctrl Pts',(-0.322166486079966,2.09041946011863,
9.49971918120443));
#44306=CARTESIAN_POINT('Ctrl Pts',(-0.322271572270834,2.09509403845348,
9.49944978350821));
#44307=CARTESIAN_POINT('Ctrl Pts',(-0.322295821129269,2.12898474965668,
9.49751447770717));
#44308=CARTESIAN_POINT('Ctrl Pts',(-0.318344304100929,2.15806660197144,
9.49593615930897));
#44309=CARTESIAN_POINT('Ctrl Pts',(-0.308064308479255,2.19509124256648,
9.49369466283714));
#44310=CARTESIAN_POINT('Ctrl Pts',(-0.305221972556378,2.20385319172744,
9.49314742522801));
#44311=CARTESIAN_POINT('Ctrl Pts',(-0.301611485794939,2.21354726856676,
9.49251831265556));
#44312=CARTESIAN_POINT('Ctrl Pts',(-0.301208674467113,2.21461153928012,
9.49244892121089));
#44313=CARTESIAN_POINT('Ctrl Pts',(-0.300614231024252,2.216157342835,9.4923476533104));
#44314=CARTESIAN_POINT('Ctrl Pts',(-0.300427057488376,2.21664059033077,
9.49231592650116));
#44315=CARTESIAN_POINT('Ctrl Pts',(-0.300094580688692,2.2174928745377,9.49225984926668));
#44316=CARTESIAN_POINT('Ctrl Pts',(-0.299949759905136,2.21786209932152,
9.49223551510948));
#44317=CARTESIAN_POINT('Ctrl Pts',(-0.299648848407667,2.21862513529977,
9.49218514218138));
#44318=CARTESIAN_POINT('Ctrl Pts',(-0.299492662128992,2.21901890776298,
9.49215910022779));
#44319=CARTESIAN_POINT('Ctrl Pts',(-0.299090617066218,2.22002672999161,
9.49209232860986));
#44320=CARTESIAN_POINT('Ctrl Pts',(-0.298843644294399,2.22064033066911,
9.49205156139769));
#44321=CARTESIAN_POINT('Ctrl Pts',(-0.29782612466657,2.22314604720145,9.49188461277093));
#44322=CARTESIAN_POINT('Ctrl Pts',(-0.297039496269313,2.22503154330978,
9.49175788796263));
#44323=CARTESIAN_POINT('Ctrl Pts',(-0.291721305874853,2.23744539282073,
9.49091611247471));
#44324=CARTESIAN_POINT('Ctrl Pts',(-0.28664925714373,2.24773187516232,9.4901825900059));
#44325=CARTESIAN_POINT('Ctrl Pts',(-0.265070843387969,2.28618103841534,
9.48729720983177));
#44326=CARTESIAN_POINT('Ctrl Pts',(-0.244875425021176,2.31204127611886,
9.48502216988599));
#44327=CARTESIAN_POINT('Ctrl Pts',(-0.220630198403759,2.33491273083497,
9.48285635970915));
#44328=CARTESIAN_POINT('Ctrl Pts',(-0.220114274394814,2.33539622295301,
9.48281050526657));
#44329=CARTESIAN_POINT('Ctrl Pts',(-0.2195051110752,2.3359633393476,9.48275664122028));
#44330=CARTESIAN_POINT('Ctrl Pts',(-0.219413413235177,2.33604860812297,
9.48274854038928));
#44331=CARTESIAN_POINT('Ctrl Pts',(-0.219140485461509,2.33630210409827,
9.48272445118711));
#44332=CARTESIAN_POINT('Ctrl Pts',(-0.218959111167809,2.33647017656975,
9.48270847147154));
#44333=CARTESIAN_POINT('Ctrl Pts',(-0.215627015577904,2.33955077884497,
9.48241543249333));
#44334=CARTESIAN_POINT('Ctrl Pts',(-0.212418438501883,2.34240048871081,
9.48214194529387));
#44335=CARTESIAN_POINT('Ctrl Pts',(-0.208738697720301,2.34553946582924,
9.48183886514223));
#44336=CARTESIAN_POINT('Ctrl Pts',(-0.208322774560329,2.3458924456251,9.48180475678231));
#44337=CARTESIAN_POINT('Ctrl Pts',(-0.207693158063705,2.3464240355158,9.481753351407));
#44338=CARTESIAN_POINT('Ctrl Pts',(-0.207480128781689,2.34660342525712,
9.48173599763598));
#44339=CARTESIAN_POINT('Ctrl Pts',(-0.20710981411159,2.34691444386232,9.48170589936214));
#44340=CARTESIAN_POINT('Ctrl Pts',(-0.206952635569413,2.34704619875762,
9.48169314557047));
#44341=CARTESIAN_POINT('Ctrl Pts',(-0.206623663824097,2.34732142501102,
9.48166649682518));
#44342=CARTESIAN_POINT('Ctrl Pts',(-0.206451847027919,2.34746486736641,
9.48165260406219));
#44343=CARTESIAN_POINT('Ctrl Pts',(-0.206040567676928,2.34780750011874,
9.48161940930763));
#44344=CARTESIAN_POINT('Ctrl Pts',(-0.205800964678699,2.34800652326703,
9.48160011963735));
#44345=CARTESIAN_POINT('Ctrl Pts',(-0.204987795963277,2.34867998149149,
9.48153481818105));
#44346=CARTESIAN_POINT('Ctrl Pts',(-0.204412869735424,2.34915278124262,
9.48148892499236));
#44347=CARTESIAN_POINT('Ctrl Pts',(-0.203041149594618,2.3502728931802,9.48138006933562));
#44348=CARTESIAN_POINT('Ctrl Pts',(-0.202242885198979,2.35091840295332,
9.48131723257269));
#44349=CARTESIAN_POINT('Ctrl Pts',(-0.192638019970065,2.35860968166988,
9.48056708541994));
#44350=CARTESIAN_POINT('Ctrl Pts',(-0.183469446992151,2.36519312827681,
9.4799102636502));
#44351=CARTESIAN_POINT('Ctrl Pts',(-0.150732574404027,2.38618726204264,
9.47769176539477));
#44352=CARTESIAN_POINT('Ctrl Pts',(-0.125673234436649,2.39804326749506,
9.47619593879675));
#44353=CARTESIAN_POINT('Ctrl Pts',(-0.0969312426862239,2.40736345216879,
9.47444282374195));
#44354=CARTESIAN_POINT('Ctrl Pts',(-0.0944444202053473,2.40813667184715,
9.47429095523788));
#44355=CARTESIAN_POINT('Ctrl Pts',(-0.0903492962067929,2.40935572491413,
9.47404037460777));
#44356=CARTESIAN_POINT('Ctrl Pts',(-0.0887463955885584,2.40981936187511,
9.47394217016029));
#44357=CARTESIAN_POINT('Ctrl Pts',(-0.0809468024205457,2.4120098904307,
9.47346358417667));
#44358=CARTESIAN_POINT('Ctrl Pts',(-0.074703291433907,2.41356333650994,
9.47307820714079));
#44359=CARTESIAN_POINT('Ctrl Pts',(-0.0674116334440075,2.41514743761793,
9.47262405648245));
#44360=CARTESIAN_POINT('Ctrl Pts',(-0.0664044420915283,2.41536119893333,
9.47256123663149));
#44361=CARTESIAN_POINT('Ctrl Pts',(-0.0649038345853793,2.41567217294197,
9.47246750458945));
#44362=CARTESIAN_POINT('Ctrl Pts',(-0.0644111804744379,2.41577306461944,
9.47243671011018));
#44363=CARTESIAN_POINT('Ctrl Pts',(-0.0635329351061396,2.41595078155366,
9.47238177349971));
#44364=CARTESIAN_POINT('Ctrl Pts',(-0.0631474347631856,2.41602805522331,
9.47235764574796));
#44365=CARTESIAN_POINT('Ctrl Pts',(-0.0623352305389417,2.41618931637414,
9.47230678220697));
#44366=CARTESIAN_POINT('Ctrl Pts',(-0.0619084964279216,2.41627314590805,
9.47228004142842));
#44367=CARTESIAN_POINT('Ctrl Pts',(-0.0607826733403173,2.41649194174401,
9.47220944774119));
#44368=CARTESIAN_POINT('Ctrl Pts',(-0.0600833073939316,2.41662545495727,
9.47216554858119));
#44369=CARTESIAN_POINT('Ctrl Pts',(-0.0569319920771485,2.41721624338403,
9.47196752869842));
#44370=CARTESIAN_POINT('Ctrl Pts',(-0.0544752795231656,2.4176473518651,
9.47181257737375));
#44371=CARTESIAN_POINT('Ctrl Pts',(-0.0363047741705893,2.42061895547945,
9.47066198464658));
#44372=CARTESIAN_POINT('Ctrl Pts',(-0.0204293873655689,2.42202027165477,
9.46963010260825));
#44373=CARTESIAN_POINT('Ctrl Pts',(0.0272025572388639,2.42268801173638,
9.46646221583151));
#44374=CARTESIAN_POINT('Ctrl Pts',(0.0588125502753527,2.41844712554706,
9.46424933432333));
#44375=CARTESIAN_POINT('Ctrl Pts',(0.0907872115822737,2.40922690063284,
9.46214358143891));
#44376=CARTESIAN_POINT('Ctrl Pts',(0.0922782957813124,2.40878521697215,
9.46204574514148));
#44377=CARTESIAN_POINT('Ctrl Pts',(0.0941749682043113,2.40820842553216,
9.46192181083258));
#44378=CARTESIAN_POINT('Ctrl Pts',(0.0945835319307011,2.40808329019573,
9.46189514457338));
#44379=CARTESIAN_POINT('Ctrl Pts',(0.0952320866716068,2.40788323841827,
9.46185286438686));
#44380=CARTESIAN_POINT('Ctrl Pts',(0.0954722391649565,2.40780885364235,
9.46183721938858));
#44381=CARTESIAN_POINT('Ctrl Pts',(0.0959206728991603,2.40766938058988,
9.46180802633098));
#44382=CARTESIAN_POINT('Ctrl Pts',(0.0961289735175954,2.40760436227867,
9.46179447432058));
#44383=CARTESIAN_POINT('Ctrl Pts',(0.0965967844523198,2.40745781962584,
9.46176405727718));
#44384=CARTESIAN_POINT('Ctrl Pts',(0.0968562570680768,2.40737617845838,
9.46174719926272));
#44385=CARTESIAN_POINT('Ctrl Pts',(0.0976252456523518,2.40713315139647,
9.46169727519125));
#44386=CARTESIAN_POINT('Ctrl Pts',(0.0981344670417091,2.40697082542735,
9.46166426430943));
#44387=CARTESIAN_POINT('Ctrl Pts',(0.102205811956428,2.40566182485233,9.46140070656974));
#44388=CARTESIAN_POINT('Ctrl Pts',(0.105748305938762,2.40445439382104,9.46117366473429));
#44389=CARTESIAN_POINT('Ctrl Pts',(0.11967302340075,2.39943587488652,9.4602873098731));
#44390=CARTESIAN_POINT('Ctrl Pts',(0.129878047711789,2.39515286808206,9.45965114437382));
#44391=CARTESIAN_POINT('Ctrl Pts',(0.171195680681954,2.37525295759648,9.45705458427353));
#44392=CARTESIAN_POINT('Ctrl Pts',(0.199892245072711,2.35517684228811,9.45517087583014));
#44393=CARTESIAN_POINT('Ctrl Pts',(0.226249860016895,2.32951281873791,9.45294637928287));
#44394=CARTESIAN_POINT('Ctrl Pts',(0.227662262295686,2.32811187425039,9.45282552617872));
#44395=CARTESIAN_POINT('Ctrl Pts',(0.229539581208921,2.32621498191669,9.4526626165103));
#44396=CARTESIAN_POINT('Ctrl Pts',(0.230016050974719,2.32573048900844,9.45262106975628));
#44397=CARTESIAN_POINT('Ctrl Pts',(0.230759977926259,2.32496923420806,9.45255588597263));
#44398=CARTESIAN_POINT('Ctrl Pts',(0.231028479608154,2.32469349202982,9.45253229469513));
#44399=CARTESIAN_POINT('Ctrl Pts',(0.231564054188112,2.32414150011792,9.4524851075071));
#44400=CARTESIAN_POINT('Ctrl Pts',(0.231831128280468,2.32386525238491,9.45246151170434));
#44401=CARTESIAN_POINT('Ctrl Pts',(0.232430285327008,2.32324329303226,9.45240842974875));
#44402=CARTESIAN_POINT('Ctrl Pts',(0.232762091715507,2.32289731733995,9.45237893166911));
#44403=CARTESIAN_POINT('Ctrl Pts',(0.233451818763828,2.32217491699996,9.45231740043061));
#44404=CARTESIAN_POINT('Ctrl Pts',(0.233809603517261,2.32179836502128,9.45228536151397));
#44405=CARTESIAN_POINT('Ctrl Pts',(0.234736613914386,2.32081799367317,9.45220203451745));
#44406=CARTESIAN_POINT('Ctrl Pts',(0.235304417832037,2.32021284061087,9.45215068546844));
#44407=CARTESIAN_POINT('Ctrl Pts',(0.236965523145545,2.31842871093038,9.4519995444195));
#44408=CARTESIAN_POINT('Ctrl Pts',(0.238052333787264,2.31724375053362,9.45189947679271));
#44409=CARTESIAN_POINT('Ctrl Pts',(0.249396074304328,2.30468822158,9.45084238320692));
#44410=CARTESIAN_POINT('Ctrl Pts',(0.258837504200833,2.29261021409117,9.44985140995903));
#44411=CARTESIAN_POINT('Ctrl Pts',(0.285522077972278,2.25295104040815,9.44667864838775));
#44412=CARTESIAN_POINT('Ctrl Pts',(0.29947837682563,2.22340780757839,9.44440858188591));
#44413=CARTESIAN_POINT('Ctrl Pts',(0.309204540203415,2.19086204917898,9.44226061495914));
#44414=CARTESIAN_POINT('Ctrl Pts',(0.309617962356751,2.18944315092948,9.44216767718748));
#44415=CARTESIAN_POINT('Ctrl Pts',(0.310137437759879,2.18761349864264,9.44204878843287));
#44416=CARTESIAN_POINT('Ctrl Pts',(0.310252452458795,2.18720533924523,9.442022327564));
#44417=CARTESIAN_POINT('Ctrl Pts',(0.310433506412475,2.1865579304315,9.44198045398585));
#44418=CARTESIAN_POINT('Ctrl Pts',(0.310500074964,2.18631883150551,9.441965010486));
#44419=CARTESIAN_POINT('Ctrl Pts',(0.310618916401937,2.18589006406086,9.44193735435746));
#44420=CARTESIAN_POINT('Ctrl Pts',(0.310671291433447,2.18570042596438,9.44192513581439));
#44421=CARTESIAN_POINT('Ctrl Pts',(0.310794090368684,2.18525420698839,9.44189641693779));
#44422=CARTESIAN_POINT('Ctrl Pts',(0.31086437009975,2.18499758714826,9.441879925123));
#44423=CARTESIAN_POINT('Ctrl Pts',(0.311067396475096,2.18425263535107,9.44183212028819));
#44424=CARTESIAN_POINT('Ctrl Pts',(0.311199311587595,2.1837640745729,9.44180085560973));
#44425=CARTESIAN_POINT('Ctrl Pts',(0.312108478272817,2.18036509228744,9.44158393535985));
#44426=CARTESIAN_POINT('Ctrl Pts',(0.312846073117789,2.17744408551942,9.44140053565276));
#44427=CARTESIAN_POINT('Ctrl Pts',(0.315015877146681,2.16831379012124,9.44083541508428));
#44428=CARTESIAN_POINT('Ctrl Pts',(0.316305046895793,2.16207177501105,9.44046070360992));
#44429=CARTESIAN_POINT('Ctrl Pts',(0.32014164373459,2.14024611150429,9.43917796551637));
#44430=CARTESIAN_POINT('Ctrl Pts',(0.321728838115565,2.1245161456337,9.43830088263462));
#44431=CARTESIAN_POINT('Ctrl Pts',(0.322836863474844,2.0836385463757,9.43601427327013));
#44432=CARTESIAN_POINT('Ctrl Pts',(0.320582960966283,2.05855550003987,9.43459728529053));
#44433=CARTESIAN_POINT('Ctrl Pts',(0.315137863248776,2.03253511113195,9.43298470670581));
#44434=CARTESIAN_POINT('Ctrl Pts',(0.314823420287229,2.03108267266997,9.43289424516316));
#44435=CARTESIAN_POINT('Ctrl Pts',(0.314380636435146,2.02910370489382,9.43277036029786));
#44436=CARTESIAN_POINT('Ctrl Pts',(0.314260993004996,2.02857523192192,9.43273721605986));
#44437=CARTESIAN_POINT('Ctrl Pts',(0.314055254382719,2.02767699566307,9.4326807759214));
#44438=CARTESIAN_POINT('Ctrl Pts',(0.31396983723826,2.02730707693113,9.4326575018391));
#44439=CARTESIAN_POINT('Ctrl Pts',(0.313796419068784,2.026562057151,9.43261056586485));
#44440=CARTESIAN_POINT('Ctrl Pts',(0.313708398646986,2.02618696126954,9.43258690338136));
#44441=CARTESIAN_POINT('Ctrl Pts',(0.313506802792778,2.02533474185148,9.43253306990223));
#44442=CARTESIAN_POINT('Ctrl Pts',(0.313392810608187,2.02485771878232,9.43250288553058));
#44443=CARTESIAN_POINT('Ctrl Pts',(0.313152120291901,2.02386057684683,9.43243968130829));
#44444=CARTESIAN_POINT('Ctrl Pts',(0.313025214333634,2.02334051012926,9.432406654827));
#44445=CARTESIAN_POINT('Ctrl Pts',(0.312689207684199,2.02197828521762,9.43231998431469));
#44446=CARTESIAN_POINT('Ctrl Pts',(0.312478001501209,2.02113665532107,9.4322662723923));
#44447=CARTESIAN_POINT('Ctrl Pts',(0.311840726480372,2.01863994996806,9.43210644315864));
#44448=CARTESIAN_POINT('Ctrl Pts',(0.311404893538419,2.01698741943461,9.4320000109115));
#44449=CARTESIAN_POINT('Ctrl Pts',(0.306470169119154,1.99886252035095,9.43082545468942));
#44450=CARTESIAN_POINT('Ctrl Pts',(0.300682810569195,1.98277186472956,9.42971485070911));
#44451=CARTESIAN_POINT('Ctrl Pts',(0.282008898053794,1.94147443563514,9.42669058196201));
#44452=CARTESIAN_POINT('Ctrl Pts',(0.267034512776537,1.9173748725589,9.42473230165862));
#44453=CARTESIAN_POINT('Ctrl Pts',(0.246891477914125,1.89283339157701,9.42269284799245));
#44454=CARTESIAN_POINT('Ctrl Pts',(0.244628802431751,1.8901663587424,9.42247072202866));
#44455=CARTESIAN_POINT('Ctrl Pts',(0.241946991163536,1.88710764580198,9.42221592976329));
#44456=CARTESIAN_POINT('Ctrl Pts',(0.241569790856374,1.88667973099932,9.42218028324992));
#44457=CARTESIAN_POINT('Ctrl Pts',(0.24100619053917,1.88604376669373,9.42212730714452));
#44458=CARTESIAN_POINT('Ctrl Pts',(0.240820655556383,1.88583495731651,9.42210991347727));
#44459=CARTESIAN_POINT('Ctrl Pts',(0.240489250025858,1.8854629538826,9.42207892672944));
#44460=CARTESIAN_POINT('Ctrl Pts',(0.240343484819296,1.88529966734829,9.42206532577764));
#44461=CARTESIAN_POINT('Ctrl Pts',(0.240033176057989,1.8849527707626,9.42203643180461));
#44462=CARTESIAN_POINT('Ctrl Pts',(0.239868588604526,1.88476920152307,9.42202114223114));
#44463=CARTESIAN_POINT('Ctrl Pts',(0.239425264635291,1.88427588935616,9.42198005455102));
#44464=CARTESIAN_POINT('Ctrl Pts',(0.239146136577251,1.88396649652528,9.4219542859741));
#44465=CARTESIAN_POINT('Ctrl Pts',(0.237793620473765,1.88247316591569,9.42182990782071));
#44466=CARTESIAN_POINT('Ctrl Pts',(0.236712012123557,1.88129665514977,9.42173191036822));
#44467=CARTESIAN_POINT('Ctrl Pts',(0.227529407989373,1.87145628166384,9.42091170271394));
#44468=CARTESIAN_POINT('Ctrl Pts',(0.218963554547288,1.86323663352581,9.42022281539558));
#44469=CARTESIAN_POINT('Ctrl Pts',(0.198821073362664,1.84593888250069,9.41871180233112));
#44470=CARTESIAN_POINT('Ctrl Pts',(0.18703781605683,1.83714309216627,9.41789830998348));
#44471=CARTESIAN_POINT('Ctrl Pts',(0.155778876424557,1.81697906378041,9.41581277989258));
#44472=CARTESIAN_POINT('Ctrl Pts',(0.135639229480557,1.80679412843478,9.41452914505569));
#44473=CARTESIAN_POINT('Ctrl Pts',(0.11336835377941,1.79832046546932,9.4130821316533));
#44474=CARTESIAN_POINT('Ctrl Pts',(0.112129232337921,1.79785771502958,9.41300155739414));
#44475=CARTESIAN_POINT('Ctrl Pts',(0.110403131216121,1.79722518243057,9.41288921601863));
#44476=CARTESIAN_POINT('Ctrl Pts',(0.109918527972368,1.79704891691886,9.41285766513238));
#44477=CARTESIAN_POINT('Ctrl Pts',(0.109083057406742,1.79674729839173,9.41280325068625));
#44478=CARTESIAN_POINT('Ctrl Pts',(0.108732390868532,1.79662138898722,9.41278040568436));
#44479=CARTESIAN_POINT('Ctrl Pts',(0.108015550749706,1.79636540476403,9.41273369287286));
#44480=CARTESIAN_POINT('Ctrl Pts',(0.107649358753522,1.79623538358497,9.41270982332368));
#44481=CARTESIAN_POINT('Ctrl Pts',(0.106800564826833,1.79593573597684,9.41265448035606));
#44482=CARTESIAN_POINT('Ctrl Pts',(0.106317793387263,1.79576659600279,9.41262299085588));
#44483=CARTESIAN_POINT('Ctrl Pts',(0.105301927956455,1.79541339875124,9.41255670367256));
#44484=CARTESIAN_POINT('Ctrl Pts',(0.104768749897887,1.79522959013385,9.41252189785917));
#44485=CARTESIAN_POINT('Ctrl Pts',(0.103349038450332,1.79474432241685,9.4124291782461));
#44486=CARTESIAN_POINT('Ctrl Pts',(0.102461673952023,1.79444532766363,9.41237118311513));
#44487=CARTESIAN_POINT('Ctrl Pts',(0.0997739715087234,1.79355273895656,
9.4121953894337));
#44488=CARTESIAN_POINT('Ctrl Pts',(0.0979697118153263,1.79297116664532,
9.41207719644391));
#44489=CARTESIAN_POINT('Ctrl Pts',(0.0914725549219662,1.79094001950794,
9.41165087742117));
#44490=CARTESIAN_POINT('Ctrl Pts',(0.0867519833413467,1.78958191260499,
9.41133980380581));
#44491=CARTESIAN_POINT('Ctrl Pts',(0.0706636807584968,1.78534894397187,
9.4102747460098));
#44492=CARTESIAN_POINT('Ctrl Pts',(0.0591717367956374,1.78298691096113,
9.40950539815993));
#44493=CARTESIAN_POINT('Ctrl Pts',(0.0203670840984569,1.77719468697395,
9.40688799931844));
#44494=CARTESIAN_POINT('Ctrl Pts',(-0.00725039676497182,1.77663410797581,
9.40498327120166));
#44495=CARTESIAN_POINT('Ctrl Pts',(-0.0388485923793428,1.78004656984481,
9.40293121428378));
#44496=CARTESIAN_POINT('Ctrl Pts',(-0.0430848778315068,1.7805894361636,
9.40265905336652));
#44497=CARTESIAN_POINT('Ctrl Pts',(-0.0478482432475965,1.78129634764236,
9.40235730253564));
#44498=CARTESIAN_POINT('Ctrl Pts',(-0.0483869203337208,1.78137768697267,
9.40232324016933));
#44499=CARTESIAN_POINT('Ctrl Pts',(-0.0492004781585769,1.78150264360463,
9.40227189236619));
#44500=CARTESIAN_POINT('Ctrl Pts',(-0.049475509518873,1.78154525118762,
9.402254550351));
#44501=CARTESIAN_POINT('Ctrl Pts',(-0.049953076272882,1.78161986896095,
9.40222446681752));
#44502=CARTESIAN_POINT('Ctrl Pts',(-0.0501556363613433,1.78165171617976,
9.40221171603243));
#44503=CARTESIAN_POINT('Ctrl Pts',(-0.0505792805874181,1.78171873741091,
9.40218506775862));
#44504=CARTESIAN_POINT('Ctrl Pts',(-0.0508003583534382,1.78175394844311,
9.40217117247011));
#44505=CARTESIAN_POINT('Ctrl Pts',(-0.051329168524085,1.78183873705242,
9.40213796151166));
#44506=CARTESIAN_POINT('Ctrl Pts',(-0.0516368671089207,1.78188853095353,
9.40211865819435));
#44507=CARTESIAN_POINT('Ctrl Pts',(-0.052680400242128,1.78205895663339,
9.40205326288432));
#44508=CARTESIAN_POINT('Ctrl Pts',(-0.0534158952564986,1.78218169689788,
9.40200728995333));
#44509=CARTESIAN_POINT('Ctrl Pts',(-0.0551651785955241,1.78247986330419,
9.40189821700345));
#44510=CARTESIAN_POINT('Ctrl Pts',(-0.0561785729207752,1.7826575947867,
9.40183524336065));
#44511=CARTESIAN_POINT('Ctrl Pts',(-0.0683362612767503,1.78484990193908,
9.4010821379189));
#44512=CARTESIAN_POINT('Ctrl Pts',(-0.0793690778292553,1.78744594371111,
9.40042274331321));
#44513=CARTESIAN_POINT('Ctrl Pts',(-0.103783857631236,1.79456747285531,
9.39897224442632));
#44514=CARTESIAN_POINT('Ctrl Pts',(-0.117050853462566,1.79940185488798,
9.3981896980009));
#44515=CARTESIAN_POINT('Ctrl Pts',(-0.137175496261895,1.80827024032479,
9.39695840127328));
#44516=CARTESIAN_POINT('Ctrl Pts',(-0.144272810896659,1.81171417062702,
9.39651517237573));
#44517=CARTESIAN_POINT('Ctrl Pts',(-0.165247437901682,1.82286067219054,
9.3951635210907));
#44518=CARTESIAN_POINT('Ctrl Pts',(-0.178687505393542,1.83132995710408,
9.39423895899712));
#44519=CARTESIAN_POINT('Ctrl Pts',(-0.192461086576651,1.84150146812387,
9.39319873037454));
#44520=CARTESIAN_POINT('Ctrl Pts',(-0.193469495165107,1.84225532944671,
9.39312201184949));
#44521=CARTESIAN_POINT('Ctrl Pts',(-0.194876037157026,1.84331973067511,
9.3930142056253));
#44522=CARTESIAN_POINT('Ctrl Pts',(-0.195277906669753,1.8436253333872,9.39298331180776));
#44523=CARTESIAN_POINT('Ctrl Pts',(-0.195972859486507,1.8441563940636,9.39292972670439));
#44524=CARTESIAN_POINT('Ctrl Pts',(-0.196266276760142,1.84438141507566,
9.39290705267579));
#44525=CARTESIAN_POINT('Ctrl Pts',(-0.196855658686899,1.84483502372851,
9.39286140721108));
#44526=CARTESIAN_POINT('Ctrl Pts',(-0.197151614027167,1.84506362253037,
9.3928384353536));
#44527=CARTESIAN_POINT('Ctrl Pts',(-0.197851824429519,1.84560642040599,
9.39278396362928));
#44528=CARTESIAN_POINT('Ctrl Pts',(-0.198255729033612,1.84592106803343,
9.39275244598307));
#44529=CARTESIAN_POINT('Ctrl Pts',(-0.199513056502274,1.84690536813841,
9.39265403079365));
#44530=CARTESIAN_POINT('Ctrl Pts',(-0.200363842529508,1.84757836274847,
9.39258700010511));
#44531=CARTESIAN_POINT('Ctrl Pts',(-0.20232268092819,1.84914399951926,9.39243164766579));
#44532=CARTESIAN_POINT('Ctrl Pts',(-0.20342824541422,1.85003970503628,9.39234320338943));
#44533=CARTESIAN_POINT('Ctrl Pts',(-0.207105321188201,1.85305934868658,
9.39204645057628));
#44534=CARTESIAN_POINT('Ctrl Pts',(-0.209649719550282,1.85521582345928,
9.39183682780877));
#44535=CARTESIAN_POINT('Ctrl Pts',(-0.218631762472412,1.86307122461314,
9.39108111120357));
#44536=CARTESIAN_POINT('Ctrl Pts',(-0.224873807262726,1.86898735664733,
9.39052620619662));
#44537=CARTESIAN_POINT('Ctrl Pts',(-0.255963669111777,1.90090916743503,
9.38760383345891));
#44538=CARTESIAN_POINT('Ctrl Pts',(-0.276562679716115,1.93068619127209,
9.38507499716765));
#44539=CARTESIAN_POINT('Ctrl Pts',(-0.292548375144975,1.96479806122941,
9.38268785766659));
#44540=CARTESIAN_POINT('Ctrl Pts',(-0.293263636606715,1.96635660959003,
9.38257987957437));
#44541=CARTESIAN_POINT('Ctrl Pts',(-0.294148086025407,1.9683251142008,9.38244493308368));
#44542=CARTESIAN_POINT('Ctrl Pts',(-0.294328896721643,1.96872977251922,
9.38241726846352));
#44543=CARTESIAN_POINT('Ctrl Pts',(-0.294612465115776,1.96936793615425,
9.38237376104588));
#44544=CARTESIAN_POINT('Ctrl Pts',(-0.294715780474092,1.96960119077682,
9.38235788408284));
#44545=CARTESIAN_POINT('Ctrl Pts',(-0.294906837521714,1.97003392635536,
9.38232847643265));
#44546=CARTESIAN_POINT('Ctrl Pts',(-0.29499465325763,1.97023337229626,9.3823149412552));
#44547=CARTESIAN_POINT('Ctrl Pts',(-0.295189713156472,1.9706776110057,9.38228483496318));
#44548=CARTESIAN_POINT('Ctrl Pts',(-0.29529685487223,1.97092244752706,9.3822682702251));
#44549=CARTESIAN_POINT('Ctrl Pts',(-0.295608231753307,1.9716364119531,9.38222004667172));
#44550=CARTESIAN_POINT('Ctrl Pts',(-0.295811655621786,1.97210589605688,
9.38218843751308));
#44551=CARTESIAN_POINT('Ctrl Pts',(-0.297255906498752,1.97546097811683,
9.38196325766307));
#44552=CARTESIAN_POINT('Ctrl Pts',(-0.29845566091156,1.97836422330409,9.38177214325877));
#44553=CARTESIAN_POINT('Ctrl Pts',(-0.301100466440746,1.98503916327875,
9.38134022383136));
#44554=CARTESIAN_POINT('Ctrl Pts',(-0.30251747062057,1.9888214594421,9.38110085470681));
#44555=CARTESIAN_POINT('Ctrl Pts',(-0.316034006210467,2.02707385082697,
9.37872416390739));
#44556=CARTESIAN_POINT('Ctrl Pts',(-0.322260403908793,2.06333603087332,
9.37679719750188));
#44557=CARTESIAN_POINT('Ctrl Pts',(-0.322274974372014,2.0998714756124,9.37464719300612));
#44558=CARTESIAN_POINT('',(-0.322274999740166,2.09998705874836,9.12407167227341));
#44559=CARTESIAN_POINT('Ctrl Pts',(-0.322274974505127,2.09987180983054,
9.37464717333835));
#44560=CARTESIAN_POINT('Ctrl Pts',(-0.322277110580648,2.10524198514739,
9.37433115401095));
#44561=CARTESIAN_POINT('Ctrl Pts',(-0.322145019382397,2.11061118994016,
9.37401147726832));
#44562=CARTESIAN_POINT('Ctrl Pts',(-0.321766823267488,2.11823169941662,
9.37355134390472));
#44563=CARTESIAN_POINT('Ctrl Pts',(-0.32163105895509,2.12048767760956,9.37341432817286));
#44564=CARTESIAN_POINT('Ctrl Pts',(-0.321429283593712,2.12333989158731,
9.3732400323371));
#44565=CARTESIAN_POINT('Ctrl Pts',(-0.321385318859788,2.12393766289022,
9.37320344377587));
#44566=CARTESIAN_POINT('Ctrl Pts',(-0.321307485198678,2.12495705288305,
9.37314094605633));
#44567=CARTESIAN_POINT('Ctrl Pts',(-0.32127445325989,2.12537873545261,9.37311506318493));
#44568=CARTESIAN_POINT('Ctrl Pts',(-0.321211268653396,2.12616544804394,
9.37306671838576));
#44569=CARTESIAN_POINT('Ctrl Pts',(-0.32118132362295,2.12653049444167,9.37304426301192));
#44570=CARTESIAN_POINT('Ctrl Pts',(-0.321119286425513,2.12727126155572,
9.37299864931778));
#44571=CARTESIAN_POINT('Ctrl Pts',(-0.321087157013343,2.12764697850471,
9.37297548986086));
#44572=CARTESIAN_POINT('Ctrl Pts',(-0.321010827792065,2.12852147971539,
9.37292152825814));
#44573=CARTESIAN_POINT('Ctrl Pts',(-0.320966124852631,2.12902021808112,
9.37289071033703));
#44574=CARTESIAN_POINT('Ctrl Pts',(-0.320830008504175,2.1305000351093,9.37279914113781));
#44575=CARTESIAN_POINT('Ctrl Pts',(-0.320735258514318,2.13148079429874,
9.37273828502976));
#44576=CARTESIAN_POINT('Ctrl Pts',(-0.320052229261279,2.13822744832209,
9.37231848046731));
#44577=CARTESIAN_POINT('Ctrl Pts',(-0.31931303157068,2.14397667660772,9.37195480216073));
#44578=CARTESIAN_POINT('Ctrl Pts',(-0.318078404834808,2.15188630773486,
9.37144578736919));
#44579=CARTESIAN_POINT('Ctrl Pts',(-0.317715092194272,2.1540664439802,9.37130457379153));
#44580=CARTESIAN_POINT('Ctrl Pts',(-0.312059811832663,2.18597438814035,
9.36922432788522));
#44581=CARTESIAN_POINT('Ctrl Pts',(-0.302638045776677,2.2148150632461,9.36715138662394));
#44582=CARTESIAN_POINT('Ctrl Pts',(-0.285505590720188,2.24974577066783,
9.36454693329608));
#44583=CARTESIAN_POINT('Ctrl Pts',(-0.28134849063823,2.257417562983,9.36397002176843));
#44584=CARTESIAN_POINT('Ctrl Pts',(-0.274805698362227,2.26840283375879,
9.36314598112024));
#44585=CARTESIAN_POINT('Ctrl Pts',(-0.27266048537398,2.27185444367139,9.36288739037192));
#44586=CARTESIAN_POINT('Ctrl Pts',(-0.270154175255612,2.27572192236349,
9.36259882847387));
#44587=CARTESIAN_POINT('Ctrl Pts',(-0.269856744492273,2.27617834676693,
9.3625647926083));
#44588=CARTESIAN_POINT('Ctrl Pts',(-0.269407906376958,2.27686331093874,
9.36251374573381));
#44589=CARTESIAN_POINT('Ctrl Pts',(-0.26925736435615,2.27709241236131,9.36249667726692));
#44590=CARTESIAN_POINT('Ctrl Pts',(-0.268987466069528,2.27750201561849,
9.36246617096688));
#44591=CARTESIAN_POINT('Ctrl Pts',(-0.268868220545551,2.27768258899724,
9.36245272574479));
#44592=CARTESIAN_POINT('Ctrl Pts',(-0.268611264692764,2.27807084601557,
9.36242382424172));
#44593=CARTESIAN_POINT('Ctrl Pts',(-0.268473495734878,2.27827848947489,
9.36240837204354));
#44594=CARTESIAN_POINT('Ctrl Pts',(-0.268098152532454,2.2788427797568,9.36236639116611));
#44595=CARTESIAN_POINT('Ctrl Pts',(-0.267860106484653,2.27919911445519,
9.36233989427731));
#44596=CARTESIAN_POINT('Ctrl Pts',(-0.266775050728669,2.28081635777428,
9.3622196905617));
#44597=CARTESIAN_POINT('Ctrl Pts',(-0.265919825825667,2.28207176984814,
9.36212652928844));
#44598=CARTESIAN_POINT('Ctrl Pts',(-0.248693577698076,2.3069784252738,9.36028023902983));
#44599=CARTESIAN_POINT('Ctrl Pts',(-0.229234814593436,2.32834312362855,
9.35872408386193));
#44600=CARTESIAN_POINT('Ctrl Pts',(-0.19892321500865,2.35378604271672,9.35649757473676));
#44601=CARTESIAN_POINT('Ctrl Pts',(-0.190308300502816,2.36030852413816,
9.35588378359829));
#44602=CARTESIAN_POINT('Ctrl Pts',(-0.175806441413843,2.37018286786351,
9.35486312597605));
#44603=CARTESIAN_POINT('Ctrl Pts',(-0.170112634274441,2.37380352318409,
9.3544653750954));
#44604=CARTESIAN_POINT('Ctrl Pts',(-0.162248670009259,2.37846415295899,
9.35391757488902));
#44605=CARTESIAN_POINT('Ctrl Pts',(-0.160174142676971,2.3796625805373,9.35377321167319));
#44606=CARTESIAN_POINT('Ctrl Pts',(-0.157116423128887,2.3813838026871,9.35356055561746));
#44607=CARTESIAN_POINT('Ctrl Pts',(-0.156143545275065,2.38192482695242,
9.35349291322107));
#44608=CARTESIAN_POINT('Ctrl Pts',(-0.15438896528472,2.38288869339273,9.35337094434498));
#44609=CARTESIAN_POINT('Ctrl Pts',(-0.153608276845747,2.38331336486435,
9.35331668355144));
#44610=CARTESIAN_POINT('Ctrl Pts',(-0.152410915075227,2.3839582904387,9.35323347146609));
#44611=CARTESIAN_POINT('Ctrl Pts',(-0.151995494242797,2.38418087104711,
9.35320460296736));
#44612=CARTESIAN_POINT('Ctrl Pts',(-0.151236680990402,2.38458529992811,
9.35315187378738));
#44613=CARTESIAN_POINT('Ctrl Pts',(-0.15089344452434,2.38476744022029,9.35312802352166));
#44614=CARTESIAN_POINT('Ctrl Pts',(-0.150204743916452,2.38513130817347,
9.35308016961704));
#44615=CARTESIAN_POINT('Ctrl Pts',(-0.149859277337966,2.38531302982753,
9.35305616581531));
#44616=CARTESIAN_POINT('Ctrl Pts',(-0.148887392592978,2.38582200658525,
9.35298863855252));
#44617=CARTESIAN_POINT('Ctrl Pts',(-0.148260229683678,2.38614782788444,
9.35294506455187));
#44618=CARTESIAN_POINT('Ctrl Pts',(-0.145683615575148,2.38747567584247,
9.35276604959449));
#44619=CARTESIAN_POINT('Ctrl Pts',(-0.143725073987598,2.38845984603363,
9.35262998268297));
#44620=CARTESIAN_POINT('Ctrl Pts',(-0.124864338201729,2.39769762829194,
9.351319475839));
#44621=CARTESIAN_POINT('Ctrl Pts',(-0.107283152810747,2.40447509752426,
9.35009318879919));
#44622=CARTESIAN_POINT('Ctrl Pts',(-0.0816840372893737,2.41184980761404,
9.34831004619962));
#44623=CARTESIAN_POINT('Ctrl Pts',(-0.0740774855128724,2.41374369200601,
9.34778096715786));
#44624=CARTESIAN_POINT('Ctrl Pts',(-0.0640304026676524,2.41585945479017,
9.3470863270942));
#44625=CARTESIAN_POINT('Ctrl Pts',(-0.0616455279271145,2.41633355263805,
9.34692175412797));
#44626=CARTESIAN_POINT('Ctrl Pts',(-0.0511467547938183,2.41829740461938,
9.34619905433089));
#44627=CARTESIAN_POINT('Ctrl Pts',(-0.0429825161552331,2.41950233027117,
9.34564164454891));
#44628=CARTESIAN_POINT('Ctrl Pts',(-0.0232151527736135,2.42164821456,9.34431378262442));
#44629=CARTESIAN_POINT('Ctrl Pts',(-0.0115884289626762,2.42227673387109,
9.34355053978316));
#44630=CARTESIAN_POINT('Ctrl Pts',(0.000796610408746042,2.42227488464974,
9.34277315938522));
#44631=CARTESIAN_POINT('Ctrl Pts',(0.00154510788851761,2.42227216530802,
9.34272631735025));
#44632=CARTESIAN_POINT('Ctrl Pts',(0.00260577185346212,2.42226461648085,
9.34266014356296));
#44633=CARTESIAN_POINT('Ctrl Pts',(0.00291794397415571,2.42226194110915,
9.34264069250031));
#44634=CARTESIAN_POINT('Ctrl Pts',(0.0034540551022078,2.42225656747896,
9.34260733166719));
#44635=CARTESIAN_POINT('Ctrl Pts',(0.00367799566596483,2.42225408939062,
9.34259340948123));
#44636=CARTESIAN_POINT('Ctrl Pts',(0.00410686413504136,2.42224889649799,
9.34256677235448));
#44637=CARTESIAN_POINT('Ctrl Pts',(0.00431179173556544,2.4222462196517,
9.34255405527032));
#44638=CARTESIAN_POINT('Ctrl Pts',(0.00479459484181479,2.42223945245172,
9.34252411988373));
#44639=CARTESIAN_POINT('Ctrl Pts',(0.00507246841567341,2.42223519814198,
9.34250691083999));
#44640=CARTESIAN_POINT('Ctrl Pts',(0.00589345896592658,2.42222156636208,
9.34245612419612));
#44641=CARTESIAN_POINT('Ctrl Pts',(0.00643656157367349,2.42221117512068,
9.34242260312503));
#44642=CARTESIAN_POINT('Ctrl Pts',(0.0112052167570492,2.42210787419832,
9.34212891647229));
#44643=CARTESIAN_POINT('Ctrl Pts',(0.0154288322364225,2.42193321483216,
9.34187322029529));
#44644=CARTESIAN_POINT('Ctrl Pts',(0.0202676568975475,2.42163765805283,
9.34158411188367));
#44645=CARTESIAN_POINT('Ctrl Pts',(0.0208871768760164,2.42159802058992,
9.34154716917964));
#44646=CARTESIAN_POINT('Ctrl Pts',(0.0489588843387423,2.4197205081397,9.33987633651391));
#44647=CARTESIAN_POINT('Ctrl Pts',(0.0760663184928047,2.41437635317203,
9.33838983614043));
#44648=CARTESIAN_POINT('Ctrl Pts',(0.114438766109626,2.40154991075901,9.33610151151518));
#44649=CARTESIAN_POINT('Ctrl Pts',(0.126450573644565,2.39671329976524,9.33535792026808));
#44650=CARTESIAN_POINT('Ctrl Pts',(0.141530119954209,2.38955913625974,9.33436793047283));
#44651=CARTESIAN_POINT('Ctrl Pts',(0.144893302184801,2.38789094720827,9.33414339686622));
#44652=CARTESIAN_POINT('Ctrl Pts',(0.149605849919691,2.38544995787496,9.33382308503411));
#44653=CARTESIAN_POINT('Ctrl Pts',(0.150980020050386,2.38472552080329,9.33372898780577));
#44654=CARTESIAN_POINT('Ctrl Pts',(0.153061967409586,2.38360864688341,9.33358534115381));
#44655=CARTESIAN_POINT('Ctrl Pts',(0.153773605586826,2.38322342533855,9.3335360466421));
#44656=CARTESIAN_POINT('Ctrl Pts',(0.155084858688188,2.38250722346743,9.33344485464043));
#44657=CARTESIAN_POINT('Ctrl Pts',(0.155684885256794,2.3821770033096,9.33340298436084));
#44658=CARTESIAN_POINT('Ctrl Pts',(0.156655845992829,2.38163860259175,9.33333499924708));
#44659=CARTESIAN_POINT('Ctrl Pts',(0.157027430821572,2.38143159474443,9.333308926464));
#44660=CARTESIAN_POINT('Ctrl Pts',(0.157724586886115,2.38104140241247,9.33325990560218));
#44661=CARTESIAN_POINT('Ctrl Pts',(0.158050251863029,2.38085838613531,9.33323696359633));
#44662=CARTESIAN_POINT('Ctrl Pts',(0.158805913695828,2.38043199092002,9.33318363006048));
#44663=CARTESIAN_POINT('Ctrl Pts',(0.159235669688544,2.38018818899204,9.33315322333217));
#44664=CARTESIAN_POINT('Ctrl Pts',(0.160334974294744,2.37956120397614,9.33307525002431));
#44665=CARTESIAN_POINT('Ctrl Pts',(0.161003707975213,2.3791766049517,9.33302763237335));
#44666=CARTESIAN_POINT('Ctrl Pts',(0.164834904872025,2.37695488075905,9.33275376002236));
#44667=CARTESIAN_POINT('Ctrl Pts',(0.167967188033252,2.3750664897984,9.33252564966688));
#44668=CARTESIAN_POINT('Ctrl Pts',(0.199581485798853,2.3552655055645,9.3301790117144));
#44669=CARTESIAN_POINT('Ctrl Pts',(0.225118985712258,2.33305278134016,9.32787946287751));
#44670=CARTESIAN_POINT('Ctrl Pts',(0.249727178731369,2.30376189741836,9.32531120635085));
#44671=CARTESIAN_POINT('Ctrl Pts',(0.252626290725504,2.30015627534537,9.32500230544863));
#44672=CARTESIAN_POINT('Ctrl Pts',(0.259330263326419,2.29144074724498,9.32427466300522));
#44673=CARTESIAN_POINT('Ctrl Pts',(0.263063425431226,2.28627772485283,9.32385853116391));
#44674=CARTESIAN_POINT('Ctrl Pts',(0.268329168608988,2.27852076498167,9.32325863793406));
#44675=CARTESIAN_POINT('Ctrl Pts',(0.269982212895564,2.27601083083979,9.32306828179713));
#44676=CARTESIAN_POINT('Ctrl Pts',(0.27187220484289,2.27305182927692,9.3228485522375));
#44677=CARTESIAN_POINT('Ctrl Pts',(0.272143430851037,2.27262498207136,9.32281696794774));
#44678=CARTESIAN_POINT('Ctrl Pts',(0.272555781322148,2.2719726502916,9.32276887269659));
#44679=CARTESIAN_POINT('Ctrl Pts',(0.272697631673513,2.27174762898313,9.32275231370925));
#44680=CARTESIAN_POINT('Ctrl Pts',(0.272954070473797,2.27133971406746,9.32272235311133));
#44681=CARTESIAN_POINT('Ctrl Pts',(0.273068753353805,2.27115688168319,9.32270894523208));
#44682=CARTESIAN_POINT('Ctrl Pts',(0.273300901565202,2.2707859537716,9.32268178570573));
#44683=CARTESIAN_POINT('Ctrl Pts',(0.273418355906973,2.27059785302247,9.32266803479882));
#44684=CARTESIAN_POINT('Ctrl Pts',(0.273755482682205,2.27005670883943,9.3226285375639));
#44685=CARTESIAN_POINT('Ctrl Pts',(0.273974667166824,2.26970335964647,9.32260282360759));
#44686=CARTESIAN_POINT('Ctrl Pts',(0.274931233425394,2.26815458742115,9.32249044589305));
#44687=CARTESIAN_POINT('Ctrl Pts',(0.275661494025509,2.26695475214609,9.32240424493475));
#44688=CARTESIAN_POINT('Ctrl Pts',(0.28910761513023,2.24453370875449,9.32080859535926));
#44689=CARTESIAN_POINT('Ctrl Pts',(0.299348349226978,2.2219188359578,9.31944699385759));
#44690=CARTESIAN_POINT('Ctrl Pts',(0.31130192090492,2.18461831162818,9.3172556486139));
#44691=CARTESIAN_POINT('Ctrl Pts',(0.31477595047952,2.17060596694544,9.31644442352887));
#44692=CARTESIAN_POINT('Ctrl Pts',(0.318793607225193,2.14800667466691,9.3151119153959));
#44693=CARTESIAN_POINT('Ctrl Pts',(0.319952904256393,2.13954902072294,9.31460819945818));
#44694=CARTESIAN_POINT('Ctrl Pts',(0.320938248737837,2.12937141438724,9.31399182851701));
#44695=CARTESIAN_POINT('Ctrl Pts',(0.321088053155284,2.12768576239751,9.31388941400643));
#44696=CARTESIAN_POINT('Ctrl Pts',(0.321294071864631,2.12514034958045,9.31373423730632));
#44697=CARTESIAN_POINT('Ctrl Pts',(0.32136012743303,2.12428139753194,9.31368178253688));
#44698=CARTESIAN_POINT('Ctrl Pts',(0.321461454138795,2.12289089148367,9.3135967168224));
#44699=CARTESIAN_POINT('Ctrl Pts',(0.321498853002195,2.12235949290298,9.31356417255085));
#44700=CARTESIAN_POINT('Ctrl Pts',(0.321568019263655,2.12134064726148,9.31350170688179));
#44701=CARTESIAN_POINT('Ctrl Pts',(0.321599996324827,2.12085321554119,9.31347179213921));
#44702=CARTESIAN_POINT('Ctrl Pts',(0.321655217439827,2.11998112168741,9.3134182151589));
#44703=CARTESIAN_POINT('Ctrl Pts',(0.321678880027556,2.1195964862227,9.31339456610235));
#44704=CARTESIAN_POINT('Ctrl Pts',(0.321724533955342,2.11883201100172,9.31334752468675));
#44705=CARTESIAN_POINT('Ctrl Pts',(0.321746542642521,2.11845217284772,9.31332413290999));
#44706=CARTESIAN_POINT('Ctrl Pts',(0.321798431584484,2.11752831718236,9.31326719268379));
#44707=CARTESIAN_POINT('Ctrl Pts',(0.321827604926024,2.11698426257558,9.31323362210826));
#44708=CARTESIAN_POINT('Ctrl Pts',(0.321932207259695,2.114936419474,9.31310711364155));
#44709=CARTESIAN_POINT('Ctrl Pts',(0.321998476014577,2.11343220080957,9.31301388898242));
#44710=CARTESIAN_POINT('Ctrl Pts',(0.322995892387522,2.08650119072519,9.31133931193541));
#44711=CARTESIAN_POINT('Ctrl Pts',(0.320923013928696,2.06105837554091,9.3096582867879));
#44712=CARTESIAN_POINT('Ctrl Pts',(0.312800650625744,2.02088783306894,9.30688949054664));
#44713=CARTESIAN_POINT('Ctrl Pts',(0.308619650234542,2.00588876243242,9.30583131655575));
#44714=CARTESIAN_POINT('Ctrl Pts',(0.301243170409902,1.98531117428011,9.30438540503579));
#44715=CARTESIAN_POINT('Ctrl Pts',(0.298940280151752,1.97943593194171,9.30397344525857));
#44716=CARTESIAN_POINT('Ctrl Pts',(0.295308214869733,1.9709149283306,9.30338097911197));
#44717=CARTESIAN_POINT('Ctrl Pts',(0.294112853359124,1.96821408078086,9.30319394952822));
#44718=CARTESIAN_POINT('Ctrl Pts',(0.292670446725865,1.96507246898396,9.30297761729861));
#44719=CARTESIAN_POINT('Ctrl Pts',(0.292459338426577,1.96461549428365,9.30294618037436));
#44720=CARTESIAN_POINT('Ctrl Pts',(0.292135248125902,1.96391824913556,9.30289826311695));
#44721=CARTESIAN_POINT('Ctrl Pts',(0.29202303967483,1.96367762320072,9.30288173530024));
#44722=CARTESIAN_POINT('Ctrl Pts',(0.291827189591217,1.96325898302014,9.30285299609391));
#44723=CARTESIAN_POINT('Ctrl Pts',(0.291743682591993,1.96308090718334,9.30284077638791));
#44724=CARTESIAN_POINT('Ctrl Pts',(0.291554252313116,1.96267791368488,9.30281313404468));
#44725=CARTESIAN_POINT('Ctrl Pts',(0.291448231986424,1.96245304254624,9.30279771756275));
#44726=CARTESIAN_POINT('Ctrl Pts',(0.291159868875873,1.96184324919072,9.30275593309625));
#44727=CARTESIAN_POINT('Ctrl Pts',(0.290977022237704,1.96145856369801,9.30272959639889));
#44728=CARTESIAN_POINT('Ctrl Pts',(0.290148970578473,1.95972532166904,9.30261103170682));
#44729=CARTESIAN_POINT('Ctrl Pts',(0.289495136126377,1.95838087392306,9.30251933133136));
#44730=CARTESIAN_POINT('Ctrl Pts',(0.274543363257353,1.92817256513347,9.30046390739913));
#44731=CARTESIAN_POINT('Ctrl Pts',(0.256004967849526,1.90160390819619,9.2987453224863));
#44732=CARTESIAN_POINT('Ctrl Pts',(0.228363851595974,1.87246051648433,9.29646740760043));
#44733=CARTESIAN_POINT('Ctrl Pts',(0.222686951139093,1.86690178928056,9.2960121333234));
#44734=CARTESIAN_POINT('Ctrl Pts',(0.210496922445429,1.85581759715336,9.29505149672199));
#44735=CARTESIAN_POINT('Ctrl Pts',(0.203958018542915,1.85033000286046,9.29454529989065));
#44736=CARTESIAN_POINT('Ctrl Pts',(0.196305459717384,1.84440921654621,9.29395908257779));
#44737=CARTESIAN_POINT('Ctrl Pts',(0.195397731720319,1.84371459564046,9.29388964422535));
#44738=CARTESIAN_POINT('Ctrl Pts',(0.193969160340216,1.84263341099055,9.29378050587156));
#44739=CARTESIAN_POINT('Ctrl Pts',(0.193450806552801,1.84224356121355,9.2937409345204));
#44740=CARTESIAN_POINT('Ctrl Pts',(0.192576251440651,1.8415899393226,9.29367421808133));
#44741=CARTESIAN_POINT('Ctrl Pts',(0.192220674880557,1.84132533130668,9.29364710565782));
#44742=CARTESIAN_POINT('Ctrl Pts',(0.191523378647588,1.84080865877599,9.29359396249883));
#44743=CARTESIAN_POINT('Ctrl Pts',(0.191181704321476,1.84055653435846,9.29356793416731));
#44744=CARTESIAN_POINT('Ctrl Pts',(0.190529806795121,1.84007748061553,9.29351829529477));
#44745=CARTESIAN_POINT('Ctrl Pts',(0.190219673731412,1.8398504293987,9.29349468954556));
#44746=CARTESIAN_POINT('Ctrl Pts',(0.189504864235509,1.83932907251583,9.29344030307948));
#44747=CARTESIAN_POINT('Ctrl Pts',(0.189099907837803,1.83903515398505,9.29340950744909));
#44748=CARTESIAN_POINT('Ctrl Pts',(0.187896856629313,1.83816624651675,9.2933180642978));
#44749=CARTESIAN_POINT('Ctrl Pts',(0.187096817428827,1.83759397097636,9.29325731237546));
#44750=CARTESIAN_POINT('Ctrl Pts',(0.181590896754036,1.83369351497535,9.29283959599465));
#44751=CARTESIAN_POINT('Ctrl Pts',(0.17679934328509,1.83048862169564,9.29247795474948));
#44752=CARTESIAN_POINT('Ctrl Pts',(0.171618477234641,1.82722095947575,9.29208854592491));
#44753=CARTESIAN_POINT('Ctrl Pts',(0.171311956884023,1.8270283529292,9.29206551298342));
#44754=CARTESIAN_POINT('Ctrl Pts',(0.169470360494686,1.82587548247755,9.29192716524804));
#44755=CARTESIAN_POINT('Ctrl Pts',(0.167927562510964,1.82492766818028,9.29181141334538));
#44756=CARTESIAN_POINT('Ctrl Pts',(0.163353928201045,1.82217068447009,9.2914686968454));
#44757=CARTESIAN_POINT('Ctrl Pts',(0.160301333767252,1.82039829159432,9.29124050567791));
#44758=CARTESIAN_POINT('Ctrl Pts',(0.151297805332135,1.81536658448345,9.29056911605386));
#44759=CARTESIAN_POINT('Ctrl Pts',(0.145272546863271,1.81224474763069,9.29012184494769));
#44760=CARTESIAN_POINT('Ctrl Pts',(0.11770263215299,1.79904675553709,9.28808725386008));
#44761=CARTESIAN_POINT('Ctrl Pts',(0.0951824520950674,1.79118453603266,
9.28645078171237));
#44762=CARTESIAN_POINT('Ctrl Pts',(0.0642590882056443,1.78409643151518,
9.28435458792234));
#44763=CARTESIAN_POINT('Ctrl Pts',(0.056451393599643,1.78260819327844,9.28383831839708));
#44764=CARTESIAN_POINT('Ctrl Pts',(0.0473419126823514,1.78121868276833,
9.28325687548702));
#44765=CARTESIAN_POINT('Ctrl Pts',(0.0460866976093846,1.78103479603152,
9.28317721509758));
#44766=CARTESIAN_POINT('Ctrl Pts',(0.044450453554328,1.78080494988878,9.28307399803282));
#44767=CARTESIAN_POINT('Ctrl Pts',(0.0440704047874012,1.78075225566622,
9.28305006775));
#44768=CARTESIAN_POINT('Ctrl Pts',(0.043453312201162,1.78066781797097,9.28301128383923));
#44769=CARTESIAN_POINT('Ctrl Pts',(0.0432163269809917,1.78063565962394,
9.28299640672087));
#44770=CARTESIAN_POINT('Ctrl Pts',(0.0427604897811242,1.78057432024666,
9.28296782431492));
#44771=CARTESIAN_POINT('Ctrl Pts',(0.0425416442583363,1.78054510040347,
9.28295411689655));
#44772=CARTESIAN_POINT('Ctrl Pts',(0.0420365571953682,1.78047819035556,
9.28292251474028));
#44773=CARTESIAN_POINT('Ctrl Pts',(0.0417502940137508,1.78044065976626,
9.28290462910152));
#44774=CARTESIAN_POINT('Ctrl Pts',(0.0408343539197486,1.78032182704167,
9.28284748093711));
#44775=CARTESIAN_POINT('Ctrl Pts',(0.0402044820601876,1.780242000312,9.28280830155863));
#44776=CARTESIAN_POINT('Ctrl Pts',(0.0345371720173955,1.77954076511402,
9.28245682994647));
#44777=CARTESIAN_POINT('Ctrl Pts',(0.0294856040697999,1.77903653844019,
9.28215098169002));
#44778=CARTESIAN_POINT('Ctrl Pts',(0.0242906896697188,1.77864170172975,
9.28184214166569));
#44779=CARTESIAN_POINT('Ctrl Pts',(0.0241574755360709,1.77863166016607,
9.28183422585626));
#44780=CARTESIAN_POINT('Ctrl Pts',(0.00125812052171418,1.77691984593806,
9.2804741601245));
#44781=CARTESIAN_POINT('Ctrl Pts',(-0.0216270361881949,1.77764168175109,
9.27922222620605));
#44782=CARTESIAN_POINT('Ctrl Pts',(-0.0665934697885276,1.78387423876048,
9.27667621406895));
#44783=CARTESIAN_POINT('Ctrl Pts',(-0.0885502459302926,1.78930913974724,
9.27538821086509));
#44784=CARTESIAN_POINT('Ctrl Pts',(-0.110837505023448,1.7973821859204,9.27394672339378));
#44785=CARTESIAN_POINT('Ctrl Pts',(-0.111914926418665,1.79777898301173,
9.27387671241612));
#44786=CARTESIAN_POINT('Ctrl Pts',(-0.113482632557522,1.79836587690632,
9.27377435864941));
#44787=CARTESIAN_POINT('Ctrl Pts',(-0.113974617256266,1.79855143270735,
9.27374216776185));
#44788=CARTESIAN_POINT('Ctrl Pts',(-0.114836681755525,1.79887897903268,
9.27368563899117));
#44789=CARTESIAN_POINT('Ctrl Pts',(-0.115206958782272,1.79902045021149,
9.27366131855748));
#44790=CARTESIAN_POINT('Ctrl Pts',(-0.11592500622157,1.79929631268795,9.27361407791087));
#44791=CARTESIAN_POINT('Ctrl Pts',(-0.11627280644981,1.79943062513123,9.27359116037632));
#44792=CARTESIAN_POINT('Ctrl Pts',(-0.117101964863913,1.79975248156063,
9.27353643941066));
#44793=CARTESIAN_POINT('Ctrl Pts',(-0.11758310558766,1.79994057958566,9.27350461738098));
#44794=CARTESIAN_POINT('Ctrl Pts',(-0.119034705668059,1.80051209828081,
9.27340840133472));
#44795=CARTESIAN_POINT('Ctrl Pts',(-0.120003750037001,1.80089907327853,
9.27334388764747));
#44796=CARTESIAN_POINT('Ctrl Pts',(-0.130151262535391,1.8050085997919,9.27266531714067));
#44797=CARTESIAN_POINT('Ctrl Pts',(-0.139154444755825,1.80914731707223,
9.27203716281452));
#44798=CARTESIAN_POINT('Ctrl Pts',(-0.155749352561397,1.81772292380553,
9.27082741857528));
#44799=CARTESIAN_POINT('Ctrl Pts',(-0.163378220903477,1.8220688112014,9.27024920684198));
#44800=CARTESIAN_POINT('Ctrl Pts',(-0.178880907023782,1.83175912273989,
9.26903009468696));
#44801=CARTESIAN_POINT('Ctrl Pts',(-0.186714857630283,1.83715195210883,
9.26838854159852));
#44802=CARTESIAN_POINT('Ctrl Pts',(-0.20116444380182,1.84807124172975,9.26716316978081));
#44803=CARTESIAN_POINT('Ctrl Pts',(-0.207819720008185,1.85353255548032,
9.26658014512682));
#44804=CARTESIAN_POINT('Ctrl Pts',(-0.221790308664973,1.86596547196683,
9.26532475042865));
#44805=CARTESIAN_POINT('Ctrl Pts',(-0.229013250206423,1.87302848568942,
9.26465501754457));
#44806=CARTESIAN_POINT('Ctrl Pts',(-0.238491223189037,1.88321058212053,
9.26375996569211));
#44807=CARTESIAN_POINT('Ctrl Pts',(-0.241039655550134,1.88604766213267,
9.26351756214457));
#44808=CARTESIAN_POINT('Ctrl Pts',(-0.243888865830784,1.88933513594731,
9.26324519764691));
#44809=CARTESIAN_POINT('Ctrl Pts',(-0.244239452458768,1.88974169767854,
9.26321166011458));
#44810=CARTESIAN_POINT('Ctrl Pts',(-0.244766466172444,1.89035595186039,
9.26316121174955));
#44811=CARTESIAN_POINT('Ctrl Pts',(-0.244943646200372,1.89056299259612,
9.26314424543863));
#44812=CARTESIAN_POINT('Ctrl Pts',(-0.245260960192934,1.89093473795321,
9.26311385030455));
#44813=CARTESIAN_POINT('Ctrl Pts',(-0.245401190675574,1.89109935853284,
9.26310041431599));
#44814=CARTESIAN_POINT('Ctrl Pts',(-0.245703387916088,1.89145484073743,
9.26307145226073));
#44815=CARTESIAN_POINT('Ctrl Pts',(-0.245865297555767,1.8916457493975,9.26305593044334));
#44816=CARTESIAN_POINT('Ctrl Pts',(-0.246299976347489,1.89215949407944,
9.26301424581426));
#44817=CARTESIAN_POINT('Ctrl Pts',(-0.246572334323191,1.89248267975581,
9.26298811332896));
#44818=CARTESIAN_POINT('Ctrl Pts',(-0.247815404618548,1.89396363534135,
9.26286877265098));
#44819=CARTESIAN_POINT('Ctrl Pts',(-0.248778624072801,1.89512771114207,
9.26277610500984));
#44820=CARTESIAN_POINT('Ctrl Pts',(-0.270015356635874,1.9211634926797,9.26072754557983));
#44821=CARTESIAN_POINT('Ctrl Pts',(-0.286473783744934,1.94892260894471,
9.25901475177345));
#44822=CARTESIAN_POINT('Ctrl Pts',(-0.305082839575014,1.99471090782702,
9.2562125617498));
#44823=CARTESIAN_POINT('Ctrl Pts',(-0.3103000924616,2.01125850975935,9.25520671904228));
#44824=CARTESIAN_POINT('Ctrl Pts',(-0.314424179314365,2.0292893755722,9.25408214394024));
#44825=CARTESIAN_POINT('Ctrl Pts',(-0.314679958019772,2.0304364973001,9.254010488205));
#44826=CARTESIAN_POINT('Ctrl Pts',(-0.315042150364789,2.03210374870938,
9.25390617363479));
#44827=CARTESIAN_POINT('Ctrl Pts',(-0.315153564583383,2.03262279190371,
9.25387367511036));
#44828=CARTESIAN_POINT('Ctrl Pts',(-0.315346095010384,2.03353065558077,
9.25381678940207));
#44829=CARTESIAN_POINT('Ctrl Pts',(-0.315427776041648,2.0339193562005,9.25379242035267));
#44830=CARTESIAN_POINT('Ctrl Pts',(-0.315584445902157,2.03467182019226,
9.25374521913995));
#44831=CARTESIAN_POINT('Ctrl Pts',(-0.315659524916964,2.03503556434659,
9.25372238990259));
#44832=CARTESIAN_POINT('Ctrl Pts',(-0.315836445533802,2.03590026035484,
9.25366809119387));
#44833=CARTESIAN_POINT('Ctrl Pts',(-0.31593772409802,2.03640132519493,9.25363660377891));
#44834=CARTESIAN_POINT('Ctrl Pts',(-0.31629157978337,2.03817369335655,9.25352514380728));
#44835=CARTESIAN_POINT('Ctrl Pts',(-0.316537676513447,2.03944626432851,
9.25344496471372));
#44836=CARTESIAN_POINT('Ctrl Pts',(-0.320452522200097,2.06036622311442,
9.25212433245832));
#44837=CARTESIAN_POINT('Ctrl Pts',(-0.322292725957246,2.08030773341298,
9.25082424572997));
#44838=CARTESIAN_POINT('Ctrl Pts',(-0.322248784874179,2.12948008707199,
9.24753308221895));
#44839=CARTESIAN_POINT('Ctrl Pts',(-0.318256680675824,2.15853321851025,
9.2455081317289));
#44840=CARTESIAN_POINT('Ctrl Pts',(-0.309997251839141,2.1881203943083,9.2435648412986));
#44841=CARTESIAN_POINT('Ctrl Pts',(-0.309576898017133,2.18958596136027,
9.24346893800038));
#44842=CARTESIAN_POINT('Ctrl Pts',(-0.309026333950325,2.191455346539,9.24334711406544));
#44843=CARTESIAN_POINT('Ctrl Pts',(-0.308905714432217,2.19186193488804,
9.24332064814244));
#44844=CARTESIAN_POINT('Ctrl Pts',(-0.30871252674617,2.19250845521428,9.24327861443535));
#44845=CARTESIAN_POINT('Ctrl Pts',(-0.308640481175702,2.1927485408877,9.24326301618634));
#44846=CARTESIAN_POINT('Ctrl Pts',(-0.308505169495327,2.1931975518534,9.24323386505611));
#44847=CARTESIAN_POINT('Ctrl Pts',(-0.308441971702367,2.19340649532863,
9.24322030833382));
#44848=CARTESIAN_POINT('Ctrl Pts',(-0.308299244740658,2.19387665244126,
9.24318982250214));
#44849=CARTESIAN_POINT('Ctrl Pts',(-0.308219596048025,2.19413782871169,
9.24317290055075));
#44850=CARTESIAN_POINT('Ctrl Pts',(-0.307981589522417,2.19491473644723,
9.24312260207076));
#44851=CARTESIAN_POINT('Ctrl Pts',(-0.307822267502995,2.19543017509621,
9.24308928197094));
#44852=CARTESIAN_POINT('Ctrl Pts',(-0.306502231125542,2.19966305495287,
9.24281604676594));
#44853=CARTESIAN_POINT('Ctrl Pts',(-0.3052754526768,2.2033597770709,9.24257993180317));
#44854=CARTESIAN_POINT('Ctrl Pts',(-0.301042285194321,2.21538223427711,
9.24181752714214));
#44855=CARTESIAN_POINT('Ctrl Pts',(-0.297759730578613,2.22360698221587,
9.24130462433327));
#44856=CARTESIAN_POINT('Ctrl Pts',(-0.283921579933928,2.25451660009095,
9.23937372389428));
#44857=CARTESIAN_POINT('Ctrl Pts',(-0.271077768142592,2.27607885477031,
9.23801286452511));
#44858=CARTESIAN_POINT('Ctrl Pts',(-0.255107782884667,2.29693339589262,
9.23650286999729));
#44859=CARTESIAN_POINT('Ctrl Pts',(-0.254340758183702,2.29792302035118,
9.23643073288618));
#44860=CARTESIAN_POINT('Ctrl Pts',(-0.246382678805956,2.30806797561422,
9.2356860906442));
#44861=CARTESIAN_POINT('Ctrl Pts',(-0.238707075100769,2.31683079106351,
9.23499907576622));
#44862=CARTESIAN_POINT('Ctrl Pts',(-0.229743389893656,2.32601010366434,
9.23421919173987));
#44863=CARTESIAN_POINT('Ctrl Pts',(-0.228907163141345,2.32685700950455,
9.23414664156011));
#44864=CARTESIAN_POINT('Ctrl Pts',(-0.227721234991966,2.328044849197,9.23404403131291));
#44865=CARTESIAN_POINT('Ctrl Pts',(-0.227375413408941,2.32838965713123,
9.23401414294733));
#44866=CARTESIAN_POINT('Ctrl Pts',(-0.226769321475982,2.32899123156108,
9.23396181741621));
#44867=CARTESIAN_POINT('Ctrl Pts',(-0.226509394782134,2.32924834430848,
9.23393939556259));
#44868=CARTESIAN_POINT('Ctrl Pts',(-0.225963071653665,2.32978691676569,
9.23389230654042));
#44869=CARTESIAN_POINT('Ctrl Pts',(-0.225676585722401,2.33006828447712,
9.23386763538982));
#44870=CARTESIAN_POINT('Ctrl Pts',(-0.224992335713205,2.33073780221853,
9.23380876165914));
#44871=CARTESIAN_POINT('Ctrl Pts',(-0.224594092963673,2.33112545922501,
9.23377453761601));
#44872=CARTESIAN_POINT('Ctrl Pts',(-0.223250307337467,2.33242677281488,
9.23365919266835));
#44873=CARTESIAN_POINT('Ctrl Pts',(-0.22230018577673,2.33333566330262,9.23357786509292));
#44874=CARTESIAN_POINT('Ctrl Pts',(-0.209290035872313,2.34562964207,9.23246722311068));
#44875=CARTESIAN_POINT('Ctrl Pts',(-0.196376254490532,2.35607118160359,
9.23139752377565));
#44876=CARTESIAN_POINT('Ctrl Pts',(-0.164463256981946,2.37803619956201,
9.22882743055535));
#44877=CARTESIAN_POINT('Ctrl Pts',(-0.144962522255172,2.38868331363324,
9.22730782442123));
#44878=CARTESIAN_POINT('Ctrl Pts',(-0.113999883711374,2.40165446173952,
9.22506730081162));
#44879=CARTESIAN_POINT('Ctrl Pts',(-0.103246949205295,2.40550207786571,
9.22431916701531));
#44880=CARTESIAN_POINT('Ctrl Pts',(-0.0915930384696644,2.40898616956389,
9.22355554197668));
#44881=CARTESIAN_POINT('Ctrl Pts',(-0.0908739940220044,2.40919840703829,
9.22350861525267));
#44882=CARTESIAN_POINT('Ctrl Pts',(-0.0898761893278974,2.40948914370782,
9.2234437637663));
#44883=CARTESIAN_POINT('Ctrl Pts',(-0.0895980612295598,2.4095697771208,
9.22342571585984));
#44884=CARTESIAN_POINT('Ctrl Pts',(-0.0891199831508987,2.40970768070441,
9.22339474299419));
#44885=CARTESIAN_POINT('Ctrl Pts',(-0.0889200863736359,2.40976513219532,
9.22338180742166));
#44886=CARTESIAN_POINT('Ctrl Pts',(-0.0885069590612355,2.4098834345241,
9.2233551045819));
#44887=CARTESIAN_POINT('Ctrl Pts',(-0.0882937217555166,2.40994425868776,
9.22334133896922));
#44888=CARTESIAN_POINT('Ctrl Pts',(-0.0877921231587887,2.41008677585772,
9.22330899812379));
#44889=CARTESIAN_POINT('Ctrl Pts',(-0.0875037094745219,2.41016828703223,
9.22329043357298));
#44890=CARTESIAN_POINT('Ctrl Pts',(-0.0865630749125925,2.41043271176501,
9.22322998703071));
#44891=CARTESIAN_POINT('Ctrl Pts',(-0.0859103854186231,2.4106139729132,
9.22318820091608));
#44892=CARTESIAN_POINT('Ctrl Pts',(-0.0727909785173573,2.41421290288505,
9.22235133140243));
#44893=CARTESIAN_POINT('Ctrl Pts',(-0.0601285950861957,2.41687997430841,
9.22159878679526));
#44894=CARTESIAN_POINT('Ctrl Pts',(-0.0161271052058792,2.42341418340386,
9.2190661744642));
#44895=CARTESIAN_POINT('Ctrl Pts',(0.0155942167075223,2.42344045047705,
9.21736335468718));
#44896=CARTESIAN_POINT('Ctrl Pts',(0.0480562626852495,2.41867435727282,
9.21542358371179));
#44897=CARTESIAN_POINT('Ctrl Pts',(0.0492967514059602,2.41848482005429,
9.21534918727704));
#44898=CARTESIAN_POINT('Ctrl Pts',(0.0555863691839977,2.41748618786691,
9.21497054562902));
#44899=CARTESIAN_POINT('Ctrl Pts',(0.0606166144981682,2.41656428331611,
9.21466301516741));
#44900=CARTESIAN_POINT('Ctrl Pts',(0.0664677751013699,2.41534735725944,
9.2142990747713));
#44901=CARTESIAN_POINT('Ctrl Pts',(0.0673122413211632,2.41516818209175,
9.21424639724153));
#44902=CARTESIAN_POINT('Ctrl Pts',(0.0686606896333905,2.41487640748671,
9.2141620347003));
#44903=CARTESIAN_POINT('Ctrl Pts',(0.0691651426531609,2.41476598502623,
9.2141304194692));
#44904=CARTESIAN_POINT('Ctrl Pts',(0.0700562669078341,2.41456867637374,
9.21407447206174));
#44905=CARTESIAN_POINT('Ctrl Pts',(0.0704430482838862,2.41448228826889,
9.21405015591157));
#44906=CARTESIAN_POINT('Ctrl Pts',(0.07124366655539,2.41430191805765,9.21399975416798));
#44907=CARTESIAN_POINT('Ctrl Pts',(0.0716574789330507,2.41420783158476,
9.2139736652637));
#44908=CARTESIAN_POINT('Ctrl Pts',(0.0727191237618679,2.41396424430588,
9.21390663553585));
#44909=CARTESIAN_POINT('Ctrl Pts',(0.0733666792505109,2.41381355615783,
9.21386565659768));
#44910=CARTESIAN_POINT('Ctrl Pts',(0.0760294514117654,2.41318522855685,
9.21369675981475));
#44911=CARTESIAN_POINT('Ctrl Pts',(0.0780404721594917,2.41269018093233,
9.21356828247209));
#44912=CARTESIAN_POINT('Ctrl Pts',(0.0913977379148219,2.4092651781221,9.21270864357123));
#44913=CARTESIAN_POINT('Ctrl Pts',(0.102580401096877,2.40573796288231,9.21195815715932));
#44914=CARTESIAN_POINT('Ctrl Pts',(0.145276297111396,2.38966452237933,9.20896947933284));
#44915=CARTESIAN_POINT('Ctrl Pts',(0.17491814387827,2.37278914454418,9.20659769555844));
#44916=CARTESIAN_POINT('Ctrl Pts',(0.204382589033286,2.34920612274939,9.20416775590719));
#44917=CARTESIAN_POINT('Ctrl Pts',(0.207338889715483,2.34675194501224,9.20392336750097));
#44918=CARTESIAN_POINT('Ctrl Pts',(0.210686342041663,2.34387039843719,9.20364666092771));
#44919=CARTESIAN_POINT('Ctrl Pts',(0.211120929197663,2.34349426938561,9.2036107375397));
#44920=CARTESIAN_POINT('Ctrl Pts',(0.211766562770423,2.3429324546685,9.20355737251683));
#44921=CARTESIAN_POINT('Ctrl Pts',(0.211978373227364,2.34274765482736,9.20353986585437));
#44922=CARTESIAN_POINT('Ctrl Pts',(0.212352036702831,2.34242077987284,9.20350898310903));
#44923=CARTESIAN_POINT('Ctrl Pts',(0.212513989281265,2.34227881947637,9.20349559846286));
#44924=CARTESIAN_POINT('Ctrl Pts',(0.212829194895273,2.34200196508985,9.20346954927287));
#44925=CARTESIAN_POINT('Ctrl Pts',(0.212982461528205,2.34186708827177,9.20345688351602));
#44926=CARTESIAN_POINT('Ctrl Pts',(0.213399442329204,2.34149943554349,9.20342242575821));
#44927=CARTESIAN_POINT('Ctrl Pts',(0.213662904715161,2.34126637251329,9.20340065528547));
#44928=CARTESIAN_POINT('Ctrl Pts',(0.214680787731406,2.34036296202908,9.20331654718097));
#44929=CARTESIAN_POINT('Ctrl Pts',(0.215432449846251,2.33968949445776,9.20325444084433));
#44930=CARTESIAN_POINT('Ctrl Pts',(0.22020021859646,2.3353771644264,9.20286043248825));
#44931=CARTESIAN_POINT('Ctrl Pts',(0.224127435672611,2.3316407705738,9.20253556745034));
#44932=CARTESIAN_POINT('Ctrl Pts',(0.233038471009759,2.32272379101292,9.20179236723782));
#44933=CARTESIAN_POINT('Ctrl Pts',(0.237947013785835,2.31747194532052,9.20137826629825));
#44934=CARTESIAN_POINT('Ctrl Pts',(0.263631855131663,2.28807887105489,9.19915701602563));
#44935=CARTESIAN_POINT('Ctrl Pts',(0.280916417198049,2.26112561489226,9.19743824819553));
#44936=CARTESIAN_POINT('Ctrl Pts',(0.296375529083666,2.2267170770787,9.19520383593953));
#44937=CARTESIAN_POINT('Ctrl Pts',(0.298635507183917,2.22129509043419,9.19485140084271));
#44938=CARTESIAN_POINT('Ctrl Pts',(0.301101523517411,2.21489137038469,9.19443365753669));
#44939=CARTESIAN_POINT('Ctrl Pts',(0.301452808295963,2.21396648099165,9.19437328780386));
#44940=CARTESIAN_POINT('Ctrl Pts',(0.301975765990522,2.21257026243526,9.19428209534672));
#44941=CARTESIAN_POINT('Ctrl Pts',(0.30215060862232,2.21210012013807,9.19425137866463));
#44942=CARTESIAN_POINT('Ctrl Pts',(0.302460485357941,2.21126088658841,9.19419652913191));
#44943=CARTESIAN_POINT('Ctrl Pts',(0.302595943533375,2.21089195210824,9.19417241049113));
#44944=CARTESIAN_POINT('Ctrl Pts',(0.302880109608514,2.21011359846548,9.19412151288739));
#44945=CARTESIAN_POINT('Ctrl Pts',(0.303028662883704,2.20970412404022,9.19409472882898));
#44946=CARTESIAN_POINT('Ctrl Pts',(0.303418905909796,2.20862161182886,9.19402389911311));
#44947=CARTESIAN_POINT('Ctrl Pts',(0.303659185421062,2.20794807138638,9.19397980664445));
#44948=CARTESIAN_POINT('Ctrl Pts',(0.304737649454518,2.2048928761645,9.19377969725775));
#44949=CARTESIAN_POINT('Ctrl Pts',(0.305550051225639,2.20250227352422,9.19362282807738));
#44950=CARTESIAN_POINT('Ctrl Pts',(0.30898060578398,2.1920040623906,9.19293251834585));
#44951=CARTESIAN_POINT('Ctrl Pts',(0.31130455336543,2.1838046264506,9.19238953671076));
#44952=CARTESIAN_POINT('Ctrl Pts',(0.316659892285136,2.16158855380709,9.19090722490897));
#44953=CARTESIAN_POINT('Ctrl Pts',(0.319085226795173,2.14744659138467,9.18995131206832));
#44954=CARTESIAN_POINT('Ctrl Pts',(0.322873885072103,2.11085602244097,9.18746970081982));
#44955=CARTESIAN_POINT('Ctrl Pts',(0.322846002755955,2.08833879227044,9.18593206406742));
#44956=CARTESIAN_POINT('Ctrl Pts',(0.32010047891312,2.06245520685477,9.18425922995424));
#44957=CARTESIAN_POINT('Ctrl Pts',(0.31966478467034,2.05891038867476,9.18403233229352));
#44958=CARTESIAN_POINT('Ctrl Pts',(0.31909235015928,2.05481632979918,9.18377339520442));
#44959=CARTESIAN_POINT('Ctrl Pts',(0.319013005767058,2.05425949119423,9.18373824377928));
#44960=CARTESIAN_POINT('Ctrl Pts',(0.318892195623884,2.05342725309844,9.18368581034115));
#44961=CARTESIAN_POINT('Ctrl Pts',(0.318851830563197,2.05315169873217,9.18366846651512));
#44962=CARTESIAN_POINT('Ctrl Pts',(0.31877983185913,2.05266459912261,9.18363783801377));
#44963=CARTESIAN_POINT('Ctrl Pts',(0.318748344770384,2.05245303286674,9.18362454499482));
#44964=CARTESIAN_POINT('Ctrl Pts',(0.31868638253136,2.05203952751024,9.18359858378368));
#44965=CARTESIAN_POINT('Ctrl Pts',(0.31865592616886,2.05183758674664,9.18358591455372));
#44966=CARTESIAN_POINT('Ctrl Pts',(0.318572047551832,2.05128499250872,9.18355127128435));
#44967=CARTESIAN_POINT('Ctrl Pts',(0.318518238120746,2.05093439673691,9.18352931930948));
#44968=CARTESIAN_POINT('Ctrl Pts',(0.31830574446174,2.04956497395864,9.18344368049867));
#44969=CARTESIAN_POINT('Ctrl Pts',(0.318142747654755,2.04854680775884,9.18338023590473));
#44970=CARTESIAN_POINT('Ctrl Pts',(0.317060019534267,2.04198540971057,9.18297274715278));
#44971=CARTESIAN_POINT('Ctrl Pts',(0.316000271256853,2.03646586493018,9.18263626742063));
#44972=CARTESIAN_POINT('Ctrl Pts',(0.313226104936017,2.02381368238275,9.18187371911683));
#44973=CARTESIAN_POINT('Ctrl Pts',(0.311411453922295,2.01670614103382,9.1814518247345));
#44974=CARTESIAN_POINT('Ctrl Pts',(0.30051338523428,1.97938473070011,9.17924226706982));
#44975=CARTESIAN_POINT('Ctrl Pts',(0.287273816074932,1.95056723682215,9.17753734320381));
#44976=CARTESIAN_POINT('Ctrl Pts',(0.266890924238613,1.91926788465284,9.17532413514828));
#44977=CARTESIAN_POINT('Ctrl Pts',(0.263592940729428,1.91449092195419,9.17497578603572));
#44978=CARTESIAN_POINT('Ctrl Pts',(0.25958617221436,1.9090100354833,9.17456246634513));
#44979=CARTESIAN_POINT('Ctrl Pts',(0.259000771036862,1.9082169248358,9.17450231487037));
#44980=CARTESIAN_POINT('Ctrl Pts',(0.258112476162487,1.90702493397563,9.17441138851136));
#44981=CARTESIAN_POINT('Ctrl Pts',(0.257812272560361,1.90662404862386,9.17438071874684));
#44982=CARTESIAN_POINT('Ctrl Pts',(0.257274879907028,1.9059099018883,9.17432592163146));
#44983=CARTESIAN_POINT('Ctrl Pts',(0.257038049620511,1.90559637076099,9.17430180838818));
#44984=CARTESIAN_POINT('Ctrl Pts',(0.256537208318572,1.90493584008329,9.17425088977127));
#44985=CARTESIAN_POINT('Ctrl Pts',(0.256273065495231,1.9045889418825,9.17422407923752));
#44986=CARTESIAN_POINT('Ctrl Pts',(0.255572681322295,1.9036729913772,9.17415310513886));
#44987=CARTESIAN_POINT('Ctrl Pts',(0.255135245252128,1.90310485945585,9.17410889441892));
#44988=CARTESIAN_POINT('Ctrl Pts',(0.253137334292922,1.90052785591324,9.17390749607163));
#44989=CARTESIAN_POINT('Ctrl Pts',(0.251555039171011,1.89853608772178,9.1737494426714));
#44990=CARTESIAN_POINT('Ctrl Pts',(0.244547562709446,1.88992645955553,9.17305553378745));
#44991=CARTESIAN_POINT('Ctrl Pts',(0.238884020454427,1.88350795528189,9.17251005970223));
#44992=CARTESIAN_POINT('Ctrl Pts',(0.226727683386967,1.87078959278926,9.17136859285812));
#44993=CARTESIAN_POINT('Ctrl Pts',(0.220211533302147,1.86452237331555,9.17077197360049));
#44994=CARTESIAN_POINT('Ctrl Pts',(0.190948838587609,1.83865556592288,9.16816286969854));
#44995=CARTESIAN_POINT('Ctrl Pts',(0.165789524914751,1.82201390988374,9.16607658136737));
#44996=CARTESIAN_POINT('Ctrl Pts',(0.137323785113586,1.80844272097868,9.16408179344562));
#44997=CARTESIAN_POINT('Ctrl Pts',(0.135952221353923,1.80780064573863,9.16398654004472));
#44998=CARTESIAN_POINT('Ctrl Pts',(0.134194982601358,1.80699307474984,9.16386564652002));
#44999=CARTESIAN_POINT('Ctrl Pts',(0.133813469911855,1.80681864507642,9.1638394679706));
#45000=CARTESIAN_POINT('Ctrl Pts',(0.133207383923417,1.80654296877555,9.16379798968754));
#45001=CARTESIAN_POINT('Ctrl Pts',(0.132983034917777,1.80644123461934,9.16378265994439));
#45002=CARTESIAN_POINT('Ctrl Pts',(0.132560040236013,1.80625000625294,9.16375380203724));
#45003=CARTESIAN_POINT('Ctrl Pts',(0.132361421845507,1.80616045687946,9.16374027054313));
#45004=CARTESIAN_POINT('Ctrl Pts',(0.131971332015904,1.80598505619314,9.16371373129254));
#45005=CARTESIAN_POINT('Ctrl Pts',(0.131779868505301,1.80589919090025,9.16370072269295));
#45006=CARTESIAN_POINT('Ctrl Pts',(0.131186650982674,1.80563384731431,9.16366047109091));
#45007=CARTESIAN_POINT('Ctrl Pts',(0.13078461098561,1.80545500381467,9.16363326719018));
#45008=CARTESIAN_POINT('Ctrl Pts',(0.128663183824598,1.80451650790113,9.16349011394637));
#45009=CARTESIAN_POINT('Ctrl Pts',(0.126937495494548,1.80377106554039,9.1633750221242));
#45010=CARTESIAN_POINT('Ctrl Pts',(0.0995909339366301,1.79224108174669,
9.16157102601071));
#45011=CARTESIAN_POINT('Ctrl Pts',(0.072682332224846,1.7847988969068,9.16006252846432));
#45012=CARTESIAN_POINT('Ctrl Pts',(0.024363515506679,1.77796232442062,9.15731991706862));
#45013=CARTESIAN_POINT('Ctrl Pts',(0.00334423127245716,1.77705966082569,
9.15611655528472));
#45014=CARTESIAN_POINT('Ctrl Pts',(-0.018909361647475,1.77827760357419,
9.15476293823062));
#45015=CARTESIAN_POINT('Ctrl Pts',(-0.0202064611593273,1.77835646567975,
9.15468376974191));
#45016=CARTESIAN_POINT('Ctrl Pts',(-0.0220136586492022,1.77847731594518,
9.15457307981676));
#45017=CARTESIAN_POINT('Ctrl Pts',(-0.0225241993204483,1.77851267836952,
9.15454176632268));
#45018=CARTESIAN_POINT('Ctrl Pts',(-0.0234052618374122,1.77857581391439,
9.15448765199493));
#45019=CARTESIAN_POINT('Ctrl Pts',(-0.0237758249497694,1.7786030121041,
9.15446486924649));
#45020=CARTESIAN_POINT('Ctrl Pts',(-0.024542325788662,1.77866060378367,
9.15441769578054));
#45021=CARTESIAN_POINT('Ctrl Pts',(-0.0249382558878842,1.77869108834821,
9.15439330223868));
#45022=CARTESIAN_POINT('Ctrl Pts',(-0.02586281170737,1.77876399354865,9.15433627743853));
#45023=CARTESIAN_POINT('Ctrl Pts',(-0.0263913899086573,1.77880698730584,
9.15430362822502));
#45024=CARTESIAN_POINT('Ctrl Pts',(-0.0280881253106708,1.77894921385831,
9.1541986701978));
#45025=CARTESIAN_POINT('Ctrl Pts',(-0.0292558379016475,1.77905351543267,
9.15412620225493));
#45026=CARTESIAN_POINT('Ctrl Pts',(-0.0470739355504622,1.7807430991598,
9.15301676544352));
#45027=CARTESIAN_POINT('Ctrl Pts',(-0.0635739325559083,1.78361555330946,
9.15193863340219));
#45028=CARTESIAN_POINT('Ctrl Pts',(-0.106843161993814,1.79467024787076,
9.14897655377452));
#45029=CARTESIAN_POINT('Ctrl Pts',(-0.13289537377269,1.80507559073,9.14704138917412));
#45030=CARTESIAN_POINT('Ctrl Pts',(-0.158653774177087,1.81947791907748,
9.14511767977599));
#45031=CARTESIAN_POINT('Ctrl Pts',(-0.160023318368942,1.82025691124188,
9.1450154057203));
#45032=CARTESIAN_POINT('Ctrl Pts',(-0.165172319279618,1.82323583327889,
9.14463107016673));
#45033=CARTESIAN_POINT('Ctrl Pts',(-0.16891279146486,1.82550269105857,9.14435223373808));
#45034=CARTESIAN_POINT('Ctrl Pts',(-0.173110100509541,1.82816471016865,
9.14404077000811));
#45035=CARTESIAN_POINT('Ctrl Pts',(-0.173613132410826,1.828485705783,9.14400346599354));
#45036=CARTESIAN_POINT('Ctrl Pts',(-0.174355667562551,1.82896244093522,
9.14394843943619));
#45037=CARTESIAN_POINT('Ctrl Pts',(-0.174595856299142,1.8291171024231,9.14393064592648));
#45038=CARTESIAN_POINT('Ctrl Pts',(-0.175017808737747,1.82938959892126,
9.14389939811565));
#45039=CARTESIAN_POINT('Ctrl Pts',(-0.17519965958223,1.82950729800834,9.14388593470682));
#45040=CARTESIAN_POINT('Ctrl Pts',(-0.17555261033988,1.82973624312907,9.14385981102049));
#45041=CARTESIAN_POINT('Ctrl Pts',(-0.175723722743999,1.82984746800987,
9.14384714937398));
#45042=CARTESIAN_POINT('Ctrl Pts',(-0.176184476109127,1.8301475855677,9.14381306388029));
#45043=CARTESIAN_POINT('Ctrl Pts',(-0.176473919941158,1.83033678267132,
9.14379166048539));
#45044=CARTESIAN_POINT('Ctrl Pts',(-0.177570856838353,1.83105632609318,
9.14371057764903));
#45045=CARTESIAN_POINT('Ctrl Pts',(-0.178376278795038,1.83158984342593,
9.14365110866441));
#45046=CARTESIAN_POINT('Ctrl Pts',(-0.195424642986039,1.84299343314277,
9.14239345424319));
#45047=CARTESIAN_POINT('Ctrl Pts',(-0.210650655458016,1.85531710214423,
9.14129078237415));
#45048=CARTESIAN_POINT('Ctrl Pts',(-0.241265745106421,1.88508608544191,
9.13889961355804));
#45049=CARTESIAN_POINT('Ctrl Pts',(-0.256074983088156,1.90296534428046,
9.13761771849584));
#45050=CARTESIAN_POINT('Ctrl Pts',(-0.273000593140756,1.92856853107664,
9.13581399083593));
#45051=CARTESIAN_POINT('Ctrl Pts',(-0.276937822320651,1.93500454240386,
9.13536355167743));
#45052=CARTESIAN_POINT('Ctrl Pts',(-0.281122452668338,1.94241737469235,
9.13484563951005));
#45053=CARTESIAN_POINT('Ctrl Pts',(-0.281595642696187,1.94326451845423,
9.13478646631951));
#45054=CARTESIAN_POINT('Ctrl Pts',(-0.2823059005357,1.94454967934448,9.13469671394541));
#45055=CARTESIAN_POINT('Ctrl Pts',(-0.282545793580845,1.94498613547637,
9.13466623581234));
#45056=CARTESIAN_POINT('Ctrl Pts',(-0.28296119281772,1.9457460716037,9.13461317300681));
#45057=CARTESIAN_POINT('Ctrl Pts',(-0.283137158886007,1.94606930025932,
9.13459060478097));
#45058=CARTESIAN_POINT('Ctrl Pts',(-0.283502984159643,1.94674402721102,
9.13454349693796));
#45059=CARTESIAN_POINT('Ctrl Pts',(-0.283692744125307,1.94709557837874,
9.13451895383695));
#45060=CARTESIAN_POINT('Ctrl Pts',(-0.284139565542224,1.94792705917192,
9.13446090782268));
#45061=CARTESIAN_POINT('Ctrl Pts',(-0.284396064861843,1.94840728802505,
9.13442738502234));
#45062=CARTESIAN_POINT('Ctrl Pts',(-0.285237507572411,1.94999232466168,
9.13431674570738));
#45063=CARTESIAN_POINT('Ctrl Pts',(-0.285817234064097,1.95109987566199,
9.13423944486843));
#45064=CARTESIAN_POINT('Ctrl Pts',(-0.299013554261432,1.97667210717097,
9.13245472904365));
#45065=CARTESIAN_POINT('Ctrl Pts',(-0.308447821529095,2.00264424990726,
9.13062875611944));
#45066=CARTESIAN_POINT('Ctrl Pts',(-0.319128359725167,2.0502795604147,9.1273266524192));
#45067=CARTESIAN_POINT('Ctrl Pts',(-0.321717030553898,2.07148038515329,
9.12587722935952));
#45068=CARTESIAN_POINT('Ctrl Pts',(-0.322236906405087,2.09469047652434,
9.12440370653434));
#45069=CARTESIAN_POINT('Ctrl Pts',(-0.322262691384833,2.09659808113352,
9.12428345727989));
#45070=CARTESIAN_POINT('Ctrl Pts',(-0.322273624006796,2.09895613655316,
9.12413596567933));
#45071=CARTESIAN_POINT('Ctrl Pts',(-0.32227476794547,2.09940642361807,9.12410785308338));
#45072=CARTESIAN_POINT('Ctrl Pts',(-0.322274987464515,2.0999001627798,9.12407708571766));
#45073=CARTESIAN_POINT('Ctrl Pts',(-0.322274997995471,2.0999436107491,9.12407437874954));
#45074=CARTESIAN_POINT('Ctrl Pts',(-0.322274999740166,2.09998705874836,
9.12407167227341));
#45075=CARTESIAN_POINT('',(-0.322274883346534,2.1001520067383,8.8746518141229));
#45076=CARTESIAN_POINT('Ctrl Pts',(-0.3222749997412,2.09998708453407,9.12407167066716));
#45077=CARTESIAN_POINT('Ctrl Pts',(-0.322275006475149,2.10015511433518,
9.12406120370388));
#45078=CARTESIAN_POINT('Ctrl Pts',(-0.322274881796435,2.10032314458241,
9.12405074409919));
#45079=CARTESIAN_POINT('Ctrl Pts',(-0.322274305347323,2.10070137001345,
9.12402721693586));
#45080=CARTESIAN_POINT('Ctrl Pts',(-0.322273779350097,2.10091156537635,
9.12401415357674));
#45081=CARTESIAN_POINT('Ctrl Pts',(-0.322272318028823,2.10133139114295,
9.12398808538069));
#45082=CARTESIAN_POINT('Ctrl Pts',(-0.322271383815394,2.10154102055415,
9.12397508051068));
#45083=CARTESIAN_POINT('Ctrl Pts',(-0.322268314721346,2.10210599808351,
9.12394006173449));
#45084=CARTESIAN_POINT('Ctrl Pts',(-0.322265796640266,2.10246134515411,
9.12391806942701));
#45085=CARTESIAN_POINT('Ctrl Pts',(-0.322254373579189,2.10376827890683,
9.12383730285121));
#45086=CARTESIAN_POINT('Ctrl Pts',(-0.322241841434686,2.10471984101178,
9.12377872995073));
#45087=CARTESIAN_POINT('Ctrl Pts',(-0.322189763451291,2.10767872028998,
9.12359728136292));
#45088=CARTESIAN_POINT('Ctrl Pts',(-0.322135674229195,2.10968577667511,
9.12347518033166));
#45089=CARTESIAN_POINT('Ctrl Pts',(-0.320775593708641,2.14714916020973,
9.12121216451682));
#45090=CARTESIAN_POINT('Ctrl Pts',(-0.313642187258192,2.18215574250312,
9.11934376937572));
#45091=CARTESIAN_POINT('Ctrl Pts',(-0.296840065034912,2.22601073377984,
9.11664109221615));
#45092=CARTESIAN_POINT('Ctrl Pts',(-0.292168132095394,2.23649347269981,
9.11596741218478));
#45093=CARTESIAN_POINT('Ctrl Pts',(-0.286017448215895,2.24852397873105,
9.11515046246578));
#45094=CARTESIAN_POINT('Ctrl Pts',(-0.285069785752339,2.25033485921376,
9.11502629301877));
#45095=CARTESIAN_POINT('Ctrl Pts',(-0.283792683116517,2.25271976387082,
9.11486112543761));
#45096=CARTESIAN_POINT('Ctrl Pts',(-0.283478593857897,2.25330198981519,
9.11482067285366));
#45097=CARTESIAN_POINT('Ctrl Pts',(-0.28296043157443,2.25425546751951,9.11475421031527));
#45098=CARTESIAN_POINT('Ctrl Pts',(-0.282757414183987,2.25462729324968,
9.11472823804613));
#45099=CARTESIAN_POINT('Ctrl Pts',(-0.282362918369925,2.25534643622598,
9.11467790027765));
#45100=CARTESIAN_POINT('Ctrl Pts',(-0.282171530714198,2.25569380260841,
9.11465353805747));
#45101=CARTESIAN_POINT('Ctrl Pts',(-0.281728610304138,2.25649419882674,
9.11459729252982));
#45102=CARTESIAN_POINT('Ctrl Pts',(-0.28147662566395,2.25694697617399,9.11456539306317));
#45103=CARTESIAN_POINT('Ctrl Pts',(-0.280667922864831,2.25839187778283,
9.11446333236868));
#45104=CARTESIAN_POINT('Ctrl Pts',(-0.280107047500515,2.25938165440284,
9.11439302182294));
#45105=CARTESIAN_POINT('Ctrl Pts',(-0.274963639465519,2.26834721675459,
9.1137524774507));
#45106=CARTESIAN_POINT('Ctrl Pts',(-0.270047256484492,2.27612563647447,
9.11317014631783));
#45107=CARTESIAN_POINT('Ctrl Pts',(-0.248100795797389,2.30776467540335,
9.11068382794482));
#45108=CARTESIAN_POINT('Ctrl Pts',(-0.22819021214043,2.32945339730725,9.10866920339826));
#45109=CARTESIAN_POINT('Ctrl Pts',(-0.20071956032415,2.3522171736639,9.1062844085321));
#45110=CARTESIAN_POINT('Ctrl Pts',(-0.195689190118125,2.35613979483159,
9.10586206442916));
#45111=CARTESIAN_POINT('Ctrl Pts',(-0.18735542194903,2.36224943723577,9.10518908383455));
#45112=CARTESIAN_POINT('Ctrl Pts',(-0.18412242358853,2.36452931363229,9.10493421699836));
#45113=CARTESIAN_POINT('Ctrl Pts',(-0.179128041178886,2.36791535800599,
9.10455082618691));
#45114=CARTESIAN_POINT('Ctrl Pts',(-0.177396676352101,2.36906488799995,
9.10441976515729));
#45115=CARTESIAN_POINT('Ctrl Pts',(-0.175379766890807,2.37037607175871,
9.10426932463242));
#45116=CARTESIAN_POINT('Ctrl Pts',(-0.175105001037186,2.37055410074208,
9.10424887758286));
#45117=CARTESIAN_POINT('Ctrl Pts',(-0.174583330062121,2.37089097933189,
9.10421014776225));
#45118=CARTESIAN_POINT('Ctrl Pts',(-0.174336478495952,2.37104991069219,
9.10419185957968));
#45119=CARTESIAN_POINT('Ctrl Pts',(-0.173906165574756,2.37132612961839,
9.10416004706679));
#45120=CARTESIAN_POINT('Ctrl Pts',(-0.173722802175522,2.37144356880211,
9.10414651255123));
#45121=CARTESIAN_POINT('Ctrl Pts',(-0.173364690584578,2.37167241787107,
9.10412012119786));
#45122=CARTESIAN_POINT('Ctrl Pts',(-0.173189954364308,2.37178384477614,
9.10410726320088));
#45123=CARTESIAN_POINT('Ctrl Pts',(-0.172773179786678,2.37204905109484,
9.10407664054567));
#45124=CARTESIAN_POINT('Ctrl Pts',(-0.172531042928088,2.37220267647992,
9.10405888620415));
#45125=CARTESIAN_POINT('Ctrl Pts',(-0.171669159522273,2.37274789223841,
9.10399581920212));
#45126=CARTESIAN_POINT('Ctrl Pts',(-0.171048276206163,2.37313769473147,
9.10395062455782));
#45127=CARTESIAN_POINT('Ctrl Pts',(-0.161843376570682,2.37887301183097,
9.10328401466832));
#45128=CARTESIAN_POINT('Ctrl Pts',(-0.15301272663086,2.38381435482472,9.10268839078678));
#45129=CARTESIAN_POINT('Ctrl Pts',(-0.14079870778581,2.38991276445583,9.10190235699172));
#45130=CARTESIAN_POINT('Ctrl Pts',(-0.13760821335037,2.39144067643971,9.10170038046581));
#45131=CARTESIAN_POINT('Ctrl Pts',(-0.127819638621634,2.39593178741434,
9.10108899745989));
#45132=CARTESIAN_POINT('Ctrl Pts',(-0.121146308434953,2.39872572677038,
9.10068345075756));
#45133=CARTESIAN_POINT('Ctrl Pts',(-0.112373389731432,2.40205632643877,
9.10015850379826));
#45134=CARTESIAN_POINT('Ctrl Pts',(-0.110354698822169,2.40279967558499,
9.10003826576948));
#45135=CARTESIAN_POINT('Ctrl Pts',(-0.106004308987429,2.4043523503846,9.09978008297492));
#45136=CARTESIAN_POINT('Ctrl Pts',(-0.103670453392564,2.40515521258909,
9.09964214750342));
#45137=CARTESIAN_POINT('Ctrl Pts',(-0.0985766591353543,2.40684233054025,
9.09934196734812));
#45138=CARTESIAN_POINT('Ctrl Pts',(-0.0958135584986513,2.4077163228883,
9.09917968738911));
#45139=CARTESIAN_POINT('Ctrl Pts',(-0.0840697375560594,2.41125747899264,
9.09849119681587));
#45140=CARTESIAN_POINT('Ctrl Pts',(-0.0749871200052161,2.41356954157238,
9.09796160452972));
#45141=CARTESIAN_POINT('Ctrl Pts',(-0.054630931912622,2.41781631868772,
9.09676470484703));
#45142=CARTESIAN_POINT('Ctrl Pts',(-0.043329717323946,2.41955319344329,
9.09609343739053));
#45143=CARTESIAN_POINT('Ctrl Pts',(-0.0299318719113969,2.4208884803287,
9.09527933110038));
#45144=CARTESIAN_POINT('Ctrl Pts',(-0.02790093661394,2.42107144252262,9.09515544489651));
#45145=CARTESIAN_POINT('Ctrl Pts',(-0.0252096008689787,2.42128817054048,
9.09499059830643));
#45146=CARTESIAN_POINT('Ctrl Pts',(-0.0245506067106484,2.42133919805262,
9.09495018078039));
#45147=CARTESIAN_POINT('Ctrl Pts',(-0.0234691162626446,2.4214195942538,
9.0948837611441));
#45148=CARTESIAN_POINT('Ctrl Pts',(-0.0230467085712403,2.42145015820458,
9.09485779662383));
#45149=CARTESIAN_POINT('Ctrl Pts',(-0.0222285681444843,2.42150773508204,
9.09480746340354));
#45150=CARTESIAN_POINT('Ctrl Pts',(-0.0218328431805213,2.42153485023517,
9.09478309796098));
#45151=CARTESIAN_POINT('Ctrl Pts',(-0.0209197311695908,2.42159572338935,
9.09472682989403));
#45152=CARTESIAN_POINT('Ctrl Pts',(-0.0204023117249965,2.42162896344358,
9.09469491106923));
#45153=CARTESIAN_POINT('Ctrl Pts',(-0.0187476560859728,2.42173125289975,
9.09459272705157));
#45154=CARTESIAN_POINT('Ctrl Pts',(-0.0176101425610071,2.42179551974307,
9.09452231203086));
#45155=CARTESIAN_POINT('Ctrl Pts',(-0.00723308905086826,2.422326612463,
9.09387838328949));
#45156=CARTESIAN_POINT('Ctrl Pts',(0.00202135993366873,2.42240137786294,
9.09329263069196));
#45157=CARTESIAN_POINT('Ctrl Pts',(0.0352820480361989,2.4212380003023,9.09114317776906));
#45158=CARTESIAN_POINT('Ctrl Pts',(0.0591264892367729,2.41771436128919,
9.08951197234216));
#45159=CARTESIAN_POINT('Ctrl Pts',(0.0990626665044819,2.40715869967483,
9.08672231035184));
#45160=CARTESIAN_POINT('Ctrl Pts',(0.115392011659044,2.40140459384369,9.08556658588));
#45161=CARTESIAN_POINT('Ctrl Pts',(0.131601180017179,2.39418109189191,9.08445380821981));
#45162=CARTESIAN_POINT('Ctrl Pts',(0.132019144096375,2.39399376014938,9.08442513979912));
#45163=CARTESIAN_POINT('Ctrl Pts',(0.132698529429929,2.39368751827354,9.08437858321099));
#45164=CARTESIAN_POINT('Ctrl Pts',(0.132960191795416,2.39356914943806,9.08436066251124));
#45165=CARTESIAN_POINT('Ctrl Pts',(0.133462747505817,2.39334099736355,9.08432626398026));
#45166=CARTESIAN_POINT('Ctrl Pts',(0.133703664329392,2.39323126683924,9.08430978294207));
#45167=CARTESIAN_POINT('Ctrl Pts',(0.134139030605454,2.39303232221435,9.08428001641208));
#45168=CARTESIAN_POINT('Ctrl Pts',(0.134333525935228,2.39294321156973,9.08426672459544));
#45169=CARTESIAN_POINT('Ctrl Pts',(0.134756214771293,2.39274904152564,9.08423785127734));
#45170=CARTESIAN_POINT('Ctrl Pts',(0.134984373566294,2.3926439092611,9.08422227440706));
#45171=CARTESIAN_POINT('Ctrl Pts',(0.135592672475447,2.39236275119539,9.08418076628492));
#45172=CARTESIAN_POINT('Ctrl Pts',(0.135972594309035,2.39218625004805,9.08415486441848));
#45173=CARTESIAN_POINT('Ctrl Pts',(0.137719369223773,2.3913706020711,9.08403587420011));
#45174=CARTESIAN_POINT('Ctrl Pts',(0.139082095910216,2.39072258807412,9.08394332569059));
#45175=CARTESIAN_POINT('Ctrl Pts',(0.166571108161113,2.37741328275147,9.08208112357642));
#45176=CARTESIAN_POINT('Ctrl Pts',(0.190877437684557,2.36128624279729,9.0805121452953));
#45177=CARTESIAN_POINT('Ctrl Pts',(0.227557527627569,2.32906331637341,9.07776389390964));
#45178=CARTESIAN_POINT('Ctrl Pts',(0.24118225007744,2.31467040042247,9.0766274197742));
#45179=CARTESIAN_POINT('Ctrl Pts',(0.254387679546605,2.29786519301612,9.07533161800282));
#45180=CARTESIAN_POINT('Ctrl Pts',(0.255365055717651,2.29660217264241,9.07523442858076));
#45181=CARTESIAN_POINT('Ctrl Pts',(0.256697291505717,2.29485388737421,9.07510014863325));
#45182=CARTESIAN_POINT('Ctrl Pts',(0.25706025239857,2.29437480165977,9.07506337732801));
#45183=CARTESIAN_POINT('Ctrl Pts',(0.257668876498846,2.2935667695236,9.07500140023602));
#45184=CARTESIAN_POINT('Ctrl Pts',(0.257915256205702,2.293238362635,9.07497622259242));
#45185=CARTESIAN_POINT('Ctrl Pts',(0.258400155899498,2.29258944590693,9.07492649511849));
#45186=CARTESIAN_POINT('Ctrl Pts',(0.258638708799228,2.29226896148886,9.07490194663601));
#45187=CARTESIAN_POINT('Ctrl Pts',(0.259161535677316,2.29156383482329,9.07484795840206));
#45188=CARTESIAN_POINT('Ctrl Pts',(0.25944555018983,2.29117900216706,9.07481850861884));
#45189=CARTESIAN_POINT('Ctrl Pts',(0.260426299051021,2.28984390124101,9.07471638930528));
#45190=CARTESIAN_POINT('Ctrl Pts',(0.261118671341194,2.28889045368603,9.0746435509255));
#45191=CARTESIAN_POINT('Ctrl Pts',(0.267971646547206,2.27934371998573,9.07391507052987));
#45192=CARTESIAN_POINT('Ctrl Pts',(0.273710394512728,2.27045688936647,9.07324336960817));
#45193=CARTESIAN_POINT('Ctrl Pts',(0.293156612953367,2.23682166995211,9.07072030861133));
#45194=CARTESIAN_POINT('Ctrl Pts',(0.304026197468064,2.21058305501842,9.06877500196839));
#45195=CARTESIAN_POINT('Ctrl Pts',(0.313509350448234,2.17512729855535,9.06632464026598));
#45196=CARTESIAN_POINT('Ctrl Pts',(0.315367144530446,2.16690150444282,9.06576913197874));
#45197=CARTESIAN_POINT('Ctrl Pts',(0.317527982219409,2.15521833912484,9.06500651763709));
#45198=CARTESIAN_POINT('Ctrl Pts',(0.318101083291201,2.15181493667886,9.06478748479683));
#45199=CARTESIAN_POINT('Ctrl Pts',(0.318675110532792,2.14803630899597,9.0645482402996));
#45200=CARTESIAN_POINT('Ctrl Pts',(0.318730156582255,2.14766970047466,9.0645250693411));
#45201=CARTESIAN_POINT('Ctrl Pts',(0.318832180235634,2.14698214219073,9.06448169098019));
#45202=CARTESIAN_POINT('Ctrl Pts',(0.318879306040537,2.14666121537159,9.06446147530497));
#45203=CARTESIAN_POINT('Ctrl Pts',(0.318958121175769,2.14611878821643,9.06442736124056));
#45204=CARTESIAN_POINT('Ctrl Pts',(0.318990064368904,2.14589732590451,9.06441344841606));
#45205=CARTESIAN_POINT('Ctrl Pts',(0.319053011537075,2.14545767286302,9.06438585885645));
#45206=CARTESIAN_POINT('Ctrl Pts',(0.3190840223818,2.14523948335588,9.06437218174185));
#45207=CARTESIAN_POINT('Ctrl Pts',(0.319152806957575,2.14475193200619,9.06434165282261));
#45208=CARTESIAN_POINT('Ctrl Pts',(0.319190463602595,2.14448255336209,9.06432480769925));
#45209=CARTESIAN_POINT('Ctrl Pts',(0.319316743859785,2.14357078417664,9.0642678669987));
#45210=CARTESIAN_POINT('Ctrl Pts',(0.319403770341209,2.14292816851452,9.06422786142024));
#45211=CARTESIAN_POINT('Ctrl Pts',(0.320269202997353,2.13638934369698,9.06382203549159));
#45212=CARTESIAN_POINT('Ctrl Pts',(0.320886251865582,2.13047246428515,9.06346508941599));
#45213=CARTESIAN_POINT('Ctrl Pts',(0.323441846839036,2.09701018556772,9.06148722178926));
#45214=CARTESIAN_POINT('Ctrl Pts',(0.321997935908956,2.06932018636643,9.05999733937826));
#45215=CARTESIAN_POINT('Ctrl Pts',(0.314292801448586,2.0270923927585,9.05756126713257));
#45216=CARTESIAN_POINT('Ctrl Pts',(0.310476159033951,2.01225065333368,9.05667383182674));
#45217=CARTESIAN_POINT('Ctrl Pts',(0.30484645385447,1.99542583108715,9.05560356648724));
#45218=CARTESIAN_POINT('Ctrl Pts',(0.304046802647151,1.9931231618751,9.05545568430393));
#45219=CARTESIAN_POINT('Ctrl Pts',(0.302981924785872,1.99016545400573,9.05526384283466));
#45220=CARTESIAN_POINT('Ctrl Pts',(0.302740543854714,1.98950186727925,9.05522067807311));
#45221=CARTESIAN_POINT('Ctrl Pts',(0.302347433612376,1.98843211482623,9.05515089164556));
#45222=CARTESIAN_POINT('Ctrl Pts',(0.302197061184328,1.98802545011126,9.05512431531084));
#45223=CARTESIAN_POINT('Ctrl Pts',(0.301908660365595,1.98725031599607,9.05507356829797));
#45224=CARTESIAN_POINT('Ctrl Pts',(0.301770776820922,1.98688179323624,9.05504940250127));
#45225=CARTESIAN_POINT('Ctrl Pts',(0.301454265192153,1.98604054668975,9.05499414814593));
#45226=CARTESIAN_POINT('Ctrl Pts',(0.301275199745717,1.9855679895534,9.05496304498086));
#45227=CARTESIAN_POINT('Ctrl Pts',(0.30072349520115,1.98412230195733,9.05486769143431));
#45228=CARTESIAN_POINT('Ctrl Pts',(0.300347249945259,1.98315056320575,9.05480332016054));
#45229=CARTESIAN_POINT('Ctrl Pts',(0.297516323594727,1.97594306553049,9.05432377768877));
#45230=CARTESIAN_POINT('Ctrl Pts',(0.2948725444212,1.96978380486147,9.0539022525128));
#45231=CARTESIAN_POINT('Ctrl Pts',(0.291217933122498,1.96195269162055,9.05335041249823));
#45232=CARTESIAN_POINT('Ctrl Pts',(0.290381143857444,1.9602010909893,9.05322593610089));
#45233=CARTESIAN_POINT('Ctrl Pts',(0.27846000916854,1.93581617674233,9.05147834770176));
#45234=CARTESIAN_POINT('Ctrl Pts',(0.264775143928008,1.91455445850191,9.0497665067054));
#45235=CARTESIAN_POINT('Ctrl Pts',(0.243445277099092,1.88865812894333,9.04750186303316));
#45236=CARTESIAN_POINT('Ctrl Pts',(0.237884061857403,1.88241742774186,9.04694088822569));
#45237=CARTESIAN_POINT('Ctrl Pts',(0.227945398587033,1.87210157551521,9.04599533383968));
#45238=CARTESIAN_POINT('Ctrl Pts',(0.223685570082029,1.86791903994608,9.04560635236445));
#45239=CARTESIAN_POINT('Ctrl Pts',(0.217255524220957,1.86194730047875,9.04504566256325));
#45240=CARTESIAN_POINT('Ctrl Pts',(0.215174351774094,1.86006448741249,9.04486806539365));
#45241=CARTESIAN_POINT('Ctrl Pts',(0.212803541462991,1.85797530428771,9.04467033448277));
#45242=CARTESIAN_POINT('Ctrl Pts',(0.2125379306748,1.85774202052125,9.04464824578138));
#45243=CARTESIAN_POINT('Ctrl Pts',(0.212088717189864,1.85734878743746,9.04461099679562));
#45244=CARTESIAN_POINT('Ctrl Pts',(0.211905316868588,1.85718860899648,9.04459581958623));
#45245=CARTESIAN_POINT('Ctrl Pts',(0.211545516882796,1.85687508448724,9.04456610439144));
#45246=CARTESIAN_POINT('Ctrl Pts',(0.211369131633147,1.85672172219908,9.04455156519638));
#45247=CARTESIAN_POINT('Ctrl Pts',(0.211030004580025,1.85642750747307,9.04452366566168));
#45248=CARTESIAN_POINT('Ctrl Pts',(0.210867288988695,1.85628662658034,9.04451030322114));
#45249=CARTESIAN_POINT('Ctrl Pts',(0.210487500401477,1.85595846666311,9.0444791699838));
#45250=CARTESIAN_POINT('Ctrl Pts',(0.210270317852951,1.85577131362137,9.04446140862002));
#45251=CARTESIAN_POINT('Ctrl Pts',(0.209606348590944,1.85520069256718,9.04440723640677));
#45252=CARTESIAN_POINT('Ctrl Pts',(0.209158757354753,1.85481815621063,9.04437089434597));
#45253=CARTESIAN_POINT('Ctrl Pts',(0.205531508013453,1.8517352685052,9.04407777831632));
#45254=CARTESIAN_POINT('Ctrl Pts',(0.202300560411064,1.8490955062827,9.04382534361546));
#45255=CARTESIAN_POINT('Ctrl Pts',(0.181547100657378,1.83280104723667,9.04225115014173));
#45256=CARTESIAN_POINT('Ctrl Pts',(0.16270130230223,1.82092443297682,9.04102735911498));
#45257=CARTESIAN_POINT('Ctrl Pts',(0.121029404880365,1.80033057584383,9.03842561374909));
#45258=CARTESIAN_POINT('Ctrl Pts',(0.0981369415389545,1.79207344374456,
9.03704870673249));
#45259=CARTESIAN_POINT('Ctrl Pts',(0.0734154974143381,1.78619644911943,
9.03550351910789));
#45260=CARTESIAN_POINT('Ctrl Pts',(0.0722928674158459,1.78593592202765,
9.03543324751682));
#45261=CARTESIAN_POINT('Ctrl Pts',(0.0706552562619125,1.78556512961063,
9.03533058278696));
#45262=CARTESIAN_POINT('Ctrl Pts',(0.0701413552161801,1.78545009420212,
9.03529834286745));
#45263=CARTESIAN_POINT('Ctrl Pts',(0.0692400311697343,1.7852506538068,9.03524175733529));
#45264=CARTESIAN_POINT('Ctrl Pts',(0.0688527290332559,1.78516570303121,
9.035217429281));
#45265=CARTESIAN_POINT('Ctrl Pts',(0.0681011762461286,1.78500231072156,
9.0351701954408));
#45266=CARTESIAN_POINT('Ctrl Pts',(0.0677369442102503,1.78492378565796,
9.03514729237321));
#45267=CARTESIAN_POINT('Ctrl Pts',(0.066868251327575,1.78473807943477,9.03509264034739));
#45268=CARTESIAN_POINT('Ctrl Pts',(0.0663636689485715,1.78463147742231,
9.03506087289785));
#45269=CARTESIAN_POINT('Ctrl Pts',(0.0648408445792485,1.78431357018751,
9.03496492944956));
#45270=CARTESIAN_POINT('Ctrl Pts',(0.063821840994417,1.78410598349297,9.03490063471555));
#45271=CARTESIAN_POINT('Ctrl Pts',(0.0532164249663374,1.7819989070027,9.03423047268535));
#45272=CARTESIAN_POINT('Ctrl Pts',(0.043550273294837,1.78053165508633,9.03361088607919));
#45273=CARTESIAN_POINT('Ctrl Pts',(0.00554897002411346,1.77652002141396,
9.03113751115445));
#45274=CARTESIAN_POINT('Ctrl Pts',(-0.0230039376590502,1.7772920234737,
9.02918395385637));
#45275=CARTESIAN_POINT('Ctrl Pts',(-0.0621378739288327,1.78357380052631,
9.02653261276485));
#45276=CARTESIAN_POINT('Ctrl Pts',(-0.0730992921926841,1.7859248409161,
9.02579509619019));
#45277=CARTESIAN_POINT('Ctrl Pts',(-0.0849046541894938,1.78910866601992,
9.02502162414042));
#45278=CARTESIAN_POINT('Ctrl Pts',(-0.0858909613162905,1.78937970981253,
9.02495716554849));
#45279=CARTESIAN_POINT('Ctrl Pts',(-0.0875907078029674,1.78985552656309,
9.02484638280143));
#45280=CARTESIAN_POINT('Ctrl Pts',(-0.0883047542407849,1.79005807495393,
9.0247999362208));
#45281=CARTESIAN_POINT('Ctrl Pts',(-0.0893171112507754,1.79034902542769,
9.02473422265243));
#45282=CARTESIAN_POINT('Ctrl Pts',(-0.0896159965050874,1.79043539351516,
9.02471483858047));
#45283=CARTESIAN_POINT('Ctrl Pts',(-0.0901296263993662,1.79058462201141,
9.0246815571545));
#45284=CARTESIAN_POINT('Ctrl Pts',(-0.0903444311065973,1.79064727339188,
9.02466764753554));
#45285=CARTESIAN_POINT('Ctrl Pts',(-0.0907560797482924,1.79076780292068,
9.02464100877524));
#45286=CARTESIAN_POINT('Ctrl Pts',(-0.0909529333496585,1.79082564524614,
9.02462827754002));
#45287=CARTESIAN_POINT('Ctrl Pts',(-0.0914171584975182,1.79096253221916,
9.02459827212528));
#45288=CARTESIAN_POINT('Ctrl Pts',(-0.0916844834848828,1.79104173607164,
9.02458100731142));
#45289=CARTESIAN_POINT('Ctrl Pts',(-0.0924757061242073,1.79127727924403,
9.02452994743874));
#45290=CARTESIAN_POINT('Ctrl Pts',(-0.0929993124530325,1.79143460591355,
9.02449620977019));
#45291=CARTESIAN_POINT('Ctrl Pts',(-0.0976615504268147,1.79284840203872,
9.02419625066563));
#45292=CARTESIAN_POINT('Ctrl Pts',(-0.101775141995487,1.79418680948757,
9.02393471142627));
#45293=CARTESIAN_POINT('Ctrl Pts',(-0.106070870010879,1.79568076689874,
9.02366367251167));
#45294=CARTESIAN_POINT('Ctrl Pts',(-0.106280882674865,1.79575404837766,
9.02365042703469));
#45295=CARTESIAN_POINT('Ctrl Pts',(-0.106622902779422,1.79587378966598,
9.02362886419469));
#45296=CARTESIAN_POINT('Ctrl Pts',(-0.106754955782624,1.79592011801898,
9.0236205408681));
#45297=CARTESIAN_POINT('Ctrl Pts',(-0.108187752979767,1.79642383678992,
9.0235302529396));
#45298=CARTESIAN_POINT('Ctrl Pts',(-0.109485598642127,1.79688949115594,
9.02344866188049));
#45299=CARTESIAN_POINT('Ctrl Pts',(-0.111181615058106,1.79751031983139,
9.02334224359467));
#45300=CARTESIAN_POINT('Ctrl Pts',(-0.111582503837899,1.79765797021254,
9.0233171044336));
#45301=CARTESIAN_POINT('Ctrl Pts',(-0.113693401612754,1.79844020018005,
9.0231848064235));
#45302=CARTESIAN_POINT('Ctrl Pts',(-0.115398322945125,1.79908850182212,
9.02307820639711));
#45303=CARTESIAN_POINT('Ctrl Pts',(-0.134534306301749,1.80655157786709,
9.02188363831265));
#45304=CARTESIAN_POINT('Ctrl Pts',(-0.151346725007813,1.8148583982693,9.0208502612785));
#45305=CARTESIAN_POINT('Ctrl Pts',(-0.187512548633575,1.83683245761938,
9.01848001257931));
#45306=CARTESIAN_POINT('Ctrl Pts',(-0.206270632575485,1.8512626085099,9.01713761193124));
#45307=CARTESIAN_POINT('Ctrl Pts',(-0.22411424970349,1.86840703063721,9.01563285797275));
#45308=CARTESIAN_POINT('Ctrl Pts',(-0.224939926906504,1.86920890483401,
9.01556267660811));
#45309=CARTESIAN_POINT('Ctrl Pts',(-0.226136895537483,1.87038389181608,
9.01546011952452));
#45310=CARTESIAN_POINT('Ctrl Pts',(-0.226511602865042,1.87075352473119,
9.01542789656799));
#45311=CARTESIAN_POINT('Ctrl Pts',(-0.227166967055043,1.87140318924002,
9.01537133067856));
#45312=CARTESIAN_POINT('Ctrl Pts',(-0.227448016554379,1.87168282461929,
9.01534700526632));
#45313=CARTESIAN_POINT('Ctrl Pts',(-0.227992252469832,1.87222632432509,
9.01529976909432));
#45314=CARTESIAN_POINT('Ctrl Pts',(-0.228255498730688,1.87249012809524,
9.01527686103908));
#45315=CARTESIAN_POINT('Ctrl Pts',(-0.228882151080609,1.87312028996735,
9.01522218523509));
#45316=CARTESIAN_POINT('Ctrl Pts',(-0.229245135157493,1.87348706458689,
9.01519039895804));
#45317=CARTESIAN_POINT('Ctrl Pts',(-0.2303378265689,1.87459648345323,9.01509436151209));
#45318=CARTESIAN_POINT('Ctrl Pts',(-0.231064812175091,1.87534178814511,
9.0150299912858));
#45319=CARTESIAN_POINT('Ctrl Pts',(-0.238609479032454,1.88315193128667,
9.01435694658384));
#45320=CARTESIAN_POINT('Ctrl Pts',(-0.24510387495697,1.89052058553551,9.01373442375532));
#45321=CARTESIAN_POINT('Ctrl Pts',(-0.261372982739389,1.91077380234019,
9.01205260599942));
#45322=CARTESIAN_POINT('Ctrl Pts',(-0.270531293858631,1.92411622972707,
9.01097237938289));
#45323=CARTESIAN_POINT('Ctrl Pts',(-0.286454423578706,1.95151977401775,
9.00883113761967));
#45324=CARTESIAN_POINT('Ctrl Pts',(-0.293278096205452,1.96549905498365,
9.00777401835445));
#45325=CARTESIAN_POINT('Ctrl Pts',(-0.301416414131682,1.98576744852609,
9.00632936518169));
#45326=CARTESIAN_POINT('Ctrl Pts',(-0.303593743880346,1.99168665674952,
9.00591764222151));
#45327=CARTESIAN_POINT('Ctrl Pts',(-0.306533254430586,2.00046483342446,
9.00532553806829));
#45328=CARTESIAN_POINT('Ctrl Pts',(-0.307431933958939,2.00327620275091,
9.0051386393623));
#45329=CARTESIAN_POINT('Ctrl Pts',(-0.308438544093791,2.00658108630446,
9.00492244088721));
#45330=CARTESIAN_POINT('Ctrl Pts',(-0.308584057440197,2.00706287921039,
9.00489100982645));
#45331=CARTESIAN_POINT('Ctrl Pts',(-0.308804604647059,2.00779933701887,
9.00484309965251));
#45332=CARTESIAN_POINT('Ctrl Pts',(-0.308880452607366,2.0080537542709,9.0048265730773));
#45333=CARTESIAN_POINT('Ctrl Pts',(-0.309011945093891,2.00849681919218,
9.00479783523089));
#45334=CARTESIAN_POINT('Ctrl Pts',(-0.309067731145831,2.00868542354199,
9.00478561564598));
#45335=CARTESIAN_POINT('Ctrl Pts',(-0.309193645609045,2.00911255887575,
9.00475797251417));
#45336=CARTESIAN_POINT('Ctrl Pts',(-0.309263670525435,2.00935111951457,
9.00474255512473));
#45337=CARTESIAN_POINT('Ctrl Pts',(-0.309452926383905,2.00999864752818,
9.00470076566954));
#45338=CARTESIAN_POINT('Ctrl Pts',(-0.309571623161641,2.01040777247811,
9.00467442490373));
#45339=CARTESIAN_POINT('Ctrl Pts',(-0.310103373853132,2.01225428872853,
9.00455581883096));
#45340=CARTESIAN_POINT('Ctrl Pts',(-0.310507238955926,2.01369433923061,
9.00446408159209));
#45341=CARTESIAN_POINT('Ctrl Pts',(-0.31842399826761,2.04269795961806,9.00263072165039));
#45342=CARTESIAN_POINT('Ctrl Pts',(-0.322250185622535,2.07114183972887,
9.00108379223631));
#45343=CARTESIAN_POINT('Ctrl Pts',(-0.322292708606286,2.12035583316686,
8.99831611482888));
#45344=CARTESIAN_POINT('Ctrl Pts',(-0.320328910151724,2.1409407739969,8.99713186083544));
#45345=CARTESIAN_POINT('Ctrl Pts',(-0.316165064019319,2.16247010811578,
8.99580001641923));
#45346=CARTESIAN_POINT('Ctrl Pts',(-0.315910768786297,2.16374361302958,
8.99572089933968));
#45347=CARTESIAN_POINT('Ctrl Pts',(-0.315545571964718,2.16551663449504,
8.99561026985634));
#45348=CARTESIAN_POINT('Ctrl Pts',(-0.315441165041495,2.16601748839965,
8.99557896509489));
#45349=CARTESIAN_POINT('Ctrl Pts',(-0.315258883359595,2.16688161270045,
8.99552486179717));
#45350=CARTESIAN_POINT('Ctrl Pts',(-0.315181572043718,2.16724500202043,
8.99550208132881));
#45351=CARTESIAN_POINT('Ctrl Pts',(-0.315020322116303,2.16799654393578,
8.99545490875717));
#45352=CARTESIAN_POINT('Ctrl Pts',(-0.314936294104923,2.16838467654912,
8.99543051382292));
#45353=CARTESIAN_POINT('Ctrl Pts',(-0.314738349805155,2.16929089534494,
8.99537347915603));
#45354=CARTESIAN_POINT('Ctrl Pts',(-0.314623871594004,2.16980885641241,
8.99534082144955));
#45355=CARTESIAN_POINT('Ctrl Pts',(-0.314252121547686,2.17147136423865,
8.99523580911401));
#45356=CARTESIAN_POINT('Ctrl Pts',(-0.313989881200544,2.17261477982269,
8.99516329512414));
#45357=CARTESIAN_POINT('Ctrl Pts',(-0.30986008649212,2.19018070326438,8.99404475084708));
#45358=CARTESIAN_POINT('Ctrl Pts',(-0.30471568917956,2.20627330785332,8.99295680877604));
#45359=CARTESIAN_POINT('Ctrl Pts',(-0.286003041000068,2.25207516615333,
8.98967376032413));
#45360=CARTESIAN_POINT('Ctrl Pts',(-0.269160515135467,2.28021407332836,
8.98739486096164));
#45361=CARTESIAN_POINT('Ctrl Pts',(-0.247449965475695,2.30647478025376,
8.98524051035267));
#45362=CARTESIAN_POINT('Ctrl Pts',(-0.246509136248264,2.307597124822,8.98514842101837));
#45363=CARTESIAN_POINT('Ctrl Pts',(-0.245287000093308,2.30903502524108,
8.98503046383317));
#45364=CARTESIAN_POINT('Ctrl Pts',(-0.245012697250623,2.30935647203548,
8.98500409571169));
#45365=CARTESIAN_POINT('Ctrl Pts',(-0.244576498250371,2.30986560834017,
8.98496233528198));
#45366=CARTESIAN_POINT('Ctrl Pts',(-0.244415017655317,2.31005365077986,
8.9849469124647));
#45367=CARTESIAN_POINT('Ctrl Pts',(-0.244124944600493,2.31039065039245,
8.98491927428553));
#45368=CARTESIAN_POINT('Ctrl Pts',(-0.243996433596923,2.31053967498084,
8.98490705305784));
#45369=CARTESIAN_POINT('Ctrl Pts',(-0.243693544845779,2.31089026260071,
8.98487830344671));
#45370=CARTESIAN_POINT('Ctrl Pts',(-0.243519053745588,2.31109172679994,
8.98486178364085));
#45371=CARTESIAN_POINT('Ctrl Pts',(-0.243011121440188,2.31167670809135,
8.98481381827052));
#45372=CARTESIAN_POINT('Ctrl Pts',(-0.242677020812362,2.31205965545101,
8.9847824215498));
#45373=CARTESIAN_POINT('Ctrl Pts',(-0.240324256752888,2.3147435601289,8.98456238353995));
#45374=CARTESIAN_POINT('Ctrl Pts',(-0.238273720840372,2.31701654455705,
8.98437607272098));
#45375=CARTESIAN_POINT('Ctrl Pts',(-0.231899027474132,2.3238834827933,8.98381206216466));
#45376=CARTESIAN_POINT('Ctrl Pts',(-0.227471905891558,2.3283801998085,8.98344111021582));
#45377=CARTESIAN_POINT('Ctrl Pts',(-0.211525873034527,2.34365281756978,
8.98216294440703));
#45378=CARTESIAN_POINT('Ctrl Pts',(-0.199350304318846,2.35371127627374,
8.98128673834704));
#45379=CARTESIAN_POINT('Ctrl Pts',(-0.166102657100906,2.37730082735027,
8.97900723737632));
#45380=CARTESIAN_POINT('Ctrl Pts',(-0.144109231529997,2.38934083550274,
8.97759673687758));
#45381=CARTESIAN_POINT('Ctrl Pts',(-0.119477176403842,2.39931404240088,
8.97598578725849));
#45382=CARTESIAN_POINT('Ctrl Pts',(-0.118002562302105,2.39989846083276,
8.97588927213166));
#45383=CARTESIAN_POINT('Ctrl Pts',(-0.115946824777426,2.40069568054871,
8.97575459766051));
#45384=CARTESIAN_POINT('Ctrl Pts',(-0.115369295456056,2.40091773648985,
8.97571674930933));
#45385=CARTESIAN_POINT('Ctrl Pts',(-0.114442717035968,2.40127093981285,
8.9756560030889));
#45386=CARTESIAN_POINT('Ctrl Pts',(-0.114094071616117,2.40140314775804,
8.97563314079787));
#45387=CARTESIAN_POINT('Ctrl Pts',(-0.113374343346964,2.40167464427719,
8.97558593383146));
#45388=CARTESIAN_POINT('Ctrl Pts',(-0.113003231529128,2.40181385387506,
8.97556158655962));
#45389=CARTESIAN_POINT('Ctrl Pts',(-0.112139327363209,2.40213610050925,
8.97550489448225));
#45390=CARTESIAN_POINT('Ctrl Pts',(-0.111646343156095,2.40231861673912,
8.97547253234952));
#45391=CARTESIAN_POINT('Ctrl Pts',(-0.110075838821987,2.40289569502334,
8.97536939972284));
#45392=CARTESIAN_POINT('Ctrl Pts',(-0.108996666007821,2.40328570540108,
8.97529847778512));
#45393=CARTESIAN_POINT('Ctrl Pts',(-0.0868648430226985,2.41115071012363,
8.97384280770841));
#45394=CARTESIAN_POINT('Ctrl Pts',(-0.0650979507228045,2.41642084420599,
8.97238249461339));
#45395=CARTESIAN_POINT('Ctrl Pts',(-0.0182843976412439,2.42271818418676,
8.96920744559877));
#45396=CARTESIAN_POINT('Ctrl Pts',(0.00669868180510105,2.42316648092403,
8.9674930727563));
#45397=CARTESIAN_POINT('Ctrl Pts',(0.0349364409174678,2.4203945215587,8.96567083961214));
#45398=CARTESIAN_POINT('Ctrl Pts',(0.0383825767318535,2.41999997588158,
8.9654505767972));
#45399=CARTESIAN_POINT('Ctrl Pts',(0.0423860005883355,2.41947601836279,
8.96519768941333));
#45400=CARTESIAN_POINT('Ctrl Pts',(0.0429499705841629,2.41940068784114,
8.96516213408975));
#45401=CARTESIAN_POINT('Ctrl Pts',(0.0437902246788931,2.41928618778304,
8.96510926699912));
#45402=CARTESIAN_POINT('Ctrl Pts',(0.044066658343582,2.41924815286904,8.96509189154038));
#45403=CARTESIAN_POINT('Ctrl Pts',(0.0445598138381334,2.41917964614282,
8.96506092495953));
#45404=CARTESIAN_POINT('Ctrl Pts',(0.0447765538375248,2.41914931262442,
8.96504732600611));
#45405=CARTESIAN_POINT('Ctrl Pts',(0.0452375734798722,2.41908431243781,
8.96501842313523));
#45406=CARTESIAN_POINT('Ctrl Pts',(0.0454818435490422,2.41904958612513,
8.96500312269235));
#45407=CARTESIAN_POINT('Ctrl Pts',(0.0461393344312507,2.41895534442267,
8.96496197539287));
#45408=CARTESIAN_POINT('Ctrl Pts',(0.0465524816531471,2.41889530629054,
8.96493615821471));
#45409=CARTESIAN_POINT('Ctrl Pts',(0.0485552434214584,2.41860029196252,
8.96481118933897));
#45410=CARTESIAN_POINT('Ctrl Pts',(0.0501432381348293,2.41835422664574,
8.96471265681813));
#45411=CARTESIAN_POINT('Ctrl Pts',(0.0635608965792229,2.41617222399697,
8.96388431309233));
#45412=CARTESIAN_POINT('Ctrl Pts',(0.0752773515315732,2.41358930501394,
8.96318852696976));
#45413=CARTESIAN_POINT('Ctrl Pts',(0.117537622248395,2.40176687051425,8.96069233819842));
#45414=CARTESIAN_POINT('Ctrl Pts',(0.146804152557456,2.38866408124679,8.9589706277231));
#45415=CARTESIAN_POINT('Ctrl Pts',(0.178498312820205,2.36838846429613,8.95674041182552));
#45416=CARTESIAN_POINT('Ctrl Pts',(0.183242155104524,2.36517224922392,8.95639639842107));
#45417=CARTESIAN_POINT('Ctrl Pts',(0.188695261160442,2.36125894847615,8.95598777410386));
#45418=CARTESIAN_POINT('Ctrl Pts',(0.189490371719116,2.36068283168546,8.9559278573092));
#45419=CARTESIAN_POINT('Ctrl Pts',(0.190686374103685,2.35980787585897,8.95583721715207));
#45420=CARTESIAN_POINT('Ctrl Pts',(0.191089228604709,2.35951171906864,8.95580659792171));
#45421=CARTESIAN_POINT('Ctrl Pts',(0.191800513675727,2.35898626659435,8.95575237864401));
#45422=CARTESIAN_POINT('Ctrl Pts',(0.192109227060549,2.35875735391853,8.95572879355539));
#45423=CARTESIAN_POINT('Ctrl Pts',(0.192758361392288,2.35827421523649,8.95567908943722));
#45424=CARTESIAN_POINT('Ctrl Pts',(0.193098690316879,2.35801986733161,8.95565296566828));
#45425=CARTESIAN_POINT('Ctrl Pts',(0.193793265388457,2.35749862647714,8.9555995166495));
#45426=CARTESIAN_POINT('Ctrl Pts',(0.194147465407783,2.35723167382755,8.95557218908974));
#45427=CARTESIAN_POINT('Ctrl Pts',(0.195018847812145,2.35657210730539,8.95550478327031));
#45428=CARTESIAN_POINT('Ctrl Pts',(0.195535395207684,2.35617866121166,8.95546467227329));
#45429=CARTESIAN_POINT('Ctrl Pts',(0.196959371378606,2.35508722482703,8.95535367046186));
#45430=CARTESIAN_POINT('Ctrl Pts',(0.197864268776542,2.35438596134803,8.95528265029677));
#45431=CARTESIAN_POINT('Ctrl Pts',(0.205501478352194,2.3484019908619,8.9546791204128));
#45432=CARTESIAN_POINT('Ctrl Pts',(0.212024090459961,2.34285833187865,8.9541361913825));
#45433=CARTESIAN_POINT('Ctrl Pts',(0.224168486834585,2.33167417619807,8.95306947637679));
#45434=CARTESIAN_POINT('Ctrl Pts',(0.229817181758235,2.32607185168192,8.95254742044238));
#45435=CARTESIAN_POINT('Ctrl Pts',(0.257242519874192,2.29678062415542,8.94988183748435));
#45436=CARTESIAN_POINT('Ctrl Pts',(0.27559034740127,2.27013588003509,8.94763543925744));
#45437=CARTESIAN_POINT('Ctrl Pts',(0.290345347851738,2.23986781376392,8.94550570342855));
#45438=CARTESIAN_POINT('Ctrl Pts',(0.290993322765,2.23851466586678,8.94541134559361));
#45439=CARTESIAN_POINT('Ctrl Pts',(0.29181335448455,2.2367710629973,8.94529089941957));
#45440=CARTESIAN_POINT('Ctrl Pts',(0.291994104369485,2.23638475188741,8.94526428490244));
#45441=CARTESIAN_POINT('Ctrl Pts',(0.292279054024963,2.23577257482244,8.94522222390675));
#45442=CARTESIAN_POINT('Ctrl Pts',(0.292383759300813,2.23554694682571,8.94520674616891));
#45443=CARTESIAN_POINT('Ctrl Pts',(0.292570783243073,2.23514270640986,8.94517906011033));
#45444=CARTESIAN_POINT('Ctrl Pts',(0.292653199038719,2.23496414114858,8.94516684579498));
#45445=CARTESIAN_POINT('Ctrl Pts',(0.292846420927111,2.23454448994531,8.94513817678665));
#45446=CARTESIAN_POINT('Ctrl Pts',(0.292957092615639,2.23430334289164,8.94512173051664));
#45447=CARTESIAN_POINT('Ctrl Pts',(0.29327652698835,2.23360504075043,8.94507418640213));
#45448=CARTESIAN_POINT('Ctrl Pts',(0.293484519488421,2.23314753105111,8.94504313608902));
#45449=CARTESIAN_POINT('Ctrl Pts',(0.294900120369972,2.23001427814458,8.94483115481095));
#45450=CARTESIAN_POINT('Ctrl Pts',(0.296072239614899,2.22732251925763,8.94465236412164));
#45451=CARTESIAN_POINT('Ctrl Pts',(0.299634455832136,2.21882661437801,8.94409727093751));
#45452=CARTESIAN_POINT('Ctrl Pts',(0.301891998853246,2.21296815128478,8.94372783939342));
#45453=CARTESIAN_POINT('Ctrl Pts',(0.30909005691855,2.19252813083278,8.9424723225053));
#45454=CARTESIAN_POINT('Ctrl Pts',(0.313156549867154,2.17766052067162,8.94161596071431));
#45455=CARTESIAN_POINT('Ctrl Pts',(0.321121207420197,2.1374103291937,8.93932219374339));
#45456=CARTESIAN_POINT('Ctrl Pts',(0.323078537173186,2.11176271215937,8.93787820700149));
#45457=CARTESIAN_POINT('Ctrl Pts',(0.321912382753885,2.08464123871511,8.9362318284216));
#45458=CARTESIAN_POINT('Ctrl Pts',(0.321836576388005,2.08312719066163,8.93613956100835));
#45459=CARTESIAN_POINT('Ctrl Pts',(0.32171891920722,2.08106824899228,8.93601358131835));
#45460=CARTESIAN_POINT('Ctrl Pts',(0.32168635952416,2.08052282714623,8.93598016047328));
#45461=CARTESIAN_POINT('Ctrl Pts',(0.321628747941538,2.07959732341589,8.93592336706059));
#45462=CARTESIAN_POINT('Ctrl Pts',(0.321604408881728,2.07921719701158,8.93590001689319));
#45463=CARTESIAN_POINT('Ctrl Pts',(0.321554098679207,2.0784527112016,8.93585300837592));
#45464=CARTESIAN_POINT('Ctrl Pts',(0.32152811215982,2.07806835343854,8.93582934957913));
#45465=CARTESIAN_POINT('Ctrl Pts',(0.321467676195962,2.07719766478742,8.93577569921355));
#45466=CARTESIAN_POINT('Ctrl Pts',(0.321432812234558,2.0767113644711,8.93574569467723));
#45467=CARTESIAN_POINT('Ctrl Pts',(0.321357647312751,2.07569525854642,8.93568291799324));
#45468=CARTESIAN_POINT('Ctrl Pts',(0.321317139388195,2.07516547013787,8.93565013941998));
#45469=CARTESIAN_POINT('Ctrl Pts',(0.321207777936866,2.07378024540166,8.93556430904741));
#45470=CARTESIAN_POINT('Ctrl Pts',(0.321136817598861,2.07292498387878,8.93551119112973));
#45471=CARTESIAN_POINT('Ctrl Pts',(0.320916543076602,2.07039287026271,8.93535355403983));
#45472=CARTESIAN_POINT('Ctrl Pts',(0.320757506625762,2.06871691317103,8.93524873011148));
#45473=CARTESIAN_POINT('Ctrl Pts',(0.319707721563203,2.05850546777471,8.93460701214871));
#45474=CARTESIAN_POINT('Ctrl Pts',(0.318489532873857,2.05000781531759,8.93405990624707));
#45475=CARTESIAN_POINT('Ctrl Pts',(0.314312099914136,2.02734893471528,8.93256479503429));
#45476=CARTESIAN_POINT('Ctrl Pts',(0.310736520749154,2.01332237691127,8.93159992639516));
#45477=CARTESIAN_POINT('Ctrl Pts',(0.29854148451261,1.97613180143265,8.92895885542711));
#45478=CARTESIAN_POINT('Ctrl Pts',(0.28818190441021,1.95363830269271,8.927266313279));
#45479=CARTESIAN_POINT('Ctrl Pts',(0.274629641904422,1.93135336991565,8.92561821836771));
#45480=CARTESIAN_POINT('Ctrl Pts',(0.273896219253183,1.93016482314203,8.92553043246503));
#45481=CARTESIAN_POINT('Ctrl Pts',(0.27293491263177,1.92862940385282,8.9254172130759));
#45482=CARTESIAN_POINT('Ctrl Pts',(0.27271406713878,1.92827817451944,8.92539132672099));
#45483=CARTESIAN_POINT('Ctrl Pts',(0.272374237248879,1.92774002321153,8.92535168458257));
#45484=CARTESIAN_POINT('Ctrl Pts',(0.27225573836794,1.92755279751037,8.92533789673751));
#45485=CARTESIAN_POINT('Ctrl Pts',(0.272020310035568,1.92718167329858,8.92531057398072));
#45486=CARTESIAN_POINT('Ctrl Pts',(0.271903387869235,1.92699777232215,8.92529703879343));
#45487=CARTESIAN_POINT('Ctrl Pts',(0.27164265878354,1.92658860193306,8.92526693226882));
#45488=CARTESIAN_POINT('Ctrl Pts',(0.271498758520322,1.92636339333629,8.92525036730849));
#45489=CARTESIAN_POINT('Ctrl Pts',(0.27107853923966,1.92570753602694,8.92520214247647));
#45490=CARTESIAN_POINT('Ctrl Pts',(0.27080147294032,1.92527736352725,8.92517053226548));
#45491=CARTESIAN_POINT('Ctrl Pts',(0.268816034559599,1.92221084392562,8.92494532654881));
#45492=CARTESIAN_POINT('Ctrl Pts',(0.267070144493558,1.91959882440127,8.92475418797184));
#45493=CARTESIAN_POINT('Ctrl Pts',(0.263025817735089,1.91373555439769,8.92432569909603));
#45494=CARTESIAN_POINT('Ctrl Pts',(0.260704740675812,1.91050048654899,8.92408968293203));
#45495=CARTESIAN_POINT('Ctrl Pts',(0.25509024589099,1.9029736130099,8.92353939919904));
#45496=CARTESIAN_POINT('Ctrl Pts',(0.251747501057024,1.89872001686354,8.92322749953457));
#45497=CARTESIAN_POINT('Ctrl Pts',(0.245814024755871,1.89154895709316,8.92269629141062));
#45498=CARTESIAN_POINT('Ctrl Pts',(0.243274575785754,1.88859079007196,8.92247550361953));
#45499=CARTESIAN_POINT('Ctrl Pts',(0.221823240302397,1.86450094371551,8.92065713405116));
#45500=CARTESIAN_POINT('Ctrl Pts',(0.200253500314111,1.8459058574269,8.91910789502148));
#45501=CARTESIAN_POINT('Ctrl Pts',(0.175953758339042,1.82999643846547,8.91739023868974));
#45502=CARTESIAN_POINT('Ctrl Pts',(0.17537734985347,1.8296216845545,8.91734951742613));
#45503=CARTESIAN_POINT('Ctrl Pts',(0.170118742585208,1.82622667405693,8.9169782062856));
#45504=CARTESIAN_POINT('Ctrl Pts',(0.165360386692497,1.82332662342835,8.91664357027405));
#45505=CARTESIAN_POINT('Ctrl Pts',(0.159685325519364,1.82006657907711,8.91624509712742));
#45506=CARTESIAN_POINT('Ctrl Pts',(0.158839002724313,1.81958549517413,8.91618568965848));
#45507=CARTESIAN_POINT('Ctrl Pts',(0.157556297828978,1.81886402428992,8.91609567093746));
#45508=CARTESIAN_POINT('Ctrl Pts',(0.157121511452811,1.81862079952774,8.91606516168915));
#45509=CARTESIAN_POINT('Ctrl Pts',(0.156357822821913,1.81819590484193,8.91601157864527));
#45510=CARTESIAN_POINT('Ctrl Pts',(0.156029162759445,1.8180137996778,8.91598852049458));
#45511=CARTESIAN_POINT('Ctrl Pts',(0.155329273446141,1.81762760067327,8.91593942104365));
#45512=CARTESIAN_POINT('Ctrl Pts',(0.15495795903092,1.8174236633738,8.91591337420449));
#45513=CARTESIAN_POINT('Ctrl Pts',(0.153991795727045,1.81689549377225,8.91584560480206));
#45514=CARTESIAN_POINT('Ctrl Pts',(0.153396326906438,1.81657240522823,8.91580384156326));
#45515=CARTESIAN_POINT('Ctrl Pts',(0.152096863839651,1.81587263924744,8.91571271172374));
#45516=CARTESIAN_POINT('Ctrl Pts',(0.151392481053797,1.81549669636357,8.91566331931151));
#45517=CARTESIAN_POINT('Ctrl Pts',(0.14933858460968,1.81441027901373,8.9155193078939));
#45518=CARTESIAN_POINT('Ctrl Pts',(0.14798542980885,1.81370676916525,8.9154244434577));
#45519=CARTESIAN_POINT('Ctrl Pts',(0.14336626766393,1.81134674842189,8.91510063054031));
#45520=CARTESIAN_POINT('Ctrl Pts',(0.140077135829765,1.8097363601954,8.91487008302287));
#45521=CARTESIAN_POINT('Ctrl Pts',(0.125637366351748,1.80296910910093,8.91385775288157));
#45522=CARTESIAN_POINT('Ctrl Pts',(0.114225613111398,1.79839670557855,8.91305666183672));
#45523=CARTESIAN_POINT('Ctrl Pts',(0.072302779921104,1.78432030579174,8.91011735455033));
#45524=CARTESIAN_POINT('Ctrl Pts',(0.0406825312678802,1.77871160054212,
8.90788832038193));
#45525=CARTESIAN_POINT('Ctrl Pts',(0.00722131733163397,1.77780226300678,
8.90577055369863));
#45526=CARTESIAN_POINT('Ctrl Pts',(0.00568744959775808,1.77777153712539,
8.90567404666536));
#45527=CARTESIAN_POINT('Ctrl Pts',(0.00372831739244894,1.77774628630985,
8.90555156317903));
#45528=CARTESIAN_POINT('Ctrl Pts',(0.00330323623296926,1.77774164871489,
8.90552503431747));
#45529=CARTESIAN_POINT('Ctrl Pts',(0.00262725833906431,1.77773561151226,
8.90548292316825));
#45530=CARTESIAN_POINT('Ctrl Pts',(0.00237636887303145,1.77773366380311,
8.9054673102258));
#45531=CARTESIAN_POINT('Ctrl Pts',(0.00190721407715574,1.77773056955404,
8.90543814596918));
#45532=CARTESIAN_POINT('Ctrl Pts',(0.00168895151087381,1.77772935177291,
8.90542459077929));
#45533=CARTESIAN_POINT('Ctrl Pts',(0.00119796797696843,1.77772711117085,
8.90539412680842));
#45534=CARTESIAN_POINT('Ctrl Pts',(0.000925247483336966,1.7777262127942,
8.90537722514122));
#45535=CARTESIAN_POINT('Ctrl Pts',(0.000114630137799438,1.77772457149672,
8.90532704559099));
#45536=CARTESIAN_POINT('Ctrl Pts',(-0.000423271175453538,1.77772482905374,
8.90529382373696));
#45537=CARTESIAN_POINT('Ctrl Pts',(-0.00480631989839939,1.77773790140136,
8.90502371724979));
#45538=CARTESIAN_POINT('Ctrl Pts',(-0.00865116152121387,1.77781818563893,
8.90479053599131));
#45539=CARTESIAN_POINT('Ctrl Pts',(-0.0213767894154967,1.77831189967048,
8.90402849727908));
#45540=CARTESIAN_POINT('Ctrl Pts',(-0.030242428481046,1.77902395309238,
8.90351328953682));
#45541=CARTESIAN_POINT('Ctrl Pts',(-0.0474653381832505,1.78112732140132,
8.90252396081068));
#45542=CARTESIAN_POINT('Ctrl Pts',(-0.0558193649145247,1.78248314833279,
8.90204943872156));
#45543=CARTESIAN_POINT('Ctrl Pts',(-0.0664106658111328,1.78463305907576,
8.90144486087313));
#45544=CARTESIAN_POINT('Ctrl Pts',(-0.0687055765129701,1.78512506014655,
8.90131368657694));
#45545=CARTESIAN_POINT('Ctrl Pts',(-0.0787911153721566,1.78740278848947,
8.90073577129273));
#45546=CARTESIAN_POINT('Ctrl Pts',(-0.0865190162529853,1.78945288146303,
8.90028908001325));
#45547=CARTESIAN_POINT('Ctrl Pts',(-0.11228109147801,1.79732351716305,8.89876881473115));
#45548=CARTESIAN_POINT('Ctrl Pts',(-0.129873411024156,1.80444487324056,
8.89767549261018));
#45549=CARTESIAN_POINT('Ctrl Pts',(-0.14788611527399,1.81365660823182,8.89644663602256));
#45550=CARTESIAN_POINT('Ctrl Pts',(-0.149031561792272,1.81425109866493,
8.89636801047566));
#45551=CARTESIAN_POINT('Ctrl Pts',(-0.150624858377512,1.81509021074049,
8.89625795906056));
#45552=CARTESIAN_POINT('Ctrl Pts',(-0.151075755514668,1.81532904597046,
8.89622673797687));
#45553=CARTESIAN_POINT('Ctrl Pts',(-0.151853660469536,1.81574346236267,
8.8961727403337));
#45554=CARTESIAN_POINT('Ctrl Pts',(-0.152180936607668,1.81591853999442,
8.8961499816763));
#45555=CARTESIAN_POINT('Ctrl Pts',(-0.152850934218001,1.81627844785031,
8.89610330576918));
#45556=CARTESIAN_POINT('Ctrl Pts',(-0.153193624537801,1.81646333456774,
8.8960793865355));
#45557=CARTESIAN_POINT('Ctrl Pts',(-0.153990038869609,1.81689487772322,
8.89602369184627));
#45558=CARTESIAN_POINT('Ctrl Pts',(-0.154443505787119,1.81714200409809,
8.8959918996666));
#45559=CARTESIAN_POINT('Ctrl Pts',(-0.155869902550256,1.81792380183361,
8.89589164128323));
#45560=CARTESIAN_POINT('Ctrl Pts',(-0.156840656921119,1.81846240680832,
8.89582303449112));
#45561=CARTESIAN_POINT('Ctrl Pts',(-0.159083827480577,1.81972219035738,
8.89566362230592));
#45562=CARTESIAN_POINT('Ctrl Pts',(-0.160354148208884,1.82044703224143,
8.8955726859007));
#45563=CARTESIAN_POINT('Ctrl Pts',(-0.164613953556208,1.82291625504607,
8.89526549019098));
#45564=CARTESIAN_POINT('Ctrl Pts',(-0.167580177155531,1.82470009417534,
8.89504781023066));
#45565=CARTESIAN_POINT('Ctrl Pts',(-0.178644464480926,1.8315990525726,8.89422126627417));
#45566=CARTESIAN_POINT('Ctrl Pts',(-0.18654123790089,1.83702614128944,8.89360122173697));
#45567=CARTESIAN_POINT('Ctrl Pts',(-0.207516830895129,1.85286233179443,
8.89187054301329));
#45568=CARTESIAN_POINT('Ctrl Pts',(-0.220045777198337,1.86394908401373,
8.89073961128161));
#45569=CARTESIAN_POINT('Ctrl Pts',(-0.24468775366206,1.88942847297504,8.88834181451892));
#45570=CARTESIAN_POINT('Ctrl Pts',(-0.256519209425027,1.9040139292652,8.88707967750188));
#45571=CARTESIAN_POINT('Ctrl Pts',(-0.267638122912724,1.92046659675861,
8.88582830665293));
#45572=CARTESIAN_POINT('Ctrl Pts',(-0.268254903786033,1.9213894896829,8.88575865488878));
#45573=CARTESIAN_POINT('Ctrl Pts',(-0.269075854877119,1.92263172898813,
8.88566564675022));
#45574=CARTESIAN_POINT('Ctrl Pts',(-0.269284238550323,1.92294826148417,
8.88564201204997));
#45575=CARTESIAN_POINT('Ctrl Pts',(-0.269609604586752,1.92344439210727,
8.88560506902315));
#45576=CARTESIAN_POINT('Ctrl Pts',(-0.269726966085424,1.92362373932187,
8.88559173519679));
#45577=CARTESIAN_POINT('Ctrl Pts',(-0.269951952671543,1.92396830469015,
8.88556615806725));
#45578=CARTESIAN_POINT('Ctrl Pts',(-0.270059604253384,1.92413350331689,
8.88555391303651));
#45579=CARTESIAN_POINT('Ctrl Pts',(-0.270314401075191,1.92452529187905,
8.88552491421587));
#45580=CARTESIAN_POINT('Ctrl Pts',(-0.270461412871649,1.92475196786405,
8.88550816947602));
#45581=CARTESIAN_POINT('Ctrl Pts',(-0.270893583714525,1.92542016673176,
8.88545890543826));
#45582=CARTESIAN_POINT('Ctrl Pts',(-0.271177949625862,1.92586220534413,
8.88542643913957));
#45583=CARTESIAN_POINT('Ctrl Pts',(-0.273343522524734,1.92924669479738,
8.88517878765719));
#45584=CARTESIAN_POINT('Ctrl Pts',(-0.275177960780942,1.93221899730117,
8.88496664930818));
#45585=CARTESIAN_POINT('Ctrl Pts',(-0.281372607860134,1.94263106254193,
8.88423977736053));
#45586=CARTESIAN_POINT('Ctrl Pts',(-0.285482604409545,1.95021604135559,
8.88373851046058));
#45587=CARTESIAN_POINT('Ctrl Pts',(-0.303220245512051,1.98634047410008,
8.88143807042266));
#45588=CARTESIAN_POINT('Ctrl Pts',(-0.312903755503468,2.01661899418232,
8.87973653620455));
#45589=CARTESIAN_POINT('Ctrl Pts',(-0.318382667603507,2.05001422405198,
8.87774438373441));
#45590=CARTESIAN_POINT('Ctrl Pts',(-0.318719327775165,2.05220783965774,
8.87761311441661));
#45591=CARTESIAN_POINT('Ctrl Pts',(-0.319758522969623,2.05947915970704,
8.87717642298226));
#45592=CARTESIAN_POINT('Ctrl Pts',(-0.320362541585604,2.06456994318815,
8.87686815458609));
#45593=CARTESIAN_POINT('Ctrl Pts',(-0.32092617521019,2.07053286432804,8.87650341668156));
#45594=CARTESIAN_POINT('Ctrl Pts',(-0.321004015653553,2.07139328870271,
8.87645069831059));
#45595=CARTESIAN_POINT('Ctrl Pts',(-0.321122870811927,2.07276868825779,
8.87636628270478));
#45596=CARTESIAN_POINT('Ctrl Pts',(-0.321166109015685,2.07328347117399,
8.87633465538975));
#45597=CARTESIAN_POINT('Ctrl Pts',(-0.321240332758155,2.0741933860506,8.87627869393556));
#45598=CARTESIAN_POINT('Ctrl Pts',(-0.321271827549024,2.07458847633085,
8.87625437584876));
#45599=CARTESIAN_POINT('Ctrl Pts',(-0.321331007833172,2.07534856953882,
8.87620755406841));
#45600=CARTESIAN_POINT('Ctrl Pts',(-0.32135880045428,2.07571356370952,8.87618505378024));
#45601=CARTESIAN_POINT('Ctrl Pts',(-0.321416849642537,2.07649345942085,
8.87613694078914));
#45602=CARTESIAN_POINT('Ctrl Pts',(-0.321446924801162,2.07690837343497,
8.87611132242547));
#45603=CARTESIAN_POINT('Ctrl Pts',(-0.321517156069859,2.07790400877492,
8.87604979563889));
#45604=CARTESIAN_POINT('Ctrl Pts',(-0.321556542209109,2.07848478141234,
8.8760138630883));
#45605=CARTESIAN_POINT('Ctrl Pts',(-0.32165802359338,2.08004374299165,8.87591729333295));
#45606=CARTESIAN_POINT('Ctrl Pts',(-0.321717229749107,2.08102210801356,
8.87585656561722));
#45607=CARTESIAN_POINT('Ctrl Pts',(-0.322110117426355,2.08804573548621,
8.87541970523543));
#45608=CARTESIAN_POINT('Ctrl Pts',(-0.322277825444617,2.09409865735488,
8.8750384054719));
#45609=CARTESIAN_POINT('Ctrl Pts',(-0.322274963997748,2.10015233269624,
8.8746519335206));
#45610=CARTESIAN_POINT('',(-0.322274890249976,2.09973403126875,8.62424191572231));
#45611=CARTESIAN_POINT('Ctrl Pts',(-0.322274964147435,2.10015201568935,
8.87465195375859));
#45612=CARTESIAN_POINT('Ctrl Pts',(-0.322258391129396,2.1352869995652,8.87240890655654));
#45613=CARTESIAN_POINT('Ctrl Pts',(-0.316495278814541,2.17018327590654,
8.86997185423784));
#45614=CARTESIAN_POINT('Ctrl Pts',(-0.303201477941531,2.20940561370631,
8.86723288440724));
#45615=CARTESIAN_POINT('Ctrl Pts',(-0.301008738192233,2.21530167007367,
8.86682227231232));
#45616=CARTESIAN_POINT('Ctrl Pts',(-0.297538892961549,2.22385652456047,
8.86623183913865));
#45617=CARTESIAN_POINT('Ctrl Pts',(-0.296395750444973,2.22656773728122,
8.86604552801538));
#45618=CARTESIAN_POINT('Ctrl Pts',(-0.295013894593567,2.22972366974637,
8.86582993012531));
#45619=CARTESIAN_POINT('Ctrl Pts',(-0.294811119235905,2.23018384108156,
8.8657985254511));
#45620=CARTESIAN_POINT('Ctrl Pts',(-0.29449968156297,2.23088614753796,8.86575064715497));
#45621=CARTESIAN_POINT('Ctrl Pts',(-0.294391797015212,2.23112862353198,
8.86573412616783));
#45622=CARTESIAN_POINT('Ctrl Pts',(-0.294203441482384,2.23155055805761,
8.86570539444121));
#45623=CARTESIAN_POINT('Ctrl Pts',(-0.294123105971324,2.23173007568437,
8.86569317539954));
#45624=CARTESIAN_POINT('Ctrl Pts',(-0.293953866619167,2.23210733109096,
8.86566750822513));
#45625=CARTESIAN_POINT('Ctrl Pts',(-0.293864927857752,2.23230505207344,
8.86565406233586));
#45626=CARTESIAN_POINT('Ctrl Pts',(-0.293614936321597,2.23285931602285,
8.86561638744191));
#45627=CARTESIAN_POINT('Ctrl Pts',(-0.293453433029836,2.23321565723309,
8.86559218621455));
#45628=CARTESIAN_POINT('Ctrl Pts',(-0.292792392733212,2.23466714243999,
8.8654936866138));
#45629=CARTESIAN_POINT('Ctrl Pts',(-0.292287362768263,2.23575979584757,
8.86541972206155));
#45630=CARTESIAN_POINT('Ctrl Pts',(-0.283205356135972,2.2551234858498,8.86411178006015));
#45631=CARTESIAN_POINT('Ctrl Pts',(-0.27293520880172,2.27255494296648,8.8629778907046));
#45632=CARTESIAN_POINT('Ctrl Pts',(-0.251610402689442,2.30202832183549,
8.86094267409749));
#45633=CARTESIAN_POINT('Ctrl Pts',(-0.241146535991518,2.31440978391395,
8.8600426420395));
#45634=CARTESIAN_POINT('Ctrl Pts',(-0.223920133129191,2.33192933691747,
8.85863237868484));
#45635=CARTESIAN_POINT('Ctrl Pts',(-0.217812387476607,2.33767454884246,
8.85814427240509));
#45636=CARTESIAN_POINT('Ctrl Pts',(-0.208804240202796,2.34550888985677,
8.85743515123233));
#45637=CARTESIAN_POINT('Ctrl Pts',(-0.206082137876216,2.34779825803244,
8.85722220078001));
#45638=CARTESIAN_POINT('Ctrl Pts',(-0.202164859817855,2.35098360985124,
8.85691731034613));
#45639=CARTESIAN_POINT('Ctrl Pts',(-0.201000427174315,2.35191711160528,
8.8568268713154));
#45640=CARTESIAN_POINT('Ctrl Pts',(-0.198944692864906,2.35354182473953,
8.8566675173254));
#45641=CARTESIAN_POINT('Ctrl Pts',(-0.198056162076588,2.35423651257091,
8.85659874174787));
#45642=CARTESIAN_POINT('Ctrl Pts',(-0.196752533285843,2.35524475873978,
8.85649797472096));
#45643=CARTESIAN_POINT('Ctrl Pts',(-0.196340286842383,2.35556200417152,
8.85646612928448));
#45644=CARTESIAN_POINT('Ctrl Pts',(-0.195617632044584,2.35611534462456,
8.85641033955645));
#45645=CARTESIAN_POINT('Ctrl Pts',(-0.195307559037038,2.35635187750379,
8.85638641258563));
#45646=CARTESIAN_POINT('Ctrl Pts',(-0.194702369016668,2.35681179903014,
8.85633973376936));
#45647=CARTESIAN_POINT('Ctrl Pts',(-0.194407294873696,2.35703524334207,
8.85631698416082));
#45648=CARTESIAN_POINT('Ctrl Pts',(-0.193707701939626,2.35756311487901,
8.85626306957427));
#45649=CARTESIAN_POINT('Ctrl Pts',(-0.193302850334388,2.35786709752282,
8.85623188724451));
#45650=CARTESIAN_POINT('Ctrl Pts',(-0.191882133025795,2.35892861660629,
8.85612252226931));
#45651=CARTESIAN_POINT('Ctrl Pts',(-0.190862527056998,2.35968110667515,
8.85604414314863));
#45652=CARTESIAN_POINT('Ctrl Pts',(-0.176489233984687,2.37015851064257,
8.85494068431225));
#45653=CARTESIAN_POINT('Ctrl Pts',(-0.162413757944563,2.37884706693344,
8.85387552979629));
#45654=CARTESIAN_POINT('Ctrl Pts',(-0.140168012870308,2.39032158777346,
8.85221547139683));
#45655=CARTESIAN_POINT('Ctrl Pts',(-0.132448189165778,2.39392373387985,
8.85164371513995));
#45656=CARTESIAN_POINT('Ctrl Pts',(-0.109471094890872,2.40355590560844,
8.84996179006769));
#45657=CARTESIAN_POINT('Ctrl Pts',(-0.0938848563783912,2.40873252822349,
8.84884450845167));
#45658=CARTESIAN_POINT('Ctrl Pts',(-0.0719279392973073,2.41420749284543,
8.84734844953099));
#45659=CARTESIAN_POINT('Ctrl Pts',(-0.0658410652126833,2.4155391290063,
8.84694188310539));
#45660=CARTESIAN_POINT('Ctrl Pts',(-0.0568570630955382,2.41723324549202,
8.84635729458988));
#45661=CARTESIAN_POINT('Ctrl Pts',(-0.0539877986153758,2.41773412899398,
8.84617288876034));
#45662=CARTESIAN_POINT('Ctrl Pts',(-0.050616877067789,2.41827560206698,
8.84595923930876));
#45663=CARTESIAN_POINT('Ctrl Pts',(-0.0501215473080758,2.4183539816285,
8.84592792090021));
#45664=CARTESIAN_POINT('Ctrl Pts',(-0.0493640942356354,2.41847202719149,
8.84588014683649));
#45665=CARTESIAN_POINT('Ctrl Pts',(-0.0491021044189213,2.41851252604255,
8.8458636441319));
#45666=CARTESIAN_POINT('Ctrl Pts',(-0.048645689122768,2.41858250301045,
8.84583493240884));
#45667=CARTESIAN_POINT('Ctrl Pts',(-0.0484512872049761,2.41861212635975,
8.84582271512735));
#45668=CARTESIAN_POINT('Ctrl Pts',(-0.0480107533808782,2.41867884325877,
8.84579505670633));
#45669=CARTESIAN_POINT('Ctrl Pts',(-0.0477646060570305,2.41871582952556,
8.84577962176556));
#45670=CARTESIAN_POINT('Ctrl Pts',(-0.0470958140158975,2.41881553049978,
8.84573773580946));
#45671=CARTESIAN_POINT('Ctrl Pts',(-0.0466730851405237,2.41887769021074,
8.8457113163409));
#45672=CARTESIAN_POINT('Ctrl Pts',(-0.0447585058983298,2.41915532866074,
8.84559190724501));
#45673=CARTESIAN_POINT('Ctrl Pts',(-0.0432652473613167,2.41936118461947,
8.84549945443645));
#45674=CARTESIAN_POINT('Ctrl Pts',(-0.010703100775816,2.42361751806054,
8.84349712853597));
#45675=CARTESIAN_POINT('Ctrl Pts',(0.0207963479565396,2.42312711933527,
8.84181961176984));
#45676=CARTESIAN_POINT('Ctrl Pts',(0.0627563563993194,2.416302898963,8.83941420827099));
#45677=CARTESIAN_POINT('Ctrl Pts',(0.07367735903237,2.41393868726541,8.83877345348209));
#45678=CARTESIAN_POINT('Ctrl Pts',(0.0890711320598588,2.40975862927589,
8.83783402705313));
#45679=CARTESIAN_POINT('Ctrl Pts',(0.0936605350674244,2.40840197086546,
8.83754928513161));
#45680=CARTESIAN_POINT('Ctrl Pts',(0.099988903899937,2.40637697769911,8.83714933946639));
#45681=CARTESIAN_POINT('Ctrl Pts',(0.101754976879823,2.40579496043265,8.83703692652034));
#45682=CARTESIAN_POINT('Ctrl Pts',(0.104390170740409,2.40490116461715,8.83686795344129));
#45683=CARTESIAN_POINT('Ctrl Pts',(0.105263169643407,2.4046008749513,8.83681177057736));
#45684=CARTESIAN_POINT('Ctrl Pts',(0.106662195909936,2.40411291242285,8.83672140087538));
#45685=CARTESIAN_POINT('Ctrl Pts',(0.107189050990016,2.40392761454058,8.83668729261168));
#45686=CARTESIAN_POINT('Ctrl Pts',(0.108188962679898,2.40357301662697,8.83662241290063));
#45687=CARTESIAN_POINT('Ctrl Pts',(0.108662110704774,2.40340397782893,8.83659165019409));
#45688=CARTESIAN_POINT('Ctrl Pts',(0.109500333444407,2.40310229869367,8.83653704010925));
#45689=CARTESIAN_POINT('Ctrl Pts',(0.10986556812357,2.40297010320586,8.83651320758313));
#45690=CARTESIAN_POINT('Ctrl Pts',(0.110580971958508,2.40270970139934,8.83646645159755));
#45691=CARTESIAN_POINT('Ctrl Pts',(0.110931159470307,2.40258154692136,8.83644352989701));
#45692=CARTESIAN_POINT('Ctrl Pts',(0.111766189101242,2.40227431538224,8.83638878909601));
#45693=CARTESIAN_POINT('Ctrl Pts',(0.11225082326147,2.40209467959262,8.8363569513661));
#45694=CARTESIAN_POINT('Ctrl Pts',(0.113980941618331,2.40144865123023,8.83624305026901));
#45695=CARTESIAN_POINT('Ctrl Pts',(0.115223955262968,2.40097572066402,8.83616076829903));
#45696=CARTESIAN_POINT('Ctrl Pts',(0.13754296612354,2.39232545996975,8.83467513619296));
#45697=CARTESIAN_POINT('Ctrl Pts',(0.15769937683074,2.38196234921396,8.83319439165369));
#45698=CARTESIAN_POINT('Ctrl Pts',(0.189249583749443,2.36129362961791,8.83065656739356));
#45699=CARTESIAN_POINT('Ctrl Pts',(0.201297763568959,2.35212888610402,8.82962637665499));
#45700=CARTESIAN_POINT('Ctrl Pts',(0.221198742087984,2.33465185199917,8.82785376456689));
#45701=CARTESIAN_POINT('Ctrl Pts',(0.229337661131533,2.3267039288392,8.82710492717565));
#45702=CARTESIAN_POINT('Ctrl Pts',(0.238098718966128,2.31719257869832,8.82628681525841));
#45703=CARTESIAN_POINT('Ctrl Pts',(0.239148793768166,2.31603580927408,8.82618855201648));
#45704=CARTESIAN_POINT('Ctrl Pts',(0.240466090493364,2.3145632910722,8.82606507154993));
#45705=CARTESIAN_POINT('Ctrl Pts',(0.240741149469571,2.31425462774352,8.82603927634103));
#45706=CARTESIAN_POINT('Ctrl Pts',(0.241178805207112,2.31376159610902,8.82599821509051));
#45707=CARTESIAN_POINT('Ctrl Pts',(0.241341785143525,2.31357757091257,8.82598292025497));
#45708=CARTESIAN_POINT('Ctrl Pts',(0.241649577653699,2.31322923161248,8.82595402839717));
#45709=CARTESIAN_POINT('Ctrl Pts',(0.241794432083298,2.31306495771965,8.8259404282607));
#45710=CARTESIAN_POINT('Ctrl Pts',(0.242124456874303,2.31268991917092,8.82590943586624));
#45711=CARTESIAN_POINT('Ctrl Pts',(0.242309519241405,2.31247906066255,8.82589205177167));
#45712=CARTESIAN_POINT('Ctrl Pts',(0.242874056093596,2.31183413538602,8.82583900487923));
#45713=CARTESIAN_POINT('Ctrl Pts',(0.243252643928795,2.31139928872137,8.82580340814456));
#45714=CARTESIAN_POINT('Ctrl Pts',(0.246000278779147,2.30822619621829,8.82554487652267));
#45715=CARTESIAN_POINT('Ctrl Pts',(0.248324314629643,2.30544907736837,8.82532519598492));
#45716=CARTESIAN_POINT('Ctrl Pts',(0.268295082413906,2.28075077150841,8.82342245628961));
#45717=CARTESIAN_POINT('Ctrl Pts',(0.283049220727119,2.25664198318754,8.82190292955994));
#45718=CARTESIAN_POINT('Ctrl Pts',(0.301411122958605,2.2153396298116,8.81935047247661));
#45719=CARTESIAN_POINT('Ctrl Pts',(0.307089414477461,2.19923643556888,8.81836789228067));
#45720=CARTESIAN_POINT('Ctrl Pts',(0.311905691228041,2.18111061368538,8.81723751338018));
#45721=CARTESIAN_POINT('Ctrl Pts',(0.312331101845052,2.17945674622789,8.81713417676748));
#45722=CARTESIAN_POINT('Ctrl Pts',(0.312952698447476,2.17695801616957,8.81697772485113));
#45723=CARTESIAN_POINT('Ctrl Pts',(0.313158655537868,2.17611559733112,8.81692492310101));
#45724=CARTESIAN_POINT('Ctrl Pts',(0.313486194032711,2.17475204431786,8.81683936336113));
#45725=CARTESIAN_POINT('Ctrl Pts',(0.31360988302727,2.17423141680598,8.81680667311262));
#45726=CARTESIAN_POINT('Ctrl Pts',(0.313844429535547,2.17323312180967,8.81674394673153));
#45727=CARTESIAN_POINT('Ctrl Pts',(0.313955494735914,2.17275550426882,8.81671391736054));
#45728=CARTESIAN_POINT('Ctrl Pts',(0.314151873092776,2.17190218831735,8.81666023202597));
#45729=CARTESIAN_POINT('Ctrl Pts',(0.314237603619513,2.17152658611943,8.81663658952335));
#45730=CARTESIAN_POINT('Ctrl Pts',(0.314406494761794,2.17078047660374,8.81658960114287));
#45731=CARTESIAN_POINT('Ctrl Pts',(0.314489674473583,2.17040997418143,8.81656625591905));
#45732=CARTESIAN_POINT('Ctrl Pts',(0.314690014970887,2.16951017183316,8.81650953071797));
#45733=CARTESIAN_POINT('Ctrl Pts',(0.314806495105262,2.1689807229917,8.81647612896315));
#45734=CARTESIAN_POINT('Ctrl Pts',(0.315237647551024,2.16699712503661,8.81635089539432));
#45735=CARTESIAN_POINT('Ctrl Pts',(0.315543580943449,2.16554111383636,8.81625878416259));
#45736=CARTESIAN_POINT('Ctrl Pts',(0.320829598311132,2.13948847596449,8.81460714097402));
#45737=CARTESIAN_POINT('Ctrl Pts',(0.322928907278759,2.11440064866209,8.81295085521546));
#45738=CARTESIAN_POINT('Ctrl Pts',(0.321575294586588,2.07354295150555,8.81019005788158));
#45739=CARTESIAN_POINT('Ctrl Pts',(0.319892513314197,2.05781640879362,8.80911470829689));
#45740=CARTESIAN_POINT('Ctrl Pts',(0.315922015802501,2.03600736377452,8.80764769451655));
#45741=CARTESIAN_POINT('Ctrl Pts',(0.314594957788282,2.02977321384923,8.80723137527691));
#45742=CARTESIAN_POINT('Ctrl Pts',(0.312369426940675,2.0206552222702,8.80663079307427));
#45743=CARTESIAN_POINT('Ctrl Pts',(0.311613989060734,2.01773836817381,8.80643994202002));
#45744=CARTESIAN_POINT('Ctrl Pts',(0.310683984893116,2.01434433315743,8.80621970739463));
#45745=CARTESIAN_POINT('Ctrl Pts',(0.310549095406724,2.01385656681047,8.8061881014509));
#45746=CARTESIAN_POINT('Ctrl Pts',(0.310341533513148,2.01311283756492,8.80613998005061));
#45747=CARTESIAN_POINT('Ctrl Pts',(0.310269692920295,2.01285664640556,8.80612341648813));
#45748=CARTESIAN_POINT('Ctrl Pts',(0.310144180310748,2.01241117793715,8.80609463807247));
#45749=CARTESIAN_POINT('Ctrl Pts',(0.310090652391283,2.01222186131375,8.80608241482701));
#45750=CARTESIAN_POINT('Ctrl Pts',(0.309969205618494,2.01179382793134,8.80605479491235));
#45751=CARTESIAN_POINT('Ctrl Pts',(0.309901184488626,2.01155514104082,8.80603940433732));
#45752=CARTESIAN_POINT('Ctrl Pts',(0.30971620053363,2.01090886373348,8.80599776224506));
#45753=CARTESIAN_POINT('Ctrl Pts',(0.309598708370879,2.01050142339561,8.8059715416524));
#45754=CARTESIAN_POINT('Ctrl Pts',(0.309068163660543,2.00867514278023,8.80585415255439));
#45755=CARTESIAN_POINT('Ctrl Pts',(0.308646150980751,2.00725889252491,8.80576349900202));
#45756=CARTESIAN_POINT('Ctrl Pts',(0.298723920763738,1.97477848725974,8.80369212014311));
#45757=CARTESIAN_POINT('Ctrl Pts',(0.284589220661479,1.94531893942745,8.8019607846075));
#45758=CARTESIAN_POINT('Ctrl Pts',(0.257658652035014,1.90581537589126,8.79924753053001));
#45759=CARTESIAN_POINT('Ctrl Pts',(0.248143700584506,1.89379558218733,8.79835979927943));
#45760=CARTESIAN_POINT('Ctrl Pts',(0.236726227343944,1.88131197069719,8.79733926168038));
#45761=CARTESIAN_POINT('Ctrl Pts',(0.235632236138761,1.88013365418685,8.79724190235935));
#45762=CARTESIAN_POINT('Ctrl Pts',(0.233960342745177,1.87835970074025,8.7970937274901));
#45763=CARTESIAN_POINT('Ctrl Pts',(0.233388871081552,1.87775801686327,8.79704318684502));
#45764=CARTESIAN_POINT('Ctrl Pts',(0.2324559235661,1.87678331373997,8.79696084756931));
#45765=CARTESIAN_POINT('Ctrl Pts',(0.232095856035157,1.87640894688689,8.79692910986779));
#45766=CARTESIAN_POINT('Ctrl Pts',(0.231401749737383,1.87569075891015,8.79686800610749));
#45767=CARTESIAN_POINT('Ctrl Pts',(0.231067845576486,1.87534680915566,8.79683864594794));
#45768=CARTESIAN_POINT('Ctrl Pts',(0.230464917885386,1.87472850848115,8.79678569136082));
#45769=CARTESIAN_POINT('Ctrl Pts',(0.230196168241127,1.87445389076271,8.79676210895446));
#45770=CARTESIAN_POINT('Ctrl Pts',(0.229657245024002,1.87390516688515,8.79671486204584));
#45771=CARTESIAN_POINT('Ctrl Pts',(0.229387070259408,1.87363106275585,8.79669119750977));
#45772=CARTESIAN_POINT('Ctrl Pts',(0.228638518691238,1.87287434059298,8.79662569077882));
#45773=CARTESIAN_POINT('Ctrl Pts',(0.228159107517079,1.87239275267227,8.79658380292305));
#45774=CARTESIAN_POINT('Ctrl Pts',(0.226270216922729,1.87050725028489,8.79641901884803));
#45775=CARTESIAN_POINT('Ctrl Pts',(0.224849296983503,1.86911490607044,8.79629561419394));
#45776=CARTESIAN_POINT('Ctrl Pts',(0.198302798233882,1.84357974910357,8.79399990217424));
#45777=CARTESIAN_POINT('Ctrl Pts',(0.169442811289288,1.82366111070891,8.79162741423922));
#45778=CARTESIAN_POINT('Ctrl Pts',(0.129260022952872,1.804625836683,8.78863726731228));
#45779=CARTESIAN_POINT('Ctrl Pts',(0.120369320674749,1.80089248638821,8.78799554522044));
#45780=CARTESIAN_POINT('Ctrl Pts',(0.106569656358533,1.79581296736276,8.78704195618732));
#45781=CARTESIAN_POINT('Ctrl Pts',(0.101774320886311,1.79417515262052,8.78671817614134));
#45782=CARTESIAN_POINT('Ctrl Pts',(0.0963975791075244,1.7924792555061,8.78636504808064));
#45783=CARTESIAN_POINT('Ctrl Pts',(0.0958526596333032,1.79230897119842,
8.78632937169529));
#45784=CARTESIAN_POINT('Ctrl Pts',(0.095040361381617,1.79205749983083,8.78627635988433));
#45785=CARTESIAN_POINT('Ctrl Pts',(0.09477332859457,1.79197521221416,8.78625896025765));
#45786=CARTESIAN_POINT('Ctrl Pts',(0.0943164914383339,1.79183508564711,
8.7862292402805));
#45787=CARTESIAN_POINT('Ctrl Pts',(0.0941267406500158,1.79177707468323,
8.78621690976533));
#45788=CARTESIAN_POINT('Ctrl Pts',(0.0937356731449697,1.79165791161053,
8.78619152589889));
#45789=CARTESIAN_POINT('Ctrl Pts',(0.0935343506301318,1.79159678155836,
8.78617847387446));
#45790=CARTESIAN_POINT('Ctrl Pts',(0.0930472530323935,1.79144939890752,
8.78614693217058));
#45791=CARTESIAN_POINT('Ctrl Pts',(0.092761417052072,1.79136334592346,8.78612845425707));
#45792=CARTESIAN_POINT('Ctrl Pts',(0.0917028979281487,1.79104627443141,
8.78606014021439));
#45793=CARTESIAN_POINT('Ctrl Pts',(0.0909294595890927,1.79081775690899,
8.78601044942425));
#45794=CARTESIAN_POINT('Ctrl Pts',(0.089729128387491,1.79046800479038,8.78593366876171));
#45795=CARTESIAN_POINT('Ctrl Pts',(0.0893028361319464,1.79034474652656,
8.78590646610379));
#45796=CARTESIAN_POINT('Ctrl Pts',(0.0705567198958229,1.78496642010374,
8.78471306299879));
#45797=CARTESIAN_POINT('Ctrl Pts',(0.0518038871183008,1.78134501789541,
8.78363676641466));
#45798=CARTESIAN_POINT('Ctrl Pts',(0.0163415571590964,1.77771266067331,
8.78164007620568));
#45799=CARTESIAN_POINT('Ctrl Pts',(-0.00026084758930146,1.77729876995707,
8.78072030726044));
#45800=CARTESIAN_POINT('Ctrl Pts',(-0.0234212244586126,1.77850924056617,
8.77939282038124));
#45801=CARTESIAN_POINT('Ctrl Pts',(-0.0300093092717888,1.7790571762351,
8.77901036164657));
#45802=CARTESIAN_POINT('Ctrl Pts',(-0.0443812583346605,1.78069888440511,
8.77816089752917));
#45803=CARTESIAN_POINT('Ctrl Pts',(-0.0521511147974133,1.78187558405598,
8.77769182383107));
#45804=CARTESIAN_POINT('Ctrl Pts',(-0.06084379941978,1.78351905215076,8.7771532245498));
#45805=CARTESIAN_POINT('Ctrl Pts',(-0.0618169696195012,1.7837076976719,
8.77709273178213));
#45806=CARTESIAN_POINT('Ctrl Pts',(-0.0632749158934978,1.78399730091927,
8.77700180710472));
#45807=CARTESIAN_POINT('Ctrl Pts',(-0.0637603611104964,1.78409489216793,
8.77697148273713));
#45808=CARTESIAN_POINT('Ctrl Pts',(-0.0645939163711931,1.78426446516969,
8.77691932695503));
#45809=CARTESIAN_POINT('Ctrl Pts',(-0.0649421367797968,1.78433590502632,
8.77689751290146));
#45810=CARTESIAN_POINT('Ctrl Pts',(-0.0656581858047297,1.78448404249139,
8.77685260305325));
#45811=CARTESIAN_POINT('Ctrl Pts',(-0.066025999823081,1.78456080752189,
8.77682950512842));
#45812=CARTESIAN_POINT('Ctrl Pts',(-0.0669098422248169,1.78474688443507,
8.77677393157729));
#45813=CARTESIAN_POINT('Ctrl Pts',(-0.0674257368630267,1.7848568200593,
8.77674143601491));
#45814=CARTESIAN_POINT('Ctrl Pts',(-0.0690042458680478,1.7851972491294,
8.77664183012726));
#45815=CARTESIAN_POINT('Ctrl Pts',(-0.0700659573848188,1.78543185241864,
8.77657458817877));
#45816=CARTESIAN_POINT('Ctrl Pts',(-0.082566391742672,1.78826046147643,
8.77577994070802));
#45817=CARTESIAN_POINT('Ctrl Pts',(-0.0938551195217636,1.79147138157918,
8.77503265697865));
#45818=CARTESIAN_POINT('Ctrl Pts',(-0.126411536034841,1.80268387264365,
8.77278632326269));
#45819=CARTESIAN_POINT('Ctrl Pts',(-0.1470369931003,1.81232543847618,8.77123987428361));
#45820=CARTESIAN_POINT('Ctrl Pts',(-0.172361167921185,1.82760312257363,
8.76924582197477));
#45821=CARTESIAN_POINT('Ctrl Pts',(-0.178132371198043,1.83134167248001,
8.76878482155745));
#45822=CARTESIAN_POINT('Ctrl Pts',(-0.189014416591842,1.83889593622301,
8.76790812777038));
#45823=CARTESIAN_POINT('Ctrl Pts',(-0.194140493756881,1.8426845090545,8.7674917744631));
#45824=CARTESIAN_POINT('Ctrl Pts',(-0.201523900810356,1.84848777219601,
8.76689082340601));
#45825=CARTESIAN_POINT('Ctrl Pts',(-0.203870408830755,1.85038601531031,
8.76669964554213));
#45826=CARTESIAN_POINT('Ctrl Pts',(-0.206579118315824,1.8526409495547,8.76647907745942));
#45827=CARTESIAN_POINT('Ctrl Pts',(-0.206967469610177,1.85296579489306,
8.76644745725479));
#45828=CARTESIAN_POINT('Ctrl Pts',(-0.207558777567178,1.85346278110653,
8.76639931863389));
#45829=CARTESIAN_POINT('Ctrl Pts',(-0.207762286952613,1.85363425853752,
8.76638275205903));
#45830=CARTESIAN_POINT('Ctrl Pts',(-0.208130462193819,1.85394526439354,
8.76635278350851));
#45831=CARTESIAN_POINT('Ctrl Pts',(-0.208295199655007,1.85408470562236,
8.76633937524737));
#45832=CARTESIAN_POINT('Ctrl Pts',(-0.208628859770835,1.85436770644124,
8.76631222004208));
#45833=CARTESIAN_POINT('Ctrl Pts',(-0.208797773646535,1.85451127421165,
8.76629847382842));
#45834=CARTESIAN_POINT('Ctrl Pts',(-0.209282801073053,1.85492438436248,
8.76625900466414));
#45835=CARTESIAN_POINT('Ctrl Pts',(-0.209598543240732,1.85519436509539,
8.76623331401213));
#45836=CARTESIAN_POINT('Ctrl Pts',(-0.210977006731922,1.85637766568778,
8.76612116226935));
#45837=CARTESIAN_POINT('Ctrl Pts',(-0.212034307586033,1.85729731826864,
8.76603516169694));
#45838=CARTESIAN_POINT('Ctrl Pts',(-0.231625129293555,1.87456338071227,
8.76444131186564));
#45839=CARTESIAN_POINT('Ctrl Pts',(-0.248227157922096,1.89298411282596,
8.76308102414789));
#45840=CARTESIAN_POINT('Ctrl Pts',(-0.270933930250317,1.92488736559119,
8.76089030280159));
#45841=CARTESIAN_POINT('Ctrl Pts',(-0.278505580799067,1.93719880935376,
8.7600782001685));
#45842=CARTESIAN_POINT('Ctrl Pts',(-0.28921599575796,1.95756142340511,8.75874263545194));
#45843=CARTESIAN_POINT('Ctrl Pts',(-0.292901504601842,1.9653028217717,8.75823672268849));
#45844=CARTESIAN_POINT('Ctrl Pts',(-0.297277709638582,1.97552652468542,
8.75756628403663));
#45845=CARTESIAN_POINT('Ctrl Pts',(-0.298253612942771,1.97788339795675,
8.75741158416918));
#45846=CARTESIAN_POINT('Ctrl Pts',(-0.299468108151004,1.9809179149308,8.75721213802128));
#45847=CARTESIAN_POINT('Ctrl Pts',(-0.299732573996378,1.9815851577869,8.75716826657549));
#45848=CARTESIAN_POINT('Ctrl Pts',(-0.300154169411509,1.98265929750893,
8.7570976132096));
#45849=CARTESIAN_POINT('Ctrl Pts',(-0.300312706761918,1.98306564221505,
8.75707087870232));
#45850=CARTESIAN_POINT('Ctrl Pts',(-0.300612479680231,1.98383861635501,
8.757020009813));
#45851=CARTESIAN_POINT('Ctrl Pts',(-0.300753870790224,1.98420518495053,
8.75699588070884));
#45852=CARTESIAN_POINT('Ctrl Pts',(-0.301073868688523,1.98503934689477,
8.7569409597348));
#45853=CARTESIAN_POINT('Ctrl Pts',(-0.301252056825614,1.98550709880833,
8.75691015389584));
#45854=CARTESIAN_POINT('Ctrl Pts',(-0.301777453038312,1.98689600562222,
8.75681865302804));
#45855=CARTESIAN_POINT('Ctrl Pts',(-0.302121528636534,1.9878183321287,8.75675785340166));
#45856=CARTESIAN_POINT('Ctrl Pts',(-0.304456251546629,1.9941654248197,8.75633918238207));
#45857=CARTESIAN_POINT('Ctrl Pts',(-0.306304800668973,1.99964100182158,
8.75597660998167));
#45858=CARTESIAN_POINT('Ctrl Pts',(-0.308349985626768,2.00628321520694,
8.75553474225812));
#45859=CARTESIAN_POINT('Ctrl Pts',(-0.30868877939069,2.00740525495893,8.75546003129757));
#45860=CARTESIAN_POINT('Ctrl Pts',(-0.31783312121401,2.03829811691552,8.75340113488072));
#45861=CARTESIAN_POINT('Ctrl Pts',(-0.322295631438074,2.06918103693808,
8.75127116455808));
#45862=CARTESIAN_POINT('Ctrl Pts',(-0.322269154620022,2.10886972844207,
8.74861283212634));
#45863=CARTESIAN_POINT('Ctrl Pts',(-0.321914745083371,2.11752141763719,
8.74803976958711));
#45864=CARTESIAN_POINT('Ctrl Pts',(-0.320867752131873,2.13038262836019,
8.74720673582359));
#45865=CARTESIAN_POINT('Ctrl Pts',(-0.320439411291253,2.13460934092905,
8.74693603903327));
#45866=CARTESIAN_POINT('Ctrl Pts',(-0.319862068320647,2.139366594609,8.74663575632411));
#45867=CARTESIAN_POINT('Ctrl Pts',(-0.319795165777148,2.13990643403366,
8.74660174514411));
#45868=CARTESIAN_POINT('Ctrl Pts',(-0.319691993869274,2.14072200905505,
8.74655046142097));
#45869=CARTESIAN_POINT('Ctrl Pts',(-0.319656734309688,2.14099786796274,
8.74653313249642));
#45870=CARTESIAN_POINT('Ctrl Pts',(-0.319594863964523,2.14147698850269,
8.74650306537378));
#45871=CARTESIAN_POINT('Ctrl Pts',(-0.319568416312683,2.14168027043694,
8.74649031793341));
#45872=CARTESIAN_POINT('Ctrl Pts',(-0.319512674810286,2.14210553878426,
8.74646367016527));
#45873=CARTESIAN_POINT('Ctrl Pts',(-0.319483343586603,2.14232751979276,
8.74644977204835));
#45874=CARTESIAN_POINT('Ctrl Pts',(-0.319412595040628,2.14285868716626,
8.74641654297014));
#45875=CARTESIAN_POINT('Ctrl Pts',(-0.319370959955131,2.1431678453887,8.74639722439659));
#45876=CARTESIAN_POINT('Ctrl Pts',(-0.319228085787161,2.14421722565805,
8.74633172405359));
#45877=CARTESIAN_POINT('Ctrl Pts',(-0.31912472062933,2.14495716305199,8.74628566186668));
#45878=CARTESIAN_POINT('Ctrl Pts',(-0.318872539392964,2.14671769445226,
8.7461763456104));
#45879=CARTESIAN_POINT('Ctrl Pts',(-0.318721394305429,2.14773795378419,
8.74611321867082));
#45880=CARTESIAN_POINT('Ctrl Pts',(-0.316844044285325,2.16000394046458,
8.74535678435133));
#45881=CARTESIAN_POINT('Ctrl Pts',(-0.314528173850799,2.17115271986926,
8.74469449513376));
#45882=CARTESIAN_POINT('Ctrl Pts',(-0.305079892523304,2.20699078096389,
8.74258112977049));
#45883=CARTESIAN_POINT('Ctrl Pts',(-0.295587837310875,2.23095296272004,
8.74118538011886));
#45884=CARTESIAN_POINT('Ctrl Pts',(-0.282704134124632,2.25473007357149,
8.73962713097325));
#45885=CARTESIAN_POINT('Ctrl Pts',(-0.282049037358633,2.2559210171223,8.73954861721519));
#45886=CARTESIAN_POINT('Ctrl Pts',(-0.279796441977427,2.25995550741794,
8.73928099367464));
#45887=CARTESIAN_POINT('Ctrl Pts',(-0.278163351384818,2.26277887541246,
8.73909090676196));
#45888=CARTESIAN_POINT('Ctrl Pts',(-0.275592896415891,2.26707113606438,
8.73879723565893));
#45889=CARTESIAN_POINT('Ctrl Pts',(-0.274685980246266,2.26855806464664,
8.73869462281087));
#45890=CARTESIAN_POINT('Ctrl Pts',(-0.27347784228096,2.27050321375478,8.73855918582393));
#45891=CARTESIAN_POINT('Ctrl Pts',(-0.273187430528504,2.27096813713506,
8.73852672307088));
#45892=CARTESIAN_POINT('Ctrl Pts',(-0.269880772797685,2.2762318653979,8.73815814483891));
#45893=CARTESIAN_POINT('Ctrl Pts',(-0.266739773217482,2.28095079222971,
8.73781782674773));
#45894=CARTESIAN_POINT('Ctrl Pts',(-0.262912613326235,2.28638425619373,
8.73741320540388));
#45895=CARTESIAN_POINT('Ctrl Pts',(-0.262345467537189,2.287181700047,8.73735349110978));
#45896=CARTESIAN_POINT('Ctrl Pts',(-0.261483480713575,2.28838209634735,
8.73726309797873));
#45897=CARTESIAN_POINT('Ctrl Pts',(-0.261191317148046,2.28878697188191,
8.7372325224252));
#45898=CARTESIAN_POINT('Ctrl Pts',(-0.260667652856102,2.28950911490108,
8.7371778303382));
#45899=CARTESIAN_POINT('Ctrl Pts',(-0.260436510309424,2.28982664189144,
8.73715372770711));
#45900=CARTESIAN_POINT('Ctrl Pts',(-0.259947022103561,2.29049648867263,
8.73710276580063));
#45901=CARTESIAN_POINT('Ctrl Pts',(-0.259688539483514,2.29084870697764,
8.7370759012338));
#45902=CARTESIAN_POINT('Ctrl Pts',(-0.259001631223251,2.29178073515796,
8.73700463245885));
#45903=CARTESIAN_POINT('Ctrl Pts',(-0.258571976689877,2.2923596324888,8.73696018039082));
#45904=CARTESIAN_POINT('Ctrl Pts',(-0.256594168726203,2.29500584291444,
8.73675612556665));
#45905=CARTESIAN_POINT('Ctrl Pts',(-0.255023175874761,2.2970558939418,8.73659562883457));
#45906=CARTESIAN_POINT('Ctrl Pts',(-0.242977289283136,2.3123897181956,8.73537646883157));
#45907=CARTESIAN_POINT('Ctrl Pts',(-0.231497352663814,2.32484699126091,
8.73427669168106));
#45908=CARTESIAN_POINT('Ctrl Pts',(-0.199231117070066,2.35475825075898,
8.7313421767124));
#45909=CARTESIAN_POINT('Ctrl Pts',(-0.177126483035226,2.37059376250626,
8.72946823584323));
#45910=CARTESIAN_POINT('Ctrl Pts',(-0.153012936905855,2.38363413902653,
8.72769287112027));
#45911=CARTESIAN_POINT('Ctrl Pts',(-0.152723549730563,2.38379006508564,
8.72767160284876));
#45912=CARTESIAN_POINT('Ctrl Pts',(-0.151945065732852,2.38420798806613,
8.72761449163078));
#45913=CARTESIAN_POINT('Ctrl Pts',(-0.151455527776677,2.38446916633555,
8.72757868699199));
#45914=CARTESIAN_POINT('Ctrl Pts',(-0.147502410743754,2.38656513613873,
8.72729044857387));
#45915=CARTESIAN_POINT('Ctrl Pts',(-0.144006102439163,2.38833796891551,
8.72704102283465));
#45916=CARTESIAN_POINT('Ctrl Pts',(-0.139947019703821,2.39030390205763,
8.72675846312227));
#45917=CARTESIAN_POINT('Ctrl Pts',(-0.139415197144291,2.39055967836607,
8.72672157901884));
#45918=CARTESIAN_POINT('Ctrl Pts',(-0.138627084666661,2.39093605353073,
8.72666712592486));
#45919=CARTESIAN_POINT('Ctrl Pts',(-0.138371337315835,2.39105777580768,
8.72664948754754));
#45920=CARTESIAN_POINT('Ctrl Pts',(-0.137917258826756,2.39127315950779,
8.72661822783701));
#45921=CARTESIAN_POINT('Ctrl Pts',(-0.137718992559633,2.39136695560995,
8.72660459809659));
#45922=CARTESIAN_POINT('Ctrl Pts',(-0.13729969437438,2.39156479422013,8.72657581455237));
#45923=CARTESIAN_POINT('Ctrl Pts',(-0.137078640476376,2.39166878754852,
8.72656066384871));
#45924=CARTESIAN_POINT('Ctrl Pts',(-0.13648933756291,2.391945203236,8.72652033719244));
#45925=CARTESIAN_POINT('Ctrl Pts',(-0.136120878597832,2.39211718089653,
8.72649518889914));
#45926=CARTESIAN_POINT('Ctrl Pts',(-0.134400945495759,2.39291599627391,
8.72637810087898));
#45927=CARTESIAN_POINT('Ctrl Pts',(-0.133045432540324,2.39353416854733,
8.72628668977969));
#45928=CARTESIAN_POINT('Ctrl Pts',(-0.122160889991647,2.39840709905856,
8.72555922142188));
#45929=CARTESIAN_POINT('Ctrl Pts',(-0.112433534147441,2.4022065990743,8.72494903641194));
#45930=CARTESIAN_POINT('Ctrl Pts',(-0.0734711500019861,2.41528273782643,
8.72259592651542));
#45931=CARTESIAN_POINT('Ctrl Pts',(-0.0431617179237742,2.42084020970614,
8.72094533364573));
#45932=CARTESIAN_POINT('Ctrl Pts',(-0.0106362385681566,2.4221049648031,
8.71904032795771));
#45933=CARTESIAN_POINT('Ctrl Pts',(-0.00874967847752063,2.42216173088752,
8.71892943022806));
#45934=CARTESIAN_POINT('Ctrl Pts',(-0.000181261329068391,2.42234423428214,
8.71842373912622));
#45935=CARTESIAN_POINT('Ctrl Pts',(0.00650263556893807,2.4222786746552,
8.71802366270603));
#45936=CARTESIAN_POINT('Ctrl Pts',(0.0142196486096833,2.42196282598536,
8.71755362294204));
#45937=CARTESIAN_POINT('Ctrl Pts',(0.0152597557318807,2.42191520550943,
8.71749010087077));
#45938=CARTESIAN_POINT('Ctrl Pts',(0.0168041393489657,2.4218369955958,8.71739552335311));
#45939=CARTESIAN_POINT('Ctrl Pts',(0.0173086112853697,2.42181025901013,
8.71736458877296));
#45940=CARTESIAN_POINT('Ctrl Pts',(0.0182058676322534,2.42176058928044,
8.71730949485646));
#45941=CARTESIAN_POINT('Ctrl Pts',(0.0185986777074702,2.42173812272669,
8.71728535020527));
#45942=CARTESIAN_POINT('Ctrl Pts',(0.0194243549030181,2.4216893814323,8.71723454561747));
#45943=CARTESIAN_POINT('Ctrl Pts',(0.0198572118083085,2.42166295221235,
8.71720788087932));
#45944=CARTESIAN_POINT('Ctrl Pts',(0.0209951273250252,2.42159116813012,
8.71713770191949));
#45945=CARTESIAN_POINT('Ctrl Pts',(0.0217000895644193,2.42154436846395,
8.71709414242385));
#45946=CARTESIAN_POINT('Ctrl Pts',(0.0248402447371625,2.42132553218599,
8.71689974205555));
#45947=CARTESIAN_POINT('Ctrl Pts',(0.0272735388199031,2.4211281503482,8.71674810739714));
#45948=CARTESIAN_POINT('Ctrl Pts',(0.0449860174032254,2.41948860011334,
8.71563682087728));
#45949=CARTESIAN_POINT('Ctrl Pts',(0.0601448649880876,2.41698451070976,
8.71464356157887));
#45950=CARTESIAN_POINT('Ctrl Pts',(0.103896583758847,2.40650541148109,8.71165709658134));
#45951=CARTESIAN_POINT('Ctrl Pts',(0.131634332567747,2.39565581002674,8.70959697358945));
#45952=CARTESIAN_POINT('Ctrl Pts',(0.160975594939883,2.37922021272131,8.70742952650427));
#45953=CARTESIAN_POINT('Ctrl Pts',(0.164417532341585,2.37720740975228,8.7071757522863));
#45954=CARTESIAN_POINT('Ctrl Pts',(0.168327723642775,2.37482231495264,8.70688879029276));
#45955=CARTESIAN_POINT('Ctrl Pts',(0.168833177704902,2.37451208618576,8.70685172200223));
#45956=CARTESIAN_POINT('Ctrl Pts',(0.16957666681898,2.37405293015971,8.70679723888245));
#45957=CARTESIAN_POINT('Ctrl Pts',(0.169815364548814,2.37390508652296,8.70677975341445));
#45958=CARTESIAN_POINT('Ctrl Pts',(0.17024042506662,2.37364104503969,8.7067486280095));
#45959=CARTESIAN_POINT('Ctrl Pts',(0.170426862352229,2.37352496859919,8.70673498005822));
#45960=CARTESIAN_POINT('Ctrl Pts',(0.17081524182776,2.37328261106572,8.70670655776558));
#45961=CARTESIAN_POINT('Ctrl Pts',(0.171017162145569,2.3731562970245,8.70669178570865));
#45962=CARTESIAN_POINT('Ctrl Pts',(0.17154678230169,2.37282416838126,8.70665305200281));
#45963=CARTESIAN_POINT('Ctrl Pts',(0.171874253045955,2.37261798641067,8.70662911471545));
#45964=CARTESIAN_POINT('Ctrl Pts',(0.172591425503731,2.37216463477988,8.70657671626444));
#45965=CARTESIAN_POINT('Ctrl Pts',(0.172980970096583,2.37191721639661,8.70654827140853));
#45966=CARTESIAN_POINT('Ctrl Pts',(0.174126761392463,2.37118601096484,8.70646464862688));
#45967=CARTESIAN_POINT('Ctrl Pts',(0.174881527030134,2.37069989494528,8.7064096202658));
#45968=CARTESIAN_POINT('Ctrl Pts',(0.183079596058085,2.36537123030725,8.70581241854418));
#45969=CARTESIAN_POINT('Ctrl Pts',(0.190322500077258,2.36022568267457,8.70528929092011));
#45970=CARTESIAN_POINT('Ctrl Pts',(0.215843560059731,2.34045844725737,8.70342668209469));
#45971=CARTESIAN_POINT('Ctrl Pts',(0.232728193425783,2.32415716309023,8.70215165548536));
#45972=CARTESIAN_POINT('Ctrl Pts',(0.258664453089838,2.29299651068582,8.69985308230382));
#45973=CARTESIAN_POINT('Ctrl Pts',(0.268559478518763,2.27897103360197,8.69885825606967));
#45974=CARTESIAN_POINT('Ctrl Pts',(0.277941236473569,2.26313022017065,8.69773987756249));
#45975=CARTESIAN_POINT('Ctrl Pts',(0.278584124497709,2.26202988974519,8.69766223044251));
#45976=CARTESIAN_POINT('Ctrl Pts',(0.279473877294604,2.2604860900134,8.69755333047804));
#45977=CARTESIAN_POINT('Ctrl Pts',(0.279726252124453,2.2600457967134,8.69752227679395));
#45978=CARTESIAN_POINT('Ctrl Pts',(0.28016104707138,2.25928308309595,8.69746849030715));
#45979=CARTESIAN_POINT('Ctrl Pts',(0.280343953721204,2.25896094006638,8.69744577507593));
#45980=CARTESIAN_POINT('Ctrl Pts',(0.28072211390609,2.25829222541008,8.69739862642809));
#45981=CARTESIAN_POINT('Ctrl Pts',(0.280917281943962,2.25794560634657,8.69737418998722));
#45982=CARTESIAN_POINT('Ctrl Pts',(0.281373186066503,2.25713240109643,8.69731686468335));
#45983=CARTESIAN_POINT('Ctrl Pts',(0.281633403543088,2.25666552688703,8.69728395729759));
#45984=CARTESIAN_POINT('Ctrl Pts',(0.282471648749979,2.25515273551754,8.69717734041653));
#45985=CARTESIAN_POINT('Ctrl Pts',(0.283045015625288,2.254104259364,8.69710346463571));
#45986=CARTESIAN_POINT('Ctrl Pts',(0.284366976014723,2.25165461486203,8.69693089244573));
#45987=CARTESIAN_POINT('Ctrl Pts',(0.285111061972586,2.25025106140082,8.69683203782606));
#45988=CARTESIAN_POINT('Ctrl Pts',(0.292770420792738,2.23554159687508,8.69579616720342));
#45989=CARTESIAN_POINT('Ctrl Pts',(0.298758351674873,2.22177592697205,8.6948266314204));
#45990=CARTESIAN_POINT('Ctrl Pts',(0.313021045284607,2.18152777249815,8.69199533007313));
#45991=CARTESIAN_POINT('Ctrl Pts',(0.318868710546923,2.15432827586823,8.69007695579631));
#45992=CARTESIAN_POINT('Ctrl Pts',(0.321231682342236,2.125923285754,8.68821573052544));
#45993=CARTESIAN_POINT('Ctrl Pts',(0.321294792914689,2.12512899825819,8.6881638080771));
#45994=CARTESIAN_POINT('Ctrl Pts',(0.321421727756294,2.12345272885341,8.688054500639));
#45995=CARTESIAN_POINT('Ctrl Pts',(0.321484869196359,2.122570699484,8.68799714219029));
#45996=CARTESIAN_POINT('Ctrl Pts',(0.321553978010025,2.12154611776537,8.68793070472324));
#45997=CARTESIAN_POINT('Ctrl Pts',(0.321563481437544,2.12140381673283,8.68792148170687));
#45998=CARTESIAN_POINT('Ctrl Pts',(0.321605169862825,2.1207732938807,8.68788063446492));
#45999=CARTESIAN_POINT('Ctrl Pts',(0.321636337643961,2.12028500268697,8.68784905216766));
#46000=CARTESIAN_POINT('Ctrl Pts',(0.321911703935198,2.11581070379754,8.68756013384366));
#46001=CARTESIAN_POINT('Ctrl Pts',(0.32208291960246,2.11182032180296,8.68730592029225));
#46002=CARTESIAN_POINT('Ctrl Pts',(0.322194337704641,2.10723439299373,8.68701851381538));
#46003=CARTESIAN_POINT('Ctrl Pts',(0.322207111241453,2.10664117231213,8.68698142708442));
#46004=CARTESIAN_POINT('Ctrl Pts',(0.322223516614468,2.10576713369397,8.68692692205073));
#46005=CARTESIAN_POINT('Ctrl Pts',(0.322228419771395,2.10548634518676,8.68690943302799));
#46006=CARTESIAN_POINT('Ctrl Pts',(0.322236503432739,2.1049859518729,8.68687830358886));
#46007=CARTESIAN_POINT('Ctrl Pts',(0.322239826477187,2.10476635014712,8.68686465515051));
#46008=CARTESIAN_POINT('Ctrl Pts',(0.322245809724694,2.10434229735707,8.68683832507757));
#46009=CARTESIAN_POINT('Ctrl Pts',(0.322248499834516,2.10413784804252,8.68682564177988));
#46010=CARTESIAN_POINT('Ctrl Pts',(0.322255335360436,2.10357783444557,8.68679093108023));
#46011=CARTESIAN_POINT('Ctrl Pts',(0.322259086890187,2.10322226429441,8.68676892587348));
#46012=CARTESIAN_POINT('Ctrl Pts',(0.322271520043536,2.1018245754331,8.68668255689034));
#46013=CARTESIAN_POINT('Ctrl Pts',(0.32227573537832,2.10078240857744,8.68661844100109));
#46014=CARTESIAN_POINT('Ctrl Pts',(0.32227024399047,2.09396989111642,8.68620107267989));
#46015=CARTESIAN_POINT('Ctrl Pts',(0.322110616304971,2.08820029600263,8.68585579985326));
#46016=CARTESIAN_POINT('Ctrl Pts',(0.321465552348071,2.07638071823564,8.68515966243809));
#46017=CARTESIAN_POINT('Ctrl Pts',(0.320964025868544,2.07033396895897,8.68480955344859));
#46018=CARTESIAN_POINT('Ctrl Pts',(0.318434778769249,2.04763916976949,8.683506608538));
#46019=CARTESIAN_POINT('Ctrl Pts',(0.315279541988409,2.03114350080364,8.68258093942984));
#46020=CARTESIAN_POINT('Ctrl Pts',(0.305273343983131,1.99456353593097,8.68045018565243));
#46021=CARTESIAN_POINT('Ctrl Pts',(0.297697551010622,1.97476171169817,8.67923820492079));
#46022=CARTESIAN_POINT('Ctrl Pts',(0.287656152311748,1.95468378242558,8.67787475135588));
#46023=CARTESIAN_POINT('Ctrl Pts',(0.287067739606546,1.95352482171781,8.67779556578777));
#46024=CARTESIAN_POINT('Ctrl Pts',(0.286237882900444,1.9519145112768,8.67768485578309));
#46025=CARTESIAN_POINT('Ctrl Pts',(0.28600234469617,1.95146011848247,8.67765353938862));
#46026=CARTESIAN_POINT('Ctrl Pts',(0.28559394088151,1.95067681150095,8.67759942139728));
#46027=CARTESIAN_POINT('Ctrl Pts',(0.285421586513365,1.9503476306834,8.67757663789139));
#46028=CARTESIAN_POINT('Ctrl Pts',(0.285063862327353,1.94966727666626,8.67752946412748));
#46029=CARTESIAN_POINT('Ctrl Pts',(0.284878412045617,1.94931614665766,8.67750507104732));
#46030=CARTESIAN_POINT('Ctrl Pts',(0.284443797413027,1.94849692103725,8.67744804952074));
#46031=CARTESIAN_POINT('Ctrl Pts',(0.284194126303987,1.94802909689388,8.67741540312527));
#46032=CARTESIAN_POINT('Ctrl Pts',(0.283388882900536,1.94652918669054,8.67731046311394));
#46033=CARTESIAN_POINT('Ctrl Pts',(0.282828839056497,1.94549952353065,8.67723801044577));
#46034=CARTESIAN_POINT('Ctrl Pts',(0.274214563591115,1.92986563272967,8.67613154935595));
#46035=CARTESIAN_POINT('Ctrl Pts',(0.265045565021325,1.9159075817146,8.6750566207295));
#46036=CARTESIAN_POINT('Ctrl Pts',(0.241044556933921,1.884903420415,8.67245642616179));
#46037=CARTESIAN_POINT('Ctrl Pts',(0.225420090506573,1.86858113400703,8.67091035566852));
#46038=CARTESIAN_POINT('Ctrl Pts',(0.205275305210201,1.85152841751818,8.66915021836058));
#46039=CARTESIAN_POINT('Ctrl Pts',(0.202284175199631,1.84908728084921,8.66889434748372));
#46040=CARTESIAN_POINT('Ctrl Pts',(0.197713232714933,1.84549169900136,8.66851228137502));
#46041=CARTESIAN_POINT('Ctrl Pts',(0.196165651671012,1.84429697871749,8.66838442758327));
#46042=CARTESIAN_POINT('Ctrl Pts',(0.194344153216916,1.84291706650916,8.66823577467614));
#46043=CARTESIAN_POINT('Ctrl Pts',(0.194080736303882,1.84271814603576,8.66821432150253));
#46044=CARTESIAN_POINT('Ctrl Pts',(0.193421458917212,1.84222187840221,8.66816074033638));
#46045=CARTESIAN_POINT('Ctrl Pts',(0.19302521664863,1.84192503707702,8.66812863705441));
#46046=CARTESIAN_POINT('Ctrl Pts',(0.192444655962163,1.8414922003465,8.66808174875481));
#46047=CARTESIAN_POINT('Ctrl Pts',(0.192260875929563,1.84135548782649,8.66806692764648));
#46048=CARTESIAN_POINT('Ctrl Pts',(0.19183431155252,1.84103887580613,8.66803257747714));
#46049=CARTESIAN_POINT('Ctrl Pts',(0.191591419232093,1.84085912130544,8.66801305582987));
#46050=CARTESIAN_POINT('Ctrl Pts',(0.187953938292499,1.83817508261139,8.66772127581678));
#46051=CARTESIAN_POINT('Ctrl Pts',(0.184510547626401,1.83573719077625,8.66745248144098));
#46052=CARTESIAN_POINT('Ctrl Pts',(0.180570920494246,1.83306252972832,8.66715410717713));
#46053=CARTESIAN_POINT('Ctrl Pts',(0.18012098300644,1.832758719779,8.66712016299084));
#46054=CARTESIAN_POINT('Ctrl Pts',(0.17943963077834,1.83230115480346,8.66706896314954));
#46055=CARTESIAN_POINT('Ctrl Pts',(0.17920878420808,1.83214656157235,8.66705165137037));
#46056=CARTESIAN_POINT('Ctrl Pts',(0.178807318988723,1.83187845984461,8.66702160573603));
#46057=CARTESIAN_POINT('Ctrl Pts',(0.178636791943103,1.83176481553672,8.66700886267069));
#46058=CARTESIAN_POINT('Ctrl Pts',(0.178279662124944,1.83152730518608,8.66698221553311));
#46059=CARTESIAN_POINT('Ctrl Pts',(0.178093038708993,1.83140347107273,8.6669683136857));
#46060=CARTESIAN_POINT('Ctrl Pts',(0.177651150088129,1.83111091854968,8.66693545079649));
#46061=CARTESIAN_POINT('Ctrl Pts',(0.17739577254133,1.83094236837222,8.66691650116615));
#46062=CARTESIAN_POINT('Ctrl Pts',(0.176541859838724,1.83038052690974,8.66685327953433));
#46063=CARTESIAN_POINT('Ctrl Pts',(0.175942248318281,1.82998886351744,8.66680911635186));
#46064=CARTESIAN_POINT('Ctrl Pts',(0.174513053800377,1.82906210270635,8.6667043866079));
#46065=CARTESIAN_POINT('Ctrl Pts',(0.173682302489093,1.8285288081647,8.66664393629909));
#46066=CARTESIAN_POINT('Ctrl Pts',(0.170714462990907,1.82664282606932,8.66642944336876));
#46067=CARTESIAN_POINT('Ctrl Pts',(0.168563856244649,1.82531144971193,8.66627670423684));
#46068=CARTESIAN_POINT('Ctrl Pts',(0.162224400721188,1.82148937745178,8.66583360380263));
#46069=CARTESIAN_POINT('Ctrl Pts',(0.157994321674343,1.81906811797425,8.6655469234706));
#46070=CARTESIAN_POINT('Ctrl Pts',(0.14145318368664,1.81009197241098,8.66445380631727));
#46071=CARTESIAN_POINT('Ctrl Pts',(0.128775924541866,1.80424252860249,8.66367400179606));
#46072=CARTESIAN_POINT('Ctrl Pts',(0.0902808838479029,1.78942662905229,
8.66136823026948));
#46073=CARTESIAN_POINT('Ctrl Pts',(0.0636645717253811,1.78289903859826,
8.65984183268163));
#46074=CARTESIAN_POINT('Ctrl Pts',(0.0348389663162673,1.77960903193642,
8.65808454882584));
#46075=CARTESIAN_POINT('Ctrl Pts',(0.0331308795251033,1.77942790103473,
8.65798009055044));
#46076=CARTESIAN_POINT('Ctrl Pts',(0.0307848122892476,1.77919806709294,
8.65783613924487));
#46077=CARTESIAN_POINT('Ctrl Pts',(0.0301479922573071,1.77913759432096,
8.65779701671745));
#46078=CARTESIAN_POINT('Ctrl Pts',(0.029135633615279,1.77904450063876,8.6577347453277));
#46079=CARTESIAN_POINT('Ctrl Pts',(0.0287602082302013,1.77901064170757,
8.65771163543769));
#46080=CARTESIAN_POINT('Ctrl Pts',(0.0280310862812035,1.77894617294702,
8.65766671981459));
#46081=CARTESIAN_POINT('Ctrl Pts',(0.0276773966718144,1.77891548873328,
8.65764491645236));
#46082=CARTESIAN_POINT('Ctrl Pts',(0.0268334391513403,1.778843676346,8.65759285357545));
#46083=CARTESIAN_POINT('Ctrl Pts',(0.0263431274379504,1.77880308639069,
8.65756257719295));
#46084=CARTESIAN_POINT('Ctrl Pts',(0.0248801056886644,1.77868534411748,
8.65747214747316));
#46085=CARTESIAN_POINT('Ctrl Pts',(0.0239071427253281,1.77861148707964,
8.65741189077025));
#46086=CARTESIAN_POINT('Ctrl Pts',(0.0156465185784834,1.77802214697242,
8.65689928105501));
#46087=CARTESIAN_POINT('Ctrl Pts',(0.00834412754341373,1.77775023218287,
8.65643932518234));
#46088=CARTESIAN_POINT('Ctrl Pts',(-0.00846630807655281,1.777696022445,
8.65536355380563));
#46089=CARTESIAN_POINT('Ctrl Pts',(-0.0179677757964866,1.7780859369684,
8.65474297159538));
#46090=CARTESIAN_POINT('Ctrl Pts',(-0.0299776977436681,1.77911214844882,
8.6539439922575));
#46091=CARTESIAN_POINT('Ctrl Pts',(-0.0325152473042243,1.77935933831432,
8.65377436331968));
#46092=CARTESIAN_POINT('Ctrl Pts',(-0.0521011873566472,1.78150215037182,
8.65245919431146));
#46093=CARTESIAN_POINT('Ctrl Pts',(-0.0689763851792746,1.78472609890834,
8.65128943391358));
#46094=CARTESIAN_POINT('Ctrl Pts',(-0.0990715853535514,1.79300857801476,
8.64919149957954));
#46095=CARTESIAN_POINT('Ctrl Pts',(-0.112372585455829,1.79762371138241,
8.64826056144807));
#46096=CARTESIAN_POINT('Ctrl Pts',(-0.126071507899858,1.80340634436363,
8.64732650314877));
#46097=CARTESIAN_POINT('Ctrl Pts',(-0.126810842476563,1.80372169851464,
8.64727617196429));
#46098=CARTESIAN_POINT('Ctrl Pts',(-0.127822785695127,1.80415781240035,
8.64720740046214));
#46099=CARTESIAN_POINT('Ctrl Pts',(-0.128096410062603,1.8042761858804,8.64718881684159));
#46100=CARTESIAN_POINT('Ctrl Pts',(-0.128562763285297,1.80447870508954,
8.64715716445705));
#46101=CARTESIAN_POINT('Ctrl Pts',(-0.128755574069192,1.80456265978081,
8.64714408402609));
#46102=CARTESIAN_POINT('Ctrl Pts',(-0.129130186427699,1.80472621185523,
8.6471186819942));
#46103=CARTESIAN_POINT('Ctrl Pts',(-0.129311995272093,1.80480578784277,
8.6471063592551));
#46104=CARTESIAN_POINT('Ctrl Pts',(-0.129688458381443,1.80497097667044,
8.64708085438204));
#46105=CARTESIAN_POINT('Ctrl Pts',(-0.129883100944394,1.80505661401916,
8.64706767383437));
#46106=CARTESIAN_POINT('Ctrl Pts',(-0.13032741240479,1.80525262390133,8.64703760044733));
#46107=CARTESIAN_POINT('Ctrl Pts',(-0.130577026536933,1.80536312131158,
8.64702071526232));
#46108=CARTESIAN_POINT('Ctrl Pts',(-0.131821572161716,1.80591594012638,
8.64693657644676));
#46109=CARTESIAN_POINT('Ctrl Pts',(-0.132814413620418,1.80636299147854,
8.64686960961929));
#46110=CARTESIAN_POINT('Ctrl Pts',(-0.135332678692076,1.80751228803068,
8.64670010185249));
#46111=CARTESIAN_POINT('Ctrl Pts',(-0.136854934403849,1.80822144908281,
8.64659796347277));
#46112=CARTESIAN_POINT('Ctrl Pts',(-0.143110068558229,1.81119520164811,
8.6461793356589));
#46113=CARTESIAN_POINT('Ctrl Pts',(-0.147793097589866,1.81356342714628,
8.64586846301345));
#46114=CARTESIAN_POINT('Ctrl Pts',(-0.161902103771534,1.82113661928987,
8.64493343972686));
#46115=CARTESIAN_POINT('Ctrl Pts',(-0.171127303605349,1.8267006159989,8.64432413352563));
#46116=CARTESIAN_POINT('Ctrl Pts',(-0.200924333795429,1.84677355785067,
8.64230755728273));
#46117=CARTESIAN_POINT('Ctrl Pts',(-0.220071752590232,1.86322467442633,
8.64092216570651));
#46118=CARTESIAN_POINT('Ctrl Pts',(-0.23748135315962,1.88213747007581,8.63940934495352));
#46119=CARTESIAN_POINT('Ctrl Pts',(-0.237850918519618,1.88254100249033,
8.63937710379));
#46120=CARTESIAN_POINT('Ctrl Pts',(-0.239477879577936,1.88432660805946,
8.63923459779455));
#46121=CARTESIAN_POINT('Ctrl Pts',(-0.240724252346865,1.88571864074143,
8.63912392117508));
#46122=CARTESIAN_POINT('Ctrl Pts',(-0.245262576263303,1.89087691312943,
8.63871519712279));
#46123=CARTESIAN_POINT('Ctrl Pts',(-0.248478687910199,1.89470866016084,
8.6384142681002));
#46124=CARTESIAN_POINT('Ctrl Pts',(-0.252139840125557,1.89928275757837,
8.63805746401904));
#46125=CARTESIAN_POINT('Ctrl Pts',(-0.252672807723355,1.89995409877028,
8.63800515596503));
#46126=CARTESIAN_POINT('Ctrl Pts',(-0.253521439701633,1.90103186171989,
8.63792127361707));
#46127=CARTESIAN_POINT('Ctrl Pts',(-0.253838822447975,1.90143693029062,
8.63788976784797));
#46128=CARTESIAN_POINT('Ctrl Pts',(-0.254398735119936,1.90215507075262,
8.63783394752902));
#46129=CARTESIAN_POINT('Ctrl Pts',(-0.254641661288021,1.90246783352127,
8.6378096487685));
#46130=CARTESIAN_POINT('Ctrl Pts',(-0.25514417470238,1.9031172773439,8.63775921738535));
#46131=CARTESIAN_POINT('Ctrl Pts',(-0.255403673335457,1.90345402571145,
8.63773308132431));
#46132=CARTESIAN_POINT('Ctrl Pts',(-0.256069373670772,1.90432144189538,
8.63766579264622));
#46133=CARTESIAN_POINT('Ctrl Pts',(-0.25647459094744,1.90485285956069,8.63762460134289));
#46134=CARTESIAN_POINT('Ctrl Pts',(-0.258145998964497,1.90705900692752,
8.63745372984919));
#46135=CARTESIAN_POINT('Ctrl Pts',(-0.259397439642892,1.90874479991227,
8.6373234735796));
#46136=CARTESIAN_POINT('Ctrl Pts',(-0.267679179050108,1.92013179688353,
8.63644556146597));
#46137=CARTESIAN_POINT('Ctrl Pts',(-0.274179448455385,1.93020517253619,
8.63567768680478));
#46138=CARTESIAN_POINT('Ctrl Pts',(-0.285679611855011,1.950415696332,8.63415273527023));
#46139=CARTESIAN_POINT('Ctrl Pts',(-0.290737323169246,1.96050060939791,
8.63339877897254));
#46140=CARTESIAN_POINT('Ctrl Pts',(-0.297226608311066,1.97533367052695,
8.63230672759021));
#46141=CARTESIAN_POINT('Ctrl Pts',(-0.299093942896654,1.97988271169898,
8.63197406213613));
#46142=CARTESIAN_POINT('Ctrl Pts',(-0.30177013758237,1.98685206103709,8.63146884727493));
#46143=CARTESIAN_POINT('Ctrl Pts',(-0.30265556106367,1.98924223080309,8.63129636395728));
#46144=CARTESIAN_POINT('Ctrl Pts',(-0.304501734207848,1.99441342345963,
8.63092511771356));
#46145=CARTESIAN_POINT('Ctrl Pts',(-0.305452948814603,1.99719762836776,
8.63072642184364));
#46146=CARTESIAN_POINT('Ctrl Pts',(-0.3110870139823,2.01445753220449,8.62950314922358));
#46147=CARTESIAN_POINT('Ctrl Pts',(-0.314778686774291,2.02923880535573,
8.62849131203339));
#46148=CARTESIAN_POINT('Ctrl Pts',(-0.317569922439361,2.0451242382985,8.6274769783564));
#46149=CARTESIAN_POINT('Ctrl Pts',(-0.317723714409241,2.04602179875248,
8.6274199126478));
#46150=CARTESIAN_POINT('Ctrl Pts',(-0.317925433403785,2.0472298088842,8.62734345101829));
#46151=CARTESIAN_POINT('Ctrl Pts',(-0.317976712078569,2.04753968306305,
8.6273238676053));
#46152=CARTESIAN_POINT('Ctrl Pts',(-0.318062283034643,2.04806151871233,
8.62729094012427));
#46153=CARTESIAN_POINT('Ctrl Pts',(-0.318096816503776,2.0482734395261,8.62727758234351));
#46154=CARTESIAN_POINT('Ctrl Pts',(-0.318162642397224,2.04867995077836,
8.62725198674318));
#46155=CARTESIAN_POINT('Ctrl Pts',(-0.318193967879006,2.0488745339878,8.62723974714242));
#46156=CARTESIAN_POINT('Ctrl Pts',(-0.31825827209253,2.04927631826446,8.627214499222));
#46157=CARTESIAN_POINT('Ctrl Pts',(-0.318291226876738,2.04948352211374,
8.62720149232054));
#46158=CARTESIAN_POINT('Ctrl Pts',(-0.318365151784295,2.04995127058588,
8.62717216071327));
#46159=CARTESIAN_POINT('Ctrl Pts',(-0.318406004522026,2.05021183401547,
8.62715584268829));
#46160=CARTESIAN_POINT('Ctrl Pts',(-0.318508334209309,2.05086978163353,
8.62711469147931));
#46161=CARTESIAN_POINT('Ctrl Pts',(-0.318569387594239,2.05126723269236,
8.62708988210395));
#46162=CARTESIAN_POINT('Ctrl Pts',(-0.318740993133279,2.05239847080447,
8.62701940593629));
#46163=CARTESIAN_POINT('Ctrl Pts',(-0.318849755864242,2.05313253265157,
8.62697383788043));
#46164=CARTESIAN_POINT('Ctrl Pts',(-0.321152835815807,2.0690556394045,8.62598881250798));
#46165=CARTESIAN_POINT('Ctrl Pts',(-0.3222622218736,2.08438373205464,8.62510777473546));
#46166=CARTESIAN_POINT('Ctrl Pts',(-0.322274890249976,2.09973403126875,
8.62424191572231));
#46167=CARTESIAN_POINT('',(-0.322193764531691,2.10029569746695,8.37437729859741));
#46168=CARTESIAN_POINT('Ctrl Pts',(-0.322274889955221,2.09973367435276,
8.62424193585475));
#46169=CARTESIAN_POINT('Ctrl Pts',(-0.322289278827864,2.11714533708805,
8.6232598019252));
#46170=CARTESIAN_POINT('Ctrl Pts',(-0.320892615123807,2.13453003690225,
8.6222992791076));
#46171=CARTESIAN_POINT('Ctrl Pts',(-0.31561710362526,2.16697805015618,8.62043450130561));
#46172=CARTESIAN_POINT('Ctrl Pts',(-0.312041398813254,2.18203832932221,
8.61953862448343));
#46173=CARTESIAN_POINT('Ctrl Pts',(-0.306662861375602,2.19912152843302,
8.61845830205772));
#46174=CARTESIAN_POINT('Ctrl Pts',(-0.305899846109963,2.20145181902264,
8.61830954980833));
#46175=CARTESIAN_POINT('Ctrl Pts',(-0.304882469788176,2.20444307536386,
8.61811673638976));
#46176=CARTESIAN_POINT('Ctrl Pts',(-0.304652404798807,2.20511226671195,
8.61807347977649));
#46177=CARTESIAN_POINT('Ctrl Pts',(-0.304277714658802,2.20619056582074,
8.6180035806767));
#46178=CARTESIAN_POINT('Ctrl Pts',(-0.304134463120211,2.20660015125213,
8.61797698378991));
#46179=CARTESIAN_POINT('Ctrl Pts',(-0.303859761421119,2.20738051859004,
8.61792622123663));
#46180=CARTESIAN_POINT('Ctrl Pts',(-0.303728458593311,2.20775135183335,
8.61790206050354));
#46181=CARTESIAN_POINT('Ctrl Pts',(-0.303427151032547,2.20859739577276,
8.61784685089513));
#46182=CARTESIAN_POINT('Ctrl Pts',(-0.303256708617738,2.20907244851964,
8.61781578749871));
#46183=CARTESIAN_POINT('Ctrl Pts',(-0.302732045036946,2.21052404099147,
8.61772067398586));
#46184=CARTESIAN_POINT('Ctrl Pts',(-0.302374220226622,2.21149926291777,
8.61765650386377));
#46185=CARTESIAN_POINT('Ctrl Pts',(-0.299697700737171,2.21868625111849,
8.61718157587235));
#46186=CARTESIAN_POINT('Ctrl Pts',(-0.297192662213035,2.22482647568947,
8.6167646005063));
#46187=CARTESIAN_POINT('Ctrl Pts',(-0.293612896988812,2.23288120842361,
8.61620193246884));
#46188=CARTESIAN_POINT('Ctrl Pts',(-0.292705341781809,2.23486857069105,
8.616061810938));
#46189=CARTESIAN_POINT('Ctrl Pts',(-0.281238644675409,2.2593173199937,8.61432194954758));
#46190=CARTESIAN_POINT('Ctrl Pts',(-0.26814029408882,2.2804926763812,8.61263682911569));
#46191=CARTESIAN_POINT('Ctrl Pts',(-0.248644309706695,2.30513625640713,
8.61051519751126));
#46192=CARTESIAN_POINT('Ctrl Pts',(-0.244384115203252,2.31019344991678,
8.61007064713891));
#46193=CARTESIAN_POINT('Ctrl Pts',(-0.233710476624205,2.32210034851475,
8.60900716801304));
#46194=CARTESIAN_POINT('Ctrl Pts',(-0.227147092450352,2.32880862399694,
8.60839360132089));
#46195=CARTESIAN_POINT('Ctrl Pts',(-0.21920078488741,2.33625083826131,8.60770513205838));
#46196=CARTESIAN_POINT('Ctrl Pts',(-0.218094601827136,2.3372723910163,8.60761045168332));
#46197=CARTESIAN_POINT('Ctrl Pts',(-0.21675887857997,2.33848868873116,8.60749755112829));
#46198=CARTESIAN_POINT('Ctrl Pts',(-0.216536198182731,2.33869089001106,
8.6074787764554));
#46199=CARTESIAN_POINT('Ctrl Pts',(-0.216148309989463,2.33904211598542,
8.60744615518428));
#46200=CARTESIAN_POINT('Ctrl Pts',(-0.215983230825327,2.33919128146539,
8.60743229797286));
#46201=CARTESIAN_POINT('Ctrl Pts',(-0.215651728743901,2.33949020363677,
8.60740452289326));
#46202=CARTESIAN_POINT('Ctrl Pts',(-0.215485303719271,2.33963995833407,
8.60739060517711));
#46203=CARTESIAN_POINT('Ctrl Pts',(-0.215166171961874,2.33992652230166,
8.60736396751872));
#46204=CARTESIAN_POINT('Ctrl Pts',(-0.21501349095821,2.34006335906808,8.60735124545063));
#46205=CARTESIAN_POINT('Ctrl Pts',(-0.214653311145667,2.34038554251016,
8.60732128537012));
#46206=CARTESIAN_POINT('Ctrl Pts',(-0.214445702298301,2.34057076672123,
8.60730405665412));
#46207=CARTESIAN_POINT('Ctrl Pts',(-0.213831128454681,2.34111764876116,
8.60725317369623));
#46208=CARTESIAN_POINT('Ctrl Pts',(-0.213423483985489,2.34147854673657,
8.60721957628624));
#46209=CARTESIAN_POINT('Ctrl Pts',(-0.209817517270556,2.34465473663088,
8.60692370565947));
#46210=CARTESIAN_POINT('Ctrl Pts',(-0.206564383351062,2.34740753931755,
8.60666597534273));
#46211=CARTESIAN_POINT('Ctrl Pts',(-0.195999380091241,2.35599393193254,
8.60585427656205));
#46212=CARTESIAN_POINT('Ctrl Pts',(-0.188487371326696,2.36157444414607,
8.60531462880073));
#46213=CARTESIAN_POINT('Ctrl Pts',(-0.172922498489049,2.37211799237987,
8.60424649194393));
#46214=CARTESIAN_POINT('Ctrl Pts',(-0.164873006885681,2.37706911390877,
8.60371865757591));
#46215=CARTESIAN_POINT('Ctrl Pts',(-0.148982057119743,2.38590531246562,
8.60270235863695));
#46216=CARTESIAN_POINT('Ctrl Pts',(-0.141177267910753,2.38983870620425,
8.60221434752027));
#46217=CARTESIAN_POINT('Ctrl Pts',(-0.117788144997574,2.40045705917763,
8.60076344184052));
#46218=CARTESIAN_POINT('Ctrl Pts',(-0.101827174683326,2.40623455535009,
8.5997862915574));
#46219=CARTESIAN_POINT('Ctrl Pts',(-0.0829942364726874,2.41141582815646,
8.59860897203718));
#46220=CARTESIAN_POINT('Ctrl Pts',(-0.0804930886085562,2.41207166388473,
8.59845218173404));
#46221=CARTESIAN_POINT('Ctrl Pts',(-0.0772845960211634,2.41287183796288,
8.59825040889319));
#46222=CARTESIAN_POINT('Ctrl Pts',(-0.0765842379138335,2.41304400691,8.59820632659876));
#46223=CARTESIAN_POINT('Ctrl Pts',(-0.0754586436800834,2.41331670821684,
8.59813541455056));
#46224=CARTESIAN_POINT('Ctrl Pts',(-0.0750337679833222,2.41341872983777,
8.59810863283789));
#46225=CARTESIAN_POINT('Ctrl Pts',(-0.0742266218374024,2.41361080733379,
8.59805772660293));
#46226=CARTESIAN_POINT('Ctrl Pts',(-0.0738443913814698,2.41370102920659,
8.59803360747543));
#46227=CARTESIAN_POINT('Ctrl Pts',(-0.0729759689617699,2.41390433694146,
8.59797878129875));
#46228=CARTESIAN_POINT('Ctrl Pts',(-0.0724896781119359,2.41401699215062,
8.59794806046244));
#46229=CARTESIAN_POINT('Ctrl Pts',(-0.071049822467201,2.41434702940355,
8.59785703965663));
#46230=CARTESIAN_POINT('Ctrl Pts',(-0.0700955340421101,2.41456119951615,
8.59779663671507));
#46231=CARTESIAN_POINT('Ctrl Pts',(-0.0636138809691888,2.41598491189389,
8.59738582991462));
#46232=CARTESIAN_POINT('Ctrl Pts',(-0.0580567645082365,2.41705298600654,
8.59703092261629));
#46233=CARTESIAN_POINT('Ctrl Pts',(-0.0520926999182333,2.41803722443612,
8.59664682972004));
#46234=CARTESIAN_POINT('Ctrl Pts',(-0.0517106023972528,2.41809957420507,
8.59662220836619));
#46235=CARTESIAN_POINT('Ctrl Pts',(-0.0284735726931505,2.42184836350535,
8.59512403328706));
#46236=CARTESIAN_POINT('Ctrl Pts',(-0.00529170856375248,2.42306154822161,
8.59357241161624));
#46237=CARTESIAN_POINT('Ctrl Pts',(0.0282928311121755,2.42120211310135,
8.59129625747692));
#46238=CARTESIAN_POINT('Ctrl Pts',(0.0387356602430444,2.42011067380137,
8.59058574465203));
#46239=CARTESIAN_POINT('Ctrl Pts',(0.0560058430313619,2.41744802418545,
8.5894211508617));
#46240=CARTESIAN_POINT('Ctrl Pts',(0.0628689017969807,2.41616042902419,
8.5889612146127));
#46241=CARTESIAN_POINT('Ctrl Pts',(0.0738716749152643,2.41372366492334,
8.58823386467368));
#46242=CARTESIAN_POINT('Ctrl Pts',(0.078039538443443,2.4127129629377,8.5879607098021));
#46243=CARTESIAN_POINT('Ctrl Pts',(0.0827173182496458,2.41147924900187,
8.58765776530736));
#46244=CARTESIAN_POINT('Ctrl Pts',(0.083248050630079,2.41133782194597,8.58762344687613));
#46245=CARTESIAN_POINT('Ctrl Pts',(0.0839928229668553,2.41113731793815,
8.58757536526593));
#46246=CARTESIAN_POINT('Ctrl Pts',(0.0842071635040732,2.41107937658899,
8.58756153668274));
#46247=CARTESIAN_POINT('Ctrl Pts',(0.0846372534775072,2.41096263594445,
8.58753380689905));
#46248=CARTESIAN_POINT('Ctrl Pts',(0.084853002280755,2.41090383341932,8.58751990587278));
#46249=CARTESIAN_POINT('Ctrl Pts',(0.0852667450966799,2.41079060469843,
8.58749326574277));
#46250=CARTESIAN_POINT('Ctrl Pts',(0.0854647479678533,2.41073621392361,
8.58748052457947));
#46251=CARTESIAN_POINT('Ctrl Pts',(0.0859320898536088,2.41060735607322,
8.58745047018639));
#46252=CARTESIAN_POINT('Ctrl Pts',(0.0862013847843693,2.4105327277052,8.58743316639711));
#46253=CARTESIAN_POINT('Ctrl Pts',(0.0871356303680149,2.4102725159339,8.58737318436096));
#46254=CARTESIAN_POINT('Ctrl Pts',(0.0878000875582233,2.4100851445476,8.58733060951985));
#46255=CARTESIAN_POINT('Ctrl Pts',(0.0958354708488177,2.40779133457556,
8.58681672730123));
#46256=CARTESIAN_POINT('Ctrl Pts',(0.103130278963668,2.40542447665799,8.58636020686218));
#46257=CARTESIAN_POINT('Ctrl Pts',(0.114138293844963,2.40141336489655,8.58567692419823));
#46258=CARTESIAN_POINT('Ctrl Pts',(0.117915886118112,2.39995568438996,8.58544348338621));
#46259=CARTESIAN_POINT('Ctrl Pts',(0.141657516319181,2.39027651047187,8.58397716809752));
#46260=CARTESIAN_POINT('Ctrl Pts',(0.160780747619045,2.38013734566603,8.58279615851553));
#46261=CARTESIAN_POINT('Ctrl Pts',(0.1916143101985,2.35958478486062,8.58069420346629));
#46262=CARTESIAN_POINT('Ctrl Pts',(0.203845959245418,2.35009405432754,8.57979816856137));
#46263=CARTESIAN_POINT('Ctrl Pts',(0.217172729885274,2.33812432606454,8.57871765776444));
#46264=CARTESIAN_POINT('Ctrl Pts',(0.218978344923815,2.33646495133719,8.57856888927991));
#46265=CARTESIAN_POINT('Ctrl Pts',(0.221280360877282,2.33430040184641,8.57837605772921));
#46266=CARTESIAN_POINT('Ctrl Pts',(0.22179431096724,2.33381394317995,8.57833279940673));
#46267=CARTESIAN_POINT('Ctrl Pts',(0.2226208087827,2.33302647791551,8.57826289821028));
#46268=CARTESIAN_POINT('Ctrl Pts',(0.222934360047665,2.3327265241007,8.57823630094102));
#46269=CARTESIAN_POINT('Ctrl Pts',(0.223531019265905,2.3321534273026,8.57818553809768));
#46270=CARTESIAN_POINT('Ctrl Pts',(0.223814234960702,2.33188039720764,8.57816137745796));
#46271=CARTESIAN_POINT('Ctrl Pts',(0.224459653028552,2.33125590695729,8.5781061686781));
#46272=CARTESIAN_POINT('Ctrl Pts',(0.224821530477681,2.3309041137992,8.57807510601844));
#46273=CARTESIAN_POINT('Ctrl Pts',(0.225925679592945,2.32982567721043,8.57797999694929));
#46274=CARTESIAN_POINT('Ctrl Pts',(0.226665260308591,2.32909629925763,8.57791583055055));
#46275=CARTESIAN_POINT('Ctrl Pts',(0.232098665018089,2.32368578489707,8.57744098757749));
#46276=CARTESIAN_POINT('Ctrl Pts',(0.236650285195752,2.31886469031296,8.57702409600658));
#46277=CARTESIAN_POINT('Ctrl Pts',(0.242274814081534,2.31252646095577,8.57648316075803));
#46278=CARTESIAN_POINT('Ctrl Pts',(0.243487961862438,2.31113548814349,8.57636487356227));
#46279=CARTESIAN_POINT('Ctrl Pts',(0.245909477499344,2.30831039599949,8.57612547851468));
#46280=CARTESIAN_POINT('Ctrl Pts',(0.247117409246144,2.30687599674828,8.57600436045813));
#46281=CARTESIAN_POINT('Ctrl Pts',(0.258471698604419,2.29315161992836,8.57484959189341));
#46282=CARTESIAN_POINT('Ctrl Pts',(0.267704716243784,2.28013675302101,8.57378376599523));
#46283=CARTESIAN_POINT('Ctrl Pts',(0.284956180894196,2.25154526519327,8.57152746918955));
#46284=CARTESIAN_POINT('Ctrl Pts',(0.292746590281897,2.23588775999119,8.57033840233793));
#46285=CARTESIAN_POINT('Ctrl Pts',(0.301030828332621,2.21517429963108,8.5688761598379));
#46286=CARTESIAN_POINT('Ctrl Pts',(0.302729430566614,2.21063261869833,8.56856213475));
#46287=CARTESIAN_POINT('Ctrl Pts',(0.30484659452487,2.20455736067678,8.56815229933356));
#46288=CARTESIAN_POINT('Ctrl Pts',(0.305357150458607,2.20305677446312,8.56805188773756));
#46289=CARTESIAN_POINT('Ctrl Pts',(0.306184769451272,2.2005641437318,8.56788651581217));
#46290=CARTESIAN_POINT('Ctrl Pts',(0.306508125747099,2.19957423848631,8.56782121077517));
#46291=CARTESIAN_POINT('Ctrl Pts',(0.306935402575118,2.19824439214856,8.56773399090108));
#46292=CARTESIAN_POINT('Ctrl Pts',(0.307043562588505,2.19790583546679,8.56771183051866));
#46293=CARTESIAN_POINT('Ctrl Pts',(0.307213062093039,2.19737223376422,8.56767697396423));
#46294=CARTESIAN_POINT('Ctrl Pts',(0.30727477600167,2.19717730940141,8.56766425570861));
#46295=CARTESIAN_POINT('Ctrl Pts',(0.307402401735869,2.1967728643523,8.56763789775847));
#46296=CARTESIAN_POINT('Ctrl Pts',(0.307468284350025,2.19656333666064,8.56762425994196));
#46297=CARTESIAN_POINT('Ctrl Pts',(0.307617949578613,2.19608564747666,8.56759320697851));
#46298=CARTESIAN_POINT('Ctrl Pts',(0.307701595659562,2.19581744404834,8.56757579997582));
#46299=CARTESIAN_POINT('Ctrl Pts',(0.307960983465421,2.19498189853027,8.5675216573617));
#46300=CARTESIAN_POINT('Ctrl Pts',(0.30813550888236,2.19441417565431,8.56748499302369));
#46301=CARTESIAN_POINT('Ctrl Pts',(0.30947530661344,2.19001259090472,8.5672016658689));
#46302=CARTESIAN_POINT('Ctrl Pts',(0.310570617794281,2.18615757000808,8.56695899955717));
#46303=CARTESIAN_POINT('Ctrl Pts',(0.311715709647907,2.18182126838335,8.56669110162066));
#46304=CARTESIAN_POINT('Ctrl Pts',(0.311836591027326,2.18135935166222,8.56666262819123));
#46305=CARTESIAN_POINT('Ctrl Pts',(0.311991942503021,2.18076028377085,8.56662578128387));
#46306=CARTESIAN_POINT('Ctrl Pts',(0.312027348865919,2.18062337862807,8.56661736611381));
#46307=CARTESIAN_POINT('Ctrl Pts',(0.312281121192132,2.179639450669,8.56655692582009));
#46308=CARTESIAN_POINT('Ctrl Pts',(0.312496130127134,2.1787915569222,8.56650504920344));
#46309=CARTESIAN_POINT('Ctrl Pts',(0.313170645801836,2.17608538953229,8.56634010826773));
#46310=CARTESIAN_POINT('Ctrl Pts',(0.313617056639271,2.1742238638879,8.56622759390601));
#46311=CARTESIAN_POINT('Ctrl Pts',(0.319926115006788,2.14684156900942,8.5645849480828));
#46312=CARTESIAN_POINT('Ctrl Pts',(0.32267409085372,2.12070134580295,8.56316716286454));
#46313=CARTESIAN_POINT('Ctrl Pts',(0.321966911334884,2.07915879202717,8.56080957855629));
#46314=CARTESIAN_POINT('Ctrl Pts',(0.320608231087173,2.06384314292637,8.55991934275485));
#46315=CARTESIAN_POINT('Ctrl Pts',(0.317774322136969,2.0462727174578,8.55884574134688));
#46316=CARTESIAN_POINT('Ctrl Pts',(0.317358036363327,2.04386608023926,8.55869756984175));
#46317=CARTESIAN_POINT('Ctrl Pts',(0.316786098720414,2.04076958037542,8.55850540512337));
#46318=CARTESIAN_POINT('Ctrl Pts',(0.316655467593175,2.04007513218849,8.55846220976323));
#46319=CARTESIAN_POINT('Ctrl Pts',(0.316440978780081,2.03895517499018,8.55839238580152));
#46320=CARTESIAN_POINT('Ctrl Pts',(0.316358543751782,2.03852939316946,8.55836580262057));
#46321=CARTESIAN_POINT('Ctrl Pts',(0.316199684300522,2.03771765841098,8.55831505044109));
#46322=CARTESIAN_POINT('Ctrl Pts',(0.316123412003408,2.03733167620957,8.55829088634132));
#46323=CARTESIAN_POINT('Ctrl Pts',(0.315947602396905,2.03645046558745,8.55823564694098));
#46324=CARTESIAN_POINT('Ctrl Pts',(0.315847607377566,2.03595533048224,8.5582045570625));
#46325=CARTESIAN_POINT('Ctrl Pts',(0.315537984811538,2.03444056623767,8.55810928374757));
#46326=CARTESIAN_POINT('Ctrl Pts',(0.315324582400139,2.03342172345565,8.55804497971556));
#46327=CARTESIAN_POINT('Ctrl Pts',(0.313705632610896,2.0258748159736,8.55756698449485));
#46328=CARTESIAN_POINT('Ctrl Pts',(0.312102518901936,2.0193912301101,8.55714698526234));
#46329=CARTESIAN_POINT('Ctrl Pts',(0.309739747417511,2.01096766388689,8.55658838978149));
#46330=CARTESIAN_POINT('Ctrl Pts',(0.309160997580292,2.00897832527316,8.55645551656806));
#46331=CARTESIAN_POINT('Ctrl Pts',(0.30126930825418,1.98279610430242,8.55469410554572));
#46332=CARTESIAN_POINT('Ctrl Pts',(0.291155009018485,1.95954242309954,8.55297656199692));
#46333=CARTESIAN_POINT('Ctrl Pts',(0.270221128211279,1.9236266338944,8.55017108654684));
#46334=CARTESIAN_POINT('Ctrl Pts',(0.260952209590638,1.91018137617041,8.54908265695147));
#46335=CARTESIAN_POINT('Ctrl Pts',(0.250304739574772,1.89699971205137,8.54801683388345));
#46336=CARTESIAN_POINT('Ctrl Pts',(0.249903911506828,1.89650647531082,8.54797695605127));
#46337=CARTESIAN_POINT('Ctrl Pts',(0.249183373178297,1.8956251606377,8.54790571378721));
#46338=CARTESIAN_POINT('Ctrl Pts',(0.248864210273479,1.8952366407631,8.5478743112462));
#46339=CARTESIAN_POINT('Ctrl Pts',(0.248376167890504,1.89464536899852,8.5478265292745));
#46340=CARTESIAN_POINT('Ctrl Pts',(0.248207948338979,1.89444207718436,8.5478101023019));
#46341=CARTESIAN_POINT('Ctrl Pts',(0.247913651623383,1.8940873102421,8.54778143834851));
#46342=CARTESIAN_POINT('Ctrl Pts',(0.247787685412635,1.89393574443108,8.54776919330902));
#46343=CARTESIAN_POINT('Ctrl Pts',(0.247524157156473,1.89361925144892,8.547743625827));
#46344=CARTESIAN_POINT('Ctrl Pts',(0.247386569703223,1.89345434674233,8.54773030535057));
#46345=CARTESIAN_POINT('Ctrl Pts',(0.247004371138156,1.89299719444839,8.54769338081598));
#46346=CARTESIAN_POINT('Ctrl Pts',(0.246759405297072,1.89270524182077,8.5476698027293));
#46347=CARTESIAN_POINT('Ctrl Pts',(0.245787644795391,1.89155125180641,8.54757661584557));
#46348=CARTESIAN_POINT('Ctrl Pts',(0.245056835066731,1.89069258342567,8.54750729738346));
#46349=CARTESIAN_POINT('Ctrl Pts',(0.231204144164507,1.87458830890502,8.54620723538208));
#46350=CARTESIAN_POINT('Ctrl Pts',(0.216685557709048,1.86059778108319,8.54507641194588));
#46351=CARTESIAN_POINT('Ctrl Pts',(0.188405562137587,1.83804162282798,8.54305240499374));
#46352=CARTESIAN_POINT('Ctrl Pts',(0.175126238737614,1.82898409710304,8.54216020050904));
#46353=CARTESIAN_POINT('Ctrl Pts',(0.156233829829782,1.81806838676072,8.54090913700315));
#46354=CARTESIAN_POINT('Ctrl Pts',(0.151163268239895,1.81531753564531,8.54057517817261));
#46355=CARTESIAN_POINT('Ctrl Pts',(0.139457460407964,1.80936790501967,8.53980517864555));
#46356=CARTESIAN_POINT('Ctrl Pts',(0.132781129652931,1.80625766952256,8.53936666972128));
#46357=CARTESIAN_POINT('Ctrl Pts',(0.124568472999773,1.80276893583573,8.53882555851535));
#46358=CARTESIAN_POINT('Ctrl Pts',(0.123128042608866,1.80216935187994,8.53873059357326));
#46359=CARTESIAN_POINT('Ctrl Pts',(0.121131914920536,1.80135541285289,8.53859889219197));
#46360=CARTESIAN_POINT('Ctrl Pts',(0.120579876001654,1.80113209650332,8.53856245899979));
#46361=CARTESIAN_POINT('Ctrl Pts',(0.119647278325489,1.80075783715867,8.53850089092351));
#46362=CARTESIAN_POINT('Ctrl Pts',(0.119267043640176,1.80060608634855,8.53847578335171));
#46363=CARTESIAN_POINT('Ctrl Pts',(0.118514311687826,1.80030733423381,8.53842606820371));
#46364=CARTESIAN_POINT('Ctrl Pts',(0.118141827483509,1.80016030185208,8.5384014617286));
#46365=CARTESIAN_POINT('Ctrl Pts',(0.11732051866197,1.7998378709188,8.5383471936368));
#46366=CARTESIAN_POINT('Ctrl Pts',(0.116871573357984,1.79966278423998,8.53831752159487));
#46367=CARTESIAN_POINT('Ctrl Pts',(0.115303233475435,1.7990551876398,8.53821383687887));
#46368=CARTESIAN_POINT('Ctrl Pts',(0.114181827616396,1.79862792777678,8.53813964833862));
#46369=CARTESIAN_POINT('Ctrl Pts',(0.102384579787537,1.79420842873743,8.53735859642527));
#46370=CARTESIAN_POINT('Ctrl Pts',(0.0915077199919616,1.79077941215271,
8.53663302107544));
#46371=CARTESIAN_POINT('Ctrl Pts',(0.059646714208816,1.7825633488805,8.53448924977191));
#46372=CARTESIAN_POINT('Ctrl Pts',(0.0383369386996806,1.77929166876649,
8.53302925433063));
#46373=CARTESIAN_POINT('Ctrl Pts',(-0.00061308625369795,1.77725076947602,
8.53039440946308));
#46374=CARTESIAN_POINT('Ctrl Pts',(-0.0181376951682772,1.77775997224327,
8.5292230118871));
#46375=CARTESIAN_POINT('Ctrl Pts',(-0.0362385210700665,1.77976813952959,
8.52808043858649));
#46376=CARTESIAN_POINT('Ctrl Pts',(-0.0369405346626418,1.77984836125532,
8.52803623408479));
#46377=CARTESIAN_POINT('Ctrl Pts',(-0.037945127639853,1.77996650816732,
8.52797313761739));
#46378=CARTESIAN_POINT('Ctrl Pts',(-0.0382479195091772,1.78000255428944,
8.52795414080838));
#46379=CARTESIAN_POINT('Ctrl Pts',(-0.0387716975116797,1.78006566195025,
8.52792131636));
#46380=CARTESIAN_POINT('Ctrl Pts',(-0.0389927072337549,1.78009252278973,
8.52790747732112));
#46381=CARTESIAN_POINT('Ctrl Pts',(-0.0394187703746862,1.78014475327584,
8.5278808204495));
#46382=CARTESIAN_POINT('Ctrl Pts',(-0.0396238267703211,1.78017009103665,
8.52786800081712));
#46383=CARTESIAN_POINT('Ctrl Pts',(-0.0401110597167236,1.78023077167172,
8.52783756325244));
#46384=CARTESIAN_POINT('Ctrl Pts',(-0.0403932147010553,1.78026629094695,
8.52781995534992));
#46385=CARTESIAN_POINT('Ctrl Pts',(-0.0412394189988933,1.78037395397081,
8.52776720208886));
#46386=CARTESIAN_POINT('Ctrl Pts',(-0.0418033285563329,1.78044721764185,
8.52773211960848));
#46387=CARTESIAN_POINT('Ctrl Pts',(-0.0472989555515489,1.78117601106265,
8.52739089903997));
#46388=CARTESIAN_POINT('Ctrl Pts',(-0.0522153922839701,1.78194420840323,
8.52709096897759));
#46389=CARTESIAN_POINT('Ctrl Pts',(-0.0576514372948319,1.78292305760914,
8.52676331364816));
#46390=CARTESIAN_POINT('Ctrl Pts',(-0.0581902392782435,1.78302149650437,
8.52673088115274));
#46391=CARTESIAN_POINT('Ctrl Pts',(-0.0594289335595994,1.7832510702173,
8.52665641441541));
#46392=CARTESIAN_POINT('Ctrl Pts',(-0.0601286495151927,1.78338315239774,
8.52661441925532));
#46393=CARTESIAN_POINT('Ctrl Pts',(-0.0640974524223875,1.78414595633043,
8.52637658892838));
#46394=CARTESIAN_POINT('Ctrl Pts',(-0.0673571468810866,1.78482500661229,
8.52618266571173));
#46395=CARTESIAN_POINT('Ctrl Pts',(-0.0939570689454248,1.79079777274573,
8.52460758253531));
#46396=CARTESIAN_POINT('Ctrl Pts',(-0.116652702769177,1.79862606677382,
8.52330505956185));
#46397=CARTESIAN_POINT('Ctrl Pts',(-0.152177925289865,1.81550042258348,
8.52107365207062));
#46398=CARTESIAN_POINT('Ctrl Pts',(-0.165589600697517,1.82309185214857,
8.52018148354223));
#46399=CARTESIAN_POINT('Ctrl Pts',(-0.18044329501253,1.83296559364849,8.51910557955796));
#46400=CARTESIAN_POINT('Ctrl Pts',(-0.182464502823773,1.83434258604206,
8.51895720877051));
#46401=CARTESIAN_POINT('Ctrl Pts',(-0.185049503894568,1.83614709296875,
8.51876482142896));
#46402=CARTESIAN_POINT('Ctrl Pts',(-0.1856278702302,1.83655366918151,8.51872160502484));
#46403=CARTESIAN_POINT('Ctrl Pts',(-0.186558927169982,1.83721276577405,
8.51865175524905));
#46404=CARTESIAN_POINT('Ctrl Pts',(-0.186912456152261,1.83746410243329,
8.51862516735949));
#46405=CARTESIAN_POINT('Ctrl Pts',(-0.187585667564541,1.83794476205304,
8.51857441162068));
#46406=CARTESIAN_POINT('Ctrl Pts',(-0.187905439826657,1.8381739583379,8.5185502486821));
#46407=CARTESIAN_POINT('Ctrl Pts',(-0.188634696279859,1.83869867586434,
8.51849501953882));
#46408=CARTESIAN_POINT('Ctrl Pts',(-0.189043906424451,1.83899457462573,
8.51846393877576));
#46409=CARTESIAN_POINT('Ctrl Pts',(-0.190293911732564,1.83990293191513,
8.51836872048318));
#46410=CARTESIAN_POINT('Ctrl Pts',(-0.191132432326863,1.84051849595587,
8.51830446256138));
#46411=CARTESIAN_POINT('Ctrl Pts',(-0.197318575266951,1.84510604319358,
8.51782752560934));
#46412=CARTESIAN_POINT('Ctrl Pts',(-0.202544537704322,1.84923866140214,
8.51740856985307));
#46413=CARTESIAN_POINT('Ctrl Pts',(-0.209063715133185,1.85473073588962,
8.51686434549041));
#46414=CARTESIAN_POINT('Ctrl Pts',(-0.210478551995268,1.85594380190856,
8.51674488268412));
#46415=CARTESIAN_POINT('Ctrl Pts',(-0.21377955950078,1.85882410445391,8.51646295705187));
#46416=CARTESIAN_POINT('Ctrl Pts',(-0.215656855500674,1.86050128853268,
8.51630011975769));
#46417=CARTESIAN_POINT('Ctrl Pts',(-0.238900199308489,1.88176186253411,
8.51425242374418));
#46418=CARTESIAN_POINT('Ctrl Pts',(-0.257548298085593,1.9041183484057,8.51225441121164));
#46419=CARTESIAN_POINT('Ctrl Pts',(-0.27700718463596,1.93511721110082,8.50981832344622));
#46420=CARTESIAN_POINT('Ctrl Pts',(-0.280830892652184,1.9417175237896,8.50931740457639));
#46421=CARTESIAN_POINT('Ctrl Pts',(-0.285971060699911,1.95136404341727,
8.50861652560779));
#46422=CARTESIAN_POINT('Ctrl Pts',(-0.287480143188643,1.95430420553925,
8.50840692419111));
#46423=CARTESIAN_POINT('Ctrl Pts',(-0.289173389079175,1.95773195936524,
8.50816762379397));
#46424=CARTESIAN_POINT('Ctrl Pts',(-0.289401853078545,1.95819727865373,
8.5081352454797));
#46425=CARTESIAN_POINT('Ctrl Pts',(-0.289747020442032,1.95890459982595,
8.50808619227389));
#46426=CARTESIAN_POINT('Ctrl Pts',(-0.289864544181349,1.9591461969519,8.50806946638598));
#46427=CARTESIAN_POINT('Ctrl Pts',(-0.290076879762431,1.95958409287362,
8.50803920358847));
#46428=CARTESIAN_POINT('Ctrl Pts',(-0.290171794236656,1.95978034026154,
8.50802566027761));
#46429=CARTESIAN_POINT('Ctrl Pts',(-0.290362409942377,1.96017548414179,
8.50799842960865));
#46430=CARTESIAN_POINT('Ctrl Pts',(-0.290458105538497,1.96037438175527,
8.50798474261956));
#46431=CARTESIAN_POINT('Ctrl Pts',(-0.290731258298616,1.9609436096115,8.50794562752195));
#46432=CARTESIAN_POINT('Ctrl Pts',(-0.290908212893175,1.96131418264468,
8.50792023079673));
#46433=CARTESIAN_POINT('Ctrl Pts',(-0.291668265761645,1.96291371798913,
8.5078108957311));
#46434=CARTESIAN_POINT('Ctrl Pts',(-0.292244299202433,1.96414605009278,
8.5077273899757));
#46435=CARTESIAN_POINT('Ctrl Pts',(-0.302951756978391,1.98743623537348,
8.50616221346712));
#46436=CARTESIAN_POINT('Ctrl Pts',(-0.310568753063442,2.0105694090921,8.50482337218961));
#46437=CARTESIAN_POINT('Ctrl Pts',(-0.318506063112586,2.04871165398499,
8.5026445285078));
#46438=CARTESIAN_POINT('Ctrl Pts',(-0.320511050883701,2.06326813640315,
8.50182002241191));
#46439=CARTESIAN_POINT('Ctrl Pts',(-0.322020665383746,2.08524009578906,
8.50054282176863));
#46440=CARTESIAN_POINT('Ctrl Pts',(-0.322273441735044,2.0925851041351,8.50011063335046));
#46441=CARTESIAN_POINT('Ctrl Pts',(-0.322275785453835,2.10368636016889,
8.49944597289085));
#46442=CARTESIAN_POINT('Ctrl Pts',(-0.322210971854595,2.10744035923576,
8.49921924710806));
#46443=CARTESIAN_POINT('Ctrl Pts',(-0.322053560396658,2.11197020470806,
8.49894302119048));
#46444=CARTESIAN_POINT('Ctrl Pts',(-0.322023708370871,2.11274805064671,
8.49889549491129));
#46445=CARTESIAN_POINT('Ctrl Pts',(-0.321970211184815,2.11402159052878,
8.49881752524605));
#46446=CARTESIAN_POINT('Ctrl Pts',(-0.321948238545141,2.11451735460327,
8.49878713432552));
#46447=CARTESIAN_POINT('Ctrl Pts',(-0.321906840582164,2.1154050511086,8.49873264716256));
#46448=CARTESIAN_POINT('Ctrl Pts',(-0.321887844281587,2.11579700335002,
8.49870856442063));
#46449=CARTESIAN_POINT('Ctrl Pts',(-0.321846097182538,2.11662701931167,
8.4986575132848));
#46450=CARTESIAN_POINT('Ctrl Pts',(-0.32182316779078,2.11706507289467,8.49863053933591));
#46451=CARTESIAN_POINT('Ctrl Pts',(-0.321759761867809,2.11823080992015,
8.49855867392898));
#46452=CARTESIAN_POINT('Ctrl Pts',(-0.321717711300987,2.1189584020656,8.49851373317104));
#46453=CARTESIAN_POINT('Ctrl Pts',(-0.321510499093469,2.12234431857016,
8.49830419113506));
#46454=CARTESIAN_POINT('Ctrl Pts',(-0.32131485862497,2.12500061082128,8.49813863609256));
#46455=CARTESIAN_POINT('Ctrl Pts',(-0.319551091077461,2.14547936150679,
8.4968529344725));
#46456=CARTESIAN_POINT('Ctrl Pts',(-0.316534473950642,2.16314276994974,
8.49568659032966));
#46457=CARTESIAN_POINT('Ctrl Pts',(-0.308147156200516,2.19567255712307,
8.49344010755191));
#46458=CARTESIAN_POINT('Ctrl Pts',(-0.303118679325512,2.21057552285883,
8.49237030271836));
#46459=CARTESIAN_POINT('Ctrl Pts',(-0.291355934509451,2.23851451077511,
8.49033006846181));
#46460=CARTESIAN_POINT('Ctrl Pts',(-0.284778302024963,2.25157830538204,
8.48936058054594));
#46461=CARTESIAN_POINT('Ctrl Pts',(-0.276872479281622,2.26493524181735,
8.48838445998296));
#46462=CARTESIAN_POINT('Ctrl Pts',(-0.276405630831196,2.26571641762082,
8.48832743180554));
#46463=CARTESIAN_POINT('Ctrl Pts',(-0.275773252301414,2.26676446724762,
8.48825101284272));
#46464=CARTESIAN_POINT('Ctrl Pts',(-0.275610637857428,2.2670330821219,8.48823143482726));
#46465=CARTESIAN_POINT('Ctrl Pts',(-0.275336178426266,2.26748495624063,
8.48819851424768));
#46466=CARTESIAN_POINT('Ctrl Pts',(-0.275224542880367,2.26766834141905,
8.48818515798214));
#46467=CARTESIAN_POINT('Ctrl Pts',(-0.275010070036646,2.26801986742623,
8.48815956355868));
#46468=CARTESIAN_POINT('Ctrl Pts',(-0.274907262497061,2.26818802424107,
8.48814732362291));
#46469=CARTESIAN_POINT('Ctrl Pts',(-0.274663545388898,2.26858583883783,
8.48811837526481));
#46470=CARTESIAN_POINT('Ctrl Pts',(-0.274522502198236,2.26881541401881,
8.48810167579746));
#46471=CARTESIAN_POINT('Ctrl Pts',(-0.274107321816106,2.26948930443415,
8.48805267440352));
#46472=CARTESIAN_POINT('Ctrl Pts',(-0.273832391017473,2.26993313340687,
8.48802042462228));
#46473=CARTESIAN_POINT('Ctrl Pts',(-0.271759371546199,2.27326157590052,
8.48777872796356));
#46474=CARTESIAN_POINT('Ctrl Pts',(-0.26991673964707,2.2761183851991,8.48757216496842));
#46475=CARTESIAN_POINT('Ctrl Pts',(-0.263489649158483,2.28574503870713,
8.48687722803608));
#46476=CARTESIAN_POINT('Ctrl Pts',(-0.258692667108727,2.29236980059292,
8.48640089321402));
#46477=CARTESIAN_POINT('Ctrl Pts',(-0.239115499277049,2.31734758910587,
8.48458271450017));
#46478=CARTESIAN_POINT('Ctrl Pts',(-0.222592864509201,2.3342407165758,8.48329903224635));
#46479=CARTESIAN_POINT('Ctrl Pts',(-0.201550953132475,2.35149897478235,
8.48174834833523));
#46480=CARTESIAN_POINT('Ctrl Pts',(-0.19868723042998,2.35376742186803,8.4815390326261));
#46481=CARTESIAN_POINT('Ctrl Pts',(-0.186348391828434,2.36320450452221,
8.48064275049407));
#46482=CARTESIAN_POINT('Ctrl Pts',(-0.176520255926883,2.36989420827705,
8.47994210978705));
#46483=CARTESIAN_POINT('Ctrl Pts',(-0.165411866279095,2.37658864728621,
8.47915376593937));
#46484=CARTESIAN_POINT('Ctrl Pts',(-0.164474824113691,2.37714688795046,
8.47908729646465));
#46485=CARTESIAN_POINT('Ctrl Pts',(-0.16307973226661,2.37796844365138,8.47898837364845));
#46486=CARTESIAN_POINT('Ctrl Pts',(-0.162623833112833,2.37823541047208,
8.4789560529578));
#46487=CARTESIAN_POINT('Ctrl Pts',(-0.161842382388833,2.3786904380095,8.47890066203942));
#46488=CARTESIAN_POINT('Ctrl Pts',(-0.161517153375179,2.37887905288648,
8.47887761192549));
#46489=CARTESIAN_POINT('Ctrl Pts',(-0.160883857216363,2.37924485028636,
8.47883273316718));
#46490=CARTESIAN_POINT('Ctrl Pts',(-0.160575825437108,2.37942209327093,
8.4788109067476));
#46491=CARTESIAN_POINT('Ctrl Pts',(-0.159838435219886,2.37984476918095,
8.47875866228929));
#46492=CARTESIAN_POINT('Ctrl Pts',(-0.159408804745186,2.38008972344024,
8.47872822705235));
#46493=CARTESIAN_POINT('Ctrl Pts',(-0.158118907401681,2.38082123057493,
8.4786368618463));
#46494=CARTESIAN_POINT('Ctrl Pts',(-0.157256970349238,2.38130481272324,
8.47857582528764));
#46495=CARTESIAN_POINT('Ctrl Pts',(-0.149619138838061,2.38554387638036,
8.47803507981947));
#46496=CARTESIAN_POINT('Ctrl Pts',(-0.142712617699471,2.38905757912737,
8.47754680689738));
#46497=CARTESIAN_POINT('Ctrl Pts',(-0.129698918525619,2.3950981941825,8.47662685578607));
#46498=CARTESIAN_POINT('Ctrl Pts',(-0.123627528937131,2.39769275836787,
8.4761977146619));
#46499=CARTESIAN_POINT('Ctrl Pts',(-0.102087708102175,2.40612504804404,
8.47467633409553));
#46500=CARTESIAN_POINT('Ctrl Pts',(-0.0862546391665527,2.41095738997894,
8.473558415275));
#46501=CARTESIAN_POINT('Ctrl Pts',(-0.0513200531372833,2.41874522977344,
8.47113669395405));
#46502=CARTESIAN_POINT('Ctrl Pts',(-0.0321773583053179,2.42124301462419,
8.46983732056639));
#46503=CARTESIAN_POINT('Ctrl Pts',(-0.0125010861032906,2.42203272781696,
8.46859627546926));
#46504=CARTESIAN_POINT('Ctrl Pts',(-0.012077936103984,2.42204887579857,
8.46856963153581));
#46505=CARTESIAN_POINT('Ctrl Pts',(-0.0108549200461107,2.42209313390064,
8.46849275730078));
#46506=CARTESIAN_POINT('Ctrl Pts',(-0.0100549721379043,2.42211909872408,
8.46844264094765));
#46507=CARTESIAN_POINT('Ctrl Pts',(-0.00895739237750149,2.42215063145364,
8.46837411265111));
#46508=CARTESIAN_POINT('Ctrl Pts',(-0.00865984582271966,2.4221587672193,
8.46835555873018));
#46509=CARTESIAN_POINT('Ctrl Pts',(-0.00815219178171078,2.42217194409805,
8.46832394409944));
#46510=CARTESIAN_POINT('Ctrl Pts',(-0.0079420906038569,2.42217719191801,
8.46831087178187));
#46511=CARTESIAN_POINT('Ctrl Pts',(-0.00753352610410729,2.42218699697156,
8.46828547464068));
#46512=CARTESIAN_POINT('Ctrl Pts',(-0.00733506520782097,2.42219157632017,
8.4682731486985));
#46513=CARTESIAN_POINT('Ctrl Pts',(-0.00685662109197878,2.42220217379484,
8.46824345940072));
#46514=CARTESIAN_POINT('Ctrl Pts',(-0.00657663424233016,2.42220801035106,
8.46822610637579));
#46515=CARTESIAN_POINT('Ctrl Pts',(-0.00572272634429809,2.42222469726816,
8.46817324667176));
#46516=CARTESIAN_POINT('Ctrl Pts',(-0.00514877965845295,2.42223437930549,
8.46813780537541));
#46517=CARTESIAN_POINT('Ctrl Pts',(0.000633699465098556,2.42231647186573,
8.46778159438697));
#46518=CARTESIAN_POINT('Ctrl Pts',(0.00584359965130935,2.42226413012393,
8.46746766646999));
#46519=CARTESIAN_POINT('Ctrl Pts',(0.0159055491386708,2.42191891892699,
8.46687100309641));
#46520=CARTESIAN_POINT('Ctrl Pts',(0.0207566471348524,2.4216425700655,8.4665876715227));
#46521=CARTESIAN_POINT('Ctrl Pts',(0.0591317254156498,2.41858458927343,
8.4643679690945));
#46522=CARTESIAN_POINT('Ctrl Pts',(0.0920384184708004,2.41067979644696,
8.46257190175339));
#46523=CARTESIAN_POINT('Ctrl Pts',(0.123606318708089,2.39762883011885,8.46056071873003));
#46524=CARTESIAN_POINT('Ctrl Pts',(0.124083288093251,2.39743029461414,8.46053026657131));
#46525=CARTESIAN_POINT('Ctrl Pts',(0.130704846505074,2.39465541277089,8.46010660320732));
#46526=CARTESIAN_POINT('Ctrl Pts',(0.136768205745549,2.39189042007938,8.45970771039502));
#46527=CARTESIAN_POINT('Ctrl Pts',(0.143673888286678,2.38847889288015,8.45923894994212));
#46528=CARTESIAN_POINT('Ctrl Pts',(0.144604321393027,2.38801362469066,8.4591754835637));
#46529=CARTESIAN_POINT('Ctrl Pts',(0.145983053473978,2.38731581708626,8.45908097307208));
#46530=CARTESIAN_POINT('Ctrl Pts',(0.146433091216151,2.38708671240903,8.45905004957351));
#46531=CARTESIAN_POINT('Ctrl Pts',(0.147232778409009,2.38667723902394,8.45899496812197));
#46532=CARTESIAN_POINT('Ctrl Pts',(0.147582640338916,2.38649728564306,8.45897082482998));
#46533=CARTESIAN_POINT('Ctrl Pts',(0.148317533156538,2.38611758619669,8.45892001568865));
#46534=CARTESIAN_POINT('Ctrl Pts',(0.148702491793071,2.3859177026773,8.45889334502304));
#46535=CARTESIAN_POINT('Ctrl Pts',(0.149701272873249,2.3853965390907,8.45882400306558));
#46536=CARTESIAN_POINT('Ctrl Pts',(0.150314462530237,2.3850740569871,8.45878128930344));
#46537=CARTESIAN_POINT('Ctrl Pts',(0.152985651004681,2.38365823971665,8.45859459350925));
#46538=CARTESIAN_POINT('Ctrl Pts',(0.155032755127375,2.38254459957924,8.45844989170558));
#46539=CARTESIAN_POINT('Ctrl Pts',(0.169542717954004,2.37444590541897,8.45741237007705));
#46540=CARTESIAN_POINT('Ctrl Pts',(0.181539300580954,2.36666209093851,8.45649054429966));
#46541=CARTESIAN_POINT('Ctrl Pts',(0.2124066727379,2.34358369364697,8.45394117253054));
#46542=CARTESIAN_POINT('Ctrl Pts',(0.230130546939323,2.32691274725929,8.45227329355706));
#46543=CARTESIAN_POINT('Ctrl Pts',(0.252479637583739,2.30055271265595,8.44997520428305));
#46544=CARTESIAN_POINT('Ctrl Pts',(0.258763476280781,2.29237689819328,8.44930239343237));
#46545=CARTESIAN_POINT('Ctrl Pts',(0.265065210977219,2.28330889483427,8.44860924859008));
#46546=CARTESIAN_POINT('Ctrl Pts',(0.265483033300111,2.28270324586698,8.44856319831509));
#46547=CARTESIAN_POINT('Ctrl Pts',(0.266061090679892,2.28185916024782,8.44849936400496));
#46548=CARTESIAN_POINT('Ctrl Pts',(0.266223082592409,2.28162193820238,8.44848146176619));
#46549=CARTESIAN_POINT('Ctrl Pts',(0.266501471483465,2.28121309093134,8.44845067305878));
#46550=CARTESIAN_POINT('Ctrl Pts',(0.266618020005385,2.28104156991339,8.44843777625843));
#46551=CARTESIAN_POINT('Ctrl Pts',(0.266859066383636,2.28068609147783,8.44841108870784));
#46552=CARTESIAN_POINT('Ctrl Pts',(0.26698353939582,2.2805021181499,8.44839729972045));
#46553=CARTESIAN_POINT('Ctrl Pts',(0.267276786472405,2.28006772679039,8.44836479511365));
#46554=CARTESIAN_POINT('Ctrl Pts',(0.267445399497575,2.27981719914357,8.44834609048887));
#46555=CARTESIAN_POINT('Ctrl Pts',(0.267980947217316,2.27901905506402,8.44828663210428));
#46556=CARTESIAN_POINT('Ctrl Pts',(0.268346557008565,2.27847054520906,8.44824596752253));
#46557=CARTESIAN_POINT('Ctrl Pts',(0.273075573071226,2.2713284044254,8.44771897692713));
#46558=CARTESIAN_POINT('Ctrl Pts',(0.277197006048649,2.26457683598257,8.4472484414298));
#46559=CARTESIAN_POINT('Ctrl Pts',(0.284822210338678,2.25098481652014,8.44634047671439));
#46560=CARTESIAN_POINT('Ctrl Pts',(0.288337954436874,2.24415735384519,8.44590276863756));
#46561=CARTESIAN_POINT('Ctrl Pts',(0.301709367289927,2.21573975733092,8.44412959504599));
#46562=CARTESIAN_POINT('Ctrl Pts',(0.30940958498516,2.19321983332688,8.44283028537474));
#46563=CARTESIAN_POINT('Ctrl Pts',(0.315331971276558,2.16662789759444,8.44125389909873));
#46564=CARTESIAN_POINT('Ctrl Pts',(0.316039833925883,2.16318505377851,8.44104916535892));
#46565=CARTESIAN_POINT('Ctrl Pts',(0.317021805566758,2.15797871684312,8.4407381637471));
#46566=CARTESIAN_POINT('Ctrl Pts',(0.317337820803846,2.15622334148638,8.440633068467));
#46567=CARTESIAN_POINT('Ctrl Pts',(0.317708020680221,2.15406435822743,8.44050347653155));
#46568=CARTESIAN_POINT('Ctrl Pts',(0.317776036828847,2.15366313120131,8.44047937901269));
#46569=CARTESIAN_POINT('Ctrl Pts',(0.317893641023428,2.15296132014564,8.44043720331767));
#46570=CARTESIAN_POINT('Ctrl Pts',(0.317943563248465,2.15266079208174,8.44041913484589));
#46571=CARTESIAN_POINT('Ctrl Pts',(0.318882065954678,2.14696109310315,8.44007629903359));
#46572=CARTESIAN_POINT('Ctrl Pts',(0.319633380678859,2.14154049495462,8.43974757154402));
#46573=CARTESIAN_POINT('Ctrl Pts',(0.320345136182677,2.13522708411542,8.43936073343787));
#46574=CARTESIAN_POINT('Ctrl Pts',(0.320440355906064,2.13435013848163,8.43930691289814));
#46575=CARTESIAN_POINT('Ctrl Pts',(0.320586183607758,2.13295370874127,8.43922106639881));
#46576=CARTESIAN_POINT('Ctrl Pts',(0.320639132422318,2.13243446923247,8.43918911417061));
#46577=CARTESIAN_POINT('Ctrl Pts',(0.320730157307969,2.13151982883124,8.43913277382025));
#46578=CARTESIAN_POINT('Ctrl Pts',(0.320768764226409,2.13112448089151,8.43910840245615));
#46579=CARTESIAN_POINT('Ctrl Pts',(0.320846891352525,2.13030884586814,8.43905808361597));
#46580=CARTESIAN_POINT('Ctrl Pts',(0.320886316885579,2.12988855067324,8.43903213321063));
#46581=CARTESIAN_POINT('Ctrl Pts',(0.320983589669415,2.12882919583166,8.43896667116294));
#46582=CARTESIAN_POINT('Ctrl Pts',(0.321040354101242,2.12819004076621,8.43892712554302));
#46583=CARTESIAN_POINT('Ctrl Pts',(0.321257221662141,2.1256625160985,8.43877054455687));
#46584=CARTESIAN_POINT('Ctrl Pts',(0.321402572872833,2.12377294905575,8.43865304664614));
#46585=CARTESIAN_POINT('Ctrl Pts',(0.322225779338296,2.11167699452783,8.43789797771844));
#46586=CARTESIAN_POINT('Ctrl Pts',(0.322433989746081,2.10144551402398,8.43724575640955));
#46587=CARTESIAN_POINT('Ctrl Pts',(0.321563493707716,2.06949692422061,8.43516507676452));
#46588=CARTESIAN_POINT('Ctrl Pts',(0.318775428963706,2.04788923723111,8.43368979177019));
#46589=CARTESIAN_POINT('Ctrl Pts',(0.310748519454833,2.01350793662296,8.43130476958646));
#46590=CARTESIAN_POINT('Ctrl Pts',(0.306828908671587,2.0004931760395,8.43039422463863));
#46591=CARTESIAN_POINT('Ctrl Pts',(0.300682585840457,1.98394952672803,8.42925620202979));
#46592=CARTESIAN_POINT('Ctrl Pts',(0.299193432046476,1.98016251080655,8.42899711582324));
#46593=CARTESIAN_POINT('Ctrl Pts',(0.297426861299292,1.97590839526436,8.42870850438163));
#46594=CARTESIAN_POINT('Ctrl Pts',(0.29721960556284,1.97541280054856,8.42867491957264));
#46595=CARTESIAN_POINT('Ctrl Pts',(0.296903849808689,1.97466303032856,8.42862416994687));
#46596=CARTESIAN_POINT('Ctrl Pts',(0.296796261687967,1.97440847541695,8.42860695037642));
#46597=CARTESIAN_POINT('Ctrl Pts',(0.296608469552856,1.97396574570263,8.42857702019208));
#46598=CARTESIAN_POINT('Ctrl Pts',(0.296528413784995,1.973777508797,8.42856430053891));
#46599=CARTESIAN_POINT('Ctrl Pts',(0.296360195310437,1.97338301624875,8.4285376561597));
#46600=CARTESIAN_POINT('Ctrl Pts',(0.296271996507548,1.97317677647808,8.42852373373438));
#46601=CARTESIAN_POINT('Ctrl Pts',(0.296059792160569,1.97268199764916,8.42849035008443));
#46602=CARTESIAN_POINT('Ctrl Pts',(0.295935579585396,1.97239354642408,8.42847090154602));
#46603=CARTESIAN_POINT('Ctrl Pts',(0.295517978832963,1.97142766707352,8.4284058228726));
#46604=CARTESIAN_POINT('Ctrl Pts',(0.295222681928338,1.97075105916104,8.42836030852752));
#46605=CARTESIAN_POINT('Ctrl Pts',(0.292143635000749,1.9637617088338,8.42789085175711));
#46606=CARTESIAN_POINT('Ctrl Pts',(0.289159934428492,1.9575383408469,8.42747880457437));
#46607=CARTESIAN_POINT('Ctrl Pts',(0.282763545180118,1.94522733872143,8.42666641568514));
#46608=CARTESIAN_POINT('Ctrl Pts',(0.279348460350714,1.93914526063271,8.42626645641119));
#46609=CARTESIAN_POINT('Ctrl Pts',(0.266007025349944,1.91709326114014,8.42480436291184));
#46610=CARTESIAN_POINT('Ctrl Pts',(0.254886617234915,1.90189029489291,8.42377037554917));
#46611=CARTESIAN_POINT('Ctrl Pts',(0.230964781842949,1.87455951953245,8.42171324401345));
#46612=CARTESIAN_POINT('Ctrl Pts',(0.218371364463552,1.86234067864355,8.42069754663236));
#46613=CARTESIAN_POINT('Ctrl Pts',(0.203861959295889,1.85039408860272,8.41955585838056));
#46614=CARTESIAN_POINT('Ctrl Pts',(0.202870376834871,1.84958750114612,8.41947797902535));
#46615=CARTESIAN_POINT('Ctrl Pts',(0.201477930148679,1.84846853575541,8.41936880569683));
#46616=CARTESIAN_POINT('Ctrl Pts',(0.201081076601369,1.84815116742341,8.41933771221324));
#46617=CARTESIAN_POINT('Ctrl Pts',(0.200393484686969,1.84760395352241,8.41928387554943));
#46618=CARTESIAN_POINT('Ctrl Pts',(0.20010309655223,1.84737366778016,8.41926115001916));
#46619=CARTESIAN_POINT('Ctrl Pts',(0.199500293510443,1.84689731991891,8.41921399781411));
#46620=CARTESIAN_POINT('Ctrl Pts',(0.199187819217273,1.84665133422842,8.41918956814596));
#46621=CARTESIAN_POINT('Ctrl Pts',(0.198567510927362,1.84616487276236,8.41914109607354));
#46622=CARTESIAN_POINT('Ctrl Pts',(0.198259693412566,1.84592437704209,8.41911705452394));
#46623=CARTESIAN_POINT('Ctrl Pts',(0.197228884254685,1.84512202676671,8.41903658410609));
#46624=CARTESIAN_POINT('Ctrl Pts',(0.196503940468409,1.84456269775824,8.41898005534832));
#46625=CARTESIAN_POINT('Ctrl Pts',(0.191265966621974,1.84055684314574,8.4185720605005));
#46626=CARTESIAN_POINT('Ctrl Pts',(0.186665168955711,1.83722722801407,8.41821603991749));
#46627=CARTESIAN_POINT('Ctrl Pts',(0.171377611646791,1.82676769722387,8.41703950718014));
#46628=CARTESIAN_POINT('Ctrl Pts',(0.160353250784354,1.82015550037184,8.41620043054406));
#46629=CARTESIAN_POINT('Ctrl Pts',(0.137801481081588,1.80840025676526,8.41450692534501));
#46630=CARTESIAN_POINT('Ctrl Pts',(0.126307138110754,1.80324060512717,8.41365461028903));
#46631=CARTESIAN_POINT('Ctrl Pts',(0.0966802994926767,1.79197528325571,
8.41151010847482));
#46632=CARTESIAN_POINT('Ctrl Pts',(0.0782485205103509,1.78678496188719,
8.41022172776056));
#46633=CARTESIAN_POINT('Ctrl Pts',(0.058344093607787,1.78304820632988,8.40894512949826));
#46634=CARTESIAN_POINT('Ctrl Pts',(0.0572235998657943,1.78284399346681,
8.40887364978822));
#46635=CARTESIAN_POINT('Ctrl Pts',(0.0557251203960356,1.78257909161456,
8.4087785922144));
#46636=CARTESIAN_POINT('Ctrl Pts',(0.0553480926923045,1.78251313292935,
8.40875472025652));
#46637=CARTESIAN_POINT('Ctrl Pts',(0.0547590036467049,1.78241115666591,
8.40871749288854));
#46638=CARTESIAN_POINT('Ctrl Pts',(0.0545470238067666,1.78237467971657,
8.40870411131649));
#46639=CARTESIAN_POINT('Ctrl Pts',(0.0541408224708725,1.78230520026609,
8.40867849709148));
#46640=CARTESIAN_POINT('Ctrl Pts',(0.0539466086350098,1.78227216386844,
8.40866626260428));
#46641=CARTESIAN_POINT('Ctrl Pts',(0.0534874977743349,1.78219450072746,
8.40863736974818));
#46642=CARTESIAN_POINT('Ctrl Pts',(0.0532225754954017,1.78215002714343,
8.40862072022937));
#46643=CARTESIAN_POINT('Ctrl Pts',(0.0526740413257244,1.78205864749855,
8.40858629285446));
#46644=CARTESIAN_POINT('Ctrl Pts',(0.0523904215075124,1.78201178953329,
8.40856851774219));
#46645=CARTESIAN_POINT('Ctrl Pts',(0.0508314461480352,1.78175636733094,
8.40847095178339));
#46646=CARTESIAN_POINT('Ctrl Pts',(0.0495548837201791,1.7815550922314,8.40839156992871));
#46647=CARTESIAN_POINT('Ctrl Pts',(0.0236233562991574,1.777626190203,8.40678874700665));
#46648=CARTESIAN_POINT('Ctrl Pts',(-0.00138522393482243,1.77676407707121,
8.40541678110286));
#46649=CARTESIAN_POINT('Ctrl Pts',(-0.0347810103223249,1.77949292861138,
8.40354215422207));
#46650=CARTESIAN_POINT('Ctrl Pts',(-0.0432842144054608,1.78053017184378,
8.40306158698686));
#46651=CARTESIAN_POINT('Ctrl Pts',(-0.0577936612301802,1.78289002405372,
8.40222543633497));
#46652=CARTESIAN_POINT('Ctrl Pts',(-0.0638219180456825,1.78404810238222,
8.40187320858196));
#46653=CARTESIAN_POINT('Ctrl Pts',(-0.072535324184587,1.78598156579259,
8.40135441934715));
#46654=CARTESIAN_POINT('Ctrl Pts',(-0.0752494111104413,1.78662087531697,
8.40119144936464));
#46655=CARTESIAN_POINT('Ctrl Pts',(-0.079838386749779,1.78776487067895,
8.40091332266734));
#46656=CARTESIAN_POINT('Ctrl Pts',(-0.0817176553062199,1.78825143373672,
8.40079868626428));
#46657=CARTESIAN_POINT('Ctrl Pts',(-0.088992108317433,1.7902051639539,8.4003519056634));
#46658=CARTESIAN_POINT('Ctrl Pts',(-0.0943529026362266,1.79179558779443,
8.40001613091516));
#46659=CARTESIAN_POINT('Ctrl Pts',(-0.100596184668807,1.7938259758455,8.39961642189194));
#46660=CARTESIAN_POINT('Ctrl Pts',(-0.101521608472813,1.79413158316484,
8.39955694895443));
#46661=CARTESIAN_POINT('Ctrl Pts',(-0.102918198846199,1.79459982252448,
8.39946685033177));
#46662=CARTESIAN_POINT('Ctrl Pts',(-0.103390403441528,1.79475935963963,
8.39943632692282));
#46663=CARTESIAN_POINT('Ctrl Pts',(-0.104233935602673,1.79504653392846,
8.399381692835));
#46664=CARTESIAN_POINT('Ctrl Pts',(-0.10460540436797,1.79517375576385,8.39935759594498));
#46665=CARTESIAN_POINT('Ctrl Pts',(-0.105390164036805,1.79544412622543,
8.3993066094367));
#46666=CARTESIAN_POINT('Ctrl Pts',(-0.105803397573905,1.79558743786579,
8.39927971445341));
#46667=CARTESIAN_POINT('Ctrl Pts',(-0.106642644603475,1.7958804086175,8.3992249969192));
#46668=CARTESIAN_POINT('Ctrl Pts',(-0.107068637754152,1.79603012268181,
8.39919717259082));
#46669=CARTESIAN_POINT('Ctrl Pts',(-0.108917066695695,1.79668411543232,
8.39907622029489));
#46670=CARTESIAN_POINT('Ctrl Pts',(-0.11033624690742,1.79719748062028,8.3989827904266));
#46671=CARTESIAN_POINT('Ctrl Pts',(-0.113762990340338,1.7984643377506,8.39875580114505));
#46672=CARTESIAN_POINT('Ctrl Pts',(-0.115766719405575,1.79922792699545,
8.39862190716099));
#46673=CARTESIAN_POINT('Ctrl Pts',(-0.123165075515661,1.80213220426508,
8.3981231198733));
#46674=CARTESIAN_POINT('Ctrl Pts',(-0.128508934187481,1.80439839912792,
8.39775406462739));
#46675=CARTESIAN_POINT('Ctrl Pts',(-0.142785921160656,1.81091321740087,
8.3967436828037));
#46676=CARTESIAN_POINT('Ctrl Pts',(-0.151588901810466,1.81543056617613,
8.39609401549238));
#46677=CARTESIAN_POINT('Ctrl Pts',(-0.167330418135048,1.82444636903274,
8.39488538772586));
#46678=CARTESIAN_POINT('Ctrl Pts',(-0.174330754932642,1.8288209983483,8.3943297014222));
#46679=CARTESIAN_POINT('Ctrl Pts',(-0.200266671530347,1.84644842700787,
8.39220992213573));
#46680=CARTESIAN_POINT('Ctrl Pts',(-0.217927563232293,1.86145663900082,
8.3906327048897));
#46681=CARTESIAN_POINT('Ctrl Pts',(-0.234696034382311,1.87913686989421,
8.38909498778569));
#46682=CARTESIAN_POINT('Ctrl Pts',(-0.235554393265944,1.88005255461656,
8.38901616330019));
#46683=CARTESIAN_POINT('Ctrl Pts',(-0.236677776230974,1.88126508249625,
8.38891288304588));
#46684=CARTESIAN_POINT('Ctrl Pts',(-0.236947616132483,1.88155741919167,
8.3888880657537));
#46685=CARTESIAN_POINT('Ctrl Pts',(-0.237364572506812,1.88201081924435,
8.38884970508989));
#46686=CARTESIAN_POINT('Ctrl Pts',(-0.23751206674639,1.88217153225899,8.38883613284982));
#46687=CARTESIAN_POINT('Ctrl Pts',(-0.23780544369527,1.88249185456545,8.38880913184293));
#46688=CARTESIAN_POINT('Ctrl Pts',(-0.23795132789488,1.88265145978188,8.3887957030185));
#46689=CARTESIAN_POINT('Ctrl Pts',(-0.238280542499722,1.883012367121,8.38876539296139));
#46690=CARTESIAN_POINT('Ctrl Pts',(-0.238463778095125,1.88321375437011,
8.38874851901017));
#46691=CARTESIAN_POINT('Ctrl Pts',(-0.238843356330097,1.88363199788749,
8.38871355548009));
#46692=CARTESIAN_POINT('Ctrl Pts',(-0.239039659474542,1.88384888989162,
8.3886954688972));
#46693=CARTESIAN_POINT('Ctrl Pts',(-0.239551123299324,1.88441554645347,
8.38864833118855));
#46694=CARTESIAN_POINT('Ctrl Pts',(-0.239865814738414,1.88476573643738,
8.38861931507781));
#46695=CARTESIAN_POINT('Ctrl Pts',(-0.243518763967195,1.88884871570301,
8.38828232115739));
#46696=CARTESIAN_POINT('Ctrl Pts',(-0.246770572182945,1.89265838646294,
8.3879806374866));
#46697=CARTESIAN_POINT('Ctrl Pts',(-0.257529154300123,1.90587451144742,
8.38697045727812));
#46698=CARTESIAN_POINT('Ctrl Pts',(-0.264597929459058,1.91562549457053,
8.38628549334185));
#46699=CARTESIAN_POINT('Ctrl Pts',(-0.273707122562489,1.92979793258131,
8.38533767482097));
#46700=CARTESIAN_POINT('Ctrl Pts',(-0.27621804062337,1.93390386019887,8.38506836014099));
#46701=CARTESIAN_POINT('Ctrl Pts',(-0.281201868151471,1.94247933827735,
8.38451379867739));
#46702=CARTESIAN_POINT('Ctrl Pts',(-0.283662348445672,1.9469545121841,8.38422866279686));
#46703=CARTESIAN_POINT('Ctrl Pts',(-0.296649314992381,1.97196548136546,
8.38265011148892));
#46704=CARTESIAN_POINT('Ctrl Pts',(-0.305051293354224,1.99352403315218,
8.38133791330004));
#46705=CARTESIAN_POINT('Ctrl Pts',(-0.311458891657275,2.01719514329423,
8.37985002401901));
#46706=CARTESIAN_POINT('Ctrl Pts',(-0.311828935184469,2.01859975085764,
8.37976159215863));
#46707=CARTESIAN_POINT('Ctrl Pts',(-0.3123226726781,2.02052666006364,8.37964006625184));
#46708=CARTESIAN_POINT('Ctrl Pts',(-0.312454579989572,2.02104685524011,
8.37960723773207));
#46709=CARTESIAN_POINT('Ctrl Pts',(-0.312677237688357,2.0219342346737,8.37955120031392));
#46710=CARTESIAN_POINT('Ctrl Pts',(-0.312768642430599,2.02230125487148,
8.37952801257533));
#46711=CARTESIAN_POINT('Ctrl Pts',(-0.312944483596293,2.02301265339138,
8.37948304659252));
#46712=CARTESIAN_POINT('Ctrl Pts',(-0.313028998241659,2.02335701200079,
8.3794612709058));
#46713=CARTESIAN_POINT('Ctrl Pts',(-0.313228666596841,2.02417640888751,
8.37940943298678));
#46714=CARTESIAN_POINT('Ctrl Pts',(-0.313343307958032,2.0246515700166,8.37937935429695));
#46715=CARTESIAN_POINT('Ctrl Pts',(-0.3135784583592,2.02563603032065,8.37931699724269));
#46716=CARTESIAN_POINT('Ctrl Pts',(-0.313698808584223,2.02614536560879,
8.37928471385741));
#46717=CARTESIAN_POINT('Ctrl Pts',(-0.314008906526423,2.02747216738436,
8.37920055996129));
#46718=CARTESIAN_POINT('Ctrl Pts',(-0.314196701951677,2.02829008197489,
8.37914862680255));
#46719=CARTESIAN_POINT('Ctrl Pts',(-0.319650775055618,2.05247723809825,
8.37761117391605));
#46720=CARTESIAN_POINT('Ctrl Pts',(-0.322297014532377,2.07635434457231,
8.37603790742453));
#46721=CARTESIAN_POINT('Ctrl Pts',(-0.322274862071682,2.10029816384487,
8.37442397213274));
#46722=CARTESIAN_POINT('',(-0.322758995413397,2.09993443928603,8.24935848523156));
#46723=CARTESIAN_POINT('Ctrl Pts',(-0.322791832858883,2.09993556662301,
8.24937734492731));
#46724=CARTESIAN_POINT('Ctrl Pts',(-0.322801292110665,2.09647160517377,
8.24959213483258));
#46725=CARTESIAN_POINT('Ctrl Pts',(-0.321180065660157,1.98619899400209,
8.25643037257877));
#46726=CARTESIAN_POINT('Ctrl Pts',(-0.195796246402531,1.77307658662262,
8.2698920581659));
#46727=CARTESIAN_POINT('Ctrl Pts',(0.168895013338677,1.75840145962115,8.2897624016887));
#46728=CARTESIAN_POINT('Ctrl Pts',(0.378648091321469,2.05709648897531,8.30963274521149));
#46729=CARTESIAN_POINT('Ctrl Pts',(0.24104309379967,2.39514964890902,8.32950308873427));
#46730=CARTESIAN_POINT('Ctrl Pts',(-0.117686127229278,2.46244318696509,
8.34937343225707));
#46731=CARTESIAN_POINT('Ctrl Pts',(-0.306460346708295,2.26280590555498,
8.36433150221144));
#46732=CARTESIAN_POINT('Ctrl Pts',(-0.322442531075311,2.12802537045353,
8.37266612432489));
#46733=CARTESIAN_POINT('Ctrl Pts',(-0.322193764531691,2.10029569746695,
8.37437729859741));
#46734=CARTESIAN_POINT('',(-0.322274935754178,2.10020349358851,7.99961864007736));
#46735=CARTESIAN_POINT('Ctrl Pts',(-0.32227498952282,2.09991782295878,8.24908050368635));
#46736=CARTESIAN_POINT('Ctrl Pts',(-0.322282430347236,2.12909862059907,
8.24731739895166));
#46737=CARTESIAN_POINT('Ctrl Pts',(-0.318326636673908,2.15815172661552,
8.24574482695574));
#46738=CARTESIAN_POINT('Ctrl Pts',(-0.306877789527729,2.19935460858732,
8.24333071811698));
#46739=CARTESIAN_POINT('Ctrl Pts',(-0.302423067387966,2.2121853311125,8.24255263359147));
#46740=CARTESIAN_POINT('Ctrl Pts',(-0.294911155652155,2.23008754209254,
8.2414018613405));
#46741=CARTESIAN_POINT('Ctrl Pts',(-0.292502791452486,2.23541590989614,
8.24105080179699));
#46742=CARTESIAN_POINT('Ctrl Pts',(-0.289546968746822,2.24150825083486,
8.24063833070744));
#46743=CARTESIAN_POINT('Ctrl Pts',(-0.289139401550848,2.24233916751049,
8.24058183290494));
#46744=CARTESIAN_POINT('Ctrl Pts',(-0.288514333431861,2.24359974558511,
8.24049574742057));
#46745=CARTESIAN_POINT('Ctrl Pts',(-0.288299436856062,2.24403069892286,
8.24046625083573));
#46746=CARTESIAN_POINT('Ctrl Pts',(-0.287925047383808,2.244777304119,8.24041503323732));
#46747=CARTESIAN_POINT('Ctrl Pts',(-0.287765998899282,2.24509317893973,
8.240393327835));
#46748=CARTESIAN_POINT('Ctrl Pts',(-0.287434350113652,2.24574915251239,
8.24034817691505));
#46749=CARTESIAN_POINT('Ctrl Pts',(-0.287261665464136,2.24608920780181,
8.24032472845817));
#46750=CARTESIAN_POINT('Ctrl Pts',(-0.286839322200057,2.2469172533412,8.24026752707046));
#46751=CARTESIAN_POINT('Ctrl Pts',(-0.286589022089496,2.24740491342343,
8.24023375158812));
#46752=CARTESIAN_POINT('Ctrl Pts',(-0.285636487836732,2.2492491402012,8.24010568470052));
#46753=CARTESIAN_POINT('Ctrl Pts',(-0.284925864602599,2.2506013299609,8.24001109740566));
#46754=CARTESIAN_POINT('Ctrl Pts',(-0.283921320898047,2.25248023763483,
8.23987868891264));
#46755=CARTESIAN_POINT('Ctrl Pts',(-0.28363548624749,2.25301127495336,8.23984115664337));
#46756=CARTESIAN_POINT('Ctrl Pts',(-0.266787156679002,2.28410347563907,
8.23763718284402));
#46757=CARTESIAN_POINT('Ctrl Pts',(-0.245393290271939,2.31177894559571,
8.23527113764941));
#46758=CARTESIAN_POINT('Ctrl Pts',(-0.213954374122118,2.34114993382704,
8.23237726724694));
#46759=CARTESIAN_POINT('Ctrl Pts',(-0.207686493921321,2.34656865521063,
8.23182484419027));
#46760=CARTESIAN_POINT('Ctrl Pts',(-0.197755079015446,2.35450685665233,
8.23099389648358));
#46761=CARTESIAN_POINT('Ctrl Pts',(-0.194236806860526,2.35720201897057,
8.23070755889719));
#46762=CARTESIAN_POINT('Ctrl Pts',(-0.189466740624686,2.36070238721776,
8.23033109808522));
#46763=CARTESIAN_POINT('Ctrl Pts',(-0.188263517250055,2.36157260707121,
8.23023711172103));
#46764=CARTESIAN_POINT('Ctrl Pts',(-0.186510893398122,2.36282181715218,
8.23010166601934));
#46765=CARTESIAN_POINT('Ctrl Pts',(-0.185966283356383,2.36320745126316,
8.23005977944542));
#46766=CARTESIAN_POINT('Ctrl Pts',(-0.185115629236839,2.3638058345674,8.22999467353943));
#46767=CARTESIAN_POINT('Ctrl Pts',(-0.184810411062298,2.36401974643168,
8.22997137695607));
#46768=CARTESIAN_POINT('Ctrl Pts',(-0.184298652055851,2.36437708997849,
8.22993242306291));
#46769=CARTESIAN_POINT('Ctrl Pts',(-0.184092314192659,2.36452080959975,
8.22991674628231));
#46770=CARTESIAN_POINT('Ctrl Pts',(-0.183689281966663,2.36480083191344,
8.229886182628));
#46771=CARTESIAN_POINT('Ctrl Pts',(-0.183492603645741,2.36493715726504,
8.22987129420697));
#46772=CARTESIAN_POINT('Ctrl Pts',(-0.183119949541493,2.36519484421937,
8.22984313501947));
#46773=CARTESIAN_POINT('Ctrl Pts',(-0.182944006291985,2.36531624881019,
8.22982986136353));
#46774=CARTESIAN_POINT('Ctrl Pts',(-0.182537022179148,2.36559647919987,
8.22979920632851));
#46775=CARTESIAN_POINT('Ctrl Pts',(-0.182305895074204,2.36575517841054,
8.22978183368115));
#46776=CARTESIAN_POINT('Ctrl Pts',(-0.181599608315366,2.3662387823416,8.22972885579778));
#46777=CARTESIAN_POINT('Ctrl Pts',(-0.181123781750677,2.36656271805986,
8.22969331637367));
#46778=CARTESIAN_POINT('Ctrl Pts',(-0.177661502568308,2.36890623587703,
8.22943580027706));
#46779=CARTESIAN_POINT('Ctrl Pts',(-0.174642067099587,2.37087695404254,
8.22921704965939));
#46780=CARTESIAN_POINT('Ctrl Pts',(-0.170435880374202,2.37352265983096,
8.22891933706323));
#46781=CARTESIAN_POINT('Ctrl Pts',(-0.169277100534252,2.37424131365929,
8.22883803919112));
#46782=CARTESIAN_POINT('Ctrl Pts',(-0.156516338341294,2.38204360353047,
8.22795023944417));
#46783=CARTESIAN_POINT('Ctrl Pts',(-0.144480681022667,2.38839445779987,
8.22717997714227));
#46784=CARTESIAN_POINT('Ctrl Pts',(-0.120292574008706,2.39926214379793,
8.22569196139057));
#46785=CARTESIAN_POINT('Ctrl Pts',(-0.108198631363857,2.40384401985012,
8.22497475516177));
#46786=CARTESIAN_POINT('Ctrl Pts',(-0.0828192209699291,2.41175116422438,
8.22347450226434));
#46787=CARTESIAN_POINT('Ctrl Pts',(-0.0695321839170615,2.41498100032869,
8.22269142277447));
#46788=CARTESIAN_POINT('Ctrl Pts',(-0.0503041495783892,2.41837883784802,
8.22153414787132));
#46789=CARTESIAN_POINT('Ctrl Pts',(-0.0445006331968898,2.41924172464982,
8.22118191122227));
#46790=CARTESIAN_POINT('Ctrl Pts',(-0.0377574753976918,2.42005688039645,
8.2207681801342));
#46791=CARTESIAN_POINT('Ctrl Pts',(-0.036837413269538,2.42016408073518,
8.22071163403207));
#46792=CARTESIAN_POINT('Ctrl Pts',(-0.0354381805681159,2.42032100000866,
8.22062548989499));
#46793=CARTESIAN_POINT('Ctrl Pts',(-0.0349593341849089,2.42037361414115,
8.22059598314825));
#46794=CARTESIAN_POINT('Ctrl Pts',(-0.0341287258698034,2.42046299440585,
8.22054475417693));
#46795=CARTESIAN_POINT('Ctrl Pts',(-0.0337770171093503,2.42050025557971,
8.22052304758494));
#46796=CARTESIAN_POINT('Ctrl Pts',(-0.033045992419723,2.42057648605206,
8.2204779002501));
#46797=CARTESIAN_POINT('Ctrl Pts',(-0.032666667409429,2.42061536123977,
8.22045445657863));
#46798=CARTESIAN_POINT('Ctrl Pts',(-0.0317421644739875,2.42070845136719,
8.2203972772143));
#46799=CARTESIAN_POINT('Ctrl Pts',(-0.0311969170151554,2.42076194934353,
8.22036351900591));
#46800=CARTESIAN_POINT('Ctrl Pts',(-0.0291327553487398,2.42095916554851,
8.22023558393343));
#46801=CARTESIAN_POINT('Ctrl Pts',(-0.0276129823642547,2.42109348554627,
8.22014111195705));
#46802=CARTESIAN_POINT('Ctrl Pts',(-0.0254893632654973,2.42126598630649,
8.22000870341162));
#46803=CARTESIAN_POINT('Ctrl Pts',(-0.0248862595631177,2.42131326719275,
8.21997105461301));
#46804=CARTESIAN_POINT('Ctrl Pts',(0.0112130011942717,2.42404105707372,
8.2177148314453));
#46805=CARTESIAN_POINT('Ctrl Pts',(0.0469020093077426,2.42082262785708,
8.21528545039867));
#46806=CARTESIAN_POINT('Ctrl Pts',(0.088677716470874,2.40992761333734,8.21238663493858));
#46807=CARTESIAN_POINT('Ctrl Pts',(0.0959575043947503,2.40775157817024,
8.21188109144788));
#46808=CARTESIAN_POINT('Ctrl Pts',(0.107255482601194,2.40393449878442,8.21110226414418));
#46809=CARTESIAN_POINT('Ctrl Pts',(0.111328869481974,2.40246620471191,8.21082268367161));
#46810=CARTESIAN_POINT('Ctrl Pts',(0.11673492184586,2.4003935175192,8.21045440107374));
#46811=CARTESIAN_POINT('Ctrl Pts',(0.118094660862702,2.39986156573622,8.21036200751817));
#46812=CARTESIAN_POINT('Ctrl Pts',(0.120062896011062,2.39907609567392,8.21022866115198));
#46813=CARTESIAN_POINT('Ctrl Pts',(0.120674280771127,2.39882993153351,8.2101872958129));
#46814=CARTESIAN_POINT('Ctrl Pts',(0.121627187826496,2.39844285766162,8.2101229151703));
#46815=CARTESIAN_POINT('Ctrl Pts',(0.12196922604661,2.39830323499525,8.2100998247213));
#46816=CARTESIAN_POINT('Ctrl Pts',(0.122542406888266,2.3980681074612,8.21006116210491));
#46817=CARTESIAN_POINT('Ctrl Pts',(0.122773678705264,2.39797292157115,8.210045570911));
#46818=CARTESIAN_POINT('Ctrl Pts',(0.123225130344947,2.39778650016235,8.21001515366888));
#46819=CARTESIAN_POINT('Ctrl Pts',(0.123445320152582,2.3976952894501,8.21000032613019));
#46820=CARTESIAN_POINT('Ctrl Pts',(0.123863081242261,2.39752169425319,8.20997220981573));
#46821=CARTESIAN_POINT('Ctrl Pts',(0.124060670004641,2.39743935786033,8.2099589183064));
#46822=CARTESIAN_POINT('Ctrl Pts',(0.124518514364245,2.39724803584759,8.20992813506939));
#46823=CARTESIAN_POINT('Ctrl Pts',(0.124778708661678,2.39713890539765,8.20991065230337));
#46824=CARTESIAN_POINT('Ctrl Pts',(0.125577592158592,2.39680260403766,8.20985700853089));
#46825=CARTESIAN_POINT('Ctrl Pts',(0.126115810589976,2.39657430729546,8.20982091578144));
#46826=CARTESIAN_POINT('Ctrl Pts',(0.130144483554119,2.39485251023115,8.20955109117706));
#46827=CARTESIAN_POINT('Ctrl Pts',(0.133609106145702,2.3932988223843,8.20932094199588));
#46828=CARTESIAN_POINT('Ctrl Pts',(0.152805736639994,2.38427942851842,8.20805202978477));
#46829=CARTESIAN_POINT('Ctrl Pts',(0.167941785555306,2.3756085821367,8.20707444435108));
#46830=CARTESIAN_POINT('Ctrl Pts',(0.198114992574998,2.35491024004541,8.20502765545664));
#46831=CARTESIAN_POINT('Ctrl Pts',(0.212925057153106,2.34267599840696,8.2039619848802));
#46832=CARTESIAN_POINT('Ctrl Pts',(0.232599103675081,2.32322846842001,8.20235533616569));
#46833=CARTESIAN_POINT('Ctrl Pts',(0.238399853019653,2.31702254170269,8.2018538756302));
#46834=CARTESIAN_POINT('Ctrl Pts',(0.245589460343964,2.30869427151331,8.20119044116371));
#46835=CARTESIAN_POINT('Ctrl Pts',(0.247208159684032,2.30677429054296,8.20103812544327));
#46836=CARTESIAN_POINT('Ctrl Pts',(0.249257867814535,2.30428460632014,8.20084133573812));
#46837=CARTESIAN_POINT('Ctrl Pts',(0.249709679740041,2.30373208112137,8.20079770805883));
#46838=CARTESIAN_POINT('Ctrl Pts',(0.250434072073226,2.30284018497108,8.20072735375276));
#46839=CARTESIAN_POINT('Ctrl Pts',(0.250707808612591,2.30250175256527,8.20070067381655));
#46840=CARTESIAN_POINT('Ctrl Pts',(0.251227438767591,2.30185664257161,8.20064984755564));
#46841=CARTESIAN_POINT('Ctrl Pts',(0.251473458767252,2.30155006741121,8.20062570637293));
#46842=CARTESIAN_POINT('Ctrl Pts',(0.252032491148034,2.3008508182728,8.20057067318188));
#46843=CARTESIAN_POINT('Ctrl Pts',(0.252345147304278,2.30045786196248,8.2005397669895));
#46844=CARTESIAN_POINT('Ctrl Pts',(0.253272695351611,2.29928648085921,8.20044769783543));
#46845=CARTESIAN_POINT('Ctrl Pts',(0.253884908760411,2.29850595137779,8.20038642833549));
#46846=CARTESIAN_POINT('Ctrl Pts',(0.25812838953016,2.29304406585205,8.19995821605619));
#46847=CARTESIAN_POINT('Ctrl Pts',(0.261633359894596,2.28826644499301,8.19958632657241));
#46848=CARTESIAN_POINT('Ctrl Pts',(0.266128018919764,2.28177170073543,8.19908381024595));
#46849=CARTESIAN_POINT('Ctrl Pts',(0.267236582505666,2.28013795363976,8.1989576538504));
#46850=CARTESIAN_POINT('Ctrl Pts',(0.270249866876016,2.2756080868366,8.19860854117602));
#46851=CARTESIAN_POINT('Ctrl Pts',(0.272122942380612,2.27269132444765,8.19838450162629));
#46852=CARTESIAN_POINT('Ctrl Pts',(0.289230961540432,2.2450809847847,8.19627088781002));
#46853=CARTESIAN_POINT('Ctrl Pts',(0.301111610925658,2.21846690481955,8.19426949047631));
#46854=CARTESIAN_POINT('Ctrl Pts',(0.311923591539632,2.18157173735003,8.19171311728566));
#46855=CARTESIAN_POINT('Ctrl Pts',(0.314179134753239,2.17240016469395,8.19109592334484));
#46856=CARTESIAN_POINT('Ctrl Pts',(0.316211087159561,2.16223012552566,8.19044070508896));
#46857=CARTESIAN_POINT('Ctrl Pts',(0.316389315880017,2.16131754244665,8.19038216683029));
#46858=CARTESIAN_POINT('Ctrl Pts',(0.316652326023318,2.15993917052633,8.19029414957183));
#46859=CARTESIAN_POINT('Ctrl Pts',(0.316740032926459,2.15947395470129,8.19026451130572));
#46860=CARTESIAN_POINT('Ctrl Pts',(0.316880476768539,2.15871988828576,8.19021658363558));
#46861=CARTESIAN_POINT('Ctrl Pts',(0.316933844216575,2.15843115803301,8.19019825903072));
#46862=CARTESIAN_POINT('Ctrl Pts',(0.31703540988877,2.15787743123977,8.19016316798674));
#46863=CARTESIAN_POINT('Ctrl Pts',(0.317083670608547,2.15761244661475,8.190146398014));
#46864=CARTESIAN_POINT('Ctrl Pts',(0.317169668282853,2.15713687876541,8.19011634216466));
#46865=CARTESIAN_POINT('Ctrl Pts',(0.317207527694683,2.15692631876811,8.19010304929872));
#46866=CARTESIAN_POINT('Ctrl Pts',(0.317288784254605,2.15647180188791,8.19007438657624));
#46867=CARTESIAN_POINT('Ctrl Pts',(0.317332109607858,2.15622783327722,8.19005902089588));
#46868=CARTESIAN_POINT('Ctrl Pts',(0.31744850067743,2.1555680062489,8.19001751554603));
#46869=CARTESIAN_POINT('Ctrl Pts',(0.317521030905066,2.1551520519893,8.18999140645455));
#46870=CARTESIAN_POINT('Ctrl Pts',(0.317840945335316,2.15329582230688,8.18987513669094));
#46871=CARTESIAN_POINT('Ctrl Pts',(0.318079353906188,2.15185398746005,8.18978547906446));
#46872=CARTESIAN_POINT('Ctrl Pts',(0.32260526546391,2.12327596818615,8.1880204851893));
#46873=CARTESIAN_POINT('Ctrl Pts',(0.323416104845217,2.09569820721821,8.18652600070428));
#46874=CARTESIAN_POINT('Ctrl Pts',(0.318553053376049,2.04642250939486,8.1837467977001));
#46875=CARTESIAN_POINT('Ctrl Pts',(0.314147029591894,2.02478020232096,8.18248670981023));
#46876=CARTESIAN_POINT('Ctrl Pts',(0.307226595764991,2.00266393809037,8.18107747313594));
#46877=CARTESIAN_POINT('Ctrl Pts',(0.306878379555554,2.00157159860289,8.18100756323167));
#46878=CARTESIAN_POINT('Ctrl Pts',(0.306362069825668,1.99998133199268,8.18090533009312));
#46879=CARTESIAN_POINT('Ctrl Pts',(0.306198572630702,1.9994819126148,8.18087315825076));
#46880=CARTESIAN_POINT('Ctrl Pts',(0.305909624303154,1.99860653637977,8.18081665151407));
#46881=CARTESIAN_POINT('Ctrl Pts',(0.305784699456504,1.99823040590516,8.1807923340269));
#46882=CARTESIAN_POINT('Ctrl Pts',(0.305540882254735,1.99750080990798,8.18074509068159));
#46883=CARTESIAN_POINT('Ctrl Pts',(0.305422069525533,1.99714731824864,8.18072216748626));
#46884=CARTESIAN_POINT('Ctrl Pts',(0.305137095528242,1.99630431160062,8.18066741957006));
#46885=CARTESIAN_POINT('Ctrl Pts',(0.304970369868646,1.99581498976703,8.18063557620863));
#46886=CARTESIAN_POINT('Ctrl Pts',(0.304463108990381,1.99433788488598,8.18053925353634));
#46887=CARTESIAN_POINT('Ctrl Pts',(0.304118949211372,1.99335136195992,8.18047465418788));
#46888=CARTESIAN_POINT('Ctrl Pts',(0.300444621649078,1.98298144091922,8.17979275631169));
#46889=CARTESIAN_POINT('Ctrl Pts',(0.296686435758453,1.97375643593979,8.17916120911585));
#46890=CARTESIAN_POINT('Ctrl Pts',(0.291548250891119,1.9626463792024,8.17836830118015));
#46891=CARTESIAN_POINT('Ctrl Pts',(0.290566802905679,1.96058216610798,8.17821958031863));
#46892=CARTESIAN_POINT('Ctrl Pts',(0.277211063063621,1.9332456522401,8.17623148089844));
#46893=CARTESIAN_POINT('Ctrl Pts',(0.261600538370055,1.90969027660268,8.17429055103117));
#46894=CARTESIAN_POINT('Ctrl Pts',(0.237084450394834,1.88151177172715,8.171809207549));
#46895=CARTESIAN_POINT('Ctrl Pts',(0.230737899374581,1.8748196292276,8.17120703853088));
#46896=CARTESIAN_POINT('Ctrl Pts',(0.223453371006296,1.86777035515342,8.17056672611689));
#46897=CARTESIAN_POINT('Ctrl Pts',(0.222791496618811,1.86713530529249,8.17050898658756));
#46898=CARTESIAN_POINT('Ctrl Pts',(0.221787294950725,1.86618000269019,8.1704220576152));
#46899=CARTESIAN_POINT('Ctrl Pts',(0.221446972184405,1.86585766324651,8.17039271348946));
#46900=CARTESIAN_POINT('Ctrl Pts',(0.220893746145429,1.8653359558628,8.1703452015258));
#46901=CARTESIAN_POINT('Ctrl Pts',(0.220681274887295,1.86513613387177,8.17032699930655));
#46902=CARTESIAN_POINT('Ctrl Pts',(0.220273084224832,1.86475328738924,8.17029211704908));
#46903=CARTESIAN_POINT('Ctrl Pts',(0.22007740739198,1.86457021814357,8.17027543357961));
#46904=CARTESIAN_POINT('Ctrl Pts',(0.219725106838865,1.86424143958026,8.17024546540707));
#46905=CARTESIAN_POINT('Ctrl Pts',(0.219568566644015,1.86409564241125,8.17023217391268));
#46906=CARTESIAN_POINT('Ctrl Pts',(0.219229658710669,1.86378062259873,8.17020345092515));
#46907=CARTESIAN_POINT('Ctrl Pts',(0.219047240663644,1.8636114556987,8.17018802374208));
#46908=CARTESIAN_POINT('Ctrl Pts',(0.218551413995459,1.86315271345567,8.17014618044394));
#46909=CARTESIAN_POINT('Ctrl Pts',(0.218237624455327,1.86286354776227,8.17011979576643));
#46910=CARTESIAN_POINT('Ctrl Pts',(0.216816627321655,1.86155926922216,8.17000074224138));
#46911=CARTESIAN_POINT('Ctrl Pts',(0.215702882059124,1.86055126048716,8.16990860632842));
#46912=CARTESIAN_POINT('Ctrl Pts',(0.190642664679395,1.83818695302956,8.16786049859883));
#46913=CARTESIAN_POINT('Ctrl Pts',(0.163642520815101,1.82051361250132,8.16614774592186));
#46914=CARTESIAN_POINT('Ctrl Pts',(0.120255612203987,1.80059316440985,8.16344111173404));
#46915=CARTESIAN_POINT('Ctrl Pts',(0.105585315746141,1.79511065825562,8.16253527455687));
#46916=CARTESIAN_POINT('Ctrl Pts',(0.0882067855719214,1.79002123579892,
8.16144308098317));
#46917=CARTESIAN_POINT('Ctrl Pts',(0.0858295223003822,1.78935460110477,
8.1612933100735));
#46918=CARTESIAN_POINT('Ctrl Pts',(0.0827596812450026,1.78853168054126,
8.16109935925991));
#46919=CARTESIAN_POINT('Ctrl Pts',(0.0820738781155888,1.78835026490526,
8.16105599573748));
#46920=CARTESIAN_POINT('Ctrl Pts',(0.0809672549164702,1.78806143572786,
8.16098596549095));
#46921=CARTESIAN_POINT('Ctrl Pts',(0.0805468043056365,1.78795260526308,
8.16095934467981));
#46922=CARTESIAN_POINT('Ctrl Pts',(0.0797451844850896,1.78774684010737,
8.16090856392216));
#46923=CARTESIAN_POINT('Ctrl Pts',(0.0793640550229795,1.78764975255392,
8.16088440896934));
#46924=CARTESIAN_POINT('Ctrl Pts',(0.0784941550613436,1.78742985231104,
8.1608292508983));
#46925=CARTESIAN_POINT('Ctrl Pts',(0.0780052731810009,1.78730748816697,
8.16079823335736));
#46926=CARTESIAN_POINT('Ctrl Pts',(0.076511424768566,1.78693730839166,8.16070339620407));
#46927=CARTESIAN_POINT('Ctrl Pts',(0.0755055569837382,1.78669318899565,
8.16063945760279));
#46928=CARTESIAN_POINT('Ctrl Pts',(0.0681265068171763,1.78493992687024,
8.16016978888479));
#46929=CARTESIAN_POINT('Ctrl Pts',(0.0617102148068972,1.78362062353308,
8.15975799494796));
#46930=CARTESIAN_POINT('Ctrl Pts',(0.0534642928833599,1.78218549140897,
8.15922390417348));
#46931=CARTESIAN_POINT('Ctrl Pts',(0.0516674542015662,1.78188843710115,
8.1591072326862));
#46932=CARTESIAN_POINT('Ctrl Pts',(0.0477904624977187,1.78128120496461,
8.15885486773092));
#46933=CARTESIAN_POINT('Ctrl Pts',(0.0457096048281793,1.78097612890661,
8.15871903149516));
#46934=CARTESIAN_POINT('Ctrl Pts',(0.0411466172690072,1.78035270479501,
8.1584203269715));
#46935=CARTESIAN_POINT('Ctrl Pts',(0.0386634778724025,1.78004285845777,
8.15825723348964));
#46936=CARTESIAN_POINT('Ctrl Pts',(0.0111390565423589,1.77693344692627,
8.15644364292251));
#46937=CARTESIAN_POINT('Ctrl Pts',(-0.0141430083672298,1.77705140828866,
8.15471514715824));
#46938=CARTESIAN_POINT('Ctrl Pts',(-0.0479516692891071,1.78118897656373,
8.15243536489083));
#46939=CARTESIAN_POINT('Ctrl Pts',(-0.0567073223628983,1.78262933894312,
8.15184895715194));
#46940=CARTESIAN_POINT('Ctrl Pts',(-0.069184241786332,1.78521482453982,
8.1510287848672));
#46941=CARTESIAN_POINT('Ctrl Pts',(-0.0729611889849623,1.78606874282712,
8.15078258998365));
#46942=CARTESIAN_POINT('Ctrl Pts',(-0.0772453047936734,1.78711882642643,
8.1505064251594));
#46943=CARTESIAN_POINT('Ctrl Pts',(-0.0777682591425823,1.7872483992537,
8.15047276697869));
#46944=CARTESIAN_POINT('Ctrl Pts',(-0.0785556144877188,1.78744557988833,
8.15042217364282));
#46945=CARTESIAN_POINT('Ctrl Pts',(-0.0788202552489524,1.7875122122983,
8.15040518253307));
#46946=CARTESIAN_POINT('Ctrl Pts',(-0.0792964180697469,1.78763274603034,
8.15037463636519));
#46947=CARTESIAN_POINT('Ctrl Pts',(-0.079507969536768,1.78768652598338,
8.15036107431972));
#46948=CARTESIAN_POINT('Ctrl Pts',(-0.0799624435325836,1.78780255264627,
8.15033195878021));
#46949=CARTESIAN_POINT('Ctrl Pts',(-0.0802053473558922,1.7878648677793,
8.15031640936243));
#46950=CARTESIAN_POINT('Ctrl Pts',(-0.0808592968577339,1.78803344732757,
8.15027457878565));
#46951=CARTESIAN_POINT('Ctrl Pts',(-0.0812702074912553,1.78814024104756,
8.15024832831689));
#46952=CARTESIAN_POINT('Ctrl Pts',(-0.0831599327597951,1.78863536024943,
8.15012775662798));
#46953=CARTESIAN_POINT('Ctrl Pts',(-0.0846362147561983,1.78903340264228,
8.15003398958839));
#46954=CARTESIAN_POINT('Ctrl Pts',(-0.114063074932086,1.79719270285057,
8.1481724075239));
#46955=CARTESIAN_POINT('Ctrl Pts',(-0.140847299161554,1.80868348236693,
8.14660467575085));
#46956=CARTESIAN_POINT('Ctrl Pts',(-0.182698745868446,1.83377905825848,
8.14385781834547));
#46957=CARTESIAN_POINT('Ctrl Pts',(-0.198687528647069,1.84548965676049,
8.14272136036028));
#46958=CARTESIAN_POINT('Ctrl Pts',(-0.214697610556417,1.85964887455668,
8.14142555104108));
#46959=CARTESIAN_POINT('Ctrl Pts',(-0.215886326524282,1.86071602360955,
8.14132833572421));
#46960=CARTESIAN_POINT('Ctrl Pts',(-0.2175113569342,1.86219683229,8.14119402579213));
#46961=CARTESIAN_POINT('Ctrl Pts',(-0.217954534668935,1.86260295330861,
8.14115725058547));
#46962=CARTESIAN_POINT('Ctrl Pts',(-0.218698488379157,1.86328853983879,
8.14109526876992));
#46963=CARTESIAN_POINT('Ctrl Pts',(-0.218999872467176,1.86356734563968,
8.14107009031381));
#46964=CARTESIAN_POINT('Ctrl Pts',(-0.219593472460228,1.86411858469106,
8.14102036267368));
#46965=CARTESIAN_POINT('Ctrl Pts',(-0.219885716236577,1.8643909869548,8.14099581484031));
#46966=CARTESIAN_POINT('Ctrl Pts',(-0.220526685983122,1.86499067014821,
8.1409418297588));
#46967=CARTESIAN_POINT('Ctrl Pts',(-0.220875191016659,1.86531818490239,
8.14091238248336));
#46968=CARTESIAN_POINT('Ctrl Pts',(-0.222079647546895,1.86645515709603,
8.14081028074599));
#46969=CARTESIAN_POINT('Ctrl Pts',(-0.222931880897983,1.86726852399858,
8.14073745751257));
#46970=CARTESIAN_POINT('Ctrl Pts',(-0.231382057801173,1.8754223301856,8.14000954127762));
#46971=CARTESIAN_POINT('Ctrl Pts',(-0.238618366913309,1.88312672024413,
8.13933841667321));
#46972=CARTESIAN_POINT('Ctrl Pts',(-0.246920442604891,1.89288522183672,
8.13850641880879));
#46973=CARTESIAN_POINT('Ctrl Pts',(-0.248360132130102,1.89461382539915,
8.13835970132909));
#46974=CARTESIAN_POINT('Ctrl Pts',(-0.257873263555637,1.90628232789558,
8.13737380049157));
#46975=CARTESIAN_POINT('Ctrl Pts',(-0.26536557026227,1.91668000027914,8.13651610213014));
#46976=CARTESIAN_POINT('Ctrl Pts',(-0.280651432665216,1.94080162503451,
8.13458739023784));
#46977=CARTESIAN_POINT('Ctrl Pts',(-0.288097051504079,1.9547090214577,8.13351493207316));
#46978=CARTESIAN_POINT('Ctrl Pts',(-0.297080486811537,1.97492060331028,
8.13205134394475));
#46979=CARTESIAN_POINT('Ctrl Pts',(-0.299492499852902,1.98081138886207,
8.13163562131806));
#46980=CARTESIAN_POINT('Ctrl Pts',(-0.30278123411088,1.98957502409179,8.13103672867207));
#46981=CARTESIAN_POINT('Ctrl Pts',(-0.303794713668879,1.99239458859537,
8.13084696337125));
#46982=CARTESIAN_POINT('Ctrl Pts',(-0.304933047195492,1.99570585974084,
8.1306278368916));
#46983=CARTESIAN_POINT('Ctrl Pts',(-0.305096201675618,1.996184111545,8.13059627854352));
#46984=CARTESIAN_POINT('Ctrl Pts',(-0.305343496255879,1.99691461971689,
8.13054821462114));
#46985=CARTESIAN_POINT('Ctrl Pts',(-0.305428449167943,1.99716659699316,
8.13053166111657));
#46986=CARTESIAN_POINT('Ctrl Pts',(-0.305575708059959,1.99760517118283,
8.13050289374372));
#46987=CARTESIAN_POINT('Ctrl Pts',(-0.305638154884436,1.99779171949217,
8.13049067150456));
#46988=CARTESIAN_POINT('Ctrl Pts',(-0.30577903712467,1.99821386274984,8.1304630453328));
#46989=CARTESIAN_POINT('Ctrl Pts',(-0.305857370930534,1.99844949074644,
8.13044764751152));
#46990=CARTESIAN_POINT('Ctrl Pts',(-0.306068905305321,1.99908825099524,
8.13040596560416));
#46991=CARTESIAN_POINT('Ctrl Pts',(-0.306201582284039,1.9994915580976,8.13037971254391));
#46992=CARTESIAN_POINT('Ctrl Pts',(-0.306793966947754,2.00130432947855,
8.13026199573931));
#46993=CARTESIAN_POINT('Ctrl Pts',(-0.307244752071184,2.00271672261873,
8.13017105046223));
#46994=CARTESIAN_POINT('Ctrl Pts',(-0.317329448824932,2.03508335760211,
8.12810347486102));
#46995=CARTESIAN_POINT('Ctrl Pts',(-0.3222497397889,2.06731825056121,8.12637519961379));
#46996=CARTESIAN_POINT('Ctrl Pts',(-0.322280798131405,2.10734791894266,
8.12410385700108));
#46997=CARTESIAN_POINT('Ctrl Pts',(-0.32201799756462,2.11494336341435,8.12366825587914));
#46998=CARTESIAN_POINT('Ctrl Pts',(-0.320825442818891,2.13196623469806,
8.12267392177088));
#46999=CARTESIAN_POINT('Ctrl Pts',(-0.319748057848399,2.14137581189172,
8.1221116942627));
#47000=CARTESIAN_POINT('Ctrl Pts',(-0.31807781083264,2.15185552477025,8.12146635855013));
#47001=CARTESIAN_POINT('Ctrl Pts',(-0.317891387048666,2.15298636787354,
8.12139647245469));
#47002=CARTESIAN_POINT('Ctrl Pts',(-0.317611661640599,2.15462854703028,
8.12129461521317));
#47003=CARTESIAN_POINT('Ctrl Pts',(-0.317523147365805,2.15514069860507,
8.12126279620024));
#47004=CARTESIAN_POINT('Ctrl Pts',(-0.317364862083589,2.15604353164617,
8.12120661147408));
#47005=CARTESIAN_POINT('Ctrl Pts',(-0.317295607453776,2.15643430351316,
8.1211822622291));
#47006=CARTESIAN_POINT('Ctrl Pts',(-0.317151045270002,2.15724132285942,
8.12113191207952));
#47007=CARTESIAN_POINT('Ctrl Pts',(-0.31707563967692,2.15765755179774,8.12110590809674));
#47008=CARTESIAN_POINT('Ctrl Pts',(-0.316880722912232,2.15872152008999,
8.12103934545384));
#47009=CARTESIAN_POINT('Ctrl Pts',(-0.316760045440997,2.15936904140195,
8.12099874970265));
#47010=CARTESIAN_POINT('Ctrl Pts',(-0.316261108836302,2.16200136438478,
8.1208333638839));
#47011=CARTESIAN_POINT('Ctrl Pts',(-0.315866179305892,2.16398292443956,
8.12070804315914));
#47012=CARTESIAN_POINT('Ctrl Pts',(-0.309111904449023,2.19628484048246,
8.11865138185862));
#47013=CARTESIAN_POINT('Ctrl Pts',(-0.298432990079732,2.22552994818758,
8.11656678492813));
#47014=CARTESIAN_POINT('Ctrl Pts',(-0.276879239790065,2.26555725999323,
8.11349330499454));
#47015=CARTESIAN_POINT('Ctrl Pts',(-0.269152359661945,2.27784376478163,
8.11251890397409));
#47016=CARTESIAN_POINT('Ctrl Pts',(-0.258255636301397,2.29282481501028,
8.11132470603438));
#47017=CARTESIAN_POINT('Ctrl Pts',(-0.255826618415604,2.29603603745829,
8.11106839629576));
#47018=CARTESIAN_POINT('Ctrl Pts',(-0.252970312195753,2.29966860167403,
8.1107788697746));
#47019=CARTESIAN_POINT('Ctrl Pts',(-0.252601397837238,2.30013511228909,
8.11074169547676));
#47020=CARTESIAN_POINT('Ctrl Pts',(-0.252056219986532,2.30082060802589,
8.11068708639589));
#47021=CARTESIAN_POINT('Ctrl Pts',(-0.251880960726807,2.3010403846658,8.1106695805063));
#47022=CARTESIAN_POINT('Ctrl Pts',(-0.251568234624152,2.3014314950665,8.11063843191607));
#47023=CARTESIAN_POINT('Ctrl Pts',(-0.251430880106592,2.30160291765399,
8.11062478115732));
#47024=CARTESIAN_POINT('Ctrl Pts',(-0.251141269832963,2.3019636036843,8.11059606240507));
#47025=CARTESIAN_POINT('Ctrl Pts',(-0.25098897573914,2.30215283496606,8.1105809972924));
#47026=CARTESIAN_POINT('Ctrl Pts',(-0.250585068277143,2.30265354551364,
8.11054113931638));
#47027=CARTESIAN_POINT('Ctrl Pts',(-0.250333087098587,2.30296472959734,
8.11051637298542));
#47028=CARTESIAN_POINT('Ctrl Pts',(-0.249180686269022,2.30438247586825,
8.11040355597999));
#47029=CARTESIAN_POINT('Ctrl Pts',(-0.248273487131715,2.30548354341945,
8.11031598804553));
#47030=CARTESIAN_POINT('Ctrl Pts',(-0.241153547190104,2.31400902160593,
8.10963801765827));
#47031=CARTESIAN_POINT('Ctrl Pts',(-0.234615772718585,2.32115689801188,
8.10906991717256));
#47032=CARTESIAN_POINT('Ctrl Pts',(-0.207269627955935,2.34847487815264,
8.10684880373399));
#47033=CARTESIAN_POINT('Ctrl Pts',(-0.184106750047878,2.36609274299049,
8.10528716620653));
#47034=CARTESIAN_POINT('Ctrl Pts',(-0.156400346483884,2.38179489212323,
8.1034422622554));
#47035=CARTESIAN_POINT('Ctrl Pts',(-0.15388208827511,2.38317791555944,8.10327490524195));
#47036=CARTESIAN_POINT('Ctrl Pts',(-0.14978271746808,2.3853584541985,8.10300274058678));
#47037=CARTESIAN_POINT('Ctrl Pts',(-0.148212907339756,2.38617694485493,
8.10289858121165));
#47038=CARTESIAN_POINT('Ctrl Pts',(-0.140888862331924,2.38991923637497,
8.1024127566277));
#47039=CARTESIAN_POINT('Ctrl Pts',(-0.135054680980648,2.3926825232469,8.10202610871462));
#47040=CARTESIAN_POINT('Ctrl Pts',(-0.128197488708028,2.3956816560813,8.10157058417493));
#47041=CARTESIAN_POINT('Ctrl Pts',(-0.127251243822355,2.39609011932349,
8.1015077026631));
#47042=CARTESIAN_POINT('Ctrl Pts',(-0.125840226378234,2.39669119660459,
8.1014138963501));
#47043=CARTESIAN_POINT('Ctrl Pts',(-0.125376929382784,2.39688727539522,
8.10138308953611));
#47044=CARTESIAN_POINT('Ctrl Pts',(-0.124550719419933,2.39723466910647,
8.10132813910128));
#47045=CARTESIAN_POINT('Ctrl Pts',(-0.124187984284231,2.39738640652206,
8.1013040098868));
#47046=CARTESIAN_POINT('Ctrl Pts',(-0.123423565323021,2.39770453168053,
8.10125315165836));
#47047=CARTESIAN_POINT('Ctrl Pts',(-0.123021820937082,2.39787077102419,
8.10122641767172));
#47048=CARTESIAN_POINT('Ctrl Pts',(-0.121961747473028,2.39830691246371,
8.10115586102524));
#47049=CARTESIAN_POINT('Ctrl Pts',(-0.121302861555754,2.39857544714145,
8.10111199220174));
#47050=CARTESIAN_POINT('Ctrl Pts',(-0.118334655978815,2.39977371831736,
8.10091429826721));
#47051=CARTESIAN_POINT('Ctrl Pts',(-0.116015549370642,2.40067883986804,
8.10075964590625));
#47052=CARTESIAN_POINT('Ctrl Pts',(-0.0988405986406615,2.40715375402819,
8.0996126434107));
#47053=CARTESIAN_POINT('Ctrl Pts',(-0.0836042491240788,2.41164577220604,
8.09858429792765));
#47054=CARTESIAN_POINT('Ctrl Pts',(-0.0370331322954221,2.4217142444337,
8.09541622575253));
#47055=CARTESIAN_POINT('Ctrl Pts',(-0.00514434239926006,2.4237977694833,
8.09319868855161));
#47056=CARTESIAN_POINT('Ctrl Pts',(0.0280788392178759,2.42105320619793,
8.09108927986223));
#47057=CARTESIAN_POINT('Ctrl Pts',(0.0296240526461253,2.42091431590997,
8.09099167726233));
#47058=CARTESIAN_POINT('Ctrl Pts',(0.0315931487973007,2.42072298144491,
8.09086799789024));
#47059=CARTESIAN_POINT('Ctrl Pts',(0.0320179788368236,2.42068084899795,
8.09084135567073));
#47060=CARTESIAN_POINT('Ctrl Pts',(0.0326927681932383,2.42061257257573,
8.09079910505747));
#47061=CARTESIAN_POINT('Ctrl Pts',(0.0329427809252583,2.42058698035278,
8.09078346566574));
#47062=CARTESIAN_POINT('Ctrl Pts',(0.0334098262780731,2.4205386197544,8.09075427766141));
#47063=CARTESIAN_POINT('Ctrl Pts',(0.0336268640815612,2.42051592356457,
8.09074072511093));
#47064=CARTESIAN_POINT('Ctrl Pts',(0.0341145111030514,2.42046442831415,
8.09071029993471));
#47065=CARTESIAN_POINT('Ctrl Pts',(0.0343851063530482,2.42043550699777,
8.09069343434404));
#47066=CARTESIAN_POINT('Ctrl Pts',(0.0351876210774871,2.42034870568617,
8.09064346597799));
#47067=CARTESIAN_POINT('Ctrl Pts',(0.0357194367227065,2.42028984336355,
8.09061041852532));
#47068=CARTESIAN_POINT('Ctrl Pts',(0.0399869735877308,2.41980674338838,
8.09034574182049));
#47069=CARTESIAN_POINT('Ctrl Pts',(0.0437153515007418,2.41931846519247,
8.09011765108091));
#47070=CARTESIAN_POINT('Ctrl Pts',(0.0571660048219259,2.41731691139565,
8.08930342408048));
#47071=CARTESIAN_POINT('Ctrl Pts',(0.0668269705067426,2.41542378623534,
8.08873493636879));
#47072=CARTESIAN_POINT('Ctrl Pts',(0.107341452473838,2.4055392035933,8.08636450045496));
#47073=CARTESIAN_POINT('Ctrl Pts',(0.137003053535719,2.3934392911723,8.08464330611275));
#47074=CARTESIAN_POINT('Ctrl Pts',(0.169195079085567,2.37434499202061,8.0824229062492));
#47075=CARTESIAN_POINT('Ctrl Pts',(0.173907220737133,2.37138242802797,8.08208864757611));
#47076=CARTESIAN_POINT('Ctrl Pts',(0.179350251390957,2.36776035921035,8.08169058398228));
#47077=CARTESIAN_POINT('Ctrl Pts',(0.180157959174098,2.36721757493116,8.08163119825907));
#47078=CARTESIAN_POINT('Ctrl Pts',(0.181375364703121,2.36639144285402,8.08154120607925));
#47079=CARTESIAN_POINT('Ctrl Pts',(0.181786889240583,2.36611078640834,8.081510701536));
#47080=CARTESIAN_POINT('Ctrl Pts',(0.182521610584391,2.36560721270858,8.08145608840837));
#47081=CARTESIAN_POINT('Ctrl Pts',(0.182845054502296,2.36538465632932,8.08143199357174));
#47082=CARTESIAN_POINT('Ctrl Pts',(0.183520779633072,2.36491787937772,8.08138154493385));
#47083=CARTESIAN_POINT('Ctrl Pts',(0.183872981683724,2.3646735460431,8.08135518686374));
#47084=CARTESIAN_POINT('Ctrl Pts',(0.184798830870546,2.36402851619395,8.08128573104));
#47085=CARTESIAN_POINT('Ctrl Pts',(0.185371659969666,2.36362665442335,8.08124258876916));
#47086=CARTESIAN_POINT('Ctrl Pts',(0.186621615639251,2.36274367390256,8.08114807545155));
#47087=CARTESIAN_POINT('Ctrl Pts',(0.187298198513749,2.36226179747038,8.081096675435));
#47088=CARTESIAN_POINT('Ctrl Pts',(0.189280718492882,2.3608382209381,8.08094534788207));
#47089=CARTESIAN_POINT('Ctrl Pts',(0.190581455807145,2.35988935423807,8.0808451439038));
#47090=CARTESIAN_POINT('Ctrl Pts',(0.204207287660511,2.34979222915017,8.07978564501094));
#47091=CARTESIAN_POINT('Ctrl Pts',(0.215869092902148,2.33978570893113,8.07879223886357));
#47092=CARTESIAN_POINT('Ctrl Pts',(0.249827228802308,2.3061561169588,8.07561967357216));
#47093=CARTESIAN_POINT('Ctrl Pts',(0.269300412909237,2.27997551747219,8.07335292145059));
#47094=CARTESIAN_POINT('Ctrl Pts',(0.285231371271979,2.25002144755127,8.07120747984751));
#47095=CARTESIAN_POINT('Ctrl Pts',(0.285917930959642,2.24870879879461,8.07111432306661));
#47096=CARTESIAN_POINT('Ctrl Pts',(0.286789543296387,2.24701399124889,8.07099519397402));
#47097=CARTESIAN_POINT('Ctrl Pts',(0.286982911174575,2.24663616356739,8.07096870927996));
#47098=CARTESIAN_POINT('Ctrl Pts',(0.287288208621398,2.24603671611384,8.07092680663794));
#47099=CARTESIAN_POINT('Ctrl Pts',(0.287400628610753,2.2458153487852,8.07091135782692));
#47100=CARTESIAN_POINT('Ctrl Pts',(0.287601668457675,2.24541834350253,8.07088369707303));
#47101=CARTESIAN_POINT('Ctrl Pts',(0.287690382656494,2.2452427555988,8.07087147920332));
#47102=CARTESIAN_POINT('Ctrl Pts',(0.287898651188018,2.24482959987472,8.07084276814432));
#47103=CARTESIAN_POINT('Ctrl Pts',(0.288018072089719,2.24459196556757,8.0708262834588));
#47104=CARTESIAN_POINT('Ctrl Pts',(0.288363626333399,2.24390222433458,8.07077851947525));
#47105=CARTESIAN_POINT('Ctrl Pts',(0.288588991585186,2.24344973023557,8.07074728839139));
#47106=CARTESIAN_POINT('Ctrl Pts',(0.290144520970642,2.24030799653598,8.07053115206648));
#47107=CARTESIAN_POINT('Ctrl Pts',(0.291438196054578,2.23760071359634,8.07034848413073));
#47108=CARTESIAN_POINT('Ctrl Pts',(0.295358461970231,2.22909333590502,8.06978435756094));
#47109=CARTESIAN_POINT('Ctrl Pts',(0.297851247751539,2.22323293309606,8.06940991441361));
#47110=CARTESIAN_POINT('Ctrl Pts',(0.305905233084847,2.20262328210052,8.06812895886749));
#47111=CARTESIAN_POINT('Ctrl Pts',(0.310557454665563,2.18754245848042,8.06725331635007));
#47112=CARTESIAN_POINT('Ctrl Pts',(0.319721363269437,2.14766667953609,8.06496549653111));
#47113=CARTESIAN_POINT('Ctrl Pts',(0.32246501364835,2.12258142371212,8.06354590502199));
#47114=CARTESIAN_POINT('Ctrl Pts',(0.322252976516264,2.09595100963283,8.06193042872737));
#47115=CARTESIAN_POINT('Ctrl Pts',(0.32223093108271,2.09446808030353,8.06184014821756));
#47116=CARTESIAN_POINT('Ctrl Pts',(0.322186867061207,2.09244411347299,8.0617164735393));
#47117=CARTESIAN_POINT('Ctrl Pts',(0.322173719369848,2.09190288510134,8.06168335723248));
#47118=CARTESIAN_POINT('Ctrl Pts',(0.322149035116158,2.09098230408023,8.06162695274458));
#47119=CARTESIAN_POINT('Ctrl Pts',(0.32213819207,2.09060293269955,8.06160368632318));
#47120=CARTESIAN_POINT('Ctrl Pts',(0.322114979699215,2.08983809997434,8.06155673500013));
#47121=CARTESIAN_POINT('Ctrl Pts',(0.322102588552658,2.08945263993107,8.061533049451));
#47122=CARTESIAN_POINT('Ctrl Pts',(0.322072873211056,2.0885772005653,8.0614792031574));
#47123=CARTESIAN_POINT('Ctrl Pts',(0.32205512275342,2.08808723754139,8.06144902910326));
#47124=CARTESIAN_POINT('Ctrl Pts',(0.322015638373761,2.08706202357254,8.06138581267104));
#47125=CARTESIAN_POINT('Ctrl Pts',(0.321993687836996,2.08652678290577,8.0613527635811));
#47126=CARTESIAN_POINT('Ctrl Pts',(0.321932647428872,2.0851238241339,8.06126601642054));
#47127=CARTESIAN_POINT('Ctrl Pts',(0.321891384041812,2.08425620932182,8.06121225029567));
#47128=CARTESIAN_POINT('Ctrl Pts',(0.321758403661928,2.08167968083096,8.06105222076367));
#47129=CARTESIAN_POINT('Ctrl Pts',(0.321656582422651,2.07997133994103,8.06094564148171));
#47130=CARTESIAN_POINT('Ctrl Pts',(0.320386574462418,2.06118415379251,8.05976822250179));
#47131=CARTESIAN_POINT('Ctrl Pts',(0.317873182981182,2.04422635672385,8.05865468110537));
#47132=CARTESIAN_POINT('Ctrl Pts',(0.307668812296663,1.9999963910589,8.05562547090836));
#47133=CARTESIAN_POINT('Ctrl Pts',(0.297713271794349,1.97339973961096,8.05366536374296));
#47134=CARTESIAN_POINT('Ctrl Pts',(0.282802134777608,1.94541704220267,8.05162954693993));
#47135=CARTESIAN_POINT('Ctrl Pts',(0.281140968310523,1.94241606506763,8.05141177186864));
#47136=CARTESIAN_POINT('Ctrl Pts',(0.279149641021507,1.93895039568105,8.05116142960734));
#47137=CARTESIAN_POINT('Ctrl Pts',(0.278865852398877,1.9384594988518,8.05112599708508));
#47138=CARTESIAN_POINT('Ctrl Pts',(0.278440672648086,1.93772848345129,8.05107327684008));
#47139=CARTESIAN_POINT('Ctrl Pts',(0.278300265221675,1.93748779846827,8.05105592594053));
#47140=CARTESIAN_POINT('Ctrl Pts',(0.278049043318752,1.93705843681698,8.05102498652711));
#47141=CARTESIAN_POINT('Ctrl Pts',(0.277938348950077,1.93686969108423,8.05101139023574));
#47142=CARTESIAN_POINT('Ctrl Pts',(0.277702307145089,1.9364681522666,8.05098247520626));
#47143=CARTESIAN_POINT('Ctrl Pts',(0.277576907679287,1.93625539110862,8.05096715997913));
#47144=CARTESIAN_POINT('Ctrl Pts',(0.2772383220944,1.93568243070774,8.05092593157139));
#47145=CARTESIAN_POINT('Ctrl Pts',(0.277024677700733,1.93532250073147,8.05090004827204));
#47146=CARTESIAN_POINT('Ctrl Pts',(0.275981272494863,1.93357243671272,8.05077427100324));
#47147=CARTESIAN_POINT('Ctrl Pts',(0.275141727071516,1.9321881205908,8.05067500593205));
#47148=CARTESIAN_POINT('Ctrl Pts',(0.270244434652842,1.92424859567591,8.05010664221756));
#47149=CARTESIAN_POINT('Ctrl Pts',(0.265962593847072,1.91783378394697,8.04965118857925));
#47150=CARTESIAN_POINT('Ctrl Pts',(0.258846929950388,1.90796007629139,8.04894594465641));
#47151=CARTESIAN_POINT('Ctrl Pts',(0.256164548235499,1.90439633901164,8.04869048776538));
#47152=CARTESIAN_POINT('Ctrl Pts',(0.232350996346277,1.87408873376574,8.04649951573247));
#47153=CARTESIAN_POINT('Ctrl Pts',(0.207177000785526,1.85079999251665,8.04466206859706));
#47154=CARTESIAN_POINT('Ctrl Pts',(0.176441898913718,1.83030089612421,8.04244823063142));
#47155=CARTESIAN_POINT('Ctrl Pts',(0.174042324733345,1.8287462097464,8.04227576912201));
#47156=CARTESIAN_POINT('Ctrl Pts',(0.17052414771124,1.82653268126704,8.04202331085988));
#47157=CARTESIAN_POINT('Ctrl Pts',(0.169421704979912,1.82584831721764,8.04194425785081));
#47158=CARTESIAN_POINT('Ctrl Pts',(0.167879023817641,1.82490352499332,8.04183370370002));
#47159=CARTESIAN_POINT('Ctrl Pts',(0.167442242613306,1.82463745246869,8.041802409827));
#47160=CARTESIAN_POINT('Ctrl Pts',(0.166687124470691,1.82417992068118,8.04174832028122));
#47161=CARTESIAN_POINT('Ctrl Pts',(0.166369085529879,1.82398796946903,8.04172554265478));
#47162=CARTESIAN_POINT('Ctrl Pts',(0.165729247570845,1.82360330534216,8.04167972517321));
#47163=CARTESIAN_POINT('Ctrl Pts',(0.165407442570144,1.82341060349548,8.04165668495841));
#47164=CARTESIAN_POINT('Ctrl Pts',(0.164649682880766,1.82295864058669,8.04160243979793));
#47165=CARTESIAN_POINT('Ctrl Pts',(0.164213452036912,1.8226998466215,8.04157121790621));
#47166=CARTESIAN_POINT('Ctrl Pts',(0.16286114084714,1.82190189802909,8.04147444841107));
#47167=CARTESIAN_POINT('Ctrl Pts',(0.161943009624968,1.82136624915834,8.04140877377581));
#47168=CARTESIAN_POINT('Ctrl Pts',(0.159821323779478,1.82014246096992,8.04125705906597));
#47169=CARTESIAN_POINT('Ctrl Pts',(0.158615951684018,1.81945753002208,8.04117090449929));
#47170=CARTESIAN_POINT('Ctrl Pts',(0.15459595947063,1.81720743165206,8.04088367720096));
#47171=CARTESIAN_POINT('Ctrl Pts',(0.151762371691778,1.81567671793193,8.04068138350955));
#47172=CARTESIAN_POINT('Ctrl Pts',(0.140237277667855,1.80967219437791,8.03985903549178));
#47173=CARTESIAN_POINT('Ctrl Pts',(0.131367954096471,1.80555279269056,8.03922697312092));
#47174=CARTESIAN_POINT('Ctrl Pts',(0.106957891818811,1.79553799378884,8.03749067738725));
#47175=CARTESIAN_POINT('Ctrl Pts',(0.0911265576373418,1.79043099203813,
8.03636679112158));
#47176=CARTESIAN_POINT('Ctrl Pts',(0.0565041212295244,1.78214924480458,
8.03395833705492));
#47177=CARTESIAN_POINT('Ctrl Pts',(0.0376777574619463,1.77937188564178,
8.0326783544761));
#47178=CARTESIAN_POINT('Ctrl Pts',(0.0180560694005134,1.77823053461519,
8.03143937899188));
#47179=CARTESIAN_POINT('Ctrl Pts',(0.0173976118359405,1.77819426105755,
8.03139791433188));
#47180=CARTESIAN_POINT('Ctrl Pts',(0.0160684112849866,1.77812512874647,
8.03131444454388));
#47181=CARTESIAN_POINT('Ctrl Pts',(0.0153976670952883,1.77809234483634,
8.03127244360918));
#47182=CARTESIAN_POINT('Ctrl Pts',(0.0144582521664072,1.77804937203362,
8.03121379127825));
#47183=CARTESIAN_POINT('Ctrl Pts',(0.0141896696482295,1.77803742270223,
8.03119704206167));
#47184=CARTESIAN_POINT('Ctrl Pts',(0.0136983283558967,1.77801617877221,
8.0311664377313));
#47185=CARTESIAN_POINT('Ctrl Pts',(0.0134755744447666,1.77800677922275,
8.03115257669639));
#47186=CARTESIAN_POINT('Ctrl Pts',(0.0130227875341184,1.77798814365037,
8.03112442978471));
#47187=CARTESIAN_POINT('Ctrl Pts',(0.0127927542748233,1.77797892295107,
8.03111014479282));
#47188=CARTESIAN_POINT('Ctrl Pts',(0.0122199240160097,1.77795657627671,
8.03107460845182));
#47189=CARTESIAN_POINT('Ctrl Pts',(0.0118771145378527,1.77794375109427,
8.03105337408625));
#47190=CARTESIAN_POINT('Ctrl Pts',(0.0105881735384436,1.7778975900774,8.03097365355546));
#47191=CARTESIAN_POINT('Ctrl Pts',(0.00964190508810644,1.77786787552944,
8.03091536880736));
#47192=CARTESIAN_POINT('Ctrl Pts',(-0.00774447003574694,1.77739859189726,
8.02984868089291));
#47193=CARTESIAN_POINT('Ctrl Pts',(-0.0241969512990017,1.77821386357081,
8.02890797098904));
#47194=CARTESIAN_POINT('Ctrl Pts',(-0.0431726124904631,1.78061862203253,
8.02783132890242));
#47195=CARTESIAN_POINT('Ctrl Pts',(-0.0458235606833914,1.78098818116031,
8.02768112836416));
#47196=CARTESIAN_POINT('Ctrl Pts',(-0.0507395309361855,1.78173604133609,
8.02740253742015));
#47197=CARTESIAN_POINT('Ctrl Pts',(-0.0530056980163761,1.78210560963006,
8.02727409024294));
#47198=CARTESIAN_POINT('Ctrl Pts',(-0.0572493169203863,1.78284430162695,
8.02703324619687));
#47199=CARTESIAN_POINT('Ctrl Pts',(-0.0592276333631066,1.78320778299841,
8.02692083934999));
#47200=CARTESIAN_POINT('Ctrl Pts',(-0.0802942156020735,1.78728263776991,
8.02572147111086));
#47201=CARTESIAN_POINT('Ctrl Pts',(-0.0990106986380144,1.79269543703586,
8.02463187995649));
#47202=CARTESIAN_POINT('Ctrl Pts',(-0.118760480290052,1.80039991969175,
8.02338511435285));
#47203=CARTESIAN_POINT('Ctrl Pts',(-0.120391310018532,1.8010515226581,8.02328143981533));
#47204=CARTESIAN_POINT('Ctrl Pts',(-0.127337026156758,1.80389275656012,
8.02283665456937));
#47205=CARTESIAN_POINT('Ctrl Pts',(-0.132597884008566,1.80621093848339,
8.02249160052005));
#47206=CARTESIAN_POINT('Ctrl Pts',(-0.13868216245179,1.80908867434641,8.022081849102));
#47207=CARTESIAN_POINT('Ctrl Pts',(-0.139568688755252,1.80951295612126,
8.02202187569209));
#47208=CARTESIAN_POINT('Ctrl Pts',(-0.140903452457763,1.81015928009845,
8.02193116648259));
#47209=CARTESIAN_POINT('Ctrl Pts',(-0.141353141979542,1.81037832423035,
8.02190053505295));
#47210=CARTESIAN_POINT('Ctrl Pts',(-0.142155098322651,1.81077127048029,
8.0218457807109));
#47211=CARTESIAN_POINT('Ctrl Pts',(-0.1425075613067,1.81094477183943,8.02182167182255));
#47212=CARTESIAN_POINT('Ctrl Pts',(-0.143188406706408,1.81128146876597,
8.02177501539759));
#47213=CARTESIAN_POINT('Ctrl Pts',(-0.143516829713927,1.81144458126705,
8.02175247079539));
#47214=CARTESIAN_POINT('Ctrl Pts',(-0.144415006273544,1.81189257669022,
8.02169070903602));
#47215=CARTESIAN_POINT('Ctrl Pts',(-0.144984192468745,1.81217858778738,
8.02165145237759));
#47216=CARTESIAN_POINT('Ctrl Pts',(-0.14721619721012,1.81330845153457,8.02149704666146));
#47217=CARTESIAN_POINT('Ctrl Pts',(-0.148872501324297,1.81416502873655,
8.02138145083343));
#47218=CARTESIAN_POINT('Ctrl Pts',(-0.152995457160653,1.8163428206353,8.02109111151884));
#47219=CARTESIAN_POINT('Ctrl Pts',(-0.155452472016573,1.81768185770983,
8.02091574193494));
#47220=CARTESIAN_POINT('Ctrl Pts',(-0.165140770078455,1.82312665666009,
8.02021470272079));
#47221=CARTESIAN_POINT('Ctrl Pts',(-0.172228893430436,1.82747933914487,
8.01968033684558));
#47222=CARTESIAN_POINT('Ctrl Pts',(-0.204623256273757,1.84914098960359,
8.01713530310441));
#47223=CARTESIAN_POINT('Ctrl Pts',(-0.227540005864991,1.8697261825693,8.0150094693528));
#47224=CARTESIAN_POINT('Ctrl Pts',(-0.252173406775543,1.89917728888999,
8.01248278497806));
#47225=CARTESIAN_POINT('Ctrl Pts',(-0.256928214477433,1.90529739525086,
8.01198192667886));
#47226=CARTESIAN_POINT('Ctrl Pts',(-0.261862786940575,1.91214490878677,
8.01145240211319));
#47227=CARTESIAN_POINT('Ctrl Pts',(-0.262265552325784,1.91270762278394,
8.01140910726975));
#47228=CARTESIAN_POINT('Ctrl Pts',(-0.262828582499762,1.91349962441437,
8.01134848498512));
#47229=CARTESIAN_POINT('Ctrl Pts',(-0.262990362339847,1.91372782497048,
8.01133105423034));
#47230=CARTESIAN_POINT('Ctrl Pts',(-0.263270425042855,1.9141239630401,8.01130085936246));
#47231=CARTESIAN_POINT('Ctrl Pts',(-0.263388844490445,1.91429180304388,
8.01128808581576));
#47232=CARTESIAN_POINT('Ctrl Pts',(-0.2636358105623,1.91464254805303,8.01126143358217));
#47233=CARTESIAN_POINT('Ctrl Pts',(-0.26376432724217,1.91482547346377,8.01124755702378));
#47234=CARTESIAN_POINT('Ctrl Pts',(-0.264070626567328,1.91526241330215,
8.01121446681223));
#47235=CARTESIAN_POINT('Ctrl Pts',(-0.264248233804852,1.91551655172469,
8.01119526527826));
#47236=CARTESIAN_POINT('Ctrl Pts',(-0.264846205066268,1.91637482479557,
8.01113056768049));
#47237=CARTESIAN_POINT('Ctrl Pts',(-0.265264870216766,1.91698014872478,
8.01108518724908));
#47238=CARTESIAN_POINT('Ctrl Pts',(-0.266254312296448,1.91842125373026,
8.01097772702684));
#47239=CARTESIAN_POINT('Ctrl Pts',(-0.266823236996412,1.9192583053797,8.01091576868092));
#47240=CARTESIAN_POINT('Ctrl Pts',(-0.273519623984519,1.92921114269453,
8.01018430688131));
#47241=CARTESIAN_POINT('Ctrl Pts',(-0.27918185940648,1.93863283160152,8.00954374620886));
#47242=CARTESIAN_POINT('Ctrl Pts',(-0.297350731841026,1.97269518293874,
8.0073387619821));
#47243=CARTESIAN_POINT('Ctrl Pts',(-0.307162667955773,1.99863346019444,
8.00584326633498));
#47244=CARTESIAN_POINT('Ctrl Pts',(-0.314057772310764,2.0276551984056,8.00411465129187));
#47245=CARTESIAN_POINT('Ctrl Pts',(-0.314546233488024,2.02980939257973,
8.00398610096488));
#47246=CARTESIAN_POINT('Ctrl Pts',(-0.315466790921449,2.03407192833006,
8.00373111862418));
#47247=CARTESIAN_POINT('Ctrl Pts',(-0.315899989087747,2.03617991376101,
8.00360472378153));
#47248=CARTESIAN_POINT('Ctrl Pts',(-0.31758361691104,2.04481010996982,8.00308579924355));
#47249=CARTESIAN_POINT('Ctrl Pts',(-0.318653347641777,2.05136552577701,
8.0026881929111));
#47250=CARTESIAN_POINT('Ctrl Pts',(-0.319655382151488,2.05897936623701,
8.00222082297327));
#47251=CARTESIAN_POINT('Ctrl Pts',(-0.319786003265718,2.06001040374796,
8.00215741729286));
#47252=CARTESIAN_POINT('Ctrl Pts',(-0.319972656238297,2.06154314483822,
8.00206297985656));
#47253=CARTESIAN_POINT('Ctrl Pts',(-0.320032500991799,2.06204438442763,
8.00203206844131));
#47254=CARTESIAN_POINT('Ctrl Pts',(-0.320136888478763,2.06293650005617,
8.0019770005772));
#47255=CARTESIAN_POINT('Ctrl Pts',(-0.320181893718432,2.06332732180967,
8.00195285876294));
#47256=CARTESIAN_POINT('Ctrl Pts',(-0.320267439814649,2.06408235925827,
8.00190618456229));
#47257=CARTESIAN_POINT('Ctrl Pts',(-0.320308075287554,2.06444656379901,
8.00188365519855));
#47258=CARTESIAN_POINT('Ctrl Pts',(-0.320394550936059,2.06523380354441,
8.00183492385856));
#47259=CARTESIAN_POINT('Ctrl Pts',(-0.320440174624997,2.06565686139799,
8.00180871509913));
#47260=CARTESIAN_POINT('Ctrl Pts',(-0.320548702743619,2.06668226342327,
8.00174513963094));
#47261=CARTESIAN_POINT('Ctrl Pts',(-0.320610747213115,2.06728469525366,
8.00170774589222));
#47262=CARTESIAN_POINT('Ctrl Pts',(-0.320774454032542,2.06891943903787,
8.00160615785621));
#47263=CARTESIAN_POINT('Ctrl Pts',(-0.32087283035391,2.06995206613025,8.00154186034191));
#47264=CARTESIAN_POINT('Ctrl Pts',(-0.321844500656401,2.08070081173445,
8.00087123075178));
#47265=CARTESIAN_POINT('Ctrl Pts',(-0.322281094240882,2.09045023344166,
8.00025125180471));
#47266=CARTESIAN_POINT('Ctrl Pts',(-0.322274935754178,2.10020349358851,
7.99961864007736));
#47267=CARTESIAN_POINT('',(-0.32227487097392,2.09971161875376,7.74930651681519));
#47268=CARTESIAN_POINT('Ctrl Pts',(-0.322274936001444,2.10020310161215,
7.99961866550156));
#47269=CARTESIAN_POINT('Ctrl Pts',(-0.322257797933066,2.12739722297387,
7.99785481310939));
#47270=CARTESIAN_POINT('Ctrl Pts',(-0.318798481849687,2.15447919365321,
7.99599019670084));
#47271=CARTESIAN_POINT('Ctrl Pts',(-0.308742202953932,2.19330785843882,
7.9933020014482));
#47272=CARTESIAN_POINT('Ctrl Pts',(-0.30475322724803,2.20561089968102,7.99245041160271));
#47273=CARTESIAN_POINT('Ctrl Pts',(-0.299759189787279,2.21834769720163,
7.99159160860261));
#47274=CARTESIAN_POINT('Ctrl Pts',(-0.299480218221135,2.2190518719575,7.99154420524644));
#47275=CARTESIAN_POINT('Ctrl Pts',(-0.299082198592176,2.22004629320163,
7.99147737890527));
#47276=CARTESIAN_POINT('Ctrl Pts',(-0.298965208053927,2.22033735247817,
7.99145783341549));
#47277=CARTESIAN_POINT('Ctrl Pts',(-0.298763859835523,2.22083617820544,
7.99142436049074));
#47278=CARTESIAN_POINT('Ctrl Pts',(-0.298679710095587,2.22104402788017,
7.99141042042675));
#47279=CARTESIAN_POINT('Ctrl Pts',(-0.298518354332567,2.22144138349115,
7.99138378489321));
#47280=CARTESIAN_POINT('Ctrl Pts',(-0.298441184853786,2.22163090347979,
7.9913710872112));
#47281=CARTESIAN_POINT('Ctrl Pts',(-0.2982592584796,2.22207647969435,7.99134124831531));
#47282=CARTESIAN_POINT('Ctrl Pts',(-0.298154352067245,2.2223324752797,7.99132411621202));
#47283=CARTESIAN_POINT('Ctrl Pts',(-0.297844338678386,2.22308621106716,
7.99127370559063));
#47284=CARTESIAN_POINT('Ctrl Pts',(-0.29763831274228,2.22358357591294,7.99124048242729));
#47285=CARTESIAN_POINT('Ctrl Pts',(-0.295854491246779,2.22785954350532,
7.99095518955837));
#47286=CARTESIAN_POINT('Ctrl Pts',(-0.294205970394984,2.23160848624457,
7.99070731249554));
#47287=CARTESIAN_POINT('Ctrl Pts',(-0.29231741459194,2.23569033353268,7.99043883484352));
#47288=CARTESIAN_POINT('Ctrl Pts',(-0.292147792798575,2.23605515298583,
7.9904148518786));
#47289=CARTESIAN_POINT('Ctrl Pts',(-0.291859556853939,2.23667206120576,
7.99037431640091));
#47290=CARTESIAN_POINT('Ctrl Pts',(-0.291741298608684,2.2369243145988,7.99035774703223));
#47291=CARTESIAN_POINT('Ctrl Pts',(-0.29048472607817,2.23959565638916,7.99018233455661));
#47292=CARTESIAN_POINT('Ctrl Pts',(-0.28931664600126,2.2420007131416,7.99002489178643));
#47293=CARTESIAN_POINT('Ctrl Pts',(-0.274229074490091,2.27210654656531,
7.98805679135534));
#47294=CARTESIAN_POINT('Ctrl Pts',(-0.256412443957212,2.29767473439104,
7.98639920127045));
#47295=CARTESIAN_POINT('Ctrl Pts',(-0.229479495099375,2.32643045870218,
7.98412801474645));
#47296=CARTESIAN_POINT('Ctrl Pts',(-0.223506540323487,2.33232821802786,
7.98363686966656));
#47297=CARTESIAN_POINT('Ctrl Pts',(-0.215229993172497,2.33988573116558,
7.98296744806809));
#47298=CARTESIAN_POINT('Ctrl Pts',(-0.213124614195332,2.34175816852431,
7.98279808062119));
#47299=CARTESIAN_POINT('Ctrl Pts',(-0.209578584924454,2.34482954009607,
7.98251416295093));
#47300=CARTESIAN_POINT('Ctrl Pts',(-0.20815151657745,2.3460439653371,7.98240025592571));
#47301=CARTESIAN_POINT('Ctrl Pts',(-0.206223883561348,2.34765559459753,
7.98224683066609));
#47302=CARTESIAN_POINT('Ctrl Pts',(-0.205732591149816,2.34806387204932,
7.98220776501346));
#47303=CARTESIAN_POINT('Ctrl Pts',(-0.204957320887053,2.34870425560182,
7.98214617614296));
#47304=CARTESIAN_POINT('Ctrl Pts',(-0.204674153299718,2.34893734374122,
7.98212369282998));
#47305=CARTESIAN_POINT('Ctrl Pts',(-0.204086946610867,2.34941902109655,
7.98207709356682));
#47306=CARTESIAN_POINT('Ctrl Pts',(-0.203782849898272,2.3496675388329,7.9820529747804));
#47307=CARTESIAN_POINT('Ctrl Pts',(-0.20309124416718,2.35023063619736,7.98199815188093));
#47308=CARTESIAN_POINT('Ctrl Pts',(-0.202703457756257,2.35054487214529,
7.98196743398704));
#47309=CARTESIAN_POINT('Ctrl Pts',(-0.201553820070784,2.35147204486863,
7.98187642977763));
#47310=CARTESIAN_POINT('Ctrl Pts',(-0.200789912587256,2.35208241252613,
7.98181604054607));
#47311=CARTESIAN_POINT('Ctrl Pts',(-0.195590021029448,2.35619853154361,
7.98140550260741));
#47312=CARTESIAN_POINT('Ctrl Pts',(-0.191065459658687,2.3595903069749,7.98105085713667));
#47313=CARTESIAN_POINT('Ctrl Pts',(-0.185434416678194,2.36358455207834,
7.98061218544199));
#47314=CARTESIAN_POINT('Ctrl Pts',(-0.184410394007974,2.36430199676815,
7.98053251910685));
#47315=CARTESIAN_POINT('Ctrl Pts',(-0.17073499061825,2.37376501065391,7.97947001574154));
#47316=CARTESIAN_POINT('Ctrl Pts',(-0.15747913243314,2.38159888527657,7.9784545934656));
#47317=CARTESIAN_POINT('Ctrl Pts',(-0.134312703593152,2.39314100956954,
7.97671574137277));
#47318=CARTESIAN_POINT('Ctrl Pts',(-0.124685757814235,2.3973634272561,7.976003088547));
#47319=CARTESIAN_POINT('Ctrl Pts',(-0.099438261127418,2.4069951227345,7.97417687156147));
#47320=CARTESIAN_POINT('Ctrl Pts',(-0.0835747797115143,2.41168792223467,
7.97306912039826));
#47321=CARTESIAN_POINT('Ctrl Pts',(-0.0656226262062978,2.41552848378936,
7.97190494435722));
#47322=CARTESIAN_POINT('Ctrl Pts',(-0.063822179623753,2.41589758295875,
7.97178917985791));
#47323=CARTESIAN_POINT('Ctrl Pts',(-0.0615900041727687,2.41633532491882,
7.97164696545227));
#47324=CARTESIAN_POINT('Ctrl Pts',(-0.0611612105061166,2.41641850884593,
7.97161970617459));
#47325=CARTESIAN_POINT('Ctrl Pts',(-0.060485718753012,2.4165481266181,7.97157685913153));
#47326=CARTESIAN_POINT('Ctrl Pts',(-0.0602391352600067,2.41659514402886,
7.97156123810791));
#47327=CARTESIAN_POINT('Ctrl Pts',(-0.0597780578645253,2.41668250197535,
7.97153206661166));
#47328=CARTESIAN_POINT('Ctrl Pts',(-0.0595635795386323,2.41672291242092,
7.97151851224435));
#47329=CARTESIAN_POINT('Ctrl Pts',(-0.0590811787736625,2.41681329551993,
7.97148806020201));
#47330=CARTESIAN_POINT('Ctrl Pts',(-0.0588132345239964,2.41686314608932,
7.97147116961659));
#47331=CARTESIAN_POINT('Ctrl Pts',(-0.0581303648987129,2.41698929679926,
7.97142818264939));
#47332=CARTESIAN_POINT('Ctrl Pts',(-0.0577153507438399,2.41706512249355,
7.97140211330305));
#47333=CARTESIAN_POINT('Ctrl Pts',(-0.0553983270936908,2.41748375726197,
7.97125687451827));
#47334=CARTESIAN_POINT('Ctrl Pts',(-0.0534933605743605,2.41781027606978,
7.971138616362));
#47335=CARTESIAN_POINT('Ctrl Pts',(-0.0163286866872248,2.4238368102578,
7.96885184931841));
#47336=CARTESIAN_POINT('Ctrl Pts',(0.0196394734100666,2.42365451397915,
7.96697235185748));
#47337=CARTESIAN_POINT('Ctrl Pts',(0.0638330293052665,2.41602154803857,
7.96439671965998));
#47338=CARTESIAN_POINT('Ctrl Pts',(0.072745358366456,2.41408974248339,7.96386487807681));
#47339=CARTESIAN_POINT('Ctrl Pts',(0.0844711198538033,2.41102224913583,
7.96314199806779));
#47340=CARTESIAN_POINT('Ctrl Pts',(0.0873680549460995,2.41022093999398,
7.96296150882049));
#47341=CARTESIAN_POINT('Ctrl Pts',(0.0915176929709229,2.40901039185598,
7.96270005411243));
#47342=CARTESIAN_POINT('Ctrl Pts',(0.0927798105124144,2.40863379122095,
7.96262014148876));
#47343=CARTESIAN_POINT('Ctrl Pts',(0.0950138548546043,2.40795223751178,
7.96247797973064));
#47344=CARTESIAN_POINT('Ctrl Pts',(0.0959867163971077,2.40765039158239,
7.96241583239976));
#47345=CARTESIAN_POINT('Ctrl Pts',(0.0974338967053205,2.40719384806247,
7.96232302143826));
#47346=CARTESIAN_POINT('Ctrl Pts',(0.0979093202017549,2.40704265099139,
7.96229247280491));
#47347=CARTESIAN_POINT('Ctrl Pts',(0.0987437452809462,2.406775146976,7.96223875249521));
#47348=CARTESIAN_POINT('Ctrl Pts',(0.09910289811385,2.40665931196969,7.96221559638444));
#47349=CARTESIAN_POINT('Ctrl Pts',(0.0998183826008016,2.40642716364788,
7.96216939822123));
#47350=CARTESIAN_POINT('Ctrl Pts',(0.10017471647126,2.40631085893971,7.96214635648142));
#47351=CARTESIAN_POINT('Ctrl Pts',(0.101028806229109,2.40603044069447,7.96209104717703));
#47352=CARTESIAN_POINT('Ctrl Pts',(0.101526365062282,2.40586573445189,7.96205876009313));
#47353=CARTESIAN_POINT('Ctrl Pts',(0.103326908276328,2.40526482551238,7.96194168004091));
#47354=CARTESIAN_POINT('Ctrl Pts',(0.104627487180078,2.40482150925027,7.96185665221425));
#47355=CARTESIAN_POINT('Ctrl Pts',(0.127990192405451,2.39669094610912,7.96032088718429));
#47356=CARTESIAN_POINT('Ctrl Pts',(0.149150047050696,2.3866371413786,7.95878714149822));
#47357=CARTESIAN_POINT('Ctrl Pts',(0.181052430784703,2.36698399885061,7.95626268561711));
#47358=CARTESIAN_POINT('Ctrl Pts',(0.192571484804247,2.35879850087038,7.95530173375331));
#47359=CARTESIAN_POINT('Ctrl Pts',(0.212462190331338,2.34259862430589,7.95358400648746));
#47360=CARTESIAN_POINT('Ctrl Pts',(0.22101101020981,2.33483711237641,7.95282346353582));
#47361=CARTESIAN_POINT('Ctrl Pts',(0.23023336385096,2.32551331174303,7.95199369111833));
#47362=CARTESIAN_POINT('Ctrl Pts',(0.231332609827026,2.32438555986114,7.95189463137462));
#47363=CARTESIAN_POINT('Ctrl Pts',(0.23271076654647,2.32295077178292,7.95177029201083));
#47364=CARTESIAN_POINT('Ctrl Pts',(0.232997386575792,2.32265121908196,7.9517444246957));
#47365=CARTESIAN_POINT('Ctrl Pts',(0.233453208411968,2.32217298589373,7.95170327542622));
#47366=CARTESIAN_POINT('Ctrl Pts',(0.233622783766887,2.32199466454121,7.95168796446432));
#47367=CARTESIAN_POINT('Ctrl Pts',(0.23394286867813,2.32165729802465,7.95165905944883));
#47368=CARTESIAN_POINT('Ctrl Pts',(0.234093419140772,2.32149829500074,7.95164546224174));
#47369=CARTESIAN_POINT('Ctrl Pts',(0.234436192140971,2.32113553740562,7.95161449969089));
#47370=CARTESIAN_POINT('Ctrl Pts',(0.234628310825407,2.32093168593453,7.95159714245215));
#47371=CARTESIAN_POINT('Ctrl Pts',(0.235200503970359,2.32032296052593,7.95154543623974));
#47372=CARTESIAN_POINT('Ctrl Pts',(0.235579800477262,2.31991735179558,7.95151114713743));
#47373=CARTESIAN_POINT('Ctrl Pts',(0.238230420286007,2.31706812892288,7.95127141065425));
#47374=CARTESIAN_POINT('Ctrl Pts',(0.240464832723468,2.3145902422779,7.95106872121094));
#47375=CARTESIAN_POINT('Ctrl Pts',(0.252421575136603,2.30090929062258,7.94997787705335));
#47376=CARTESIAN_POINT('Ctrl Pts',(0.261401163742051,2.28907863262666,7.94913524804617));
#47377=CARTESIAN_POINT('Ctrl Pts',(0.286078058984446,2.25143064639639,7.9466074532951));
#47378=CARTESIAN_POINT('Ctrl Pts',(0.298992798346094,2.22399612680732,7.94494945878449));
#47379=CARTESIAN_POINT('Ctrl Pts',(0.308487998416017,2.19327512416568,7.94301594897095));
#47380=CARTESIAN_POINT('Ctrl Pts',(0.309055082084787,2.19137860759553,7.94289637272178));
#47381=CARTESIAN_POINT('Ctrl Pts',(0.309873049027505,2.18854831249368,7.9427175551475));
#47382=CARTESIAN_POINT('Ctrl Pts',(0.310137266634798,2.18761841114559,7.94265874568608));
#47383=CARTESIAN_POINT('Ctrl Pts',(0.310552377666413,2.18613204258623,7.94256464512358));
#47384=CARTESIAN_POINT('Ctrl Pts',(0.310705969973351,2.18557632996613,7.94252944155155));
#47385=CARTESIAN_POINT('Ctrl Pts',(0.310995237259413,2.18451868650653,7.94246239842274));
#47386=CARTESIAN_POINT('Ctrl Pts',(0.311131190516677,2.18401683313181,7.94243056799322));
#47387=CARTESIAN_POINT('Ctrl Pts',(0.311366908701548,2.18313829224161,7.94237481293953));
#47388=CARTESIAN_POINT('Ctrl Pts',(0.311467206278036,2.18276174770029,7.94235090563529));
#47389=CARTESIAN_POINT('Ctrl Pts',(0.311661361731219,2.18202748321121,7.94230426526997));
#47390=CARTESIAN_POINT('Ctrl Pts',(0.311755287308431,2.1816697816306,7.9422815344422));
#47391=CARTESIAN_POINT('Ctrl Pts',(0.31197603700959,2.1808231593365,7.94222771095885));
#47392=CARTESIAN_POINT('Ctrl Pts',(0.312102327545793,2.18033410165805,7.94219660109135));
#47393=CARTESIAN_POINT('Ctrl Pts',(0.312539735739782,2.17862364667735,7.94208773051031));
#47394=CARTESIAN_POINT('Ctrl Pts',(0.312844834399213,2.17740073481879,7.94200977565775));
#47395=CARTESIAN_POINT('Ctrl Pts',(0.316922081367403,2.16064008835287,7.9409396995577));
#47396=CARTESIAN_POINT('Ctrl Pts',(0.319539418380532,2.14484690618175,7.93991011923873));
#47397=CARTESIAN_POINT('Ctrl Pts',(0.322930326010057,2.10722107428564,7.93740867701181));
#47398=CARTESIAN_POINT('Ctrl Pts',(0.322679543694788,2.08537342549922,7.93591609115748));
#47399=CARTESIAN_POINT('Ctrl Pts',(0.319231820324013,2.05494123163268,7.93386609340602));
#47400=CARTESIAN_POINT('Ctrl Pts',(0.31787641775254,2.04620542715606,7.93328180917602));
#47401=CARTESIAN_POINT('Ctrl Pts',(0.315404922342017,2.03369592568333,7.9324608087739));
#47402=CARTESIAN_POINT('Ctrl Pts',(0.314576360130593,2.02987003216489,7.93221187891341));
#47403=CARTESIAN_POINT('Ctrl Pts',(0.313554334980625,2.02553426040452,7.9319329751747));
#47404=CARTESIAN_POINT('Ctrl Pts',(0.313429091100962,2.02500885238682,7.93189923149284));
#47405=CARTESIAN_POINT('Ctrl Pts',(0.313238513826322,2.02421818352803,7.93184853544579));
#47406=CARTESIAN_POINT('Ctrl Pts',(0.31317416387825,2.02395269016987,7.93183152678729));
#47407=CARTESIAN_POINT('Ctrl Pts',(0.313057783481313,2.0234751838766,7.93180096166106));
#47408=CARTESIAN_POINT('Ctrl Pts',(0.313005875302479,2.02326314244093,7.93178739816735));
#47409=CARTESIAN_POINT('Ctrl Pts',(0.312893923254408,2.02280782940814,7.93175829345114));
#47410=CARTESIAN_POINT('Ctrl Pts',(0.312833811292982,2.02256457578634,7.93174275627582));
#47411=CARTESIAN_POINT('Ctrl Pts',(0.312671288363382,2.02191017616747,7.93170099044551));
#47412=CARTESIAN_POINT('Ctrl Pts',(0.312568349725254,2.02149915982671,7.93167479231909));
#47413=CARTESIAN_POINT('Ctrl Pts',(0.3120921951187,2.01961374177849,7.93155476814143));
#47414=CARTESIAN_POINT('Ctrl Pts',(0.311709347641557,2.01814175929524,7.93146149018665));
#47415=CARTESIAN_POINT('Ctrl Pts',(0.303754752831987,1.98842295618111,7.92958587525625));
#47416=CARTESIAN_POINT('Ctrl Pts',(0.292382139559771,1.96132875076995,7.92800688573116));
#47417=CARTESIAN_POINT('Ctrl Pts',(0.267410735147483,1.9190387151782,7.92524112964321));
#47418=CARTESIAN_POINT('Ctrl Pts',(0.255757166163526,1.90291224619023,7.92409895428312));
#47419=CARTESIAN_POINT('Ctrl Pts',(0.242079092787087,1.88725657427769,7.92283673157989));
#47420=CARTESIAN_POINT('Ctrl Pts',(0.24145997203141,1.88655414215673,7.92277975575125));
#47421=CARTESIAN_POINT('Ctrl Pts',(0.240463067695954,1.88543297843627,7.92268825914674));
#47422=CARTESIAN_POINT('Ctrl Pts',(0.240087227712111,1.88501251954675,7.92265381959869));
#47423=CARTESIAN_POINT('Ctrl Pts',(0.239368382859633,1.88421257085575,7.922588053281));
#47424=CARTESIAN_POINT('Ctrl Pts',(0.239025573988094,1.88383290661061,7.92255673480699));
#47425=CARTESIAN_POINT('Ctrl Pts',(0.238420760373258,1.88316626727149,7.92250155770633));
#47426=CARTESIAN_POINT('Ctrl Pts',(0.238159137144458,1.88287894616504,7.92247771525793));
#47427=CARTESIAN_POINT('Ctrl Pts',(0.237645644266715,1.88231706035975,7.92243096855573));
#47428=CARTESIAN_POINT('Ctrl Pts',(0.237393816769984,1.88204245778838,7.92240806611322));
#47429=CARTESIAN_POINT('Ctrl Pts',(0.236792314067117,1.8813888347922,7.92235341706822));
#47430=CARTESIAN_POINT('Ctrl Pts',(0.236442205040468,1.88101021661859,7.92232165197905));
#47431=CARTESIAN_POINT('Ctrl Pts',(0.235383425253319,1.87987072004602,7.92222572031245));
#47432=CARTESIAN_POINT('Ctrl Pts',(0.234671984588109,1.87911243496771,7.92216143504011));
#47433=CARTESIAN_POINT('Ctrl Pts',(0.227239609495639,1.87126711525361,7.92149163325118));
#47434=CARTESIAN_POINT('Ctrl Pts',(0.220204130304307,1.86448634771157,7.92087241350607));
#47435=CARTESIAN_POINT('Ctrl Pts',(0.195193912095052,1.84248315365438,7.9187163178867));
#47436=CARTESIAN_POINT('Ctrl Pts',(0.175866265963533,1.82891633264268,7.91711755013175));
#47437=CARTESIAN_POINT('Ctrl Pts',(0.147839351214534,1.81351096267461,7.9149578351609));
#47438=CARTESIAN_POINT('Ctrl Pts',(0.140284045480136,1.80973659905472,7.9143905783939));
#47439=CARTESIAN_POINT('Ctrl Pts',(0.125319535028243,1.80298181714127,7.91330560824192));
#47440=CARTESIAN_POINT('Ctrl Pts',(0.117930112759263,1.79997116909613,7.91278726333764));
#47441=CARTESIAN_POINT('Ctrl Pts',(0.109241385718556,1.79680186005571,7.91220366808825));
#47442=CARTESIAN_POINT('Ctrl Pts',(0.108044248116191,1.79637320112335,7.91212382073251));
#47443=CARTESIAN_POINT('Ctrl Pts',(0.106482288030301,1.79582431815522,7.91202039786929));
#47444=CARTESIAN_POINT('Ctrl Pts',(0.106119765142266,1.79569765275354,7.91199644691518));
#47445=CARTESIAN_POINT('Ctrl Pts',(0.105531032421204,1.79549312971287,7.91195763776548));
#47446=CARTESIAN_POINT('Ctrl Pts',(0.105304962133066,1.79541487592629,7.91194275602299));
#47447=CARTESIAN_POINT('Ctrl Pts',(0.104870106553759,1.79526489353509,7.91191417058083));
#47448=CARTESIAN_POINT('Ctrl Pts',(0.104661335316596,1.79519312794698,7.91190046473836));
#47449=CARTESIAN_POINT('Ctrl Pts',(0.104179517818542,1.79502805546729,7.91186887424831));
#47450=CARTESIAN_POINT('Ctrl Pts',(0.103906419015623,1.79493490043293,7.91185099867832));
#47451=CARTESIAN_POINT('Ctrl Pts',(0.103032845071531,1.79463823021166,7.91179391474199));
#47452=CARTESIAN_POINT('Ctrl Pts',(0.102431889586267,1.79443611858779,7.91175478925918));
#47453=CARTESIAN_POINT('Ctrl Pts',(0.0970392932046791,1.79264019263358,
7.91140495965208));
#47454=CARTESIAN_POINT('Ctrl Pts',(0.0922110822577378,1.79115732346877,
7.91110063342681));
#47455=CARTESIAN_POINT('Ctrl Pts',(0.0863691812529429,1.78951235485459,
7.91074079754704));
#47456=CARTESIAN_POINT('Ctrl Pts',(0.0853873538144352,1.7892409082366,7.91068060317246));
#47457=CARTESIAN_POINT('Ctrl Pts',(0.0534910390827794,1.78058508723307,
7.90873373668274));
#47458=CARTESIAN_POINT('Ctrl Pts',(0.0214973645616857,1.77685057596685,
7.90702716714788));
#47459=CARTESIAN_POINT('Ctrl Pts',(-0.0218462293014116,1.77826683355827,
7.9045300110437));
#47460=CARTESIAN_POINT('Ctrl Pts',(-0.0331392048114361,1.77923335752483,
7.90386436326444));
#47461=CARTESIAN_POINT('Ctrl Pts',(-0.0463659463247003,1.78107134308125,
7.90305687892157));
#47462=CARTESIAN_POINT('Ctrl Pts',(-0.0483721174638344,1.78136945039266,
7.90293365370172));
#47463=CARTESIAN_POINT('Ctrl Pts',(-0.0510268182456624,1.78178957505528,
7.90276955642636));
#47464=CARTESIAN_POINT('Ctrl Pts',(-0.0516780082948458,1.78189468069167,
7.9027292209795));
#47465=CARTESIAN_POINT('Ctrl Pts',(-0.0527464657651205,1.7820705029648,
7.90266290177858));
#47466=CARTESIAN_POINT('Ctrl Pts',(-0.0531639268907506,1.78214004402786,
7.90263695539164));
#47467=CARTESIAN_POINT('Ctrl Pts',(-0.0539725016791286,1.78227637462965,
7.90258663273277));
#47468=CARTESIAN_POINT('Ctrl Pts',(-0.0543636315459367,1.78234306458243,
7.90256225966737));
#47469=CARTESIAN_POINT('Ctrl Pts',(-0.0552663115410769,1.78249869287234,
7.90250593846617));
#47470=CARTESIAN_POINT('Ctrl Pts',(-0.055777770865429,1.78258814532003,
7.90247397403264));
#47471=CARTESIAN_POINT('Ctrl Pts',(-0.0571484585988294,1.7828312890581,
7.90238816809724));
#47472=CARTESIAN_POINT('Ctrl Pts',(-0.0580072780052151,1.78298723496492,
7.90233425494789));
#47473=CARTESIAN_POINT('Ctrl Pts',(-0.0640702884933305,1.78411362936393,
7.90195256709336));
#47474=CARTESIAN_POINT('Ctrl Pts',(-0.0692502457351405,1.78520864193262,
7.90162083846191));
#47475=CARTESIAN_POINT('Ctrl Pts',(-0.0759430026804297,1.78679663356211,
7.9011845348271));
#47476=CARTESIAN_POINT('Ctrl Pts',(-0.0774826135918362,1.78717395752025,
7.90108363462428));
#47477=CARTESIAN_POINT('Ctrl Pts',(-0.0795557971862356,1.78769829181636,
7.90094704312417));
#47478=CARTESIAN_POINT('Ctrl Pts',(-0.0800918846675346,1.78783534504265,
7.90091165764534));
#47479=CARTESIAN_POINT('Ctrl Pts',(-0.0834399470897636,1.78870048478004,
7.90069025301422));
#47480=CARTESIAN_POINT('Ctrl Pts',(-0.0862422543900602,1.78946516191003,
7.90050313053605));
#47481=CARTESIAN_POINT('Ctrl Pts',(-0.116064224383297,1.79803760223737,
7.89849246057288));
#47482=CARTESIAN_POINT('Ctrl Pts',(-0.141959182766014,1.80931229895432,
7.89656090106894));
#47483=CARTESIAN_POINT('Ctrl Pts',(-0.175686060832555,1.8295895141688,7.89392813877432));
#47484=CARTESIAN_POINT('Ctrl Pts',(-0.185007447698949,1.83587933720208,
7.89318827318453));
#47485=CARTESIAN_POINT('Ctrl Pts',(-0.194800235201608,1.84326065039731,
7.89241251273499));
#47486=CARTESIAN_POINT('Ctrl Pts',(-0.195615444804508,1.84388123245592,
7.89234794770617));
#47487=CARTESIAN_POINT('Ctrl Pts',(-0.197016866630122,1.84495866572273,
7.89223699842934));
#47488=CARTESIAN_POINT('Ctrl Pts',(-0.19760447793628,1.84541367229913,7.89219049127293));
#47489=CARTESIAN_POINT('Ctrl Pts',(-0.198435973282791,1.84606213944095,
7.89212470718168));
#47490=CARTESIAN_POINT('Ctrl Pts',(-0.198681153415577,1.846253922597,7.89210531282292));
#47491=CARTESIAN_POINT('Ctrl Pts',(-0.199102121590258,1.8465841937001,7.89207201920991));
#47492=CARTESIAN_POINT('Ctrl Pts',(-0.199278043628648,1.84672250981771,
7.89205810766765));
#47493=CARTESIAN_POINT('Ctrl Pts',(-0.199614954285152,1.84698796919347,
7.89203146918543));
#47494=CARTESIAN_POINT('Ctrl Pts',(-0.199775965326588,1.84711508272431,
7.89201874014399));
#47495=CARTESIAN_POINT('Ctrl Pts',(-0.200155414152943,1.84741523508469,
7.89198874556836));
#47496=CARTESIAN_POINT('Ctrl Pts',(-0.200373749504362,1.84758840400453,
7.8919714893833));
#47497=CARTESIAN_POINT('Ctrl Pts',(-0.201019344344136,1.84810181196337,
7.89192047182162));
#47498=CARTESIAN_POINT('Ctrl Pts',(-0.20144596654637,1.84844285637419,7.8918867677015));
#47499=CARTESIAN_POINT('Ctrl Pts',(-0.205231054702886,1.85148448298315,
7.89158779935572));
#47500=CARTESIAN_POINT('Ctrl Pts',(-0.208536100993626,1.85425125227808,
7.89132718336066));
#47501=CARTESIAN_POINT('Ctrl Pts',(-0.232491599691991,1.87513667857228,
7.88943298318641));
#47502=CARTESIAN_POINT('Ctrl Pts',(-0.250807788085938,1.89576549787855,
7.8879476237939));
#47503=CARTESIAN_POINT('Ctrl Pts',(-0.276926822112255,1.9340796124684,7.88532867787026));
#47504=CARTESIAN_POINT('Ctrl Pts',(-0.286172938612336,1.9505914096165,7.88423695872313));
#47505=CARTESIAN_POINT('Ctrl Pts',(-0.294384116166399,1.96884950856838,
7.88301941628957));
#47506=CARTESIAN_POINT('Ctrl Pts',(-0.294843357859363,1.9698852293984,7.88295032683834));
#47507=CARTESIAN_POINT('Ctrl Pts',(-0.295506575852445,1.97140251661407,
7.88284907346148));
#47508=CARTESIAN_POINT('Ctrl Pts',(-0.295714860012506,1.9718822000348,7.88281705682201));
#47509=CARTESIAN_POINT('Ctrl Pts',(-0.296078787629978,1.97272594958408,
7.88276072935585));
#47510=CARTESIAN_POINT('Ctrl Pts',(-0.296234929826972,1.97308980048138,
7.8827364355922));
#47511=CARTESIAN_POINT('Ctrl Pts',(-0.296537132656912,1.97379760612631,
7.88268916908606));
#47512=CARTESIAN_POINT('Ctrl Pts',(-0.296683266426591,1.97414152915098,
7.88266619887845));
#47513=CARTESIAN_POINT('Ctrl Pts',(-0.297071416963216,1.97505946649003,
7.88260488146495));
#47514=CARTESIAN_POINT('Ctrl Pts',(-0.297312367222174,1.97563392754318,
7.88256649809822));
#47515=CARTESIAN_POINT('Ctrl Pts',(-0.298170841851653,1.97769741121766,
7.88242858583727));
#47516=CARTESIAN_POINT('Ctrl Pts',(-0.298778849927427,1.97919034460017,
7.88232873531422));
#47517=CARTESIAN_POINT('Ctrl Pts',(-0.308724402663005,2.00414550366828,
7.88065832628991));
#47518=CARTESIAN_POINT('Ctrl Pts',(-0.315281750750485,2.02861555758866,
7.87898980458297));
#47519=CARTESIAN_POINT('Ctrl Pts',(-0.321160253429432,2.06901465873945,
7.87623186467879));
#47520=CARTESIAN_POINT('Ctrl Pts',(-0.322282781442665,2.08457794132063,
7.87517139817404));
#47521=CARTESIAN_POINT('Ctrl Pts',(-0.322270477898228,2.10909031257621,
7.87354994536088));
#47522=CARTESIAN_POINT('Ctrl Pts',(-0.321894950252477,2.11801582031185,
7.87297001678884));
#47523=CARTESIAN_POINT('Ctrl Pts',(-0.321089454267323,2.12762694870816,
7.87236476429156));
#47524=CARTESIAN_POINT('Ctrl Pts',(-0.321027426366448,2.12833862170505,
7.87232006202176));
#47525=CARTESIAN_POINT('Ctrl Pts',(-0.320937469335541,2.12933252157952,
7.87225779812213));
#47526=CARTESIAN_POINT('Ctrl Pts',(-0.320911533849697,2.12961492004832,
7.87224012569037));
#47527=CARTESIAN_POINT('Ctrl Pts',(-0.320866077205716,2.13010280265549,
7.87220962688306));
#47528=CARTESIAN_POINT('Ctrl Pts',(-0.320846731384682,2.13030830231822,
7.87219679061606));
#47529=CARTESIAN_POINT('Ctrl Pts',(-0.320806094279767,2.13073556784925,
7.87217012313495));
#47530=CARTESIAN_POINT('Ctrl Pts',(-0.320784770493705,2.13095732994989,
7.87215629385888));
#47531=CARTESIAN_POINT('Ctrl Pts',(-0.320733634342674,2.13148340709602,
7.87212351501082));
#47532=CARTESIAN_POINT('Ctrl Pts',(-0.320703618702171,2.13178770319188,
7.87210457695863));
#47533=CARTESIAN_POINT('Ctrl Pts',(-0.320602332856928,2.13279978395838,
7.87204166148262));
#47534=CARTESIAN_POINT('Ctrl Pts',(-0.320529151641634,2.13350738174752,
7.87199779117199));
#47535=CARTESIAN_POINT('Ctrl Pts',(-0.319263965687572,2.14535705344153,
7.87126500036173));
#47536=CARTESIAN_POINT('Ctrl Pts',(-0.317493822310917,2.15643117280002,
7.87060789502809));
#47537=CARTESIAN_POINT('Ctrl Pts',(-0.311051974490813,2.1865557332177,7.86884240183433));
#47538=CARTESIAN_POINT('Ctrl Pts',(-0.305214368565636,2.20530663398111,
7.86776609413679));
#47539=CARTESIAN_POINT('Ctrl Pts',(-0.290272041468378,2.24135238093017,
7.86556628450477));
#47540=CARTESIAN_POINT('Ctrl Pts',(-0.28122973353486,2.2585812752271,7.86444722091061));
#47541=CARTESIAN_POINT('Ctrl Pts',(-0.269990992051644,2.27597645382458,
7.86318932760815));
#47542=CARTESIAN_POINT('Ctrl Pts',(-0.269282661703714,2.27705845396168,
7.86311053822641));
#47543=CARTESIAN_POINT('Ctrl Pts',(-0.268285555485195,2.27856174608138,
7.86300029409817));
#47544=CARTESIAN_POINT('Ctrl Pts',(-0.268002254918617,2.27898666933443,
7.86296904508655));
#47545=CARTESIAN_POINT('Ctrl Pts',(-0.267511252695481,2.27971934553032,
7.86291501218814));
#47546=CARTESIAN_POINT('Ctrl Pts',(-0.267304026441358,2.28002741714227,
7.86289224625872));
#47547=CARTESIAN_POINT('Ctrl Pts',(-0.266873969698084,2.28066437873853,
7.86284507929959));
#47548=CARTESIAN_POINT('Ctrl Pts',(-0.266651062603541,2.28099321605406,
7.86282067539631));
#47549=CARTESIAN_POINT('Ctrl Pts',(-0.266128598902884,2.28176090557921,
7.86276357736239));
#47550=CARTESIAN_POINT('Ctrl Pts',(-0.265828564530426,2.28219942981603,
7.86273086513824));
#47551=CARTESIAN_POINT('Ctrl Pts',(-0.264859935705621,2.28360767265562,
7.86262550376776));
#47552=CARTESIAN_POINT('Ctrl Pts',(-0.264187114821185,2.28457446005182,
7.86255269376736));
#47553=CARTESIAN_POINT('Ctrl Pts',(-0.262610733758786,2.28681330967597,
7.86238295917557));
#47554=CARTESIAN_POINT('Ctrl Pts',(-0.261703211062829,2.28808253331707,
7.86228588335337));
#47555=CARTESIAN_POINT('Ctrl Pts',(-0.252244973159093,2.3011094400684,7.86128060590163));
#47556=CARTESIAN_POINT('Ctrl Pts',(-0.242918415110829,2.31228064449698,
7.86034188266902));
#47557=CARTESIAN_POINT('Ctrl Pts',(-0.211466585408964,2.34515664796652,
7.85732973503402));
#47558=CARTESIAN_POINT('Ctrl Pts',(-0.186952015504273,2.36432682548592,
7.85517309581899));
#47559=CARTESIAN_POINT('Ctrl Pts',(-0.156952016439864,2.38149642729502,
7.85295107799569));
#47560=CARTESIAN_POINT('Ctrl Pts',(-0.15379291719028,2.38323473544812,7.85272196742056));
#47561=CARTESIAN_POINT('Ctrl Pts',(-0.150096099100366,2.38518882902178,
7.85246004215881));
#47562=CARTESIAN_POINT('Ctrl Pts',(-0.149586320936729,2.38545654619357,
7.85242405836527));
#47563=CARTESIAN_POINT('Ctrl Pts',(-0.148827226456137,2.38585260347645,
7.85237067927247));
#47564=CARTESIAN_POINT('Ctrl Pts',(-0.148578459258549,2.38598198491283,
7.85235321846998));
#47565=CARTESIAN_POINT('Ctrl Pts',(-0.148135096729644,2.3862118388593,7.85232215718805));
#47566=CARTESIAN_POINT('Ctrl Pts',(-0.147940567961566,2.38631243762472,
7.85230854869031));
#47567=CARTESIAN_POINT('Ctrl Pts',(-0.147527390943119,2.38652557480514,
7.85227968668254));
#47568=CARTESIAN_POINT('Ctrl Pts',(-0.147308717014252,2.38663806095577,
7.85226443652256));
#47569=CARTESIAN_POINT('Ctrl Pts',(-0.146721699348348,2.38693917442856,
7.85222356495147));
#47570=CARTESIAN_POINT('Ctrl Pts',(-0.146353119119047,2.38712734354304,
7.8521979725338));
#47571=CARTESIAN_POINT('Ctrl Pts',(-0.14458755156591,2.38802442548806,7.85207571120106));
#47572=CARTESIAN_POINT('Ctrl Pts',(-0.143185739294593,2.3887238716172,7.85197962949085));
#47573=CARTESIAN_POINT('Ctrl Pts',(-0.131518960131977,2.39443924045445,
7.85118770091166));
#47574=CARTESIAN_POINT('Ctrl Pts',(-0.120997805956815,2.39891687007916,
7.85052279783495));
#47575=CARTESIAN_POINT('Ctrl Pts',(-0.0787653261399857,2.41429381830125,
7.8479604802253));
#47576=CARTESIAN_POINT('Ctrl Pts',(-0.0456767017644045,2.42077771202408,
7.84615748053733));
#47577=CARTESIAN_POINT('Ctrl Pts',(-0.0114046110692441,2.42207408320491,
7.84411523672295));
#47578=CARTESIAN_POINT('Ctrl Pts',(-0.0106275070147806,2.42210066175847,
7.84406885376787));
#47579=CARTESIAN_POINT('Ctrl Pts',(-0.0091320901766239,2.42214639046467,
7.8439794461186));
#47580=CARTESIAN_POINT('Ctrl Pts',(-0.00841379395454737,2.42216595105535,
7.84393643385516));
#47581=CARTESIAN_POINT('Ctrl Pts',(-0.00509858566691138,2.4222451358241,
7.84373759889337));
#47582=CARTESIAN_POINT('Ctrl Pts',(-0.00250113361318201,2.42227576215142,
7.8435809134893));
#47583=CARTESIAN_POINT('Ctrl Pts',(0.00148793349062841,2.42227456956377,
7.84333878550451));
#47584=CARTESIAN_POINT('Ctrl Pts',(0.00287948367095603,2.42226514023795,
7.84325404188193));
#47585=CARTESIAN_POINT('Ctrl Pts',(0.00479782112107145,2.42223971545906,
7.84313681858831));
#47586=CARTESIAN_POINT('Ctrl Pts',(0.00532470950535287,2.4222314397605,
7.84310458067905));
#47587=CARTESIAN_POINT('Ctrl Pts',(0.00622710974699833,2.42221505210609,
7.84304929498346));
#47588=CARTESIAN_POINT('Ctrl Pts',(0.00660263325183739,2.42220757584473,
7.84302626714191));
#47589=CARTESIAN_POINT('Ctrl Pts',(0.00737308272021299,2.42219088957926,
7.84297897753579));
#47590=CARTESIAN_POINT('Ctrl Pts',(0.00776800642997994,2.42218160988892,
7.84295471362583));
#47591=CARTESIAN_POINT('Ctrl Pts',(0.00867961107137652,2.42215851242409,
7.84289864973776));
#47592=CARTESIAN_POINT('Ctrl Pts',(0.00919627676571361,2.42214417775949,
7.84286683361891));
#47593=CARTESIAN_POINT('Ctrl Pts',(0.0108134490212011,2.422095416371,7.84276711879866));
#47594=CARTESIAN_POINT('Ctrl Pts',(0.0119138062860855,2.42205659300582,
7.84269908251303));
#47595=CARTESIAN_POINT('Ctrl Pts',(0.0275545387255845,2.42142448194293,
7.84172927021112));
#47596=CARTESIAN_POINT('Ctrl Pts',(0.0420364847399454,2.41985274197984,
7.84079658266717));
#47597=CARTESIAN_POINT('Ctrl Pts',(0.0889056384387882,2.41152773410653,
7.83766175515394));
#47598=CARTESIAN_POINT('Ctrl Pts',(0.120362751052646,2.40077605220694,7.83535117881836));
#47599=CARTESIAN_POINT('Ctrl Pts',(0.152485647198109,2.38393603584016,7.83302589136675));
#47600=CARTESIAN_POINT('Ctrl Pts',(0.155315231038123,2.38239816926301,7.83282161463496));
#47601=CARTESIAN_POINT('Ctrl Pts',(0.15860006563939,2.38054856361472,7.83258553873825));
#47602=CARTESIAN_POINT('Ctrl Pts',(0.159078028161934,2.38027782347842,7.83255121508975));
#47603=CARTESIAN_POINT('Ctrl Pts',(0.159797559024813,2.37986781433505,7.83249958697359));
#47604=CARTESIAN_POINT('Ctrl Pts',(0.160039639597334,2.37972945345446,7.83248222447836));
#47605=CARTESIAN_POINT('Ctrl Pts',(0.160471388037626,2.37948194419821,7.83245127224259));
#47606=CARTESIAN_POINT('Ctrl Pts',(0.160661124128403,2.37937291691641,7.83243767469911));
#47607=CARTESIAN_POINT('Ctrl Pts',(0.161064657112157,2.37914048934187,7.83240876543298));
#47608=CARTESIAN_POINT('Ctrl Pts',(0.161278422692253,2.37901703699873,7.83239345720409));
#47609=CARTESIAN_POINT('Ctrl Pts',(0.161846567929465,2.37868805482285,7.83235278651482));
#47610=CARTESIAN_POINT('Ctrl Pts',(0.162200699358362,2.37848209382931,7.83232745202431));
#47611=CARTESIAN_POINT('Ctrl Pts',(0.16387747713634,2.3775026051066,7.83220756699285));
#47612=CARTESIAN_POINT('Ctrl Pts',(0.165195017150495,2.37672030984514,7.83211357715743));
#47613=CARTESIAN_POINT('Ctrl Pts',(0.175953208509584,2.37022836400244,7.83134742632148));
#47614=CARTESIAN_POINT('Ctrl Pts',(0.185101634170977,2.36404609661573,7.8307041494326));
#47615=CARTESIAN_POINT('Ctrl Pts',(0.213256392276101,2.34283581956301,7.82869121814771));
#47616=CARTESIAN_POINT('Ctrl Pts',(0.230893448297282,2.32613231349738,7.82737263657334));
#47617=CARTESIAN_POINT('Ctrl Pts',(0.250508229107794,2.30284387645286,7.82562952772105));
#47618=CARTESIAN_POINT('Ctrl Pts',(0.254383502849539,2.2979622145223,7.82526908205368));
#47619=CARTESIAN_POINT('Ctrl Pts',(0.259126448953529,2.29161814689843,7.82480458479692));
#47620=CARTESIAN_POINT('Ctrl Pts',(0.260127543554704,2.290256909749,7.82470514305407));
#47621=CARTESIAN_POINT('Ctrl Pts',(0.264888924039722,2.28367479578576,7.82422523863973));
#47622=CARTESIAN_POINT('Ctrl Pts',(0.268502793292778,2.27835025618281,7.82383978787106));
#47623=CARTESIAN_POINT('Ctrl Pts',(0.272507207444315,2.27205248551882,7.82338555750276));
#47624=CARTESIAN_POINT('Ctrl Pts',(0.273055529071874,2.27118093902943,7.82332273406909));
#47625=CARTESIAN_POINT('Ctrl Pts',(0.273865413876963,2.2698798505051,7.82322899771151));
#47626=CARTESIAN_POINT('Ctrl Pts',(0.27413016729602,2.26945229387459,7.82319820251538));
#47627=CARTESIAN_POINT('Ctrl Pts',(0.274600124939966,2.26868936419242,7.82314326510158));
#47628=CARTESIAN_POINT('Ctrl Pts',(0.274805718675819,2.26835423127911,7.82311913726494));
#47629=CARTESIAN_POINT('Ctrl Pts',(0.275237426062742,2.26764761866576,7.82306827403339));
#47630=CARTESIAN_POINT('Ctrl Pts',(0.275463401936569,2.2672760560885,7.82304153365009));
#47631=CARTESIAN_POINT('Ctrl Pts',(0.276057348758979,2.2662949870648,7.82297094211839));
#47632=CARTESIAN_POINT('Ctrl Pts',(0.276424051678866,2.26568471917216,7.82292704472378));
#47633=CARTESIAN_POINT('Ctrl Pts',(0.278035297684738,2.26298304131534,7.82273276488769));
#47634=CARTESIAN_POINT('Ctrl Pts',(0.279258123269032,2.26087883198473,7.82258159514348));
#47635=CARTESIAN_POINT('Ctrl Pts',(0.288030838082574,2.24538152012065,7.82146905131287));
#47636=CARTESIAN_POINT('Ctrl Pts',(0.294636451811711,2.23147923092952,7.82047393843302));
#47637=CARTESIAN_POINT('Ctrl Pts',(0.308967308678145,2.19475633390234,7.81785692729135));
#47638=CARTESIAN_POINT('Ctrl Pts',(0.315174460220739,2.17144588057499,7.81620222464014));
#47639=CARTESIAN_POINT('Ctrl Pts',(0.319342237946461,2.14357515414677,7.81433518532233));
#47640=CARTESIAN_POINT('Ctrl Pts',(0.319874849284993,2.13947584845354,7.81406354140369));
#47641=CARTESIAN_POINT('Ctrl Pts',(0.320442326152691,2.13433609640617,7.81372751935797));
#47642=CARTESIAN_POINT('Ctrl Pts',(0.320551198992344,2.13330436585477,7.81366029756568));
#47643=CARTESIAN_POINT('Ctrl Pts',(0.321089447693236,2.12795633749529,7.81331309910152));
#47644=CARTESIAN_POINT('Ctrl Pts',(0.321436658164977,2.12363196151648,7.81303656585807));
#47645=CARTESIAN_POINT('Ctrl Pts',(0.32173240778931,2.11870276309451,7.81272712705058));
#47646=CARTESIAN_POINT('Ctrl Pts',(0.321766668059672,2.11810378161634,7.81268962187897));
#47647=CARTESIAN_POINT('Ctrl Pts',(0.321814809025999,2.11721877786667,7.81263435407362));
#47648=CARTESIAN_POINT('Ctrl Pts',(0.321829981259079,2.11693283154018,7.81261651955036));
#47649=CARTESIAN_POINT('Ctrl Pts',(0.32185615801111,2.11642673917481,7.81258499493885));
#47650=CARTESIAN_POINT('Ctrl Pts',(0.321867317800919,2.1162066018156,7.81257129608775));
#47651=CARTESIAN_POINT('Ctrl Pts',(0.321890169427502,2.1157464971031,7.81254269289034));
#47652=CARTESIAN_POINT('Ctrl Pts',(0.321901818751774,2.11550652863439,7.81252779099392));
#47653=CARTESIAN_POINT('Ctrl Pts',(0.321931237283365,2.11488620407804,7.81248931045475));
#47654=CARTESIAN_POINT('Ctrl Pts',(0.321948600829022,2.1145058277403,7.81246575467461));
#47655=CARTESIAN_POINT('Ctrl Pts',(0.322019912069162,2.11288040736809,7.8123652641658));
#47656=CARTESIAN_POINT('Ctrl Pts',(0.322067312896367,2.11163506534729,7.81228869239922));
#47657=CARTESIAN_POINT('Ctrl Pts',(0.322358024204151,2.10262205350728,7.81173735516827));
#47658=CARTESIAN_POINT('Ctrl Pts',(0.322327541151314,2.09484740359178,7.81127702313948));
#47659=CARTESIAN_POINT('Ctrl Pts',(0.321193541598255,2.06658206212645,7.80963461122789));
#47660=CARTESIAN_POINT('Ctrl Pts',(0.318415639706246,2.0462072741071,7.80850787964424));
#47661=CARTESIAN_POINT('Ctrl Pts',(0.30886144148997,2.00557443408854,7.80616293623721));
#47662=CARTESIAN_POINT('Ctrl Pts',(0.301975871178473,1.98544892950335,7.80494729352734));
#47663=CARTESIAN_POINT('Ctrl Pts',(0.29262343557792,1.96496522569044,7.80357965753719));
#47664=CARTESIAN_POINT('Ctrl Pts',(0.292076404651883,1.96378605397924,7.80350046569507));
#47665=CARTESIAN_POINT('Ctrl Pts',(0.291304061465788,1.96214724750963,7.80338974831441));
#47666=CARTESIAN_POINT('Ctrl Pts',(0.291084760153022,1.96168478031134,7.8033584308546));
#47667=CARTESIAN_POINT('Ctrl Pts',(0.290704351213278,1.96088747762754,7.80330431151757));
#47668=CARTESIAN_POINT('Ctrl Pts',(0.290543764013779,1.96055239376027,7.80328152773345));
#47669=CARTESIAN_POINT('Ctrl Pts',(0.290210364532327,1.95985979297222,7.80323435385998));
#47670=CARTESIAN_POINT('Ctrl Pts',(0.290037470330294,1.95950231635369,7.80320996094933));
#47671=CARTESIAN_POINT('Ctrl Pts',(0.289632157402543,1.95866822649327,7.80315294062472));
#47672=CARTESIAN_POINT('Ctrl Pts',(0.289399222685224,1.958191866566,7.80312029526398));
#47673=CARTESIAN_POINT('Ctrl Pts',(0.288661173058712,1.95669192044654,7.80301724783825));
#47674=CARTESIAN_POINT('Ctrl Pts',(0.288151799398091,1.95567045019522,7.80294669705111));
#47675=CARTESIAN_POINT('Ctrl Pts',(0.277433365328805,1.9344592027054,7.80147376874622));
#47676=CARTESIAN_POINT('Ctrl Pts',(0.265134044538047,1.91540156826889,7.7999937643473));
#47677=CARTESIAN_POINT('Ctrl Pts',(0.241190608143404,1.88568735815783,7.79742737684056));
#47678=CARTESIAN_POINT('Ctrl Pts',(0.230574289135217,1.87430482335346,7.79636776524988));
#47679=CARTESIAN_POINT('Ctrl Pts',(0.215579665281473,1.86039475149057,7.79499943926648));
#47680=CARTESIAN_POINT('Ctrl Pts',(0.21190533034636,1.85713913050409,7.79467331343826));
#47681=CARTESIAN_POINT('Ctrl Pts',(0.206941185223378,1.85293915387112,7.79424607118036));
#47682=CARTESIAN_POINT('Ctrl Pts',(0.205716802756097,1.85191873696992,7.79414173770608));
#47683=CARTESIAN_POINT('Ctrl Pts',(0.203821834602831,1.85036312118565,7.79398191917302));
#47684=CARTESIAN_POINT('Ctrl Pts',(0.203156611486783,1.84982145822758,7.79392612561931));
#47685=CARTESIAN_POINT('Ctrl Pts',(0.198555301630045,1.84610526171244,7.79354238142064));
#47686=CARTESIAN_POINT('Ctrl Pts',(0.194546861882251,1.84302087326813,7.79321900835275));
#47687=CARTESIAN_POINT('Ctrl Pts',(0.189955585531988,1.83965704649889,7.79286222943857));
#47688=CARTESIAN_POINT('Ctrl Pts',(0.189442838143511,1.83928370015503,7.79282257190303));
#47689=CARTESIAN_POINT('Ctrl Pts',(0.188695186450588,1.83874268331621,7.79276502173149));
#47690=CARTESIAN_POINT('Ctrl Pts',(0.188461157912089,1.83857381372472,7.79274704661614));
#47691=CARTESIAN_POINT('Ctrl Pts',(0.188047701791405,1.8382763170549,7.79271535960726));
#47692=CARTESIAN_POINT('Ctrl Pts',(0.187868368622466,1.83814755980572,7.79270163864908));
#47693=CARTESIAN_POINT('Ctrl Pts',(0.187494445363039,1.8378796730423,7.79267307751555));
#47694=CARTESIAN_POINT('Ctrl Pts',(0.187299833058516,1.8377405761778,7.79265823961578));
#47695=CARTESIAN_POINT('Ctrl Pts',(0.186798742204781,1.83738326961243,7.79262010377106));
#47696=CARTESIAN_POINT('Ctrl Pts',(0.186492035004327,1.83716537889367,7.79259682792221));
#47697=CARTESIAN_POINT('Ctrl Pts',(0.185199766979882,1.83625072751848,7.7924990338178));
#47698=CARTESIAN_POINT('Ctrl Pts',(0.184210661079955,1.83555895765477,7.79242485472668));
#47699=CARTESIAN_POINT('Ctrl Pts',(0.181638965088731,1.8337817727217,7.79223365772499));
#47700=CARTESIAN_POINT('Ctrl Pts',(0.180050500735718,1.83270489013688,7.79211718438396));
#47701=CARTESIAN_POINT('Ctrl Pts',(0.173279097251479,1.82820204424906,7.79162708281972));
#47702=CARTESIAN_POINT('Ctrl Pts',(0.168006968349553,1.82491193524463,7.79126124294117));
#47703=CARTESIAN_POINT('Ctrl Pts',(0.148814489564583,1.81369249653791,7.78997259269385));
#47704=CARTESIAN_POINT('Ctrl Pts',(0.134401953137314,1.80665050933854,7.78908277337192));
#47705=CARTESIAN_POINT('Ctrl Pts',(0.107807982682133,1.79602995155379,7.78748154422638));
#47706=CARTESIAN_POINT('Ctrl Pts',(0.095827080469099,1.79204302629998,7.78677393003545));
#47707=CARTESIAN_POINT('Ctrl Pts',(0.0831665505998361,1.78864048950478,
7.78602043641045));
#47708=CARTESIAN_POINT('Ctrl Pts',(0.0826889382886714,1.78851330783432,
7.78599200376236));
#47709=CARTESIAN_POINT('Ctrl Pts',(0.0781513405067462,1.78731617906237,
7.78572179722553));
#47710=CARTESIAN_POINT('Ctrl Pts',(0.0740712218140315,1.78632460083417,
7.78547822022259));
#47711=CARTESIAN_POINT('Ctrl Pts',(0.068162845360006,1.78501041139755,7.78512387540157));
#47712=CARTESIAN_POINT('Ctrl Pts',(0.0663492696363843,1.78462341772982,
7.78501489174729));
#47713=CARTESIAN_POINT('Ctrl Pts',(0.0580182189914081,1.78292071959369,
7.78451307846395));
#47714=CARTESIAN_POINT('Ctrl Pts',(0.0514647109437782,1.78179133002675,
7.78411500331623));
#47715=CARTESIAN_POINT('Ctrl Pts',(0.0438517848115576,1.78072069052314,
7.78364712664919));
#47716=CARTESIAN_POINT('Ctrl Pts',(0.0428215837490908,1.78058088908663,
7.7835836988295));
#47717=CARTESIAN_POINT('Ctrl Pts',(0.0412901229764387,1.7803806071797,7.78348923474597));
#47718=CARTESIAN_POINT('Ctrl Pts',(0.0407893614334045,1.78031631491192,
7.7834583189227));
#47719=CARTESIAN_POINT('Ctrl Pts',(0.0398981248011359,1.7802040181031,7.78340324610236));
#47720=CARTESIAN_POINT('Ctrl Pts',(0.0395077081308421,1.78015555125011,
7.78337910374955));
#47721=CARTESIAN_POINT('Ctrl Pts',(0.0386865863317237,1.78005514245692,
7.78332829144348));
#47722=CARTESIAN_POINT('Ctrl Pts',(0.0382558634025644,1.78000335510719,
7.78330161666375));
#47723=CARTESIAN_POINT('Ctrl Pts',(0.037122686434553,1.77986942981624,7.78323138293221));
#47724=CARTESIAN_POINT('Ctrl Pts',(0.0364200671591778,1.77978873456782,
7.78318777857784));
#47725=CARTESIAN_POINT('Ctrl Pts',(0.0333332740169484,1.77944450993963,
7.78299596113615));
#47726=CARTESIAN_POINT('Ctrl Pts',(0.0309465155826444,1.77920529611985,
7.78284698432698));
#47727=CARTESIAN_POINT('Ctrl Pts',(0.0167979750887183,1.77794661748474,
7.78195975887065));
#47728=CARTESIAN_POINT('Ctrl Pts',(0.00499137278360443,1.77754755055566,
7.78120213407256));
#47729=CARTESIAN_POINT('Ctrl Pts',(-0.0257814858978446,1.77819789996264,
7.7791821709975));
#47730=CARTESIAN_POINT('Ctrl Pts',(-0.0446796350378662,1.78027373916416,
7.77789484631387));
#47731=CARTESIAN_POINT('Ctrl Pts',(-0.0778640185065421,1.78691934844391,
7.77560742949979));
#47732=CARTESIAN_POINT('Ctrl Pts',(-0.0922267060310288,1.79084530901711,
7.77460903173696));
#47733=CARTESIAN_POINT('Ctrl Pts',(-0.10945807921497,1.79686385551595,7.77343754464171));
#47734=CARTESIAN_POINT('Ctrl Pts',(-0.112630522582811,1.79802821188475,
7.77322303686281));
#47735=CARTESIAN_POINT('Ctrl Pts',(-0.116311044104446,1.799445120942,7.77297603392202));
#47736=CARTESIAN_POINT('Ctrl Pts',(-0.116837342481726,1.79964932209244,
7.77294075833967));
#47737=CARTESIAN_POINT('Ctrl Pts',(-0.117622149121257,1.79995619815735,
7.77288822583045));
#47738=CARTESIAN_POINT('Ctrl Pts',(-0.117881061867879,1.80005782516892,
7.77287090638192));
#47739=CARTESIAN_POINT('Ctrl Pts',(-0.118343373540004,1.80023998028533,
7.77284000170296));
#47740=CARTESIAN_POINT('Ctrl Pts',(-0.118546821825374,1.80032038021194,
7.77282640876402));
#47741=CARTESIAN_POINT('Ctrl Pts',(-0.118980067191222,1.8004921029728,7.77279747789632));
#47742=CARTESIAN_POINT('Ctrl Pts',(-0.119209840400209,1.80058348288175,
7.77278214352556));
#47743=CARTESIAN_POINT('Ctrl Pts',(-0.119678695294262,1.80077056990174,
7.77275087194513));
#47744=CARTESIAN_POINT('Ctrl Pts',(-0.119917767958958,1.80086629933572,
7.77273493609914));
#47745=CARTESIAN_POINT('Ctrl Pts',(-0.120993186746647,1.80129841477808,
7.77266329488608));
#47746=CARTESIAN_POINT('Ctrl Pts',(-0.121828244761371,1.80163802675737,
7.77260778261008));
#47747=CARTESIAN_POINT('Ctrl Pts',(-0.123881823364054,1.80248326122163,
7.772471528839));
#47748=CARTESIAN_POINT('Ctrl Pts',(-0.125098697203112,1.80299287532788,
7.77239101835187));
#47749=CARTESIAN_POINT('Ctrl Pts',(-0.129775397177239,1.80498527054054,
7.77208235476825));
#47750=CARTESIAN_POINT('Ctrl Pts',(-0.133212416317876,1.80652121177343,
7.77185710908267));
#47751=CARTESIAN_POINT('Ctrl Pts',(-0.144854536844566,1.81197054956875,
7.77109703406402));
#47752=CARTESIAN_POINT('Ctrl Pts',(-0.152921085902793,1.8161708845498,7.77057531927611));
#47753=CARTESIAN_POINT('Ctrl Pts',(-0.167594311899711,1.82461882649015,
7.76961642600287));
#47754=CARTESIAN_POINT('Ctrl Pts',(-0.17424398551058,1.82877742907326,7.76917782360765));
#47755=CARTESIAN_POINT('Ctrl Pts',(-0.203386322053105,1.84851712571542,
7.76721017529219));
#47756=CARTESIAN_POINT('Ctrl Pts',(-0.223987804625232,1.86667868438678,
7.76568090521249));
#47757=CARTESIAN_POINT('Ctrl Pts',(-0.24318432273746,1.88851589594493,7.76391988439744));
#47758=CARTESIAN_POINT('Ctrl Pts',(-0.244310881627447,1.88981833088322,
7.76381516093574));
#47759=CARTESIAN_POINT('Ctrl Pts',(-0.245841954379403,1.89161737320788,
7.76367090161053));
#47760=CARTESIAN_POINT('Ctrl Pts',(-0.246255520541489,1.89210626686843,
7.76363173832799));
#47761=CARTESIAN_POINT('Ctrl Pts',(-0.246910299660286,1.89288500359133,
7.76356941807465));
#47762=CARTESIAN_POINT('Ctrl Pts',(-0.2471524672449,1.89317404479008,7.76354630018665));
#47763=CARTESIAN_POINT('Ctrl Pts',(-0.24762161709205,1.8937360031932,7.76350137950916));
#47764=CARTESIAN_POINT('Ctrl Pts',(-0.247848656937928,1.89400887183544,
7.76347957910988));
#47765=CARTESIAN_POINT('Ctrl Pts',(-0.248389082951357,1.89466057168666,
7.7634275399302));
#47766=CARTESIAN_POINT('Ctrl Pts',(-0.248702053249451,1.89503974518287,
7.76339728432509));
#47767=CARTESIAN_POINT('Ctrl Pts',(-0.249632530575102,1.89617231731244,
7.76330697660469));
#47768=CARTESIAN_POINT('Ctrl Pts',(-0.250247486510243,1.89692779605999,
7.76324682154055));
#47769=CARTESIAN_POINT('Ctrl Pts',(-0.254626095356384,1.9023570480641,7.76281510071163));
#47770=CARTESIAN_POINT('Ctrl Pts',(-0.25826177073284,1.90713207926455,7.76243845132368));
#47771=CARTESIAN_POINT('Ctrl Pts',(-0.270341435707547,1.92395170213854,
7.76112079081288));
#47772=CARTESIAN_POINT('Ctrl Pts',(-0.278092077954107,1.9364695980472,7.76015454211314));
#47773=CARTESIAN_POINT('Ctrl Pts',(-0.287404480967353,1.95409858011864,
7.75881948955918));
#47774=CARTESIAN_POINT('Ctrl Pts',(-0.289735606609377,1.95878443393202,
7.75846707721003));
#47775=CARTESIAN_POINT('Ctrl Pts',(-0.293054948665906,1.9658852669772,7.75793768164209));
#47776=CARTESIAN_POINT('Ctrl Pts',(-0.294129664125993,1.96825894671478,
7.75776147727899));
#47777=CARTESIAN_POINT('Ctrl Pts',(-0.296410399793889,1.97346337827838,
7.75737702106168));
#47778=CARTESIAN_POINT('Ctrl Pts',(-0.297604909631107,1.97629891056668,
7.75716875407674));
#47779=CARTESIAN_POINT('Ctrl Pts',(-0.30573389346498,1.99639511638255,7.75570246028156));
#47780=CARTESIAN_POINT('Ctrl Pts',(-0.311204040011075,2.01421299714702,
7.75445062100555));
#47781=CARTESIAN_POINT('Ctrl Pts',(-0.31533074080164,2.03345045320751,7.75321125411676));
#47782=CARTESIAN_POINT('Ctrl Pts',(-0.315549746591385,2.03449674988814,
7.75314419601279));
#47783=CARTESIAN_POINT('Ctrl Pts',(-0.315838129484753,2.03590951199907,
7.75305413930554));
#47784=CARTESIAN_POINT('Ctrl Pts',(-0.315912079169682,2.03627502117175,
7.7530308839035));
#47785=CARTESIAN_POINT('Ctrl Pts',(-0.316027294024683,2.03684962014129,
7.7529943952908));
#47786=CARTESIAN_POINT('Ctrl Pts',(-0.316068986202367,2.03705862246095,
7.75298113762487));
#47787=CARTESIAN_POINT('Ctrl Pts',(-0.316148915213874,2.03746138760873,
7.75295561722452));
#47788=CARTESIAN_POINT('Ctrl Pts',(-0.316187180965619,2.03765514276249,
7.75294335293531));
#47789=CARTESIAN_POINT('Ctrl Pts',(-0.316265905696554,2.03805569501419,
7.75291802476659));
#47790=CARTESIAN_POINT('Ctrl Pts',(-0.316306339842971,2.03826249598511,
7.75290496236235));
#47791=CARTESIAN_POINT('Ctrl Pts',(-0.316397511664129,2.03873123614969,
7.75287538681526));
#47792=CARTESIAN_POINT('Ctrl Pts',(-0.316448127018677,2.03899319940705,
7.75285888067552));
#47793=CARTESIAN_POINT('Ctrl Pts',(-0.31657558598801,2.03965729871342,7.75281709289158));
#47794=CARTESIAN_POINT('Ctrl Pts',(-0.316651989016194,2.04005952036704,
7.75279183615509));
#47795=CARTESIAN_POINT('Ctrl Pts',(-0.316868191400554,2.04120966213146,
7.75271976285643));
#47796=CARTESIAN_POINT('Ctrl Pts',(-0.317006109978373,2.04195793929017,
7.75267305061626));
#47797=CARTESIAN_POINT('Ctrl Pts',(-0.320539387253856,2.0615160473925,7.75145659810435));
#47798=CARTESIAN_POINT('Ctrl Pts',(-0.322257763038556,2.08059297725488,
7.75037734620028));
#47799=CARTESIAN_POINT('Ctrl Pts',(-0.32227487097392,2.09971161875376,7.74930651681519));
#47800=CARTESIAN_POINT('',(-0.32227487212353,2.10029338639761,7.49935789418026));
#47801=CARTESIAN_POINT('Ctrl Pts',(-0.322274870797116,2.09971142123794,
7.74930652787799));
#47802=CARTESIAN_POINT('Ctrl Pts',(-0.322301050256033,2.12894774368805,
7.7476690100838));
#47803=CARTESIAN_POINT('Ctrl Pts',(-0.318349214822576,2.15804910749707,
7.74605150154093));
#47804=CARTESIAN_POINT('Ctrl Pts',(-0.310113917334948,2.18770931960783,
7.74419354706404));
#47805=CARTESIAN_POINT('Ctrl Pts',(-0.30968953566173,2.18919617617591,7.74409988129185));
#47806=CARTESIAN_POINT('Ctrl Pts',(-0.309027553797149,2.19145379722797,
7.74395683415946));
#47807=CARTESIAN_POINT('Ctrl Pts',(-0.308797728825796,2.1922268327919,7.74390770512513));
#47808=CARTESIAN_POINT('Ctrl Pts',(-0.308365837219326,2.19365982290545,
7.74381635512585));
#47809=CARTESIAN_POINT('Ctrl Pts',(-0.308164547040277,2.19432000809183,
7.74377415967596));
#47810=CARTESIAN_POINT('Ctrl Pts',(-0.307834406928609,2.19539045260446,
7.74370556200655));
#47811=CARTESIAN_POINT('Ctrl Pts',(-0.307706853144732,2.19580111200868,
7.74367920232366));
#47812=CARTESIAN_POINT('Ctrl Pts',(-0.307460730257454,2.19658794198916,
7.74362861327715));
#47813=CARTESIAN_POINT('Ctrl Pts',(-0.307342291671044,2.19696415284186,
7.74360438823824));
#47814=CARTESIAN_POINT('Ctrl Pts',(-0.307070938927745,2.19782059135435,
7.74354915632064));
#47815=CARTESIAN_POINT('Ctrl Pts',(-0.306917588571903,2.1983006787743,7.74351813514352));
#47816=CARTESIAN_POINT('Ctrl Pts',(-0.306437332376391,2.19979211717981,
7.74342157625674));
#47817=CARTESIAN_POINT('Ctrl Pts',(-0.306106551526138,2.20080220431422,
7.7433559110671));
#47818=CARTESIAN_POINT('Ctrl Pts',(-0.303503738106729,2.20861930868389,
7.74284560374043));
#47819=CARTESIAN_POINT('Ctrl Pts',(-0.30101007300084,2.21534988466393,7.74239365819215));
#47820=CARTESIAN_POINT('Ctrl Pts',(-0.289540160427978,2.24339621664072,
7.74045450421555));
#47821=CARTESIAN_POINT('Ctrl Pts',(-0.278509062640986,2.26379363343003,
7.73889819641893));
#47822=CARTESIAN_POINT('Ctrl Pts',(-0.261344909783403,2.28870861029079,
7.73685087185366));
#47823=CARTESIAN_POINT('Ctrl Pts',(-0.257102249814327,2.29444932126274,
7.73636836253759));
#47824=CARTESIAN_POINT('Ctrl Pts',(-0.246959242325551,2.3072607599163,7.73527271011933));
#47825=CARTESIAN_POINT('Ctrl Pts',(-0.240939051096981,2.31422952870395,
7.73466265478897));
#47826=CARTESIAN_POINT('Ctrl Pts',(-0.231746745709577,2.32399171840051,
7.73379767694872));
#47827=CARTESIAN_POINT('Ctrl Pts',(-0.228805399025349,2.32699545733285,
7.73353000558546));
#47828=CARTESIAN_POINT('Ctrl Pts',(-0.225529287577843,2.33021265480593,
7.73324247882924));
#47829=CARTESIAN_POINT('Ctrl Pts',(-0.225252126764099,2.33048385058421,
7.73321823497732));
#47830=CARTESIAN_POINT('Ctrl Pts',(-0.224789930044353,2.33093446993655,
7.73317794141341));
#47831=CARTESIAN_POINT('Ctrl Pts',(-0.224605168099941,2.33111417204084,
7.73316187013503));
#47832=CARTESIAN_POINT('Ctrl Pts',(-0.224242614408547,2.33146595155246,
7.73313040465807));
#47833=CARTESIAN_POINT('Ctrl Pts',(-0.224064839725677,2.33163804619398,
7.73311500911103));
#47834=CARTESIAN_POINT('Ctrl Pts',(-0.22372953212983,2.33196189325583,7.73308603386103));
#47835=CARTESIAN_POINT('Ctrl Pts',(-0.223572044189869,2.33211368879702,
7.73307245079983));
#47836=CARTESIAN_POINT('Ctrl Pts',(-0.223214115221895,2.33245797818098,
7.73304163905084));
#47837=CARTESIAN_POINT('Ctrl Pts',(-0.223013580060107,2.33265037280101,
7.73302441817162));
#47838=CARTESIAN_POINT('Ctrl Pts',(-0.222405796373231,2.33323197614759,
7.73297235064468));
#47839=CARTESIAN_POINT('Ctrl Pts',(-0.221997773265584,2.33362037932207,
7.73293756653933));
#47840=CARTESIAN_POINT('Ctrl Pts',(-0.21915214938016,2.33631498358247,7.73269614050075));
#47841=CARTESIAN_POINT('Ctrl Pts',(-0.21667956413232,2.33858416686921,7.73249228730989));
#47842=CARTESIAN_POINT('Ctrl Pts',(-0.203072647094565,2.35068567989956,
7.73139919443846));
#47843=CARTESIAN_POINT('Ctrl Pts',(-0.191302870889532,2.35977899251178,
7.73055553404026));
#47844=CARTESIAN_POINT('Ctrl Pts',(-0.167788575390083,2.37547806028539,
7.72896796469071));
#47845=CARTESIAN_POINT('Ctrl Pts',(-0.156176523573257,2.38222342241932,
7.72822378081531));
#47846=CARTESIAN_POINT('Ctrl Pts',(-0.132047898606532,2.39429319186261,
7.72670072915251));
#47847=CARTESIAN_POINT('Ctrl Pts',(-0.119548121083918,2.39958858683744,
7.72592301762301));
#47848=CARTESIAN_POINT('Ctrl Pts',(-0.101243987875153,2.4060145708186,7.72477312804479));
#47849=CARTESIAN_POINT('Ctrl Pts',(-0.0956839501782412,2.40779837177179,
7.72442256392184));
#47850=CARTESIAN_POINT('Ctrl Pts',(-0.0891863663322832,2.40968989586137,
7.72401036242171));
#47851=CARTESIAN_POINT('Ctrl Pts',(-0.0882928305514554,2.40994582685202,
7.72395362321472));
#47852=CARTESIAN_POINT('Ctrl Pts',(-0.0869338885493985,2.41032870855437,
7.72386724461564));
#47853=CARTESIAN_POINT('Ctrl Pts',(-0.0864692785510927,2.4104584870706,
7.7238376972781));
#47854=CARTESIAN_POINT('Ctrl Pts',(-0.0856634521705343,2.4106816276064,
7.72378642283914));
#47855=CARTESIAN_POINT('Ctrl Pts',(-0.0853223692893016,2.41077547211322,
7.72376471145582));
#47856=CARTESIAN_POINT('Ctrl Pts',(-0.0846136117890121,2.41096922273947,
7.72371957827158));
#47857=CARTESIAN_POINT('Ctrl Pts',(-0.0842459132938679,2.41106903877196,
7.72369615358426));
#47858=CARTESIAN_POINT('Ctrl Pts',(-0.0833501229305022,2.41131050669605,
7.72363906163552));
#47859=CARTESIAN_POINT('Ctrl Pts',(-0.0828218473107328,2.41145146680347,
7.72360537200116));
#47860=CARTESIAN_POINT('Ctrl Pts',(-0.0808251892907754,2.41197879708945,
7.72347795942955));
#47861=CARTESIAN_POINT('Ctrl Pts',(-0.0793544593852882,2.41235612801141,
7.72338394445073));
#47862=CARTESIAN_POINT('Ctrl Pts',(-0.0525607468767134,2.4190288847524,
7.72166805119647));
#47863=CARTESIAN_POINT('Ctrl Pts',(-0.0265738969956599,2.42223487768055,
7.71994089152942));
#47864=CARTESIAN_POINT('Ctrl Pts',(0.010581188389925,2.42229149911656,7.71742930079981));
#47865=CARTESIAN_POINT('Ctrl Pts',(0.0216471582448338,2.42173775042511,
7.71667778989407));
#47866=CARTESIAN_POINT('Ctrl Pts',(0.0408945858164924,2.41977691277874,
7.71538190785904));
#47867=CARTESIAN_POINT('Ctrl Pts',(0.0490916420477925,2.41862151790631,
7.7148337327451));
#47868=CARTESIAN_POINT('Ctrl Pts',(0.0603456261109347,2.41659053655771,
7.71409376263111));
#47869=CARTESIAN_POINT('Ctrl Pts',(0.0634472896557928,2.41598355267001,
7.71389117422289));
#47870=CARTESIAN_POINT('Ctrl Pts',(0.0682586692445174,2.41496827824923,
7.71357953996668));
#47871=CARTESIAN_POINT('Ctrl Pts',(0.0699747396147304,2.41459147855192,
7.71346891304632));
#47872=CARTESIAN_POINT('Ctrl Pts',(0.0721075518984737,2.4141048583619,7.71333214673509));
#47873=CARTESIAN_POINT('Ctrl Pts',(0.0725272260829327,2.41400822054398,
7.71330527028156));
#47874=CARTESIAN_POINT('Ctrl Pts',(0.073151048274662,2.41386325648438,7.71326537345835));
#47875=CARTESIAN_POINT('Ctrl Pts',(0.0733553426411092,2.41381557217778,
7.71325231626606));
#47876=CARTESIAN_POINT('Ctrl Pts',(0.0737514675816805,2.41372270478033,
7.71322701525823));
#47877=CARTESIAN_POINT('Ctrl Pts',(0.0739433030856167,2.41367754525097,
7.71321477012738));
#47878=CARTESIAN_POINT('Ctrl Pts',(0.0743440969143607,2.41358280724529,
7.71318920293883));
#47879=CARTESIAN_POINT('Ctrl Pts',(0.0745530464658049,2.41353319602426,
7.71317588284638));
#47880=CARTESIAN_POINT('Ctrl Pts',(0.0750676123437887,2.41341047836239,
7.71314310239469));
#47881=CARTESIAN_POINT('Ctrl Pts',(0.0753731724152606,2.41333713353568,
7.71312365582883));
#47882=CARTESIAN_POINT('Ctrl Pts',(0.0765648017193995,2.41304925794744,
7.71304789074373));
#47883=CARTESIAN_POINT('Ctrl Pts',(0.0774500773701396,2.41283141198785,
7.71299176155946));
#47884=CARTESIAN_POINT('Ctrl Pts',(0.0926054603769788,2.40903374396154,
7.71203338075983));
#47885=CARTESIAN_POINT('Ctrl Pts',(0.106617024733881,2.40448408924046,7.71118531400371));
#47886=CARTESIAN_POINT('Ctrl Pts',(0.136233246272949,2.39257088816415,7.7093804451085));
#47887=CARTESIAN_POINT('Ctrl Pts',(0.151656361097163,2.38488170619499,7.70843153731973));
#47888=CARTESIAN_POINT('Ctrl Pts',(0.17744460247778,2.36933463666151,7.7067282617686));
#47889=CARTESIAN_POINT('Ctrl Pts',(0.188085877727286,2.362014095635,7.70598646466654));
#47890=CARTESIAN_POINT('Ctrl Pts',(0.201214769239499,2.3517694350158,7.70499867108858));
#47891=CARTESIAN_POINT('Ctrl Pts',(0.20412996516913,2.34941168246824,7.70477442262453));
#47892=CARTESIAN_POINT('Ctrl Pts',(0.208192744827544,2.34600683963365,7.70445448997691));
#47893=CARTESIAN_POINT('Ctrl Pts',(0.209374978224071,2.34500143368869,7.70436048223005));
#47894=CARTESIAN_POINT('Ctrl Pts',(0.211437782899015,2.34322132929878,7.70419481985811));
#47895=CARTESIAN_POINT('Ctrl Pts',(0.212321479357396,2.34245028440836,7.70412331598305));
#47896=CARTESIAN_POINT('Ctrl Pts',(0.213598689401639,2.3413235521861,7.70401918228323));
#47897=CARTESIAN_POINT('Ctrl Pts',(0.213995571597392,2.3409716835755,7.70398671198336));
#47898=CARTESIAN_POINT('Ctrl Pts',(0.214688078406281,2.34035465944349,7.7039298591007));
#47899=CARTESIAN_POINT('Ctrl Pts',(0.21498408573375,2.34008993357682,7.70390549458936));
#47900=CARTESIAN_POINT('Ctrl Pts',(0.215556087166141,2.33957647412051,7.70385829007633));
#47901=CARTESIAN_POINT('Ctrl Pts',(0.21583214206669,2.33932780890549,7.70383545297818));
#47902=CARTESIAN_POINT('Ctrl Pts',(0.216487355882004,2.33873554864701,7.70378111652768));
#47903=CARTESIAN_POINT('Ctrl Pts',(0.216866126853119,2.33839152766715,7.70374959917338));
#47904=CARTESIAN_POINT('Ctrl Pts',(0.218203581893468,2.33717095079696,7.70363793241633));
#47905=CARTESIAN_POINT('Ctrl Pts',(0.219157774017282,2.33628951111215,7.70355757546932));
#47906=CARTESIAN_POINT('Ctrl Pts',(0.235278189763927,2.32121655156853,7.70218812143246));
#47907=CARTESIAN_POINT('Ctrl Pts',(0.249039851878306,2.30560019795321,7.70083435499544));
#47908=CARTESIAN_POINT('Ctrl Pts',(0.261841737704375,2.28788633079693,7.69936901788218));
#47909=CARTESIAN_POINT('Ctrl Pts',(0.262477083560678,2.28699772588632,7.69929569518324));
#47910=CARTESIAN_POINT('Ctrl Pts',(0.272256013528746,2.27317272881833,7.69815787819737));
#47911=CARTESIAN_POINT('Ctrl Pts',(0.280437930912508,2.25958286663693,7.69707776077898));
#47912=CARTESIAN_POINT('Ctrl Pts',(0.291550362917102,2.23761057363008,7.69542957510191));
#47913=CARTESIAN_POINT('Ctrl Pts',(0.295191809411358,2.22961521710622,7.69484881458794));
#47914=CARTESIAN_POINT('Ctrl Pts',(0.29882960426638,2.22067641400162,7.69422716191465));
#47915=CARTESIAN_POINT('Ctrl Pts',(0.299153598030281,2.21987098941035,7.69417139075256));
#47916=CARTESIAN_POINT('Ctrl Pts',(0.300248535594524,2.21711696640552,7.69398153965908));
#47917=CARTESIAN_POINT('Ctrl Pts',(0.301003746243188,2.21516211277538,7.69384822763014));
#47918=CARTESIAN_POINT('Ctrl Pts',(0.302193423898459,2.21199097101762,7.69363445990351));
#47919=CARTESIAN_POINT('Ctrl Pts',(0.302639729339874,2.21077922817762,7.69355335862578));
#47920=CARTESIAN_POINT('Ctrl Pts',(0.303209873544261,2.20920209233019,7.69344858729164));
#47921=CARTESIAN_POINT('Ctrl Pts',(0.303340348301456,2.20883913579255,7.69342452942272));
#47922=CARTESIAN_POINT('Ctrl Pts',(0.303551417213515,2.20824865354474,7.69338547895445));
#47923=CARTESIAN_POINT('Ctrl Pts',(0.303632407403628,2.20802127133939,7.69337046275133));
#47924=CARTESIAN_POINT('Ctrl Pts',(0.303786753505378,2.20758639530125,7.69334178477227));
#47925=CARTESIAN_POINT('Ctrl Pts',(0.303860151728064,2.20737891902645,7.69332812057505));
#47926=CARTESIAN_POINT('Ctrl Pts',(0.304027795567048,2.20690348838222,7.69329684979915));
#47927=CARTESIAN_POINT('Ctrl Pts',(0.304121899395974,2.20663548478306,7.69327925177198));
#47928=CARTESIAN_POINT('Ctrl Pts',(0.304417013387696,2.20579144486279,7.69322392111731));
#47929=CARTESIAN_POINT('Ctrl Pts',(0.304616743712643,2.20521495763587,7.69318626434405));
#47930=CARTESIAN_POINT('Ctrl Pts',(0.306243275281436,2.20047679917998,7.69287783985467));
#47931=CARTESIAN_POINT('Ctrl Pts',(0.307586443668984,2.19628663032616,7.69261190017591));
#47932=CARTESIAN_POINT('Ctrl Pts',(0.309068066355403,2.19131661433761,7.6923030020691));
#47933=CARTESIAN_POINT('Ctrl Pts',(0.309289911141217,2.19056237951671,7.6922563005768));
#47934=CARTESIAN_POINT('Ctrl Pts',(0.309580368312466,2.18956135761991,7.69219454212545));
#47935=CARTESIAN_POINT('Ctrl Pts',(0.309651447808156,2.18931529597151,7.69217937915355));
#47936=CARTESIAN_POINT('Ctrl Pts',(0.310049387808336,2.18793152990474,7.69209420707266));
#47937=CARTESIAN_POINT('Ctrl Pts',(0.310370275394789,2.18679210248744,7.69202445125741));
#47938=CARTESIAN_POINT('Ctrl Pts',(0.310865343323021,2.1849963234899,7.69191506889997));
#47939=CARTESIAN_POINT('Ctrl Pts',(0.311043736859899,2.18434115519104,7.69187527800773));
#47940=CARTESIAN_POINT('Ctrl Pts',(0.312250913383368,2.17985175269101,7.6916033822025));
#47941=CARTESIAN_POINT('Ctrl Pts',(0.313210878349691,2.17599923096801,7.69137386166672));
#47942=CARTESIAN_POINT('Ctrl Pts',(0.319194996612592,2.14994055075332,7.68984102013498));
#47943=CARTESIAN_POINT('Ctrl Pts',(0.321925106773675,2.12727320697862,7.68859865064319));
#47944=CARTESIAN_POINT('Ctrl Pts',(0.322452276600562,2.08957678888074,7.68645655304354));
#47945=CARTESIAN_POINT('Ctrl Pts',(0.321623277967013,2.07465250924172,7.68558980112057));
#47946=CARTESIAN_POINT('Ctrl Pts',(0.319565568121816,2.05826830383893,7.68459345918561));
#47947=CARTESIAN_POINT('Ctrl Pts',(0.319356507955438,2.05669748873085,7.68449749010102));
#47948=CARTESIAN_POINT('Ctrl Pts',(0.318969817998894,2.05394727782015,7.68432865493393));
#47949=CARTESIAN_POINT('Ctrl Pts',(0.318797208936006,2.05276719858829,7.68425594770765));
#47950=CARTESIAN_POINT('Ctrl Pts',(0.318537829094903,2.05106011563028,7.68415038172025));
#47951=CARTESIAN_POINT('Ctrl Pts',(0.318456290863451,2.05053231710819,7.68411768876079));
#47952=CARTESIAN_POINT('Ctrl Pts',(0.318311742732613,2.04961182438213,7.68406057651435));
#47953=CARTESIAN_POINT('Ctrl Pts',(0.318249316970781,2.04921903851926,7.68403617579677));
#47954=CARTESIAN_POINT('Ctrl Pts',(0.318127323567945,2.04846051086689,7.68398899565218));
#47955=CARTESIAN_POINT('Ctrl Pts',(0.318067851856139,2.04809475407585,7.68396621930408));
#47956=CARTESIAN_POINT('Ctrl Pts',(0.317925366198668,2.04722789421895,7.68391217535038));
#47957=CARTESIAN_POINT('Ctrl Pts',(0.317841798330907,2.04672688435821,7.68388089019409));
#47958=CARTESIAN_POINT('Ctrl Pts',(0.317543980476996,2.04496704026556,7.68377082123326));
#47959=CARTESIAN_POINT('Ctrl Pts',(0.317323435633818,2.04370929636171,7.683691837601));
#47960=CARTESIAN_POINT('Ctrl Pts',(0.313989508940211,2.02533872515421,7.68253346398495));
#47961=CARTESIAN_POINT('Ctrl Pts',(0.309503761528585,2.00850705349701,7.68140947520557));
#47962=CARTESIAN_POINT('Ctrl Pts',(0.29633089604837,1.97142476521467,7.67879294243829));
#47963=CARTESIAN_POINT('Ctrl Pts',(0.286882759074541,1.95153521874486,7.67728633007985));
#47964=CARTESIAN_POINT('Ctrl Pts',(0.270324818629718,1.92425989159784,7.67516073364978));
#47965=CARTESIAN_POINT('Ctrl Pts',(0.264772292228484,1.91600062753646,7.67450910296599));
#47966=CARTESIAN_POINT('Ctrl Pts',(0.258275410574658,1.90724132861538,7.67381983589781));
#47967=CARTESIAN_POINT('Ctrl Pts',(0.257701353896647,1.90647453564209,7.67375951421455));
#47968=CARTESIAN_POINT('Ctrl Pts',(0.256703317221129,1.90515372931929,7.67365565571933));
#47969=CARTESIAN_POINT('Ctrl Pts',(0.256280945013804,1.90459851711187,7.67361201209042));
#47970=CARTESIAN_POINT('Ctrl Pts',(0.255672196735265,1.90380368100727,7.67354955802662));
#47971=CARTESIAN_POINT('Ctrl Pts',(0.255487283471672,1.90356294709039,7.67353064581493));
#47972=CARTESIAN_POINT('Ctrl Pts',(0.255165626488035,1.90314541244769,7.67349785046666));
#47973=CARTESIAN_POINT('Ctrl Pts',(0.255029038665879,1.90296849231727,7.673483956254));
#47974=CARTESIAN_POINT('Ctrl Pts',(0.254766535228941,1.9026292058856,7.67345731488647));
#47975=CARTESIAN_POINT('Ctrl Pts',(0.254640648610336,1.90246681818537,7.67344456569951));
#47976=CARTESIAN_POINT('Ctrl Pts',(0.254342872797104,1.90208345936735,7.67341447181077));
#47977=CARTESIAN_POINT('Ctrl Pts',(0.254170850469058,1.90186259118507,7.67339713661001));
#47978=CARTESIAN_POINT('Ctrl Pts',(0.253571825685649,1.9010955367722,7.67333694270671));
#47979=CARTESIAN_POINT('Ctrl Pts',(0.253143344844011,1.90055049948498,7.67329418838059));
#47980=CARTESIAN_POINT('Ctrl Pts',(0.247865730512999,1.89388165981178,7.67277121500526));
#47981=CARTESIAN_POINT('Ctrl Pts',(0.242796793238019,1.88793413484025,7.6723063513108));
#47982=CARTESIAN_POINT('Ctrl Pts',(0.235061795773159,1.87949985309156,7.67163948122397));
#47983=CARTESIAN_POINT('Ctrl Pts',(0.232562226727042,1.8768651195644,7.67143000010558));
#47984=CARTESIAN_POINT('Ctrl Pts',(0.220114113797254,1.86418033252392,7.67041245032402));
#47985=CARTESIAN_POINT('Ctrl Pts',(0.209555669042481,1.85474993233711,7.66962698761722));
#47986=CARTESIAN_POINT('Ctrl Pts',(0.187017419806823,1.8371412325432,7.6680269456287));
#47987=CARTESIAN_POINT('Ctrl Pts',(0.175037743125708,1.82901661985489,7.66721372768));
#47988=CARTESIAN_POINT('Ctrl Pts',(0.155142907425573,1.81739512364424,7.66587635244263));
#47989=CARTESIAN_POINT('Ctrl Pts',(0.147562577890504,1.8133641607922,7.66536979145524));
#47990=CARTESIAN_POINT('Ctrl Pts',(0.138313832672107,1.80891016080787,7.66475095368425));
#47991=CARTESIAN_POINT('Ctrl Pts',(0.136791108982915,1.80819149579284,7.66464904792931));
#47992=CARTESIAN_POINT('Ctrl Pts',(0.134126284729243,1.80695924625846,7.66447064072923));
#47993=CARTESIAN_POINT('Ctrl Pts',(0.132986683523375,1.80644032030109,7.6643943240974));
#47994=CARTESIAN_POINT('Ctrl Pts',(0.131346967133883,1.8057051705048,7.66428447475699));
#47995=CARTESIAN_POINT('Ctrl Pts',(0.130849272853981,1.80548354845492,7.66425112738441));
#47996=CARTESIAN_POINT('Ctrl Pts',(0.129985601072845,1.80510157886302,7.66419324787234));
#47997=CARTESIAN_POINT('Ctrl Pts',(0.129619881822688,1.80494064748038,7.6641687357784));
#47998=CARTESIAN_POINT('Ctrl Pts',(0.128916815425657,1.8046328289998,7.66412160670282));
#47999=CARTESIAN_POINT('Ctrl Pts',(0.1285795139396,1.80448583858389,7.66409899329681));
#48000=CARTESIAN_POINT('Ctrl Pts',(0.127785359018117,1.80414137606551,7.66404574435649));
#48001=CARTESIAN_POINT('Ctrl Pts',(0.127328299366518,1.80394438442787,7.66401509248783));
#48002=CARTESIAN_POINT('Ctrl Pts',(0.125979991339732,1.80336696668039,7.66392465332999));
#48003=CARTESIAN_POINT('Ctrl Pts',(0.125087487227659,1.80298950324854,7.66386476537995));
#48004=CARTESIAN_POINT('Ctrl Pts',(0.117265435853685,1.79972286270666,7.66333968117115));
#48005=CARTESIAN_POINT('Ctrl Pts',(0.110239103848264,1.79707283652941,7.66286644664725));
#48006=CARTESIAN_POINT('Ctrl Pts',(0.0981072334794383,1.79297521244836,
7.66204572664159));
#48007=CARTESIAN_POINT('Ctrl Pts',(0.0930465495521231,1.79140384948237,
7.66170234868581));
#48008=CARTESIAN_POINT('Ctrl Pts',(0.0603274886091704,1.78212242975367,
7.6594764318773));
#48009=CARTESIAN_POINT('Ctrl Pts',(0.0317869188846806,1.77801428794589,
7.65749237595424));
#48010=CARTESIAN_POINT('Ctrl Pts',(-0.0032785813727824,1.77767890100403,
7.65517154459606));
#48011=CARTESIAN_POINT('Ctrl Pts',(-0.00964031750125043,1.77780640050279,
7.65475588859718));
#48012=CARTESIAN_POINT('Ctrl Pts',(-0.0190281107768603,1.77827289205018,
7.6541543236124));
#48013=CARTESIAN_POINT('Ctrl Pts',(-0.0220595511489733,1.77846651987733,
7.65396189790555));
#48014=CARTESIAN_POINT('Ctrl Pts',(-0.0255935536621075,1.77874246647417,
7.65374005698777));
#48015=CARTESIAN_POINT('Ctrl Pts',(-0.026099084727614,1.77878314082089,
7.65370838260688));
#48016=CARTESIAN_POINT('Ctrl Pts',(-0.0268699155485872,1.7788469925712,
7.65366017857142));
#48017=CARTESIAN_POINT('Ctrl Pts',(-0.0271352831383519,1.77886930549637,
7.65364360055792));
#48018=CARTESIAN_POINT('Ctrl Pts',(-0.0275966724623211,1.77890867652815,
7.65361480626225));
#48019=CARTESIAN_POINT('Ctrl Pts',(-0.0277927057233755,1.77892558518442,
7.65360258155675));
#48020=CARTESIAN_POINT('Ctrl Pts',(-0.0282042132336269,1.77896145905994,
7.65357693936672));
#48021=CARTESIAN_POINT('Ctrl Pts',(-0.0284196831959511,1.7789804616215,
7.65356352405902));
#48022=CARTESIAN_POINT('Ctrl Pts',(-0.0290223604883649,1.77903422401482,
7.65352603197075));
#48023=CARTESIAN_POINT('Ctrl Pts',(-0.0294095259536415,1.77906946772076,
7.65350198252304));
#48024=CARTESIAN_POINT('Ctrl Pts',(-0.0309763745742602,1.77921495726464,
7.65340479660584));
#48025=CARTESIAN_POINT('Ctrl Pts',(-0.0321555284653409,1.77933100942571,
7.6533319829053));
#48026=CARTESIAN_POINT('Ctrl Pts',(-0.053145567281961,1.7815137906095,7.65204119512836));
#48027=CARTESIAN_POINT('Ctrl Pts',(-0.0727268769049766,1.78540664800537,
7.65092082264426));
#48028=CARTESIAN_POINT('Ctrl Pts',(-0.107433872294403,1.79572335754646,
7.64889468959375));
#48029=CARTESIAN_POINT('Ctrl Pts',(-0.122667531086389,1.80153901420385,
7.64798993551845));
#48030=CARTESIAN_POINT('Ctrl Pts',(-0.149568954146757,1.81421790492987,
7.64628410424557));
#48031=CARTESIAN_POINT('Ctrl Pts',(-0.161369344547343,1.82071136276686,
7.6454942299687));
#48032=CARTESIAN_POINT('Ctrl Pts',(-0.173786365843938,1.82859431669487,
7.644600482914));
#48033=CARTESIAN_POINT('Ctrl Pts',(-0.174840344003534,1.8292720924564,7.64452411125783));
#48034=CARTESIAN_POINT('Ctrl Pts',(-0.176346978998829,1.83025342334575,
7.64441419676429));
#48035=CARTESIAN_POINT('Ctrl Pts',(-0.176802869575741,1.83055201258365,
7.64438083956893));
#48036=CARTESIAN_POINT('Ctrl Pts',(-0.177591717370694,1.83107153884446,
7.64432294848826));
#48037=CARTESIAN_POINT('Ctrl Pts',(-0.177925026087404,1.83129194208652,
7.64429843467079));
#48038=CARTESIAN_POINT('Ctrl Pts',(-0.17856442200477,1.83171645937319,7.64425130614526));
#48039=CARTESIAN_POINT('Ctrl Pts',(-0.178870571488163,1.83192047890429,
7.64422869502012));
#48040=CARTESIAN_POINT('Ctrl Pts',(-0.179589942148884,1.83240165196644,
7.64417545733146));
#48041=CARTESIAN_POINT('Ctrl Pts',(-0.180002871277948,1.83267923851936,
7.64414481445069));
#48042=CARTESIAN_POINT('Ctrl Pts',(-0.181217654310668,1.83349995243937,
7.64405441912576));
#48043=CARTESIAN_POINT('Ctrl Pts',(-0.18201769938503,1.83404573577127,7.64399456615848));
#48044=CARTESIAN_POINT('Ctrl Pts',(-0.188985559195315,1.83884531256288,
7.64347046600645));
#48045=CARTESIAN_POINT('Ctrl Pts',(-0.195005300669939,1.84330907706944,
7.64299821369596));
#48046=CARTESIAN_POINT('Ctrl Pts',(-0.20397453112219,1.85045763658458,7.64226315361172));
#48047=CARTESIAN_POINT('Ctrl Pts',(-0.207039114221632,1.85299432486107,
7.64200607128229));
#48048=CARTESIAN_POINT('Ctrl Pts',(-0.210778729385711,1.85620826231229,
7.64168493909231));
#48049=CARTESIAN_POINT('Ctrl Pts',(-0.21149883458691,1.85683271793421,7.64162275255913));
#48050=CARTESIAN_POINT('Ctrl Pts',(-0.232341510556716,1.87506954066465,
7.63981268522344));
#48051=CARTESIAN_POINT('Ctrl Pts',(-0.250195821429652,1.89511460141647,
7.63797371214083));
#48052=CARTESIAN_POINT('Ctrl Pts',(-0.267835062377407,1.92071118793796,
7.63589935327861));
#48053=CARTESIAN_POINT('Ctrl Pts',(-0.270230772097741,1.92434285849792,
7.63561102781066));
#48054=CARTESIAN_POINT('Ctrl Pts',(-0.27521311259121,1.93223891925396,7.63499848803226));
#48055=CARTESIAN_POINT('Ctrl Pts',(-0.27777586338533,1.93651723863508,7.63467526186131));
#48056=CARTESIAN_POINT('Ctrl Pts',(-0.281451229785814,1.94298913276123,
7.63420096549317));
#48057=CARTESIAN_POINT('Ctrl Pts',(-0.282639611846494,1.94513858492036,
7.634045792782));
#48058=CARTESIAN_POINT('Ctrl Pts',(-0.284029823044681,1.9477224123098,7.63386224360101));
#48059=CARTESIAN_POINT('Ctrl Pts',(-0.284255362659158,1.94814384142204,
7.63383240020002));
#48060=CARTESIAN_POINT('Ctrl Pts',(-0.284602165231953,1.94879533472415,
7.63378641161154));
#48061=CARTESIAN_POINT('Ctrl Pts',(-0.284724087499885,1.94902504428084,
7.63377022462839));
#48062=CARTESIAN_POINT('Ctrl Pts',(-0.284937529398125,1.94942836096993,
7.63374185365469));
#48063=CARTESIAN_POINT('Ctrl Pts',(-0.285029168105033,1.94960190337098,
7.63372966207365));
#48064=CARTESIAN_POINT('Ctrl Pts',(-0.285223201931387,1.94997017260727,
7.63370382483848));
#48065=CARTESIAN_POINT('Ctrl Pts',(-0.285325555848573,1.95016491996903,
7.63369018184432));
#48066=CARTESIAN_POINT('Ctrl Pts',(-0.28561674014468,1.95072033256433,7.63365132961324));
#48067=CARTESIAN_POINT('Ctrl Pts',(-0.28580508751784,1.95108125264486,7.63362615108747));
#48068=CARTESIAN_POINT('Ctrl Pts',(-0.286606060792816,1.95262323200482,
7.6335188676442));
#48069=CARTESIAN_POINT('Ctrl Pts',(-0.287212064810507,1.95380774370986,
7.63343717555367));
#48070=CARTESIAN_POINT('Ctrl Pts',(-0.298832582732669,1.97687269148309,
7.63185974129093));
#48071=CARTESIAN_POINT('Ctrl Pts',(-0.307326241200577,1.99993876185725,
7.63050971479041));
#48072=CARTESIAN_POINT('Ctrl Pts',(-0.316576616682861,2.03792484663418,
7.62832296292454));
#48073=CARTESIAN_POINT('Ctrl Pts',(-0.319062011034038,2.05231909367544,
7.62750290103042));
#48074=CARTESIAN_POINT('Ctrl Pts',(-0.321307279135699,2.07401883205741,
7.62623727577414));
#48075=CARTESIAN_POINT('Ctrl Pts',(-0.321808983891043,2.08122886849482,
7.62581216283101));
#48076=CARTESIAN_POINT('Ctrl Pts',(-0.322205907641382,2.09229629730358,
7.625149169922));
#48077=CARTESIAN_POINT('Ctrl Pts',(-0.322274934450132,2.09614531122044,
7.62491667787055));
#48078=CARTESIAN_POINT('Ctrl Pts',(-0.322275012560333,2.10073534831961,
7.62463685322158));
#48079=CARTESIAN_POINT('Ctrl Pts',(-0.322272470674025,2.10147617382821,
7.62459161021307));
#48080=CARTESIAN_POINT('Ctrl Pts',(-0.322264040947298,2.10270154660044,
7.62451664118377));
#48081=CARTESIAN_POINT('Ctrl Pts',(-0.322259614566028,2.10318610379868,
7.62448696097681));
#48082=CARTESIAN_POINT('Ctrl Pts',(-0.322249638207019,2.10406195006513,
7.62443325001728));
#48083=CARTESIAN_POINT('Ctrl Pts',(-0.322244468355237,2.10445324322182,
7.62440923121972));
#48084=CARTESIAN_POINT('Ctrl Pts',(-0.322231878006127,2.10529070336594,
7.62435777590945));
#48085=CARTESIAN_POINT('Ctrl Pts',(-0.322224243519934,2.10573686589341,
7.62433033274114));
#48086=CARTESIAN_POINT('Ctrl Pts',(-0.322201049386374,2.10694558371266,
7.62425590326289));
#48087=CARTESIAN_POINT('Ctrl Pts',(-0.322183709335855,2.10770809842889,
7.62420886126446));
#48088=CARTESIAN_POINT('Ctrl Pts',(-0.322083778834763,2.11150879818129,
7.62397393648265));
#48089=CARTESIAN_POINT('Ctrl Pts',(-0.32196092150771,2.11454568759986,7.62378479630448));
#48090=CARTESIAN_POINT('Ctrl Pts',(-0.320149619479709,2.14770030120993,
7.62170360951507));
#48091=CARTESIAN_POINT('Ctrl Pts',(-0.314283651835385,2.17743423378051,
7.61966890457982));
#48092=CARTESIAN_POINT('Ctrl Pts',(-0.299501198459806,2.21991722276558,
7.61662892371279));
#48093=CARTESIAN_POINT('Ctrl Pts',(-0.29366599319579,2.23357200756451,7.61563349308438));
#48094=CARTESIAN_POINT('Ctrl Pts',(-0.285393098602287,2.24974329184827,
7.61446801931277));
#48095=CARTESIAN_POINT('Ctrl Pts',(-0.2838298458655,2.25268560811725,7.61425657520329));
#48096=CARTESIAN_POINT('Ctrl Pts',(-0.281953167585538,2.25608938152167,
7.61401314920497));
#48097=CARTESIAN_POINT('Ctrl Pts',(-0.281683903331657,2.25657478197366,
7.61397846339922));
#48098=CARTESIAN_POINT('Ctrl Pts',(-0.281276896181146,2.25730404233566,
7.61392639733413));
#48099=CARTESIAN_POINT('Ctrl Pts',(-0.281140089068572,2.2575484191618,7.61390895758748));
#48100=CARTESIAN_POINT('Ctrl Pts',(-0.280895753895735,2.25798354032395,
7.61387791971167));
#48101=CARTESIAN_POINT('Ctrl Pts',(-0.280788350070565,2.25817435328037,
7.61386431361034));
#48102=CARTESIAN_POINT('Ctrl Pts',(-0.280559814423472,2.2585794019552,7.61383544171803));
#48103=CARTESIAN_POINT('Ctrl Pts',(-0.280438631993344,2.25879360780736,
7.61382017930754));
#48104=CARTESIAN_POINT('Ctrl Pts',(-0.280112584150046,2.25936840282566,
7.61377924057742));
#48105=CARTESIAN_POINT('Ctrl Pts',(-0.279907267003762,2.25972873724372,
7.61375359341748));
#48106=CARTESIAN_POINT('Ctrl Pts',(-0.278918237708143,2.26145673412273,
7.61363067831788));
#48107=CARTESIAN_POINT('Ctrl Pts',(-0.278125176680091,2.26281906108981,
7.61353400522015));
#48108=CARTESIAN_POINT('Ctrl Pts',(-0.271434516950736,2.27412079307144,
7.61273348041306));
#48109=CARTESIAN_POINT('Ctrl Pts',(-0.265015456679295,2.28374334872336,
7.61206128561747));
#48110=CARTESIAN_POINT('Ctrl Pts',(-0.245219124383414,2.31021616496064,
7.6101777642012));
#48111=CARTESIAN_POINT('Ctrl Pts',(-0.230655604560742,2.32610020952501,
7.60900129228236));
#48112=CARTESIAN_POINT('Ctrl Pts',(-0.2103688989993,2.34421006175128,7.60745496164659));
#48113=CARTESIAN_POINT('Ctrl Pts',(-0.206019484597079,2.34789028970342,
7.60712836035628));
#48114=CARTESIAN_POINT('Ctrl Pts',(-0.193324407773146,2.35806717188198,
7.60618467668596));
#48115=CARTESIAN_POINT('Ctrl Pts',(-0.184754129243422,2.36427044351863,
7.60555871226171));
#48116=CARTESIAN_POINT('Ctrl Pts',(-0.174907758963399,2.37068402242334,
7.60484427687951));
#48117=CARTESIAN_POINT('Ctrl Pts',(-0.173916883153688,2.37132173122931,
7.60477243577162));
#48118=CARTESIAN_POINT('Ctrl Pts',(-0.172518929807106,2.37221062295483,
7.60467114932794));
#48119=CARTESIAN_POINT('Ctrl Pts',(-0.172114748051081,2.37246636102584,
7.60464187304257));
#48120=CARTESIAN_POINT('Ctrl Pts',(-0.171371907842553,2.37293406611667,
7.60458808062709));
#48121=CARTESIAN_POINT('Ctrl Pts',(-0.171033421154564,2.37314630528429,
7.60456357462077));
#48122=CARTESIAN_POINT('Ctrl Pts',(-0.17034630544416,2.37357536511947,7.6045138387218));
#48123=CARTESIAN_POINT('Ctrl Pts',(-0.169997655088973,2.37379215007099,
7.60448860757195));
#48124=CARTESIAN_POINT('Ctrl Pts',(-0.169137563833894,2.37432466418967,
7.60442637723015));
#48125=CARTESIAN_POINT('Ctrl Pts',(-0.168625653609846,2.37463962900368,
7.60438935000865));
#48126=CARTESIAN_POINT('Ctrl Pts',(-0.16675038675377,2.37578621153987,7.60425374743221));
#48127=CARTESIAN_POINT('Ctrl Pts',(-0.165381752374354,2.37660911371873,
7.60415485354738));
#48128=CARTESIAN_POINT('Ctrl Pts',(-0.146978990865274,2.38748851527267,
7.60282595798942));
#48129=CARTESIAN_POINT('Ctrl Pts',(-0.12906353312393,2.39596421313499,7.60153778345662));
#48130=CARTESIAN_POINT('Ctrl Pts',(-0.0832043903394734,2.41270066680676,
7.59826908696113));
#48131=CARTESIAN_POINT('Ctrl Pts',(-0.0547007130052508,2.41892415240699,
7.59625520978267));
#48132=CARTESIAN_POINT('Ctrl Pts',(-0.0242493089166614,2.4213649157781,
7.59432298354425));
#48133=CARTESIAN_POINT('Ctrl Pts',(-0.0227491149093209,2.4214745962844,
7.59422837807063));
#48134=CARTESIAN_POINT('Ctrl Pts',(-0.0208221765119838,2.42160191985776,
7.59410766053092));
#48135=CARTESIAN_POINT('Ctrl Pts',(-0.0203961209035794,2.42162922153932,
7.59408101942023));
#48136=CARTESIAN_POINT('Ctrl Pts',(-0.0197216549529017,2.42167109579288,
7.59403892598978));
#48137=CARTESIAN_POINT('Ctrl Pts',(-0.0194732817371178,2.42168622731175,
7.59402344232937));
#48138=CARTESIAN_POINT('Ctrl Pts',(-0.0190285844068785,2.42171280247151,
7.59399575106658));
#48139=CARTESIAN_POINT('Ctrl Pts',(-0.0188322687539985,2.42172435399345,
7.5939835374557));
#48140=CARTESIAN_POINT('Ctrl Pts',(-0.0183711820407109,2.42175106158005,
7.59395487694845));
#48141=CARTESIAN_POINT('Ctrl Pts',(-0.0181064031620623,2.4217660704972,
7.59393843845871));
#48142=CARTESIAN_POINT('Ctrl Pts',(-0.0173404047640351,2.4218085423998,
7.5938909388223));
#48143=CARTESIAN_POINT('Ctrl Pts',(-0.0168391363612734,2.42183516136918,
7.59385992506942));
#48144=CARTESIAN_POINT('Ctrl Pts',(-0.0134187945711616,2.42200877961112,
7.59364877140263));
#48145=CARTESIAN_POINT('Ctrl Pts',(-0.0104977808456938,2.42211723989591,
7.59347075270674));
#48146=CARTESIAN_POINT('Ctrl Pts',(-0.00132634554620723,2.42233288829333,
7.59291792362431));
#48147=CARTESIAN_POINT('Ctrl Pts',(0.00492627010779293,2.42229798725449,
7.59254993392689));
#48148=CARTESIAN_POINT('Ctrl Pts',(0.0258773434048393,2.4215711085741,7.59133511651112));
#48149=CARTESIAN_POINT('Ctrl Pts',(0.0405291705360306,2.42005477347917,
7.59051509368766));
#48150=CARTESIAN_POINT('Ctrl Pts',(0.0809207473943615,2.41305532048777,
7.58822377012808));
#48151=CARTESIAN_POINT('Ctrl Pts',(0.106164201112711,2.40541889452105,7.58674752101773));
#48152=CARTESIAN_POINT('Ctrl Pts',(0.131638097417043,2.39416842278127,7.58505924560763));
#48153=CARTESIAN_POINT('Ctrl Pts',(0.133072233736145,2.39352245250589,7.58496353428421));
#48154=CARTESIAN_POINT('Ctrl Pts',(0.135061868145168,2.39260869357318,7.58482980213474));
#48155=CARTESIAN_POINT('Ctrl Pts',(0.135621429216146,2.39234976263117,7.58479208656868));
#48156=CARTESIAN_POINT('Ctrl Pts',(0.13651780691399,2.39193184605432,7.5847314989662));
#48157=CARTESIAN_POINT('Ctrl Pts',(0.13685509887333,2.39177387863853,7.58470866216084));
#48158=CARTESIAN_POINT('Ctrl Pts',(0.137550978047257,2.3914464982619,7.58466146640298));
#48159=CARTESIAN_POINT('Ctrl Pts',(0.137909527772785,2.39127700743138,7.58463710478184));
#48160=CARTESIAN_POINT('Ctrl Pts',(0.138743923894916,2.39088069218651,7.58458030846892));
#48161=CARTESIAN_POINT('Ctrl Pts',(0.139219527416752,2.39065336173052,7.5845478562532));
#48162=CARTESIAN_POINT('Ctrl Pts',(0.140711811462084,2.38993557203582,7.58444578394137));
#48163=CARTESIAN_POINT('Ctrl Pts',(0.14172646585146,2.38944094154418,7.58437601881658));
#48164=CARTESIAN_POINT('Ctrl Pts',(0.14407832963174,2.38827910749902,7.58421345639649));
#48165=CARTESIAN_POINT('Ctrl Pts',(0.14541353019546,2.38760791714572,7.58412052052132));
#48166=CARTESIAN_POINT('Ctrl Pts',(0.158768703088818,2.38077764948709,7.58318435867983));
#48167=CARTESIAN_POINT('Ctrl Pts',(0.170393314493812,2.37387884731757,7.58231487139548));
#48168=CARTESIAN_POINT('Ctrl Pts',(0.203905702221498,2.35102941570835,7.57963934501254));
#48169=CARTESIAN_POINT('Ctrl Pts',(0.224250369378604,2.33303403981466,7.57777069744263));
#48170=CARTESIAN_POINT('Ctrl Pts',(0.247673522535706,2.30637378384858,7.5754281009044));
#48171=CARTESIAN_POINT('Ctrl Pts',(0.25299007412235,2.2998208301106,7.57488132485539));
#48172=CARTESIAN_POINT('Ctrl Pts',(0.258466467468066,2.29250132071328,7.57430772057541));
#48173=CARTESIAN_POINT('Ctrl Pts',(0.258887231028642,2.29193507994713,7.57426357916349));
#48174=CARTESIAN_POINT('Ctrl Pts',(0.259473622729053,2.29114050928364,7.57420196883209));
#48175=CARTESIAN_POINT('Ctrl Pts',(0.259640811652717,2.29091334187836,7.57418439212511));
#48176=CARTESIAN_POINT('Ctrl Pts',(0.259929596537574,2.29051987536498,7.57415401382545));
#48177=CARTESIAN_POINT('Ctrl Pts',(0.260051331302166,2.29035367911808,7.57414120252334));
#48178=CARTESIAN_POINT('Ctrl Pts',(0.26030455590277,2.29000727240368,7.57411454183504));
#48179=CARTESIAN_POINT('Ctrl Pts',(0.260436017847515,2.28982704232549,7.57410069446151));
#48180=CARTESIAN_POINT('Ctrl Pts',(0.260744560786202,2.28940311610561,7.5740681789972));
#48181=CARTESIAN_POINT('Ctrl Pts',(0.260921488019095,2.28915930709794,7.57404952166692));
#48182=CARTESIAN_POINT('Ctrl Pts',(0.261504069283991,2.28835412674925,7.57398804619438));
#48183=CARTESIAN_POINT('Ctrl Pts',(0.26190825908423,2.28779169087037,7.57394532904591));
#48184=CARTESIAN_POINT('Ctrl Pts',(0.26285971052841,2.28645868565359,7.57384460599064));
#48185=CARTESIAN_POINT('Ctrl Pts',(0.263405405254352,2.2856869984904,7.57378670440569));
#48186=CARTESIAN_POINT('Ctrl Pts',(0.269521128736105,2.27695731504426,7.57313614234069));
#48187=CARTESIAN_POINT('Ctrl Pts',(0.274732630187969,2.2687529322488,7.5725662089561));
#48188=CARTESIAN_POINT('Ctrl Pts',(0.291256749695207,2.23993903986594,7.57065786270303));
#48189=CARTESIAN_POINT('Ctrl Pts',(0.300683125987645,2.21833512994233,7.56937754214408));
#48190=CARTESIAN_POINT('Ctrl Pts',(0.309340247696754,2.19055961705398,7.56772329617016));
#48191=CARTESIAN_POINT('Ctrl Pts',(0.310864643604397,2.18517982460951,7.56740283203414));
#48192=CARTESIAN_POINT('Ctrl Pts',(0.312738450200803,2.1778444570412,7.56696393816779));
#48193=CARTESIAN_POINT('Ctrl Pts',(0.313210903433455,2.17592119258759,7.56684868834335));
#48194=CARTESIAN_POINT('Ctrl Pts',(0.314233673941263,2.17158558258391,7.56658836759382));
#48195=CARTESIAN_POINT('Ctrl Pts',(0.314773991934716,2.16917102735421,7.56644303590235));
#48196=CARTESIAN_POINT('Ctrl Pts',(0.316625658353819,2.16042495009888,7.56591499409328));
#48197=CARTESIAN_POINT('Ctrl Pts',(0.317774126741131,2.15406086912351,7.56552767751639));
#48198=CARTESIAN_POINT('Ctrl Pts',(0.31888288275281,2.14664703678556,7.56507143013392));
#48199=CARTESIAN_POINT('Ctrl Pts',(0.319030504679153,2.14562648352688,7.56500851625671));
#48200=CARTESIAN_POINT('Ctrl Pts',(0.319242869932705,2.14410690220001,7.56491467096175));
#48201=CARTESIAN_POINT('Ctrl Pts',(0.319311347510404,2.14360839564927,7.56488385767587));
#48202=CARTESIAN_POINT('Ctrl Pts',(0.319431255130404,2.14272005948985,7.56482889998561));
#48203=CARTESIAN_POINT('Ctrl Pts',(0.319483139871732,2.14233029142974,7.5648047700017));
#48204=CARTESIAN_POINT('Ctrl Pts',(0.319590885417222,2.14150940337449,7.56475391455107));
#48205=CARTESIAN_POINT('Ctrl Pts',(0.319646587440673,2.14107826365432,7.56472718412046));
#48206=CARTESIAN_POINT('Ctrl Pts',(0.319791123668784,2.13994144123875,7.5646566468676));
#48207=CARTESIAN_POINT('Ctrl Pts',(0.319878494007736,2.13923557778284,7.56461279392752));
#48208=CARTESIAN_POINT('Ctrl Pts',(0.320254082230644,2.13611654603187,7.56441876834588));
#48209=CARTESIAN_POINT('Ctrl Pts',(0.320517328251993,2.13370050225922,7.56426781063846));
#48210=CARTESIAN_POINT('Ctrl Pts',(0.322241461733275,2.11602178832246,7.56315813270546));
#48211=CARTESIAN_POINT('Ctrl Pts',(0.322638615669189,2.10067736613264,7.56216586445049));
#48212=CARTESIAN_POINT('Ctrl Pts',(0.321024072160057,2.06516094890958,7.55980589436602));
#48213=CARTESIAN_POINT('Ctrl Pts',(0.318205749563082,2.04508888687443,7.55842310022286));
#48214=CARTESIAN_POINT('Ctrl Pts',(0.3112213683268,2.01572921455733,7.55639931242098));
#48215=CARTESIAN_POINT('Ctrl Pts',(0.30846929553496,2.00615419812249,7.55573987930658));
#48216=CARTESIAN_POINT('Ctrl Pts',(0.304164835325749,1.99343079867157,7.55487721536471));
#48217=CARTESIAN_POINT('Ctrl Pts',(0.302998466266723,1.99015841596484,7.55465660527946));
#48218=CARTESIAN_POINT('Ctrl Pts',(0.301579595397936,1.98637233037963,7.55440336276679));
#48219=CARTESIAN_POINT('Ctrl Pts',(0.301378419201365,1.98583981379132,7.55436779039634));
#48220=CARTESIAN_POINT('Ctrl Pts',(0.301076507557982,1.98504700911461,7.55431490292469));
#48221=CARTESIAN_POINT('Ctrl Pts',(0.300976844606996,1.9847863179625,7.55429752406024));
#48222=CARTESIAN_POINT('Ctrl Pts',(0.300798423864968,1.98432142927908,7.55426655370896));
#48223=CARTESIAN_POINT('Ctrl Pts',(0.300719796781136,1.98411718268589,7.55425295438335));
#48224=CARTESIAN_POINT('Ctrl Pts',(0.300552099837198,1.98368288274994,7.55422405318424));
#48225=CARTESIAN_POINT('Ctrl Pts',(0.300462974131646,1.98345285220625,7.5542087547803));
#48226=CARTESIAN_POINT('Ctrl Pts',(0.300225395873851,1.98284175425108,7.55416813741884));
#48227=CARTESIAN_POINT('Ctrl Pts',(0.300076481336337,1.98246086512246,7.55414284630165));
#48228=CARTESIAN_POINT('Ctrl Pts',(0.299389780388169,1.98071425303928,7.55402698182272));
#48229=CARTESIAN_POINT('Ctrl Pts',(0.29884338172013,1.97935190252861,7.55393691957966));
#48230=CARTESIAN_POINT('Ctrl Pts',(0.297341554388725,1.97568016480934,7.55369490980117));
#48231=CARTESIAN_POINT('Ctrl Pts',(0.296368519725182,1.97337803210946,7.55354394858653));
#48232=CARTESIAN_POINT('Ctrl Pts',(0.291443737818718,1.96209421278481,7.55280675364703));
#48233=CARTESIAN_POINT('Ctrl Pts',(0.287109661761195,1.95328416956538,7.55223970998044));
#48234=CARTESIAN_POINT('Ctrl Pts',(0.274293111893614,1.92998226696738,7.55072790677214));
#48235=CARTESIAN_POINT('Ctrl Pts',(0.265070226324213,1.91593330454104,7.54980203519208));
#48236=CARTESIAN_POINT('Ctrl Pts',(0.242464370990616,1.88674490658963,7.54772382239498));
#48237=CARTESIAN_POINT('Ctrl Pts',(0.228670644922105,1.87201697627745,7.54656617174874));
#48238=CARTESIAN_POINT('Ctrl Pts',(0.212623316888819,1.85781374409654,7.54526457019303));
#48239=CARTESIAN_POINT('Ctrl Pts',(0.211647041977099,1.85696011237066,7.54518556233573));
#48240=CARTESIAN_POINT('Ctrl Pts',(0.210278703804204,1.85577816683088,7.54507506127651));
#48241=CARTESIAN_POINT('Ctrl Pts',(0.209890962046846,1.85544485056259,7.54504377508017));
#48242=CARTESIAN_POINT('Ctrl Pts',(0.209220181226333,1.85487099444814,7.54498969522928));
#48243=CARTESIAN_POINT('Ctrl Pts',(0.208937515696878,1.85463001787552,7.54496691960581));
#48244=CARTESIAN_POINT('Ctrl Pts',(0.208351743984256,1.85413238491025,7.54491974892185));
#48245=CARTESIAN_POINT('Ctrl Pts',(0.208048578798419,1.85387579918065,7.54489535101623));
#48246=CARTESIAN_POINT('Ctrl Pts',(0.207339177167758,1.85327763997268,7.54483829532017));
#48247=CARTESIAN_POINT('Ctrl Pts',(0.206932570588245,1.8529365090702,7.54480561951618));
#48248=CARTESIAN_POINT('Ctrl Pts',(0.205653023738887,1.85186838169474,7.54470287462788));
#48249=CARTESIAN_POINT('Ctrl Pts',(0.204777088236436,1.85114500154472,7.5446326586909));
#48250=CARTESIAN_POINT('Ctrl Pts',(0.197609528716323,1.84528923114833,7.54405903884289));
#48251=CARTESIAN_POINT('Ctrl Pts',(0.191130324921618,1.84039206238747,7.54354625952028));
#48252=CARTESIAN_POINT('Ctrl Pts',(0.178579007283364,1.83163011975778,7.54256219323574));
#48253=CARTESIAN_POINT('Ctrl Pts',(0.172548761275471,1.8277138130265,7.54209317529982));
#48254=CARTESIAN_POINT('Ctrl Pts',(0.151675411926663,1.81512971494047,7.540483732037));
#48255=CARTESIAN_POINT('Ctrl Pts',(0.136272606435354,1.80744879769435,7.53931750175913));
#48256=CARTESIAN_POINT('Ctrl Pts',(0.106556436857898,1.79548822311279,7.53715255983061));
#48257=CARTESIAN_POINT('Ctrl Pts',(0.0924122603638716,1.7909016995955,7.53615570693693));
#48258=CARTESIAN_POINT('Ctrl Pts',(0.0747580804812318,1.78649788599447,
7.53498818197458));
#48259=CARTESIAN_POINT('Ctrl Pts',(0.0715026797447825,1.78573941538994,
7.53477604367247));
#48260=CARTESIAN_POINT('Ctrl Pts',(0.0676928872400136,1.7849140476611,7.53453190674288));
#48261=CARTESIAN_POINT('Ctrl Pts',(0.067149551285568,1.78479780756267,7.53449718650707));
#48262=CARTESIAN_POINT('Ctrl Pts',(0.0663317815304237,1.78462506617525,
7.53444507882713));
#48263=CARTESIAN_POINT('Ctrl Pts',(0.0660575737829031,1.78456751740933,
7.53442763175605));
#48264=CARTESIAN_POINT('Ctrl Pts',(0.065568924220027,1.78446562825542,7.5343965857413));
#48265=CARTESIAN_POINT('Ctrl Pts',(0.0653545124012318,1.78442114886214,
7.5343829788094));
#48266=CARTESIAN_POINT('Ctrl Pts',(0.0648990938932745,1.78432715705738,
7.53435411036995));
#48267=CARTESIAN_POINT('Ctrl Pts',(0.0646580764842503,1.78427770223506,
7.53433885223227));
#48268=CARTESIAN_POINT('Ctrl Pts',(0.0641663974572591,1.78417740030453,
7.53430776508113));
#48269=CARTESIAN_POINT('Ctrl Pts',(0.0639157314028306,1.78412657547466,
7.534291937355));
#48270=CARTESIAN_POINT('Ctrl Pts',(0.0628083458540102,1.78390341510573,
7.53422210579653));
#48271=CARTESIAN_POINT('Ctrl Pts',(0.0619509773232575,1.78373426404194,
7.53416828266879));
#48272=CARTESIAN_POINT('Ctrl Pts',(0.0519130690448392,1.78179626065547,
7.53354085279353));
#48273=CARTESIAN_POINT('Ctrl Pts',(0.042659420702781,1.78042403395442,7.53298901330319));
#48274=CARTESIAN_POINT('Ctrl Pts',(0.0178512208005186,1.7778423027169,7.53154894943875));
#48275=CARTESIAN_POINT('Ctrl Pts',(0.00224658758511204,1.77735583104859,
7.53068321965015));
#48276=CARTESIAN_POINT('Ctrl Pts',(-0.0379802010981444,1.77902146602183,
7.52843150563953));
#48277=CARTESIAN_POINT('Ctrl Pts',(-0.0624248212311037,1.78286815416693,
7.52703754896194));
#48278=CARTESIAN_POINT('Ctrl Pts',(-0.0877004801231903,1.7898834753987,
7.52544722052646));
#48279=CARTESIAN_POINT('Ctrl Pts',(-0.0892078935221977,1.79031373191127,
7.52535182891117));
#48280=CARTESIAN_POINT('Ctrl Pts',(-0.091243820050598,1.79091093840867,
7.52522223193371));
#48281=CARTESIAN_POINT('Ctrl Pts',(-0.0917751468354167,1.79106828406568,
7.52518833999142));
#48282=CARTESIAN_POINT('Ctrl Pts',(-0.0926730664815594,1.79133671241478,
7.52513094405815));
#48283=CARTESIAN_POINT('Ctrl Pts',(-0.0930398732411064,1.79144708016412,
7.52510746347001));
#48284=CARTESIAN_POINT('Ctrl Pts',(-0.0937445739298334,1.7916604870061,
7.52506228750086));
#48285=CARTESIAN_POINT('Ctrl Pts',(-0.0940824971307662,1.79176342827843,
7.52504059534894));
#48286=CARTESIAN_POINT('Ctrl Pts',(-0.0948773456276642,1.79200699120386,
7.52498950329017));
#48287=CARTESIAN_POINT('Ctrl Pts',(-0.0953341277067271,1.79214807411492,
7.52496008829877));
#48288=CARTESIAN_POINT('Ctrl Pts',(-0.0962761231922259,1.79244131891022,
7.52489931628724));
#48289=CARTESIAN_POINT('Ctrl Pts',(-0.0967612934914672,1.79259361378182,
7.52486795496452));
#48290=CARTESIAN_POINT('Ctrl Pts',(-0.0993671534427551,1.79341837305484,
7.5246991825705));
#48291=CARTESIAN_POINT('Ctrl Pts',(-0.101481155332473,1.7941116218667,7.52456108919647));
#48292=CARTESIAN_POINT('Ctrl Pts',(-0.106910936629241,1.795954702199,7.52420328642237));
#48293=CARTESIAN_POINT('Ctrl Pts',(-0.110215347118491,1.79713688375507,
7.52398252026518));
#48294=CARTESIAN_POINT('Ctrl Pts',(-0.123256843566522,1.80204428469662,
7.52309891674368));
#48295=CARTESIAN_POINT('Ctrl Pts',(-0.132829150366764,1.80618673115128,
7.522422561808));
#48296=CARTESIAN_POINT('Ctrl Pts',(-0.148908090752129,1.81409142863004,
7.52123918277111));
#48297=CARTESIAN_POINT('Ctrl Pts',(-0.155515365740656,1.81763092905609,
7.52073843167385));
#48298=CARTESIAN_POINT('Ctrl Pts',(-0.168562369622535,1.82521708521451,
7.51972297983916));
#48299=CARTESIAN_POINT('Ctrl Pts',(-0.174994489767446,1.82926794067524,
7.51920848888541));
#48300=CARTESIAN_POINT('Ctrl Pts',(-0.187441691855888,1.83773605815151,
7.5181898347031));
#48301=CARTESIAN_POINT('Ctrl Pts',(-0.193458833235073,1.84214258220365,
7.5176859579647));
#48302=CARTESIAN_POINT('Ctrl Pts',(-0.203570969802908,1.85010135992561,
7.51682453662116));
#48303=CARTESIAN_POINT('Ctrl Pts',(-0.207739287428554,1.85355555682766,
7.51646488231769));
#48304=CARTESIAN_POINT('Ctrl Pts',(-0.212515825302974,1.85772112144741,
7.51604902183058));
#48305=CARTESIAN_POINT('Ctrl Pts',(-0.213210247398883,1.85833200163361,
7.51598846870124));
#48306=CARTESIAN_POINT('Ctrl Pts',(-0.214971466007757,1.85989483835236,
7.5158346700473));
#48307=CARTESIAN_POINT('Ctrl Pts',(-0.216034585987816,1.86085093008981,
7.51574162411408));
#48308=CARTESIAN_POINT('Ctrl Pts',(-0.220696159768779,1.86509965827603,
7.51533283979826));
#48309=CARTESIAN_POINT('Ctrl Pts',(-0.224226190465064,1.86846687622728,
7.51502116480095));
#48310=CARTESIAN_POINT('Ctrl Pts',(-0.228078878583547,1.87231266928341,
7.51467995886498));
#48311=CARTESIAN_POINT('Ctrl Pts',(-0.228478062748095,1.87271324218259,
7.51464459312363));
#48312=CARTESIAN_POINT('Ctrl Pts',(-0.229075844019567,1.87331626936495,
7.5145916164118));
#48313=CARTESIAN_POINT('Ctrl Pts',(-0.22927522902502,1.87351793579856,7.51457394373858));
#48314=CARTESIAN_POINT('Ctrl Pts',(-0.229619274895249,1.87386683828749,
7.51454344462709));
#48315=CARTESIAN_POINT('Ctrl Pts',(-0.229764060532985,1.87401395017069,
7.51453060829693));
#48316=CARTESIAN_POINT('Ctrl Pts',(-0.230064824307084,1.87432013409637,
7.51450394079749));
#48317=CARTESIAN_POINT('Ctrl Pts',(-0.230220778636816,1.87447922858003,
7.51449011156606));
#48318=CARTESIAN_POINT('Ctrl Pts',(-0.230590386026518,1.87485706097979,
7.5144573330169));
#48319=CARTESIAN_POINT('Ctrl Pts',(-0.230803893717613,1.87507594222682,
7.51443839521842));
#48320=CARTESIAN_POINT('Ctrl Pts',(-0.231253604834724,1.87553828624729,
7.51439849951627));
#48321=CARTESIAN_POINT('Ctrl Pts',(-0.231489736260967,1.8757818189839,7.51437754723012));
#48322=CARTESIAN_POINT('Ctrl Pts',(-0.233345248485676,1.87770154601116,
7.5142128681196));
#48323=CARTESIAN_POINT('Ctrl Pts',(-0.234946842027292,1.87939494610053,
7.5140705035166));
#48324=CARTESIAN_POINT('Ctrl Pts',(-0.244971942730091,1.89022773659585,
7.51317680826665));
#48325=CARTESIAN_POINT('Ctrl Pts',(-0.252880151030457,1.89983168073971,
7.51245997667805));
#48326=CARTESIAN_POINT('Ctrl Pts',(-0.262793871626641,1.9133997002042,7.51150813021452));
#48327=CARTESIAN_POINT('Ctrl Pts',(-0.26530118673752,1.91698204352252,7.51126216520915));
#48328=CARTESIAN_POINT('Ctrl Pts',(-0.270338993073633,1.92450101960656,
7.51075461215123));
#48329=CARTESIAN_POINT('Ctrl Pts',(-0.272858184186224,1.92844395931527,
7.5104931973824));
#48330=CARTESIAN_POINT('Ctrl Pts',(-0.289000375558909,1.95496463270848,
7.50875785285587));
#48331=CARTESIAN_POINT('Ctrl Pts',(-0.299891877787051,1.97908236426809,
7.50727732056974));
#48332=CARTESIAN_POINT('Ctrl Pts',(-0.308198753504487,2.00578081184131,
7.50558244820183));
#48333=CARTESIAN_POINT('Ctrl Pts',(-0.308661949323304,2.00730950439274,
7.50548526057534));
#48334=CARTESIAN_POINT('Ctrl Pts',(-0.309289288275958,2.0094367796197,7.50534979821011));
#48335=CARTESIAN_POINT('Ctrl Pts',(-0.309463100668061,2.01003250562389,
7.50531183930185));
#48336=CARTESIAN_POINT('Ctrl Pts',(-0.309738690007361,2.01098731083547,
7.50525096096381));
#48337=CARTESIAN_POINT('Ctrl Pts',(-0.309841566292714,2.01134607332355,
7.50522807740225));
#48338=CARTESIAN_POINT('Ctrl Pts',(-0.310052361187806,2.01208603123744,
7.50518086075317));
#48339=CARTESIAN_POINT('Ctrl Pts',(-0.310160200518773,2.01246724845129,
7.50515652512878));
#48340=CARTESIAN_POINT('Ctrl Pts',(-0.310409172756363,2.01335361411052,
7.50509991841269));
#48341=CARTESIAN_POINT('Ctrl Pts',(-0.31054977567526,2.01385890909759,7.50506763015492));
#48342=CARTESIAN_POINT('Ctrl Pts',(-0.310841336687314,2.01491670506265,
7.50499999828144));
#48343=CARTESIAN_POINT('Ctrl Pts',(-0.310992056538391,2.01546926929101,
7.50496464704371));
#48344=CARTESIAN_POINT('Ctrl Pts',(-0.311390816912086,2.0169466938652,7.50487006571209));
#48345=CARTESIAN_POINT('Ctrl Pts',(-0.311636208425057,2.01787225752665,
7.50481074990936));
#48346=CARTESIAN_POINT('Ctrl Pts',(-0.318807568914593,2.04541604167657,
7.50304362771498));
#48347=CARTESIAN_POINT('Ctrl Pts',(-0.32229988735354,2.07280360298413,7.50121750797054));
#48348=CARTESIAN_POINT('Ctrl Pts',(-0.322274866506699,2.10029333102401,
7.49935788809917));
#48349=CARTESIAN_POINT('',(-0.322274930854165,2.09978888878902,7.24958594529397));
#48350=CARTESIAN_POINT('Ctrl Pts',(-0.3222748664569,2.10029338573071,7.49935788439838));
#48351=CARTESIAN_POINT('Ctrl Pts',(-0.322256148867363,2.12085406076409,
7.49796699976951));
#48352=CARTESIAN_POINT('Ctrl Pts',(-0.32026987284514,2.14136841321006,7.49656915266215));
#48353=CARTESIAN_POINT('Ctrl Pts',(-0.316036440817217,2.16312446084035,
7.49515703326928));
#48354=CARTESIAN_POINT('Ctrl Pts',(-0.315719530582268,2.16469086279529,
7.49505578198484));
#48355=CARTESIAN_POINT('Ctrl Pts',(-0.315246160168358,2.16694423279244,
7.49491079344328));
#48356=CARTESIAN_POINT('Ctrl Pts',(-0.315099084757041,2.16763311771638,
7.4948665587458));
#48357=CARTESIAN_POINT('Ctrl Pts',(-0.314867627852968,2.16870009180598,
7.49479819198427));
#48358=CARTESIAN_POINT('Ctrl Pts',(-0.314784822419493,2.16907851519781,
7.49477397283448));
#48359=CARTESIAN_POINT('Ctrl Pts',(-0.314645821839494,2.169708312048,7.49473371422418));
#48360=CARTESIAN_POINT('Ctrl Pts',(-0.314590007564058,2.1699597678068,7.49471765325297));
#48361=CARTESIAN_POINT('Ctrl Pts',(-0.314480012267058,2.17045252779108,
7.49468620532467));
#48362=CARTESIAN_POINT('Ctrl Pts',(-0.314425854843617,2.1706938370333,7.49467081702622));
#48363=CARTESIAN_POINT('Ctrl Pts',(-0.3143232702153,2.17114847348537,7.49464184787286));
#48364=CARTESIAN_POINT('Ctrl Pts',(-0.314274903972807,2.17136181199602,
7.49462826367718));
#48365=CARTESIAN_POINT('Ctrl Pts',(-0.314164558954814,2.17184624453556,
7.49459743937047));
#48366=CARTESIAN_POINT('Ctrl Pts',(-0.3141024466065,2.17211730717617,7.49458020709278));
#48367=CARTESIAN_POINT('Ctrl Pts',(-0.313913245118711,2.17293811440616,
7.49452807148614));
#48368=CARTESIAN_POINT('Ctrl Pts',(-0.313785062160527,2.17348760963862,
7.49449323094113));
#48369=CARTESIAN_POINT('Ctrl Pts',(-0.312880417515829,2.17732012028061,
7.49425064696944));
#48370=CARTESIAN_POINT('Ctrl Pts',(-0.312053854676782,2.1805912565325,7.49404572263869));
#48371=CARTESIAN_POINT('Ctrl Pts',(-0.306216681283326,2.20225387933492,
7.49269916672607));
#48372=CARTESIAN_POINT('Ctrl Pts',(-0.299633534603359,2.22018505556726,
7.49163389924475));
#48373=CARTESIAN_POINT('Ctrl Pts',(-0.289457747551807,2.24176878259547,
7.49029993250223));
#48374=CARTESIAN_POINT('Ctrl Pts',(-0.287316058560702,2.2460604585875,7.4900320691688));
#48375=CARTESIAN_POINT('Ctrl Pts',(-0.282909093467116,2.25441915591365,
7.48950273342651));
#48376=CARTESIAN_POINT('Ctrl Pts',(-0.280649907131427,2.25848804179969,
7.48924137168973));
#48377=CARTESIAN_POINT('Ctrl Pts',(-0.2717069996401,2.27380337679313,7.48823955893468));
#48378=CARTESIAN_POINT('Ctrl Pts',(-0.264429468513943,2.28468706850848,
7.48748912588319));
#48379=CARTESIAN_POINT('Ctrl Pts',(-0.252879255027259,2.29987309179203,
7.48635933114148));
#48380=CARTESIAN_POINT('Ctrl Pts',(-0.249114815842532,2.30454576941058,
7.48599934154322));
#48381=CARTESIAN_POINT('Ctrl Pts',(-0.244780983532403,2.3096280239124,7.48559262678683));
#48382=CARTESIAN_POINT('Ctrl Pts',(-0.244337990561368,2.31014419969589,
7.48555114017175));
#48383=CARTESIAN_POINT('Ctrl Pts',(-0.243500167241692,2.31111420138257,
7.48547283803754));
#48384=CARTESIAN_POINT('Ctrl Pts',(-0.243105693402326,2.31156833245967,
7.48543603732991));
#48385=CARTESIAN_POINT('Ctrl Pts',(-0.242439786592579,2.31233062459253,
7.48537402463752));
#48386=CARTESIAN_POINT('Ctrl Pts',(-0.242169030773929,2.31263937733743,
7.4853488408685));
#48387=CARTESIAN_POINT('Ctrl Pts',(-0.241633748075659,2.31324743133717,
7.48529911212876));
#48388=CARTESIAN_POINT('Ctrl Pts',(-0.241369253353059,2.31354676001872,
7.48527456852713));
#48389=CARTESIAN_POINT('Ctrl Pts',(-0.240787036270638,2.31420319152479,
7.48522060400899));
#48390=CARTESIAN_POINT('Ctrl Pts',(-0.240469074986136,2.31456008031968,
7.48519117309404));
#48391=CARTESIAN_POINT('Ctrl Pts',(-0.239365751913833,2.31579294838065,
7.48508918597513));
#48392=CARTESIAN_POINT('Ctrl Pts',(-0.23857639527869,2.31666532559936,7.4850164615074));
#48393=CARTESIAN_POINT('Ctrl Pts',(-0.230690068668203,2.32528574526313,
7.48429221632307));
#48394=CARTESIAN_POINT('Ctrl Pts',(-0.223223729345604,2.33268584008681,
7.48362484107357));
#48395=CARTESIAN_POINT('Ctrl Pts',(-0.203788037593394,2.35015147042133,
7.48192838818911));
#48396=CARTESIAN_POINT('Ctrl Pts',(-0.191423099767726,2.35973529640472,
7.4808829546149));
#48397=CARTESIAN_POINT('Ctrl Pts',(-0.166958339490506,2.37599871630057,
7.4788978917401));
#48398=CARTESIAN_POINT('Ctrl Pts',(-0.155027370340201,2.38287260654162,
7.47796288691117));
#48399=CARTESIAN_POINT('Ctrl Pts',(-0.135936493037989,2.39229990637292,
7.47654621627203));
#48400=CARTESIAN_POINT('Ctrl Pts',(-0.129064034909462,2.39539881158071,
7.47605130926519));
#48401=CARTESIAN_POINT('Ctrl Pts',(-0.120069346449577,2.39908073987667,
7.47542816131802));
#48402=CARTESIAN_POINT('Ctrl Pts',(-0.11804153945444,2.39988686612559,7.47528925393823));
#48403=CARTESIAN_POINT('Ctrl Pts',(-0.114763121449796,2.40115174787086,
7.47506738763831));
#48404=CARTESIAN_POINT('Ctrl Pts',(-0.113517617810498,2.40162344054064,
7.47498372271904));
#48405=CARTESIAN_POINT('Ctrl Pts',(-0.111997193671826,2.40218849819525,
7.47488238022768));
#48406=CARTESIAN_POINT('Ctrl Pts',(-0.111725049195026,2.40228922113732,
7.47486427140049));
#48407=CARTESIAN_POINT('Ctrl Pts',(-0.111198881186578,2.40248315269234,
7.47482931938073));
#48408=CARTESIAN_POINT('Ctrl Pts',(-0.110944875725595,2.40257640917852,
7.47481247334759));
#48409=CARTESIAN_POINT('Ctrl Pts',(-0.110505523445552,2.40273708694421,
7.47478338171066));
#48410=CARTESIAN_POINT('Ctrl Pts',(-0.110320232472824,2.40280465787592,
7.47477112711516));
#48411=CARTESIAN_POINT('Ctrl Pts',(-0.109933632884527,2.4029452390131,7.47474558868799));
#48412=CARTESIAN_POINT('Ctrl Pts',(-0.109732314139043,2.40301821845265,
7.47473230673486));
#48413=CARTESIAN_POINT('Ctrl Pts',(-0.109175432523116,2.40321946414261,
7.47469561317175));
#48414=CARTESIAN_POINT('Ctrl Pts',(-0.108819715038369,2.40334730610965,
7.47467222698715));
#48415=CARTESIAN_POINT('Ctrl Pts',(-0.107422883494162,2.40384654280272,
7.47458059674391));
#48416=CARTESIAN_POINT('Ctrl Pts',(-0.106380070833977,2.40421321155415,
7.47451263094273));
#48417=CARTESIAN_POINT('Ctrl Pts',(-0.0863796914773394,2.41113022973626,
7.47321715804945));
#48418=CARTESIAN_POINT('Ctrl Pts',(-0.0668500557929338,2.41590315961686,
7.47208915106601));
#48419=CARTESIAN_POINT('Ctrl Pts',(-0.029756093109937,2.42137141781679,
7.46999106991032));
#48420=CARTESIAN_POINT('Ctrl Pts',(-0.0123341175448777,2.42251022386957,
7.46902278526492));
#48421=CARTESIAN_POINT('Ctrl Pts',(0.0158488738851317,2.42206473698776,
7.46739919359314));
#48422=CARTESIAN_POINT('Ctrl Pts',(0.0265879506236351,2.42135638527742,
7.46676748368368));
#48423=CARTESIAN_POINT('Ctrl Pts',(0.0396630146128743,2.41983405270604,
7.46597331126771));
#48424=CARTESIAN_POINT('Ctrl Pts',(0.042052001768259,2.41952872274597,7.46582718977463));
#48425=CARTESIAN_POINT('Ctrl Pts',(0.0449529182336699,2.41912486864711,
7.46564845260593));
#48426=CARTESIAN_POINT('Ctrl Pts',(0.0454683659394383,2.41905183644757,
7.46561664366199));
#48427=CARTESIAN_POINT('Ctrl Pts',(0.0464654502293034,2.41890809731526,
7.46555501431353));
#48428=CARTESIAN_POINT('Ctrl Pts',(0.0469471082955741,2.4188375473761,7.46552519894448));
#48429=CARTESIAN_POINT('Ctrl Pts',(0.0477790582931503,2.41871376304104,
7.46547362275445));
#48430=CARTESIAN_POINT('Ctrl Pts',(0.0481294266619008,2.4186610416269,7.46545187821662));
#48431=CARTESIAN_POINT('Ctrl Pts',(0.0488544601962142,2.41855071972302,
7.46540683191041));
#48432=CARTESIAN_POINT('Ctrl Pts',(0.0492291119619132,2.41849303579615,
7.46538352752728));
#48433=CARTESIAN_POINT('Ctrl Pts',(0.0501369425737913,2.41835161991995,
7.46532699138407));
#48434=CARTESIAN_POINT('Ctrl Pts',(0.0506700131728285,2.41826720955152,
7.46529373815168));
#48435=CARTESIAN_POINT('Ctrl Pts',(0.0526563749244304,2.41794755731416,
7.46516961848217));
#48436=CARTESIAN_POINT('Ctrl Pts',(0.0541082435990096,2.41770369982331,
7.46507847896578));
#48437=CARTESIAN_POINT('Ctrl Pts',(0.0783998173217289,2.41345231953319,
7.46354645000756));
#48438=CARTESIAN_POINT('Ctrl Pts',(0.100738229690627,2.40700209701137,7.46202394020688));
#48439=CARTESIAN_POINT('Ctrl Pts',(0.139974304090959,2.39092586057203,7.45916737392671));
#48440=CARTESIAN_POINT('Ctrl Pts',(0.157073803193341,2.38206120185136,7.45785326633061));
#48441=CARTESIAN_POINT('Ctrl Pts',(0.176562180793679,2.36963328845313,7.45633337378648));
#48442=CARTESIAN_POINT('Ctrl Pts',(0.179804689857287,2.36748194349376,7.4560798043916));
#48443=CARTESIAN_POINT('Ctrl Pts',(0.185168879024069,2.36378126602448,7.45566014921166));
#48444=CARTESIAN_POINT('Ctrl Pts',(0.187311954218957,2.3622638039696,7.4554924455028));
#48445=CARTESIAN_POINT('Ctrl Pts',(0.190257157140956,2.36012385369726,7.45526217518852));
#48446=CARTESIAN_POINT('Ctrl Pts',(0.191075186377482,2.35952356024068,7.45519823978699));
#48447=CARTESIAN_POINT('Ctrl Pts',(0.192478318089588,2.35848367110059,7.45508863166866));
#48448=CARTESIAN_POINT('Ctrl Pts',(0.193064777710871,2.35804593155583,7.45504283681663));
#48449=CARTESIAN_POINT('Ctrl Pts',(0.193899626310528,2.35741835261863,7.45497767713172));
#48450=CARTESIAN_POINT('Ctrl Pts',(0.194149232494296,2.35723014767346,7.45495819943117));
#48451=CARTESIAN_POINT('Ctrl Pts',(0.194577250795883,2.3569064407297,7.45492480699595));
#48452=CARTESIAN_POINT('Ctrl Pts',(0.194755795848042,2.35677111558819,7.45491087978578));
#48453=CARTESIAN_POINT('Ctrl Pts',(0.195097331117153,2.35651169365386,7.45488424319191));
#48454=CARTESIAN_POINT('Ctrl Pts',(0.195260343893612,2.35638762780864,7.45487153164527));
#48455=CARTESIAN_POINT('Ctrl Pts',(0.195643937640691,2.35609510405909,7.4548416237388));
#48456=CARTESIAN_POINT('Ctrl Pts',(0.195864419927916,2.35592651614522,7.45482443659565));
#48457=CARTESIAN_POINT('Ctrl Pts',(0.19651466827868,2.35542798268336,7.45477375709313));
#48458=CARTESIAN_POINT('Ctrl Pts',(0.196943823100979,2.35509723585095,7.45474032092688));
#48459=CARTESIAN_POINT('Ctrl Pts',(0.200684744625027,2.35219906486205,7.45444894098944));
#48460=CARTESIAN_POINT('Ctrl Pts',(0.203947168455363,2.34956821030212,7.45419538982303));
#48461=CARTESIAN_POINT('Ctrl Pts',(0.207909278925225,2.34624351847994,7.45388685497364));
#48462=CARTESIAN_POINT('Ctrl Pts',(0.20865814578828,2.3456092768959,7.45382851242839));
#48463=CARTESIAN_POINT('Ctrl Pts',(0.209524006723595,2.34486913057721,7.45376100769521));
#48464=CARTESIAN_POINT('Ctrl Pts',(0.209643825882845,2.34476655566586,7.45375166522729));
#48465=CARTESIAN_POINT('Ctrl Pts',(0.218689053673119,2.33701159333229,7.45304631180361));
#48466=CARTESIAN_POINT('Ctrl Pts',(0.227189922892183,2.32887591523492,7.4523770134302));
#48467=CARTESIAN_POINT('Ctrl Pts',(0.248365887101111,2.30626434631992,7.45063386979542));
#48468=CARTESIAN_POINT('Ctrl Pts',(0.260222348964725,2.29108875917186,7.44957440173897));
#48469=CARTESIAN_POINT('Ctrl Pts',(0.274087031677675,2.26963909701135,7.44811295759442));
#48470=CARTESIAN_POINT('Ctrl Pts',(0.277361063397851,2.26423141685269,7.44774753750449));
#48471=CARTESIAN_POINT('Ctrl Pts',(0.284404303374136,2.25178619502868,7.44690917036536));
#48472=CARTESIAN_POINT('Ctrl Pts',(0.288075151265587,2.24469812598262,7.44643345189702));
#48473=CARTESIAN_POINT('Ctrl Pts',(0.291969671682161,2.23644123099065,7.44587833913174));
#48474=CARTESIAN_POINT('Ctrl Pts',(0.292454786025875,2.23539828940314,7.44580820716518));
#48475=CARTESIAN_POINT('Ctrl Pts',(0.293156055662486,2.2338692854938,7.44570536061037));
#48476=CARTESIAN_POINT('Ctrl Pts',(0.293376611096474,2.23338524141147,7.44567279767047));
#48477=CARTESIAN_POINT('Ctrl Pts',(0.293759832181104,2.23253865292845,7.44561583698913));
#48478=CARTESIAN_POINT('Ctrl Pts',(0.293923028004244,2.23217634860174,7.44559145752605));
#48479=CARTESIAN_POINT('Ctrl Pts',(0.294237347332648,2.23147508050822,7.44554426361299));
#48480=CARTESIAN_POINT('Ctrl Pts',(0.294388556292057,2.23113615551207,7.44552145213994));
#48481=CARTESIAN_POINT('Ctrl Pts',(0.294746207760265,2.23033076706264,7.44546723883642));
#48482=CARTESIAN_POINT('Ctrl Pts',(0.294952128409696,2.22986407422381,7.44543581919425));
#48483=CARTESIAN_POINT('Ctrl Pts',(0.295674766276936,2.22821572262734,7.44532482639256));
#48484=CARTESIAN_POINT('Ctrl Pts',(0.296185492182256,2.22703146494067,7.44524504896239));
#48485=CARTESIAN_POINT('Ctrl Pts',(0.304054344869696,2.20847993073549,7.44399469654815));
#48486=CARTESIAN_POINT('Ctrl Pts',(0.309879654226826,2.19050586986265,7.44277131467218));
#48487=CARTESIAN_POINT('Ctrl Pts',(0.318939143645388,2.15105428844335,7.44006934895851));
#48488=CARTESIAN_POINT('Ctrl Pts',(0.321645163145963,2.1295476166933,7.43858568653543));
#48489=CARTESIAN_POINT('Ctrl Pts',(0.322396680236011,2.09902481245934,7.4365598366538));
#48490=CARTESIAN_POINT('Ctrl Pts',(0.322246503158223,2.09011092691619,7.43597847884219));
#48491=CARTESIAN_POINT('Ctrl Pts',(0.321674558105754,2.08031590912717,7.4353588626651));
#48492=CARTESIAN_POINT('Ctrl Pts',(0.321618362843058,2.07941812708317,7.43530224939695));
#48493=CARTESIAN_POINT('Ctrl Pts',(0.321513969064208,2.07785529637812,7.43520402412813));
#48494=CARTESIAN_POINT('Ctrl Pts',(0.321467464533293,2.07719014539081,7.43516232148929));
#48495=CARTESIAN_POINT('Ctrl Pts',(0.321397069694121,2.07622629606025,7.43510204505617));
#48496=CARTESIAN_POINT('Ctrl Pts',(0.321374826981954,2.07592748473781,7.43508337963269));
#48497=CARTESIAN_POINT('Ctrl Pts',(0.321335399694965,2.07540760906809,7.43505094304603));
#48498=CARTESIAN_POINT('Ctrl Pts',(0.321318403685415,2.07518653101374,7.43503716121823));
#48499=CARTESIAN_POINT('Ctrl Pts',(0.321285021172363,2.07475808916135,7.4350104757295));
#48500=CARTESIAN_POINT('Ctrl Pts',(0.321268662115585,2.07455072426189,7.43499757053294));
#48501=CARTESIAN_POINT('Ctrl Pts',(0.321229042514617,2.07405463875162,7.43496672189154));
#48502=CARTESIAN_POINT('Ctrl Pts',(0.32120559341837,2.07376593276972,7.43494878911579));
#48503=CARTESIAN_POINT('Ctrl Pts',(0.321120017701663,2.07272963877179,7.43488449151448));
#48504=CARTESIAN_POINT('Ctrl Pts',(0.321055669488469,2.07198222910308,7.43483825079642));
#48505=CARTESIAN_POINT('Ctrl Pts',(0.319967583479091,2.05984025664069,7.43408911240768));
#48506=CARTESIAN_POINT('Ctrl Pts',(0.318340287821569,2.04850644511515,7.43341925405515));
#48507=CARTESIAN_POINT('Ctrl Pts',(0.311727611273277,2.0151770601363,7.4314744492046));
#48508=CARTESIAN_POINT('Ctrl Pts',(0.305035414923231,1.99359268157072,7.43024399081669));
#48509=CARTESIAN_POINT('Ctrl Pts',(0.293109356794663,1.96580857784914,7.42852521655843));
#48510=CARTESIAN_POINT('Ctrl Pts',(0.289820706986139,1.95884625418442,7.42808278107872));
#48511=CARTESIAN_POINT('Ctrl Pts',(0.282339133133295,1.94437331146014,7.42713050809979));
#48512=CARTESIAN_POINT('Ctrl Pts',(0.278088604211423,1.93689953913959,7.42661919375738));
#48513=CARTESIAN_POINT('Ctrl Pts',(0.272900112816633,1.92857015848397,7.42602278861851));
#48514=CARTESIAN_POINT('Ctrl Pts',(0.272249616564854,1.92753896569388,7.42594847575003));
#48515=CARTESIAN_POINT('Ctrl Pts',(0.271299672872987,1.92605184502713,7.42584060437575));
#48516=CARTESIAN_POINT('Ctrl Pts',(0.271004889310201,1.92559293854994,7.42580721922041));
#48517=CARTESIAN_POINT('Ctrl Pts',(0.270492082739039,1.92479906239208,7.42574929520246));
#48518=CARTESIAN_POINT('Ctrl Pts',(0.270274598308973,1.92446374485652,7.42572477647119));
#48519=CARTESIAN_POINT('Ctrl Pts',(0.269855777399204,1.92382063030852,7.42567764947841));
#48520=CARTESIAN_POINT('Ctrl Pts',(0.269654536532754,1.92351277149273,7.42565504482042));
#48521=CARTESIAN_POINT('Ctrl Pts',(0.269180042305668,1.92278959509691,7.42560183905484));
#48522=CARTESIAN_POINT('Ctrl Pts',(0.268906354645396,1.92237456486049,7.42557122167855));
#48523=CARTESIAN_POINT('Ctrl Pts',(0.268097555778,1.92115422543596,7.42548095069198));
#48524=CARTESIAN_POINT('Ctrl Pts',(0.267559783040139,1.92035069451732,7.42542119694882));
#48525=CARTESIAN_POINT('Ctrl Pts',(0.262847412993501,1.91337764506534,7.42489988256722));
#48526=CARTESIAN_POINT('Ctrl Pts',(0.258463992951908,1.90735261399201,7.42443041024048));
#48527=CARTESIAN_POINT('Ctrl Pts',(0.250763755561469,1.8975049543118,7.42362941149909));
#48528=CARTESIAN_POINT('Ctrl Pts',(0.247558409786082,1.89359860930794,7.42330221495336));
#48529=CARTESIAN_POINT('Ctrl Pts',(0.227274373922959,1.87003099896178,7.42126938137369));
#48530=CARTESIAN_POINT('Ctrl Pts',(0.207956845486481,1.85242568746729,7.41948098683476));
#48531=CARTESIAN_POINT('Ctrl Pts',(0.179563963667948,1.83224002846542,7.41715202669159));
#48532=CARTESIAN_POINT('Ctrl Pts',(0.172185123793336,1.82743637720393,7.41657118559141));
#48533=CARTESIAN_POINT('Ctrl Pts',(0.161585891772989,1.8211387134216,7.41577940151565));
#48534=CARTESIAN_POINT('Ctrl Pts',(0.158523928902531,1.81938677137533,7.41555543760338));
#48535=CARTESIAN_POINT('Ctrl Pts',(0.154973502691873,1.81743201698207,7.41530171542751));
#48536=CARTESIAN_POINT('Ctrl Pts',(0.154512715852589,1.81717978818243,7.4152689006621));
#48537=CARTESIAN_POINT('Ctrl Pts',(0.153812099487223,1.81679850310144,7.41521918209965));
#48538=CARTESIAN_POINT('Ctrl Pts',(0.153572722482009,1.81666862386063,7.41520222597913));
#48539=CARTESIAN_POINT('Ctrl Pts',(0.153142985802857,1.81643616541774,7.41517184189014));
#48540=CARTESIAN_POINT('Ctrl Pts',(0.152952687946802,1.81633347459669,7.41515840677859));
#48541=CARTESIAN_POINT('Ctrl Pts',(0.152541771750175,1.81611226476928,7.41512943847377));
#48542=CARTESIAN_POINT('Ctrl Pts',(0.15232111922182,1.81599381171681,7.41511390954674));
#48543=CARTESIAN_POINT('Ctrl Pts',(0.151727283766248,1.81567591373809,7.4150721873302));
#48544=CARTESIAN_POINT('Ctrl Pts',(0.151353844124926,1.81547694550141,7.41504602446059));
#48545=CARTESIAN_POINT('Ctrl Pts',(0.149641106194355,1.81456872682307,7.41492636783102));
#48546=CARTESIAN_POINT('Ctrl Pts',(0.14829717899231,1.81386817848286,7.41483341810335));
#48547=CARTESIAN_POINT('Ctrl Pts',(0.120073828011739,1.79940847331795,7.41289997768157));
#48548=CARTESIAN_POINT('Ctrl Pts',(0.0913925902575469,1.78948255503498,
7.4112758604954));
#48549=CARTESIAN_POINT('Ctrl Pts',(0.0510839991317009,1.78161411153394,
7.40895832228526));
#48550=CARTESIAN_POINT('Ctrl Pts',(0.0403259421009782,1.78007353913178,
7.40833791785853));
#48551=CARTESIAN_POINT('Ctrl Pts',(0.021815880439857,1.7783713901974,7.40724988394123));
#48552=CARTESIAN_POINT('Ctrl Pts',(0.0140980684805651,1.77794080501521,
7.40679024682563));
#48553=CARTESIAN_POINT('Ctrl Pts',(0.00476685903712009,1.77775625320704,
7.40622443236651));
#48554=CARTESIAN_POINT('Ctrl Pts',(0.00316084701995865,1.77773649881983,
7.40612669214987));
#48555=CARTESIAN_POINT('Ctrl Pts',(0.000952368904519933,1.77772584416042,
7.4059917745739));
#48556=CARTESIAN_POINT('Ctrl Pts',(0.000349957359429053,1.77772462698692,
7.40595492045286));
#48557=CARTESIAN_POINT('Ctrl Pts',(-0.000663289832376256,1.77772542070407,
7.4058928430748));
#48558=CARTESIAN_POINT('Ctrl Pts',(-0.00107412630767911,1.77772652814113,
7.40586764816554));
#48559=CARTESIAN_POINT('Ctrl Pts',(-0.00188425704504076,1.77773026104912,
7.40581791704918));
#48560=CARTESIAN_POINT('Ctrl Pts',(-0.00228355084812315,1.77773284303032,
7.40579338224959));
#48561=CARTESIAN_POINT('Ctrl Pts',(-0.00316025595985665,1.77774014157586,
7.40573946056711));
#48562=CARTESIAN_POINT('Ctrl Pts',(-0.00363766303676176,1.77774517695929,
7.40571006374594));
#48563=CARTESIAN_POINT('Ctrl Pts',(-0.00528814499552276,1.77776625330087,
7.40560831521979));
#48564=CARTESIAN_POINT('Ctrl Pts',(-0.00646113167826603,1.77778763880269,
7.40553579630545));
#48565=CARTESIAN_POINT('Ctrl Pts',(-0.0180192627843161,1.77806150153445,
7.40481914240755));
#48566=CARTESIAN_POINT('Ctrl Pts',(-0.0283854975871893,1.77880953589107,
7.40415951578061));
#48567=CARTESIAN_POINT('Ctrl Pts',(-0.0543160398544716,1.7819457943076,
7.40246458473418));
#48568=CARTESIAN_POINT('Ctrl Pts',(-0.0697744874143692,1.78497597981778,
7.40141207689148));
#48569=CARTESIAN_POINT('Ctrl Pts',(-0.0998122426420859,1.79318389065096,
7.39930800134372));
#48570=CARTESIAN_POINT('Ctrl Pts',(-0.114366181895931,1.79830641822693,
7.39825972134003));
#48571=CARTESIAN_POINT('Ctrl Pts',(-0.135591841955927,1.80753485634069,
7.39672907835154));
#48572=CARTESIAN_POINT('Ctrl Pts',(-0.142572839622313,1.81087370443397,
7.39622558390925));
#48573=CARTESIAN_POINT('Ctrl Pts',(-0.15087120020387,1.81521637737996,7.395632696245));
#48574=CARTESIAN_POINT('Ctrl Pts',(-0.152309204673227,1.815982857558,7.39553016773378));
#48575=CARTESIAN_POINT('Ctrl Pts',(-0.154110048343997,1.81696034801517,
7.39540209529559));
#48576=CARTESIAN_POINT('Ctrl Pts',(-0.154478338858534,1.81716118649566,
7.39537592046855));
#48577=CARTESIAN_POINT('Ctrl Pts',(-0.155063011207673,1.8174815063136,7.39533439588912));
#48578=CARTESIAN_POINT('Ctrl Pts',(-0.155279647931368,1.81760051760154,
7.39531901621088));
#48579=CARTESIAN_POINT('Ctrl Pts',(-0.155687774342498,1.81782533705452,
7.39529005428929));
#48580=CARTESIAN_POINT('Ctrl Pts',(-0.155879291648286,1.81793109011507,
7.3952764687259));
#48581=CARTESIAN_POINT('Ctrl Pts',(-0.156314198211469,1.81817181738217,
7.39524562939809));
#48582=CARTESIAN_POINT('Ctrl Pts',(-0.156557519949924,1.81830691164196,
7.39522838349663));
#48583=CARTESIAN_POINT('Ctrl Pts',(-0.157185567195963,1.81865667382187,
7.39518388956498));
#48584=CARTESIAN_POINT('Ctrl Pts',(-0.157570029661558,1.81887181664303,
7.39515667191887));
#48585=CARTESIAN_POINT('Ctrl Pts',(-0.159858453728367,1.82015857381842,
7.39499477447028));
#48586=CARTESIAN_POINT('Ctrl Pts',(-0.161751978224847,1.82124877185239,
7.39486126629297));
#48587=CARTESIAN_POINT('Ctrl Pts',(-0.174017628969615,1.82847780356479,
7.39399842437981));
#48588=CARTESIAN_POINT('Ctrl Pts',(-0.18405070328038,1.83517582507081,7.39330179875718));
#48589=CARTESIAN_POINT('Ctrl Pts',(-0.199162291029895,1.84653894597844,
7.39222913160857));
#48590=CARTESIAN_POINT('Ctrl Pts',(-0.204506090248203,1.85083060498966,
7.39184481462303));
#48591=CARTESIAN_POINT('Ctrl Pts',(-0.219921744576921,1.86404132753134,
7.39070892830626));
#48592=CARTESIAN_POINT('Ctrl Pts',(-0.229576323321482,1.8734238163882,7.38996066094249));
#48593=CARTESIAN_POINT('Ctrl Pts',(-0.248461513796116,1.89422682883049,
7.38836275525745));
#48594=CARTESIAN_POINT('Ctrl Pts',(-0.257554822598136,1.90572917544507,
7.38751164783962));
#48595=CARTESIAN_POINT('Ctrl Pts',(-0.266719764257067,1.91910168910019,
7.3865333247983));
#48596=CARTESIAN_POINT('Ctrl Pts',(-0.267596255156557,1.92040079169268,
7.3864384064434));
#48597=CARTESIAN_POINT('Ctrl Pts',(-0.269117157659774,1.92269086813482,
7.38627127035067));
#48598=CARTESIAN_POINT('Ctrl Pts',(-0.269765661814303,1.92367909812705,
7.38619920709758));
#48599=CARTESIAN_POINT('Ctrl Pts',(-0.270698194424697,1.92511733562127,
7.38609440733066));
#48600=CARTESIAN_POINT('Ctrl Pts',(-0.270986573188863,1.9255645222124,7.38606183324483));
#48601=CARTESIAN_POINT('Ctrl Pts',(-0.271488384100493,1.92634692388116,
7.3860048595828));
#48602=CARTESIAN_POINT('Ctrl Pts',(-0.271702306769198,1.92668182426231,
7.38598047830991));
#48603=CARTESIAN_POINT('Ctrl Pts',(-0.272114786630695,1.92733021045796,
7.38593328562743));
#48604=CARTESIAN_POINT('Ctrl Pts',(-0.272313423004919,1.92764364539386,
7.38591047720357));
#48605=CARTESIAN_POINT('Ctrl Pts',(-0.272783729899214,1.92838860077905,
7.38585627857566));
#48606=CARTESIAN_POINT('Ctrl Pts',(-0.273054917859889,1.92882042333252,
7.38582487058257));
#48607=CARTESIAN_POINT('Ctrl Pts',(-0.273863835219354,1.93011530554338,
7.38573071464839));
#48608=CARTESIAN_POINT('Ctrl Pts',(-0.274398502031193,1.9309802624049,7.38566785401126));
#48609=CARTESIAN_POINT('Ctrl Pts',(-0.279601652634539,1.93948741660023,
7.3850498996918));
#48610=CARTESIAN_POINT('Ctrl Pts',(-0.283953360639575,1.94731785685706,
7.38448331429251));
#48611=CARTESIAN_POINT('Ctrl Pts',(-0.298619715273436,1.97650971785774,
7.38237605312307));
#48612=CARTESIAN_POINT('Ctrl Pts',(-0.306893409966522,1.99880857378941,
7.38076884517529));
#48613=CARTESIAN_POINT('Ctrl Pts',(-0.316887498560611,2.03876964914914,
7.37798522620881));
#48614=CARTESIAN_POINT('Ctrl Pts',(-0.319742721260156,2.05605004994587,
7.37681345156066));
#48615=CARTESIAN_POINT('Ctrl Pts',(-0.321261833893553,2.07444704097285,
7.37565202786818));
#48616=CARTESIAN_POINT('Ctrl Pts',(-0.32133741256755,2.07541571693818,7.37559112814168));
#48617=CARTESIAN_POINT('Ctrl Pts',(-0.321434005681985,2.07673036905404,
7.37550883516746));
#48618=CARTESIAN_POINT('Ctrl Pts',(-0.321458843523721,2.07707604623518,
7.37548723044815));
#48619=CARTESIAN_POINT('Ctrl Pts',(-0.321499305517873,2.0776521695738,7.37545127958592));
#48620=CARTESIAN_POINT('Ctrl Pts',(-0.321515239552147,2.0778825926075,7.37543691598533));
#48621=CARTESIAN_POINT('Ctrl Pts',(-0.32154603052663,2.07833492804234,7.37540874921072));
#48622=CARTESIAN_POINT('Ctrl Pts',(-0.321560905463228,2.07855683865426,
7.37539494505593));
#48623=CARTESIAN_POINT('Ctrl Pts',(-0.321593115302456,2.07904492979591,
7.37536461366112));
#48624=CARTESIAN_POINT('Ctrl Pts',(-0.321610349513846,2.07931111738218,
7.37534809211314));
#48625=CARTESIAN_POINT('Ctrl Pts',(-0.321669001228642,2.08023479618238,
7.37529083070595));
#48626=CARTESIAN_POINT('Ctrl Pts',(-0.321708733508872,2.08089239848766,
7.37525018514761));
#48627=CARTESIAN_POINT('Ctrl Pts',(-0.322080389763401,2.08737369330454,
7.37485073649377));
#48628=CARTESIAN_POINT('Ctrl Pts',(-0.322256185453299,2.09320570549333,
7.37450046333265));
#48629=CARTESIAN_POINT('Ctrl Pts',(-0.322274376855821,2.09931072574119,
7.37414039069863));
#48630=CARTESIAN_POINT('Ctrl Pts',(-0.322274842551218,2.09958174618492,
7.37412441958737));
#48631=CARTESIAN_POINT('Ctrl Pts',(-0.322278290200018,2.10712826112714,
7.37368007800356));
#48632=CARTESIAN_POINT('Ctrl Pts',(-0.322035241626426,2.11440222611218,
7.37326136337437));
#48633=CARTESIAN_POINT('Ctrl Pts',(-0.319419132538126,2.15323497249832,
7.37104886101296));
#48634=CARTESIAN_POINT('Ctrl Pts',(-0.312654214176339,2.18432051894227,
7.36933920997919));
#48635=CARTESIAN_POINT('Ctrl Pts',(-0.299421176891205,2.21933839096461,
7.36712088884723));
#48636=CARTESIAN_POINT('Ctrl Pts',(-0.297229201161761,2.22469758712452,
7.3667734060394));
#48637=CARTESIAN_POINT('Ctrl Pts',(-0.294496872142401,2.23089590572305,
7.36636102440279));
#48638=CARTESIAN_POINT('Ctrl Pts',(-0.294095433399209,2.23179537873788,
7.36630091956592));
#48639=CARTESIAN_POINT('Ctrl Pts',(-0.293483736966334,2.23314924869876,
7.36621005007693));
#48640=CARTESIAN_POINT('Ctrl Pts',(-0.293276530989509,2.23360502482712,
7.36617939034792));
#48641=CARTESIAN_POINT('Ctrl Pts',(-0.292904822714833,2.23441761354625,
7.36612460443478));
#48642=CARTESIAN_POINT('Ctrl Pts',(-0.292740728037082,2.23477461239872,
7.36610049233638));
#48643=CARTESIAN_POINT('Ctrl Pts',(-0.292393119059852,2.23552722878661,
7.36604956917819));
#48644=CARTESIAN_POINT('Ctrl Pts',(-0.292209453885833,2.23592277540167,
7.36602275294438));
#48645=CARTESIAN_POINT('Ctrl Pts',(-0.291721520536685,2.23696804298165,
7.36595174776038));
#48646=CARTESIAN_POINT('Ctrl Pts',(-0.291415885950898,2.23761712009997,
7.365907511581));
#48647=CARTESIAN_POINT('Ctrl Pts',(-0.290014994441877,2.24056660374801,
7.36570583464253));
#48648=CARTESIAN_POINT('Ctrl Pts',(-0.288894673052914,2.24285494171508,
7.36554752517551));
#48649=CARTESIAN_POINT('Ctrl Pts',(-0.283890170236317,2.25277732455363,
7.36485284545483));
#48650=CARTESIAN_POINT('Ctrl Pts',(-0.279729958162931,2.26026748869724,
7.36430684009744));
#48651=CARTESIAN_POINT('Ctrl Pts',(-0.267773658320616,2.27990730521597,
7.36281498674291));
#48652=CARTESIAN_POINT('Ctrl Pts',(-0.259452143329316,2.2917130106613,7.36185234121339));
#48653=CARTESIAN_POINT('Ctrl Pts',(-0.234796304168245,2.32213403456118,
7.35921017214327));
#48654=CARTESIAN_POINT('Ctrl Pts',(-0.217062901940522,2.33949266701768,
7.35751392852395));
#48655=CARTESIAN_POINT('Ctrl Pts',(-0.19640863781921,2.35551280017933,7.35586215333832));
#48656=CARTESIAN_POINT('Ctrl Pts',(-0.19529438906468,2.3563654536708,7.35577395969225));
#48657=CARTESIAN_POINT('Ctrl Pts',(-0.193842865654234,2.35746124331218,
7.35566029047177));
#48658=CARTESIAN_POINT('Ctrl Pts',(-0.193510661323753,2.35771102485451,
7.35563435763584));
#48659=CARTESIAN_POINT('Ctrl Pts',(-0.193000497357154,2.35809307004673,
7.35559465980004));
#48660=CARTESIAN_POINT('Ctrl Pts',(-0.192822884481934,2.3582257926835,7.35558086259655));
#48661=CARTESIAN_POINT('Ctrl Pts',(-0.192472112117746,2.35848734642757,
7.35555366079469));
#48662=CARTESIAN_POINT('Ctrl Pts',(-0.192298961230918,2.35861618610652,
7.35554025565808));
#48663=CARTESIAN_POINT('Ctrl Pts',(-0.191912071493919,2.35890346313909,
7.35551035304808));
#48664=CARTESIAN_POINT('Ctrl Pts',(-0.191698266364508,2.35906180939029,
7.35549386202222));
#48665=CARTESIAN_POINT('Ctrl Pts',(-0.191077273525782,2.35952053328038,
7.35544606170872));
#48666=CARTESIAN_POINT('Ctrl Pts',(-0.190669571831301,2.35982021868611,
7.35541480074855));
#48667=CARTESIAN_POINT('Ctrl Pts',(-0.187830833735565,2.3618965826768,7.35519796744824));
#48668=CARTESIAN_POINT('Ctrl Pts',(-0.185375605020601,2.36364015012853,
7.35501464890999));
#48669=CARTESIAN_POINT('Ctrl Pts',(-0.17765005402529,2.36896511163954,7.35444962176683));
#48670=CARTESIAN_POINT('Ctrl Pts',(-0.172297462719188,2.37242497771716,
7.35407492401959));
#48671=CARTESIAN_POINT('Ctrl Pts',(-0.153340559219655,2.38389613067127,
7.35279234112182));
#48672=CARTESIAN_POINT('Ctrl Pts',(-0.139252632784307,2.39106547286348,
7.35191539258484));
#48673=CARTESIAN_POINT('Ctrl Pts',(-0.101588582525585,2.4068694483464,7.34963142863199));
#48674=CARTESIAN_POINT('Ctrl Pts',(-0.0774340145900101,2.41383565326267,
7.34821703666872));
#48675=CARTESIAN_POINT('Ctrl Pts',(-0.0512172280476047,2.4181827870406,
7.34660539321477));
#48676=CARTESIAN_POINT('Ctrl Pts',(-0.0497145547213379,2.41842103156508,
7.34651279331844));
#48677=CARTESIAN_POINT('Ctrl Pts',(-0.0476692025243479,2.41873048522473,
7.3463864282776));
#48678=CARTESIAN_POINT('Ctrl Pts',(-0.0471279295340625,2.41881096802479,
7.34635295686699));
#48679=CARTESIAN_POINT('Ctrl Pts',(-0.0462093245374925,2.41894516647066,
7.34629609883186));
#48680=CARTESIAN_POINT('Ctrl Pts',(-0.045832096123273,2.41899959224447,
7.34627273471443));
#48681=CARTESIAN_POINT('Ctrl Pts',(-0.0451045850859807,2.41910323901535,
7.34622764582581));
#48682=CARTESIAN_POINT('Ctrl Pts',(-0.044754316030545,2.41915255277207,
7.34620592402186));
#48683=CARTESIAN_POINT('Ctrl Pts',(-0.0439264503351217,2.41926771684787,
7.34615455270768));
#48684=CARTESIAN_POINT('Ctrl Pts',(-0.0434487867006476,2.41933307218411,
7.34612488759609));
#48685=CARTESIAN_POINT('Ctrl Pts',(-0.0420511389371274,2.41952110847646,
7.34603801376608));
#48686=CARTESIAN_POINT('Ctrl Pts',(-0.0411307751156371,2.4196408865547,
7.34598071348627));
#48687=CARTESIAN_POINT('Ctrl Pts',(-0.0343431254920052,2.42049444434363,
7.34555742397848));
#48688=CARTESIAN_POINT('Ctrl Pts',(-0.0284574843661114,2.42107055802009,
7.34518648974109));
#48689=CARTESIAN_POINT('Ctrl Pts',(-0.00870833655251587,2.42245642108072,
7.34392765343439));
#48690=CARTESIAN_POINT('Ctrl Pts',(0.00518957568460903,2.42253211086154,
7.34301767762375));
#48691=CARTESIAN_POINT('Ctrl Pts',(0.0489910324575595,2.41993875249917,
7.34008622731899));
#48692=CARTESIAN_POINT('Ctrl Pts',(0.078539777553973,2.41399441471167,7.3380017372432));
#48693=CARTESIAN_POINT('Ctrl Pts',(0.108262393998951,2.40355016344988,7.33600904021338));
#48694=CARTESIAN_POINT('Ctrl Pts',(0.109680997160865,2.40304047049415,7.33591423234958));
#48695=CARTESIAN_POINT('Ctrl Pts',(0.111492385849615,2.40237526656436,7.33579360610496));
#48696=CARTESIAN_POINT('Ctrl Pts',(0.111888483445022,2.40222892186143,7.33576725524625));
#48697=CARTESIAN_POINT('Ctrl Pts',(0.112518848244431,2.40199461424174,7.3357253631349));
#48698=CARTESIAN_POINT('Ctrl Pts',(0.112753300881688,2.40190715689195,7.3357097917631));
#48699=CARTESIAN_POINT('Ctrl Pts',(0.11319018783606,2.40174360601668,7.33568079382722));
#48700=CARTESIAN_POINT('Ctrl Pts',(0.113392645876778,2.40166758237466,7.33566736324266));
#48701=CARTESIAN_POINT('Ctrl Pts',(0.113850159354271,2.40149525894406,7.33563702940329));
#48702=CARTESIAN_POINT('Ctrl Pts',(0.114105168649582,2.40139883947936,7.33562013347761));
#48703=CARTESIAN_POINT('Ctrl Pts',(0.114862524619515,2.40111138289487,7.33556998756576));
#48704=CARTESIAN_POINT('Ctrl Pts',(0.115364519260963,2.40091941143166,7.33553679349584));
#48705=CARTESIAN_POINT('Ctrl Pts',(0.119441232509193,2.39934870482761,7.33526756255857));
#48706=CARTESIAN_POINT('Ctrl Pts',(0.122991774349946,2.39790750529514,7.33503520221813));
#48707=CARTESIAN_POINT('Ctrl Pts',(0.134701895679969,2.39290918897779,7.33427326269652));
#48708=CARTESIAN_POINT('Ctrl Pts',(0.142740276788091,2.38907720998697,7.33375740712057));
#48709=CARTESIAN_POINT('Ctrl Pts',(0.17305098587776,2.37305463345284,7.3318024839643));
#48710=CARTESIAN_POINT('Ctrl Pts',(0.194011581735737,2.35858279349514,7.33042234579628));
#48711=CARTESIAN_POINT('Ctrl Pts',(0.216621816156593,2.33866028603005,7.32868778452313));
#48712=CARTESIAN_POINT('Ctrl Pts',(0.220116126001885,2.33544135487682,7.32841201642164));
#48713=CARTESIAN_POINT('Ctrl Pts',(0.224759684467164,2.33096999089431,7.32803388701573));
#48714=CARTESIAN_POINT('Ctrl Pts',(0.225972140637662,2.32978390710425,7.32793403796357));
#48715=CARTESIAN_POINT('Ctrl Pts',(0.231690653957768,2.3241007463158,7.32745761168318));
#48716=CARTESIAN_POINT('Ctrl Pts',(0.236071923382834,2.31948061893626,7.32707615316345));
#48717=CARTESIAN_POINT('Ctrl Pts',(0.240997240512356,2.31396859428939,7.32662623892424));
#48718=CARTESIAN_POINT('Ctrl Pts',(0.241677520921126,2.31319991819872,7.32656361045812));
#48719=CARTESIAN_POINT('Ctrl Pts',(0.242685170795305,2.31205031421141,7.32647010897869));
#48720=CARTESIAN_POINT('Ctrl Pts',(0.243015345379898,2.31167184457665,7.32643935282436));
#48721=CARTESIAN_POINT('Ctrl Pts',(0.243602356099082,2.31099578728265,7.32638445913555));
#48722=CARTESIAN_POINT('Ctrl Pts',(0.243859535582839,2.31069849798041,7.32636033589695));
#48723=CARTESIAN_POINT('Ctrl Pts',(0.244394548530188,2.3100777524857,7.32630999841056));
#48724=CARTESIAN_POINT('Ctrl Pts',(0.244672285099172,2.30975421412282,7.3262837802298));
#48725=CARTESIAN_POINT('Ctrl Pts',(0.245395711272452,2.30890809521097,7.32621526111521));
#48726=CARTESIAN_POINT('Ctrl Pts',(0.245840372102121,2.30838464144127,7.32617291798999));
#48727=CARTESIAN_POINT('Ctrl Pts',(0.246808426734418,2.30723763864586,7.32608023395456));
#48728=CARTESIAN_POINT('Ctrl Pts',(0.247331136827681,2.30661352113219,7.32602986541983));
#48729=CARTESIAN_POINT('Ctrl Pts',(0.248852594441432,2.3047828487348,7.32588230456728));
#48730=CARTESIAN_POINT('Ctrl Pts',(0.249844906689727,2.30357099832226,7.32578485201683));
#48731=CARTESIAN_POINT('Ctrl Pts',(0.260016978710572,2.29096205888096,7.32477314469144));
#48732=CARTESIAN_POINT('Ctrl Pts',(0.268417835096313,2.27896115781958,7.32382795414517));
#48733=CARTESIAN_POINT('Ctrl Pts',(0.291978748267486,2.23989314833037,7.3208065539014));
#48734=CARTESIAN_POINT('Ctrl Pts',(0.304070818390767,2.21118658079329,7.31864771893823));
#48735=CARTESIAN_POINT('Ctrl Pts',(0.312755132968237,2.17782998656093,7.31643387634912));
#48736=CARTESIAN_POINT('Ctrl Pts',(0.313577163844854,2.17444894059029,7.31621291104345));
#48737=CARTESIAN_POINT('Ctrl Pts',(0.314469887312247,2.17049957413541,7.31595930531014));
#48738=CARTESIAN_POINT('Ctrl Pts',(0.314593983555409,2.16994373096986,7.31592371552658));
#48739=CARTESIAN_POINT('Ctrl Pts',(0.314776708573758,2.16911495704464,7.31587080723701));
#48740=CARTESIAN_POINT('Ctrl Pts',(0.31483645641633,2.16884227814676,7.31585342489455));
#48741=CARTESIAN_POINT('Ctrl Pts',(0.314942417145779,2.16835566844569,7.31582245069202));
#48742=CARTESIAN_POINT('Ctrl Pts',(0.31498876635459,2.16814176837854,7.31580885098557));
#48743=CARTESIAN_POINT('Ctrl Pts',(0.315086887659804,2.16768670246147,7.31577995149014));
#48744=CARTESIAN_POINT('Ctrl Pts',(0.315138600646858,2.1674455250448,7.31576465516559));
#48745=CARTESIAN_POINT('Ctrl Pts',(0.315277032718001,2.16679627465888,7.3157235304565));
#48746=CARTESIAN_POINT('Ctrl Pts',(0.315363236774179,2.16638809052636,7.31569773169403));
#48747=CARTESIAN_POINT('Ctrl Pts',(0.315776943715895,2.16441016062326,7.31557298699603));
#48748=CARTESIAN_POINT('Ctrl Pts',(0.316093527682285,2.16283811726516,7.31547465755566));
#48749=CARTESIAN_POINT('Ctrl Pts',(0.318667947646501,2.14954244991579,7.31464941495535));
#48750=CARTESIAN_POINT('Ctrl Pts',(0.32028470968847,2.13770262998914,7.31395625829021));
#48751=CARTESIAN_POINT('Ctrl Pts',(0.324139463425932,2.08970468478024,7.31121669033309));
#48752=CARTESIAN_POINT('Ctrl Pts',(0.320935100326457,2.05338302844752,7.30926952101144));
#48753=CARTESIAN_POINT('Ctrl Pts',(0.31124500741935,2.01638261234087,7.30695739214416));
#48754=CARTESIAN_POINT('Ctrl Pts',(0.310710466001575,2.01441771103415,7.30683370819671));
#48755=CARTESIAN_POINT('Ctrl Pts',(0.309970980285469,2.01179774532138,7.30666754204549));
#48756=CARTESIAN_POINT('Ctrl Pts',(0.309782504609037,2.01113804989642,7.30662559594255));
#48757=CARTESIAN_POINT('Ctrl Pts',(0.309484649409622,2.01010797283249,7.30655993157993));
#48758=CARTESIAN_POINT('Ctrl Pts',(0.309376707495542,2.00973717473065,7.3065362602307));
#48759=CARTESIAN_POINT('Ctrl Pts',(0.309159687876581,2.008996639508,7.30648891677847));
#48760=CARTESIAN_POINT('Ctrl Pts',(0.309050612745041,2.0086269022705,7.30646524479162));
#48761=CARTESIAN_POINT('Ctrl Pts',(0.308804991032578,2.00779977772831,7.3064122122064));
#48762=CARTESIAN_POINT('Ctrl Pts',(0.308668091338972,2.00734249701817,7.3063828401054));
#48763=CARTESIAN_POINT('Ctrl Pts',(0.308265331067375,2.00600797092438,7.30629696566834));
#48764=CARTESIAN_POINT('Ctrl Pts',(0.307996744711551,2.00513155905609,7.30624037418203));
#48765=CARTESIAN_POINT('Ctrl Pts',(0.307380861954413,2.00315208477729,7.30611210750035));
#48766=CARTESIAN_POINT('Ctrl Pts',(0.307031361305398,2.002049726403,7.30604036042177));
#48767=CARTESIAN_POINT('Ctrl Pts',(0.305900734768139,1.99854913629999,7.30581150506724));
#48768=CARTESIAN_POINT('Ctrl Pts',(0.305097399451094,1.99615822833283,7.30565366891226));
#48769=CARTESIAN_POINT('Ctrl Pts',(0.301881967844222,1.9869479132987,7.30503960144201));
#48770=CARTESIAN_POINT('Ctrl Pts',(0.299268761965905,1.98020145383,7.30457682750811));
#48771=CARTESIAN_POINT('Ctrl Pts',(0.289827622316989,1.95806919196521,7.3030145896575));
#48772=CARTESIAN_POINT('Ctrl Pts',(0.282022575789474,1.94313204305789,7.301885805813));
#48773=CARTESIAN_POINT('Ctrl Pts',(0.271817677192594,1.92684674367971,7.30058602440199));
#48774=CARTESIAN_POINT('Ctrl Pts',(0.270524726215543,1.92483358688585,7.30042410662612));
#48775=CARTESIAN_POINT('Ctrl Pts',(0.258182562717563,1.90607916164526,7.29890477822406));
#48776=CARTESIAN_POINT('Ctrl Pts',(0.245613975609272,1.89038726377007,7.29754825329908));
#48777=CARTESIAN_POINT('Ctrl Pts',(0.231396138878017,1.87568514613716,7.29625874382856));
#48778=CARTESIAN_POINT('Ctrl Pts',(0.231125385486507,1.87540618232358,7.29623426971602));
#48779=CARTESIAN_POINT('Ctrl Pts',(0.230249748547268,1.87450725254282,7.29615538581831));
#48780=CARTESIAN_POINT('Ctrl Pts',(0.22964286354414,1.87388922819549,7.29610112328574));
#48781=CARTESIAN_POINT('Ctrl Pts',(0.228817129157504,1.8730550912507,7.29602785625103));
#48782=CARTESIAN_POINT('Ctrl Pts',(0.228600458447214,1.87283684144923,7.29600868333411));
#48783=CARTESIAN_POINT('Ctrl Pts',(0.22823327278429,1.87246803710312,7.29597628024674));
#48784=CARTESIAN_POINT('Ctrl Pts',(0.22808292103852,1.87231732152694,7.29596303721644));
#48785=CARTESIAN_POINT('Ctrl Pts',(0.227792749712988,1.87202702389206,7.29593752734882));
#48786=CARTESIAN_POINT('Ctrl Pts',(0.227652952182814,1.87188742248624,7.29592525899036));
#48787=CARTESIAN_POINT('Ctrl Pts',(0.227319451894788,1.87155500199331,7.29589604312272));
#48788=CARTESIAN_POINT('Ctrl Pts',(0.227125632332043,1.87136230087075,7.29587910506971));
#48789=CARTESIAN_POINT('Ctrl Pts',(0.226547598482039,1.87078906292596,7.29582871208519));
#48790=CARTESIAN_POINT('Ctrl Pts',(0.22616266886089,1.87040924392279,7.29579531390105));
#48791=CARTESIAN_POINT('Ctrl Pts',(0.222969415901182,1.86727421062912,7.29551955498801));
#48792=CARTESIAN_POINT('Ctrl Pts',(0.220111660465156,1.86456951385418,7.29528107340163));
#48793=CARTESIAN_POINT('Ctrl Pts',(0.210688956881642,1.85597308488106,7.29451835985857));
#48794=CARTESIAN_POINT('Ctrl Pts',(0.203931126806355,1.85029799200357,7.29400730422448));
#48795=CARTESIAN_POINT('Ctrl Pts',(0.1734673723503,1.82677799396694,7.29181303135831));
#48796=CARTESIAN_POINT('Ctrl Pts',(0.147596644908991,1.81197826098531,7.29021000069539));
#48797=CARTESIAN_POINT('Ctrl Pts',(0.118345943486315,1.80023534701301,7.28836471931974));
#48798=CARTESIAN_POINT('Ctrl Pts',(0.116620372055996,1.79955982600164,7.28825581183764));
#48799=CARTESIAN_POINT('Ctrl Pts',(0.108679066119182,1.79652971267431,7.2877542004246));
#48800=CARTESIAN_POINT('Ctrl Pts',(0.102397595624481,1.79435301826717,7.28735625377473));
#48801=CARTESIAN_POINT('Ctrl Pts',(0.0950613449120288,1.79206234886448,
7.2868885159972));
#48802=CARTESIAN_POINT('Ctrl Pts',(0.0940675603863193,1.79175731910293,
7.28682509424341));
#48803=CARTESIAN_POINT('Ctrl Pts',(0.0925889846090709,1.79131130498307,
7.28673063746083));
#48804=CARTESIAN_POINT('Ctrl Pts',(0.0921053029886499,1.79116664095506,
7.28669972284522));
#48805=CARTESIAN_POINT('Ctrl Pts',(0.0912441069411747,1.79091126946035,
7.2866446513828));
#48806=CARTESIAN_POINT('Ctrl Pts',(0.0908667251276105,1.79080011536143,
7.2866205091776));
#48807=CARTESIAN_POINT('Ctrl Pts',(0.0900811212604811,1.7905702859341,7.28657023161557));
#48808=CARTESIAN_POINT('Ctrl Pts',(0.0896728662436124,1.79045172684806,
7.28654409252053));
#48809=CARTESIAN_POINT('Ctrl Pts',(0.0886198605506465,1.79014818725219,
7.28647664255024));
#48810=CARTESIAN_POINT('Ctrl Pts',(0.0879747671850356,1.78996441192181,
7.28643529250194));
#48811=CARTESIAN_POINT('Ctrl Pts',(0.0852195342448476,1.78918878786623,
7.28625855750337));
#48812=CARTESIAN_POINT('Ctrl Pts',(0.0831040002562024,1.78861646902098,
7.2861225395628));
#48813=CARTESIAN_POINT('Ctrl Pts',(0.0776514756705943,1.78720091127522,
7.28577109309131));
#48814=CARTESIAN_POINT('Ctrl Pts',(0.0743065844201144,1.78638949058253,
7.28555465393187));
#48815=CARTESIAN_POINT('Ctrl Pts',(0.0679548724346423,1.78495597905047,
7.28514194708354));
#48816=CARTESIAN_POINT('Ctrl Pts',(0.0649508852388535,1.78432297944141,
7.2849460474936));
#48817=CARTESIAN_POINT('Ctrl Pts',(0.0489983094532829,1.78119879345297,
7.28390188830195));
#48818=CARTESIAN_POINT('Ctrl Pts',(0.0359162941350299,1.77946139715869,
7.28303152000872));
#48819=CARTESIAN_POINT('Ctrl Pts',(-0.00555322865300899,1.77652460416277,
7.28024367511505));
#48820=CARTESIAN_POINT('Ctrl Pts',(-0.0340136046465727,1.77826971293727,
7.27827820440472));
#48821=CARTESIAN_POINT('Ctrl Pts',(-0.0633128102330076,1.78400189561135,
7.27639060802813));
#48822=CARTESIAN_POINT('Ctrl Pts',(-0.0647459983417925,1.78429242991623,
7.27629865686531));
#48823=CARTESIAN_POINT('Ctrl Pts',(-0.0665905215442268,1.78467943862106,
7.27618085146625));
#48824=CARTESIAN_POINT('Ctrl Pts',(-0.0670036838563688,1.78476697453727,
7.27615449851696));
#48825=CARTESIAN_POINT('Ctrl Pts',(-0.0676590006165786,1.78490716182497,
7.27611275659796));
#48826=CARTESIAN_POINT('Ctrl Pts',(-0.0679012666437988,1.78495928037348,
7.27609733716511));
#48827=CARTESIAN_POINT('Ctrl Pts',(-0.0683358148372503,1.78505328901188,
7.27606970191354));
#48828=CARTESIAN_POINT('Ctrl Pts',(-0.0685281173265546,1.78509507547883,
7.276057480237));
#48829=CARTESIAN_POINT('Ctrl Pts',(-0.0689808490857485,1.78519388640205,
7.27602872555198));
#48830=CARTESIAN_POINT('Ctrl Pts',(-0.0692412455857805,1.78525105780925,
7.27601220113079));
#48831=CARTESIAN_POINT('Ctrl Pts',(-0.0699981593338604,1.78541822693875,
7.27596420926816));
#48832=CARTESIAN_POINT('Ctrl Pts',(-0.0704944904180976,1.78552907752615,
7.2759327907536));
#48833=CARTESIAN_POINT('Ctrl Pts',(-0.0739842212752878,1.78631715113921,
7.27571223246819));
#48834=CARTESIAN_POINT('Ctrl Pts',(-0.0769682045136018,1.78703595761215,
7.27552543574102));
#48835=CARTESIAN_POINT('Ctrl Pts',(-0.0860205776454299,1.7893538785347,
7.27496298339328));
#48836=CARTESIAN_POINT('Ctrl Pts',(-0.0920532223458251,1.79108776736191,
7.27459396855571));
#48837=CARTESIAN_POINT('Ctrl Pts',(-0.111760921955877,1.79738079926167,
7.27339623264802));
#48838=CARTESIAN_POINT('Ctrl Pts',(-0.125181427419761,1.80268106761229,
7.27259261632321));
#48839=CARTESIAN_POINT('Ctrl Pts',(-0.144647510666331,1.81192159420228,
7.27138821056239));
#48840=CARTESIAN_POINT('Ctrl Pts',(-0.150988848894312,1.81519403910854,
7.27098941848078));
#48841=CARTESIAN_POINT('Ctrl Pts',(-0.166525370870993,1.82387647757747,
7.26998649998931));
#48842=CARTESIAN_POINT('Ctrl Pts',(-0.175569966390266,1.82953731988906,
7.26937888016225));
#48843=CARTESIAN_POINT('Ctrl Pts',(-0.19188632089873,1.84091321148929,7.26821868469773));
#48844=CARTESIAN_POINT('Ctrl Pts',(-0.1992249911041,1.84651291494113,7.26767031249534));
#48845=CARTESIAN_POINT('Ctrl Pts',(-0.207187543968832,1.85314823555549,
7.26703997234601));
#48846=CARTESIAN_POINT('Ctrl Pts',(-0.208058353732799,1.85388174920354,
7.2669705429999));
#48847=CARTESIAN_POINT('Ctrl Pts',(-0.209319919431502,1.85495589042277,
7.26686922992957));
#48848=CARTESIAN_POINT('Ctrl Pts',(-0.209713776154376,1.85529287628796,
7.26683749604175));
#48849=CARTESIAN_POINT('Ctrl Pts',(-0.210407566836464,1.85588939236692,
7.26678141056158));
#48850=CARTESIAN_POINT('Ctrl Pts',(-0.210707838619506,1.85614852946292,
7.26675707525264));
#48851=CARTESIAN_POINT('Ctrl Pts',(-0.211284315302471,1.8566478935153,7.26671023613378));
#48852=CARTESIAN_POINT('Ctrl Pts',(-0.211560590942305,1.85688803817631,
7.26668773576168));
#48853=CARTESIAN_POINT('Ctrl Pts',(-0.212149412531254,1.85740161822488,
7.2666396679338));
#48854=CARTESIAN_POINT('Ctrl Pts',(-0.21246184006064,1.85767518783101,7.26661409490643));
#48855=CARTESIAN_POINT('Ctrl Pts',(-0.213627323604747,1.85869970190939,
7.26651844039135));
#48856=CARTESIAN_POINT('Ctrl Pts',(-0.214476926434748,1.85945454645074,
7.26644819590931));
#48857=CARTESIAN_POINT('Ctrl Pts',(-0.22189152129636,1.86611268435279,7.26583058983186));
#48858=CARTESIAN_POINT('Ctrl Pts',(-0.228214778132141,1.8722784287313,7.26527210261639));
#48859=CARTESIAN_POINT('Ctrl Pts',(-0.239122452551744,1.8838254684735,7.2642479296849));
#48860=CARTESIAN_POINT('Ctrl Pts',(-0.243798290583492,1.88911292612937,
7.26378641386881));
#48861=CARTESIAN_POINT('Ctrl Pts',(-0.267588791183756,1.91786483594508,
7.26131770250931));
#48862=CARTESIAN_POINT('Ctrl Pts',(-0.283499060041731,1.94377876755195,
7.25921302538708));
#48863=CARTESIAN_POINT('Ctrl Pts',(-0.295689210127076,1.9718236785051,7.25723575291577));
#48864=CARTESIAN_POINT('Ctrl Pts',(-0.295816554758344,1.9721178499161,7.25721504582762));
#48865=CARTESIAN_POINT('Ctrl Pts',(-0.297604260642345,1.97626448396694,
7.25692363007918));
#48866=CARTESIAN_POINT('Ctrl Pts',(-0.299189785584497,1.98014904983922,
7.25665635035427));
#48867=CARTESIAN_POINT('Ctrl Pts',(-0.30089409443695,1.98456944352242,7.25635949622716));
#48868=CARTESIAN_POINT('Ctrl Pts',(-0.301087816299495,1.98507569307629,
7.25632560577614));
#48869=CARTESIAN_POINT('Ctrl Pts',(-0.301378821179852,1.98584195676327,
7.2562744732263));
#48870=CARTESIAN_POINT('Ctrl Pts',(-0.30147704579176,1.98610160864396,7.25625717520928));
#48871=CARTESIAN_POINT('Ctrl Pts',(-0.301647174900279,1.98655309845104,
7.25622714681826));
#48872=CARTESIAN_POINT('Ctrl Pts',(-0.301719231992952,1.98674487807388,
7.25621440725977));
#48873=CARTESIAN_POINT('Ctrl Pts',(-0.301869699123188,1.98714650842186,
7.25618776060194));
#48874=CARTESIAN_POINT('Ctrl Pts',(-0.301948073192932,1.98735637210419,
7.25617385573868));
#48875=CARTESIAN_POINT('Ctrl Pts',(-0.302135264606568,1.98785921711975,
7.25614058355759));
#48876=CARTESIAN_POINT('Ctrl Pts',(-0.30224387508507,1.98815227637806,7.25612122871087));
#48877=CARTESIAN_POINT('Ctrl Pts',(-0.302611870904131,1.98914967485583,
7.25605547816358));
#48878=CARTESIAN_POINT('Ctrl Pts',(-0.302869224389366,1.9898547688685,7.25600920329117));
#48879=CARTESIAN_POINT('Ctrl Pts',(-0.307001271438203,2.00129968706809,
7.25526132317705));
#48880=CARTESIAN_POINT('Ctrl Pts',(-0.310305510150295,2.01223845869604,
7.25459265640517));
#48881=CARTESIAN_POINT('Ctrl Pts',(-0.31915179159861,2.04835576843892,7.25246396644035));
#48882=CARTESIAN_POINT('Ctrl Pts',(-0.322258053448205,2.07402443595143,
7.25106566728904));
#48883=CARTESIAN_POINT('Ctrl Pts',(-0.322274930854165,2.09978888878902,
7.24958594529397));
#48884=CARTESIAN_POINT('',(-0.32227506499556,2.10009833267788,6.99910083188333));
#48885=CARTESIAN_POINT('Ctrl Pts',(-0.322274931120346,2.09978929552436,
7.24958592193406));
#48886=CARTESIAN_POINT('Ctrl Pts',(-0.322283452356173,2.11282262422254,
7.24883738236764));
#48887=CARTESIAN_POINT('Ctrl Pts',(-0.321501354546834,2.1258433373128,7.24807165738387));
#48888=CARTESIAN_POINT('Ctrl Pts',(-0.319826940648638,2.13965707673027,
7.24722632872068));
#48889=CARTESIAN_POINT('Ctrl Pts',(-0.319717057343064,2.14053342964926,
7.2471725611068));
#48890=CARTESIAN_POINT('Ctrl Pts',(-0.319533956312919,2.14194663212223,
7.24708562656257));
#48891=CARTESIAN_POINT('Ctrl Pts',(-0.319462984208659,2.14248377217532,
7.24705253038902));
#48892=CARTESIAN_POINT('Ctrl Pts',(-0.319337231928368,2.14341737105474,
7.24699491222241));
#48893=CARTESIAN_POINT('Ctrl Pts',(-0.319283066976374,2.14381391268599,
7.24697040968315));
#48894=CARTESIAN_POINT('Ctrl Pts',(-0.319177694297875,2.14457477356838,
7.24692333860086));
#48895=CARTESIAN_POINT('Ctrl Pts',(-0.319126601089601,2.14493910825994,
7.24690077371063));
#48896=CARTESIAN_POINT('Ctrl Pts',(-0.319018574666174,2.14569994638594,
7.24685359875328));
#48897=CARTESIAN_POINT('Ctrl Pts',(-0.318961525871904,2.1460964325396,7.24682898506544));
#48898=CARTESIAN_POINT('Ctrl Pts',(-0.318834156186697,2.14697008738754,
7.24677468240347));
#48899=CARTESIAN_POINT('Ctrl Pts',(-0.318763503085519,2.14744720599876,
7.24674498295549));
#48900=CARTESIAN_POINT('Ctrl Pts',(-0.318512924792828,2.14911353125983,
7.24664110415633));
#48901=CARTESIAN_POINT('Ctrl Pts',(-0.31832741533508,2.15030187666567,7.24656674805855));
#48902=CARTESIAN_POINT('Ctrl Pts',(-0.316296556871367,2.16284991393677,
7.24577864937169));
#48903=CARTESIAN_POINT('Ctrl Pts',(-0.313850853114973,2.17410270972909,
7.24504582241275));
#48904=CARTESIAN_POINT('Ctrl Pts',(-0.310214584241275,2.18736785440093,
7.24414927831901));
#48905=CARTESIAN_POINT('Ctrl Pts',(-0.309597553368278,2.18952979871242,
7.24400211942851));
#48906=CARTESIAN_POINT('Ctrl Pts',(-0.301800144268388,2.21580530406082,
7.24220109132334));
#48907=CARTESIAN_POINT('Ctrl Pts',(-0.291842408872386,2.23900352168179,
7.24047239287601));
#48908=CARTESIAN_POINT('Ctrl Pts',(-0.274060586976526,2.26988773744483,
7.23809391218775));
#48909=CARTESIAN_POINT('Ctrl Pts',(-0.268389740630484,2.27871218273794,
7.23740569282578));
#48910=CARTESIAN_POINT('Ctrl Pts',(-0.261430469991157,2.28846091259432,
7.23664836597244));
#48911=CARTESIAN_POINT('Ctrl Pts',(-0.260554260953618,2.28967046032523,
7.23655446062713));
#48912=CARTESIAN_POINT('Ctrl Pts',(-0.259428615238428,2.29120181706741,
7.23643569119007));
#48913=CARTESIAN_POINT('Ctrl Pts',(-0.25918695297812,2.29152927887054,7.23641030085365));
#48914=CARTESIAN_POINT('Ctrl Pts',(-0.258799189393296,2.29205263578715,
7.23636973391332));
#48915=CARTESIAN_POINT('Ctrl Pts',(-0.258653485436018,2.29224882266524,
7.23635452970303));
#48916=CARTESIAN_POINT('Ctrl Pts',(-0.258376594279502,2.29262076537378,
7.23632571030804));
#48917=CARTESIAN_POINT('Ctrl Pts',(-0.258245451913623,2.29279655155334,
7.2363120922314));
#48918=CARTESIAN_POINT('Ctrl Pts',(-0.257944620829139,2.29319893464911,
7.23628092516512));
#48919=CARTESIAN_POINT('Ctrl Pts',(-0.25777481316914,2.29342544160819,7.23626338467904));
#48920=CARTESIAN_POINT('Ctrl Pts',(-0.257250553497054,2.29412283667948,
7.2362093900317));
#48921=CARTESIAN_POINT('Ctrl Pts',(-0.256895105495645,2.29459297978185,
7.23617300543413));
#48922=CARTESIAN_POINT('Ctrl Pts',(-0.254176224270459,2.29816874960579,
7.23589637041318));
#48923=CARTESIAN_POINT('Ctrl Pts',(-0.251757717603252,2.30123235637591,
7.23565990846408));
#48924=CARTESIAN_POINT('Ctrl Pts',(-0.248922716738761,2.30469240756672,
7.23539250741941));
#48925=CARTESIAN_POINT('Ctrl Pts',(-0.248560235133508,2.30513242099549,
7.23535849571771));
#48926=CARTESIAN_POINT('Ctrl Pts',(-0.230754892628871,2.32662968975361,
7.23369637788475));
#48927=CARTESIAN_POINT('Ctrl Pts',(-0.210701969959911,2.34538526312127,
7.23221755769256));
#48928=CARTESIAN_POINT('Ctrl Pts',(-0.182759237044992,2.36553844137126,
7.23027168470304));
#48929=CARTESIAN_POINT('Ctrl Pts',(-0.176864236352622,2.36950071870509,
7.22986729058592));
#48930=CARTESIAN_POINT('Ctrl Pts',(-0.164008127537361,2.37753827124735,
7.22899173371935));
#48931=CARTESIAN_POINT('Ctrl Pts',(-0.157015396014096,2.38155338428239,
7.22851923169706));
#48932=CARTESIAN_POINT('Ctrl Pts',(-0.147459909293703,2.38657324243066,
7.22787412491723));
#48933=CARTESIAN_POINT('Ctrl Pts',(-0.1450239141004,2.38781367544894,7.22770972491688));
#48934=CARTESIAN_POINT('Ctrl Pts',(-0.140931092834088,2.38983262837445,
7.22743345155086));
#48935=CARTESIAN_POINT('Ctrl Pts',(-0.139282856150741,2.39062830413719,
7.22732217731717));
#48936=CARTESIAN_POINT('Ctrl Pts',(-0.137055832033402,2.39168008994256,
7.2271717769355));
#48937=CARTESIAN_POINT('Ctrl Pts',(-0.136482915396772,2.39194860807866,
7.22713308091363));
#48938=CARTESIAN_POINT('Ctrl Pts',(-0.135576847432173,2.39237001971763,
7.22707187461942));
#48939=CARTESIAN_POINT('Ctrl Pts',(-0.135244217538043,2.39252403595277,
7.22704940314875));
#48940=CARTESIAN_POINT('Ctrl Pts',(-0.134554268963572,2.39284207161545,
7.22700278823431));
#48941=CARTESIAN_POINT('Ctrl Pts',(-0.13419691161445,2.3930060052547,7.2269786418824));
#48942=CARTESIAN_POINT('Ctrl Pts',(-0.133381823548148,2.3933781137486,7.22692356145044));
#48943=CARTESIAN_POINT('Ctrl Pts',(-0.132923904620972,2.39358587168912,
7.22689261309599));
#48944=CARTESIAN_POINT('Ctrl Pts',(-0.131527027136855,2.39421569731012,
7.22679819208082));
#48945=CARTESIAN_POINT('Ctrl Pts',(-0.130586537632414,2.39463433533946,
7.22673460195383));
#48946=CARTESIAN_POINT('Ctrl Pts',(-0.123758000289313,2.3976347894515,7.2262727436864));
#48947=CARTESIAN_POINT('Ctrl Pts',(-0.117796231391091,2.40004424473148,
7.22586863626217));
#48948=CARTESIAN_POINT('Ctrl Pts',(-0.109381659778622,2.40315556137205,
7.22529648608735));
#48949=CARTESIAN_POINT('Ctrl Pts',(-0.106986294552996,2.40400916777737,
7.22513342106656));
#48950=CARTESIAN_POINT('Ctrl Pts',(-0.102696646688279,2.40548084007299,
7.22484105811657));
#48951=CARTESIAN_POINT('Ctrl Pts',(-0.100806240241989,2.40610986027482,
7.22471209885077));
#48952=CARTESIAN_POINT('Ctrl Pts',(-0.0818356509240542,2.41222741356439,
7.2234168413967));
#48953=CARTESIAN_POINT('Ctrl Pts',(-0.0643330111444237,2.41629758176658,
7.22221007407652));
#48954=CARTESIAN_POINT('Ctrl Pts',(-0.0445865415088202,2.41918222730724,
7.22085969722923));
#48955=CARTESIAN_POINT('Ctrl Pts',(-0.0425855737631327,2.41945535341325,
7.22072301703244));
#48956=CARTESIAN_POINT('Ctrl Pts',(-0.0382597680252735,2.42000444720887,
7.22042799224471));
#48957=CARTESIAN_POINT('Ctrl Pts',(-0.0359342134313587,2.42027392723696,
7.22026967150053));
#48958=CARTESIAN_POINT('Ctrl Pts',(-0.0254534482507859,2.42137282252102,
7.21955785388726));
#48959=CARTESIAN_POINT('Ctrl Pts',(-0.01727097020149,2.42191628428832,7.21900666982303));
#48960=CARTESIAN_POINT('Ctrl Pts',(-0.00280235358057257,2.42232393161631,
7.21804835948033));
#48961=CARTESIAN_POINT('Ctrl Pts',(0.00347592742284909,2.42231738827091,
7.21763796222558));
#48962=CARTESIAN_POINT('Ctrl Pts',(0.0129542458582698,2.42203049093876,
7.21703034426879));
#48963=CARTESIAN_POINT('Ctrl Pts',(0.0161566071396098,2.42188571815457,
7.21682712315192));
#48964=CARTESIAN_POINT('Ctrl Pts',(0.0198698412155998,2.42166229121435,
7.21659429571405));
#48965=CARTESIAN_POINT('Ctrl Pts',(0.0203831905111379,2.42163016918893,
7.21656217014895));
#48966=CARTESIAN_POINT('Ctrl Pts',(0.0211637200462756,2.42157945255515,
7.21651342167115));
#48967=CARTESIAN_POINT('Ctrl Pts',(0.021430954593989,2.42156175384879,7.2164967487164));
#48968=CARTESIAN_POINT('Ctrl Pts',(0.02191562384272,2.42152904776861,7.21646654171307));
#48969=CARTESIAN_POINT('Ctrl Pts',(0.0221330646196678,2.42151415299919,
7.21645300138065));
#48970=CARTESIAN_POINT('Ctrl Pts',(0.0225711882357416,2.42148369481008,
7.21642574234697));
#48971=CARTESIAN_POINT('Ctrl Pts',(0.0227918691725042,2.42146812480782,
7.21641202407988));
#48972=CARTESIAN_POINT('Ctrl Pts',(0.0234246533828474,2.42142282425357,
7.21637272202498));
#48973=CARTESIAN_POINT('Ctrl Pts',(0.0238367176664254,2.42139252827758,
7.21634717010233));
#48974=CARTESIAN_POINT('Ctrl Pts',(0.0256265963099393,2.42125747076871,
7.2162363554662));
#48975=CARTESIAN_POINT('Ctrl Pts',(0.0270038134870397,2.42114463903562,
7.2161515398941));
#48976=CARTESIAN_POINT('Ctrl Pts',(0.0528606683919066,2.41885874305175,
7.21456690480974));
#48977=CARTESIAN_POINT('Ctrl Pts',(0.0770176488386212,2.41390102689392,
7.21321323595677));
#48978=CARTESIAN_POINT('Ctrl Pts',(0.111858026860497,2.40248120113176,7.21116231304548));
#48979=CARTESIAN_POINT('Ctrl Pts',(0.123115759289336,2.39807647027641,7.21048383269289));
#48980=CARTESIAN_POINT('Ctrl Pts',(0.14217600910191,2.38935454503934,7.2092785936688));
#48981=CARTESIAN_POINT('Ctrl Pts',(0.150095990881827,2.38532655719339,7.20875984162946));
#48982=CARTESIAN_POINT('Ctrl Pts',(0.16040558235378,2.37953513259278,7.20805425119851));
#48983=CARTESIAN_POINT('Ctrl Pts',(0.162952150547441,2.37805833376962,7.20787741967476));
#48984=CARTESIAN_POINT('Ctrl Pts',(0.167143308929037,2.37555045963621,7.20758194130487));
#48985=CARTESIAN_POINT('Ctrl Pts',(0.168799484830783,2.37453902307455,7.20746400610214));
#48986=CARTESIAN_POINT('Ctrl Pts',(0.170995316034169,2.37317063503339,7.20730603118219));
#48987=CARTESIAN_POINT('Ctrl Pts',(0.17154320036794,2.3728269128002,7.20726647971671));
#48988=CARTESIAN_POINT('Ctrl Pts',(0.172442212527231,2.37225912740773,7.20720135671229));
#48989=CARTESIAN_POINT('Ctrl Pts',(0.172793949054234,2.37203602755107,7.20717582091043));
#48990=CARTESIAN_POINT('Ctrl Pts',(0.173479283756202,2.37159946720459,7.20712595518569));
#48991=CARTESIAN_POINT('Ctrl Pts',(0.173812923027298,2.37138607234871,7.2071016277334));
#48992=CARTESIAN_POINT('Ctrl Pts',(0.174579293328633,2.37089391084596,7.20704562852869));
#48993=CARTESIAN_POINT('Ctrl Pts',(0.1750117506886,2.37061472189915,7.20701394106837));
#48994=CARTESIAN_POINT('Ctrl Pts',(0.176348513768312,2.36974718023817,7.20691571981464));
#48995=CARTESIAN_POINT('Ctrl Pts',(0.1772505283705,2.36915532634849,7.20684905515689));
#48996=CARTESIAN_POINT('Ctrl Pts',(0.184745182303619,2.36418372089218,7.20629188372911));
#48997=CARTESIAN_POINT('Ctrl Pts',(0.191176880967053,2.35956733831276,7.20579245929526));
#48998=CARTESIAN_POINT('Ctrl Pts',(0.221493360286612,2.33606917130516,7.20332955709552));
#48999=CARTESIAN_POINT('Ctrl Pts',(0.242788511786008,2.31410523930215,7.20123790681877));
#49000=CARTESIAN_POINT('Ctrl Pts',(0.267246908682123,2.28045755534402,7.19845556444525));
#49001=CARTESIAN_POINT('Ctrl Pts',(0.273338805890672,2.27109001494013,7.197720550736));
#49002=CARTESIAN_POINT('Ctrl Pts',(0.279707582150361,2.26008509503176,7.19691624185754));
#49003=CARTESIAN_POINT('Ctrl Pts',(0.280472877734172,2.25874046190918,7.19681893842351));
#49004=CARTESIAN_POINT('Ctrl Pts',(0.281429705662243,2.25703078096227,7.19669649382041));
#49005=CARTESIAN_POINT('Ctrl Pts',(0.281630244482385,2.25667083581845,7.19667078626457));
#49006=CARTESIAN_POINT('Ctrl Pts',(0.28194916988366,2.25609580872142,7.19662983201779));
#49007=CARTESIAN_POINT('Ctrl Pts',(0.282068001113144,2.25588097589982,7.19661455679174));
#49008=CARTESIAN_POINT('Ctrl Pts',(0.28229240760431,2.25547417865965,7.19658568082903));
#49009=CARTESIAN_POINT('Ctrl Pts',(0.282398031738879,2.25528224396638,7.19657207702599));
#49010=CARTESIAN_POINT('Ctrl Pts',(0.282638730010926,2.25484380172487,7.19654104785051));
#49011=CARTESIAN_POINT('Ctrl Pts',(0.282773677190077,2.25459722547524,7.19652363071332));
#49012=CARTESIAN_POINT('Ctrl Pts',(0.283185728641204,2.25384197817957,7.19647038434953));
#49013=CARTESIAN_POINT('Ctrl Pts',(0.283461786178493,2.25333273279072,7.19643462191522));
#49014=CARTESIAN_POINT('Ctrl Pts',(0.28548153736812,2.24958278646854,7.19617228674096));
#49015=CARTESIAN_POINT('Ctrl Pts',(0.287171070719426,2.24631301081048,7.19594907724824));
#49016=CARTESIAN_POINT('Ctrl Pts',(0.302361229488563,2.21563799025867,7.19389941648426));
#49017=CARTESIAN_POINT('Ctrl Pts',(0.311958621743741,2.18646885261908,7.19226380063331));
#49018=CARTESIAN_POINT('Ctrl Pts',(0.319899085488931,2.14178086863705,7.18968402947187));
#49019=CARTESIAN_POINT('Ctrl Pts',(0.321482264034047,2.12702101796481,7.18882292142128));
#49020=CARTESIAN_POINT('Ctrl Pts',(0.322103555244842,2.11062857255866,7.18783308231737));
#49021=CARTESIAN_POINT('Ctrl Pts',(0.322151745455651,2.10905094579071,7.18773749094881));
#49022=CARTESIAN_POINT('Ctrl Pts',(0.322207327936335,2.10665459790115,7.18759176924137));
#49023=CARTESIAN_POINT('Ctrl Pts',(0.322223192788896,2.10583608248001,7.18754190287468));
#49024=CARTESIAN_POINT('Ctrl Pts',(0.322246691969549,2.10432691490307,7.18744978567184));
#49025=CARTESIAN_POINT('Ctrl Pts',(0.322255225146649,2.10363627995097,7.18740756312882));
#49026=CARTESIAN_POINT('Ctrl Pts',(0.322265440813055,2.10251865160049,7.18733912528933));
#49027=CARTESIAN_POINT('Ctrl Pts',(0.322268494985945,2.10209167039304,7.18731295300251));
#49028=CARTESIAN_POINT('Ctrl Pts',(0.322272730437829,2.10127171873353,7.18726264246497));
#49029=CARTESIAN_POINT('Ctrl Pts',(0.322274041538524,2.10087874947667,7.18723850832613));
#49030=CARTESIAN_POINT('Ctrl Pts',(0.32227538940038,2.09998455555533,7.18718354025327));
#49031=CARTESIAN_POINT('Ctrl Pts',(0.322274975605423,2.09948333212159,7.18715269225989));
#49032=CARTESIAN_POINT('Ctrl Pts',(0.322270273270931,2.09799452374927,7.1870609528806));
#49033=CARTESIAN_POINT('Ctrl Pts',(0.322262614428274,2.09700696204574,7.18699995608483));
#49034=CARTESIAN_POINT('Ctrl Pts',(0.322178293038253,2.09018060126358,7.18657731245154));
#49035=CARTESIAN_POINT('Ctrl Pts',(0.321947496486012,2.08434511578091,7.18621086310904));
#49036=CARTESIAN_POINT('Ctrl Pts',(0.321477691783002,2.07731227200151,7.18576259765456));
#49037=CARTESIAN_POINT('Ctrl Pts',(0.321390257004349,2.07610560827591,7.18568545150122));
#49038=CARTESIAN_POINT('Ctrl Pts',(0.318790910766332,2.04283300790411,7.18355171448453));
#49039=CARTESIAN_POINT('Ctrl Pts',(0.311499134134056,2.01132532123274,7.18133757903775));
#49040=CARTESIAN_POINT('Ctrl Pts',(0.295798277110193,1.97164390027254,7.17848903387987));
#49041=CARTESIAN_POINT('Ctrl Pts',(0.291449283442329,1.96205336831098,7.17779801476112));
#49042=CARTESIAN_POINT('Ctrl Pts',(0.285954104211748,1.95136061629933,7.17703786589357));
#49043=CARTESIAN_POINT('Ctrl Pts',(0.285260641862588,1.95003406215632,7.17694375095188));
#49044=CARTESIAN_POINT('Ctrl Pts',(0.284366748121627,1.94835273139477,7.17682475446838));
#49045=CARTESIAN_POINT('Ctrl Pts',(0.284174867034911,1.94799346572355,7.17679934424736));
#49046=CARTESIAN_POINT('Ctrl Pts',(0.283866735423601,1.94741916274283,7.17675875302679));
#49047=CARTESIAN_POINT('Ctrl Pts',(0.283750921223578,1.94720389375421,7.17674354436303));
#49048=CARTESIAN_POINT('Ctrl Pts',(0.28353074111487,1.94679574888189,7.17671472146792));
#49049=CARTESIAN_POINT('Ctrl Pts',(0.283426424129419,1.94660284936382,7.17670110433362));
#49050=CARTESIAN_POINT('Ctrl Pts',(0.283187056040634,1.94616129556381,7.17666994613733));
#49051=CARTESIAN_POINT('Ctrl Pts',(0.283051874501126,1.945912712937,7.17665241356167));
#49052=CARTESIAN_POINT('Ctrl Pts',(0.282634426323312,1.94514747892531,7.17659846707671));
#49053=CARTESIAN_POINT('Ctrl Pts',(0.282351069217079,1.94463141903462,7.176562122551));
#49054=CARTESIAN_POINT('Ctrl Pts',(0.280185720668092,1.94071329805586,7.17628643305963));
#49055=CARTESIAN_POINT('Ctrl Pts',(0.278243618191722,1.93734458600179,7.17605084763942));
#49056=CARTESIAN_POINT('Ctrl Pts',(0.260393911615578,1.90763876687956,7.17397891215303));
#49057=CARTESIAN_POINT('Ctrl Pts',(0.240849895705048,1.88366751165079,7.17233310962732));
#49058=CARTESIAN_POINT('Ctrl Pts',(0.207576909654839,1.8530559290688,7.16975997429924));
#49059=CARTESIAN_POINT('Ctrl Pts',(0.196310401855277,1.84400840893766,7.16892059427436));
#49060=CARTESIAN_POINT('Ctrl Pts',(0.183202319638029,1.83485758504372,7.16795576493343));
#49061=CARTESIAN_POINT('Ctrl Pts',(0.181921810003649,1.83397735990221,7.16786164168983));
#49062=CARTESIAN_POINT('Ctrl Pts',(0.179964709856736,1.8326527839542,7.1677179588935));
#49063=CARTESIAN_POINT('Ctrl Pts',(0.179292716059318,1.83220165670666,7.16766865440905));
#49064=CARTESIAN_POINT('Ctrl Pts',(0.178048956329662,1.83137346768915,7.16757745218211));
#49065=CARTESIAN_POINT('Ctrl Pts',(0.177477672792633,1.83099568709752,7.1675355816879));
#49066=CARTESIAN_POINT('Ctrl Pts',(0.176549676601648,1.83038626107404,7.16746759838611));
#49067=CARTESIAN_POINT('Ctrl Pts',(0.176193699927816,1.83015349431801,7.16744152763448));
#49068=CARTESIAN_POINT('Ctrl Pts',(0.175507634159402,1.82970682455841,7.1673912958986));
#49069=CARTESIAN_POINT('Ctrl Pts',(0.17517761200932,1.82949281971256,7.16736713877706));
#49070=CARTESIAN_POINT('Ctrl Pts',(0.174423620714499,1.8290058479909,7.16731196131098));
#49071=CARTESIAN_POINT('Ctrl Pts',(0.173999401822543,1.82873327139681,7.16728092650671));
#49072=CARTESIAN_POINT('Ctrl Pts',(0.172701248092291,1.82790345682002,7.1671859853633));
#49073=CARTESIAN_POINT('Ctrl Pts',(0.171825269655629,1.82734944237963,7.16712195965318));
#49074=CARTESIAN_POINT('Ctrl Pts',(0.165368791278093,1.82330950109726,7.16665031864639));
#49075=CARTESIAN_POINT('Ctrl Pts',(0.159685725592238,1.81999120001971,7.16623658213313));
#49076=CARTESIAN_POINT('Ctrl Pts',(0.152298047535376,1.81597565727743,7.16569995259205));
#49077=CARTESIAN_POINT('Ctrl Pts',(0.150683302517143,1.81511569950088,7.16558273528386));
#49078=CARTESIAN_POINT('Ctrl Pts',(0.146910906440143,1.81314769627703,7.16530906169921));
#49079=CARTESIAN_POINT('Ctrl Pts',(0.144747913307431,1.8120501785095,7.16515227313494));
#49080=CARTESIAN_POINT('Ctrl Pts',(0.122072477424548,1.80086455584873,7.16351000926168));
#49081=CARTESIAN_POINT('Ctrl Pts',(0.100556459459548,1.79296278833644,7.16195680674421));
#49082=CARTESIAN_POINT('Ctrl Pts',(0.0620117514286712,1.78329695932595,
7.15927393789732));
#49083=CARTESIAN_POINT('Ctrl Pts',(0.0453341799327445,1.78048279742726,
7.15814572829134));
#49084=CARTESIAN_POINT('Ctrl Pts',(0.0277536615550807,1.77892136813086,
7.15703775031985));
#49085=CARTESIAN_POINT('Ctrl Pts',(0.0269961689228732,1.77885679134695,
7.15699016954855));
#49086=CARTESIAN_POINT('Ctrl Pts',(0.0259253251524913,1.77876931678384,
7.15692313712521));
#49087=CARTESIAN_POINT('Ctrl Pts',(0.0256121656616808,1.77874419647902,
7.15690356195035));
#49088=CARTESIAN_POINT('Ctrl Pts',(0.0250753340672944,1.77870192411281,
7.15687005374922));
#49089=CARTESIAN_POINT('Ctrl Pts',(0.0248516802945224,1.77868454762483,
7.1568561080264));
#49090=CARTESIAN_POINT('Ctrl Pts',(0.0244240745994598,1.77865177449096,
7.15682947282573));
#49091=CARTESIAN_POINT('Ctrl Pts',(0.024220126413474,1.77863633849651,7.15681678111387));
#49092=CARTESIAN_POINT('Ctrl Pts',(0.023740661801027,1.77860050882581,7.15678697202778));
#49093=CARTESIAN_POINT('Ctrl Pts',(0.0234651330276437,1.77858027521153,
7.15676986371813));
#49094=CARTESIAN_POINT('Ctrl Pts',(0.0226541240340236,1.77852176669058,
7.15671956916412));
#49095=CARTESIAN_POINT('Ctrl Pts',(0.0221185704567568,1.77848447521429,
7.15668643791462));
#49096=CARTESIAN_POINT('Ctrl Pts',(0.0208332337005212,1.77839820186648,
7.15660711139009));
#49097=CARTESIAN_POINT('Ctrl Pts',(0.0200833634576213,1.77835050330016,
7.15656098624244));
#49098=CARTESIAN_POINT('Ctrl Pts',(0.000145393721831734,1.77715226349491,
7.15533852202367));
#49099=CARTESIAN_POINT('Ctrl Pts',(-0.0191105344568808,1.7777179681163,
7.1542536386443));
#49100=CARTESIAN_POINT('Ctrl Pts',(-0.0546232763953682,1.78195767842658,
7.15225072680636));
#49101=CARTESIAN_POINT('Ctrl Pts',(-0.0708673817861991,1.78517876452074,
7.15133331209747));
#49102=CARTESIAN_POINT('Ctrl Pts',(-0.0990689251306978,1.79306509479421,
7.14965661530244));
#49103=CARTESIAN_POINT('Ctrl Pts',(-0.111130108241283,1.79722330131339,
7.14891107296106));
#49104=CARTESIAN_POINT('Ctrl Pts',(-0.124928979902279,1.80291636860456,
7.14800926632561));
#49105=CARTESIAN_POINT('Ctrl Pts',(-0.12693694404102,1.8037687627243,7.14787680670359));
#49106=CARTESIAN_POINT('Ctrl Pts',(-0.129557369474019,1.80491268542092,
7.14770227054132));
#49107=CARTESIAN_POINT('Ctrl Pts',(-0.130177815104248,1.80518586931061,
7.14766082124836));
#49108=CARTESIAN_POINT('Ctrl Pts',(-0.131187896054326,1.80563442096466,
7.1475931381474));
#49109=CARTESIAN_POINT('Ctrl Pts',(-0.131578054911789,1.80580861050191,
7.14756694477202));
#49110=CARTESIAN_POINT('Ctrl Pts',(-0.132328472658957,1.80614543191475,
7.1475164689827));
#49111=CARTESIAN_POINT('Ctrl Pts',(-0.132688781231137,1.8063079517692,7.14749219045345));
#49112=CARTESIAN_POINT('Ctrl Pts',(-0.133513071423839,1.8066815804788,7.14743654892749));
#49113=CARTESIAN_POINT('Ctrl Pts',(-0.133976852114343,1.80689312774312,
7.14740517087892));
#49114=CARTESIAN_POINT('Ctrl Pts',(-0.135433397999181,1.80756169064322,
7.14730639813092));
#49115=CARTESIAN_POINT('Ctrl Pts',(-0.13642433360054,1.80802265288629,7.14723886737813));
#49116=CARTESIAN_POINT('Ctrl Pts',(-0.144574516915071,1.81186449389571,
7.14668066831389));
#49117=CARTESIAN_POINT('Ctrl Pts',(-0.151608737753756,1.81550284077843,
7.14618108099469));
#49118=CARTESIAN_POINT('Ctrl Pts',(-0.162680773043203,1.82175697325576,
7.14536455693147));
#49119=CARTESIAN_POINT('Ctrl Pts',(-0.166806697777298,1.82421070039919,
7.14505326363114));
#49120=CARTESIAN_POINT('Ctrl Pts',(-0.181464483258324,1.83337709232269,
7.14392204760567));
#49121=CARTESIAN_POINT('Ctrl Pts',(-0.191658172177291,1.84060795558669,
7.14308657625044));
#49122=CARTESIAN_POINT('Ctrl Pts',(-0.20941687879557,1.85482445180407,7.14155109658215));
#49123=CARTESIAN_POINT('Ctrl Pts',(-0.217116957025728,1.86161647230335,
7.1408544777012));
#49124=CARTESIAN_POINT('Ctrl Pts',(-0.232798327961972,1.87683969192324,
7.1393831028209));
#49125=CARTESIAN_POINT('Ctrl Pts',(-0.240675779895153,1.8853588955521,7.13861094035751));
#49126=CARTESIAN_POINT('Ctrl Pts',(-0.250469529860458,1.89716944848208,
7.13762416207072));
#49127=CARTESIAN_POINT('Ctrl Pts',(-0.25281116226563,1.90009567968783,7.13738600744693));
#49128=CARTESIAN_POINT('Ctrl Pts',(-0.255428053182532,1.90348544300511,
7.13711790691739));
#49129=CARTESIAN_POINT('Ctrl Pts',(-0.255753712611385,1.90390945979272,
7.13708450761479));
#49130=CARTESIAN_POINT('Ctrl Pts',(-0.256243489388205,1.90455045719791,
7.1370342254007));
#49131=CARTESIAN_POINT('Ctrl Pts',(-0.256408387587222,1.90476683577931,
7.13701728755449));
#49132=CARTESIAN_POINT('Ctrl Pts',(-0.256705059680292,1.90515715158784,
7.1369867987769));
#49133=CARTESIAN_POINT('Ctrl Pts',(-0.256836930584162,1.90533101343083,
7.13697324097551));
#49134=CARTESIAN_POINT('Ctrl Pts',(-0.257120336103367,1.90570545149304,
7.13694409187519));
#49135=CARTESIAN_POINT('Ctrl Pts',(-0.257271812194207,1.90590607049994,
7.13692850474179));
#49136=CARTESIAN_POINT('Ctrl Pts',(-0.257680062459309,1.90644808572561,
7.13688647459834));
#49137=CARTESIAN_POINT('Ctrl Pts',(-0.257936393968769,1.9067898170911,7.13686006277904));
#49138=CARTESIAN_POINT('Ctrl Pts',(-0.259122036675068,1.90837703535284,
7.13673778931918));
#49139=CARTESIAN_POINT('Ctrl Pts',(-0.26004303137767,1.90962875077835,7.13664250099883));
#49140=CARTESIAN_POINT('Ctrl Pts',(-0.279578882735,1.93658607356592,7.13461346247785));
#49141=CARTESIAN_POINT('Ctrl Pts',(-0.294308035287303,1.96489990757853,
7.13291710837441));
#49142=CARTESIAN_POINT('Ctrl Pts',(-0.309845184768981,2.00994492344333,
7.13021776030257));
#49143=CARTESIAN_POINT('Ctrl Pts',(-0.313909469118058,2.02533607985318,
7.1292978828455));
#49144=CARTESIAN_POINT('Ctrl Pts',(-0.317278022014857,2.04341338299091,
7.12818894739764));
#49145=CARTESIAN_POINT('Ctrl Pts',(-0.317706176241206,2.0458689228088,7.12803775565299));
#49146=CARTESIAN_POINT('Ctrl Pts',(-0.318219923563956,2.04903174938022,
7.12784221936802));
#49147=CARTESIAN_POINT('Ctrl Pts',(-0.318331723197484,2.0497347404502,7.12779870784932));
#49148=CARTESIAN_POINT('Ctrl Pts',(-0.318508067211456,2.05086777184486,
7.12772849604789));
#49149=CARTESIAN_POINT('Ctrl Pts',(-0.318574072251585,2.05129758518951,
7.12770184211314));
#49150=CARTESIAN_POINT('Ctrl Pts',(-0.318698099767292,2.05211627187661,
7.12765103595224));
#49151=CARTESIAN_POINT('Ctrl Pts',(-0.318756280958212,2.05250512067823,
7.12762688880299));
#49152=CARTESIAN_POINT('Ctrl Pts',(-0.318887264988565,2.05339162293256,
7.12757180112378));
#49153=CARTESIAN_POINT('Ctrl Pts',(-0.318959614596547,2.05388934139922,
7.12754084630556));
#49154=CARTESIAN_POINT('Ctrl Pts',(-0.319176575755416,2.05540683932996,
7.12744638645482));
#49155=CARTESIAN_POINT('Ctrl Pts',(-0.319317462827825,2.05642713707765,
7.12738276381433));
#49156=CARTESIAN_POINT('Ctrl Pts',(-0.320303813363428,2.06383204644101,
7.12692018234204));
#49157=CARTESIAN_POINT('Ctrl Pts',(-0.320962562003768,2.07023965959339,
7.1265153636209));
#49158=CARTESIAN_POINT('Ctrl Pts',(-0.321549566091602,2.07832445353951,
7.12599837015445));
#49159=CARTESIAN_POINT('Ctrl Pts',(-0.321657348866209,2.07998744078261,
7.12589170114141));
#49160=CARTESIAN_POINT('Ctrl Pts',(-0.322105333914157,2.08784299069095,
7.12538627388136));
#49161=CARTESIAN_POINT('Ctrl Pts',(-0.322279614612699,2.0940433830894,7.12498276239407));
#49162=CARTESIAN_POINT('Ctrl Pts',(-0.322262348256002,2.11678883775222,
7.1234866357659));
#49163=CARTESIAN_POINT('Ctrl Pts',(-0.320975845377665,2.13330628802755,
7.1223677248446));
#49164=CARTESIAN_POINT('Ctrl Pts',(-0.317188867608192,2.15759362591997,
7.12070459164423));
#49165=CARTESIAN_POINT('Ctrl Pts',(-0.315653523635841,2.16548788791474,
7.12016148990717));
#49166=CARTESIAN_POINT('Ctrl Pts',(-0.31289075550399,2.1773136375016,7.11935032801859));
#49167=CARTESIAN_POINT('Ctrl Pts',(-0.311880661653496,2.18129254918058,
7.11907784050749));
#49168=CARTESIAN_POINT('Ctrl Pts',(-0.31029086461408,2.18708836943625,7.11868251662596));
#49169=CARTESIAN_POINT('Ctrl Pts',(-0.309770638876115,2.18892106800197,
7.11855774716158));
#49170=CARTESIAN_POINT('Ctrl Pts',(-0.307596896968879,2.19632825372172,
7.11805470582299));
#49171=CARTESIAN_POINT('Ctrl Pts',(-0.305808790659011,2.20186254260865,
7.1176816975331));
#49172=CARTESIAN_POINT('Ctrl Pts',(-0.303652508737178,2.20796648955053,
7.11727578633766));
#49173=CARTESIAN_POINT('Ctrl Pts',(-0.303431347827496,2.208586491342,7.11723462030247));
#49174=CARTESIAN_POINT('Ctrl Pts',(-0.303117928155636,2.20945669627928,
7.11717693595468));
#49175=CARTESIAN_POINT('Ctrl Pts',(-0.303027258038863,2.20970746381378,
7.11716032404706));
#49176=CARTESIAN_POINT('Ctrl Pts',(-0.302860400179207,2.21016715973139,
7.11712989245255));
#49177=CARTESIAN_POINT('Ctrl Pts',(-0.302784307253642,2.21037612224525,
7.11711606708295));
#49178=CARTESIAN_POINT('Ctrl Pts',(-0.302628730876535,2.21080198660882,
7.11708790725663));
#49179=CARTESIAN_POINT('Ctrl Pts',(-0.302549230493761,2.21101888180324,
7.11707357384942));
#49180=CARTESIAN_POINT('Ctrl Pts',(-0.302349824077097,2.21156110307517,
7.11703776239858));
#49181=CARTESIAN_POINT('Ctrl Pts',(-0.302229625753394,2.21188632248157,
7.11701630190445));
#49182=CARTESIAN_POINT('Ctrl Pts',(-0.301770226153508,2.21312317338741,
7.11693475455009));
#49183=CARTESIAN_POINT('Ctrl Pts',(-0.30142741867156,2.21403347350754,7.11687488127779));
#49184=CARTESIAN_POINT('Ctrl Pts',(-0.295780582292549,2.22882483775608,
7.11590414141355));
#49185=CARTESIAN_POINT('Ctrl Pts',(-0.289526029835463,2.24232637429556,
7.11504838364258));
#49186=CARTESIAN_POINT('Ctrl Pts',(-0.267594551687138,2.28218867479503,
7.11247749035381));
#49187=CARTESIAN_POINT('Ctrl Pts',(-0.249078737845497,2.30678322651194,
7.11081119414682));
#49188=CARTESIAN_POINT('Ctrl Pts',(-0.223852827843128,2.33189590955406,
7.10869325372474));
#49189=CARTESIAN_POINT('Ctrl Pts',(-0.220255734483652,2.33531512638742,
7.10839467644041));
#49190=CARTESIAN_POINT('Ctrl Pts',(-0.215948150496158,2.33922437776374,
7.10804041553106));
#49191=CARTESIAN_POINT('Ctrl Pts',(-0.215312743509094,2.33979643258324,
7.10798824093273));
#49192=CARTESIAN_POINT('Ctrl Pts',(-0.214291747086897,2.3407083025167,7.10790453209253));
#49193=CARTESIAN_POINT('Ctrl Pts',(-0.213907605090611,2.34104973812388,
7.10787306592459));
#49194=CARTESIAN_POINT('Ctrl Pts',(-0.213226098019814,2.34165256775135,
7.10781729151451));
#49195=CARTESIAN_POINT('Ctrl Pts',(-0.212929064214269,2.34191433605347,
7.10779299897608));
#49196=CARTESIAN_POINT('Ctrl Pts',(-0.212311869174775,2.34245623689717,
7.10774255652722));
#49197=CARTESIAN_POINT('Ctrl Pts',(-0.21199163428715,2.34273628404572,7.10771640313179));
#49198=CARTESIAN_POINT('Ctrl Pts',(-0.211165966089647,2.3434554552358,7.10764901933406));
#49199=CARTESIAN_POINT('Ctrl Pts',(-0.2106597189778,2.34389363810488,7.10760775003477));
#49200=CARTESIAN_POINT('Ctrl Pts',(-0.208552391588162,2.34570618209572,
7.10743614801881));
#49201=CARTESIAN_POINT('Ctrl Pts',(-0.20693922697647,2.34706635536878,7.10730523302298));
#49202=CARTESIAN_POINT('Ctrl Pts',(-0.196002764203761,2.35610540881497,
7.10642051758089));
#49203=CARTESIAN_POINT('Ctrl Pts',(-0.186268585298666,2.36326985527563,
7.10564615994524));
#49204=CARTESIAN_POINT('Ctrl Pts',(-0.1605784018685,2.38003896309464,7.10363346739836));
#49205=CARTESIAN_POINT('Ctrl Pts',(-0.144150501134148,2.38883863456212,
7.10237260273249));
#49206=CARTESIAN_POINT('Ctrl Pts',(-0.113994571491387,2.40177550134341,
7.10015395213956));
#49207=CARTESIAN_POINT('Ctrl Pts',(-0.100574161219286,2.40650958317826,
7.0991980225727));
#49208=CARTESIAN_POINT('Ctrl Pts',(-0.0862582124319157,2.410517501423,7.0982371937021));
#49209=CARTESIAN_POINT('Ctrl Pts',(-0.0856319112603594,2.41069080078061,
7.0981952756991));
#49210=CARTESIAN_POINT('Ctrl Pts',(-0.0813239415530555,2.41186881253136,
7.09790776731883));
#49211=CARTESIAN_POINT('Ctrl Pts',(-0.0776250036226671,2.41281000893629,
7.09766502291111));
#49212=CARTESIAN_POINT('Ctrl Pts',(-0.0733401069799455,2.41381960928317,
7.09738923748937));
#49213=CARTESIAN_POINT('Ctrl Pts',(-0.0727698195909753,2.4139523400645,
7.09735264254896));
#49214=CARTESIAN_POINT('Ctrl Pts',(-0.0719240158753521,2.4141467670927,
7.09729853413486));
#49215=CARTESIAN_POINT('Ctrl Pts',(-0.0716487791612777,2.41420965577238,
7.09728095253309));
#49216=CARTESIAN_POINT('Ctrl Pts',(-0.071159679167616,2.4143207338766,7.09724975646111));
#49217=CARTESIAN_POINT('Ctrl Pts',(-0.070945849412669,2.414369066761,7.09723613370798));
#49218=CARTESIAN_POINT('Ctrl Pts',(-0.0704931399376714,2.41447090926267,
7.09720732600517));
#49219=CARTESIAN_POINT('Ctrl Pts',(-0.07025424918716,2.41452436475235,7.09719214423422));
#49220=CARTESIAN_POINT('Ctrl Pts',(-0.0696161940843432,2.41466637621393,
7.09715164741341));
#49221=CARTESIAN_POINT('Ctrl Pts',(-0.0692169200641963,2.41475444521024,
7.09712636043669));
#49222=CARTESIAN_POINT('Ctrl Pts',(-0.067339035429188,2.41516490945325,
7.09700768152716));
#49223=CARTESIAN_POINT('Ctrl Pts',(-0.0658583020331896,2.41547765389543,
7.09691483588526));
#49224=CARTESIAN_POINT('Ctrl Pts',(-0.0538617142636338,2.41792329663941,
7.09616814619585));
#49225=CARTESIAN_POINT('Ctrl Pts',(-0.0432463287161987,2.41954047285849,
7.0955416361842));
#49226=CARTESIAN_POINT('Ctrl Pts',(-0.00374570487007546,2.4235529263946,
7.09327136828312));
#49227=CARTESIAN_POINT('Ctrl Pts',(0.0253402457034932,2.4225810377561,7.09170666032807));
#49228=CARTESIAN_POINT('Ctrl Pts',(0.0635246185721014,2.41610280457003,
7.08945268296261));
#49229=CARTESIAN_POINT('Ctrl Pts',(0.0730635150517995,2.41403511591887,
7.08887377639065));
#49230=CARTESIAN_POINT('Ctrl Pts',(0.0834981643884885,2.41127208791527,
7.08821739663599));
#49231=CARTESIAN_POINT('Ctrl Pts',(0.0845017236306666,2.41100114925064,
7.08815403158137));
#49232=CARTESIAN_POINT('Ctrl Pts',(0.0860010778749563,2.41058856399406,
7.0880590003116));
#49233=CARTESIAN_POINT('Ctrl Pts',(0.0864978790376826,2.41045057319428,
7.08802745278791));
#49234=CARTESIAN_POINT('Ctrl Pts',(0.0873530860885475,2.41021081990455,
7.08797304259636));
#49235=CARTESIAN_POINT('Ctrl Pts',(0.0877116516631416,2.41010962673816,
7.08795019847981));
#49236=CARTESIAN_POINT('Ctrl Pts',(0.0884514726111471,2.40989945119519,
7.0879029995511));
#49237=CARTESIAN_POINT('Ctrl Pts',(0.0888327038064695,2.40979038653645,
7.08787864209107));
#49238=CARTESIAN_POINT('Ctrl Pts',(0.0897198698529599,2.40953480905256,
7.0878218759029));
#49239=CARTESIAN_POINT('Ctrl Pts',(0.0902256476431692,2.40938775923387,
7.08778944970768));
#49240=CARTESIAN_POINT('Ctrl Pts',(0.0918374350681469,2.40891485976337,
7.08768591146829));
#49241=CARTESIAN_POINT('Ctrl Pts',(0.0929420481157377,2.40858431700137,
7.08761464628972));
#49242=CARTESIAN_POINT('Ctrl Pts',(0.117515345708149,2.40108712898436,7.08602233493944));
#49243=CARTESIAN_POINT('Ctrl Pts',(0.140085985852169,2.39127091521655,7.08440889888853));
#49244=CARTESIAN_POINT('Ctrl Pts',(0.180693468313031,2.36779067969438,7.08124504750092));
#49245=CARTESIAN_POINT('Ctrl Pts',(0.198848083068947,2.35460074146565,7.07971244089955));
#49246=CARTESIAN_POINT('Ctrl Pts',(0.218288566364723,2.33711904232689,7.07802996917359));
#49247=CARTESIAN_POINT('Ctrl Pts',(0.221042759673337,2.33455370363494,7.07779064833099));
#49248=CARTESIAN_POINT('Ctrl Pts',(0.224171193438992,2.33153572441439,7.0775183391751));
#49249=CARTESIAN_POINT('Ctrl Pts',(0.224589764226304,2.33112973297562,7.07748189552711));
#49250=CARTESIAN_POINT('Ctrl Pts',(0.225209018172919,2.33052581894337,7.07742796755386));
#49251=CARTESIAN_POINT('Ctrl Pts',(0.22541054436719,2.33032876840609,7.0774104157548));
#49252=CARTESIAN_POINT('Ctrl Pts',(0.225764574135038,2.32998169156504,7.07737957899283));
#49253=CARTESIAN_POINT('Ctrl Pts',(0.225917186819065,2.32983177780779,7.07736628520659));
#49254=CARTESIAN_POINT('Ctrl Pts',(0.22623960122763,2.32951443380739,7.07733819856865));
#49255=CARTESIAN_POINT('Ctrl Pts',(0.226409365975204,2.32934696747321,7.07732340869076));
#49256=CARTESIAN_POINT('Ctrl Pts',(0.226756926662201,2.32900335035898,7.07729312663948));
#49257=CARTESIAN_POINT('Ctrl Pts',(0.22693470365029,2.3288271805208,7.07727763598735));
#49258=CARTESIAN_POINT('Ctrl Pts',(0.22737470564928,2.32839013917179,7.07723929222329));
#49259=CARTESIAN_POINT('Ctrl Pts',(0.227636687924422,2.32812902216508,7.0772164583242));
#49260=CARTESIAN_POINT('Ctrl Pts',(0.228365022906173,2.32740058883793,7.07715296595715));
#49261=CARTESIAN_POINT('Ctrl Pts',(0.228830393255474,2.32693228644475,7.07711238368087));
#49262=CARTESIAN_POINT('Ctrl Pts',(0.232941528664527,2.32276974384338,7.07675371606796));
#49263=CARTESIAN_POINT('Ctrl Pts',(0.23649923837744,2.31898911404884,7.07644221605307));
#49264=CARTESIAN_POINT('Ctrl Pts',(0.244120794150171,2.3104874973938,7.07576797649159));
#49265=CARTESIAN_POINT('Ctrl Pts',(0.248142275551042,2.30573130113206,7.07540755742528));
#49266=CARTESIAN_POINT('Ctrl Pts',(0.270140389399782,2.27812994762096,7.07338966899759));
#49267=CARTESIAN_POINT('Ctrl Pts',(0.285098472785188,2.25305259135261,7.07181989266189));
#49268=CARTESIAN_POINT('Ctrl Pts',(0.300266264072809,2.21744826514252,7.06956643019965));
#49269=CARTESIAN_POINT('Ctrl Pts',(0.303641391143685,2.20842417619989,7.06899477192354));
#49270=CARTESIAN_POINT('Ctrl Pts',(0.30695721761685,2.19818214310459,7.06834012956416));
#49271=CARTESIAN_POINT('Ctrl Pts',(0.307301465948203,2.19709930816444,7.06827084926733));
#49272=CARTESIAN_POINT('Ctrl Pts',(0.307782621052962,2.19555764249331,7.0681721080388));
#49273=CARTESIAN_POINT('Ctrl Pts',(0.307924245447499,2.19510028350532,7.06814280187033));
#49274=CARTESIAN_POINT('Ctrl Pts',(0.308182215087405,2.19426058375324,7.068088971861));
#49275=CARTESIAN_POINT('Ctrl Pts',(0.308298869499309,2.19387833833664,7.06806445819768));
#49276=CARTESIAN_POINT('Ctrl Pts',(0.308533871648709,2.19310313685073,7.06801472465271));
#49277=CARTESIAN_POINT('Ctrl Pts',(0.308652180384782,2.19271016981555,7.06798950354797));
#49278=CARTESIAN_POINT('Ctrl Pts',(0.308941688302218,2.19174186166235,7.06792733107386));
#49279=CARTESIAN_POINT('Ctrl Pts',(0.309112030743056,2.19116626785396,7.06789035179104));
#49280=CARTESIAN_POINT('Ctrl Pts',(0.309728214511656,2.18906257698508,7.06775511683512));
#49281=CARTESIAN_POINT('Ctrl Pts',(0.310164335041205,2.18753167773042,7.0676565448922));
#49282=CARTESIAN_POINT('Ctrl Pts',(0.312620747519642,2.17866009722345,7.06708434329595));
#49283=CARTESIAN_POINT('Ctrl Pts',(0.314391596739544,2.17125342618661,7.06660268708062));
#49284=CARTESIAN_POINT('Ctrl Pts',(0.317330007324402,2.15670227733301,7.06564785982438));
#49285=CARTESIAN_POINT('Ctrl Pts',(0.318522446416637,2.14956733737658,7.06517574758331));
#49286=CARTESIAN_POINT('Ctrl Pts',(0.323976617061947,2.10847023081411,7.06243676288768));
#49287=CARTESIAN_POINT('Ctrl Pts',(0.323045970377624,2.07404492333451,7.06003718736388));
#49288=CARTESIAN_POINT('Ctrl Pts',(0.316474364236885,2.0391157400501,7.05779294239871));
#49289=CARTESIAN_POINT('Ctrl Pts',(0.316222454182139,2.03782061481557,7.05771004776966));
#49290=CARTESIAN_POINT('Ctrl Pts',(0.315882676039987,2.03612923009927,7.0576022405151));
#49291=CARTESIAN_POINT('Ctrl Pts',(0.31580200781607,2.0357315619177,7.0575769261146));
#49292=CARTESIAN_POINT('Ctrl Pts',(0.315676497389088,2.03511877848992,7.05753796949047));
#49293=CARTESIAN_POINT('Ctrl Pts',(0.315632186242368,2.03490355680197,7.0575242969312));
#49294=CARTESIAN_POINT('Ctrl Pts',(0.315544326903235,2.034479017911,7.05749734644004));
#49295=CARTESIAN_POINT('Ctrl Pts',(0.315500790824919,2.03426970010696,7.05748406797733));
#49296=CARTESIAN_POINT('Ctrl Pts',(0.315405367894482,2.03381319374924,7.05745512907025));
#49297=CARTESIAN_POINT('Ctrl Pts',(0.31535339888674,2.03356602352724,7.05743947345737));
#49298=CARTESIAN_POINT('Ctrl Pts',(0.315243172507686,2.03304481871844,7.05740648766453));
#49299=CARTESIAN_POINT('Ctrl Pts',(0.315184848227973,2.03277079829383,7.05738916133066));
#49300=CARTESIAN_POINT('Ctrl Pts',(0.31503374645828,2.03206540715891,7.05734459916072));
#49301=CARTESIAN_POINT('Ctrl Pts',(0.314940439874659,2.03163414851711,7.05731739327539));
#49302=CARTESIAN_POINT('Ctrl Pts',(0.314666085167614,2.03037857559652,7.05723829371443));
#49303=CARTESIAN_POINT('Ctrl Pts',(0.314482682716142,2.02955477163909,7.05718653086192));
#49304=CARTESIAN_POINT('Ctrl Pts',(0.312531345229022,2.02094929709104,7.05664714546488));
#49305=CARTESIAN_POINT('Ctrl Pts',(0.31047803265197,2.01323439415378,7.0561749505838));
#49306=CARTESIAN_POINT('Ctrl Pts',(0.308061057403647,2.00534465918494,7.05569644159124));
#49307=CARTESIAN_POINT('Ctrl Pts',(0.307981588315334,2.00508640828148,7.0556807837279));
#49308=CARTESIAN_POINT('Ctrl Pts',(0.30328152645721,1.98988066091884,7.05475912775252));
#49309=CARTESIAN_POINT('Ctrl Pts',(0.297578603027083,1.97528836196526,7.05388947261322));
#49310=CARTESIAN_POINT('Ctrl Pts',(0.284102340143277,1.94705720713177,7.05214041432178));
#49311=CARTESIAN_POINT('Ctrl Pts',(0.276349279724215,1.93345672455976,7.051263060015));
#49312=CARTESIAN_POINT('Ctrl Pts',(0.266616700666186,1.9189472796498,7.05024803770579));
#49313=CARTESIAN_POINT('Ctrl Pts',(0.265579992063179,1.91742995792557,7.05014088697745));
#49314=CARTESIAN_POINT('Ctrl Pts',(0.263466573161175,1.91439286333949,7.04992429425137));
#49315=CARTESIAN_POINT('Ctrl Pts',(0.262389553014563,1.91287339411709,7.04981484509499));
#49316=CARTESIAN_POINT('Ctrl Pts',(0.257400862899707,1.90596306129242,7.0493119011768));
#49317=CARTESIAN_POINT('Ctrl Pts',(0.25333604974078,1.90068523893572,7.04891314660957));
#49318=CARTESIAN_POINT('Ctrl Pts',(0.24845093764706,1.89473337053546,7.04844453558066));
#49319=CARTESIAN_POINT('Ctrl Pts',(0.247787131298227,1.89393254717773,7.04838107571662));
#49320=CARTESIAN_POINT('Ctrl Pts',(0.246795325312391,1.89274774299909,7.04828657306534));
#49321=CARTESIAN_POINT('Ctrl Pts',(0.246470276735994,1.8923612913999,7.04825565086332));
#49322=CARTESIAN_POINT('Ctrl Pts',(0.245890370136613,1.89167511842218,7.04820057086992));
#49323=CARTESIAN_POINT('Ctrl Pts',(0.245635868468282,1.89137509609352,7.04817642773671));
#49324=CARTESIAN_POINT('Ctrl Pts',(0.245099613774348,1.89074526741301,7.04812561806141));
#49325=CARTESIAN_POINT('Ctrl Pts',(0.244817743184334,1.89041556259687,7.04809894670132));
#49326=CARTESIAN_POINT('Ctrl Pts',(0.244074708871005,1.88954997753592,7.04802873162201));
#49327=CARTESIAN_POINT('Ctrl Pts',(0.243612447782053,1.88901504617982,7.04798514254404));
#49328=CARTESIAN_POINT('Ctrl Pts',(0.241543161637114,1.88663632268509,7.04779042954016));
#49329=CARTESIAN_POINT('Ctrl Pts',(0.23991697205436,1.88480937817624,7.04763850868369));
#49330=CARTESIAN_POINT('Ctrl Pts',(0.227903786403204,1.87161859838849,7.04652387378808));
#49331=CARTESIAN_POINT('Ctrl Pts',(0.216736665122448,1.86099519923503,7.04552733244548));
#49332=CARTESIAN_POINT('Ctrl Pts',(0.193710829799644,1.84203551557076,7.0435470418137));
#49333=CARTESIAN_POINT('Ctrl Pts',(0.18196352586825,1.83361908252853,7.04256875825986));
#49334=CARTESIAN_POINT('Ctrl Pts',(0.157242853619734,1.8183081315146,7.04060212307349));
#49335=CARTESIAN_POINT('Ctrl Pts',(0.144281038323525,1.81145419656402,7.03961618300631));
#49336=CARTESIAN_POINT('Ctrl Pts',(0.130346571959502,1.80526060731785,7.03863058960457));
#49337=CARTESIAN_POINT('Ctrl Pts',(0.129795478809724,1.80501750541462,7.03859172872708));
#49338=CARTESIAN_POINT('Ctrl Pts',(0.125701075398107,1.80322505030837,7.03830390128516));
#49339=CARTESIAN_POINT('Ctrl Pts',(0.122130619371397,1.80173795709965,7.03805786104215));
#49340=CARTESIAN_POINT('Ctrl Pts',(0.117987463328093,1.80009921700317,7.03777873233548));
#49341=CARTESIAN_POINT('Ctrl Pts',(0.11744026196051,1.79988451218187,7.03774199378621));
#49342=CARTESIAN_POINT('Ctrl Pts',(0.116628948483193,1.79956873670526,7.03768771415969));
#49343=CARTESIAN_POINT('Ctrl Pts',(0.116365289754814,1.79946651612355,7.03767010433063));
#49344=CARTESIAN_POINT('Ctrl Pts',(0.115904223122728,1.79928845814008,7.03763936213499));
#49345=CARTESIAN_POINT('Ctrl Pts',(0.115706875086156,1.79921246800396,7.03762622052711));
#49346=CARTESIAN_POINT('Ctrl Pts',(0.115288021760231,1.79905165904837,7.03759836445504));
#49347=CARTESIAN_POINT('Ctrl Pts',(0.115066498124971,1.79896689070295,7.03758365307852));
#49348=CARTESIAN_POINT('Ctrl Pts',(0.114486317669273,1.7987456125459,7.03754517822606));
#49349=CARTESIAN_POINT('Ctrl Pts',(0.114127508899802,1.79860949814274,7.03752143859003));
#49350=CARTESIAN_POINT('Ctrl Pts',(0.113341821941568,1.79831305140509,7.0374695739202));
#49351=CARTESIAN_POINT('Ctrl Pts',(0.112914844016257,1.79815298318473,7.03744146454163));
#49352=CARTESIAN_POINT('Ctrl Pts',(0.111659957412499,1.79768557855027,7.03735907087312));
#49353=CARTESIAN_POINT('Ctrl Pts',(0.110831115537407,1.79738073528566,7.03730493092383));
#49354=CARTESIAN_POINT('Ctrl Pts',(0.107958577736139,1.79633761711331,7.03711823122184));
#49355=CARTESIAN_POINT('Ctrl Pts',(0.105908624798248,1.79561658874118,7.03698662746997));
#49356=CARTESIAN_POINT('Ctrl Pts',(0.0968195354459518,1.79252263314644,
7.03640965729422));
#49357=CARTESIAN_POINT('Ctrl Pts',(0.0897063901530078,1.79037258860609,
7.03597532285138));
#49358=CARTESIAN_POINT('Ctrl Pts',(0.0543872650622043,1.78101649230613,
7.03387397843983));
#49359=CARTESIAN_POINT('Ctrl Pts',(0.0253694705129781,1.77740887647372,
7.03230575919116));
#49360=CARTESIAN_POINT('Ctrl Pts',(-0.00698259479660888,1.77778433352114,
7.0304318434941));
#49361=CARTESIAN_POINT('Ctrl Pts',(-0.010224497878336,1.77787090933579,
7.03024284387156));
#49362=CARTESIAN_POINT('Ctrl Pts',(-0.021276461800953,1.7783330578041,7.0295935880953));
#49363=CARTESIAN_POINT('Ctrl Pts',(-0.0290734210578596,1.7789438829891,
7.02912704993763));
#49364=CARTESIAN_POINT('Ctrl Pts',(-0.0379084492797415,1.7799604996421,
7.028586007225));
#49365=CARTESIAN_POINT('Ctrl Pts',(-0.0389762625904412,1.78008878852612,
7.02852041092111));
#49366=CARTESIAN_POINT('Ctrl Pts',(-0.040553489288687,1.78028629307028,
7.02842321109846));
#49367=CARTESIAN_POINT('Ctrl Pts',(-0.0410634189600968,1.78035138744131,
7.0283917376933));
#49368=CARTESIAN_POINT('Ctrl Pts',(-0.0419658189716715,1.78046877706466,
7.02833595489603));
#49369=CARTESIAN_POINT('Ctrl Pts',(-0.0423583537076367,1.78052057615322,
7.02831166122327));
#49370=CARTESIAN_POINT('Ctrl Pts',(-0.0431723950779367,1.78062952412216,
7.02826122081048));
#49371=CARTESIAN_POINT('Ctrl Pts',(-0.0435938858058917,1.78068678436872,
7.02823507059398));
#49372=CARTESIAN_POINT('Ctrl Pts',(-0.0446783049670126,1.7808362917329,
7.02816770423745));
#49373=CARTESIAN_POINT('Ctrl Pts',(-0.0453410591795403,1.78092976956286,
7.02812644923911));
#49374=CARTESIAN_POINT('Ctrl Pts',(-0.0480900439311412,1.78132623662172,
7.02795498138124));
#49375=CARTESIAN_POINT('Ctrl Pts',(-0.0501735304390813,1.78164762244515,
7.02782418738384));
#49376=CARTESIAN_POINT('Ctrl Pts',(-0.0641545443459592,1.78394490247736,
7.02694072312956));
#49377=CARTESIAN_POINT('Ctrl Pts',(-0.0759348263133994,1.7865666399145,
7.02616755813896));
#49378=CARTESIAN_POINT('Ctrl Pts',(-0.102770014943821,1.79414063616274,
7.0243383787038));
#49379=CARTESIAN_POINT('Ctrl Pts',(-0.117662081075645,1.79955502941144,
7.02327128856972));
#49380=CARTESIAN_POINT('Ctrl Pts',(-0.139114226304058,1.80919486349171,
7.02167973772876));
#49381=CARTESIAN_POINT('Ctrl Pts',(-0.146018417557063,1.81259954576611,
7.02115887252852));
#49382=CARTESIAN_POINT('Ctrl Pts',(-0.159072875774539,1.81962908825824,
7.02016372087672));
#49383=CARTESIAN_POINT('Ctrl Pts',(-0.165237959194082,1.82321767393432,
7.01968909304237));
#49384=CARTESIAN_POINT('Ctrl Pts',(-0.176789487094563,1.83046527398876,
7.01879714209522));
#49385=CARTESIAN_POINT('Ctrl Pts',(-0.182194315061004,1.83408885459154,
7.01837865058815));
#49386=CARTESIAN_POINT('Ctrl Pts',(-0.187982182717425,1.83822863698592,
7.01793236177384));
#49387=CARTESIAN_POINT('Ctrl Pts',(-0.188477189113209,1.83858481927819,
7.01789420844203));
#49388=CARTESIAN_POINT('Ctrl Pts',(-0.189209832866408,1.839115156504,7.01783776548697));
#49389=CARTESIAN_POINT('Ctrl Pts',(-0.189448243638212,1.83928823309377,
7.01781940249247));
#49390=CARTESIAN_POINT('Ctrl Pts',(-0.189855654552497,1.83958485089738,
7.01778803034999));
#49391=CARTESIAN_POINT('Ctrl Pts',(-0.190024771683044,1.8397082298745,7.01777500997241));
#49392=CARTESIAN_POINT('Ctrl Pts',(-0.190368614716663,1.83995959340003,
7.0177485422127));
#49393=CARTESIAN_POINT('Ctrl Pts',(-0.190543331373119,1.84008758897803,
7.01773509574301));
#49394=CARTESIAN_POINT('Ctrl Pts',(-0.190948932848502,1.8403853571173,7.01770388571654));
#49395=CARTESIAN_POINT('Ctrl Pts',(-0.191179721085091,1.84055526214154,
7.01768613142032));
#49396=CARTESIAN_POINT('Ctrl Pts',(-0.191665781114701,1.8409140975815,7.01764874766298));
#49397=CARTESIAN_POINT('Ctrl Pts',(-0.191921001122467,1.84110309810175,
7.01762912308646));
#49398=CARTESIAN_POINT('Ctrl Pts',(-0.192602322693779,1.84160920481811,
7.01757674613616));
#49399=CARTESIAN_POINT('Ctrl Pts',(-0.193027922628295,1.84192698932877,
7.01754404024286));
#49400=CARTESIAN_POINT('Ctrl Pts',(-0.194323272981757,1.8428991911382,7.01744452808297));
#49401=CARTESIAN_POINT('Ctrl Pts',(-0.195190506016894,1.84355697167317,
7.01737794786246));
#49402=CARTESIAN_POINT('Ctrl Pts',(-0.198348405524655,1.84597748161646,
7.0171355953482));
#49403=CARTESIAN_POINT('Ctrl Pts',(-0.200618737009237,1.84776666861259,
7.01696153207827));
#49404=CARTESIAN_POINT('Ctrl Pts',(-0.208549356609901,1.85419140850358,
7.01635289538663));
#49405=CARTESIAN_POINT('Ctrl Pts',(-0.214075883094494,1.85898915188719,
7.01592762920278));
#49406=CARTESIAN_POINT('Ctrl Pts',(-0.238614424206793,1.88180249401936,
7.01400894883816));
#49407=CARTESIAN_POINT('Ctrl Pts',(-0.255549485726991,1.90190513946523,
7.01258879534681));
#49408=CARTESIAN_POINT('Ctrl Pts',(-0.270952827447319,1.92550158926302,
7.01096842668715));
#49409=CARTESIAN_POINT('Ctrl Pts',(-0.27202438237476,1.92717678035148,7.01085367388661));
#49410=CARTESIAN_POINT('Ctrl Pts',(-0.274571356972268,1.93124091425272,
7.01057581224792));
#49411=CARTESIAN_POINT('Ctrl Pts',(-0.27603117631089,1.93363940314634,7.01041226987453));
#49412=CARTESIAN_POINT('Ctrl Pts',(-0.278372731157117,1.93760227423902,
7.01014253190899));
#49413=CARTESIAN_POINT('Ctrl Pts',(-0.27927307574866,1.93915551680862,7.01003692579288));
#49414=CARTESIAN_POINT('Ctrl Pts',(-0.283365489180155,1.94635356190852,
7.00954790329499));
#49415=CARTESIAN_POINT('Ctrl Pts',(-0.28639952388579,1.95208606518621,7.0091594690034));
#49416=CARTESIAN_POINT('Ctrl Pts',(-0.289713480954574,1.95883222838706,
7.00870201336474));
#49417=CARTESIAN_POINT('Ctrl Pts',(-0.290164072810823,1.95976073445727,
7.00863904550273));
#49418=CARTESIAN_POINT('Ctrl Pts',(-0.290827781224833,1.96114528934606,
7.00854513519034));
#49419=CARTESIAN_POINT('Ctrl Pts',(-0.291044304912739,1.96159970528837,
7.00851431111334));
#49420=CARTESIAN_POINT('Ctrl Pts',(-0.291428078337402,1.96241000977351,
7.00845934132245));
#49421=CARTESIAN_POINT('Ctrl Pts',(-0.291595743367116,1.96276570143743,
7.00843521005259));
#49422=CARTESIAN_POINT('Ctrl Pts',(-0.291947354211031,1.96351517704731,
7.00838435921913));
#49423=CARTESIAN_POINT('Ctrl Pts',(-0.29213115512795,1.96390902775014,7.00835763470621));
#49424=CARTESIAN_POINT('Ctrl Pts',(-0.292613457736634,1.96494799057286,
7.00828712972692));
#49425=CARTESIAN_POINT('Ctrl Pts',(-0.292910621554807,1.96559371790599,
7.00824330321898));
#49426=CARTESIAN_POINT('Ctrl Pts',(-0.294236129383136,1.9684992770775,7.00804606305707));
#49427=CARTESIAN_POINT('Ctrl Pts',(-0.295240452219731,1.97076991533785,
7.00789182680763));
#49428=CARTESIAN_POINT('Ctrl Pts',(-0.302439557748369,1.98756817643144,
7.00674980513678));
#49429=CARTESIAN_POINT('Ctrl Pts',(-0.307584287626813,2.00251987872177,
7.00572636306098));
#49430=CARTESIAN_POINT('Ctrl Pts',(-0.318700063766326,2.04465176146148,
7.00282978814953));
#49431=CARTESIAN_POINT('Ctrl Pts',(-0.322283427778208,2.07231762602878,
7.00090542424288));
#49432=CARTESIAN_POINT('Ctrl Pts',(-0.322274985117328,2.10009794195348,
6.99910071866258));
#49433=CARTESIAN_POINT('',(-0.322274994862272,2.1000575458305,6.74968051971722));
#49434=CARTESIAN_POINT('Ctrl Pts',(-0.32227498500109,2.10009832368563,6.99910069386394));
#49435=CARTESIAN_POINT('Ctrl Pts',(-0.322273394266979,2.10531226383204,
6.99876197848564));
#49436=CARTESIAN_POINT('Ctrl Pts',(-0.322145272370923,2.11052583289153,
6.99842819032332));
#49437=CARTESIAN_POINT('Ctrl Pts',(-0.321867792789241,2.11620244344203,
6.99807173565523));
#49438=CARTESIAN_POINT('Ctrl Pts',(-0.321843893543514,2.11667043502029,
6.99804240060918));
#49439=CARTESIAN_POINT('Ctrl Pts',(-0.321803465791486,2.11742957447782,
6.99799490147959));
#49440=CARTESIAN_POINT('Ctrl Pts',(-0.321787562812519,2.11772075288088,
6.99797670303981));
#49441=CARTESIAN_POINT('Ctrl Pts',(-0.321759019854199,2.11823065457684,
6.99794487094262));
#49442=CARTESIAN_POINT('Ctrl Pts',(-0.321746552046533,2.11844938672925,
6.99793122768086));
#49443=CARTESIAN_POINT('Ctrl Pts',(-0.321721866840363,2.11887482176612,
6.99790471451509));
#49444=CARTESIAN_POINT('Ctrl Pts',(-0.321709673247518,2.11908152614001,
6.99789184325585));
#49445=CARTESIAN_POINT('Ctrl Pts',(-0.321685015419126,2.11949278007728,
6.99786625615442));
#49446=CARTESIAN_POINT('Ctrl Pts',(-0.321672555309565,2.11969732929989,
6.99785354009536));
#49447=CARTESIAN_POINT('Ctrl Pts',(-0.321642742305764,2.12017917593869,
6.99782360979231));
#49448=CARTESIAN_POINT('Ctrl Pts',(-0.321625225872823,2.12045646360296,
6.99780640479926));
#49449=CARTESIAN_POINT('Ctrl Pts',(-0.321572420438914,2.12127554517366,
6.99775563797857));
#49450=CARTESIAN_POINT('Ctrl Pts',(-0.321536120631604,2.12181727638075,
6.99772213261776));
#49451=CARTESIAN_POINT('Ctrl Pts',(-0.32120570653987,2.12656829426715,6.99742889318035));
#49452=CARTESIAN_POINT('Ctrl Pts',(-0.320830302455053,2.13077176228369,
6.99717361353515));
#49453=CARTESIAN_POINT('Ctrl Pts',(-0.32033974101806,2.13526636794511,6.99690396535509));
#49454=CARTESIAN_POINT('Ctrl Pts',(-0.320306634053047,2.13556580614128,
6.9968860167309));
#49455=CARTESIAN_POINT('Ctrl Pts',(-0.320118844803548,2.13724274782419,
6.99678558545158));
#49456=CARTESIAN_POINT('Ctrl Pts',(-0.319955694016345,2.13861930930996,
6.99670346994184));
#49457=CARTESIAN_POINT('Ctrl Pts',(-0.315779900155303,2.17200741899123,
6.99471878398271));
#49458=CARTESIAN_POINT('Ctrl Pts',(-0.306991855219437,2.20324023676939,
6.99300120510939));
#49459=CARTESIAN_POINT('Ctrl Pts',(-0.289054325424564,2.24295688091424,
6.99049160961168));
#49460=CARTESIAN_POINT('Ctrl Pts',(-0.283860587421136,2.2530104494352,6.98982699886512));
#49461=CARTESIAN_POINT('Ctrl Pts',(-0.277126329547365,2.26451832250975,
6.98902073630722));
#49462=CARTESIAN_POINT('Ctrl Pts',(-0.276086535752685,2.26625734707131,
6.98889763324885));
#49463=CARTESIAN_POINT('Ctrl Pts',(-0.274686733095346,2.2685491295007,6.98873367449715));
#49464=CARTESIAN_POINT('Ctrl Pts',(-0.27434131110749,2.26911077849646,6.98869335426107));
#49465=CARTESIAN_POINT('Ctrl Pts',(-0.273771384873471,2.27003112513138,
6.98862705367126));
#49466=CARTESIAN_POINT('Ctrl Pts',(-0.273547892310323,2.27039044955294,
6.9886011106434));
#49467=CARTESIAN_POINT('Ctrl Pts',(-0.273113459798528,2.27108585900339,
6.98855078992826));
#49468=CARTESIAN_POINT('Ctrl Pts',(-0.272902605469578,2.27142199683741,
6.98852641543805));
#49469=CARTESIAN_POINT('Ctrl Pts',(-0.27241433569225,2.27219719820903,6.98847008433365));
#49470=CARTESIAN_POINT('Ctrl Pts',(-0.272136479151973,2.2726359813927,6.98843811140357));
#49471=CARTESIAN_POINT('Ctrl Pts',(-0.271243171722151,2.27403915146648,
6.98833558221727));
#49472=CARTESIAN_POINT('Ctrl Pts',(-0.270623651009538,2.27500092545252,
6.98826487470105));
#49473=CARTESIAN_POINT('Ctrl Pts',(-0.264866287043823,2.28383525279775,
6.98761137079271));
#49474=CARTESIAN_POINT('Ctrl Pts',(-0.259391885455071,2.29148203631538,
6.9870159303062));
#49475=CARTESIAN_POINT('Ctrl Pts',(-0.235552082798775,2.32188042687472,
6.98451933145408));
#49476=CARTESIAN_POINT('Ctrl Pts',(-0.214467866925369,2.34231946544718,
6.98250932336448));
#49477=CARTESIAN_POINT('Ctrl Pts',(-0.184030761605687,2.36470187333624,
6.97998487286626));
#49478=CARTESIAN_POINT('Ctrl Pts',(-0.176937026545758,2.36949529789416,
6.97942031534484));
#49479=CARTESIAN_POINT('Ctrl Pts',(-0.167631499824653,2.37525724384033,
6.97871713224788));
#49480=CARTESIAN_POINT('Ctrl Pts',(-0.165588693619503,2.37649096789478,
6.97856498740824));
#49481=CARTESIAN_POINT('Ctrl Pts',(-0.162717171365165,2.37818194158573,
6.97835440533843));
#49482=CARTESIAN_POINT('Ctrl Pts',(-0.161899916087764,2.37865837095621,
6.97829483936127));
#49483=CARTESIAN_POINT('Ctrl Pts',(-0.160665351903121,2.37937081117379,
6.97820542327895));
#49484=CARTESIAN_POINT('Ctrl Pts',(-0.160249603381173,2.37960949565634,
6.97817540791408));
#49485=CARTESIAN_POINT('Ctrl Pts',(-0.159486550367137,2.38004530946413,
6.97812049680117));
#49486=CARTESIAN_POINT('Ctrl Pts',(-0.159139409983029,2.38024272210929,
6.97809558313884));
#49487=CARTESIAN_POINT('Ctrl Pts',(-0.158582223805795,2.38055821495373,
6.97805570390672));
#49488=CARTESIAN_POINT('Ctrl Pts',(-0.158372412372924,2.380676704921,6.9780407119037));
#49489=CARTESIAN_POINT('Ctrl Pts',(-0.157982181064083,2.38089650924615,
6.97801287429366));
#49490=CARTESIAN_POINT('Ctrl Pts',(-0.157801797929628,2.38099788435305,
6.97800002481374));
#49491=CARTESIAN_POINT('Ctrl Pts',(-0.157382180554519,2.38123317733665,
6.97797017614492));
#49492=CARTESIAN_POINT('Ctrl Pts',(-0.157142873320758,2.38136696351348,
6.97795318554275));
#49493=CARTESIAN_POINT('Ctrl Pts',(-0.156530316076124,2.38170839214302,
6.97790977569463));
#49494=CARTESIAN_POINT('Ctrl Pts',(-0.156156821997096,2.38191559907786,
6.97788338440571));
#49495=CARTESIAN_POINT('Ctrl Pts',(-0.154031874119382,2.38308895846926,
6.97773366502484));
#49496=CARTESIAN_POINT('Ctrl Pts',(-0.152271817580715,2.38403955833609,
6.97761131482827));
#49497=CARTESIAN_POINT('Ctrl Pts',(-0.132996409234559,2.39421946570283,
6.97628812709693));
#49498=CARTESIAN_POINT('Ctrl Pts',(-0.114672298495858,2.40183379499441,
6.97517851398256));
#49499=CARTESIAN_POINT('Ctrl Pts',(-0.0938863658221463,2.40830242909191,
6.97396111011352));
#49500=CARTESIAN_POINT('Ctrl Pts',(-0.0920046665540028,2.40886919369937,
6.97385127803034));
#49501=CARTESIAN_POINT('Ctrl Pts',(-0.0879526054814601,2.41004935255688,
6.97361538203055));
#49502=CARTESIAN_POINT('Ctrl Pts',(-0.0857807539178932,2.41065724530525,
6.97348932208326));
#49503=CARTESIAN_POINT('Ctrl Pts',(-0.0810520792391858,2.41192741328235,
6.97321539659832));
#49504=CARTESIAN_POINT('Ctrl Pts',(-0.0784931409081298,2.41258115331239,
6.9730675001931));
#49505=CARTESIAN_POINT('Ctrl Pts',(-0.0667661940520024,2.41542398889303,
6.97239038693641));
#49506=CARTESIAN_POINT('Ctrl Pts',(-0.0575132821026026,2.41724158985611,
6.97185778658866));
#49507=CARTESIAN_POINT('Ctrl Pts',(-0.0367958541192967,2.42037499802886,
6.97065226152938));
#49508=CARTESIAN_POINT('Ctrl Pts',(-0.0253141728361465,2.42148596013398,
6.96997527966138));
#49509=CARTESIAN_POINT('Ctrl Pts',(-0.0117501107282478,2.42206725093508,
6.96915443788295));
#49510=CARTESIAN_POINT('Ctrl Pts',(-0.00970096885915303,2.42213548411976,
6.96902988130061));
#49511=CARTESIAN_POINT('Ctrl Pts',(-0.00698920707422366,2.42219988406561,
6.96886427509015));
#49512=CARTESIAN_POINT('Ctrl Pts',(-0.00632701975015583,2.42221356755757,
6.96882377469974));
#49513=CARTESIAN_POINT('Ctrl Pts',(-0.00524104965174637,2.42223265918029,
6.96875725365457));
#49514=CARTESIAN_POINT('Ctrl Pts',(-0.00481728781338862,2.42223927286918,
6.96873127081524));
#49515=CARTESIAN_POINT('Ctrl Pts',(-0.00399701985856119,2.42225045647054,
6.96868092680914));
#49516=CARTESIAN_POINT('Ctrl Pts',(-0.00360051573593683,2.42225513052149,
6.96865656895111));
#49517=CARTESIAN_POINT('Ctrl Pts',(-0.00268628056280024,2.42226422014744,
6.96860035401023));
#49518=CARTESIAN_POINT('Ctrl Pts',(-0.00216854650016921,2.42226811988093,
6.96856848082419));
#49519=CARTESIAN_POINT('Ctrl Pts',(-0.000515452643909905,2.42227658772934,
6.96846658740692));
#49520=CARTESIAN_POINT('Ctrl Pts',(0.000619913366854447,2.42227640364203,
6.96839641854809));
#49521=CARTESIAN_POINT('Ctrl Pts',(0.0108824700208385,2.42222050867727,
6.96776043564784));
#49522=CARTESIAN_POINT('Ctrl Pts',(0.0200026256392138,2.42178308238356,
6.96718271374627));
#49523=CARTESIAN_POINT('Ctrl Pts',(0.0596250680880687,2.41819176736287,
6.96461456766074));
#49524=CARTESIAN_POINT('Ctrl Pts',(0.0896057403424972,2.4110809580207,6.96250024377681));
#49525=CARTESIAN_POINT('Ctrl Pts',(0.125298904738283,2.39701996736983,6.95994595440756));
#49526=CARTESIAN_POINT('Ctrl Pts',(0.132372546605577,2.39393571427577,6.95943902950059));
#49527=CARTESIAN_POINT('Ctrl Pts',(0.141312269856743,2.38964953762658,6.95880326612892));
#49528=CARTESIAN_POINT('Ctrl Pts',(0.143285631997231,2.3886784379294,6.95866324562129));
#49529=CARTESIAN_POINT('Ctrl Pts',(0.146044286349171,2.38728563458223,6.95846811341724));
#49530=CARTESIAN_POINT('Ctrl Pts',(0.146837956253646,2.38688078370494,6.95841204504113));
#49531=CARTESIAN_POINT('Ctrl Pts',(0.148037893508134,2.38626241165553,6.95832739632403));
#49532=CARTESIAN_POINT('Ctrl Pts',(0.148445392674245,2.38605130945526,6.95829867067977));
#49533=CARTESIAN_POINT('Ctrl Pts',(0.149194454012507,2.38566123154884,6.95824590825582));
#49534=CARTESIAN_POINT('Ctrl Pts',(0.149536147759728,2.38548251231025,6.9582218556822));
#49535=CARTESIAN_POINT('Ctrl Pts',(0.150087939196921,2.38519264125609,6.95818304023658));
#49536=CARTESIAN_POINT('Ctrl Pts',(0.150298234827975,2.38508187021884,6.95816825331665));
#49537=CARTESIAN_POINT('Ctrl Pts',(0.150694815817619,2.38487241451412,6.95814037974676));
#49538=CARTESIAN_POINT('Ctrl Pts',(0.15088112537651,2.38477378051843,6.95812729007382));
#49539=CARTESIAN_POINT('Ctrl Pts',(0.151316019368364,2.38454299703938,6.95809674700003));
#49540=CARTESIAN_POINT('Ctrl Pts',(0.15156452726259,2.38441070471899,6.95807930282999));
#49541=CARTESIAN_POINT('Ctrl Pts',(0.152325769628742,2.38400417889688,6.95802589296917));
#49542=CARTESIAN_POINT('Ctrl Pts',(0.152837939128523,2.38372888132738,6.95798999467129));
#49543=CARTESIAN_POINT('Ctrl Pts',(0.156627816565253,2.38167853454191,6.95772460772769));
#49544=CARTESIAN_POINT('Ctrl Pts',(0.159875421734633,2.37984803408106,6.95749857086763));
#49545=CARTESIAN_POINT('Ctrl Pts',(0.164132834958942,2.377350046031,6.95720310573676));
#49546=CARTESIAN_POINT('Ctrl Pts',(0.165171534876961,2.37673272248986,6.95713108838754));
#49547=CARTESIAN_POINT('Ctrl Pts',(0.190569902439562,2.3614439357857,6.95537118471046));
#49548=CARTESIAN_POINT('Ctrl Pts',(0.212887726553306,2.34361663975742,6.95383950088785));
#49549=CARTESIAN_POINT('Ctrl Pts',(0.243368060118813,2.31183989033175,6.95134275884058));
#49550=CARTESIAN_POINT('Ctrl Pts',(0.253326655899653,2.29982407804502,6.95043992887395));
#49551=CARTESIAN_POINT('Ctrl Pts',(0.263806903086126,2.28513012725054,6.94935131992476));
#49552=CARTESIAN_POINT('Ctrl Pts',(0.265214503632972,2.2831079263007,6.94920185564619));
#49553=CARTESIAN_POINT('Ctrl Pts',(0.266997025919563,2.28048342380292,6.94900824714265));
#49554=CARTESIAN_POINT('Ctrl Pts',(0.267393363670245,2.27989571192773,6.94896491573033));
#49555=CARTESIAN_POINT('Ctrl Pts',(0.268029330631227,2.27894591939361,6.9488949248741));
#49556=CARTESIAN_POINT('Ctrl Pts',(0.268270174264727,2.27858465147739,6.94886831124896));
#49557=CARTESIAN_POINT('Ctrl Pts',(0.268727803179391,2.27789518861216,6.94881753597199));
#49558=CARTESIAN_POINT('Ctrl Pts',(0.268944719300638,2.27756708110204,6.94879337929579));
#49559=CARTESIAN_POINT('Ctrl Pts',(0.269438315988197,2.27681748699173,6.94873820580667));
#49560=CARTESIAN_POINT('Ctrl Pts',(0.269714608703757,2.27639574732913,6.94870717454158));
#49561=CARTESIAN_POINT('Ctrl Pts',(0.270555703094034,2.27510528498643,6.94861225472244));
#49562=CARTESIAN_POINT('Ctrl Pts',(0.271117301563292,2.27423449159038,6.9485482468758));
#49563=CARTESIAN_POINT('Ctrl Pts',(0.275210790886447,2.26781956931179,6.9480770109686));
#49564=CARTESIAN_POINT('Ctrl Pts',(0.278576293876997,2.26217159275179,6.94766367350334));
#49565=CARTESIAN_POINT('Ctrl Pts',(0.282653724290684,2.25482696303102,6.94712756585211));
#49566=CARTESIAN_POINT('Ctrl Pts',(0.283527253119232,2.25322145039925,6.94701046102636));
#49567=CARTESIAN_POINT('Ctrl Pts',(0.285298737847155,2.24989850383514,6.94676826308245));
#49568=CARTESIAN_POINT('Ctrl Pts',(0.286194952593266,2.24818022855193,6.94664311911745));
#49569=CARTESIAN_POINT('Ctrl Pts',(0.298091782716582,2.22486034925084,6.94494602460441));
#49570=CARTESIAN_POINT('Ctrl Pts',(0.306635215845854,2.20209484628449,6.94329581408604));
#49571=CARTESIAN_POINT('Ctrl Pts',(0.316142480546548,2.16428602616906,6.94066684637796));
#49572=CARTESIAN_POINT('Ctrl Pts',(0.318753728565432,2.14974864251369,6.93968324102719));
#49573=CARTESIAN_POINT('Ctrl Pts',(0.320486526218191,2.13392515833847,6.93867441178746));
#49574=CARTESIAN_POINT('Ctrl Pts',(0.320606940511019,2.13276766160089,6.93860097298848));
#49575=CARTESIAN_POINT('Ctrl Pts',(0.320775798152535,2.13105437365884,6.93849282528215));
#49576=CARTESIAN_POINT('Ctrl Pts',(0.320829070886706,2.13049908340601,6.93845785974242));
#49577=CARTESIAN_POINT('Ctrl Pts',(0.320911428320434,2.12961652816779,6.93840242657818));
#49578=CARTESIAN_POINT('Ctrl Pts',(0.320941454527024,2.12928935533131,6.93838190737019));
#49579=CARTESIAN_POINT('Ctrl Pts',(0.320997415878419,2.12866916729754,6.9383430696867));
#49580=CARTESIAN_POINT('Ctrl Pts',(0.32102345023802,2.12837616170463,6.93832474569242));
#49581=CARTESIAN_POINT('Ctrl Pts',(0.321068071608576,2.12786604564961,6.93829288756417));
#49582=CARTESIAN_POINT('Ctrl Pts',(0.321086839633682,2.12764895154931,6.93827934317457));
#49583=CARTESIAN_POINT('Ctrl Pts',(0.321123004925041,2.12722561607012,6.93825295843833));
#49584=CARTESIAN_POINT('Ctrl Pts',(0.321140423656682,2.12701937742996,6.93824011688432));
#49585=CARTESIAN_POINT('Ctrl Pts',(0.321181417325203,2.1265283704418,6.93820957339484));
#49586=CARTESIAN_POINT('Ctrl Pts',(0.321204812283448,2.12624358665925,6.93819188165318));
#49587=CARTESIAN_POINT('Ctrl Pts',(0.321286379545042,2.12523422938029,6.93812925889149));
#49588=CARTESIAN_POINT('Ctrl Pts',(0.32134247968654,2.12450948360557,6.93808444370854));
#49589=CARTESIAN_POINT('Ctrl Pts',(0.322111366347603,2.11411966174511,6.93744404656483));
#49590=CARTESIAN_POINT('Ctrl Pts',(0.32239036438792,2.10442631684681,6.93687214513714));
#49591=CARTESIAN_POINT('Ctrl Pts',(0.321852418837991,2.07150810366417,6.93497269784012));
#49592=CARTESIAN_POINT('Ctrl Pts',(0.318962891790567,2.04839014403216,6.93370646204764));
#49593=CARTESIAN_POINT('Ctrl Pts',(0.309982060241883,2.01044081060017,6.93149636702036));
#49594=CARTESIAN_POINT('Ctrl Pts',(0.305231036311781,1.99538813201605,6.9305837977769));
#49595=CARTESIAN_POINT('Ctrl Pts',(0.298480471687236,1.97844040335145,6.9294835779352));
#49596=CARTESIAN_POINT('Ctrl Pts',(0.297536105993452,1.9761468909733,6.92933312352238));
#49597=CARTESIAN_POINT('Ctrl Pts',(0.296287271464342,1.97321067355542,6.92913840986515));
#49598=CARTESIAN_POINT('Ctrl Pts',(0.296007001659939,1.97255771703389,6.9290949749859));
#49599=CARTESIAN_POINT('Ctrl Pts',(0.295551847947904,1.97150692761235,6.929024857203));
#49600=CARTESIAN_POINT('Ctrl Pts',(0.295378313704991,1.97110850971881,6.92899822042185));
#49601=CARTESIAN_POINT('Ctrl Pts',(0.295046214880956,1.97035023583254,6.928947427445));
#49602=CARTESIAN_POINT('Ctrl Pts',(0.294887796349065,1.9699903164127,6.92892327628318));
#49603=CARTESIAN_POINT('Ctrl Pts',(0.294525050592844,1.96917024923822,6.92886815228869));
#49604=CARTESIAN_POINT('Ctrl Pts',(0.294320303394191,1.96871028937319,6.92883716509837));
#49605=CARTESIAN_POINT('Ctrl Pts',(0.293692340120795,1.9673084356217,6.92874251061871));
#49606=CARTESIAN_POINT('Ctrl Pts',(0.293265677318592,1.96636810122615,6.92867872501006));
#49607=CARTESIAN_POINT('Ctrl Pts',(0.290121850734225,1.95952690461709,6.92821250125667));
#49608=CARTESIAN_POINT('Ctrl Pts',(0.287231503819866,1.95370771684781,6.92780409887163));
#49609=CARTESIAN_POINT('Ctrl Pts',(0.283899414759614,1.94747911349576,6.92735345722573));
#49610=CARTESIAN_POINT('Ctrl Pts',(0.283630048128706,1.94697877822692,6.92731716159109));
#49611=CARTESIAN_POINT('Ctrl Pts',(0.271417985970904,1.92443850200028,6.92567768107543));
#49612=CARTESIAN_POINT('Ctrl Pts',(0.256947513233204,1.90386961286809,6.92398352181387));
#49613=CARTESIAN_POINT('Ctrl Pts',(0.228040005636204,1.87153956041951,6.92105111557454));
#49614=CARTESIAN_POINT('Ctrl Pts',(0.214693091686178,1.85895338038718,6.91982126999722));
#49615=CARTESIAN_POINT('Ctrl Pts',(0.199886318280011,1.84720169636082,6.91863315240455));
#49616=CARTESIAN_POINT('Ctrl Pts',(0.199423949828565,1.84683679018081,6.91859621737979));
#49617=CARTESIAN_POINT('Ctrl Pts',(0.198692118076695,1.84626246967197,6.91853802232602));
#49618=CARTESIAN_POINT('Ctrl Pts',(0.198423320908865,1.84605221441247,6.91851670391454));
#49619=CARTESIAN_POINT('Ctrl Pts',(0.197914904149887,1.84565582687712,6.91847648815419));
#49620=CARTESIAN_POINT('Ctrl Pts',(0.197675354960741,1.84546960549047,6.91845758452485));
#49621=CARTESIAN_POINT('Ctrl Pts',(0.197262134182775,1.84514931002756,6.91842505337062));
#49622=CARTESIAN_POINT('Ctrl Pts',(0.197088588311663,1.8450150747198,6.9184114143137));
#49623=CARTESIAN_POINT('Ctrl Pts',(0.196752807257615,1.84475590038029,6.91838507069755));
#49624=CARTESIAN_POINT('Ctrl Pts',(0.196590590281329,1.84463093889852,6.91837236450968));
#49625=CARTESIAN_POINT('Ctrl Pts',(0.196208491037982,1.84433717416897,6.91834248324089));
#49626=CARTESIAN_POINT('Ctrl Pts',(0.195988509435892,1.8441684995202,6.91832531733573));
#49627=CARTESIAN_POINT('Ctrl Pts',(0.195338983689398,1.84367179400804,6.91827474164998));
#49628=CARTESIAN_POINT('Ctrl Pts',(0.194908828971717,1.84334455755875,6.91824138773807));
#49629=CARTESIAN_POINT('Ctrl Pts',(0.191166823699058,1.84051269277339,6.91795243149008));
#49630=CARTESIAN_POINT('Ctrl Pts',(0.187807489204289,1.83807106295716,6.91770114147994));
#49631=CARTESIAN_POINT('Ctrl Pts',(0.183566128132596,1.83511192874879,6.91739255719391));
#49632=CARTESIAN_POINT('Ctrl Pts',(0.182727772609372,1.83453291191579,6.91733197590658));
#49633=CARTESIAN_POINT('Ctrl Pts',(0.181778311629421,1.833883788022,6.91726381478149));
#49634=CARTESIAN_POINT('Ctrl Pts',(0.181669902560216,1.83380976847332,6.91725603875078));
#49635=CARTESIAN_POINT('Ctrl Pts',(0.154562124296756,1.81532539184354,6.91531327142513));
#49636=CARTESIAN_POINT('Ctrl Pts',(0.124917153115547,1.80112648572427,6.91357604414492));
#49637=CARTESIAN_POINT('Ctrl Pts',(0.0826551035956213,1.78829325885977,
6.91103437492983));
#49638=CARTESIAN_POINT('Ctrl Pts',(0.0715014141846555,1.78554736039482,
6.91036013049811));
#49639=CARTESIAN_POINT('Ctrl Pts',(0.0582169252453551,1.78302027344488,
6.90954251553464));
#49640=CARTESIAN_POINT('Ctrl Pts',(0.0562044489489573,1.78265725618581,
6.90941827987079));
#49641=CARTESIAN_POINT('Ctrl Pts',(0.0535364302666989,1.78220216476578,
6.90925303725696));
#49642=CARTESIAN_POINT('Ctrl Pts',(0.0528838338990607,1.78209291680256,
6.90921257648701));
#49643=CARTESIAN_POINT('Ctrl Pts',(0.0518128402288578,1.78191701600195,
6.90914610393067));
#49644=CARTESIAN_POINT('Ctrl Pts',(0.0513946375285838,1.78184917672231,
6.90912012985185));
#49645=CARTESIAN_POINT('Ctrl Pts',(0.0505847061135226,1.78171943129307,
6.9090697910182));
#49646=CARTESIAN_POINT('Ctrl Pts',(0.0501929943173326,1.78165742316143,
6.90904542954759));
#49647=CARTESIAN_POINT('Ctrl Pts',(0.0492892917034664,1.78151607610713,
6.90898918926951));
#49648=CARTESIAN_POINT('Ctrl Pts',(0.0487772230392013,1.78143724862688,
6.90895729431251));
#49649=CARTESIAN_POINT('Ctrl Pts',(0.0471405363606278,1.78118933704483,
6.90885526233408));
#49650=CARTESIAN_POINT('Ctrl Pts',(0.0460152219047196,1.78102497232196,
6.90878497611335));
#49651=CARTESIAN_POINT('Ctrl Pts',(0.0357923533436014,1.77958703118773,
6.90814521714678));
#49652=CARTESIAN_POINT('Ctrl Pts',(0.0266459279117729,1.77869713677329,
6.90756367982536));
#49653=CARTESIAN_POINT('Ctrl Pts',(0.00364717829017836,1.77744824073949,
6.90607653057318));
#49654=CARTESIAN_POINT('Ctrl Pts',(-0.010212887235651,1.77758945001044,
6.90515729329815));
#49655=CARTESIAN_POINT('Ctrl Pts',(-0.0265538545387822,1.77881076178086,
6.90405449597907));
#49656=CARTESIAN_POINT('Ctrl Pts',(-0.0290857581000178,1.77903013784536,
6.90388311388462));
#49657=CARTESIAN_POINT('Ctrl Pts',(-0.0473557742994512,1.78083109058061,
6.90264333602232));
#49658=CARTESIAN_POINT('Ctrl Pts',(-0.0629615621932782,1.78353952297314,
6.90156639038665));
#49659=CARTESIAN_POINT('Ctrl Pts',(-0.0844770125753363,1.78892881189273,
6.90009845058249));
#49660=CARTESIAN_POINT('Ctrl Pts',(-0.0906016051843381,1.79065713166265,
6.8996827449379));
#49661=CARTESIAN_POINT('Ctrl Pts',(-0.0995682394324341,1.79347665235741,
6.89908117617267));
#49662=CARTESIAN_POINT('Ctrl Pts',(-0.102452177267187,1.79442848631939,
6.89888879313964));
#49663=CARTESIAN_POINT('Ctrl Pts',(-0.105801639720041,1.79558671868842,
6.89866699574018));
#49664=CARTESIAN_POINT('Ctrl Pts',(-0.106280535921204,1.79575358588968,
6.89863532320484));
#49665=CARTESIAN_POINT('Ctrl Pts',(-0.107010300769191,1.79600979938799,
6.89858712139764));
#49666=CARTESIAN_POINT('Ctrl Pts',(-0.107261453077407,1.79609832638862,
6.89857054377367));
#49667=CARTESIAN_POINT('Ctrl Pts',(-0.107697985044939,1.79625280518676,
6.89854174990624));
#49668=CARTESIAN_POINT('Ctrl Pts',(-0.107883413551028,1.79631861528745,
6.89852952524031));
#49669=CARTESIAN_POINT('Ctrl Pts',(-0.108272567874009,1.79645713076986,
6.89850388288329));
#49670=CARTESIAN_POINT('Ctrl Pts',(-0.108476280120566,1.7965298712124,6.89849046736948));
#49671=CARTESIAN_POINT('Ctrl Pts',(-0.109045926371561,1.79673392422367,
6.89845297404889));
#49672=CARTESIAN_POINT('Ctrl Pts',(-0.109411697792418,1.79686569450991,
6.89842892357794));
#49673=CARTESIAN_POINT('Ctrl Pts',(-0.11089131205112,1.79740175706444,6.8983317290609));
#49674=CARTESIAN_POINT('Ctrl Pts',(-0.112003177681355,1.79781153561437,
6.89825890785515));
#49675=CARTESIAN_POINT('Ctrl Pts',(-0.133033896288026,1.80569443604825,
6.89688516202767));
#49676=CARTESIAN_POINT('Ctrl Pts',(-0.15217022967051,1.81511702769419,6.89569552689938));
#49677=CARTESIAN_POINT('Ctrl Pts',(-0.177466088700415,1.83085434710069,
6.89402990459643));
#49678=CARTESIAN_POINT('Ctrl Pts',(-0.184510869422828,1.83563409586334,
6.89355506812021));
#49679=CARTESIAN_POINT('Ctrl Pts',(-0.199152301628688,1.84643863259523,
6.89253001432184));
#49680=CARTESIAN_POINT('Ctrl Pts',(-0.206682798440024,1.85253846872658,
6.89197893038096));
#49681=CARTESIAN_POINT('Ctrl Pts',(-0.220306927764705,1.86463049405708,
6.89092121995001));
#49682=CARTESIAN_POINT('Ctrl Pts',(-0.226459214838741,1.87054379084444,
6.89041759134046));
#49683=CARTESIAN_POINT('Ctrl Pts',(-0.233524292252185,1.87789561282,6.88980282404033));
#49684=CARTESIAN_POINT('Ctrl Pts',(-0.234669875517236,1.87910635309918,
6.8897019350941));
#49685=CARTESIAN_POINT('Ctrl Pts',(-0.236652622161543,1.88123470401018,
6.88952516406352));
#49686=CARTESIAN_POINT('Ctrl Pts',(-0.23749397519268,1.88214837621656,6.88944946219417));
#49687=CARTESIAN_POINT('Ctrl Pts',(-0.238695527869264,1.88346844236531,
6.88934034107425));
#49688=CARTESIAN_POINT('Ctrl Pts',(-0.239060021999111,1.8838709266374,6.88930710375749));
#49689=CARTESIAN_POINT('Ctrl Pts',(-0.239690743247952,1.88457093366397,
6.88924935376238));
#49690=CARTESIAN_POINT('Ctrl Pts',(-0.239957438701744,1.88486803438226,
6.88922486087993));
#49691=CARTESIAN_POINT('Ctrl Pts',(-0.240469132796051,1.88544020068298,
6.88917772522342));
#49692=CARTESIAN_POINT('Ctrl Pts',(-0.240714213426203,1.88571519241089,
6.88915508594329));
#49693=CARTESIAN_POINT('Ctrl Pts',(-0.241290417501792,1.88636395576756,
6.88910170962166));
#49694=CARTESIAN_POINT('Ctrl Pts',(-0.241621144049332,1.8867380771978,6.88907095605185));
#49695=CARTESIAN_POINT('Ctrl Pts',(-0.242595339857808,1.88784527307461,
6.8889800203446));
#49696=CARTESIAN_POINT('Ctrl Pts',(-0.24323634765787,1.88858049706319,6.88891973597902));
#49697=CARTESIAN_POINT('Ctrl Pts',(-0.248896934846785,1.89513290339866,
6.8883833424007));
#49698=CARTESIAN_POINT('Ctrl Pts',(-0.253709947105928,1.90112451670273,
6.88789880889892));
#49699=CARTESIAN_POINT('Ctrl Pts',(-0.260527534124088,1.91026227071752,
6.8871675209828));
#49700=CARTESIAN_POINT('Ctrl Pts',(-0.262699276584188,1.91328071790586,
6.88692715164194));
#49701=CARTESIAN_POINT('Ctrl Pts',(-0.281289752809788,1.94008562529847,
6.88480315419676));
#49702=CARTESIAN_POINT('Ctrl Pts',(-0.294490548636968,1.9659424422099,6.88280943712105));
#49703=CARTESIAN_POINT('Ctrl Pts',(-0.307179345549023,2.00206989929026,
6.88026384908122));
#49704=CARTESIAN_POINT('Ctrl Pts',(-0.309904056222915,2.01106762273589,
6.87964961110476));
#49705=CARTESIAN_POINT('Ctrl Pts',(-0.312461565013822,2.02107087994329,
6.87899732298811));
#49706=CARTESIAN_POINT('Ctrl Pts',(-0.312687394113057,2.02197033118506,
6.87893894090026));
#49707=CARTESIAN_POINT('Ctrl Pts',(-0.313073645753839,2.02353733407688,
6.87883771157851));
#49708=CARTESIAN_POINT('Ctrl Pts',(-0.313235822130052,2.02420444141819,
6.87879476785278));
#49709=CARTESIAN_POINT('Ctrl Pts',(-0.313466119452912,2.02516512579215,
6.87873314904285));
#49710=CARTESIAN_POINT('Ctrl Pts',(-0.313535960878004,2.02545828227995,
6.87871437571435));
#49711=CARTESIAN_POINT('Ctrl Pts',(-0.313656541818026,2.02596758350624,
6.87868181318834));
#49712=CARTESIAN_POINT('Ctrl Pts',(-0.313707469283368,2.02618368314408,
6.87866801308739));
#49713=CARTESIAN_POINT('Ctrl Pts',(-0.313805570426962,2.02660188922292,
6.87864133836506));
#49714=CARTESIAN_POINT('Ctrl Pts',(-0.313852772069803,2.02680398807755,
6.87862846212074));
#49715=CARTESIAN_POINT('Ctrl Pts',(-0.31396498253148,2.02728653326359,6.878597751885));
#49716=CARTESIAN_POINT('Ctrl Pts',(-0.31402981099746,2.02756702196365,6.87857992834657));
#49717=CARTESIAN_POINT('Ctrl Pts',(-0.314259826703629,2.02856832770421,
6.87851639724098));
#49718=CARTESIAN_POINT('Ctrl Pts',(-0.314422910300101,2.02928963307569,
6.87847080995378));
#49719=CARTESIAN_POINT('Ctrl Pts',(-0.316881278798396,2.04033948004058,
6.87777508543917));
#49720=CARTESIAN_POINT('Ctrl Pts',(-0.318669321288063,2.05077562108578,
6.87715319211522));
#49721=CARTESIAN_POINT('Ctrl Pts',(-0.321483557307957,2.07403065497136,
6.87580740051804));
#49722=CARTESIAN_POINT('Ctrl Pts',(-0.322263057020988,2.08686078247903,
6.87509105270776));
#49723=CARTESIAN_POINT('Ctrl Pts',(-0.32229897683579,2.1259328765377,6.87290714437496));
#49724=CARTESIAN_POINT('Ctrl Pts',(-0.319121269284702,2.15206247705772,
6.87143427884424));
#49725=CARTESIAN_POINT('Ctrl Pts',(-0.312412576650348,2.17913492690807,
6.86974437954497));
#49726=CARTESIAN_POINT('Ctrl Pts',(-0.311999056071249,2.18074988268878,
6.86964297814424));
#49727=CARTESIAN_POINT('Ctrl Pts',(-0.311411575133442,2.18297231841413,
6.86950258942168));
#49728=CARTESIAN_POINT('Ctrl Pts',(-0.311248325083948,2.18358262303603,
6.86946394908589));
#49729=CARTESIAN_POINT('Ctrl Pts',(-0.310985212132392,2.18455480106472,
6.86940225547506));
#49730=CARTESIAN_POINT('Ctrl Pts',(-0.310886509077829,2.18491698899272,
6.86937923987444));
#49731=CARTESIAN_POINT('Ctrl Pts',(-0.310682617946147,2.1856600411719,6.86933195692072));
#49732=CARTESIAN_POINT('Ctrl Pts',(-0.310577361835775,2.18604088598107,
6.86930768738985));
#49733=CARTESIAN_POINT('Ctrl Pts',(-0.310332637111067,2.18692006533615,
6.86925157974321));
#49734=CARTESIAN_POINT('Ctrl Pts',(-0.310192668355467,2.18741825843543,
6.86921972540395));
#49735=CARTESIAN_POINT('Ctrl Pts',(-0.30975026040475,2.18897848726297,6.86911977358952));
#49736=CARTESIAN_POINT('Ctrl Pts',(-0.309443564630033,2.19003929851373,
6.86905153759129));
#49737=CARTESIAN_POINT('Ctrl Pts',(-0.304922044419433,2.20538251446122,
6.86806050901316));
#49738=CARTESIAN_POINT('Ctrl Pts',(-0.299728364704512,2.21935543494935,
6.86710530776711));
#49739=CARTESIAN_POINT('Ctrl Pts',(-0.286623742590941,2.24830088184217,
6.865010509881));
#49740=CARTESIAN_POINT('Ctrl Pts',(-0.278461422492394,2.26311184977095,
6.86386619262422));
#49741=CARTESIAN_POINT('Ctrl Pts',(-0.264277391184683,2.28465653957756,
6.86212181823417));
#49742=CARTESIAN_POINT('Ctrl Pts',(-0.259070742834407,2.29189304234128,
6.86152105719952));
#49743=CARTESIAN_POINT('Ctrl Pts',(-0.247524583768418,2.30661249131161,
6.86027935079376));
#49744=CARTESIAN_POINT('Ctrl Pts',(-0.241129453047439,2.31404151835647,
6.85964095243054));
#49745=CARTESIAN_POINT('Ctrl Pts',(-0.233905121393545,2.3216982194773,6.85898023644451));
#49746=CARTESIAN_POINT('Ctrl Pts',(-0.233403373055781,2.32222639763064,
6.85893464449148));
#49747=CARTESIAN_POINT('Ctrl Pts',(-0.232702142086055,2.32295957144292,
6.85887134358677));
#49748=CARTESIAN_POINT('Ctrl Pts',(-0.232504175859916,2.32316600466628,
6.85885351897409));
#49749=CARTESIAN_POINT('Ctrl Pts',(-0.232162429756917,2.32352141888784,
6.85882282828141));
#49750=CARTESIAN_POINT('Ctrl Pts',(-0.232018781097537,2.323670524904,6.85880995201896));
#49751=CARTESIAN_POINT('Ctrl Pts',(-0.231720573372341,2.32397946543423,
6.85878327182027));
#49752=CARTESIAN_POINT('Ctrl Pts',(-0.231565992828797,2.32413927818585,
6.85876946970545));
#49753=CARTESIAN_POINT('Ctrl Pts',(-0.231200200171516,2.32451666979619,
6.85873687470835));
#49754=CARTESIAN_POINT('Ctrl Pts',(-0.230988845431208,2.32473411148262,
6.85871809299356));
#49755=CARTESIAN_POINT('Ctrl Pts',(-0.230290663800027,2.32545037505574,
6.85865621896251));
#49756=CARTESIAN_POINT('Ctrl Pts',(-0.229802521242896,2.32594792032229,
6.85861322893988));
#49757=CARTESIAN_POINT('Ctrl Pts',(-0.228648662338361,2.32711639778117,
6.85851223275554));
#49758=CARTESIAN_POINT('Ctrl Pts',(-0.227981596976511,2.32778599698203,
6.85845432939142));
#49759=CARTESIAN_POINT('Ctrl Pts',(-0.220425463057356,2.3353043895243,6.85780373342245));
#49760=CARTESIAN_POINT('Ctrl Pts',(-0.213232313120236,2.34184201700761,
6.85723377035717));
#49761=CARTESIAN_POINT('Ctrl Pts',(-0.183443347434048,2.36655202265659,
6.85501013840131));
#49762=CARTESIAN_POINT('Ctrl Pts',(-0.15873783914129,2.38196439317632,6.85344755253178));
#49763=CARTESIAN_POINT('Ctrl Pts',(-0.130108501637404,2.39485376929827,
6.85162830829598));
#49764=CARTESIAN_POINT('Ctrl Pts',(-0.127903065425039,2.39581712753053,
6.85148821155526));
#49765=CARTESIAN_POINT('Ctrl Pts',(-0.123915760194919,2.39750589979528,
6.85123483952028));
#49766=CARTESIAN_POINT('Ctrl Pts',(-0.12213778270846,2.3982402351489,6.85112182866806));
#49767=CARTESIAN_POINT('Ctrl Pts',(-0.114141343490906,2.4014594044659,6.85061323526348));
#49768=CARTESIAN_POINT('Ctrl Pts',(-0.107853266991351,2.40376583374826,
6.85021236641828));
#49769=CARTESIAN_POINT('Ctrl Pts',(-0.100509445077585,2.4062027309649,6.8497414701628));
#49770=CARTESIAN_POINT('Ctrl Pts',(-0.0995190729652453,2.40652604306379,
6.84967791088624));
#49771=CARTESIAN_POINT('Ctrl Pts',(-0.0980460503357955,2.4069990276365,
6.84958328859491));
#49772=CARTESIAN_POINT('Ctrl Pts',(-0.09756458057457,2.40715237841976,6.84955234661465));
#49773=CARTESIAN_POINT('Ctrl Pts',(-0.0967075634716787,2.40742312471526,
6.84949724437207));
#49774=CARTESIAN_POINT('Ctrl Pts',(-0.0963321572107734,2.40754096625859,
6.8494730988111));
#49775=CARTESIAN_POINT('Ctrl Pts',(-0.0955426029602389,2.4077872230194,
6.84942229725377));
#49776=CARTESIAN_POINT('Ctrl Pts',(-0.0951284100125031,2.40791549041901,
6.84939563646569));
#49777=CARTESIAN_POINT('Ctrl Pts',(-0.0940389174119513,2.40825047672355,
6.84932547905196));
#49778=CARTESIAN_POINT('Ctrl Pts',(-0.0933631976591074,2.40845581158163,
6.84928193720288));
#49779=CARTESIAN_POINT('Ctrl Pts',(-0.0903512998932886,2.40936025070143,
6.84908772309549));
#49780=CARTESIAN_POINT('Ctrl Pts',(-0.0880079557402935,2.41003503238706,
6.84893625892184));
#49781=CARTESIAN_POINT('Ctrl Pts',(-0.0708900370722528,2.41475454659498,
6.84782696330667));
#49782=CARTESIAN_POINT('Ctrl Pts',(-0.0558535904380975,2.41776733076539,
6.84683565476908));
#49783=CARTESIAN_POINT('Ctrl Pts',(-0.0084360295732362,2.42379825147446,
6.84366292540376));
#49784=CARTESIAN_POINT('Ctrl Pts',(0.0242217874111559,2.42300106358828,
6.84139332157182));
#49785=CARTESIAN_POINT('Ctrl Pts',(0.0576635840449153,2.41707770709369,
6.83924570235275));
#49786=CARTESIAN_POINT('Ctrl Pts',(0.0591175564900687,2.41680984197825,
6.83915273031766));
#49787=CARTESIAN_POINT('Ctrl Pts',(0.0609862200646404,2.4164522656853,6.83903380395928));
#49788=CARTESIAN_POINT('Ctrl Pts',(0.0614026183801611,2.4163717338134,6.83900733935989));
#49789=CARTESIAN_POINT('Ctrl Pts',(0.0620624551829938,2.41624276890923,
6.83896546123088));
#49790=CARTESIAN_POINT('Ctrl Pts',(0.0623059969285247,2.41619487658477,
6.83895001689938));
#49791=CARTESIAN_POINT('Ctrl Pts',(0.0627424798570227,2.41610851863211,
6.83892236004706));
#49792=CARTESIAN_POINT('Ctrl Pts',(0.0629354397345218,2.41607015796517,
6.83891014160984));
#49793=CARTESIAN_POINT('Ctrl Pts',(0.0633892619933564,2.41597950546135,
6.83888142395937));
#49794=CARTESIAN_POINT('Ctrl Pts',(0.0636500944522861,2.41592706735115,
6.8388649332625));
#49795=CARTESIAN_POINT('Ctrl Pts',(0.0644067798867987,2.41577396715256,
6.83881713483455));
#49796=CARTESIAN_POINT('Ctrl Pts',(0.0649024639811346,2.4156724596858,6.83878587542501));
#49797=CARTESIAN_POINT('Ctrl Pts',(0.068345772989074,2.41495887674165,6.83856907837135));
#49798=CARTESIAN_POINT('Ctrl Pts',(0.0712850587277251,2.41430666665237,
6.83838579366968));
#49799=CARTESIAN_POINT('Ctrl Pts',(0.0804151148176153,2.412146088264,6.83782080679787));
#49800=CARTESIAN_POINT('Ctrl Pts',(0.0865708906523456,2.41049519025302,
6.83744611603596));
#49801=CARTESIAN_POINT('Ctrl Pts',(0.107791226756848,2.40412391628117,6.83616360107376));
#49802=CARTESIAN_POINT('Ctrl Pts',(0.122555507493681,2.39848034728892,6.83528671044205));
#49803=CARTESIAN_POINT('Ctrl Pts',(0.159571907990576,2.38111914319243,6.83300050531444));
#49804=CARTESIAN_POINT('Ctrl Pts',(0.180969608144942,2.367844939343,6.83158375222105));
#49805=CARTESIAN_POINT('Ctrl Pts',(0.201777977571167,2.35129475219088,6.82997103345412));
#49806=CARTESIAN_POINT('Ctrl Pts',(0.202939975357017,2.35035728668555,6.82988015308394));
#49807=CARTESIAN_POINT('Ctrl Pts',(0.20451556422199,2.34906797137611,6.82975578208097));
#49808=CARTESIAN_POINT('Ctrl Pts',(0.204934854792214,2.34872309032347,6.82972257337272));
#49809=CARTESIAN_POINT('Ctrl Pts',(0.205646093080466,2.34813505271073,6.82966605093025));
#49810=CARTESIAN_POINT('Ctrl Pts',(0.205938486916981,2.34789243551863,6.82964275914944));
#49811=CARTESIAN_POINT('Ctrl Pts',(0.206526704280569,2.3474025963376,6.82959579084211));
#49812=CARTESIAN_POINT('Ctrl Pts',(0.206822514587469,2.34715535946705,6.82957211372939));
#49813=CARTESIAN_POINT('Ctrl Pts',(0.207493628714051,2.34659239689058,6.82951826641001));
#49814=CARTESIAN_POINT('Ctrl Pts',(0.207868656210486,2.34627634462565,6.82948808285596));
#49815=CARTESIAN_POINT('Ctrl Pts',(0.208651132964943,2.345613856227,6.82942491089571));
#49816=CARTESIAN_POINT('Ctrl Pts',(0.209058443910769,2.34526725970321,6.82939191593651));
#49817=CARTESIAN_POINT('Ctrl Pts',(0.210123416734037,2.34435645319552,6.82930535228262));
#49818=CARTESIAN_POINT('Ctrl Pts',(0.210779665852636,2.34379060465451,6.82925171592332));
#49819=CARTESIAN_POINT('Ctrl Pts',(0.212720980003528,2.34210301523256,6.82909216584899));
#49820=CARTESIAN_POINT('Ctrl Pts',(0.213999414412069,2.34097372423042,6.82898593850427));
#49821=CARTESIAN_POINT('Ctrl Pts',(0.22793187112628,2.32846832941638,6.82781535843901));
#49822=CARTESIAN_POINT('Ctrl Pts',(0.239672819686541,2.3161191580839,6.82670883251865));
#49823=CARTESIAN_POINT('Ctrl Pts',(0.267889521755142,2.28129964699207,6.82371882625848));
#49824=CARTESIAN_POINT('Ctrl Pts',(0.282526080774365,2.2575225591566,6.82179283285765));
#49825=CARTESIAN_POINT('Ctrl Pts',(0.295558266089832,2.22853898313847,6.81974494487966));
#49826=CARTESIAN_POINT('Ctrl Pts',(0.297120437427373,2.22488557991926,6.81949206996655));
#49827=CARTESIAN_POINT('Ctrl Pts',(0.298837551465325,2.220655063975,6.81920601798216));
#49828=CARTESIAN_POINT('Ctrl Pts',(0.299058855293361,2.22010548577184,6.8191689875341));
#49829=CARTESIAN_POINT('Ctrl Pts',(0.299382760412788,2.21929466526526,6.81911454938806));
#49830=CARTESIAN_POINT('Ctrl Pts',(0.299486536384487,2.21903389819288,6.81909707121797));
#49831=CARTESIAN_POINT('Ctrl Pts',(0.299670905680956,2.21856884978255,6.81906595409309));
#49832=CARTESIAN_POINT('Ctrl Pts',(0.299751630875945,2.2183646215672,6.81905230713962));
#49833=CARTESIAN_POINT('Ctrl Pts',(0.299921294321935,2.21793410005134,6.81902357743977));
#49834=CARTESIAN_POINT('Ctrl Pts',(0.30001018501429,2.21770778917002,6.81900849761224));
#49835=CARTESIAN_POINT('Ctrl Pts',(0.300245173059328,2.21710752692598,6.81896855906664));
#49836=CARTESIAN_POINT('Ctrl Pts',(0.300390828484742,2.21673340128064,6.81894372707333));
#49837=CARTESIAN_POINT('Ctrl Pts',(0.301054724659993,2.21501866881518,6.81883018714444));
#49838=CARTESIAN_POINT('Ctrl Pts',(0.301564703095411,2.21367484965571,6.81874196955917));
#49839=CARTESIAN_POINT('Ctrl Pts',(0.305483327820432,2.2031370859973,6.81805581328721));
#49840=CARTESIAN_POINT('Ctrl Pts',(0.308480122244055,2.19379433520338,6.81748074788653));
#49841=CARTESIAN_POINT('Ctrl Pts',(0.319061978375157,2.15476307504405,6.81515837965903));
#49842=CARTESIAN_POINT('Ctrl Pts',(0.322821624500453,2.12420609338202,6.81351150595117));
#49843=CARTESIAN_POINT('Ctrl Pts',(0.322172002217396,2.09162150838969,6.81160982536418));
#49844=CARTESIAN_POINT('Ctrl Pts',(0.322115245046206,2.08966719658889,6.81149528676064));
#49845=CARTESIAN_POINT('Ctrl Pts',(0.322018291033916,2.08712593059078,6.81134565910995));
#49846=CARTESIAN_POINT('Ctrl Pts',(0.321994264107614,2.08653837679902,6.81131101653794));
#49847=CARTESIAN_POINT('Ctrl Pts',(0.321893102422582,2.08422001642839,6.81117413068363));
#49848=CARTESIAN_POINT('Ctrl Pts',(0.321803620214547,2.08248979946459,6.81107154488311));
#49849=CARTESIAN_POINT('Ctrl Pts',(0.321393227526319,2.07562772936836,6.81066288040297));
#49850=CARTESIAN_POINT('Ctrl Pts',(0.320963484599196,2.07050336874538,6.81035367325783));
#49851=CARTESIAN_POINT('Ctrl Pts',(0.320318493414498,2.06453189781462,6.80998792087809));
#49852=CARTESIAN_POINT('Ctrl Pts',(0.320222165529317,2.06367248732965,6.80993515068211));
#49853=CARTESIAN_POINT('Ctrl Pts',(0.320062742517292,2.06230008474536,6.80985066774492));
#49854=CARTESIAN_POINT('Ctrl Pts',(0.320001869904903,2.06178683459401,6.80981902510063));
#49855=CARTESIAN_POINT('Ctrl Pts',(0.319893131738617,2.06088848657177,6.80976355611619));
#49856=CARTESIAN_POINT('Ctrl Pts',(0.319845804671344,2.06050332357986,6.80973974681107));
#49857=CARTESIAN_POINT('Ctrl Pts',(0.319750186911184,2.05973659828906,6.80969229622416));
#49858=CARTESIAN_POINT('Ctrl Pts',(0.319701908613051,2.05935503506945,6.80966865537079));
#49859=CARTESIAN_POINT('Ctrl Pts',(0.319599651449307,2.05855830973338,6.80961923534234));
#49860=CARTESIAN_POINT('Ctrl Pts',(0.319545546428318,2.05814316478924,6.80959345221928));
#49861=CARTESIAN_POINT('Ctrl Pts',(0.31941341308455,2.05714450152621,6.80953135109108));
#49862=CARTESIAN_POINT('Ctrl Pts',(0.319334594700967,2.05656109085662,6.8094950081545));
#49863=CARTESIAN_POINT('Ctrl Pts',(0.319118104673788,2.05499107602903,6.80939703194188));
#49864=CARTESIAN_POINT('Ctrl Pts',(0.318977457243133,2.05400489479819,6.80933530467881));
#49865=CARTESIAN_POINT('Ctrl Pts',(0.318531696418294,2.05097975477293,6.80914537860551));
#49866=CARTESIAN_POINT('Ctrl Pts',(0.318211592553417,2.04894308948167,6.80901670702187));
#49867=CARTESIAN_POINT('Ctrl Pts',(0.316965477796275,2.04148212658251,6.8085423195098));
#49868=CARTESIAN_POINT('Ctrl Pts',(0.3159201674228,2.03607897456854,6.80819287481917));
#49869=CARTESIAN_POINT('Ctrl Pts',(0.313334566034227,2.02433512054876,6.80742009749783));
#49870=CARTESIAN_POINT('Ctrl Pts',(0.311739024109159,2.01800917022823,6.80699524967654));
#49871=CARTESIAN_POINT('Ctrl Pts',(0.305364395151487,1.99562359446648,6.80546207902814));
#49872=CARTESIAN_POINT('Ctrl Pts',(0.299526940903849,1.97989431047808,6.80432762766083));
#49873=CARTESIAN_POINT('Ctrl Pts',(0.284669060012023,1.94777630409352,6.80193392169563));
#49874=CARTESIAN_POINT('Ctrl Pts',(0.275390438610115,1.93156956110162,6.80067945065099));
#49875=CARTESIAN_POINT('Ctrl Pts',(0.264145249917297,1.91536622449466,6.7994369097627));
#49876=CARTESIAN_POINT('Ctrl Pts',(0.26352446078985,1.91448126036564,6.79936909254201));
#49877=CARTESIAN_POINT('Ctrl Pts',(0.262682575530885,1.91329386609797,6.79927817938233));
#49878=CARTESIAN_POINT('Ctrl Pts',(0.262465396915214,1.91298868657294,6.7992548203999));
#49879=CARTESIAN_POINT('Ctrl Pts',(0.262123621460219,1.91251019158715,6.79921820771644));
#49880=CARTESIAN_POINT('Ctrl Pts',(0.261999384522274,1.91233662132237,6.79920492927662));
#49881=CARTESIAN_POINT('Ctrl Pts',(0.26175991707467,1.91200276489418,6.79917939371607));
#49882=CARTESIAN_POINT('Ctrl Pts',(0.261644712601713,1.91184246238282,6.79916713499311));
#49883=CARTESIAN_POINT('Ctrl Pts',(0.261370387743824,1.91146148921364,6.79913800632488));
#49884=CARTESIAN_POINT('Ctrl Pts',(0.261211135329216,1.91124091433729,6.79912114567315));
#49885=CARTESIAN_POINT('Ctrl Pts',(0.260738077005979,1.91058744314044,6.79907120618498));
#49886=CARTESIAN_POINT('Ctrl Pts',(0.260423470946366,1.91015512309568,6.79903818257503));
#49887=CARTESIAN_POINT('Ctrl Pts',(0.257894764071611,1.9066983817606,6.79877423614928));
#49888=CARTESIAN_POINT('Ctrl Pts',(0.255629014007278,1.90371185691124,6.79854682997036));
#49889=CARTESIAN_POINT('Ctrl Pts',(0.246040120440922,1.89152031289622,6.79761804841922));
#49890=CARTESIAN_POINT('Ctrl Pts',(0.238267247308925,1.88267928084757,6.79694323285052));
#49891=CARTESIAN_POINT('Ctrl Pts',(0.22752539411124,1.87173231880931,6.79607665375847));
#49892=CARTESIAN_POINT('Ctrl Pts',(0.224980911478192,1.86922407116253,6.79587580155609));
#49893=CARTESIAN_POINT('Ctrl Pts',(0.207204920223891,1.85227469650503,6.79449852697421));
#49894=CARTESIAN_POINT('Ctrl Pts',(0.190637026185683,1.83931018601051,6.79333886599811));
#49895=CARTESIAN_POINT('Ctrl Pts',(0.172260752225997,1.82762520011724,6.79207606014041));
#49896=CARTESIAN_POINT('Ctrl Pts',(0.171593287026336,1.82720421153734,6.79203022820089));
#49897=CARTESIAN_POINT('Ctrl Pts',(0.16256510514686,1.82155613443301,6.79141073870724));
#49898=CARTESIAN_POINT('Ctrl Pts',(0.153971076620843,1.81671343587372,6.79082583959229));
#49899=CARTESIAN_POINT('Ctrl Pts',(0.144238471231809,1.81180297394246,6.79016297302303));
#49900=CARTESIAN_POINT('Ctrl Pts',(0.143305470210486,1.81133790588388,6.79009942632262));
#49901=CARTESIAN_POINT('Ctrl Pts',(0.141906994298655,1.81064926607465,6.79000416693733));
#49902=CARTESIAN_POINT('Ctrl Pts',(0.141443205558482,1.81042226976084,6.7899725737397));
#49903=CARTESIAN_POINT('Ctrl Pts',(0.140643664047032,1.81003332200704,6.78991810574866));
#49904=CARTESIAN_POINT('Ctrl Pts',(0.140308171142027,1.80987083619233,6.78989524959784));
#49905=CARTESIAN_POINT('Ctrl Pts',(0.139622471154554,1.80954020572264,6.78984853243412));
#49906=CARTESIAN_POINT('Ctrl Pts',(0.139272240515917,1.80937211151961,6.78982466971401));
#49907=CARTESIAN_POINT('Ctrl Pts',(0.138460753886303,1.80898443988319,6.78976937622959));
#49908=CARTESIAN_POINT('Ctrl Pts',(0.13799927896742,1.80876532555936,6.78973792947409));
#49909=CARTESIAN_POINT('Ctrl Pts',(0.137028056991712,1.80830700336677,6.78967174032411));
#49910=CARTESIAN_POINT('Ctrl Pts',(0.136518200538118,1.80806803257746,6.7896369898424));
#49911=CARTESIAN_POINT('Ctrl Pts',(0.135160752017659,1.80743612740108,6.78954445888791));
#49912=CARTESIAN_POINT('Ctrl Pts',(0.134312077867387,1.80704554254033,6.78948659752109));
#49913=CARTESIAN_POINT('Ctrl Pts',(0.131741608758437,1.80587605433886,6.78931130655577));
#49914=CARTESIAN_POINT('Ctrl Pts',(0.130014673004526,1.80510861075978,6.7891934851662));
#49915=CARTESIAN_POINT('Ctrl Pts',(0.123794281070761,1.80240955399807,6.78876884843833));
#49916=CARTESIAN_POINT('Ctrl Pts',(0.119263917830329,1.80056518024148,6.78845911112701));
#49917=CARTESIAN_POINT('Ctrl Pts',(0.103822662913714,1.79468484420899,6.78740141787451));
#49918=CARTESIAN_POINT('Ctrl Pts',(0.0927367257244031,1.79113701958502,
6.78663835755958));
#49919=CARTESIAN_POINT('Ctrl Pts',(0.0564731557588297,1.78166018872476,
6.78413870243388));
#49920=CARTESIAN_POINT('Ctrl Pts',(0.0307677559615217,1.77815724856511,
6.78235368600718));
#49921=CARTESIAN_POINT('Ctrl Pts',(-0.00104048037457064,1.77767154216208,
6.78027899071168));
#49922=CARTESIAN_POINT('Ctrl Pts',(-0.00700333927351832,1.77774593582544,
6.77989630499279));
#49923=CARTESIAN_POINT('Ctrl Pts',(-0.0135572761897419,1.77800973333096,
6.77948500394351));
#49924=CARTESIAN_POINT('Ctrl Pts',(-0.0141533403636898,1.77803538309729,
6.77944768216212));
#49925=CARTESIAN_POINT('Ctrl Pts',(-0.0150403895254106,1.77807602264171,
6.77939227074251));
#49926=CARTESIAN_POINT('Ctrl Pts',(-0.0153314267565426,1.77808975183987,
6.7793741113149));
#49927=CARTESIAN_POINT('Ctrl Pts',(-0.0158306651621511,1.77811398116298,
6.77934299726925));
#49928=CARTESIAN_POINT('Ctrl Pts',(-0.0160388748045849,1.77812428861782,
6.77933003182086));
#49929=CARTESIAN_POINT('Ctrl Pts',(-0.0164682598830051,1.77814596306891,
6.77930331602088));
#49930=CARTESIAN_POINT('Ctrl Pts',(-0.0166894331312736,1.77815735600392,
6.77928956724223));
#49931=CARTESIAN_POINT('Ctrl Pts',(-0.0172082157112406,1.77818461540867,
6.779257346841));
#49932=CARTESIAN_POINT('Ctrl Pts',(-0.0175058159926783,1.77820066678786,
6.77923888567066));
#49933=CARTESIAN_POINT('Ctrl Pts',(-0.0184705385395573,1.77825404233466,
6.77917911103764));
#49934=CARTESIAN_POINT('Ctrl Pts',(-0.0191375726896217,1.77829302867626,
6.77913789050687));
#49935=CARTESIAN_POINT('Ctrl Pts',(-0.0206991607475864,1.77838917331149,
6.77904163515628));
#49936=CARTESIAN_POINT('Ctrl Pts',(-0.0215936121264193,1.77844799012012,
6.77898669057593));
#49937=CARTESIAN_POINT('Ctrl Pts',(-0.031322465876583,1.77912851226527,
6.77839100680657));
#49938=CARTESIAN_POINT('Ctrl Pts',(-0.0401287939413119,1.78011045691583,
6.7778692134471));
#49939=CARTESIAN_POINT('Ctrl Pts',(-0.0576488989979258,1.78279910574574,
6.77684634475258));
#49940=CARTESIAN_POINT('Ctrl Pts',(-0.0663546813269928,1.78450535033996,
6.77634571202855));
#49941=CARTESIAN_POINT('Ctrl Pts',(-0.0777661773666632,1.78723521934586,
6.7756875040365));
#49942=CARTESIAN_POINT('Ctrl Pts',(-0.0805439835741911,1.787939023216,6.77552713176508));
#49943=CARTESIAN_POINT('Ctrl Pts',(-0.0927683553202072,1.79121037332254,
6.77481945176136));
#49944=CARTESIAN_POINT('Ctrl Pts',(-0.102104358231319,1.79417047730929,
6.77427370759598));
#49945=CARTESIAN_POINT('Ctrl Pts',(-0.129126432464411,1.80411368146494,
6.77264892522838));
#49946=CARTESIAN_POINT('Ctrl Pts',(-0.146343650576667,1.81224016443036,
6.77155238611826));
#49947=CARTESIAN_POINT('Ctrl Pts',(-0.163857420050215,1.82248677966368,
6.77031991618886));
#49948=CARTESIAN_POINT('Ctrl Pts',(-0.164967534365567,1.8231452472928,6.77024127968918));
#49949=CARTESIAN_POINT('Ctrl Pts',(-0.166510958814107,1.82407331299188,
6.77013121538963));
#49950=CARTESIAN_POINT('Ctrl Pts',(-0.166947639720453,1.82433730467197,
6.77009999243773));
#49951=CARTESIAN_POINT('Ctrl Pts',(-0.167700871900095,1.82479511094921,
6.77004599243645));
#49952=CARTESIAN_POINT('Ctrl Pts',(-0.168017719628093,1.82498843791103,
6.77002323329284));
#49953=CARTESIAN_POINT('Ctrl Pts',(-0.168666242689812,1.82538567810225,
6.76997655935361));
#49954=CARTESIAN_POINT('Ctrl Pts',(-0.168997883813226,1.82558964582392,
6.76995264257946));
#49955=CARTESIAN_POINT('Ctrl Pts',(-0.169768424540372,1.82606547461862,
6.76989696010574));
#49956=CARTESIAN_POINT('Ctrl Pts',(-0.170207041186248,1.82633778979823,
6.76986517770135));
#49957=CARTESIAN_POINT('Ctrl Pts',(-0.171129068123141,1.82691330445432,
6.7697981846339));
#49958=CARTESIAN_POINT('Ctrl Pts',(-0.171612330832229,1.82721673595988,
6.76976296545157));
#49959=CARTESIAN_POINT('Ctrl Pts',(-0.172900036528971,1.82803003825541,
6.7696688352144));
#49960=CARTESIAN_POINT('Ctrl Pts',(-0.173703024868347,1.82854219141202,
6.76960983952191));
#49961=CARTESIAN_POINT('Ctrl Pts',(-0.176134603562278,1.83010828071922,
6.76943027710532));
#49962=CARTESIAN_POINT('Ctrl Pts',(-0.17775593615286,1.83117335398858,6.76930929578685));
#49963=CARTESIAN_POINT('Ctrl Pts',(-0.204482774166398,1.84907804195431,
6.76729383632073));
#49964=CARTESIAN_POINT('Ctrl Pts',(-0.227100796113425,1.86934998064091,
6.76525511184102));
#49965=CARTESIAN_POINT('Ctrl Pts',(-0.256122004173941,1.90382857844438,
6.76220928080569));
#49966=CARTESIAN_POINT('Ctrl Pts',(-0.264889324021546,1.91583854269372,
6.76121240058435));
#49967=CARTESIAN_POINT('Ctrl Pts',(-0.274577314951453,1.93124086312546,
6.76004482899131));
#49968=CARTESIAN_POINT('Ctrl Pts',(-0.276312938994576,1.93409789007875,
6.75983267062555));
#49969=CARTESIAN_POINT('Ctrl Pts',(-0.278284942628973,1.93746085066125,
6.75958851315101));
#49970=CARTESIAN_POINT('Ctrl Pts',(-0.278564768508545,1.93794089313306,
6.75955379192174));
#49971=CARTESIAN_POINT('Ctrl Pts',(-0.278983829012849,1.9386640855941,6.75950168304108));
#49972=CARTESIAN_POINT('Ctrl Pts',(-0.279123988519422,1.938906694235,6.75948423575871));
#49973=CARTESIAN_POINT('Ctrl Pts',(-0.279373125432313,1.93933923826284,
6.75945318950914));
#49974=CARTESIAN_POINT('Ctrl Pts',(-0.279482225574177,1.93952910181294,
6.75943958255324));
#49975=CARTESIAN_POINT('Ctrl Pts',(-0.279713497114305,1.93993252769301,
6.75941071421316));
#49976=CARTESIAN_POINT('Ctrl Pts',(-0.279835617139131,1.94014611815788,
6.75939545619856));
#49977=CARTESIAN_POINT('Ctrl Pts',(-0.280162768393026,1.94071983626291,
6.75935454156856));
#49978=CARTESIAN_POINT('Ctrl Pts',(-0.280367350679459,1.94108022139677,
6.75932891405313));
#49979=CARTESIAN_POINT('Ctrl Pts',(-0.281345051647101,1.94281026999613,
6.75920623397734));
#49980=CARTESIAN_POINT('Ctrl Pts',(-0.282108849152745,1.94418521645598,
6.75910977350736));
#49981=CARTESIAN_POINT('Ctrl Pts',(-0.288377918613924,1.9556676750672,6.75831235244484));
#49982=CARTESIAN_POINT('Ctrl Pts',(-0.293348821378168,1.96605906077359,
6.75764279027653));
#49983=CARTESIAN_POINT('Ctrl Pts',(-0.311735391401225,2.01045854564617,
6.75490404792567));
#49984=CARTESIAN_POINT('Ctrl Pts',(-0.319872695744452,2.04635092979291,
6.75294300284295));
#49985=CARTESIAN_POINT('Ctrl Pts',(-0.321932128880303,2.08498432471426,
6.75060575887161));
#49986=CARTESIAN_POINT('Ctrl Pts',(-0.322024838845627,2.08712487153331,
6.75047567308695));
#49987=CARTESIAN_POINT('Ctrl Pts',(-0.322119515216439,2.08996587295851,
6.7503021900407));
#49988=CARTESIAN_POINT('Ctrl Pts',(-0.322140553303645,2.0906656712187,6.75025939087309));
#49989=CARTESIAN_POINT('Ctrl Pts',(-0.322169733260274,2.09175439961882,
6.75019269949785));
#49990=CARTESIAN_POINT('Ctrl Pts',(-0.322179451600182,2.09214328827607,
6.75016885671481));
#49991=CARTESIAN_POINT('Ctrl Pts',(-0.32219744674238,2.09291966434493,6.7501212148784));
#49992=CARTESIAN_POINT('Ctrl Pts',(-0.322205728705603,2.09330715101484,
6.75009741602585));
#49993=CARTESIAN_POINT('Ctrl Pts',(-0.322220666759002,2.09407050910491,
6.7500504900366));
#49994=CARTESIAN_POINT('Ctrl Pts',(-0.322227364204921,2.09444637915127,
6.7500273642363));
#49995=CARTESIAN_POINT('Ctrl Pts',(-0.322240973981441,2.09529337486586,
6.74997520672424));
#49996=CARTESIAN_POINT('Ctrl Pts',(-0.322247510790505,2.09576450496247,
6.74994616328499));
#49997=CARTESIAN_POINT('Ctrl Pts',(-0.32226789559115,2.09750957541692,6.74983846825088));
#49998=CARTESIAN_POINT('Ctrl Pts',(-0.322275222346017,2.09878356433945,
6.74975961279031));
#49999=CARTESIAN_POINT('Ctrl Pts',(-0.322274994862272,2.1000575458305,6.74968051971722));
#50000=CARTESIAN_POINT('',(-0.322274936831736,2.09979822016873,6.49915140185063));
#50001=CARTESIAN_POINT('Ctrl Pts',(-0.322274994880076,2.10005744603766,
6.7496805259127));
#50002=CARTESIAN_POINT('Ctrl Pts',(-0.322274683587777,2.10180381058933,
6.74957210572105));
#50003=CARTESIAN_POINT('Ctrl Pts',(-0.32226017734277,2.10355012243384,6.74946324132778));
#50004=CARTESIAN_POINT('Ctrl Pts',(-0.321619076867645,2.14255589360676,
6.74702138683848));
#50005=CARTESIAN_POINT('Ctrl Pts',(-0.314547986542146,2.17942209619581,
6.74445563806546));
#50006=CARTESIAN_POINT('Ctrl Pts',(-0.297384809473874,2.22469255122695,
6.74122753131725));
#50007=CARTESIAN_POINT('Ctrl Pts',(-0.292883902559978,2.23492604703357,
6.74049609629811));
#50008=CARTESIAN_POINT('Ctrl Pts',(-0.287540268053849,2.24554131882432,
6.73975045817491));
#50009=CARTESIAN_POINT('Ctrl Pts',(-0.287218443693046,2.24617539759807,
6.73970597109837));
#50010=CARTESIAN_POINT('Ctrl Pts',(-0.286755253236832,2.24708056917944,
6.73964254404661));
#50011=CARTESIAN_POINT('Ctrl Pts',(-0.286615598852468,2.24735252826254,
6.73962349772094));
#50012=CARTESIAN_POINT('Ctrl Pts',(-0.28637351084408,2.24782231746359,6.73959061505136));
#50013=CARTESIAN_POINT('Ctrl Pts',(-0.286271258863422,2.24802024051934,
6.7395767671977));
#50014=CARTESIAN_POINT('Ctrl Pts',(-0.286073865934775,2.24840135263357,
6.73955011351327));
#50015=CARTESIAN_POINT('Ctrl Pts',(-0.285978754418912,2.2485845559133,6.73953730584442));
#50016=CARTESIAN_POINT('Ctrl Pts',(-0.285752536085183,2.24901927457349,
6.73950692628023));
#50017=CARTESIAN_POINT('Ctrl Pts',(-0.285621272855375,2.24927070900693,
6.73948936432509));
#50018=CARTESIAN_POINT('Ctrl Pts',(-0.285227222460133,2.25002308887097,
6.73943683911131));
#50019=CARTESIAN_POINT('Ctrl Pts',(-0.284963446344544,2.25052351937679,
6.73940193797667));
#50020=CARTESIAN_POINT('Ctrl Pts',(-0.282410092139383,2.25533692193904,
6.739066552762));
#50021=CARTESIAN_POINT('Ctrl Pts',(-0.280023936749332,2.25959831015863,
6.73877204756151));
#50022=CARTESIAN_POINT('Ctrl Pts',(-0.277142026443082,2.26448127893417,
6.73843548548519));
#50023=CARTESIAN_POINT('Ctrl Pts',(-0.276739874174369,2.26515700410437,
6.73838893106606));
#50024=CARTESIAN_POINT('Ctrl Pts',(-0.275946688624445,2.26647874001302,
6.73829789596583));
#50025=CARTESIAN_POINT('Ctrl Pts',(-0.275555850389802,2.26712486102769,
6.73825340663306));
#50026=CARTESIAN_POINT('Ctrl Pts',(-0.274970328856967,2.26808518818476,
6.73818729190111));
#50027=CARTESIAN_POINT('Ctrl Pts',(-0.274777372553752,2.26840043875641,
6.73816558969062));
#50028=CARTESIAN_POINT('Ctrl Pts',(-0.273824553752443,2.26995114925842,
6.73805884111184));
#50029=CARTESIAN_POINT('Ctrl Pts',(-0.273056889174893,2.27118181785375,
6.73797413656782));
#50030=CARTESIAN_POINT('Ctrl Pts',(-0.261082301664139,2.29009315307375,
6.73667204301447));
#50031=CARTESIAN_POINT('Ctrl Pts',(-0.248186346764666,2.30664716869184,
6.73552313425646));
#50032=CARTESIAN_POINT('Ctrl Pts',(-0.219273126019941,2.3371166885887,6.73316315955346));
#50033=CARTESIAN_POINT('Ctrl Pts',(-0.203310226533078,2.35093780220172,
6.73195629172405));
#50034=CARTESIAN_POINT('Ctrl Pts',(-0.185340867568427,2.36364907846595,
6.73062005994007));
#50035=CARTESIAN_POINT('Ctrl Pts',(-0.184564768947334,2.36419295940752,
6.73056239791093));
#50036=CARTESIAN_POINT('Ctrl Pts',(-0.183319151871102,2.36505770611472,
6.73046992651676));
#50037=CARTESIAN_POINT('Ctrl Pts',(-0.182851159502597,2.36538076885031,
6.73043520071061));
#50038=CARTESIAN_POINT('Ctrl Pts',(-0.181957771642656,2.36599400392637,
6.7303689404597));
#50039=CARTESIAN_POINT('Ctrl Pts',(-0.181532530558714,2.36628439896102,
6.73033741458115));
#50040=CARTESIAN_POINT('Ctrl Pts',(-0.180784710427824,2.36679245779261,
6.73028199606463));
#50041=CARTESIAN_POINT('Ctrl Pts',(-0.180462428895546,2.36701055936885,
6.73025812005145));
#50042=CARTESIAN_POINT('Ctrl Pts',(-0.179831632944389,2.36743578200776,
6.73021140168496));
#50043=CARTESIAN_POINT('Ctrl Pts',(-0.179523153650696,2.36764295433853,
6.73018856131456));
#50044=CARTESIAN_POINT('Ctrl Pts',(-0.178788879918758,2.368134246354,6.73013420916219));
#50045=CARTESIAN_POINT('Ctrl Pts',(-0.178362766481501,2.36841788535541,
6.73010267935393));
#50046=CARTESIAN_POINT('Ctrl Pts',(-0.176851890242351,2.36941840168938,
6.72999092402845));
#50047=CARTESIAN_POINT('Ctrl Pts',(-0.175763477759199,2.37012972079664,
6.72991049053158));
#50048=CARTESIAN_POINT('Ctrl Pts',(-0.156532484412484,2.38253247589564,
6.72849050645493));
#50049=CARTESIAN_POINT('Ctrl Pts',(-0.137268674712566,2.39237646035813,
6.72708081041956));
#50050=CARTESIAN_POINT('Ctrl Pts',(-0.114781937834227,2.40115253818674,
6.72545975906167));
#50051=CARTESIAN_POINT('Ctrl Pts',(-0.112383339659688,2.40205583792874,
6.72528722165743));
#50052=CARTESIAN_POINT('Ctrl Pts',(-0.0939417376466633,2.40875077877548,
6.72396414575715));
#50053=CARTESIAN_POINT('Ctrl Pts',(-0.0774722289411833,2.41328928236835,
6.72280076151746));
#50054=CARTESIAN_POINT('Ctrl Pts',(-0.0544847525141653,2.41769939331023,
6.7212520867488));
#50055=CARTESIAN_POINT('Ctrl Pts',(-0.0482144467502013,2.41871126620656,
6.72083733263755));
#50056=CARTESIAN_POINT('Ctrl Pts',(-0.0389616864876357,2.41992507303045,
6.72024031619092));
#50057=CARTESIAN_POINT('Ctrl Pts',(-0.0360000767159645,2.42027185546765,
6.7200514709824));
#50058=CARTESIAN_POINT('Ctrl Pts',(-0.0325319478012861,2.42062922930276,
6.71983328394203));
#50059=CARTESIAN_POINT('Ctrl Pts',(-0.0320298168376149,2.42067977976887,
6.71980176619068));
#50060=CARTESIAN_POINT('Ctrl Pts',(-0.0312630656450533,2.42075515114722,
6.71975375129936));
#50061=CARTESIAN_POINT('Ctrl Pts',(-0.0309985329217474,2.42078082426936,
6.71973720637868));
#50062=CARTESIAN_POINT('Ctrl Pts',(-0.0305381546025398,2.42082492956925,
6.71970844842392));
#50063=CARTESIAN_POINT('Ctrl Pts',(-0.0303423244299566,2.42084350962504,
6.71969622703716));
#50064=CARTESIAN_POINT('Ctrl Pts',(-0.0298991573435592,2.42088514724345,
6.71966859549216));
#50065=CARTESIAN_POINT('Ctrl Pts',(-0.0296518112256919,2.4209080980956,
6.71965319145988));
#50066=CARTESIAN_POINT('Ctrl Pts',(-0.028981191449886,2.4209695418703,6.71961147542123));
#50067=CARTESIAN_POINT('Ctrl Pts',(-0.0285578659038651,2.42100748366077,
6.71958519452755));
#50068=CARTESIAN_POINT('Ctrl Pts',(-0.0266534817364965,2.42117437271335,
6.71946719615054));
#50069=CARTESIAN_POINT('Ctrl Pts',(-0.0251715860297762,2.42129391098022,
6.71937600016424));
#50070=CARTESIAN_POINT('Ctrl Pts',(0.00853843822551648,2.42377849369015,
6.71731459576104));
#50071=CARTESIAN_POINT('Ctrl Pts',(0.0409458027228496,2.42129378125581,
6.71559116419884));
#50072=CARTESIAN_POINT('Ctrl Pts',(0.0887280113091252,2.41027040967293,
6.71280947680115));
#50073=CARTESIAN_POINT('Ctrl Pts',(0.104690886584727,2.40525413371082,6.71183939542702));
#50074=CARTESIAN_POINT('Ctrl Pts',(0.121113537403473,2.39865309957655,6.71076540163711));
#50075=CARTESIAN_POINT('Ctrl Pts',(0.122033707666776,2.39827828782492,6.71070497083213));
#50076=CARTESIAN_POINT('Ctrl Pts',(0.123495322589924,2.39767503465,6.71060857005303));
#50077=CARTESIAN_POINT('Ctrl Pts',(0.124037906079948,2.39744935502298,6.71057269337264));
#50078=CARTESIAN_POINT('Ctrl Pts',(0.125067376440773,2.39701785534778,6.71050444913373));
#50079=CARTESIAN_POINT('Ctrl Pts',(0.125554380616749,2.3968123187266,6.71047209126576));
#50080=CARTESIAN_POINT('Ctrl Pts',(0.126401210108036,2.39645246329958,6.7104156957374));
#50081=CARTESIAN_POINT('Ctrl Pts',(0.126761264982699,2.39629868479452,6.71039167651049));
#50082=CARTESIAN_POINT('Ctrl Pts',(0.127459206657714,2.39599909069644,6.7103450369494));
#50083=CARTESIAN_POINT('Ctrl Pts',(0.127797125848452,2.39585335164243,6.71032241925458));
#50084=CARTESIAN_POINT('Ctrl Pts',(0.128591719167727,2.39550904109501,6.71026914916756));
#50085=CARTESIAN_POINT('Ctrl Pts',(0.129048183165817,2.39530998971346,6.71023848040879));
#50086=CARTESIAN_POINT('Ctrl Pts',(0.130620761706771,2.39461988914456,6.71013258962299));
#50087=CARTESIAN_POINT('Ctrl Pts',(0.131734539042031,2.39412356863438,6.71005718722562));
#50088=CARTESIAN_POINT('Ctrl Pts',(0.145084998032035,2.38808330513215,6.70914842351874));
#50089=CARTESIAN_POINT('Ctrl Pts',(0.156964640335449,2.38178655763873,6.7082888756615));
#50090=CARTESIAN_POINT('Ctrl Pts',(0.185469585128621,2.36431479954132,6.70609391199285));
#50091=CARTESIAN_POINT('Ctrl Pts',(0.201512117558669,2.35229745704333,6.70473402588221));
#50092=CARTESIAN_POINT('Ctrl Pts',(0.219593507946827,2.33592199226662,6.70308718197745));
#50093=CARTESIAN_POINT('Ctrl Pts',(0.222790770202542,2.33290506507437,6.70279126565455));
#50094=CARTESIAN_POINT('Ctrl Pts',(0.234061645222341,2.32182536589768,6.70173336434311));
#50095=CARTESIAN_POINT('Ctrl Pts',(0.241768421741876,2.31339971067415,6.70098159539294));
#50096=CARTESIAN_POINT('Ctrl Pts',(0.249668431686356,2.30378399526349,6.70019425095516));
#50097=CARTESIAN_POINT('Ctrl Pts',(0.250320292091769,2.3029827429618,6.70012915236932));
#50098=CARTESIAN_POINT('Ctrl Pts',(0.251437547999195,2.30159586942359,6.70001736870282));
#50099=CARTESIAN_POINT('Ctrl Pts',(0.251904773128048,2.3010117419812,6.69997055827822));
#50100=CARTESIAN_POINT('Ctrl Pts',(0.252564061745699,2.30018158692492,6.69990442126327));
#50101=CARTESIAN_POINT('Ctrl Pts',(0.252757803520423,2.29993690452432,6.69988497554123));
#50102=CARTESIAN_POINT('Ctrl Pts',(0.253089949152957,2.29951617330578,6.69985162104213));
#50103=CARTESIAN_POINT('Ctrl Pts',(0.253228525252826,2.29934026129268,6.69983769986165));
#50104=CARTESIAN_POINT('Ctrl Pts',(0.253493584458275,2.29900306598931,6.6998110626201));
#50105=CARTESIAN_POINT('Ctrl Pts',(0.253620096873674,2.29884180671335,6.6997983444196));
#50106=CARTESIAN_POINT('Ctrl Pts',(0.253917826415134,2.29846155880798,6.69976840349856));
#50107=CARTESIAN_POINT('Ctrl Pts',(0.254088914547036,2.29824246871329,6.69975119004522));
#50108=CARTESIAN_POINT('Ctrl Pts',(0.254593660243662,2.29759438037056,6.69970038181837));
#50109=CARTESIAN_POINT('Ctrl Pts',(0.254926518462334,2.29716475644778,6.6996668436417));
#50110=CARTESIAN_POINT('Ctrl Pts',(0.257843096552387,2.29338056232744,6.6993726692429));
#50111=CARTESIAN_POINT('Ctrl Pts',(0.26036170831508,2.28997602312923,6.69911651878526));
#50112=CARTESIAN_POINT('Ctrl Pts',(0.263477862549883,2.28558532447237,6.69879544708528));
#50113=CARTESIAN_POINT('Ctrl Pts',(0.264138080915469,2.28464444479839,6.69872717473694));
#50114=CARTESIAN_POINT('Ctrl Pts',(0.265510483958018,2.28266620312225,6.6985846895177));
#50115=CARTESIAN_POINT('Ctrl Pts',(0.266221656538199,2.28162816006969,6.69851052763677));
#50116=CARTESIAN_POINT('Ctrl Pts',(0.267308511790982,2.28002166351271,6.69839663762457));
#50117=CARTESIAN_POINT('Ctrl Pts',(0.267688494904383,2.27945614929111,6.69835671393887));
#50118=CARTESIAN_POINT('Ctrl Pts',(0.268545856470267,2.27817138880126,6.69826638243771));
#50119=CARTESIAN_POINT('Ctrl Pts',(0.26902214551959,2.27745141887039,6.69821602203589));
#50120=CARTESIAN_POINT('Ctrl Pts',(0.281902741157039,2.25780974995223,6.69684895660928));
#50121=CARTESIAN_POINT('Ctrl Pts',(0.29228400663753,2.23763466477447,6.6956127065966));
#50122=CARTESIAN_POINT('Ctrl Pts',(0.307582521662921,2.19819060504509,6.69322840279192));
#50123=CARTESIAN_POINT('Ctrl Pts',(0.313001933961916,2.17923393432893,6.69209495183434));
#50124=CARTESIAN_POINT('Ctrl Pts',(0.3168181236952,2.15906087500548,6.6908473451199));
#50125=CARTESIAN_POINT('Ctrl Pts',(0.316974098547536,2.158217963602,6.69079514824213));
#50126=CARTESIAN_POINT('Ctrl Pts',(0.317221227853585,2.15685200177996,6.6907104497536));
#50127=CARTESIAN_POINT('Ctrl Pts',(0.317314456682427,2.15632932701864,6.690678014028));
#50128=CARTESIAN_POINT('Ctrl Pts',(0.317490834435083,2.1553261553484,6.6906157081945));
#50129=CARTESIAN_POINT('Ctrl Pts',(0.317574185263021,2.15484569505729,6.69058584458403));
#50130=CARTESIAN_POINT('Ctrl Pts',(0.317721372180488,2.15398567794411,6.69053234771643));
#50131=CARTESIAN_POINT('Ctrl Pts',(0.317785619522712,2.1536061916743,6.69050872757399));
#50132=CARTESIAN_POINT('Ctrl Pts',(0.317912120046597,2.15285077813563,6.69046167976442));
#50133=CARTESIAN_POINT('Ctrl Pts',(0.317974386626068,2.15247485369105,6.69043825256271));
#50134=CARTESIAN_POINT('Ctrl Pts',(0.318124398872332,2.15155910758006,6.69038114903178));
#50135=CARTESIAN_POINT('Ctrl Pts',(0.318211437165747,2.15101917270357,6.69034745031074));
#50136=CARTESIAN_POINT('Ctrl Pts',(0.31853500360557,2.14897891406945,6.69021999823612));
#50137=CARTESIAN_POINT('Ctrl Pts',(0.318762295857689,2.14747716459709,6.69012595264792));
#50138=CARTESIAN_POINT('Ctrl Pts',(0.322629609821283,2.12064471846475,6.68844127334209));
#50139=CARTESIAN_POINT('Ctrl Pts',(0.323249581840282,2.09497651837931,6.68674972250763));
#50140=CARTESIAN_POINT('Ctrl Pts',(0.319370138550048,2.0541539967077,6.68397895336181));
#50141=CARTESIAN_POINT('Ctrl Pts',(0.316809963252761,2.03892119311113,6.68292946436056));
#50142=CARTESIAN_POINT('Ctrl Pts',(0.311341951084789,2.01641024425161,6.68139743627792));
#50143=CARTESIAN_POINT('Ctrl Pts',(0.309244962437868,2.00895807270674,6.68089372185862));
#50144=CARTESIAN_POINT('Ctrl Pts',(0.306383513590788,2.0000351176264,6.68030053879013));
#50145=CARTESIAN_POINT('Ctrl Pts',(0.305873731840747,1.99848598350857,6.68019792569656));
#50146=CARTESIAN_POINT('Ctrl Pts',(0.305218015435695,1.99654317447165,6.68006976237897));
#50147=CARTESIAN_POINT('Ctrl Pts',(0.305083053505842,1.99614586111659,6.68004358018279));
#50148=CARTESIAN_POINT('Ctrl Pts',(0.30486734968666,1.9955149014087,6.68000204661094));
#50149=CARTESIAN_POINT('Ctrl Pts',(0.304787114877964,1.99528108414447,6.67998666528726));
#50150=CARTESIAN_POINT('Ctrl Pts',(0.304635365116556,1.99484051252263,6.67995770198681));
#50151=CARTESIAN_POINT('Ctrl Pts',(0.304563909243897,1.99463374035012,6.67994411668606));
#50152=CARTESIAN_POINT('Ctrl Pts',(0.304401086219191,1.99416412817387,6.67991328023284));
#50153=CARTESIAN_POINT('Ctrl Pts',(0.304309589334357,1.99390133414047,6.67989603693768));
#50154=CARTESIAN_POINT('Ctrl Pts',(0.304031240038526,1.99310519152697,6.67984383548219));
#50155=CARTESIAN_POINT('Ctrl Pts',(0.303843323739952,1.99257221203078,6.67980894033994));
#50156=CARTESIAN_POINT('Ctrl Pts',(0.302518036455546,1.98884464843654,6.67956523079434));
#50157=CARTESIAN_POINT('Ctrl Pts',(0.301331655613393,1.98566754571356,6.67935926515628));
#50158=CARTESIAN_POINT('Ctrl Pts',(0.296482616776541,1.97328207549909,6.67856106051052));
#50159=CARTESIAN_POINT('Ctrl Pts',(0.292445915489521,1.96422519738477,6.67798764672803));
#50160=CARTESIAN_POINT('Ctrl Pts',(0.278777642612646,1.93700830394182,6.67625495843062));
#50161=CARTESIAN_POINT('Ctrl Pts',(0.267822884818316,1.91957213052554,6.67512851917487));
#50162=CARTESIAN_POINT('Ctrl Pts',(0.245149353689464,1.89014625266057,6.67301937148484));
#50163=CARTESIAN_POINT('Ctrl Pts',(0.234016658136712,1.87779989626547,6.67205428344464));
#50164=CARTESIAN_POINT('Ctrl Pts',(0.221332805272072,1.86574848780848,6.67099155635364));
#50165=CARTESIAN_POINT('Ctrl Pts',(0.220679376069303,1.86513281496587,6.67093690838455));
#50166=CARTESIAN_POINT('Ctrl Pts',(0.219623048756993,1.86414582413511,6.67084872126541));
#50167=CARTESIAN_POINT('Ctrl Pts',(0.21922175830618,1.86377278628926,6.67081525567561));
#50168=CARTESIAN_POINT('Ctrl Pts',(0.218452498066158,1.86306133359068,6.67075117085958));
#50169=CARTESIAN_POINT('Ctrl Pts',(0.218084687976577,1.86272274778884,6.67072055903436));
#50170=CARTESIAN_POINT('Ctrl Pts',(0.217430900771802,1.86212371149742,6.67066619733387));
#50171=CARTESIAN_POINT('Ctrl Pts',(0.217145239140507,1.86186291687623,6.67064246212712));
#50172=CARTESIAN_POINT('Ctrl Pts',(0.216580697541484,1.86134937936236,6.67059558880442));
#50173=CARTESIAN_POINT('Ctrl Pts',(0.216301842895133,1.86109660940751,6.67057245188582));
#50174=CARTESIAN_POINT('Ctrl Pts',(0.2156293854293,1.8604891976153,6.67051669556292));
#50175=CARTESIAN_POINT('Ctrl Pts',(0.215235350598025,1.86013503764165,6.67048405593303));
#50176=CARTESIAN_POINT('Ctrl Pts',(0.21379002602807,1.8588424035141,6.67036444674036));
#50177=CARTESIAN_POINT('Ctrl Pts',(0.212733468911141,1.85790986662868,6.67027722895001));
#50178=CARTESIAN_POINT('Ctrl Pts',(0.195215194089538,1.84265114872117,6.66883457321651));
#50179=CARTESIAN_POINT('Ctrl Pts',(0.177349721712035,1.83002938176795,6.66740739418118));
#50180=CARTESIAN_POINT('Ctrl Pts',(0.149206804324877,1.81415265074855,6.66523581012651));
#50181=CARTESIAN_POINT('Ctrl Pts',(0.139817253751994,1.80944448751456,6.66452363951018));
#50182=CARTESIAN_POINT('Ctrl Pts',(0.114051836474589,1.79806363136894,6.66262037585208));
#50183=CARTESIAN_POINT('Ctrl Pts',(0.0973266116169021,1.79226457097825,
6.66143664365141));
#50184=CARTESIAN_POINT('Ctrl Pts',(0.0794711688895155,1.78767630875198,
6.66027932505747));
#50185=CARTESIAN_POINT('Ctrl Pts',(0.0787334030158195,1.787489510453,6.66023169352785));
#50186=CARTESIAN_POINT('Ctrl Pts',(0.0776900177401195,1.78722926039604,
6.66016460215941));
#50187=CARTESIAN_POINT('Ctrl Pts',(0.0773849492829744,1.78715364148619,
6.66014501850574));
#50188=CARTESIAN_POINT('Ctrl Pts',(0.0768619283202994,1.78702480939567,
6.66011150022548));
#50189=CARTESIAN_POINT('Ctrl Pts',(0.0766440303894269,1.78697137740181,
6.66009755288307));
#50190=CARTESIAN_POINT('Ctrl Pts',(0.0762274060677701,1.78686967567683,
6.66007091776301));
#50191=CARTESIAN_POINT('Ctrl Pts',(0.0760286897687639,1.78682136762039,
6.6600582277452));
#50192=CARTESIAN_POINT('Ctrl Pts',(0.0755615208815455,1.78670826941778,
6.66002842712831));
#50193=CARTESIAN_POINT('Ctrl Pts',(0.0752930301973353,1.786643634987,6.66001132558069));
#50194=CARTESIAN_POINT('Ctrl Pts',(0.0745027738047079,1.78645446891009,
6.65996106399379));
#50195=CARTESIAN_POINT('Ctrl Pts',(0.0739807766175856,1.78633089397923,
6.65992795884736));
#50196=CARTESIAN_POINT('Ctrl Pts',(0.0695162087752438,1.78528573996641,
6.65964560542984));
#50197=CARTESIAN_POINT('Ctrl Pts',(0.0655566839218102,1.78443717957543,
6.65940045551308));
#50198=CARTESIAN_POINT('Ctrl Pts',(0.0611487147152334,1.78357906964804,
6.65913229563636));
#50199=CARTESIAN_POINT('Ctrl Pts',(0.0607152539548016,1.78349561074529,
6.65910597671003));
#50200=CARTESIAN_POINT('Ctrl Pts',(0.0595554264597815,1.78327476689968,
6.65903568659392));
#50201=CARTESIAN_POINT('Ctrl Pts',(0.0588287522527045,1.78313898941248,
6.65899178608695));
#50202=CARTESIAN_POINT('Ctrl Pts',(0.0573186857530803,1.78286221061923,
6.65890083470527));
#50203=CARTESIAN_POINT('Ctrl Pts',(0.056535224593241,1.78272160869003,6.65885380085295));
#50204=CARTESIAN_POINT('Ctrl Pts',(0.0533255441466637,1.78215785756886,
6.65866171373051));
#50205=CARTESIAN_POINT('Ctrl Pts',(0.0508949808578761,1.78175961494985,
6.65851765789609));
#50206=CARTESIAN_POINT('Ctrl Pts',(0.0186080583378787,1.77684884085909,
6.65661985516059));
#50207=CARTESIAN_POINT('Ctrl Pts',(-0.0117351319805428,1.77652583954778,
6.65500079427766));
#50208=CARTESIAN_POINT('Ctrl Pts',(-0.052449832174843,1.78183634691832,
6.65263182345073));
#50209=CARTESIAN_POINT('Ctrl Pts',(-0.0631388059993833,1.78378401613556,
6.65199269758384));
#50210=CARTESIAN_POINT('Ctrl Pts',(-0.0756320651681918,1.78671918144156,
6.65121644061594));
#50211=CARTESIAN_POINT('Ctrl Pts',(-0.0775515454949799,1.78718881401112,
6.65109635786801));
#50212=CARTESIAN_POINT('Ctrl Pts',(-0.0800995077087255,1.7878371081348,
6.65093582770652));
#50213=CARTESIAN_POINT('Ctrl Pts',(-0.0807319677813652,1.78800007762649,
6.65089588767806));
#50214=CARTESIAN_POINT('Ctrl Pts',(-0.081772041175835,1.78827145333573,
6.65083005213778));
#50215=CARTESIAN_POINT('Ctrl Pts',(-0.0821799469248575,1.78837873974289,
6.65080419292628));
#50216=CARTESIAN_POINT('Ctrl Pts',(-0.0829717573599277,1.78858866266157,
6.65075391938526));
#50217=CARTESIAN_POINT('Ctrl Pts',(-0.0833556853040245,1.78869120913865,
6.65072950801464));
#50218=CARTESIAN_POINT('Ctrl Pts',(-0.0842443294158892,1.78893032616989,
6.65067292348749));
#50219=CARTESIAN_POINT('Ctrl Pts',(-0.0847489038191593,1.78906741516558,
6.65064073355104));
#50220=CARTESIAN_POINT('Ctrl Pts',(-0.0861068966897092,1.78943992253722,
6.65055393295223));
#50221=CARTESIAN_POINT('Ctrl Pts',(-0.0869596778412041,1.7896776292693,
6.6504992480142));
#50222=CARTESIAN_POINT('Ctrl Pts',(-0.0931358100975883,1.79142663979053,
6.65010190515683));
#50223=CARTESIAN_POINT('Ctrl Pts',(-0.0984201520415046,1.79307123743203,
6.64975492026018));
#50224=CARTESIAN_POINT('Ctrl Pts',(-0.104356550236686,1.79508783506183,
6.64935678025263));
#50225=CARTESIAN_POINT('Ctrl Pts',(-0.105052995335693,1.79532708347909,
6.64930994029951));
#50226=CARTESIAN_POINT('Ctrl Pts',(-0.107361402723205,1.79612894217185,
6.64915425023359));
#50227=CARTESIAN_POINT('Ctrl Pts',(-0.108969693556249,1.79670196787344,
6.64904507154335));
#50228=CARTESIAN_POINT('Ctrl Pts',(-0.131573253173491,1.80495849131003,
6.64750060308036));
#50229=CARTESIAN_POINT('Ctrl Pts',(-0.151715020338753,1.81479257245665,
6.64599557362508));
#50230=CARTESIAN_POINT('Ctrl Pts',(-0.178132692410752,1.83128595671305,
6.64388808287417));
#50231=CARTESIAN_POINT('Ctrl Pts',(-0.185397917293255,1.83624611096482,
6.64329358844632));
#50232=CARTESIAN_POINT('Ctrl Pts',(-0.200944456264922,1.84782027489546,
6.64199956642229));
#50233=CARTESIAN_POINT('Ctrl Pts',(-0.209121766107187,1.85455871397967,
6.6413040805885));
#50234=CARTESIAN_POINT('Ctrl Pts',(-0.218063950077104,1.86269946160966,
6.64053943237398));
#50235=CARTESIAN_POINT('Ctrl Pts',(-0.219167625175041,1.86371842194622,
6.64044498466496));
#50236=CARTESIAN_POINT('Ctrl Pts',(-0.220561844094178,1.86502379939275,
6.64032562780793));
#50237=CARTESIAN_POINT('Ctrl Pts',(-0.220858999989643,1.86530308044206,
6.64030018610429));
#50238=CARTESIAN_POINT('Ctrl Pts',(-0.221333513363865,1.86575074963799,
6.64025955644224));
#50239=CARTESIAN_POINT('Ctrl Pts',(-0.221511209425123,1.8659187757783,6.6402443407279));
#50240=CARTESIAN_POINT('Ctrl Pts',(-0.221847869402671,1.86623784192354,
6.64021551227828));
#50241=CARTESIAN_POINT('Ctrl Pts',(-0.222006869105227,1.86638884064017,
6.64020189662269));
#50242=CARTESIAN_POINT('Ctrl Pts',(-0.222370549312114,1.86673492679859,
6.64017075240676));
#50243=CARTESIAN_POINT('Ctrl Pts',(-0.222575126952611,1.86693012112131,
6.64015323230564));
#50244=CARTESIAN_POINT('Ctrl Pts',(-0.223204117903708,1.86753184569167,
6.64009936172257));
#50245=CARTESIAN_POINT('Ctrl Pts',(-0.223627679310309,1.86793927071596,
6.64006308034086));
#50246=CARTESIAN_POINT('Ctrl Pts',(-0.226828153979922,1.8710347169569,6.63978887407476));
#50247=CARTESIAN_POINT('Ctrl Pts',(-0.229557774110707,1.87377147869617,
6.63955466358746));
#50248=CARTESIAN_POINT('Ctrl Pts',(-0.249557216689278,1.89455807697346,
6.63782982519433));
#50249=CARTESIAN_POINT('Ctrl Pts',(-0.26472750346581,1.91451445679514,6.63646622893819));
#50250=CARTESIAN_POINT('Ctrl Pts',(-0.287956828664474,1.9538179526262,6.63390288772782));
#50251=CARTESIAN_POINT('Ctrl Pts',(-0.296735117575865,1.97257781282311,
6.63272161881677));
#50252=CARTESIAN_POINT('Ctrl Pts',(-0.304327901150404,1.99393530565438,
6.63135078366399));
#50253=CARTESIAN_POINT('Ctrl Pts',(-0.304981477499188,1.99582951998574,
6.63122902998334));
#50254=CARTESIAN_POINT('Ctrl Pts',(-0.305825698700041,1.99835233029592,
6.63106660212111));
#50255=CARTESIAN_POINT('Ctrl Pts',(-0.306032157021054,1.99897561878129,
6.63102645076121));
#50256=CARTESIAN_POINT('Ctrl Pts',(-0.306368346594824,2.00000104812995,
6.63096035676862));
#50257=CARTESIAN_POINT('Ctrl Pts',(-0.306499194946625,2.00040282300822,
6.63093445100502));
#50258=CARTESIAN_POINT('Ctrl Pts',(-0.306751464593718,2.00118263185218,
6.63088415158185));
#50259=CARTESIAN_POINT('Ctrl Pts',(-0.30687297821767,2.00156063533511,6.63085976101402));
#50260=CARTESIAN_POINT('Ctrl Pts',(-0.307152291179562,2.0024350627221,6.63080331875745));
#50261=CARTESIAN_POINT('Ctrl Pts',(-0.307309585804897,2.00293164557779,
6.6307712505493));
#50262=CARTESIAN_POINT('Ctrl Pts',(-0.307728945588953,2.00426681050409,
6.63068498735583));
#50263=CARTESIAN_POINT('Ctrl Pts',(-0.3079887852483,2.00510608206454,6.63063071952063));
#50264=CARTESIAN_POINT('Ctrl Pts',(-0.309822187866375,2.011114757208,6.63024186974474));
#50265=CARTESIAN_POINT('Ctrl Pts',(-0.311268868949222,2.01632168745286,
6.6299031653194));
#50266=CARTESIAN_POINT('Ctrl Pts',(-0.313038737743376,2.02337483111253,
6.62944167140359));
#50267=CARTESIAN_POINT('Ctrl Pts',(-0.313477785404343,2.02519127282414,
6.62932258423232));
#50268=CARTESIAN_POINT('Ctrl Pts',(-0.319487064661382,2.05103529236545,
6.62762483912698));
#50269=CARTESIAN_POINT('Ctrl Pts',(-0.322295879094073,2.07561755170173,
6.6259589500366));
#50270=CARTESIAN_POINT('Ctrl Pts',(-0.322259321826866,2.11854910398288,
6.62305557491489));
#50271=CARTESIAN_POINT('Ctrl Pts',(-0.320689372072886,2.13679183935199,
6.6218268495696));
#50272=CARTESIAN_POINT('Ctrl Pts',(-0.317394801190109,2.15588302548084,
6.6206061851641));
#50273=CARTESIAN_POINT('Ctrl Pts',(-0.317203276167546,2.15696010910883,
6.62053754730237));
#50274=CARTESIAN_POINT('Ctrl Pts',(-0.316938468303947,2.15840654651988,
6.62044569989732));
#50275=CARTESIAN_POINT('Ctrl Pts',(-0.316870020188938,2.15877676136142,
6.62042222051305));
#50276=CARTESIAN_POINT('Ctrl Pts',(-0.316761677966465,2.15935706126999,
6.62038546358732));
#50277=CARTESIAN_POINT('Ctrl Pts',(-0.31672222352666,2.15956722652362,6.62037216097588));
#50278=CARTESIAN_POINT('Ctrl Pts',(-0.316645962703296,2.15997123358497,
6.62034660747485));
#50279=CARTESIAN_POINT('Ctrl Pts',(-0.316609187759051,2.16016507941311,
6.62033435492812));
#50280=CARTESIAN_POINT('Ctrl Pts',(-0.316521437390518,2.16062531532674,
6.62030528387959));
#50281=CARTESIAN_POINT('Ctrl Pts',(-0.316470303736836,2.16089167463815,
6.62028847456349));
#50282=CARTESIAN_POINT('Ctrl Pts',(-0.316318133471877,2.16167897247615,
6.62023883476007));
#50283=CARTESIAN_POINT('Ctrl Pts',(-0.316216145789568,2.1621997295841,6.62020605850546));
#50284=CARTESIAN_POINT('Ctrl Pts',(-0.315406065560184,2.16628257111189,
6.61994952374986));
#50285=CARTESIAN_POINT('Ctrl Pts',(-0.314639056723921,2.16983288710256,
6.61972906385438));
#50286=CARTESIAN_POINT('Ctrl Pts',(-0.311705713359139,2.18237920164775,
6.61895685616938));
#50287=CARTESIAN_POINT('Ctrl Pts',(-0.309212061746471,2.19129466079152,
6.61842067977414));
#50288=CARTESIAN_POINT('Ctrl Pts',(-0.300363237591256,2.21837728376119,
6.61679696242207));
#50289=CARTESIAN_POINT('Ctrl Pts',(-0.292763112877847,2.2360921192581,6.61573995573784));
#50290=CARTESIAN_POINT('Ctrl Pts',(-0.274898359517753,2.26920426749017,
6.61361374702799));
#50291=CARTESIAN_POINT('Ctrl Pts',(-0.264801439263323,2.28460563208022,
6.61255083334303));
#50292=CARTESIAN_POINT('Ctrl Pts',(-0.252653501148617,2.3000725817429,6.61135621500177));
#50293=CARTESIAN_POINT('Ctrl Pts',(-0.251853088440833,2.30107921666802,
6.61127785958688));
#50294=CARTESIAN_POINT('Ctrl Pts',(-0.250727208068352,2.30247790580335,
6.61116812599454));
#50295=CARTESIAN_POINT('Ctrl Pts',(-0.250406796002273,2.30287402917928,
6.6111369510394));
#50296=CARTESIAN_POINT('Ctrl Pts',(-0.249851466942024,2.3035572590397,6.61108301161048));
#50297=CARTESIAN_POINT('Ctrl Pts',(-0.24961699040183,2.30384472360525,6.61106026494753));
#50298=CARTESIAN_POINT('Ctrl Pts',(-0.249130262527172,2.30443934527068,
6.61101310518142));
#50299=CARTESIAN_POINT('Ctrl Pts',(-0.248877938352919,2.30474644172868,
6.61098868914785));
#50300=CARTESIAN_POINT('Ctrl Pts',(-0.248286218312451,2.30546389708571,
6.61093150591951));
#50301=CARTESIAN_POINT('Ctrl Pts',(-0.247946372907587,2.3058738821854,6.61089872047034));
#50302=CARTESIAN_POINT('Ctrl Pts',(-0.246847473299658,2.30719291271606,
6.61079288914048));
#50303=CARTESIAN_POINT('Ctrl Pts',(-0.246084430639593,2.30809860905581,
6.61071968038369));
#50304=CARTESIAN_POINT('Ctrl Pts',(-0.234651407080719,2.32151826212848,
6.60962679361422));
#50305=CARTESIAN_POINT('Ctrl Pts',(-0.223045665703547,2.33319970181887,
6.60856737408695));
#50306=CARTESIAN_POINT('Ctrl Pts',(-0.187577046801874,2.36382045285604,
6.60546187578407));
#50307=CARTESIAN_POINT('Ctrl Pts',(-0.161857270970549,2.38033632784369,
6.60334532445197));
#50308=CARTESIAN_POINT('Ctrl Pts',(-0.130766477397451,2.39457700068702,
6.60114438517799));
#50309=CARTESIAN_POINT('Ctrl Pts',(-0.127300139510424,2.39609146985853,
6.60090384315475));
#50310=CARTESIAN_POINT('Ctrl Pts',(-0.123268595509839,2.39776898766724,
6.60063029361198));
#50311=CARTESIAN_POINT('Ctrl Pts',(-0.122728816269785,2.39799186956201,
6.60059379574177));
#50312=CARTESIAN_POINT('Ctrl Pts',(-0.121927462265375,2.39832021236869,
6.60053980309165));
#50313=CARTESIAN_POINT('Ctrl Pts',(-0.121666353910043,2.39842679753981,
6.6005222406038));
#50314=CARTESIAN_POINT('Ctrl Pts',(-0.121202064911155,2.3986156109941,6.60049106591567));
#50315=CARTESIAN_POINT('Ctrl Pts',(-0.120998940352899,2.39869797472143,
6.60047744547432));
#50316=CARTESIAN_POINT('Ctrl Pts',(-0.120568619413325,2.39887195192582,
6.60044862944556));
#50317=CARTESIAN_POINT('Ctrl Pts',(-0.120341403196061,2.39896351334728,
6.6004334370636));
#50318=CARTESIAN_POINT('Ctrl Pts',(-0.119733958469073,2.39920749091188,
6.60039288211408));
#50319=CARTESIAN_POINT('Ctrl Pts',(-0.119353541801786,2.39935944196272,
6.60036754776159));
#50320=CARTESIAN_POINT('Ctrl Pts',(-0.117558821456246,2.40007234800676,
6.60024832034533));
#50321=CARTESIAN_POINT('Ctrl Pts',(-0.116140816368967,2.400624020211,6.60015497973448));
#50322=CARTESIAN_POINT('Ctrl Pts',(-0.104595262146491,2.40502191088111,
6.59940154865229));
#50323=CARTESIAN_POINT('Ctrl Pts',(-0.09428240192044,2.40836571941136,6.59876931500065));
#50324=CARTESIAN_POINT('Ctrl Pts',(-0.0556052603918844,2.418783681615,6.59647997861232));
#50325=CARTESIAN_POINT('Ctrl Pts',(-0.0264890291801961,2.42251114144918,
6.5949021085755));
#50326=CARTESIAN_POINT('Ctrl Pts',(0.0121434294342142,2.4221836344091,6.5926504233315));
#50327=CARTESIAN_POINT('Ctrl Pts',(0.0215460517823926,2.4216916204006,6.59209140229217));
#50328=CARTESIAN_POINT('Ctrl Pts',(0.0320521523153674,2.42067919291897,
6.59144953770405));
#50329=CARTESIAN_POINT('Ctrl Pts',(0.0331906547719284,2.42056335664285,
6.59137975629247));
#50330=CARTESIAN_POINT('Ctrl Pts',(0.0348449754134277,2.42038613128017,
6.59127802374368));
#50331=CARTESIAN_POINT('Ctrl Pts',(0.0353613091545143,2.42032955411283,
6.59124622421171));
#50332=CARTESIAN_POINT('Ctrl Pts',(0.0362718440417313,2.42022755411161,
6.59119006221195));
#50333=CARTESIAN_POINT('Ctrl Pts',(0.0366661032686878,2.42018265092185,
6.59116571617009));
#50334=CARTESIAN_POINT('Ctrl Pts',(0.0374806038395108,2.42008836124264,
6.59111536128445));
#50335=CARTESIAN_POINT('Ctrl Pts',(0.0379008326709435,2.42003887505631,
6.59108934934049));
#50336=CARTESIAN_POINT('Ctrl Pts',(0.0389755377077947,2.41991017129936,
6.5910227428645));
#50337=CARTESIAN_POINT('Ctrl Pts',(0.0396298681788365,2.41982977312659,
6.59098211114579));
#50338=CARTESIAN_POINT('Ctrl Pts',(0.0422932818733531,2.41949421819349,
6.590816398588));
#50339=CARTESIAN_POINT('Ctrl Pts',(0.0443001514093276,2.41922213807145,
6.59069078444226));
#50340=CARTESIAN_POINT('Ctrl Pts',(0.0770672839228347,2.41446481462806,
6.58862720030297));
#50341=CARTESIAN_POINT('Ctrl Pts',(0.107015769672301,2.40557188925545,6.58653480559351));
#50342=CARTESIAN_POINT('Ctrl Pts',(0.151410314067701,2.38505132634152,6.5832286254383));
#50343=CARTESIAN_POINT('Ctrl Pts',(0.166954479375147,2.37623488579184,6.58203155674657));
#50344=CARTESIAN_POINT('Ctrl Pts',(0.182507440372719,2.3656185005857,6.58084632664786));
#50345=CARTESIAN_POINT('Ctrl Pts',(0.183321683230509,2.36505719036264,6.58078431960711));
#50346=CARTESIAN_POINT('Ctrl Pts',(0.184429686807892,2.3642858237448,6.5807000153466));
#50347=CARTESIAN_POINT('Ctrl Pts',(0.184725686528502,2.36407901610719,6.58067750093006));
#50348=CARTESIAN_POINT('Ctrl Pts',(0.185193907746836,2.36375070915435,6.58064189919249));
#50349=CARTESIAN_POINT('Ctrl Pts',(0.185366357590892,2.36362953840584,6.58062878940705));
#50350=CARTESIAN_POINT('Ctrl Pts',(0.185715250200877,2.36338387972074,6.58060227183979));
#50351=CARTESIAN_POINT('Ctrl Pts',(0.185891686187882,2.36325938399297,6.58058886474506));
#50352=CARTESIAN_POINT('Ctrl Pts',(0.186298200620303,2.36297192922799,6.58055798082721));
#50353=CARTESIAN_POINT('Ctrl Pts',(0.186528191075332,2.36280884507922,6.58054051265102));
#50354=CARTESIAN_POINT('Ctrl Pts',(0.187011833072078,2.36246494422835,6.58050378857623));
#50355=CARTESIAN_POINT('Ctrl Pts',(0.187265437283023,2.36228406100809,6.58048453725561));
#50356=CARTESIAN_POINT('Ctrl Pts',(0.187938784062659,2.36180232192658,6.58043343623169));
#50357=CARTESIAN_POINT('Ctrl Pts',(0.188358068536367,2.36150082284181,6.58040163007021));
#50358=CARTESIAN_POINT('Ctrl Pts',(0.189625570720635,2.36058475724289,6.58030551549271));
#50359=CARTESIAN_POINT('Ctrl Pts',(0.190471528581842,2.35996705492589,6.58024141536082));
#50360=CARTESIAN_POINT('Ctrl Pts',(0.200744108929318,2.35238915075826,6.57946343371671));
#50361=CARTESIAN_POINT('Ctrl Pts',(0.209788514531976,2.34492310024092,6.57878242133047));
#50362=CARTESIAN_POINT('Ctrl Pts',(0.241488246609738,2.31570780049324,6.57632765415075));
#50363=CARTESIAN_POINT('Ctrl Pts',(0.261337113803508,2.29117905325402,6.57463365179721));
#50364=CARTESIAN_POINT('Ctrl Pts',(0.280620525559445,2.25860356985345,6.57239771115475));
#50365=CARTESIAN_POINT('Ctrl Pts',(0.283745449642445,2.25294274294638,6.57201044179386));
#50366=CARTESIAN_POINT('Ctrl Pts',(0.287168828737621,2.24627475064916,6.5715542454528));
#50367=CARTESIAN_POINT('Ctrl Pts',(0.287635370120244,2.24535519492971,6.57149133385925));
#50368=CARTESIAN_POINT('Ctrl Pts',(0.28832299634454,2.24398360530252,6.57139749131474));
#50369=CARTESIAN_POINT('Ctrl Pts',(0.288547451679594,2.24353326075053,6.57136667848545));
#50370=CARTESIAN_POINT('Ctrl Pts',(0.288945424648095,2.24273006624821,6.57131172130711));
#50371=CARTESIAN_POINT('Ctrl Pts',(0.289119353320351,2.24237742015409,6.57128759137753));
#50372=CARTESIAN_POINT('Ctrl Pts',(0.289484217494473,2.24163422056622,6.57123673573114));
#50373=CARTESIAN_POINT('Ctrl Pts',(0.289675008868199,2.24124359754711,6.57121000504982));
#50374=CARTESIAN_POINT('Ctrl Pts',(0.290175874567537,2.24021285016091,6.57113946642967));
#50375=CARTESIAN_POINT('Ctrl Pts',(0.290484619836224,2.23957208588011,6.57109561236978));
#50376=CARTESIAN_POINT('Ctrl Pts',(0.291863423442889,2.23668614966501,6.57089807687009));
#50377=CARTESIAN_POINT('Ctrl Pts',(0.292909567846075,2.23442970639169,6.57074356980709));
#50378=CARTESIAN_POINT('Ctrl Pts',(0.300425392804924,2.21771437256489,6.56959830864876));
#50379=CARTESIAN_POINT('Ctrl Pts',(0.305846362315273,2.20281030430877,6.5685716778259));
#50380=CARTESIAN_POINT('Ctrl Pts',(0.318018798573217,2.15969884950924,6.56559334462402));
#50381=CARTESIAN_POINT('Ctrl Pts',(0.322095117045738,2.1308960169106,6.56358322026048));
#50382=CARTESIAN_POINT('Ctrl Pts',(0.322293895382364,2.09782486587061,6.56145005689894));
#50383=CARTESIAN_POINT('Ctrl Pts',(0.322239903828466,2.09371235099165,6.56118814585552));
#50384=CARTESIAN_POINT('Ctrl Pts',(0.322089815645785,2.0890630536818,6.56089668321325));
#50385=CARTESIAN_POINT('Ctrl Pts',(0.322071073429158,2.08852438203574,6.56086298454879));
#50386=CARTESIAN_POINT('Ctrl Pts',(0.322040659918391,2.08770912471258,6.56081209224406));
#50387=CARTESIAN_POINT('Ctrl Pts',(0.322029983631112,2.0874325062179,6.56079484341768));
#50388=CARTESIAN_POINT('Ctrl Pts',(0.322010793865534,2.0869513928304,6.56076487662479));
#50389=CARTESIAN_POINT('Ctrl Pts',(0.322002441993572,2.08674689222477,6.56075214956509));
#50390=CARTESIAN_POINT('Ctrl Pts',(0.321984727422373,2.08632304373972,6.56072579345984));
#50391=CARTESIAN_POINT('Ctrl Pts',(0.321975335398093,2.08610369756302,6.5607121661422));
#50392=CARTESIAN_POINT('Ctrl Pts',(0.321952401135233,2.08558058654588,6.56067969570443));
#50393=CARTESIAN_POINT('Ctrl Pts',(0.321938653077535,2.0852768299085,6.56066086420566));
#50394=CARTESIAN_POINT('Ctrl Pts',(0.321908527065373,2.08463143429872,6.5606209011622));
#50395=CARTESIAN_POINT('Ctrl Pts',(0.321892035080365,2.08428980065445,6.56059977600045));
#50396=CARTESIAN_POINT('Ctrl Pts',(0.321845567337499,2.08335801747154,6.56054223570543));
#50397=CARTESIAN_POINT('Ctrl Pts',(0.321814512123512,2.08276791954618,6.56050587992766));
#50398=CARTESIAN_POINT('Ctrl Pts',(0.321712228515039,2.08092116656538,6.56039235709828));
#50399=CARTESIAN_POINT('Ctrl Pts',(0.321635260149936,2.0796648234084,6.56031549756488));
#50400=CARTESIAN_POINT('Ctrl Pts',(0.319682461462954,2.05058221953155,6.55854420973092));
#50401=CARTESIAN_POINT('Ctrl Pts',(0.314209481574766,2.02311080257267,6.55703144130547));
#50402=CARTESIAN_POINT('Ctrl Pts',(0.298576707610294,1.97692099675488,6.5542902562956));
#50403=CARTESIAN_POINT('Ctrl Pts',(0.289985835959451,1.95785743138839,6.55309371855112));
#50404=CARTESIAN_POINT('Ctrl Pts',(0.278968116826452,1.93863193183028,6.55174788249451));
#50405=CARTESIAN_POINT('Ctrl Pts',(0.278315312194932,1.93750861391712,6.55166873007036));
#50406=CARTESIAN_POINT('Ctrl Pts',(0.277395952932744,1.93594841427286,6.55155805903196));
#50407=CARTESIAN_POINT('Ctrl Pts',(0.277135117037612,1.93550816317265,6.5515267482663));
#50408=CARTESIAN_POINT('Ctrl Pts',(0.276683086279855,1.93474933149786,6.55147263738485));
#50409=CARTESIAN_POINT('Ctrl Pts',(0.276492386439839,1.93443045596283,6.55144985534888));
#50410=CARTESIAN_POINT('Ctrl Pts',(0.276096727534256,1.93377145141046,6.55140268216278));
#50411=CARTESIAN_POINT('Ctrl Pts',(0.275891690461676,1.93343137014039,6.55137828818624));
#50412=CARTESIAN_POINT('Ctrl Pts',(0.27541134477959,1.93263797299754,6.55132126030504));
#50413=CARTESIAN_POINT('Ctrl Pts',(0.275135545264565,1.93218495704413,6.55128860843934));
#50414=CARTESIAN_POINT('Ctrl Pts',(0.274246389646173,1.93073255370815,6.55118363345457));
#50415=CARTESIAN_POINT('Ctrl Pts',(0.27362870226348,1.92973584097797,6.55111115113403));
#50416=CARTESIAN_POINT('Ctrl Pts',(0.264093491446308,1.91453553504728,6.54999889305642));
#50417=CARTESIAN_POINT('Ctrl Pts',(0.254087554383901,1.90104826643011,6.54891772302961));
#50418=CARTESIAN_POINT('Ctrl Pts',(0.224088785208224,1.86658626590658,6.54588687498637));
#50419=CARTESIAN_POINT('Ctrl Pts',(0.20224961482957,1.8474277936976,6.54387976400894));
#50420=CARTESIAN_POINT('Ctrl Pts',(0.17407181074574,1.82873607912093,6.54168805340087));
#50421=CARTESIAN_POINT('Ctrl Pts',(0.169933617456621,1.82612469589766,6.54137541301936));
#50422=CARTESIAN_POINT('Ctrl Pts',(0.165251892355717,1.82331731525357,6.54103324705182));
#50423=CARTESIAN_POINT('Ctrl Pts',(0.164765717023042,1.82302752037242,6.54099785125269));
#50424=CARTESIAN_POINT('Ctrl Pts',(0.164034693755202,1.82259438477016,6.54094483703856));
#50425=CARTESIAN_POINT('Ctrl Pts',(0.163790419073719,1.82245008604291,6.54092715680016));
#50426=CARTESIAN_POINT('Ctrl Pts',(0.163368070351908,1.82220134659791,6.54089664815838));
#50427=CARTESIAN_POINT('Ctrl Pts',(0.163190086470525,1.82209675438957,6.54088380984867));
#50428=CARTESIAN_POINT('Ctrl Pts',(0.162832538957146,1.82188710356793,6.54085805654472));
#50429=CARTESIAN_POINT('Ctrl Pts',(0.162652974385194,1.82178204797511,6.54084514179551));
#50430=CARTESIAN_POINT('Ctrl Pts',(0.162222596407782,1.82153081119143,6.54081423277895));
#50431=CARTESIAN_POINT('Ctrl Pts',(0.161971686160794,1.82138479441208,6.54079624928597));
#50432=CARTESIAN_POINT('Ctrl Pts',(0.161173558919852,1.82092176819127,6.540739159766));
#50433=CARTESIAN_POINT('Ctrl Pts',(0.16062560167473,1.82060602786211,6.54070013580343));
#50434=CARTESIAN_POINT('Ctrl Pts',(0.15934374980918,1.81987242510667,6.54060923626793));
#50435=CARTESIAN_POINT('Ctrl Pts',(0.15860913112974,1.8194558281167,6.54055744002598));
#50436=CARTESIAN_POINT('Ctrl Pts',(0.15609027469624,1.8180404590163,6.54038082736188));
#50437=CARTESIAN_POINT('Ctrl Pts',(0.154298131855275,1.81705575886691,6.54025685479047));
#50438=CARTESIAN_POINT('Ctrl Pts',(0.147105768656463,1.81319254716358,6.53976552330466));
#50439=CARTESIAN_POINT('Ctrl Pts',(0.141633105896393,1.81045087565736,6.53940550745751));
#50440=CARTESIAN_POINT('Ctrl Pts',(0.125456476851448,1.80291527153451,6.53837163266596));
#50441=CARTESIAN_POINT('Ctrl Pts',(0.11456465480888,1.79854745620502,6.53771292899801));
#50442=CARTESIAN_POINT('Ctrl Pts',(0.081371271700429,1.78729600772826,6.53575177434347));
#50443=CARTESIAN_POINT('Ctrl Pts',(0.0585390382962561,1.78222942980033,
6.53445747884568));
#50444=CARTESIAN_POINT('Ctrl Pts',(0.0287112392533252,1.7789367734667,6.53268686712636));
#50445=CARTESIAN_POINT('Ctrl Pts',(0.0220408696398692,1.7784100111886,6.53228638481466));
#50446=CARTESIAN_POINT('Ctrl Pts',(0.0143189535286426,1.77804157419437,
6.53181590634271));
#50447=CARTESIAN_POINT('Ctrl Pts',(0.0132783977728525,1.77799698061966,
6.53175236520624));
#50448=CARTESIAN_POINT('Ctrl Pts',(0.0117327741854933,1.77793824675036,
6.53165776474484));
#50449=CARTESIAN_POINT('Ctrl Pts',(0.011227852623753,1.77792024866939,6.53162682637236));
#50450=CARTESIAN_POINT('Ctrl Pts',(0.0103296500411853,1.7778903466729,6.53157172818916));
#50451=CARTESIAN_POINT('Ctrl Pts',(0.00993638474178478,1.77787797546184,
6.53154758307193));
#50452=CARTESIAN_POINT('Ctrl Pts',(0.00910965772366165,1.77785348395876,
6.53149678003822));
#50453=CARTESIAN_POINT('Ctrl Pts',(0.00867619251796588,1.7778415182836,
6.5314701173252));
#50454=CARTESIAN_POINT('Ctrl Pts',(0.00753656667565948,1.77781236096473,
6.53139994941154));
#50455=CARTESIAN_POINT('Ctrl Pts',(0.00683037423865473,1.77779661615768,
6.53135639896288));
#50456=CARTESIAN_POINT('Ctrl Pts',(0.00368471339536192,1.77773682887269,
6.53116209410805));
#50457=CARTESIAN_POINT('Ctrl Pts',(0.00124489460553541,1.77771816947155,
6.53101054687556));
#50458=CARTESIAN_POINT('Ctrl Pts',(-0.0165269742594732,1.77778405987537,
6.52990028164857));
#50459=CARTESIAN_POINT('Ctrl Pts',(-0.0318331850297289,1.77893493016606,
6.52890802311551));
#50460=CARTESIAN_POINT('Ctrl Pts',(-0.0501437711971647,1.78163402893598,
6.52767945594422));
#50461=CARTESIAN_POINT('Ctrl Pts',(-0.0532828805152529,1.78214433586042,
6.52746739989681));
#50462=CARTESIAN_POINT('Ctrl Pts',(-0.0589618837880661,1.78315402873722,
6.52708135720204));
#50463=CARTESIAN_POINT('Ctrl Pts',(-0.0615043211097875,1.78363772124545,
6.52690764804384));
#50464=CARTESIAN_POINT('Ctrl Pts',(-0.0661756015597744,1.78458485945539,
6.52658699788433));
#50465=CARTESIAN_POINT('Ctrl Pts',(-0.0683061159734176,1.78503937466598,
6.52644017877712));
#50466=CARTESIAN_POINT('Ctrl Pts',(-0.0876362694546695,1.789368548689,6.52510332449872));
#50467=CARTESIAN_POINT('Ctrl Pts',(-0.104495958698296,1.794627030072,6.52390086560803));
#50468=CARTESIAN_POINT('Ctrl Pts',(-0.122261377290685,1.80181268025934,
6.52263909205611));
#50469=CARTESIAN_POINT('Ctrl Pts',(-0.123677324419373,1.80239717474075,
6.52253857815013));
#50470=CARTESIAN_POINT('Ctrl Pts',(-0.125393920482938,1.80312014256981,
6.52241682921519));
#50471=CARTESIAN_POINT('Ctrl Pts',(-0.125698572189652,1.80324900338345,
6.52239522603158));
#50472=CARTESIAN_POINT('Ctrl Pts',(-0.126382642550114,1.80353959218792,
6.52234672794862));
#50473=CARTESIAN_POINT('Ctrl Pts',(-0.126761950886306,1.80370158024603,
6.52231984336279));
#50474=CARTESIAN_POINT('Ctrl Pts',(-0.127960824949597,1.80421629692631,
6.52223489401904));
#50475=CARTESIAN_POINT('Ctrl Pts',(-0.128779244231137,1.80457170410686,
6.52217693884462));
#50476=CARTESIAN_POINT('Ctrl Pts',(-0.130189726635036,1.8051911959381,6.52207713244787));
#50477=CARTESIAN_POINT('Ctrl Pts',(-0.130782484686598,1.805453674974,6.5220352115436));
#50478=CARTESIAN_POINT('Ctrl Pts',(-0.13521274680968,1.80743144848045,6.52172208842481));
#50479=CARTESIAN_POINT('Ctrl Pts',(-0.139017384045852,1.8092199880199,6.52145426517325));
#50480=CARTESIAN_POINT('Ctrl Pts',(-0.143272370870119,1.81132284899061,
6.5211568654486));
#50481=CARTESIAN_POINT('Ctrl Pts',(-0.143757981903908,1.81156437040699,
6.52112295564231));
#50482=CARTESIAN_POINT('Ctrl Pts',(-0.144491305824928,1.81193140525848,
6.52107179885324));
#50483=CARTESIAN_POINT('Ctrl Pts',(-0.144739466957916,1.81205601336108,
6.52105449587812));
#50484=CARTESIAN_POINT('Ctrl Pts',(-0.145170451377914,1.81227311969275,
6.52102446127536));
#50485=CARTESIAN_POINT('Ctrl Pts',(-0.145353347558678,1.81236547154656,
6.52101172045395));
#50486=CARTESIAN_POINT('Ctrl Pts',(-0.145720881774483,1.81255149486372,
6.52098612754868));
#50487=CARTESIAN_POINT('Ctrl Pts',(-0.145905517457611,1.81264516975367,
6.52097327575344));
#50488=CARTESIAN_POINT('Ctrl Pts',(-0.146353135063906,1.81287281113039,
6.52094213095631));
#50489=CARTESIAN_POINT('Ctrl Pts',(-0.146616024364182,1.81300696152606,
6.52092384957982));
#50490=CARTESIAN_POINT('Ctrl Pts',(-0.147462792210968,1.81344052781285,
6.52086499689225));
#50491=CARTESIAN_POINT('Ctrl Pts',(-0.148045945500632,1.81374136829523,
6.52082451482246));
#50492=CARTESIAN_POINT('Ctrl Pts',(-0.149413585612766,1.81445221142105,
6.52072967924024));
#50493=CARTESIAN_POINT('Ctrl Pts',(-0.150197314667897,1.81486367148941,
6.52067541496352));
#50494=CARTESIAN_POINT('Ctrl Pts',(-0.152905147709779,1.81629955416785,
6.5204881765639));
#50495=CARTESIAN_POINT('Ctrl Pts',(-0.154820594487153,1.81734029070577,
6.5203561646394));
#50496=CARTESIAN_POINT('Ctrl Pts',(-0.163287939903117,1.82205282611388,
6.5197738823267));
#50497=CARTESIAN_POINT('Ctrl Pts',(-0.169721322019515,1.82593381658319,
6.51933490045365));
#50498=CARTESIAN_POINT('Ctrl Pts',(-0.200372413392151,1.84591802950562,
6.51723139287794));
#50499=CARTESIAN_POINT('Ctrl Pts',(-0.222469960322216,1.86502329037212,
6.51566445214189));
#50500=CARTESIAN_POINT('Ctrl Pts',(-0.243555069483027,1.88893148170922,
6.51381768202279));
#50501=CARTESIAN_POINT('Ctrl Pts',(-0.245376823130721,1.8910521468113,6.51365484733399));
#50502=CARTESIAN_POINT('Ctrl Pts',(-0.248325045853791,1.89457584586999,
6.51338562341313));
#50503=CARTESIAN_POINT('Ctrl Pts',(-0.249467782282284,1.89596510855371,
6.5132798133605));
#50504=CARTESIAN_POINT('Ctrl Pts',(-0.254680453659486,1.90241158535197,
6.51279020298307));
#50505=CARTESIAN_POINT('Ctrl Pts',(-0.258608409855853,1.90758119530096,
6.51240137608929));
#50506=CARTESIAN_POINT('Ctrl Pts',(-0.262976867573813,1.91370612314425,
6.51194349605141));
#50507=CARTESIAN_POINT('Ctrl Pts',(-0.263572288430144,1.91454949402686,
6.511880509261));
#50508=CARTESIAN_POINT('Ctrl Pts',(-0.264452013394673,1.91580835611516,
6.51178657615299));
#50509=CARTESIAN_POINT('Ctrl Pts',(-0.264739416852172,1.91622168183999,
6.51175574829349));
#50510=CARTESIAN_POINT('Ctrl Pts',(-0.265249588533674,1.916959059108,6.51170077426023));
#50511=CARTESIAN_POINT('Ctrl Pts',(-0.265472734831055,1.91728284886455,
6.51167664253873));
#50512=CARTESIAN_POINT('Ctrl Pts',(-0.265941248375334,1.91796534145726,
6.51162579331938));
#50513=CARTESIAN_POINT('Ctrl Pts',(-0.266186483607361,1.9183241335785,6.51159907087729));
#50514=CARTESIAN_POINT('Ctrl Pts',(-0.266830828512369,1.91927094964538,
6.51152857719188));
#50515=CARTESIAN_POINT('Ctrl Pts',(-0.267228718532436,1.91985979719879,
6.51148475993368));
#50516=CARTESIAN_POINT('Ctrl Pts',(-0.269007101821032,1.9225105300736,6.51128761882485));
#50517=CARTESIAN_POINT('Ctrl Pts',(-0.270365672135567,1.92458695732144,
6.51113347339291));
#50518=CARTESIAN_POINT('Ctrl Pts',(-0.280185294478183,1.93998030029493,
6.5099925363232));
#50519=CARTESIAN_POINT('Ctrl Pts',(-0.287680961252544,1.95388485552828,
6.5089701615377));
#50520=CARTESIAN_POINT('Ctrl Pts',(-0.303379233991276,1.98893886939149,
6.50641705632829));
#50521=CARTESIAN_POINT('Ctrl Pts',(-0.310427924740421,2.01051284673528,
6.50486282108069));
#50522=CARTESIAN_POINT('Ctrl Pts',(-0.315478494361835,2.0341452786251,6.50325608655099));
#50523=CARTESIAN_POINT('Ctrl Pts',(-0.315788123068088,2.03564639730103,
6.50315445543284));
#50524=CARTESIAN_POINT('Ctrl Pts',(-0.317795972171665,2.04574427959782,
6.50247388880638));
#50525=CARTESIAN_POINT('Ctrl Pts',(-0.319153847160087,2.05440594942296,
6.50190508699605));
#50526=CARTESIAN_POINT('Ctrl Pts',(-0.320238466186652,2.06381980468292,
6.50131044081574));
#50527=CARTESIAN_POINT('Ctrl Pts',(-0.320317555548087,2.0645268356471,6.50126592293545));
#50528=CARTESIAN_POINT('Ctrl Pts',(-0.320424842001705,2.06551556307584,
6.50120387381596));
#50529=CARTESIAN_POINT('Ctrl Pts',(-0.320455009451085,2.06579703695569,
6.50118623277031));
#50530=CARTESIAN_POINT('Ctrl Pts',(-0.320506518066305,2.06628368270037,
6.50115577349179));
#50531=CARTESIAN_POINT('Ctrl Pts',(-0.320528033126031,2.06648883535089,
6.50114294542723));
#50532=CARTESIAN_POINT('Ctrl Pts',(-0.320570840292977,2.06690082758617,
6.50111720908857));
#50533=CARTESIAN_POINT('Ctrl Pts',(-0.320592129157454,2.06710766680324,
6.50110430106405));
#50534=CARTESIAN_POINT('Ctrl Pts',(-0.320635302441027,2.06753115540728,
6.5010778987879));
#50535=CARTESIAN_POINT('Ctrl Pts',(-0.320657167529375,2.06774780699946,
6.5010644056214));
#50536=CARTESIAN_POINT('Ctrl Pts',(-0.320707432770591,2.06825096719705,
6.5010331005255));
#50537=CARTESIAN_POINT('Ctrl Pts',(-0.320735668654021,2.06853749258546,
6.50101529785008));
#50538=CARTESIAN_POINT('Ctrl Pts',(-0.32080799544783,2.06928164960522,6.50096912274472));
#50539=CARTESIAN_POINT('Ctrl Pts',(-0.320851491318806,2.06973934040992,
6.50094078339405));
#50540=CARTESIAN_POINT('Ctrl Pts',(-0.321807863194267,2.08003680381599,
6.50030451225739));
#50541=CARTESIAN_POINT('Ctrl Pts',(-0.3222687483972,2.08991429204376,6.49972142836674));
#50542=CARTESIAN_POINT('Ctrl Pts',(-0.322274936831736,2.09979822016873,
6.49915140185063));
#50543=CARTESIAN_POINT('',(-0.322023435600497,2.1002684890243,6.24937721618673));
#50544=CARTESIAN_POINT('Ctrl Pts',(-0.322274936536932,2.09979774986705,
6.49915142897391));
#50545=CARTESIAN_POINT('Ctrl Pts',(-0.322289363947956,2.1227870695989,6.49782558650495));
#50546=CARTESIAN_POINT('Ctrl Pts',(-0.319843928885221,2.14571420094704,
6.49657169036954));
#50547=CARTESIAN_POINT('Ctrl Pts',(-0.311612842615433,2.1837356855591,6.49436792214443));
#50548=CARTESIAN_POINT('Ctrl Pts',(-0.307100997708914,2.1990106369823,6.49344757464164));
#50549=CARTESIAN_POINT('Ctrl Pts',(-0.300599370908085,2.21622138617848,
6.49233807854255));
#50550=CARTESIAN_POINT('Ctrl Pts',(-0.299691227544351,2.21854349408354,
6.49218683954317));
#50551=CARTESIAN_POINT('Ctrl Pts',(-0.298489281371814,2.22151473715201,
6.49199125054724));
#50552=CARTESIAN_POINT('Ctrl Pts',(-0.298220127618156,2.22217380205915,
6.49194773412867));
#50553=CARTESIAN_POINT('Ctrl Pts',(-0.297783047106699,2.22323401151387,
6.49187751631622));
#50554=CARTESIAN_POINT('Ctrl Pts',(-0.29761648725322,2.22363571996017,6.49185086128474));
#50555=CARTESIAN_POINT('Ctrl Pts',(-0.297297790657745,2.22439997540648,
6.49180005427881));
#50556=CARTESIAN_POINT('Ctrl Pts',(-0.297145802414634,2.22476258379937,
6.49177590738404));
#50557=CARTESIAN_POINT('Ctrl Pts',(-0.296797891151552,2.22558837668843,
6.49172082201667));
#50558=CARTESIAN_POINT('Ctrl Pts',(-0.296601547063761,2.22605138169038,
6.49168986926025));
#50559=CARTESIAN_POINT('Ctrl Pts',(-0.295999851158662,2.22746106958395,
6.49159542179813));
#50560=CARTESIAN_POINT('Ctrl Pts',(-0.295591047716872,2.22840626392683,
6.49153180952966));
#50561=CARTESIAN_POINT('Ctrl Pts',(-0.292594228172048,2.23524505768283,
6.49106945889191));
#50562=CARTESIAN_POINT('Ctrl Pts',(-0.289834848081017,2.24106154398097,
6.49066486721432));
#50563=CARTESIAN_POINT('Ctrl Pts',(-0.286125349130607,2.24831175802512,
6.49014545875881));
#50564=CARTESIAN_POINT('Ctrl Pts',(-0.285335305315419,2.24982608701353,
6.49003612210623));
#50565=CARTESIAN_POINT('Ctrl Pts',(-0.2835144315212,2.2532496338463,6.48978699802224));
#50566=CARTESIAN_POINT('Ctrl Pts',(-0.282476290661486,2.25515485175525,
6.48964697498925));
#50567=CARTESIAN_POINT('Ctrl Pts',(-0.2677530676533,2.28153759911828,6.48768865786246));
#50568=CARTESIAN_POINT('Ctrl Pts',(-0.250950017996872,2.30413538369285,
6.48576277429686));
#50569=CARTESIAN_POINT('Ctrl Pts',(-0.225800962349839,2.33008861624592,
6.48334496710722));
#50570=CARTESIAN_POINT('Ctrl Pts',(-0.219943703483876,2.3356939382323,6.48280894383016));
#50571=CARTESIAN_POINT('Ctrl Pts',(-0.211651583520814,2.34305074571383,
6.48209278810084));
#50572=CARTESIAN_POINT('Ctrl Pts',(-0.2093947969536,2.34499771068934,6.48190196452543));
#50573=CARTESIAN_POINT('Ctrl Pts',(-0.20625844784051,2.34762848635439,6.48164269728681));
#50574=CARTESIAN_POINT('Ctrl Pts',(-0.20540194377157,2.34833939707171,6.48157248912644));
#50575=CARTESIAN_POINT('Ctrl Pts',(-0.203933791101918,2.34954519314751,
6.48145318042146));
#50576=CARTESIAN_POINT('Ctrl Pts',(-0.203323988830277,2.35004229676827,
6.48140392726026));
#50577=CARTESIAN_POINT('Ctrl Pts',(-0.202464492465143,2.35073772468319,
6.48133493731194));
#50578=CARTESIAN_POINT('Ctrl Pts',(-0.202216321377405,2.35093791395315,
6.48131506734327));
#50579=CARTESIAN_POINT('Ctrl Pts',(-0.20180856549008,2.35126583592247,6.48128250298456));
#50580=CARTESIAN_POINT('Ctrl Pts',(-0.201649156285479,2.35139378508009,
6.48126979291162));
#50581=CARTESIAN_POINT('Ctrl Pts',(-0.20131603602293,2.35166064200735,6.48124327588829));
#50582=CARTESIAN_POINT('Ctrl Pts',(-0.201142302867778,2.35179952162991,
6.48122947102099));
#50583=CARTESIAN_POINT('Ctrl Pts',(-0.200759863460464,2.352104589456,6.48119913610942));
#50584=CARTESIAN_POINT('Ctrl Pts',(-0.200551093888112,2.3522706989385,6.48118261176222));
#50585=CARTESIAN_POINT('Ctrl Pts',(-0.199825873323962,2.35284625831607,
6.48112533067243));
#50586=CARTESIAN_POINT('Ctrl Pts',(-0.199308368275348,2.35325438663055,
6.48108466831767));
#50587=CARTESIAN_POINT('Ctrl Pts',(-0.194190853107202,2.3572648932811,6.48068461575392));
#50588=CARTESIAN_POINT('Ctrl Pts',(-0.189494583313289,2.36074341045987,
6.48033378367909));
#50589=CARTESIAN_POINT('Ctrl Pts',(-0.18447679041442,2.36425284793337,6.47997265898156));
#50590=CARTESIAN_POINT('Ctrl Pts',(-0.18424739863405,2.36441283996816,6.47995617935902));
#50591=CARTESIAN_POINT('Ctrl Pts',(-0.175526387870635,2.37047855350393,
6.47933076280088));
#50592=CARTESIAN_POINT('Ctrl Pts',(-0.166754906978743,2.37597281329973,
6.47874137675951));
#50593=CARTESIAN_POINT('Ctrl Pts',(-0.151404828794657,2.38458817026186,
6.47774971628733));
#50594=CARTESIAN_POINT('Ctrl Pts',(-0.144957628901577,2.38792557628404,
6.47734441041212));
#50595=CARTESIAN_POINT('Ctrl Pts',(-0.123511210229985,2.39812426725498,
6.47601701437642));
#50596=CARTESIAN_POINT('Ctrl Pts',(-0.108098394190558,2.40405226722575,
6.47509403400635));
#50597=CARTESIAN_POINT('Ctrl Pts',(-0.0841368473669129,2.41121499016093,
6.47364181076376));
#50598=CARTESIAN_POINT('Ctrl Pts',(-0.0758800500399938,2.41333046198254,
6.47313873599704));
#50599=CARTESIAN_POINT('Ctrl Pts',(-0.065080345361436,2.41564553192866,
6.4724727765412));
#50600=CARTESIAN_POINT('Ctrl Pts',(-0.0626049803084835,2.41614580348251,
6.4723196109083));
#50601=CARTESIAN_POINT('Ctrl Pts',(-0.0594214273306145,2.41675034502254,
6.47212187386891));
#50602=CARTESIAN_POINT('Ctrl Pts',(-0.0587183723840552,2.41688142865982,
6.47207815888319));
#50603=CARTESIAN_POINT('Ctrl Pts',(-0.0575864055162117,2.41708858584607,
6.47200769746833));
#50604=CARTESIAN_POINT('Ctrl Pts',(-0.0571577627961288,2.41716613237124,
6.47198099798796));
#50605=CARTESIAN_POINT('Ctrl Pts',(-0.0563420881641146,2.41731199029763,
6.47193015652836));
#50606=CARTESIAN_POINT('Ctrl Pts',(-0.0559550856398134,2.41738046328375,
6.47190601973988));
#50607=CARTESIAN_POINT('Ctrl Pts',(-0.0550738918905029,2.41753471249628,
6.47185102706832));
#50608=CARTESIAN_POINT('Ctrl Pts',(-0.0545796246052274,2.41762004310414,
6.47182015707875));
#50609=CARTESIAN_POINT('Ctrl Pts',(-0.0531099387033823,2.4178702387132,
6.4717282931277));
#50610=CARTESIAN_POINT('Ctrl Pts',(-0.0521339646449518,2.41803176562116,
6.47166719333083));
#50611=CARTESIAN_POINT('Ctrl Pts',(-0.0453603506710568,2.41912080335949,
6.47124245674088));
#50612=CARTESIAN_POINT('Ctrl Pts',(-0.039539377326593,2.41989416823157,
6.47087396350974));
#50613=CARTESIAN_POINT('Ctrl Pts',(-0.0320972914708534,2.42067668959275,
6.47039798598908));
#50614=CARTESIAN_POINT('Ctrl Pts',(-0.0304925402671953,2.42083325919869,
6.47029506547638));
#50615=CARTESIAN_POINT('Ctrl Pts',(-0.00503455224490297,2.42312437534797,
6.46865778193836));
#50616=CARTESIAN_POINT('Ctrl Pts',(0.0189791195497994,2.42260524840724,
6.4670418216056));
#50617=CARTESIAN_POINT('Ctrl Pts',(0.0533982698818474,2.41800330445526,
6.46469280613183));
#50618=CARTESIAN_POINT('Ctrl Pts',(0.0640095259891257,2.41603841596354,
6.46396537252836));
#50619=CARTESIAN_POINT('Ctrl Pts',(0.0803395995316524,2.41215816008537,
6.46285722129163));
#50620=CARTESIAN_POINT('Ctrl Pts',(0.0861370094362089,2.41060842480609,
6.46246615024676));
#50621=CARTESIAN_POINT('Ctrl Pts',(0.0936712751173715,2.40836719794631,
6.46196386841972));
#50622=CARTESIAN_POINT('Ctrl Pts',(0.0954498318041072,2.40782132241288,
6.4618457402919));
#50623=CARTESIAN_POINT('Ctrl Pts',(0.0979746948723314,2.40702240211754,
6.46167877253147));
#50624=CARTESIAN_POINT('Ctrl Pts',(0.0987249161520031,2.40678198643061,
6.46162925285656));
#50625=CARTESIAN_POINT('Ctrl Pts',(0.100041727193081,2.40635467089282,6.46154250567203));
#50626=CARTESIAN_POINT('Ctrl Pts',(0.100608689968227,2.40616894531293,6.46150521197922));
#50627=CARTESIAN_POINT('Ctrl Pts',(0.101444892264135,2.40589244871556,6.46145029433889));
#50628=CARTESIAN_POINT('Ctrl Pts',(0.101714528609893,2.40580289570055,6.46143259919309));
#50629=CARTESIAN_POINT('Ctrl Pts',(0.102182880734432,2.40564665619653,6.46140188658492));
#50630=CARTESIAN_POINT('Ctrl Pts',(0.102381650135989,2.40558013233155,6.46138885946049));
#50631=CARTESIAN_POINT('Ctrl Pts',(0.102778272056816,2.40544696103385,6.4613628801426));
#50632=CARTESIAN_POINT('Ctrl Pts',(0.102976124204597,2.40538031543671,6.46134992788447));
#50633=CARTESIAN_POINT('Ctrl Pts',(0.103451033522702,2.40521983037496,6.4613188555992));
#50634=CARTESIAN_POINT('Ctrl Pts',(0.103728028562485,2.4051258056657,6.46130074659236));
#50635=CARTESIAN_POINT('Ctrl Pts',(0.104731721777431,2.40478358185627,6.46123517860861));
#50636=CARTESIAN_POINT('Ctrl Pts',(0.105457667747819,2.40453316019308,6.46118785025016));
#50637=CARTESIAN_POINT('Ctrl Pts',(0.118774015255495,2.39988623847911,6.4603213181985));
#50638=CARTESIAN_POINT('Ctrl Pts',(0.131082250697227,2.3947143772435,6.45954705233825));
#50639=CARTESIAN_POINT('Ctrl Pts',(0.150001398865264,2.38534395801593,6.45834743941981));
#50640=CARTESIAN_POINT('Ctrl Pts',(0.156839893794392,2.38164312183618,6.45791176460744));
#50641=CARTESIAN_POINT('Ctrl Pts',(0.17600601978327,2.37035609647484,6.4566677193847));
#50642=CARTESIAN_POINT('Ctrl Pts',(0.187965092694424,2.36218245694159,6.45586235071449));
#50643=CARTESIAN_POINT('Ctrl Pts',(0.210828236076154,2.34418559972121,6.45419992600459));
#50644=CARTESIAN_POINT('Ctrl Pts',(0.221691605684149,2.33436701470591,6.4533442289927));
#50645=CARTESIAN_POINT('Ctrl Pts',(0.232718862428239,2.32294544660744,6.45237948023086));
#50646=CARTESIAN_POINT('Ctrl Pts',(0.233582651805598,2.3220402796776,6.45230322449737));
#50647=CARTESIAN_POINT('Ctrl Pts',(0.234814839582412,2.32073391982234,6.4521934472704));
#50648=CARTESIAN_POINT('Ctrl Pts',(0.235187533489121,2.3203367793488,6.4521601107745));
#50649=CARTESIAN_POINT('Ctrl Pts',(0.235831879751446,2.31964667022975,6.45210224407062));
#50650=CARTESIAN_POINT('Ctrl Pts',(0.236103998133837,2.31935413675837,6.45207773388347));
#50651=CARTESIAN_POINT('Ctrl Pts',(0.236625699030957,2.3187912009022,6.4520306041917));
#50652=CARTESIAN_POINT('Ctrl Pts',(0.23687536394108,2.31852087541046,6.4520079882547));
#50653=CARTESIAN_POINT('Ctrl Pts',(0.237461728223945,2.31788380188759,6.45195472683323));
#50654=CARTESIAN_POINT('Ctrl Pts',(0.237798041090985,2.31751670084144,6.45192406499543));
#50655=CARTESIAN_POINT('Ctrl Pts',(0.238786863962891,2.31643232079314,6.45183357720972));
#50656=CARTESIAN_POINT('Ctrl Pts',(0.239436984592098,2.31571287922061,6.45177365044802));
#50657=CARTESIAN_POINT('Ctrl Pts',(0.245103592139093,2.30938487503538,6.45124747350817));
#50658=CARTESIAN_POINT('Ctrl Pts',(0.249925100396565,2.30360556382501,6.45077314818341));
#50659=CARTESIAN_POINT('Ctrl Pts',(0.2561745967295,2.29555781066855,6.45012003526765));
#50660=CARTESIAN_POINT('Ctrl Pts',(0.257783316577663,2.29343226817753,6.44994821312508));
#50661=CARTESIAN_POINT('Ctrl Pts',(0.268732731424178,2.2785859954076,6.4487527531376));
#50662=CARTESIAN_POINT('Ctrl Pts',(0.277153410662394,2.26521539087319,6.44769796780946));
#50663=CARTESIAN_POINT('Ctrl Pts',(0.292006516322775,2.23727706702139,6.44556054302719));
#50664=CARTESIAN_POINT('Ctrl Pts',(0.298408762742111,2.22273973513529,6.44448080440771));
#50665=CARTESIAN_POINT('Ctrl Pts',(0.306201657860934,2.20078200736725,6.44294094298618));
#50666=CARTESIAN_POINT('Ctrl Pts',(0.30844565149192,2.19368974073746,6.44245705377273));
#50667=CARTESIAN_POINT('Ctrl Pts',(0.310751821596372,2.18541550831121,6.44191275565621));
#50668=CARTESIAN_POINT('Ctrl Pts',(0.31105527515164,2.18430373406987,6.44184003792293));
#50669=CARTESIAN_POINT('Ctrl Pts',(0.311495732869811,2.18265525261129,6.44173285732982));
#50670=CARTESIAN_POINT('Ctrl Pts',(0.311637323649435,2.18211979602763,6.44169814306428));
#50671=CARTESIAN_POINT('Ctrl Pts',(0.311891230656627,2.18114947675622,6.4416354203436));
#50672=CARTESIAN_POINT('Ctrl Pts',(0.312004019164279,2.18071474071982,6.44160738526735));
#50673=CARTESIAN_POINT('Ctrl Pts',(0.312178744652064,2.18003543378289,6.44156368427713));
#50674=CARTESIAN_POINT('Ctrl Pts',(0.312241303321947,2.17979102564959,6.44154798245798));
#50675=CARTESIAN_POINT('Ctrl Pts',(0.312352297791932,2.17935525599371,6.44152002516878));
#50676=CARTESIAN_POINT('Ctrl Pts',(0.312400844535814,2.17916392438202,6.44150776328692));
#50677=CARTESIAN_POINT('Ctrl Pts',(0.312511908507595,2.17872450774421,6.44147963266823));
#50678=CARTESIAN_POINT('Ctrl Pts',(0.312574306001454,2.17847639331306,6.44146377097749));
#50679=CARTESIAN_POINT('Ctrl Pts',(0.312744756837474,2.17779519223009,6.44142028256408));
#50680=CARTESIAN_POINT('Ctrl Pts',(0.312852206493233,2.17736195293195,6.44139269079699));
#50681=CARTESIAN_POINT('Ctrl Pts',(0.31337600675642,2.17523104042144,6.44125729990608));
#50682=CARTESIAN_POINT('Ctrl Pts',(0.313779451004771,2.17353018089215,6.4411502333291));
#50683=CARTESIAN_POINT('Ctrl Pts',(0.322172721522925,2.13681780770209,6.43885909545669));
#50684=CARTESIAN_POINT('Ctrl Pts',(0.324270547994527,2.10071170233846,6.43697061180949));
#50685=CARTESIAN_POINT('Ctrl Pts',(0.3190658519913,2.05307430468784,6.43421870425496));
#50686=CARTESIAN_POINT('Ctrl Pts',(0.317098679172003,2.04123421732518,6.43351545444353));
#50687=CARTESIAN_POINT('Ctrl Pts',(0.314017085343398,2.0274820025562,6.43266362593403));
#50688=CARTESIAN_POINT('Ctrl Pts',(0.313537656528364,2.02543642004531,6.43253601057297));
#50689=CARTESIAN_POINT('Ctrl Pts',(0.312879375934788,2.02274640081529,6.43236694271357));
#50690=CARTESIAN_POINT('Ctrl Pts',(0.312718463593273,2.02209759317205,6.43232606902748));
#50691=CARTESIAN_POINT('Ctrl Pts',(0.312451903445196,2.02103694261136,6.43225909099663));
#50692=CARTESIAN_POINT('Ctrl Pts',(0.312347456591276,2.02062479759457,6.43223302548911));
#50693=CARTESIAN_POINT('Ctrl Pts',(0.312144153118055,2.01982918160539,6.43218263140641));
#50694=CARTESIAN_POINT('Ctrl Pts',(0.312045404632114,2.01944568358178,6.43215830636888));
#50695=CARTESIAN_POINT('Ctrl Pts',(0.311816733873345,2.01856435166032,6.43210232449799));
#50696=CARTESIAN_POINT('Ctrl Pts',(0.31168632601449,2.01806664589657,6.43207065198851));
#50697=CARTESIAN_POINT('Ctrl Pts',(0.311279085370032,2.01652744167327,6.43197251945149));
#50698=CARTESIAN_POINT('Ctrl Pts',(0.310998222106825,2.01548702594509,6.4319059288978));
#50699=CARTESIAN_POINT('Ctrl Pts',(0.308619378795712,2.00684741570483,6.43135078062598));
#50700=CARTESIAN_POINT('Ctrl Pts',(0.30624859182181,1.99932672990657,6.43085337694266));
#50701=CARTESIAN_POINT('Ctrl Pts',(0.302544833359033,1.98892442792998,6.43014446820187));
#50702=CARTESIAN_POINT('Ctrl Pts',(0.301441327045913,1.98596367161763,6.42994027856186));
#50703=CARTESIAN_POINT('Ctrl Pts',(0.289729204402164,1.95589804664805,6.42784213712809));
#50704=CARTESIAN_POINT('Ctrl Pts',(0.27553841285741,1.93033407979231,6.42583467983948));
#50705=CARTESIAN_POINT('Ctrl Pts',(0.252410612194767,1.89939891360368,6.42326561523751));
#50706=CARTESIAN_POINT('Ctrl Pts',(0.246370783741228,1.89202551100613,6.42264255788634));
#50707=CARTESIAN_POINT('Ctrl Pts',(0.239388787016557,1.88423378888635,6.42198153092982));
#50708=CARTESIAN_POINT('Ctrl Pts',(0.238762010188218,1.88354041543885,6.42192268431332));
#50709=CARTESIAN_POINT('Ctrl Pts',(0.237812022163772,1.88249863550182,6.42183424717789));
#50710=CARTESIAN_POINT('Ctrl Pts',(0.237491048838352,1.88214820824095,6.42180449560569));
#50711=CARTESIAN_POINT('Ctrl Pts',(0.236969991577548,1.88158185659127,6.42175640783133));
#50712=CARTESIAN_POINT('Ctrl Pts',(0.236770386300256,1.88136549574404,6.42173803611027));
#50713=CARTESIAN_POINT('Ctrl Pts',(0.236387188681781,1.88095127138636,6.42170286201616));
#50714=CARTESIAN_POINT('Ctrl Pts',(0.236203643794556,1.88075336458777,6.42168605607586));
#50715=CARTESIAN_POINT('Ctrl Pts',(0.235873870837986,1.88039868251449,6.42165593637765));
#50716=CARTESIAN_POINT('Ctrl Pts',(0.235727735165243,1.88024182276808,6.42164261559855));
#50717=CARTESIAN_POINT('Ctrl Pts',(0.23541250002525,1.87990413054572,6.42161393787557));
#50718=CARTESIAN_POINT('Ctrl Pts',(0.235243349137294,1.87972334756804,6.42159858502973));
#50719=CARTESIAN_POINT('Ctrl Pts',(0.234785797049737,1.8792354588778,6.42155715015281));
#50720=CARTESIAN_POINT('Ctrl Pts',(0.234497000445035,1.87892872212735,6.4215310985218));
#50721=CARTESIAN_POINT('Ctrl Pts',(0.233209516047678,1.87756662028266,6.42141540193207));
#50722=CARTESIAN_POINT('Ctrl Pts',(0.232204279171961,1.87651742862455,6.42132625397931));
#50723=CARTESIAN_POINT('Ctrl Pts',(0.212037763859331,1.85575209211646,6.41956038104622));
#50724=CARTESIAN_POINT('Ctrl Pts',(0.190434914493815,1.83855755336527,6.41806487081776));
#50725=CARTESIAN_POINT('Ctrl Pts',(0.148069031379972,1.81290819384524,6.41528504843489));
#50726=CARTESIAN_POINT('Ctrl Pts',(0.128114465860215,1.80346567503014,6.41402550333459));
#50727=CARTESIAN_POINT('Ctrl Pts',(0.106273995211203,1.79574956375146,6.4126168923438));
#50728=CARTESIAN_POINT('Ctrl Pts',(0.105190986995312,1.79537343153075,6.41254698449813));
#50729=CARTESIAN_POINT('Ctrl Pts',(0.103608682969578,1.79483333638086,6.41244475381663));
#50730=CARTESIAN_POINT('Ctrl Pts',(0.103110948141975,1.79466480035996,6.41241258236234));
#50731=CARTESIAN_POINT('Ctrl Pts',(0.102237098729272,1.79437129004487,6.41235607607454));
#50732=CARTESIAN_POINT('Ctrl Pts',(0.101861160679929,1.79424579046548,6.41233175864732));
#50733=CARTESIAN_POINT('Ctrl Pts',(0.101131038889841,1.79400354957456,6.4122845152467));
#50734=CARTESIAN_POINT('Ctrl Pts',(0.100776881961416,1.79388672887274,6.41226159193578));
#50735=CARTESIAN_POINT('Ctrl Pts',(0.0999313076776484,1.7936094377871,6.41220684346942));
#50736=CARTESIAN_POINT('Ctrl Pts',(0.0994397065629825,1.79344953495224,
6.41217499967255));
#50737=CARTESIAN_POINT('Ctrl Pts',(0.0979533280768954,1.79297001305426,
6.41207867482322));
#50738=CARTESIAN_POINT('Ctrl Pts',(0.0969573863139982,1.7926540506804,6.41201407372568));
#50739=CARTESIAN_POINT('Ctrl Pts',(0.0864537241506893,1.78937790048161,
6.41133210771968));
#50740=CARTESIAN_POINT('Ctrl Pts',(0.0768161575802389,1.78685534040216,
6.41070049103915));
#50741=CARTESIAN_POINT('Ctrl Pts',(0.0432147845312039,1.77970497602335,
6.40847516740393));
#50742=CARTESIAN_POINT('Ctrl Pts',(0.0188544607156668,1.77735373049607,
6.40681451785875));
#50743=CARTESIAN_POINT('Ctrl Pts',(-0.0136818548719435,1.77791242859161,
6.40462002506499));
#50744=CARTESIAN_POINT('Ctrl Pts',(-0.0218227583717758,1.77836141819219,
6.40407378936623));
#50745=CARTESIAN_POINT('Ctrl Pts',(-0.0372070247184155,1.77979677079254,
6.40305602296137));
#50746=CARTESIAN_POINT('Ctrl Pts',(-0.0444513346089827,1.78072180071052,
6.40258294040968));
#50747=CARTESIAN_POINT('Ctrl Pts',(-0.0528487570085928,1.78208548568207,
6.40204645032855));
#50748=CARTESIAN_POINT('Ctrl Pts',(-0.0540378743147184,1.78228544606827,
6.40197076139817));
#50749=CARTESIAN_POINT('Ctrl Pts',(-0.0555968006123472,1.78255659851908,
6.40187192742467));
#50750=CARTESIAN_POINT('Ctrl Pts',(-0.0559676266981874,1.7826217680002,
6.4018484468026));
#50751=CARTESIAN_POINT('Ctrl Pts',(-0.0565722364219961,1.78272911554425,
6.4018102117882));
#50752=CARTESIAN_POINT('Ctrl Pts',(-0.0568060877925933,1.78277090226825,
6.40179543512127));
#50753=CARTESIAN_POINT('Ctrl Pts',(-0.0572577912522653,1.78285213230937,
6.40176691603119));
#50754=CARTESIAN_POINT('Ctrl Pts',(-0.0574756483474143,1.78289154144508,
6.40175317174224));
#50755=CARTESIAN_POINT('Ctrl Pts',(-0.057981157954074,1.78298352337026,
6.40172130394564));
#50756=CARTESIAN_POINT('Ctrl Pts',(-0.0582687806467032,1.78303626337387,
6.40170319002785));
#50757=CARTESIAN_POINT('Ctrl Pts',(-0.0592004356534144,1.78320840750382,
6.40164457365094));
#50758=CARTESIAN_POINT('Ctrl Pts',(-0.0598441811182826,1.78332938459364,
6.40160416048426));
#50759=CARTESIAN_POINT('Ctrl Pts',(-0.0660960446177321,1.78452402286641,
6.40121250573043));
#50760=CARTESIAN_POINT('Ctrl Pts',(-0.0716754831360531,1.78574466721573,
6.40086943519134));
#50761=CARTESIAN_POINT('Ctrl Pts',(-0.0783162065420704,1.78738358582074,
6.40046569052639));
#50762=CARTESIAN_POINT('Ctrl Pts',(-0.0794110545744859,1.78765990476213,
6.40039927628031));
#50763=CARTESIAN_POINT('Ctrl Pts',(-0.110914987317835,1.79578726019632,
6.39849198513312));
#50764=CARTESIAN_POINT('Ctrl Pts',(-0.140017630672197,1.80803591730383,
6.39681510435875));
#50765=CARTESIAN_POINT('Ctrl Pts',(-0.176445759980808,1.83008737510312,
6.39436148348804));
#50766=CARTESIAN_POINT('Ctrl Pts',(-0.185692775037244,1.83636372811502,
6.39370477741718));
#50767=CARTESIAN_POINT('Ctrl Pts',(-0.196197495324445,1.84432097985333,
6.39290782572882));
#50768=CARTESIAN_POINT('Ctrl Pts',(-0.197788841202085,1.84555001959808,
6.39278565573822));
#50769=CARTESIAN_POINT('Ctrl Pts',(-0.199885105265159,1.84720056850615,
6.39262275541329));
#50770=CARTESIAN_POINT('Ctrl Pts',(-0.200400407015625,1.84760886559082,
6.3925825517828));
#50771=CARTESIAN_POINT('Ctrl Pts',(-0.201244982773947,1.84828227865517,
6.39251639385029));
#50772=CARTESIAN_POINT('Ctrl Pts',(-0.201574992636699,1.84854647214339,
6.39249047655854));
#50773=CARTESIAN_POINT('Ctrl Pts',(-0.202213892193419,1.84906001709925,
6.39244017060201));
#50774=CARTESIAN_POINT('Ctrl Pts',(-0.202522843000473,1.84930929160616,
6.39241578506164));
#50775=CARTESIAN_POINT('Ctrl Pts',(-0.203235752530189,1.84988667497086,
6.39235937744638));
#50776=CARTESIAN_POINT('Ctrl Pts',(-0.203639377825494,1.85021519210044,
6.39232733891551));
#50777=CARTESIAN_POINT('Ctrl Pts',(-0.204720997214866,1.85109990366835,
6.39224120657079));
#50778=CARTESIAN_POINT('Ctrl Pts',(-0.205397516209399,1.85165788724983,
6.39218704025213));
#50779=CARTESIAN_POINT('Ctrl Pts',(-0.210202059126783,1.85565366990804,
6.39180024885751));
#50780=CARTESIAN_POINT('Ctrl Pts',(-0.214245623151399,1.85919127499756,
6.39146355010964));
#50781=CARTESIAN_POINT('Ctrl Pts',(-0.218658434380346,1.86325107192618,
6.39108306711187));
#50782=CARTESIAN_POINT('Ctrl Pts',(-0.219116933460809,1.86367536029479,
6.39104337295234));
#50783=CARTESIAN_POINT('Ctrl Pts',(-0.221004000953644,1.86543183777833,
6.39087933353415));
#50784=CARTESIAN_POINT('Ctrl Pts',(-0.222421653920957,1.86677564713456,
6.39075451176141));
#50785=CARTESIAN_POINT('Ctrl Pts',(-0.226398825430387,1.87061489704599,
6.39039978941472));
#50786=CARTESIAN_POINT('Ctrl Pts',(-0.228929106863807,1.87314009584905,
6.39016869218125));
#50787=CARTESIAN_POINT('Ctrl Pts',(-0.232813196038101,1.87714754406849,
6.3898053799369));
#50788=CARTESIAN_POINT('Ctrl Pts',(-0.234196096327211,1.87860128822133,
6.38967426757451));
#50789=CARTESIAN_POINT('Ctrl Pts',(-0.252435623848281,1.89813731121435,
6.38792149041848));
#50790=CARTESIAN_POINT('Ctrl Pts',(-0.267169934448722,1.91808716056105,
6.38622603546088));
#50791=CARTESIAN_POINT('Ctrl Pts',(-0.283870766547797,1.94717197893642,
6.38398110724936));
#50792=CARTESIAN_POINT('Ctrl Pts',(-0.287948435399427,1.95500089705326,
6.38339766794261));
#50793=CARTESIAN_POINT('Ctrl Pts',(-0.293371144050865,1.9665458887325,6.38257633250866));
#50794=CARTESIAN_POINT('Ctrl Pts',(-0.29497720647738,1.97013438056736,6.38232630887702));
#50795=CARTESIAN_POINT('Ctrl Pts',(-0.29672909443182,1.97424900613177,6.38204631038258));
#50796=CARTESIAN_POINT('Ctrl Pts',(-0.296939644058674,1.97474699309961,
6.38201253285904));
#50797=CARTESIAN_POINT('Ctrl Pts',(-0.297254733445657,1.97549749497851,
6.38196179616467));
#50798=CARTESIAN_POINT('Ctrl Pts',(-0.297360205501846,1.97574961369193,
6.3819447805662));
#50799=CARTESIAN_POINT('Ctrl Pts',(-0.297549354402469,1.97620337250346,
6.38191420793582));
#50800=CARTESIAN_POINT('Ctrl Pts',(-0.297633146883127,1.97640496303552,
6.38190064386266));
#50801=CARTESIAN_POINT('Ctrl Pts',(-0.297812644013417,1.97683804387409,
6.38187154339523));
#50802=CARTESIAN_POINT('Ctrl Pts',(-0.297908283341287,1.97706955995891,
6.38185601103669));
#50803=CARTESIAN_POINT('Ctrl Pts',(-0.298164842522028,1.97769267579839,
6.38181427067643));
#50804=CARTESIAN_POINT('Ctrl Pts',(-0.298325261497764,1.97808448324068,
6.38178809313983));
#50805=CARTESIAN_POINT('Ctrl Pts',(-0.299057220305958,1.97988231537185,
6.38166828372946));
#50806=CARTESIAN_POINT('Ctrl Pts',(-0.299619607448771,1.981292080205,6.38157519757541));
#50807=CARTESIAN_POINT('Ctrl Pts',(-0.311833799180416,2.01254988000695,
6.37952915335565));
#50808=CARTESIAN_POINT('Ctrl Pts',(-0.31898197133815,2.04397181165803,6.37781852027982));
#50809=CARTESIAN_POINT('Ctrl Pts',(-0.32197094173668,2.08389069771,6.37554919832595));
#50810=CARTESIAN_POINT('Ctrl Pts',(-0.322270983047103,2.09186371415243,
6.3750922213039));
#50811=CARTESIAN_POINT('Ctrl Pts',(-0.322279658999331,2.10926320332244,
6.37407818456919));
#50812=CARTESIAN_POINT('Ctrl Pts',(-0.321871004133448,2.11868196904564,
6.37351846291403));
#50813=CARTESIAN_POINT('Ctrl Pts',(-0.320950643579636,2.12920908232873,
6.37287583992183));
#50814=CARTESIAN_POINT('Ctrl Pts',(-0.320844865489146,2.13034894299608,
6.37280603558363));
#50815=CARTESIAN_POINT('Ctrl Pts',(-0.320682259757542,2.13200521485414,
6.3727042757247));
#50816=CARTESIAN_POINT('Ctrl Pts',(-0.320630252085865,2.13252209930841,
6.37267247192477));
#50817=CARTESIAN_POINT('Ctrl Pts',(-0.320536314002029,2.13343358338143,
6.37261630494672));
#50818=CARTESIAN_POINT('Ctrl Pts',(-0.320494904022522,2.13382823650577,
6.37259195820381));
#50819=CARTESIAN_POINT('Ctrl Pts',(-0.320407835250848,2.13464352397203,
6.37254160435922));
#50820=CARTESIAN_POINT('Ctrl Pts',(-0.320362076807994,2.13506414670125,
6.37251559416221));
#50821=CARTESIAN_POINT('Ctrl Pts',(-0.320242916052121,2.13613979511352,
6.37244899730391));
#50822=CARTESIAN_POINT('Ctrl Pts',(-0.320168332558716,2.13679468560369,
6.3724083734769));
#50823=CARTESIAN_POINT('Ctrl Pts',(-0.3198565238103,2.13945981690589,6.37224273265895));
#50824=CARTESIAN_POINT('Ctrl Pts',(-0.319602374762253,2.14146799633634,
6.3721171829437));
#50825=CARTESIAN_POINT('Ctrl Pts',(-0.315139226506289,2.1742514267203,6.37005515926047));
#50826=CARTESIAN_POINT('Ctrl Pts',(-0.30652227252851,2.20425532833066,6.36796452482249));
#50827=CARTESIAN_POINT('Ctrl Pts',(-0.287706828389105,2.24595206613429,
6.36487206179435));
#50828=CARTESIAN_POINT('Ctrl Pts',(-0.280751059027885,2.25892183637936,
6.36388439727701));
#50829=CARTESIAN_POINT('Ctrl Pts',(-0.270935901922103,2.27455378561885,
6.36269663883162));
#50830=CARTESIAN_POINT('Ctrl Pts',(-0.268882762962979,2.27770016838185,
6.36245776004872));
#50831=CARTESIAN_POINT('Ctrl Pts',(-0.266447994067274,2.28129253084408,
6.3621859000184));
#50832=CARTESIAN_POINT('Ctrl Pts',(-0.266119706461407,2.28177408266266,
6.36214947607037));
#50833=CARTESIAN_POINT('Ctrl Pts',(-0.265630751533016,2.28248714713907,
6.36209557159766));
#50834=CARTESIAN_POINT('Ctrl Pts',(-0.265471086269037,2.28271934048574,
6.36207802368417));
#50835=CARTESIAN_POINT('Ctrl Pts',(-0.265186701639432,2.28313174746536,
6.36204686528725));
#50836=CARTESIAN_POINT('Ctrl Pts',(-0.26506210303209,2.28331204323071,6.36203324659469));
#50837=CARTESIAN_POINT('Ctrl Pts',(-0.264797766878953,2.28369370799222,
6.36200442415109));
#50838=CARTESIAN_POINT('Ctrl Pts',(-0.264657983892939,2.28389504414937,
6.36198922362599));
#50839=CARTESIAN_POINT('Ctrl Pts',(-0.264283631773973,2.2844329305986,6.36194862406341));
#50840=CARTESIAN_POINT('Ctrl Pts',(-0.264048648522266,2.28476919421489,
6.36192325335017));
#50841=CARTESIAN_POINT('Ctrl Pts',(-0.262935523687632,2.28635562791608,
6.36180360319612));
#50842=CARTESIAN_POINT('Ctrl Pts',(-0.26204912287177,2.28760001890148,6.36170988098252));
#50843=CARTESIAN_POINT('Ctrl Pts',(-0.254759027443678,2.29768186609809,
6.36095121166694));
#50844=CARTESIAN_POINT('Ctrl Pts',(-0.247918305474229,2.30619614527469,
6.36031453124));
#50845=CARTESIAN_POINT('Ctrl Pts',(-0.221175995114525,2.33622095573845,
6.35801732521308));
#50846=CARTESIAN_POINT('Ctrl Pts',(-0.198803623089132,2.35533585936913,
6.35643548996213));
#50847=CARTESIAN_POINT('Ctrl Pts',(-0.166364232920986,2.37616999642665,
6.3541870180284));
#50848=CARTESIAN_POINT('Ctrl Pts',(-0.158361285235065,2.38083554485971,
6.35363676609995));
#50849=CARTESIAN_POINT('Ctrl Pts',(-0.149160794628448,2.38568082134411,
6.35300439204209));
#50850=CARTESIAN_POINT('Ctrl Pts',(-0.148149664534789,2.38620648347659,
6.35293490006585));
#50851=CARTESIAN_POINT('Ctrl Pts',(-0.146674435006571,2.38696350747775,
6.35283351235944));
#50852=CARTESIAN_POINT('Ctrl Pts',(-0.146212523763191,2.38719913370041,
6.35280176677961));
#50853=CARTESIAN_POINT('Ctrl Pts',(-0.145396268924729,2.38761303508169,
6.3527456676773));
#50854=CARTESIAN_POINT('Ctrl Pts',(-0.145042160231166,2.38779177319614,
6.35272133046359));
#50855=CARTESIAN_POINT('Ctrl Pts',(-0.144309311028023,2.38815998632901,
6.35267096224757));
#50856=CARTESIAN_POINT('Ctrl Pts',(-0.143930525399679,2.38834936938715,
6.35264492808395));
#50857=CARTESIAN_POINT('Ctrl Pts',(-0.142959678225297,2.38883237834536,
6.35257819932122));
#50858=CARTESIAN_POINT('Ctrl Pts',(-0.142367086900955,2.38912492963399,
6.35253746726808));
#50859=CARTESIAN_POINT('Ctrl Pts',(-0.139943062903458,2.39031236580648,
6.35237084018093));
#50860=CARTESIAN_POINT('Ctrl Pts',(-0.138104090918512,2.39119167288872,
6.35224440438688));
#50861=CARTESIAN_POINT('Ctrl Pts',(-0.107779265025426,2.40533965737482,
6.35015871170442));
#50862=CARTESIAN_POINT('Ctrl Pts',(-0.0775173176241014,2.41438635670066,
6.34804123372469));
#50863=CARTESIAN_POINT('Ctrl Pts',(-0.0318070638249608,2.42104209142762,
6.3449195645139));
#50864=CARTESIAN_POINT('Ctrl Pts',(-0.0170475108066564,2.42216328814894,
6.34392744061303));
#50865=CARTESIAN_POINT('Ctrl Pts',(0.00106464553053257,2.42229040994249,
6.34276534014247));
#50866=CARTESIAN_POINT('Ctrl Pts',(0.00439147682843307,2.42226225171435,
6.34255420930228));
#50867=CARTESIAN_POINT('Ctrl Pts',(0.00827210163636751,2.42216929679074,
6.34231110418144));
#50868=CARTESIAN_POINT('Ctrl Pts',(0.00882674113468483,2.42215457797767,
6.34227643394949));
#50869=CARTESIAN_POINT('Ctrl Pts',(0.00966123643497917,2.42213027572916,
6.34222438670926));
#50870=CARTESIAN_POINT('Ctrl Pts',(0.00994111865508915,2.42212175988608,
6.34220695027683));
#50871=CARTESIAN_POINT('Ctrl Pts',(0.0104398380334422,2.42210593497981,
6.34217591608274));
#50872=CARTESIAN_POINT('Ctrl Pts',(0.0106586786929119,2.42209876767379,
6.34216231035613));
#50873=CARTESIAN_POINT('Ctrl Pts',(0.0111235123960802,2.42208306953528,
6.34213343689633));
#50874=CARTESIAN_POINT('Ctrl Pts',(0.0113695023111731,2.4220744799382,6.34211817254844));
#50875=CARTESIAN_POINT('Ctrl Pts',(0.0120300751653904,2.42205065599475,
6.34207722319629));
#50876=CARTESIAN_POINT('Ctrl Pts',(0.0124446406956274,2.4220349028563,6.34205156737804));
#50877=CARTESIAN_POINT('Ctrl Pts',(0.0144357563873208,2.42195539151796,
6.34192854854323));
#50878=CARTESIAN_POINT('Ctrl Pts',(0.0160118895148559,2.42188085501084,
6.34183178158524));
#50879=CARTESIAN_POINT('Ctrl Pts',(0.0291487266945746,2.42116287107689,
6.34102988192683));
#50880=CARTESIAN_POINT('Ctrl Pts',(0.0406689722397397,2.41990832425369,
6.34035652100778));
#50881=CARTESIAN_POINT('Ctrl Pts',(0.0712823096949903,2.41489351435652,
6.3385890888098));
#50882=CARTESIAN_POINT('Ctrl Pts',(0.0901433877386156,2.41002147007769,
6.3375213288434));
#50883=CARTESIAN_POINT('Ctrl Pts',(0.125510873020275,2.3973825942262,6.33539743380953));
#50884=CARTESIAN_POINT('Ctrl Pts',(0.142023863982611,2.38985938489501,6.33434915493812));
#50885=CARTESIAN_POINT('Ctrl Pts',(0.158935555980923,2.3803610406494,6.33317096256294));
#50886=CARTESIAN_POINT('Ctrl Pts',(0.160051216314129,2.3797256372784,6.33309273768266));
#50887=CARTESIAN_POINT('Ctrl Pts',(0.161603927162409,2.37882898980609,6.33298315770425));
#50888=CARTESIAN_POINT('Ctrl Pts',(0.162044210829552,2.37857334503238,6.33295200507567));
#50889=CARTESIAN_POINT('Ctrl Pts',(0.162804168625354,2.37812967451918,6.3328980938153));
#50890=CARTESIAN_POINT('Ctrl Pts',(0.163124128291243,2.37794213775046,6.3328753529502));
#50891=CARTESIAN_POINT('Ctrl Pts',(0.163786368400199,2.37755244400827,6.33282819529313));
#50892=CARTESIAN_POINT('Ctrl Pts',(0.164128599818109,2.37735020527886,6.33280377555355));
#50893=CARTESIAN_POINT('Ctrl Pts',(0.164919533580994,2.37688083314492,6.33274722338193));
#50894=CARTESIAN_POINT('Ctrl Pts',(0.165367961644774,2.37661324186656,6.33271507428852));
#50895=CARTESIAN_POINT('Ctrl Pts',(0.166793355891906,2.37575795890948,6.33261260737066));
#50896=CARTESIAN_POINT('Ctrl Pts',(0.167767846575844,2.3751661771973,6.33254214002349));
#50897=CARTESIAN_POINT('Ctrl Pts',(0.170026989353347,2.37377779929526,6.3323778007028));
#50898=CARTESIAN_POINT('Ctrl Pts',(0.171309209826656,2.37297731590511,6.33228378641074));
#50899=CARTESIAN_POINT('Ctrl Pts',(0.184215586495756,2.36479318809067,6.33132987479509));
#50900=CARTESIAN_POINT('Ctrl Pts',(0.195359216269885,2.35668171262402,6.33044265522849));
#50901=CARTESIAN_POINT('Ctrl Pts',(0.223245723064859,2.33351278602647,6.3280488289331));
#50902=CARTESIAN_POINT('Ctrl Pts',(0.238990301411144,2.31737149432935,6.32650854239552));
#50903=CARTESIAN_POINT('Ctrl Pts',(0.258078878926114,2.29319843079551,6.324445706739));
#50904=CARTESIAN_POINT('Ctrl Pts',(0.262978786223548,2.28647391164881,6.32389487193158));
#50905=CARTESIAN_POINT('Ctrl Pts',(0.267744127801934,2.27937199541742,6.32334175700654));
#50906=CARTESIAN_POINT('Ctrl Pts',(0.267874690604353,2.27917695400555,6.32332658834258));
#50907=CARTESIAN_POINT('Ctrl Pts',(0.27039753737059,2.27539927513003,6.3230332138234));
#50908=CARTESIAN_POINT('Ctrl Pts',(0.272718109649788,2.2717689468539,6.32275860573346));
#50909=CARTESIAN_POINT('Ctrl Pts',(0.275250172934361,2.26762701504709,6.32245440266168));
#50910=CARTESIAN_POINT('Ctrl Pts',(0.27553383806854,2.26716033609556,6.32242025581485));
#50911=CARTESIAN_POINT('Ctrl Pts',(0.275960449211904,2.26645444945866,6.32236880226892));
#50912=CARTESIAN_POINT('Ctrl Pts',(0.276104271713305,2.26621577667878,6.32235143866574));
#50913=CARTESIAN_POINT('Ctrl Pts',(0.276353433279654,2.26580107846497,6.32232132806152));
#50914=CARTESIAN_POINT('Ctrl Pts',(0.276458913862855,2.26562513894909,6.32230857175316));
#50915=CARTESIAN_POINT('Ctrl Pts',(0.276679114865641,2.26525705159953,6.32228192260095));
#50916=CARTESIAN_POINT('Ctrl Pts',(0.276793803064095,2.2650648850963,6.32226803193974));
#50917=CARTESIAN_POINT('Ctrl Pts',(0.277067545918565,2.26460512606663,6.32223485068834));
#50918=CARTESIAN_POINT('Ctrl Pts',(0.277226413758572,2.26433742131742,6.32221557239331));
#50919=CARTESIAN_POINT('Ctrl Pts',(0.277763292041226,2.26342974536991,6.32215034909471));
#50920=CARTESIAN_POINT('Ctrl Pts',(0.278139479927671,2.26278869066561,6.3221045223025));
#50921=CARTESIAN_POINT('Ctrl Pts',(0.279029007384789,2.26126077845419,6.32199584751489));
#50922=CARTESIAN_POINT('Ctrl Pts',(0.279540345199131,2.2603727567268,6.32193312466767));
#50923=CARTESIAN_POINT('Ctrl Pts',(0.285609502903421,2.24971544777673,6.32118542955653));
#50924=CARTESIAN_POINT('Ctrl Pts',(0.290657480614463,2.23966313388838,6.32053074067335));
#50925=CARTESIAN_POINT('Ctrl Pts',(0.307691021756868,2.20079839090929,6.31810972396772));
#50926=CARTESIAN_POINT('Ctrl Pts',(0.315998018233188,2.17056521578605,6.31642829071561));
#50927=CARTESIAN_POINT('Ctrl Pts',(0.320708489629304,2.13252888794293,6.31417160182846));
#50928=CARTESIAN_POINT('Ctrl Pts',(0.321349871299121,2.12542267143638,6.31374510675447));
#50929=CARTESIAN_POINT('Ctrl Pts',(0.321815184075115,2.1172420641479,6.3132465153317));
#50930=CARTESIAN_POINT('Ctrl Pts',(0.321870207197683,2.11618243349123,6.31318178806824));
#50931=CARTESIAN_POINT('Ctrl Pts',(0.321943628742833,2.11461947965904,6.31308609547695));
#50932=CARTESIAN_POINT('Ctrl Pts',(0.321966082106739,2.1141163466198,6.31305525732445));
#50933=CARTESIAN_POINT('Ctrl Pts',(0.322004014199881,2.11321915231268,6.31300020562241));
#50934=CARTESIAN_POINT('Ctrl Pts',(0.32201994920617,2.11282511051667,6.31297600642531));
#50935=CARTESIAN_POINT('Ctrl Pts',(0.322049286528548,2.11206510588908,6.31292929184389));
#50936=CARTESIAN_POINT('Ctrl Pts',(0.32206278841824,2.11169914732651,6.31290677961988));
#50937=CARTESIAN_POINT('Ctrl Pts',(0.322097425426804,2.11071480315456,6.31284617771041));
#50938=CARTESIAN_POINT('Ctrl Pts',(0.322117403383106,2.11009638065918,6.31280805181309));
#50939=CARTESIAN_POINT('Ctrl Pts',(0.322186462863438,2.10774918364025,6.3126631456919));
#50940=CARTESIAN_POINT('Ctrl Pts',(0.322223408273475,2.10602010572221,6.31255598599726));
#50941=CARTESIAN_POINT('Ctrl Pts',(0.322363696864557,2.09548429232617,6.31190042859222));
#50942=CARTESIAN_POINT('Ctrl Pts',(0.322119898456523,2.08667741254037,6.31134122847299));
#50943=CARTESIAN_POINT('Ctrl Pts',(0.320150950356518,2.05804280162445,6.30948458001554));
#50944=CARTESIAN_POINT('Ctrl Pts',(0.316951020075525,2.03836479888312,6.30814505236117));
#50945=CARTESIAN_POINT('Ctrl Pts',(0.308328024362657,2.0051095425196,6.30582013776111));
#50946=CARTESIAN_POINT('Ctrl Pts',(0.30375910474414,1.99136838009444,6.30484155112728));
#50947=CARTESIAN_POINT('Ctrl Pts',(0.297808557870049,1.97682206575994,6.30381345685935));
#50948=CARTESIAN_POINT('Ctrl Pts',(0.2973281587744,1.97566695245521,6.30373187800446));
#50949=CARTESIAN_POINT('Ctrl Pts',(0.296446460770463,1.97358125757994,6.30358472483933));
#50950=CARTESIAN_POINT('Ctrl Pts',(0.296047477301656,1.97264972017492,6.30351905506936));
#50951=CARTESIAN_POINT('Ctrl Pts',(0.293905142099454,1.96771232457915,6.30317132926428));
#50952=CARTESIAN_POINT('Ctrl Pts',(0.292084759526937,1.96374010289443,6.30289277112668));
#50953=CARTESIAN_POINT('Ctrl Pts',(0.289922542997893,1.95926458837135,6.30258129785063));
#50954=CARTESIAN_POINT('Ctrl Pts',(0.289659511150677,1.95872401252002,6.30254371653472));
#50955=CARTESIAN_POINT('Ctrl Pts',(0.289268851825449,1.95792681771759,6.30248835755455));
#50956=CARTESIAN_POINT('Ctrl Pts',(0.289142394115857,1.95766963188854,6.30247050766336));
#50957=CARTESIAN_POINT('Ctrl Pts',(0.288918054098805,1.95721490889505,6.30243896534237));
#50958=CARTESIAN_POINT('Ctrl Pts',(0.288820312056765,1.95701730324721,6.30242526411675));
#50959=CARTESIAN_POINT('Ctrl Pts',(0.288615680003369,1.95660466344608,6.30239666572005));
#50960=CARTESIAN_POINT('Ctrl Pts',(0.288508752644802,1.9563896489195,6.30238177097953));
#50961=CARTESIAN_POINT('Ctrl Pts',(0.288228404409888,1.95582748840154,6.30234284625592));
#50962=CARTESIAN_POINT('Ctrl Pts',(0.288054596023228,1.95548053444977,6.30231884061697));
#50963=CARTESIAN_POINT('Ctrl Pts',(0.287292092145774,1.95396527499257,6.30221407492678));
#50964=CARTESIAN_POINT('Ctrl Pts',(0.286696901818601,1.95280022505996,6.30213371714956));
#50965=CARTESIAN_POINT('Ctrl Pts',(0.282244268729266,1.94421392047236,6.30154269059245));
#50966=CARTESIAN_POINT('Ctrl Pts',(0.278105951896118,1.93694100376658,6.301048716059));
#50967=CARTESIAN_POINT('Ctrl Pts',(0.259022180913485,1.90624685825345,6.29895737526667));
#50968=CARTESIAN_POINT('Ctrl Pts',(0.241366732071269,1.88465122610918,6.29745883793543));
#50969=CARTESIAN_POINT('Ctrl Pts',(0.21782893338931,1.86244433573146,6.29560241270325));
#50970=CARTESIAN_POINT('Ctrl Pts',(0.214432224574083,1.85937382421525,6.29533769621932));
#50971=CARTESIAN_POINT('Ctrl Pts',(0.204159274414884,1.85047771662669,6.29454429144009));
#50972=CARTESIAN_POINT('Ctrl Pts',(0.197103332379081,1.84486742183,6.29400843946359));
#50973=CARTESIAN_POINT('Ctrl Pts',(0.18890758960432,1.83889393195384,6.29339164215806));
#50974=CARTESIAN_POINT('Ctrl Pts',(0.187989603426542,1.83823223053052,6.29332263500699));
#50975=CARTESIAN_POINT('Ctrl Pts',(0.186647132462481,1.83727525638094,6.29322182521874));
#50976=CARTESIAN_POINT('Ctrl Pts',(0.186225384851042,1.83697614367072,6.29319017031004));
#50977=CARTESIAN_POINT('Ctrl Pts',(0.185479018731242,1.83644949936867,6.29313417676769));
#50978=CARTESIAN_POINT('Ctrl Pts',(0.185154696019132,1.83622154880967,6.29310985424618));
#50979=CARTESIAN_POINT('Ctrl Pts',(0.184530086419158,1.83578426082886,6.29306302803668));
#50980=CARTESIAN_POINT('Ctrl Pts',(0.184229861668978,1.83557483537439,6.29304052776248));
#50981=CARTESIAN_POINT('Ctrl Pts',(0.183436256789134,1.83502325419877,6.29298106982739));
#50982=CARTESIAN_POINT('Ctrl Pts',(0.182942277871348,1.83468196616198,6.29294407919581));
#50983=CARTESIAN_POINT('Ctrl Pts',(0.181125874256248,1.8334345047443,6.29280812841259));
#50984=CARTESIAN_POINT('Ctrl Pts',(0.17979766399946,1.83253683345691,6.29270884676044));
#50985=CARTESIAN_POINT('Ctrl Pts',(0.176537858695669,1.83036894756828,6.29246547064173));
#50986=CARTESIAN_POINT('Ctrl Pts',(0.17459920962841,1.82910955067247,6.29232097637716));
#50987=CARTESIAN_POINT('Ctrl Pts',(0.16721998492646,1.82442793531935,6.29177180417491));
#50988=CARTESIAN_POINT('Ctrl Pts',(0.161691296857596,1.82114806559705,6.29136199151765));
#50989=CARTESIAN_POINT('Ctrl Pts',(0.142508366477141,1.81053021890289,6.2899450487336));
#50990=CARTESIAN_POINT('Ctrl Pts',(0.128425929393326,1.80401339499451,6.2889119709889));
#50991=CARTESIAN_POINT('Ctrl Pts',(0.0908525249739169,1.78981347864258,
6.28620148156929));
#50992=CARTESIAN_POINT('Ctrl Pts',(0.0668471699242258,1.7837698255814,6.28450966927148));
#50993=CARTESIAN_POINT('Ctrl Pts',(0.0410026721338429,1.78034095792689,
6.28286230561994));
#50994=CARTESIAN_POINT('Ctrl Pts',(0.0396183514507363,1.78016643594321,
6.2827746048338));
#50995=CARTESIAN_POINT('Ctrl Pts',(0.0378211073686939,1.77995170447906,
6.28266147937228));
#50996=CARTESIAN_POINT('Ctrl Pts',(0.0374092058753349,1.77990329750398,
6.28263560274289));
#50997=CARTESIAN_POINT('Ctrl Pts',(0.0367771312134968,1.77983025232553,
6.28259597225865));
#50998=CARTESIAN_POINT('Ctrl Pts',(0.0365570261324934,1.7798050460309,6.28258218637196));
#50999=CARTESIAN_POINT('Ctrl Pts',(0.0361203580484547,1.77975549520529,
6.28255486543507));
#51000=CARTESIAN_POINT('Ctrl Pts',(0.035903797691152,1.77973114352368,6.28254133011345));
#51001=CARTESIAN_POINT('Ctrl Pts',(0.0354215485262551,1.77967741107197,
6.28251122033203));
#51002=CARTESIAN_POINT('Ctrl Pts',(0.0351558484881496,1.77964814126359,
6.28249465225606));
#51003=CARTESIAN_POINT('Ctrl Pts',(0.0343812071433696,1.77956378126819,
6.2824464094988));
#51004=CARTESIAN_POINT('Ctrl Pts',(0.033872167628838,1.7795095727663,6.2824147845349));
#51005=CARTESIAN_POINT('Ctrl Pts',(0.0302327759318581,1.77913077536966,
6.28218921576922));
#51006=CARTESIAN_POINT('Ctrl Pts',(0.0270978084068554,1.77885082807592,
6.28199773791169));
#51007=CARTESIAN_POINT('Ctrl Pts',(0.0210770887529826,1.77840198364539,
6.28163455904428));
#51008=CARTESIAN_POINT('Ctrl Pts',(0.0181922143148818,1.77822589866855,
6.28146253871198));
#51009=CARTESIAN_POINT('Ctrl Pts',(0.00674542941357853,1.77768166170732,
6.28078654124249));
#51010=CARTESIAN_POINT('Ctrl Pts',(-0.00182783710657208,1.77761623644072,
6.28029471906875));
#51011=CARTESIAN_POINT('Ctrl Pts',(-0.0127601962555898,1.7779690115748,
6.2796749766125));
#51012=CARTESIAN_POINT('Ctrl Pts',(-0.0151254562761947,1.77807143507532,
6.27954134026152));
#51013=CARTESIAN_POINT('Ctrl Pts',(-0.035332817951963,1.77916967762503,
6.27840198635974));
#51014=CARTESIAN_POINT('Ctrl Pts',(-0.0530643443972307,1.78162180121795,
6.27741600552117));
#51015=CARTESIAN_POINT('Ctrl Pts',(-0.0764141372474246,1.78685662211536,
6.2760537143401));
#51016=CARTESIAN_POINT('Ctrl Pts',(-0.0822882659357707,1.78834870190204,
6.27570562767723));
#51017=CARTESIAN_POINT('Ctrl Pts',(-0.0975895275659313,1.79269811925516,
6.27478022025353));
#51018=CARTESIAN_POINT('Ctrl Pts',(-0.106933168102199,1.79582335785212,
6.27419601582167));
#51019=CARTESIAN_POINT('Ctrl Pts',(-0.117090421518247,1.79974661618089,
6.27353391246958));
#51020=CARTESIAN_POINT('Ctrl Pts',(-0.118060561102096,1.80012675147904,
6.27347039791165));
#51021=CARTESIAN_POINT('Ctrl Pts',(-0.119508559791905,1.80070224482395,
6.27337517888793));
#51022=CARTESIAN_POINT('Ctrl Pts',(-0.1199878272125,1.80089405985021,6.27334359376837));
#51023=CARTESIAN_POINT('Ctrl Pts',(-0.120812344967181,1.80122635347103,
6.27328913600132));
#51024=CARTESIAN_POINT('Ctrl Pts',(-0.12115781729771,1.80136628143753,6.27326628198026));
#51025=CARTESIAN_POINT('Ctrl Pts',(-0.121870227687585,1.80165627140686,
6.27321907869855));
#51026=CARTESIAN_POINT('Ctrl Pts',(-0.122237133038708,1.80180641171921,
6.27319472681807));
#51027=CARTESIAN_POINT('Ctrl Pts',(-0.122962841890948,1.80210494146638,
6.27314647866278));
#51028=CARTESIAN_POINT('Ctrl Pts',(-0.123321656128986,1.80225330310456,
6.27312258336512));
#51029=CARTESIAN_POINT('Ctrl Pts',(-0.12450518139215,1.80274517064069,6.27304363414393));
#51030=CARTESIAN_POINT('Ctrl Pts',(-0.125328726679441,1.80309145513457,
6.27298848592717));
#51031=CARTESIAN_POINT('Ctrl Pts',(-0.130910950126545,1.80546603290428,
6.27261321932604));
#51032=CARTESIAN_POINT('Ctrl Pts',(-0.135621403141066,1.80760512208367,
6.27228933568671));
#51033=CARTESIAN_POINT('Ctrl Pts',(-0.146938836682586,1.81307685811564,
6.27149281764672));
#51034=CARTESIAN_POINT('Ctrl Pts',(-0.153486218056481,1.81652534845163,
6.27101634969844));
#51035=CARTESIAN_POINT('Ctrl Pts',(-0.167653070494215,1.82462173927933,
6.26995041910129));
#51036=CARTESIAN_POINT('Ctrl Pts',(-0.17520980331825,1.82936695576433,6.26935828932215));
#51037=CARTESIAN_POINT('Ctrl Pts',(-0.205956175787806,1.85050193397043,
6.26685635537638));
#51038=CARTESIAN_POINT('Ctrl Pts',(-0.227125413261808,1.8696059663331,6.2648908044307));
#51039=CARTESIAN_POINT('Ctrl Pts',(-0.246465487858104,1.89235107073042,
6.2630031230539));
#51040=CARTESIAN_POINT('Ctrl Pts',(-0.24740529161617,1.89347170555832,6.26291115855634));
#51041=CARTESIAN_POINT('Ctrl Pts',(-0.248606641161095,1.89492417992802,
6.26279333850767));
#51042=CARTESIAN_POINT('Ctrl Pts',(-0.248875189131882,1.89525016667402,
6.26276698409329));
#51043=CARTESIAN_POINT('Ctrl Pts',(-0.249300288299547,1.89576826081635,
6.26272524038679));
#51044=CARTESIAN_POINT('Ctrl Pts',(-0.249457258910454,1.89596002103976,
6.26270982062711));
#51045=CARTESIAN_POINT('Ctrl Pts',(-0.249738484227849,1.89630438432064,
6.26268218509296));
#51046=CARTESIAN_POINT('Ctrl Pts',(-0.249862819423746,1.89645691900402,
6.26266996345988));
#51047=CARTESIAN_POINT('Ctrl Pts',(-0.25015526323524,1.8968163614582,6.26264120926538));
#51048=CARTESIAN_POINT('Ctrl Pts',(-0.250323254646118,1.89702336370907,
6.26262468529031));
#51049=CARTESIAN_POINT('Ctrl Pts',(-0.250810941065243,1.89762582659935,
6.26257669598879));
#51050=CARTESIAN_POINT('Ctrl Pts',(-0.251129959032216,1.89802183805551,
6.26254527958115));
#51051=CARTESIAN_POINT('Ctrl Pts',(-0.253367222983191,1.90081255016796,
6.26232477166439));
#51052=CARTESIAN_POINT('Ctrl Pts',(-0.255252204521904,1.90323388603487,
6.26213802198015));
#51053=CARTESIAN_POINT('Ctrl Pts',(-0.260888244066879,1.91069093268913,
6.26157539141749));
#51054=CARTESIAN_POINT('Ctrl Pts',(-0.264527157038789,1.91580990058281,
6.26120616292196));
#51055=CARTESIAN_POINT('Ctrl Pts',(-0.280725121447392,1.94006727641345,
6.25951748273053));
#51056=CARTESIAN_POINT('Ctrl Pts',(-0.291372574948194,1.96040329119677,
6.25826853624167));
#51057=CARTESIAN_POINT('Ctrl Pts',(-0.300648402140433,1.98390795472358,
6.25684030201397));
#51058=CARTESIAN_POINT('Ctrl Pts',(-0.301496391502955,1.9861283601449,6.25670557691139));
#51059=CARTESIAN_POINT('Ctrl Pts',(-0.304477866575999,1.99420200716584,
6.25621597003656));
#51060=CARTESIAN_POINT('Ctrl Pts',(-0.306466006636432,2.00010721877873,
6.25585833992316));
#51061=CARTESIAN_POINT('Ctrl Pts',(-0.311173390847604,2.01555638927262,
6.25491908409505));
#51062=CARTESIAN_POINT('Ctrl Pts',(-0.313625064429223,2.0251742612823,6.25433068022026));
#51063=CARTESIAN_POINT('Ctrl Pts',(-0.31584005359885,2.03591157761723,6.25366403910757));
#51064=CARTESIAN_POINT('Ctrl Pts',(-0.316045986100183,2.03693495444631,
6.25360040732598));
#51065=CARTESIAN_POINT('Ctrl Pts',(-0.316346412621837,2.03846635198416,
6.25350504111151));
#51066=CARTESIAN_POINT('Ctrl Pts',(-0.316444664157109,2.0389736357102,6.2534734265395));
#51067=CARTESIAN_POINT('Ctrl Pts',(-0.316611713492429,2.03984738134122,
6.25341893149327));
#51068=CARTESIAN_POINT('Ctrl Pts',(-0.316681096289379,2.04021373148304,
6.25339606970442));
#51069=CARTESIAN_POINT('Ctrl Pts',(-0.316822923714335,2.04096977264355,
6.25334886296308));
#51070=CARTESIAN_POINT('Ctrl Pts',(-0.316895285480426,2.04135947842366,
6.25332451541268));
#51071=CARTESIAN_POINT('Ctrl Pts',(-0.317037084279483,2.04213106643138,
6.25327627990272));
#51072=CARTESIAN_POINT('Ctrl Pts',(-0.317106550720927,2.0425129425994,6.25325239292746));
#51073=CARTESIAN_POINT('Ctrl Pts',(-0.31726550323091,2.04339580334904,6.2531971354726));
#51074=CARTESIAN_POINT('Ctrl Pts',(-0.317354492658577,2.04389687527847,
6.25316574923566));
#51075=CARTESIAN_POINT('Ctrl Pts',(-0.317581153164674,2.04519092638957,
6.25308462777441));
#51076=CARTESIAN_POINT('Ctrl Pts',(-0.317717040598631,2.04598421073572,
6.25303483595291));
#51077=CARTESIAN_POINT('Ctrl Pts',(-0.320810706929163,2.064460057515,6.25187368436787));
#51078=CARTESIAN_POINT('Ctrl Pts',(-0.322290242970631,2.0823546240026,6.25071470024017));
#51079=CARTESIAN_POINT('Ctrl Pts',(-0.322274881613702,2.1002762351798,6.24952200414216));
#51080=CARTESIAN_POINT('',(-0.3227631030959,2.10004611274009,6.12435703103352));
#51081=CARTESIAN_POINT('Ctrl Pts',(-0.322798597665563,2.10004734253964,
6.12437741302984));
#51082=CARTESIAN_POINT('Ctrl Pts',(-0.322580086172827,1.99582903567067,
6.13084004242903));
#51083=CARTESIAN_POINT('Ctrl Pts',(-0.211048222901441,1.78439851022638,
6.14392611966916));
#51084=CARTESIAN_POINT('Ctrl Pts',(0.149287431151383,1.74938860369369,6.16363564475023));
#51085=CARTESIAN_POINT('Ctrl Pts',(0.375612323430391,2.03573126104505,6.18350598827301));
#51086=CARTESIAN_POINT('Ctrl Pts',(0.257364043962396,2.38103173698883,6.20337633179581));
#51087=CARTESIAN_POINT('Ctrl Pts',(-0.0969807088903252,2.46852385326159,
6.22324667531859));
#51088=CARTESIAN_POINT('Ctrl Pts',(-0.301768811357061,2.27515652580511,
6.2385803034489));
#51089=CARTESIAN_POINT('Ctrl Pts',(-0.322286541621404,2.13412944815347,
6.24729048373829));
#51090=CARTESIAN_POINT('Ctrl Pts',(-0.322023435600497,2.1002684890243,6.24937721618673));
#51091=CARTESIAN_POINT('',(-0.322274893287392,2.10011804807506,5.87466618688513));
#51092=CARTESIAN_POINT('Ctrl Pts',(-0.322274998677053,2.10002920112239,
6.1240767475264));
#51093=CARTESIAN_POINT('Ctrl Pts',(-0.322274898616863,2.10113350447985,
6.12400672680945));
#51094=CARTESIAN_POINT('Ctrl Pts',(-0.32226912256732,2.10223782043467,6.12393698681781));
#51095=CARTESIAN_POINT('Ctrl Pts',(-0.32224942848518,2.10413679398095,6.12381757158123));
#51096=CARTESIAN_POINT('Ctrl Pts',(-0.322238247202919,2.10493145967723,
6.12376775308541));
#51097=CARTESIAN_POINT('Ctrl Pts',(-0.322218942390711,2.10601779972598,
6.12369986631237));
#51098=CARTESIAN_POINT('Ctrl Pts',(-0.322213362324257,2.10630950792266,
6.12368165850064));
#51099=CARTESIAN_POINT('Ctrl Pts',(-0.322202897407712,2.10682030422494,
6.12364981362972));
#51100=CARTESIAN_POINT('Ctrl Pts',(-0.322198185229367,2.10703939508986,
6.12363616694993));
#51101=CARTESIAN_POINT('Ctrl Pts',(-0.322188586701757,2.10746545950735,
6.12360965235869));
#51102=CARTESIAN_POINT('Ctrl Pts',(-0.322183724369211,2.10767243370905,
6.12359678308214));
#51103=CARTESIAN_POINT('Ctrl Pts',(-0.322173653480351,2.10808421934652,
6.12357120111331));
#51104=CARTESIAN_POINT('Ctrl Pts',(-0.322168449070601,2.10828903030222,
6.12355848820197));
#51105=CARTESIAN_POINT('Ctrl Pts',(-0.322155731978818,2.10877137734158,
6.12352857351878));
#51106=CARTESIAN_POINT('Ctrl Pts',(-0.322148055939749,2.1090489094846,6.12351138097397));
#51107=CARTESIAN_POINT('Ctrl Pts',(-0.322124331639828,2.10986835962504,
6.12346067505366));
#51108=CARTESIAN_POINT('Ctrl Pts',(-0.322107274433623,2.11041025086683,
6.12342721795403));
#51109=CARTESIAN_POINT('Ctrl Pts',(-0.322063618093307,2.11169413423134,
6.12334811926339));
#51110=CARTESIAN_POINT('Ctrl Pts',(-0.322035822007876,2.11243608634034,
6.12330254295059));
#51111=CARTESIAN_POINT('Ctrl Pts',(-0.321948266027934,2.11457553263276,
6.12317149312285));
#51112=CARTESIAN_POINT('Ctrl Pts',(-0.321881970882867,2.11597276205806,
6.12308636392612));
#51113=CARTESIAN_POINT('Ctrl Pts',(-0.32011194219942,2.14876619021454,6.12109815840227));
#51114=CARTESIAN_POINT('Ctrl Pts',(-0.313831599476083,2.17975114258912,
6.11941763538675));
#51115=CARTESIAN_POINT('Ctrl Pts',(-0.29794204085832,2.22380738493369,6.11676031854832));
#51116=CARTESIAN_POINT('Ctrl Pts',(-0.291695607772656,2.23788150193843,
6.11586886754736));
#51117=CARTESIAN_POINT('Ctrl Pts',(-0.283320200627048,2.253612547653,6.11479381841947));
#51118=CARTESIAN_POINT('Ctrl Pts',(-0.28214693977033,2.25575703756126,6.11464552157857));
#51119=CARTESIAN_POINT('Ctrl Pts',(-0.280603125080307,2.25850413702551,
6.11445321684188));
#51120=CARTESIAN_POINT('Ctrl Pts',(-0.280254804239856,2.2591192004347,6.11441000824338));
#51121=CARTESIAN_POINT('Ctrl Pts',(-0.27968948582083,2.26010982254473,6.11434016804255));
#51122=CARTESIAN_POINT('Ctrl Pts',(-0.279473747274201,2.26048610013216,
6.11431358189952));
#51123=CARTESIAN_POINT('Ctrl Pts',(-0.279060869291288,2.2612028586807,6.11426282748151));
#51124=CARTESIAN_POINT('Ctrl Pts',(-0.27886386454668,2.26154341665432,6.11423866411277));
#51125=CARTESIAN_POINT('Ctrl Pts',(-0.278412547935586,2.26232031247752,
6.11418343116762));
#51126=CARTESIAN_POINT('Ctrl Pts',(-0.278157833480306,2.26275641418911,
6.1141523470256));
#51127=CARTESIAN_POINT('Ctrl Pts',(-0.277375219009772,2.26408914077643,
6.11405710833899));
#51128=CARTESIAN_POINT('Ctrl Pts',(-0.276844004867481,2.26498380274963,
6.11399283332681));
#51129=CARTESIAN_POINT('Ctrl Pts',(-0.272876742437086,2.27159228795988,
6.11351550439498));
#51130=CARTESIAN_POINT('Ctrl Pts',(-0.269268669897204,2.27720045869222,
6.11309616215871));
#51131=CARTESIAN_POINT('Ctrl Pts',(-0.264430243480757,2.28423168398243,
6.11255122659846));
#51132=CARTESIAN_POINT('Ctrl Pts',(-0.263357652006095,2.28576171282842,
6.11243144755916));
#51133=CARTESIAN_POINT('Ctrl Pts',(-0.261166401172612,2.28883036033382,
6.1121887821376));
#51134=CARTESIAN_POINT('Ctrl Pts',(-0.260047302936068,2.29036857432157,
6.11206588349018));
#51135=CARTESIAN_POINT('Ctrl Pts',(-0.257804110611697,2.29339517769355,
6.11182156540464));
#51136=CARTESIAN_POINT('Ctrl Pts',(-0.256680581279543,2.29488389668715,
6.11170016844418));
#51137=CARTESIAN_POINT('Ctrl Pts',(-0.238222666097382,2.31890481292924,
6.10972152273238));
#51138=CARTESIAN_POINT('Ctrl Pts',(-0.217997998291099,2.33905200559161,
6.1077600500686));
#51139=CARTESIAN_POINT('Ctrl Pts',(-0.188977541424347,2.36117772422409,
6.10533712570136));
#51140=CARTESIAN_POINT('Ctrl Pts',(-0.182377142941742,2.3658287334372,6.10480920820219));
#51141=CARTESIAN_POINT('Ctrl Pts',(-0.174371764272286,2.37103106641102,
6.10420180647337));
#51142=CARTESIAN_POINT('Ctrl Pts',(-0.173129480306708,2.37182629448551,
6.1041084563732));
#51143=CARTESIAN_POINT('Ctrl Pts',(-0.171320054569274,2.37296713255524,
6.1039738489586));
#51144=CARTESIAN_POINT('Ctrl Pts',(-0.170757256368001,2.37331954918914,
6.10393217031264));
#51145=CARTESIAN_POINT('Ctrl Pts',(-0.169877975506854,2.37386636705761,
6.10386735366194));
#51146=CARTESIAN_POINT('Ctrl Pts',(-0.169562243150448,2.37406196246232,
6.10384413924988));
#51147=CARTESIAN_POINT('Ctrl Pts',(-0.168969732293502,2.37442760559793,
6.10380068787249));
#51148=CARTESIAN_POINT('Ctrl Pts',(-0.168693033856916,2.37459778126547,
6.10378044258198));
#51149=CARTESIAN_POINT('Ctrl Pts',(-0.168225132829522,2.37488457662624,
6.10374628611977));
#51150=CARTESIAN_POINT('Ctrl Pts',(-0.168034065868195,2.3750014154346,6.10373236045696));
#51151=CARTESIAN_POINT('Ctrl Pts',(-0.167653623978817,2.37523351383682,
6.10370467664237));
#51152=CARTESIAN_POINT('Ctrl Pts',(-0.167464251707707,2.3753487773222,6.1036909182416));
#51153=CARTESIAN_POINT('Ctrl Pts',(-0.167041871855284,2.37560526647514,
6.10366027932226));
#51154=CARTESIAN_POINT('Ctrl Pts',(-0.166808803420858,2.37574639247744,
6.10364340539893));
#51155=CARTESIAN_POINT('Ctrl Pts',(-0.166005329703341,2.37623151490913,
6.10358534582964));
#51156=CARTESIAN_POINT('Ctrl Pts',(-0.165434032082281,2.37657404138233,
6.10354425613104));
#51157=CARTESIAN_POINT('Ctrl Pts',(-0.159353654254091,2.38019400411052,
6.10310893216183));
#51158=CARTESIAN_POINT('Ctrl Pts',(-0.153748564696659,2.38330841758884,
6.1027250154061));
#51159=CARTESIAN_POINT('Ctrl Pts',(-0.141208622479554,2.38979422418645,
6.1018954175983));
#51160=CARTESIAN_POINT('Ctrl Pts',(-0.134238177005032,2.39308820090093,
6.10145318747766));
#51161=CARTESIAN_POINT('Ctrl Pts',(-0.120689053002301,2.3989061051128,6.10061709886834));
#51162=CARTESIAN_POINT('Ctrl Pts',(-0.114132783964845,2.40147042849115,
6.10022260601275));
#51163=CARTESIAN_POINT('Ctrl Pts',(-0.105491723022323,2.4045278306303,6.09970990897851));
#51164=CARTESIAN_POINT('Ctrl Pts',(-0.103478779845182,2.40521770164515,
6.09959098089353));
#51165=CARTESIAN_POINT('Ctrl Pts',(-0.0991404590385739,2.40665666929372,
6.09933550552864));
#51166=CARTESIAN_POINT('Ctrl Pts',(-0.0968131012961575,2.40739936048031,
6.09919896541882));
#51167=CARTESIAN_POINT('Ctrl Pts',(-0.0917337361133889,2.40895684733647,
6.0989017312117));
#51168=CARTESIAN_POINT('Ctrl Pts',(-0.0889788427003446,2.4097614844295,
6.09874100001503));
#51169=CARTESIAN_POINT('Ctrl Pts',(-0.0771559418465538,2.41304392814447,
6.09805218602418));
#51170=CARTESIAN_POINT('Ctrl Pts',(-0.0679929879320068,2.41516103852153,
6.09752063192441));
#51171=CARTESIAN_POINT('Ctrl Pts',(-0.047621525561036,2.41893806387761,
6.09632756279444));
#51172=CARTESIAN_POINT('Ctrl Pts',(-0.036392189163703,2.42041358372475,
6.09566238885254));
#51173=CARTESIAN_POINT('Ctrl Pts',(-0.023088225797105,2.4214532924999,6.09485546277121));
#51174=CARTESIAN_POINT('Ctrl Pts',(-0.0210657145563982,2.42159216534073,
6.09473229336176));
#51175=CARTESIAN_POINT('Ctrl Pts',(-0.0183837091142796,2.42175091268301,
6.09456825937055));
#51176=CARTESIAN_POINT('Ctrl Pts',(-0.0177252411940359,2.42178785929176,
6.09452793087126));
#51177=CARTESIAN_POINT('Ctrl Pts',(-0.0166440726068344,2.4218451950262,
6.09446162017107));
#51178=CARTESIAN_POINT('Ctrl Pts',(-0.0162214347506905,2.42186677331827,
6.09443567531845));
#51179=CARTESIAN_POINT('Ctrl Pts',(-0.0154024481545931,2.4219069704978,
6.0943853535479));
#51180=CARTESIAN_POINT('Ctrl Pts',(-0.0150061049320919,2.42192568999189,
6.09436097983218));
#51181=CARTESIAN_POINT('Ctrl Pts',(-0.0140909762060335,2.42196721832163,
6.0943046541099));
#51182=CARTESIAN_POINT('Ctrl Pts',(-0.0135721691582012,2.42198950526922,
6.09427268579729));
#51183=CARTESIAN_POINT('Ctrl Pts',(-0.0119106150685491,2.42205685954152,
6.09417018609633));
#51184=CARTESIAN_POINT('Ctrl Pts',(-0.01076769074757,2.42209709764446,6.09409950357062));
#51185=CARTESIAN_POINT('Ctrl Pts',(-0.000240865812410066,2.42241161650631,
6.0934468237269));
#51186=CARTESIAN_POINT('Ctrl Pts',(0.00914973685938343,2.42228180401299,
6.09285221746115));
#51187=CARTESIAN_POINT('Ctrl Pts',(0.0486213469336585,2.42000968734767,
6.09029724669452));
#51188=CARTESIAN_POINT('Ctrl Pts',(0.0783280863433009,2.41406111751519,
6.0882193768987));
#51189=CARTESIAN_POINT('Ctrl Pts',(0.114232440335848,2.40145434908952,6.08568376177453));
#51190=CARTESIAN_POINT('Ctrl Pts',(0.121599176659267,2.3985589308198,6.08516340436872));
#51191=CARTESIAN_POINT('Ctrl Pts',(0.130888543138024,2.39450687539588,6.08451335216291));
#51192=CARTESIAN_POINT('Ctrl Pts',(0.132915518547507,2.39359764292307,6.08437189446203));
#51193=CARTESIAN_POINT('Ctrl Pts',(0.135748078563823,2.39229170425354,6.08417492564908));
#51194=CARTESIAN_POINT('Ctrl Pts',(0.136561602216125,2.39191250410641,6.08411843815546));
#51195=CARTESIAN_POINT('Ctrl Pts',(0.137790921447534,2.39133322927272,6.08403321714094));
#51196=CARTESIAN_POINT('Ctrl Pts',(0.138207880937534,2.39113565594891,6.08400433599126));
#51197=CARTESIAN_POINT('Ctrl Pts',(0.13888495529807,2.39081304665947,6.08395747856859));
#51198=CARTESIAN_POINT('Ctrl Pts',(0.139145327220876,2.39068855641331,6.08393946918626));
#51199=CARTESIAN_POINT('Ctrl Pts',(0.13964509880361,2.3904487779416,6.08390492045685));
#51200=CARTESIAN_POINT('Ctrl Pts',(0.139884523634199,2.39033354314735,6.08388837782777));
#51201=CARTESIAN_POINT('Ctrl Pts',(0.140316533203192,2.39012495917646,6.08385854477205));
#51202=CARTESIAN_POINT('Ctrl Pts',(0.140509167030384,2.39003171448762,6.08384524788853));
#51203=CARTESIAN_POINT('Ctrl Pts',(0.140927025622294,2.38982893540355,6.08381641696886));
#51204=CARTESIAN_POINT('Ctrl Pts',(0.141152214995471,2.38971933064744,6.08380088745265));
#51205=CARTESIAN_POINT('Ctrl Pts',(0.141757559941735,2.38942382227757,6.08375916212097));
#51206=CARTESIAN_POINT('Ctrl Pts',(0.142137479152578,2.38923743140782,6.08373299673318));
#51207=CARTESIAN_POINT('Ctrl Pts',(0.143876640267258,2.38837993328814,6.08361331388479));
#51208=CARTESIAN_POINT('Ctrl Pts',(0.145231532451431,2.38769997520186,6.08352034074589));
#51209=CARTESIAN_POINT('Ctrl Pts',(0.172013478160711,2.37402193517599,6.08168684957241));
#51210=CARTESIAN_POINT('Ctrl Pts',(0.195610944716856,2.35770840732004,6.08014059976619));
#51211=CARTESIAN_POINT('Ctrl Pts',(0.21970093544351,2.3358146653514,6.07830988589373));
#51212=CARTESIAN_POINT('Ctrl Pts',(0.222600108438508,2.33307991808217,6.07808494552923));
#51213=CARTESIAN_POINT('Ctrl Pts',(0.237489126892852,2.31850410163867,6.07690208155974));
#51214=CARTESIAN_POINT('Ctrl Pts',(0.248585689296406,2.30579154243007,6.07592233106721));
#51215=CARTESIAN_POINT('Ctrl Pts',(0.259336645921011,2.29132970403322,6.07482669604394));
#51216=CARTESIAN_POINT('Ctrl Pts',(0.260031314459109,2.29038452407359,6.07475517924895));
#51217=CARTESIAN_POINT('Ctrl Pts',(0.261032599098126,2.28900645280984,6.07465103015971));
#51218=CARTESIAN_POINT('Ctrl Pts',(0.261343336403448,2.28857655609296,6.07461855745714));
#51219=CARTESIAN_POINT('Ctrl Pts',(0.261884851598014,2.2878234751956,6.0745617017807));
#51220=CARTESIAN_POINT('Ctrl Pts',(0.262116096734501,2.28750062709616,6.07453733688364));
#51221=CARTESIAN_POINT('Ctrl Pts',(0.262562527474419,2.28687491223974,6.07449013265401));
#51222=CARTESIAN_POINT('Ctrl Pts',(0.262777787356236,2.28657209900929,6.07446729622688));
#51223=CARTESIAN_POINT('Ctrl Pts',(0.26328824182051,2.28585138988293,6.07441296299691));
#51224=CARTESIAN_POINT('Ctrl Pts',(0.263582965130955,2.28543316286551,6.07438144819709));
#51225=CARTESIAN_POINT('Ctrl Pts',(0.264622296203507,2.28395081617401,6.0742697990933));
#51226=CARTESIAN_POINT('Ctrl Pts',(0.265361458400782,2.28288290990497,6.07418945733113));
#51227=CARTESIAN_POINT('Ctrl Pts',(0.277759066222317,2.26473803186194,6.07282581644883));
#51228=CARTESIAN_POINT('Ctrl Pts',(0.28775159622199,2.2465859498543,6.07147846067998));
#51229=CARTESIAN_POINT('Ctrl Pts',(0.307045587093238,2.20184029626405,6.06821207150958));
#51230=CARTESIAN_POINT('Ctrl Pts',(0.314743218343517,2.17473457287738,6.06627012501356));
#51231=CARTESIAN_POINT('Ctrl Pts',(0.319018726307291,2.14571485425047,6.06440853122825));
#51232=CARTESIAN_POINT('Ctrl Pts',(0.319196788323489,2.1444545394894,6.06432812477893));
#51233=CARTESIAN_POINT('Ctrl Pts',(0.319447231821962,2.14260277756494,6.06421066551856));
#51234=CARTESIAN_POINT('Ctrl Pts',(0.319525444722583,2.14201215018338,6.06417330289743));
#51235=CARTESIAN_POINT('Ctrl Pts',(0.319646234143863,2.14108015289036,6.06411450918562));
#51236=CARTESIAN_POINT('Ctrl Pts',(0.319689902232793,2.14073892950041,6.06409301818327));
#51237=CARTESIAN_POINT('Ctrl Pts',(0.319771303055945,2.14009467071225,6.06405250745693));
#51238=CARTESIAN_POINT('Ctrl Pts',(0.319809151549059,2.13979165069384,6.06403348127638));
#51239=CARTESIAN_POINT('Ctrl Pts',(0.31986406256352,2.13934688662655,6.06400559614002));
#51240=CARTESIAN_POINT('Ctrl Pts',(0.319881461542806,2.13920518547679,6.06399671807524));
#51241=CARTESIAN_POINT('Ctrl Pts',(0.31992475544746,2.13885064283601,6.06397452009062));
#51242=CARTESIAN_POINT('Ctrl Pts',(0.319950531945824,2.13863778855871,6.06396120709976));
#51243=CARTESIAN_POINT('Ctrl Pts',(0.320009959259841,2.13814291891631,6.06393028741672));
#51244=CARTESIAN_POINT('Ctrl Pts',(0.320043449674723,2.13786088497024,6.06391268992212));
#51245=CARTESIAN_POINT('Ctrl Pts',(0.320145841709243,2.13698876329907,6.06385834746378));
#51246=CARTESIAN_POINT('Ctrl Pts',(0.320213485006274,2.13639852479885,6.06382167337149));
#51247=CARTESIAN_POINT('Ctrl Pts',(0.320725128806687,2.13182221295607,6.06353810997254));
#51248=CARTESIAN_POINT('Ctrl Pts',(0.321096340773843,2.12782813358008,6.0632952246199));
#51249=CARTESIAN_POINT('Ctrl Pts',(0.323652420562508,2.09335156088208,6.06123025031372));
#51250=CARTESIAN_POINT('Ctrl Pts',(0.321566044928294,2.06270473051419,6.05959456051045));
#51251=CARTESIAN_POINT('Ctrl Pts',(0.312168733057205,2.01862317056703,6.0570299914393));
#51252=CARTESIAN_POINT('Ctrl Pts',(0.308191371039751,2.00466110367454,6.05618687050992));
#51253=CARTESIAN_POINT('Ctrl Pts',(0.302760946680964,1.98954904935848,6.05521773809992));
#51254=CARTESIAN_POINT('Ctrl Pts',(0.302223416544587,1.98808659734486,6.055123360547));
#51255=CARTESIAN_POINT('Ctrl Pts',(0.301261419243848,1.98552678415206,6.05495709954516));
#51256=CARTESIAN_POINT('Ctrl Pts',(0.300841505221578,1.98442773451244,6.05488536835715));
#51257=CARTESIAN_POINT('Ctrl Pts',(0.300223320311237,1.98283594565119,6.05478096393333));
#51258=CARTESIAN_POINT('Ctrl Pts',(0.300029831274837,1.98234134953173,6.05474845139882));
#51259=CARTESIAN_POINT('Ctrl Pts',(0.299689489102198,1.98147766650431,6.05469154939092));
#51260=CARTESIAN_POINT('Ctrl Pts',(0.299543174120842,1.98110836761603,6.05466717808328));
#51261=CARTESIAN_POINT('Ctrl Pts',(0.299258755925108,1.98039435411291,6.05461997848561));
#51262=CARTESIAN_POINT('Ctrl Pts',(0.299120738862869,1.98004960564362,6.05459715313265));
#51263=CARTESIAN_POINT('Ctrl Pts',(0.298791401571291,1.97923106751874,6.05454287308536));
#51264=CARTESIAN_POINT('Ctrl Pts',(0.298599550252134,1.97875749388097,6.05451140047626));
#51265=CARTESIAN_POINT('Ctrl Pts',(0.297917581837151,1.97708553214206,6.0544000426733));
#51266=CARTESIAN_POINT('Ctrl Pts',(0.297421375003508,1.97588965559209,6.05431995143931));
#51267=CARTESIAN_POINT('Ctrl Pts',(0.289258050740357,1.95654587140993,6.05301716211879));
#51268=CARTESIAN_POINT('Ctrl Pts',(0.279951422758845,1.93913903503645,6.05173661004203));
#51269=CARTESIAN_POINT('Ctrl Pts',(0.267917009404502,1.92087322533996,6.05027353164486));
#51270=CARTESIAN_POINT('Ctrl Pts',(0.266699556357598,1.91906555946356,6.05012739444293));
#51271=CARTESIAN_POINT('Ctrl Pts',(0.264039097231468,1.91520052727369,6.0498121116476));
#51272=CARTESIAN_POINT('Ctrl Pts',(0.262590172888067,1.91314740873039,6.04964287749077));
#51273=CARTESIAN_POINT('Ctrl Pts',(0.251571583443207,1.89791543399322,6.04837467838568));
#51274=CARTESIAN_POINT('Ctrl Pts',(0.241039042175458,1.88546180525178,6.04726459935883));
#51275=CARTESIAN_POINT('Ctrl Pts',(0.223491816647637,1.86764551801355,6.0456066973702));
#51276=CARTESIAN_POINT('Ctrl Pts',(0.217123386040066,1.86168369121783,6.04503827155683));
#51277=CARTESIAN_POINT('Ctrl Pts',(0.209847767465566,1.85540670646291,6.04443154508124));
#51278=CARTESIAN_POINT('Ctrl Pts',(0.209172756613997,1.85482919691145,6.04437564307485));
#51279=CARTESIAN_POINT('Ctrl Pts',(0.208146156011534,1.85395820867236,6.04429122161121));
#51280=CARTESIAN_POINT('Ctrl Pts',(0.207796321034468,1.85366268185127,6.04426255776883));
#51281=CARTESIAN_POINT('Ctrl Pts',(0.207226096709322,1.85318305785927,6.04421600765573));
#51282=CARTESIAN_POINT('Ctrl Pts',(0.207006090655745,1.85299850907732,6.04419808886513));
#51283=CARTESIAN_POINT('Ctrl Pts',(0.206582817225344,1.85264441523491,6.0441636944625));
#51284=CARTESIAN_POINT('Ctrl Pts',(0.20637958719456,1.85247482617348,6.04414721564308));
#51285=CARTESIAN_POINT('Ctrl Pts',(0.206011739110834,1.85216863650514,6.04411745291724));
#51286=CARTESIAN_POINT('Ctrl Pts',(0.205847194409926,1.85203194976444,6.04410416268811));
#51287=CARTESIAN_POINT('Ctrl Pts',(0.205514161518965,1.85175586037013,6.04407731052548));
#51288=CARTESIAN_POINT('Ctrl Pts',(0.205345668240044,1.85161646596211,6.04406374918618));
#51289=CARTESIAN_POINT('Ctrl Pts',(0.204868163875743,1.85122224480677,6.04402538465059));
#51290=CARTESIAN_POINT('Ctrl Pts',(0.204558818052361,1.85096782133639,6.04400061093507));
#51291=CARTESIAN_POINT('Ctrl Pts',(0.203261494048787,1.84990487717544,6.04389704770142));
#51292=CARTESIAN_POINT('Ctrl Pts',(0.202269173123293,1.84910163979189,6.04381863644171));
#51293=CARTESIAN_POINT('Ctrl Pts',(0.18359681564177,1.83417002034061,6.04235760867634));
#51294=CARTESIAN_POINT('Ctrl Pts',(0.164478638829028,1.82193436586509,6.04110004981311));
#51295=CARTESIAN_POINT('Ctrl Pts',(0.129208477798294,1.80428286553856,6.03889556054818));
#51296=CARTESIAN_POINT('Ctrl Pts',(0.113619585297817,1.79795035378823,6.03795578657513));
#51297=CARTESIAN_POINT('Ctrl Pts',(0.0895193974025224,1.79029125458355,
6.03648707606282));
#51298=CARTESIAN_POINT('Ctrl Pts',(0.0813318235494002,1.78804111587925,
6.03598582363374));
#51299=CARTESIAN_POINT('Ctrl Pts',(0.0706213690562402,1.78554794455058,
6.03532271352782));
#51300=CARTESIAN_POINT('Ctrl Pts',(0.06817076142114,1.78500758789841,6.03517050621778));
#51301=CARTESIAN_POINT('Ctrl Pts',(0.0650155828222821,1.78435041774936,
6.034973837378));
#51302=CARTESIAN_POINT('Ctrl Pts',(0.0643165432968785,1.78420724037722,
6.0349302208678));
#51303=CARTESIAN_POINT('Ctrl Pts',(0.0631903630350583,1.7839804704168,6.03485988026399));
#51304=CARTESIAN_POINT('Ctrl Pts',(0.0627635156971211,1.78389541896251,
6.03483320282798));
#51305=CARTESIAN_POINT('Ctrl Pts',(0.0619508297192864,1.78373519822124,
6.0347823785058));
#51306=CARTESIAN_POINT('Ctrl Pts',(0.0615650229858371,1.78365986961872,
6.03475823675538));
#51307=CARTESIAN_POINT('Ctrl Pts',(0.0606859728769294,1.78348990447915,
6.03470319835396));
#51308=CARTESIAN_POINT('Ctrl Pts',(0.0601926450416233,1.78339571489164,
6.03467228750895));
#51309=CARTESIAN_POINT('Ctrl Pts',(0.0586904424509208,1.78311254184685,
6.03457809168736));
#51310=CARTESIAN_POINT('Ctrl Pts',(0.0576808905213132,1.78292722601983,
6.03451469006433));
#51311=CARTESIAN_POINT('Ctrl Pts',(0.0504045683259694,1.78162746737534,
6.03405700118663));
#51312=CARTESIAN_POINT('Ctrl Pts',(0.0441072663605818,1.78069414384619,
6.03365699270359));
#51313=CARTESIAN_POINT('Ctrl Pts',(0.0361042220939283,1.77974926804714,
6.03314320680647));
#51314=CARTESIAN_POINT('Ctrl Pts',(0.0344201255587868,1.77956388943266,
6.03303479003378));
#51315=CARTESIAN_POINT('Ctrl Pts',(0.028005107675333,1.77890890463891,6.03262066645843));
#51316=CARTESIAN_POINT('Ctrl Pts',(0.0232656360752081,1.77853074142744,
6.03231232921712));
#51317=CARTESIAN_POINT('Ctrl Pts',(-0.00681942210835438,1.77679902498352,
6.03034053974536));
#51318=CARTESIAN_POINT('Ctrl Pts',(-0.0322408423240995,1.77833925592178,
6.02859929749724));
#51319=CARTESIAN_POINT('Ctrl Pts',(-0.0659607766006114,1.78442218769125,
6.02630594916846));
#51320=CARTESIAN_POINT('Ctrl Pts',(-0.0746397359638249,1.78636148937369,
6.02571827721844));
#51321=CARTESIAN_POINT('Ctrl Pts',(-0.0869442518918768,1.78965072944109,
6.02489858896583));
#51322=CARTESIAN_POINT('Ctrl Pts',(-0.0906425813657495,1.79071065588619,
6.02465401329631));
#51323=CARTESIAN_POINT('Ctrl Pts',(-0.0948356343225887,1.79199404636649,
6.02437947101997));
#51324=CARTESIAN_POINT('Ctrl Pts',(-0.0953496345896853,1.7921527778189,
6.02434586406068));
#51325=CARTESIAN_POINT('Ctrl Pts',(-0.0961236252215004,1.79239392287948,
6.02429533226696));
#51326=CARTESIAN_POINT('Ctrl Pts',(-0.0963839091117196,1.79247537972893,
6.0242783516804));
#51327=CARTESIAN_POINT('Ctrl Pts',(-0.0968523120901613,1.79262262134587,
6.02424781686923));
#51328=CARTESIAN_POINT('Ctrl Pts',(-0.0970604672825517,1.79268828698317,
6.02423425568043));
#51329=CARTESIAN_POINT('Ctrl Pts',(-0.0974768055761168,1.79282009226945,
6.02420714811128));
#51330=CARTESIAN_POINT('Ctrl Pts',(-0.0976849872237315,1.79288623181229,
6.02419360179971));
#51331=CARTESIAN_POINT('Ctrl Pts',(-0.0982735534011247,1.79307387895018,
6.02415532701133));
#51332=CARTESIAN_POINT('Ctrl Pts',(-0.0986537812620749,1.79319588247947,
6.02413062779119));
#51333=CARTESIAN_POINT('Ctrl Pts',(-0.100239395561168,1.79370791020667,
6.02402773766455));
#51334=CARTESIAN_POINT('Ctrl Pts',(-0.10144272454605,1.79410434057707,6.02394991893403));
#51335=CARTESIAN_POINT('Ctrl Pts',(-0.123522920440769,1.80152316715299,
6.02252634616796));
#51336=CARTESIAN_POINT('Ctrl Pts',(-0.143631667616612,1.81066178225136,
6.02129917779544));
#51337=CARTESIAN_POINT('Ctrl Pts',(-0.167219570451243,1.82445187487074,
6.01977193663774));
#51338=CARTESIAN_POINT('Ctrl Pts',(-0.171719484167394,1.82723348412446,
6.01947642355334));
#51339=CARTESIAN_POINT('Ctrl Pts',(-0.194915174171536,1.84237341179173,
6.017922588068));
#51340=CARTESIAN_POINT('Ctrl Pts',(-0.21234955954777,1.85654400640881,6.01664255370566));
#51341=CARTESIAN_POINT('Ctrl Pts',(-0.228982619826251,1.8732193732273,6.01521028728399));
#51342=CARTESIAN_POINT('Ctrl Pts',(-0.229788786618955,1.87403627204184,
6.01514030420375));
#51343=CARTESIAN_POINT('Ctrl Pts',(-0.230957840826026,1.87523361510915,
6.01503798373026));
#51344=CARTESIAN_POINT('Ctrl Pts',(-0.231324194338672,1.87561067511062,
6.01500579809776));
#51345=CARTESIAN_POINT('Ctrl Pts',(-0.231965136335691,1.87627358613908,
6.01494927540759));
#51346=CARTESIAN_POINT('Ctrl Pts',(-0.232240123869646,1.87655905120806,
6.01492495578768));
#51347=CARTESIAN_POINT('Ctrl Pts',(-0.232772764683201,1.87711403213526,
6.01487771439952));
#51348=CARTESIAN_POINT('Ctrl Pts',(-0.233030478376079,1.87738348939204,
6.01485479530534));
#51349=CARTESIAN_POINT('Ctrl Pts',(-0.233644207721466,1.87802741880968,
6.01480006691302));
#51350=CARTESIAN_POINT('Ctrl Pts',(-0.233999790721992,1.87840230023941,
6.01476823900474));
#51351=CARTESIAN_POINT('Ctrl Pts',(-0.235070999297314,1.87953709946738,
6.01467199357934));
#51352=CARTESIAN_POINT('Ctrl Pts',(-0.235783830624478,1.88029963496426,
6.0146074562905));
#51353=CARTESIAN_POINT('Ctrl Pts',(-0.243231301159998,1.88834439308857,
6.0139279708177));
#51354=CARTESIAN_POINT('Ctrl Pts',(-0.249629361385848,1.8959296471515,6.01329888364502));
#51355=CARTESIAN_POINT('Ctrl Pts',(-0.265389497456274,1.91646628861794,
6.01162228023401));
#51356=CARTESIAN_POINT('Ctrl Pts',(-0.274155777794372,1.92983915337881,
6.01055499286846));
#51357=CARTESIAN_POINT('Ctrl Pts',(-0.28945346325023,1.95744777940985,6.0084227322202));
#51358=CARTESIAN_POINT('Ctrl Pts',(-0.296012625978673,1.97162165460656,
6.00736126844103));
#51359=CARTESIAN_POINT('Ctrl Pts',(-0.303660631090676,1.99188819007557,
6.00592835565451));
#51360=CARTESIAN_POINT('Ctrl Pts',(-0.305641090502209,1.9976209205101,6.00553215993073));
#51361=CARTESIAN_POINT('Ctrl Pts',(-0.308417703654822,2.00645892476852,
6.00493858320126));
#51362=CARTESIAN_POINT('Ctrl Pts',(-0.309331217813061,2.00952562635994,
6.00473573256383));
#51363=CARTESIAN_POINT('Ctrl Pts',(-0.310338365460684,2.01310040933991,
6.00450328143803));
#51364=CARTESIAN_POINT('Ctrl Pts',(-0.310476598396289,2.01359559160164,
6.00447117085603));
#51365=CARTESIAN_POINT('Ctrl Pts',(-0.310685026021027,2.01434918604418,
6.00442244044864));
#51366=CARTESIAN_POINT('Ctrl Pts',(-0.310756083753009,2.01460735548816,
6.00440577063749));
#51367=CARTESIAN_POINT('Ctrl Pts',(-0.310884394583346,2.01507582010488,
6.00437556693913));
#51368=CARTESIAN_POINT('Ctrl Pts',(-0.310941755916316,2.01528608405448,
6.00436202677507));
#51369=CARTESIAN_POINT('Ctrl Pts',(-0.311056920752505,2.01570992565782,
6.00433476602475));
#51370=CARTESIAN_POINT('Ctrl Pts',(-0.311114717347823,2.0159235036949,6.00432104587656));
#51371=CARTESIAN_POINT('Ctrl Pts',(-0.311279850196348,2.01653622747345,
6.00428173257542));
#51372=CARTESIAN_POINT('Ctrl Pts',(-0.311386639094199,2.01693552226874,
6.00425617131675));
#51373=CARTESIAN_POINT('Ctrl Pts',(-0.31184742928036,2.01867184117808,6.0041452671306));
#51374=CARTESIAN_POINT('Ctrl Pts',(-0.312193596421089,2.02001095649239,
6.00406037223381));
#51375=CARTESIAN_POINT('Ctrl Pts',(-0.31897751323838,2.04696895907943,6.0023633848848));
#51376=CARTESIAN_POINT('Ctrl Pts',(-0.322251150394464,2.07328580773895,
6.00091967657762));
#51377=CARTESIAN_POINT('Ctrl Pts',(-0.322280469809755,2.10594897631948,
5.99908929551111));
#51378=CARTESIAN_POINT('Ctrl Pts',(-0.322104937854925,2.112185954157,5.99873841020408));
#51379=CARTESIAN_POINT('Ctrl Pts',(-0.320793648356167,2.13509843943699,
5.99743568333589));
#51380=CARTESIAN_POINT('Ctrl Pts',(-0.318542619957099,2.15168117635893,
5.99646440228957));
#51381=CARTESIAN_POINT('Ctrl Pts',(-0.314748459050056,2.16925457357357,
5.99537224748659));
#51382=CARTESIAN_POINT('Ctrl Pts',(-0.314473112307703,2.17049432600674,
5.99529486771595));
#51383=CARTESIAN_POINT('Ctrl Pts',(-0.314077656726483,2.17222643531318,
5.99518628253308));
#51384=CARTESIAN_POINT('Ctrl Pts',(-0.313963700776544,2.17272019666445,
5.99515527475656));
#51385=CARTESIAN_POINT('Ctrl Pts',(-0.313764468169048,2.17357425654713,
5.99510154612708));
#51386=CARTESIAN_POINT('Ctrl Pts',(-0.313679734047849,2.17393468169731,
5.99507884275521));
#51387=CARTESIAN_POINT('Ctrl Pts',(-0.313502646682352,2.17468215640289,
5.99503169809773));
#51388=CARTESIAN_POINT('Ctrl Pts',(-0.313410197371313,2.17506918238056,
5.99500725375206));
#51389=CARTESIAN_POINT('Ctrl Pts',(-0.313191710054619,2.17597640998326,
5.99494987381673));
#51390=CARTESIAN_POINT('Ctrl Pts',(-0.313065092673072,2.17649646962422,
5.99491691960107));
#51391=CARTESIAN_POINT('Ctrl Pts',(-0.312650611472097,2.17818061612235,
5.9948100000381));
#51392=CARTESIAN_POINT('Ctrl Pts',(-0.312357548481293,2.17934340196638,
5.99473586708172));
#51393=CARTESIAN_POINT('Ctrl Pts',(-0.308566050590067,2.194040308164,5.99379485257451));
#51394=CARTESIAN_POINT('Ctrl Pts',(-0.304197626761239,2.20733263945151,
5.99289954700486));
#51395=CARTESIAN_POINT('Ctrl Pts',(-0.292819429928974,2.23561126620143,
5.99089506870974));
#51396=CARTESIAN_POINT('Ctrl Pts',(-0.285491080960554,2.25042736661268,
5.98977897714405));
#51397=CARTESIAN_POINT('Ctrl Pts',(-0.267166092671871,2.28126974924426,
5.98735155126453));
#51398=CARTESIAN_POINT('Ctrl Pts',(-0.255788347070542,2.29699988415692,
5.98604459277556));
#51399=CARTESIAN_POINT('Ctrl Pts',(-0.242347743162633,2.31243808630275,
5.98475490369902));
#51400=CARTESIAN_POINT('Ctrl Pts',(-0.241626197965943,2.31325841053967,
5.98468635928188));
#51401=CARTESIAN_POINT('Ctrl Pts',(-0.240650576329608,2.31435628583397,
5.98459462144937));
#51402=CARTESIAN_POINT('Ctrl Pts',(-0.240400175807708,2.31463707191295,
5.98457115895934));
#51403=CARTESIAN_POINT('Ctrl Pts',(-0.240006716806598,2.31507672402036,
5.98453442227436));
#51404=CARTESIAN_POINT('Ctrl Pts',(-0.239863991975023,2.31523588613906,
5.98452112305604));
#51405=CARTESIAN_POINT('Ctrl Pts',(-0.239589229170906,2.31554168001766,
5.9844955720926));
#51406=CARTESIAN_POINT('Ctrl Pts',(-0.239457215891181,2.31568833143547,
5.98448331869795));
#51407=CARTESIAN_POINT('Ctrl Pts',(-0.239143346022571,2.31603636106496,
5.98445423965154));
#51408=CARTESIAN_POINT('Ctrl Pts',(-0.238961369928544,2.31623763070342,
5.98443742320047));
#51409=CARTESIAN_POINT('Ctrl Pts',(-0.238422384903588,2.31683224893654,
5.98438774179642));
#51410=CARTESIAN_POINT('Ctrl Pts',(-0.238064655185021,2.3172249473775,5.98435493121354));
#51411=CARTESIAN_POINT('Ctrl Pts',(-0.235242868563442,2.3203072259192,5.98409738544989));
#51412=CARTESIAN_POINT('Ctrl Pts',(-0.232734156049585,2.32295581704951,
5.98387597818845));
#51413=CARTESIAN_POINT('Ctrl Pts',(-0.223654953127177,2.33222096258806,
5.9830986238959));
#51414=CARTESIAN_POINT('Ctrl Pts',(-0.216842491176209,2.33859479822104,
5.98255849530007));
#51415=CARTESIAN_POINT('Ctrl Pts',(-0.202823565989846,2.35061388665305,
5.98150648290134));
#51416=CARTESIAN_POINT('Ctrl Pts',(-0.195634323301723,2.35626537271202,
5.98099471313661));
#51417=CARTESIAN_POINT('Ctrl Pts',(-0.171817592218757,2.37340064265486,
5.9793542666704));
#51418=CARTESIAN_POINT('Ctrl Pts',(-0.154349536410973,2.38362886316792,
5.97822903294836));
#51419=CARTESIAN_POINT('Ctrl Pts',(-0.134316469745295,2.39295712208554,
5.97693582857045));
#51420=CARTESIAN_POINT('Ctrl Pts',(-0.132586098954645,2.39374430306898,
5.97682413904472));
#51421=CARTESIAN_POINT('Ctrl Pts',(-0.124735168498417,2.39723234825744,
5.97631725263981));
#51422=CARTESIAN_POINT('Ctrl Pts',(-0.118538725756981,2.39975738815499,
5.97591676848745));
#51423=CARTESIAN_POINT('Ctrl Pts',(-0.11129224617215,2.40245048573662,5.97544628802601));
#51424=CARTESIAN_POINT('Ctrl Pts',(-0.110314226952202,2.40280857265338,
5.97538274680311));
#51425=CARTESIAN_POINT('Ctrl Pts',(-0.108859218324699,2.40333331746174,
5.97528814623771));
#51426=CARTESIAN_POINT('Ctrl Pts',(-0.108383538341173,2.40350360707685,
5.97525720784803));
#51427=CARTESIAN_POINT('Ctrl Pts',(-0.107536712262193,2.40380451930862,
5.97520210964551));
#51428=CARTESIAN_POINT('Ctrl Pts',(-0.107165722875459,2.40393558244291,
5.97517796452618));
#51429=CARTESIAN_POINT('Ctrl Pts',(-0.10638536511117,2.40420966084493,5.97512716149948));
#51430=CARTESIAN_POINT('Ctrl Pts',(-0.10597594651758,2.4043525298367,5.97510049879563));
#51431=CARTESIAN_POINT('Ctrl Pts',(-0.104898844066915,2.40472595409132,
5.97503033093204));
#51432=CARTESIAN_POINT('Ctrl Pts',(-0.104230691092841,2.40495514031584,
5.97498678052436));
#51433=CARTESIAN_POINT('Ctrl Pts',(-0.101251338948475,2.40596616628005,
5.97479247610219));
#51434=CARTESIAN_POINT('Ctrl Pts',(-0.0989321074319765,2.4067239249546,
5.97464092926571));
#51435=CARTESIAN_POINT('Ctrl Pts',(-0.0819774272182834,2.41205120143762,
5.97353066866323));
#51436=CARTESIAN_POINT('Ctrl Pts',(-0.0670431956381767,2.41559679751256,
5.97253841466143));
#51437=CARTESIAN_POINT('Ctrl Pts',(-0.0198712624586704,2.42329627054299,
5.96936576727488));
#51438=CARTESIAN_POINT('Ctrl Pts',(0.0127766637380169,2.42365415414283,
5.96709745798501));
#51439=CARTESIAN_POINT('Ctrl Pts',(0.0463915859274049,2.41892191238083,
5.96495081979399));
#51440=CARTESIAN_POINT('Ctrl Pts',(0.0478555348947601,2.418705527754,5.96485775813468));
#51441=CARTESIAN_POINT('Ctrl Pts',(0.0497372436924342,2.41841413633344,
5.96473873342076));
#51442=CARTESIAN_POINT('Ctrl Pts',(0.050156387219199,2.41834838220591,5.96471225906882));
#51443=CARTESIAN_POINT('Ctrl Pts',(0.0508205663555086,2.41824284325534,
5.96467036904285));
#51444=CARTESIAN_POINT('Ctrl Pts',(0.0510656860861607,2.41820360298634,
5.96465492253723));
#51445=CARTESIAN_POINT('Ctrl Pts',(0.0515049839696522,2.41813275680895,
5.96462726379184));
#51446=CARTESIAN_POINT('Ctrl Pts',(0.0516991771013884,2.41810125654566,
5.96461504563065));
#51447=CARTESIAN_POINT('Ctrl Pts',(0.052155874544087,2.41802674593969,5.96458633118205));
#51448=CARTESIAN_POINT('Ctrl Pts',(0.0524183541499164,2.41798358846312,
5.9645698434049));
#51449=CARTESIAN_POINT('Ctrl Pts',(0.0531797206979818,2.41785743456257,
5.96452206170778));
#51450=CARTESIAN_POINT('Ctrl Pts',(0.0536784689623207,2.41777358823274,
5.96449081605724));
#51451=CARTESIAN_POINT('Ctrl Pts',(0.0571397491327742,2.41718331879781,
5.96427434027958));
#51452=CARTESIAN_POINT('Ctrl Pts',(0.0600953926362167,2.41663662770907,
5.96409135548428));
#51453=CARTESIAN_POINT('Ctrl Pts',(0.0692896417962748,2.41480262583709,
5.9635267581205));
#51454=CARTESIAN_POINT('Ctrl Pts',(0.0754983272270876,2.41337160280435,
5.96315216030322));
#51455=CARTESIAN_POINT('Ctrl Pts',(0.0969192142704502,2.40776067135472,
5.96187032881164));
#51456=CARTESIAN_POINT('Ctrl Pts',(0.111864507978248,2.4026489085701,5.96099399972733));
#51457=CARTESIAN_POINT('Ctrl Pts',(0.149486696795473,2.38661132924035,5.95870712660777));
#51458=CARTESIAN_POINT('Ctrl Pts',(0.171362192526894,2.37409317631907,5.95728915670301));
#51459=CARTESIAN_POINT('Ctrl Pts',(0.192758675081555,2.35827792592324,5.95567521945505));
#51460=CARTESIAN_POINT('Ctrl Pts',(0.193950208734088,2.35738436287842,5.95558455959877));
#51461=CARTESIAN_POINT('Ctrl Pts',(0.195567120419863,2.35615419414918,5.95546044452395));
#51462=CARTESIAN_POINT('Ctrl Pts',(0.195997918702762,2.35582471660894,5.95542726973295));
#51463=CARTESIAN_POINT('Ctrl Pts',(0.196728973389977,2.35526267039162,5.95537079059267));
#51464=CARTESIAN_POINT('Ctrl Pts',(0.197029655144076,2.35503065474241,5.95534750812562));
#51465=CARTESIAN_POINT('Ctrl Pts',(0.197634769294365,2.35456202045618,5.95530054611185));
#51466=CARTESIAN_POINT('Ctrl Pts',(0.197939188567127,2.35432538591369,5.9552768659565));
#51467=CARTESIAN_POINT('Ctrl Pts',(0.198630086993066,2.35378633727417,5.9552229976437));
#51468=CARTESIAN_POINT('Ctrl Pts',(0.19901630085039,2.35348358613033,5.95519279610282));
#51469=CARTESIAN_POINT('Ctrl Pts',(0.199822355441396,2.35284874617137,5.95512957622368));
#51470=CARTESIAN_POINT('Ctrl Pts',(0.200242062958403,2.35251649132525,5.9550965512988));
#51471=CARTESIAN_POINT('Ctrl Pts',(0.201339898443672,2.35164294897854,5.95500988606244));
#51472=CARTESIAN_POINT('Ctrl Pts',(0.20201666823648,2.35109996855222,5.95495617787136));
#51473=CARTESIAN_POINT('Ctrl Pts',(0.204019806043015,2.3494794873847,5.95479636242501));
#51474=CARTESIAN_POINT('Ctrl Pts',(0.2053397895926,2.34839417568146,5.95468994029806));
#51475=CARTESIAN_POINT('Ctrl Pts',(0.219751845991815,2.33635096671437,5.95351558082101));
#51476=CARTESIAN_POINT('Ctrl Pts',(0.231959863109446,2.32438161509491,5.95240517867696));
#51477=CARTESIAN_POINT('Ctrl Pts',(0.26169602417353,2.29019459162271,5.94938181885288));
#51478=CARTESIAN_POINT('Ctrl Pts',(0.277348821603544,2.26654253993711,5.94742428259788));
#51479=CARTESIAN_POINT('Ctrl Pts',(0.291255757088953,2.23799846794826,5.94538451040464));
#51480=CARTESIAN_POINT('Ctrl Pts',(0.292741384938226,2.23481831193916,5.94516157700682));
#51481=CARTESIAN_POINT('Ctrl Pts',(0.294408049282037,2.23109310524211,5.94490595951939));
#51482=CARTESIAN_POINT('Ctrl Pts',(0.294639877845851,2.23057122239967,5.94487027366271));
#51483=CARTESIAN_POINT('Ctrl Pts',(0.294983088645123,2.22979303190937,5.94481725053138));
#51484=CARTESIAN_POINT('Ctrl Pts',(0.295095525055178,2.22953719470743,5.94479984901571));
#51485=CARTESIAN_POINT('Ctrl Pts',(0.295295439818329,2.22908069864701,5.94476885356888));
#51486=CARTESIAN_POINT('Ctrl Pts',(0.295383046435053,2.22888009706898,5.94475525174929));
#51487=CARTESIAN_POINT('Ctrl Pts',(0.295568862161798,2.22845343161714,5.94472636158116));
#51488=CARTESIAN_POINT('Ctrl Pts',(0.295667016053899,2.22822734494873,5.94471107666885));
#51489=CARTESIAN_POINT('Ctrl Pts',(0.295930278788776,2.22761903883301,5.9446700145525));
#51490=CARTESIAN_POINT('Ctrl Pts',(0.296094907169749,2.22723661002017,5.94464426681456));
#51491=CARTESIAN_POINT('Ctrl Pts',(0.296886350987121,2.22538824537119,5.94452014105262));
#51492=CARTESIAN_POINT('Ctrl Pts',(0.297503037678857,2.22391795792926,5.94442237215243));
#51493=CARTESIAN_POINT('Ctrl Pts',(0.30259505039819,2.2115205784368,5.94360560637735));
#51494=CARTESIAN_POINT('Ctrl Pts',(0.306478168540586,2.20035837091534,5.94291963772146));
#51495=CARTESIAN_POINT('Ctrl Pts',(0.318341698799888,2.15907383377874,5.94047450910394));
#51496=CARTESIAN_POINT('Ctrl Pts',(0.322558887653065,2.12805354962461,5.938792774593));
#51497=CARTESIAN_POINT('Ctrl Pts',(0.322196875576618,2.09030905245233,5.9365647005873));
#51498=CARTESIAN_POINT('Ctrl Pts',(0.32193083116601,2.08371284050106,5.93616947414742));
#51499=CARTESIAN_POINT('Ctrl Pts',(0.321388863541718,2.07609497404383,5.9357046766006));
#51500=CARTESIAN_POINT('Ctrl Pts',(0.321310247240895,2.07506053622989,5.93564138366107));
#51501=CARTESIAN_POINT('Ctrl Pts',(0.321185984072488,2.07352371415354,5.93554708193351));
#51502=CARTESIAN_POINT('Ctrl Pts',(0.321144149535001,2.07302102129983,5.93551619297808));
#51503=CARTESIAN_POINT('Ctrl Pts',(0.321068297467126,2.07213474784566,5.93546165762858));
#51504=CARTESIAN_POINT('Ctrl Pts',(0.321034772239056,2.07175112520049,5.93543802675674));
#51505=CARTESIAN_POINT('Ctrl Pts',(0.320978950135475,2.0711252990556,5.93539943475082));
#51506=CARTESIAN_POINT('Ctrl Pts',(0.320957066428401,2.07088305830175,5.93538448663814));
#51507=CARTESIAN_POINT('Ctrl Pts',(0.320886475169926,2.07011140129722,5.93533683694479));
#51508=CARTESIAN_POINT('Ctrl Pts',(0.32083673197218,2.0695820827241,5.93530410280659));
#51509=CARTESIAN_POINT('Ctrl Pts',(0.320728813819431,2.06846344513909,5.93523481985232));
#51510=CARTESIAN_POINT('Ctrl Pts',(0.320670323927075,2.06787415913122,5.93519826122022));
#51511=CARTESIAN_POINT('Ctrl Pts',(0.320508231973931,2.06628564010189,5.93509954486852));
#51512=CARTESIAN_POINT('Ctrl Pts',(0.320401581985314,2.06528673090893,5.93503729130609));
#51513=CARTESIAN_POINT('Ctrl Pts',(0.320059188162592,2.06221587322731,5.93484535594972));
#51514=CARTESIAN_POINT('Ctrl Pts',(0.319808006812089,2.0601457328145,5.93471518963316));
#51515=CARTESIAN_POINT('Ctrl Pts',(0.318809805718197,2.05253723199526,5.93423384800152));
#51516=CARTESIAN_POINT('Ctrl Pts',(0.317938890031717,2.04701639357965,5.93387882298313));
#51517=CARTESIAN_POINT('Ctrl Pts',(0.315646134731852,2.03459083195782,5.93306639739291));
#51518=CARTESIAN_POINT('Ctrl Pts',(0.314140434454107,2.02770464798979,5.93260667301109));
#51519=CARTESIAN_POINT('Ctrl Pts',(0.30393310534402,1.98740356213598,5.92986235944173));
#51520=CARTESIAN_POINT('Ctrl Pts',(0.29013392484836,1.95551699005566,5.92744024977939));
#51521=CARTESIAN_POINT('Ctrl Pts',(0.270843158176367,1.92533794121575,5.92517912198665));
#51522=CARTESIAN_POINT('Ctrl Pts',(0.270139436771538,1.92425149802984,5.925097807124));
#51523=CARTESIAN_POINT('Ctrl Pts',(0.269208202228769,1.92283261681688,5.92499175440138));
#51524=CARTESIAN_POINT('Ctrl Pts',(0.268986597510482,1.92249634320628,5.92496663063386));
#51525=CARTESIAN_POINT('Ctrl Pts',(0.268643444793574,1.92197774518707,5.92492790254007));
#51526=CARTESIAN_POINT('Ctrl Pts',(0.268522341214268,1.92179512939111,5.92491426844442));
#51527=CARTESIAN_POINT('Ctrl Pts',(0.268280286740075,1.92143093501072,5.92488708464774));
#51528=CARTESIAN_POINT('Ctrl Pts',(0.268159338552588,1.92124935700265,5.92487353499762));
#51529=CARTESIAN_POINT('Ctrl Pts',(0.267887485681955,1.92084212456348,5.92484315436187));
#51530=CARTESIAN_POINT('Ctrl Pts',(0.267736480586475,1.92061653844238,5.92482633032064));
#51531=CARTESIAN_POINT('Ctrl Pts',(0.267288810770249,1.91994959019485,5.92477660464376));
#51532=CARTESIAN_POINT('Ctrl Pts',(0.266991336582043,1.91950876854076,5.92474375752465));
#51533=CARTESIAN_POINT('Ctrl Pts',(0.264635364772894,1.91603606600753,5.92448512958724));
#51534=CARTESIAN_POINT('Ctrl Pts',(0.26252627535475,1.91303860604383,5.92426270821507));
#51535=CARTESIAN_POINT('Ctrl Pts',(0.254826313706799,1.90248265486284,5.92347983189168));
#51536=CARTESIAN_POINT('Ctrl Pts',(0.248956048744244,1.89513304706535,5.92293546255686));
#51537=CARTESIAN_POINT('Ctrl Pts',(0.240214227597833,1.88511996399137,5.92217846587377));
#51538=CARTESIAN_POINT('Ctrl Pts',(0.237603242617463,1.88223635465301,5.92195854345257));
#51539=CARTESIAN_POINT('Ctrl Pts',(0.223202400523936,1.86689930359885,5.9207741241878));
#51540=CARTESIAN_POINT('Ctrl Pts',(0.2104852581215,1.85535494589176,5.91982723580088));
#51541=CARTESIAN_POINT('Ctrl Pts',(0.183908419261698,1.83484229327832,5.91791995835766));
#51542=CARTESIAN_POINT('Ctrl Pts',(0.170160638361421,1.82581729145374,5.9169645702399));
#51543=CARTESIAN_POINT('Ctrl Pts',(0.154677802223691,1.81726769444894,5.91589011279933));
#51544=CARTESIAN_POINT('Ctrl Pts',(0.153565708197699,1.81666212343355,5.91581295591814));
#51545=CARTESIAN_POINT('Ctrl Pts',(0.152004181626461,1.81582371572771,5.91570463324324));
#51546=CARTESIAN_POINT('Ctrl Pts',(0.151557715509892,1.81558535438634,5.91567366381129));
#51547=CARTESIAN_POINT('Ctrl Pts',(0.150783807351327,1.81517451653371,5.91561998349051));
#51548=CARTESIAN_POINT('Ctrl Pts',(0.150456625356693,1.81500155004704,5.91559729000737));
#51549=CARTESIAN_POINT('Ctrl Pts',(0.149784034438824,1.81464746231234,5.91555063996773));
#51550=CARTESIAN_POINT('Ctrl Pts',(0.149438593308637,1.8144664037886,5.91552668123942));
#51551=CARTESIAN_POINT('Ctrl Pts',(0.14863175401872,1.81404537458357,5.91547072238281));
#51552=CARTESIAN_POINT('Ctrl Pts',(0.148170102946865,1.81380589333917,5.91543870505292));
#51553=CARTESIAN_POINT('Ctrl Pts',(0.147195913044414,1.81330352179404,5.91537114187637));
#51554=CARTESIAN_POINT('Ctrl Pts',(0.14668324550012,1.81304088633512,5.91533558718313));
#51555=CARTESIAN_POINT('Ctrl Pts',(0.145309441885275,1.81234174126003,5.91524031041911));
#51556=CARTESIAN_POINT('Ctrl Pts',(0.144447048815092,1.81190772697215,5.91518050097489));
#51557=CARTESIAN_POINT('Ctrl Pts',(0.141813698011413,1.8105972440271,5.91499786258184));
#51558=CARTESIAN_POINT('Ctrl Pts',(0.140036643444441,1.8097331945932,5.91487460219325));
#51559=CARTESIAN_POINT('Ctrl Pts',(0.133558834654711,1.80665684898303,5.91442518824468));
#51560=CARTESIAN_POINT('Ctrl Pts',(0.128812910809411,1.8045420578942,5.91409572371327));
#51561=CARTESIAN_POINT('Ctrl Pts',(0.117912560090552,1.79999739637808,5.91333825560152));
#51562=CARTESIAN_POINT('Ctrl Pts',(0.111730389756813,1.79764053745451,5.91290809901338));
#51563=CARTESIAN_POINT('Ctrl Pts',(0.0898216704454556,1.79005184795571,
5.91138272337882));
#51564=CARTESIAN_POINT('Ctrl Pts',(0.0737690610956677,1.78584425642561,
5.91026178316174));
#51565=CARTESIAN_POINT('Ctrl Pts',(0.0386575877370288,1.77948147245121,
5.90784752432679));
#51566=CARTESIAN_POINT('Ctrl Pts',(0.0195810999141629,1.77775273338049,
5.90655871763368));
#51567=CARTESIAN_POINT('Ctrl Pts',(-0.00067661604709986,1.77772369924387,
5.90528177230881));
#51568=CARTESIAN_POINT('Ctrl Pts',(-0.00181514948180812,1.77772810056933,
5.90521031844886));
#51569=CARTESIAN_POINT('Ctrl Pts',(-0.00333633254758036,1.77774204282283,
5.90511529014557));
#51570=CARTESIAN_POINT('Ctrl Pts',(-0.00371900521102961,1.77774623185643,
5.9050914218328));
#51571=CARTESIAN_POINT('Ctrl Pts',(-0.00431673729365212,1.77775383995341,
5.90505419883373));
#51572=CARTESIAN_POINT('Ctrl Pts',(-0.00453180069685644,1.77775679267247,
5.90504081799572));
#51573=CARTESIAN_POINT('Ctrl Pts',(-0.00494384746416748,1.77776286246143,
5.90501520434944));
#51574=CARTESIAN_POINT('Ctrl Pts',(-0.0051408295034581,1.77776594483344,
5.90500296970853));
#51575=CARTESIAN_POINT('Ctrl Pts',(-0.00560642471079884,1.77777365750069,
5.90497407526306));
#51576=CARTESIAN_POINT('Ctrl Pts',(-0.00587503466236217,1.77777844304346,
5.90495742431161));
#51577=CARTESIAN_POINT('Ctrl Pts',(-0.006661859954345,1.77779344529164,
5.90490870366227));
#51578=CARTESIAN_POINT('Ctrl Pts',(-0.00718006010154157,1.77780457635019,
5.90487668520465));
#51579=CARTESIAN_POINT('Ctrl Pts',(-0.0110002526933215,1.77789585595836,
5.90464113614396));
#51580=CARTESIAN_POINT('Ctrl Pts',(-0.0143010184661592,1.77802551638261,
5.90444032608791));
#51581=CARTESIAN_POINT('Ctrl Pts',(-0.0252021534360486,1.77862171443231,
5.90378438381918));
#51582=CARTESIAN_POINT('Ctrl Pts',(-0.0327884255692302,1.77930686316088,
5.90333955409475));
#51583=CARTESIAN_POINT('Ctrl Pts',(-0.048701459578559,1.78131472395007,
5.90241798501008));
#51584=CARTESIAN_POINT('Ctrl Pts',(-0.0570148664733614,1.78269659004878,
5.90194321083976));
#51585=CARTESIAN_POINT('Ctrl Pts',(-0.0679019689247061,1.78494802029648,
5.90132001395504));
#51586=CARTESIAN_POINT('Ctrl Pts',(-0.0705321362106861,1.78552639987211,
5.90116935253939));
#51587=CARTESIAN_POINT('Ctrl Pts',(-0.0819974202267397,1.78819871822848,
5.90051110452581));
#51588=CARTESIAN_POINT('Ctrl Pts',(-0.0907489467655755,1.79063251411109,
5.90000464139583));
#51589=CARTESIAN_POINT('Ctrl Pts',(-0.117835699815279,1.79941375014011,
5.89839925779277));
#51590=CARTESIAN_POINT('Ctrl Pts',(-0.135705014915195,1.8070472301034,5.89728159624567));
#51591=CARTESIAN_POINT('Ctrl Pts',(-0.153916945577696,1.81685265044588,
5.89602528760817));
#51592=CARTESIAN_POINT('Ctrl Pts',(-0.155051783402283,1.81747249322744,
5.89594650745762));
#51593=CARTESIAN_POINT('Ctrl Pts',(-0.156629550318885,1.81834663079213,
5.89583627418678));
#51594=CARTESIAN_POINT('Ctrl Pts',(-0.157075662291097,1.81859517998031,
5.89580502674775));
#51595=CARTESIAN_POINT('Ctrl Pts',(-0.157845084446694,1.81902625961212,
5.89575099583474));
#51596=CARTESIAN_POINT('Ctrl Pts',(-0.158168674379394,1.81920829087252,
5.89572823031501));
#51597=CARTESIAN_POINT('Ctrl Pts',(-0.158830932280142,1.81958234337956,
5.89568155170728));
#51598=CARTESIAN_POINT('Ctrl Pts',(-0.159169568217506,1.81977441989558,
5.89565763665518));
#51599=CARTESIAN_POINT('Ctrl Pts',(-0.15995575866852,1.82022223711906,5.89560200563611));
#51600=CARTESIAN_POINT('Ctrl Pts',(-0.16040304837092,1.82047843839467,5.89557027308259));
#51601=CARTESIAN_POINT('Ctrl Pts',(-0.161343566306664,1.82102015479653,
5.89550337467035));
#51602=CARTESIAN_POINT('Ctrl Pts',(-0.161836655254916,1.82130590708175,
5.89546820029038));
#51603=CARTESIAN_POINT('Ctrl Pts',(-0.163150253157912,1.82207181807494,
5.89537422304531));
#51604=CARTESIAN_POINT('Ctrl Pts',(-0.163969395150256,1.82255429930054,
5.89531533590432));
#51605=CARTESIAN_POINT('Ctrl Pts',(-0.16644935368748,1.82402983359876,5.89513618307501));
#51606=CARTESIAN_POINT('Ctrl Pts',(-0.168103348797263,1.82503421313449,
5.89501550500858));
#51607=CARTESIAN_POINT('Ctrl Pts',(-0.174041054638061,1.82871345111793,
5.89457789583224));
#51608=CARTESIAN_POINT('Ctrl Pts',(-0.178270611938832,1.83147390330209,
5.89425784224812));
#51609=CARTESIAN_POINT('Ctrl Pts',(-0.192682497592627,1.84137051750531,
5.89313756238466));
#51610=CARTESIAN_POINT('Ctrl Pts',(-0.202514669711804,1.84899501149601,
5.89231987447261));
#51611=CARTESIAN_POINT('Ctrl Pts',(-0.230444874012216,1.87336523848365,
5.88984146873517));
#51612=CARTESIAN_POINT('Ctrl Pts',(-0.247089556813021,1.89163758085672,
5.88814351750745));
#51613=CARTESIAN_POINT('Ctrl Pts',(-0.262043626896891,1.91239613418237,
5.88647352223353));
#51614=CARTESIAN_POINT('Ctrl Pts',(-0.262593904793257,1.91316714937911,
5.8864118434075));
#51615=CARTESIAN_POINT('Ctrl Pts',(-0.263208974171841,1.91403703193323,
5.88634265559898));
#51616=CARTESIAN_POINT('Ctrl Pts',(-0.263277114147539,1.91413351366381,
5.88633498725024));
#51617=CARTESIAN_POINT('Ctrl Pts',(-0.264038756012179,1.91521320772448,
5.88624923522975));
#51618=CARTESIAN_POINT('Ctrl Pts',(-0.264726809884665,1.91620027342262,
5.88617141342366));
#51619=CARTESIAN_POINT('Ctrl Pts',(-0.267660306862063,1.92045924452959,
5.88583816182218));
#51620=CARTESIAN_POINT('Ctrl Pts',(-0.269850860759941,1.92376879036839,
5.88558558128835));
#51621=CARTESIAN_POINT('Ctrl Pts',(-0.272297556971187,1.92761796247287,
5.88529982723488));
#51622=CARTESIAN_POINT('Ctrl Pts',(-0.272613893620358,1.92811867055181,
5.88526280920225));
#51623=CARTESIAN_POINT('Ctrl Pts',(-0.273079692903399,1.92886047385743,
5.88520819655203));
#51624=CARTESIAN_POINT('Ctrl Pts',(-0.27323021814581,1.92910089532711,5.88519053196105));
#51625=CARTESIAN_POINT('Ctrl Pts',(-0.273496599953841,1.92952761640603,
5.88515924280856));
#51626=CARTESIAN_POINT('Ctrl Pts',(-0.273612583707076,1.92971383558029,
5.88514560978239));
#51627=CARTESIAN_POINT('Ctrl Pts',(-0.273857197190315,1.93010747297492,
5.88511683710837));
#51628=CARTESIAN_POINT('Ctrl Pts',(-0.273985781126848,1.93031491835414,
5.88510170052476));
#51629=CARTESIAN_POINT('Ctrl Pts',(-0.274327421485821,1.93086748996669,
5.88506145119716));
#51630=CARTESIAN_POINT('Ctrl Pts',(-0.274540063124544,1.93121287408965,
5.88503636592523));
#51631=CARTESIAN_POINT('Ctrl Pts',(-0.275525158899786,1.93281970700101,
5.88491999366527));
#51632=CARTESIAN_POINT('Ctrl Pts',(-0.276289590659075,1.93408608905652,
5.88482922745906));
#51633=CARTESIAN_POINT('Ctrl Pts',(-0.282310292381125,1.94421718692567,
5.88411025696604));
#51634=CARTESIAN_POINT('Ctrl Pts',(-0.287147891904193,1.95332511813037,
5.88350729218234));
#51635=CARTESIAN_POINT('Ctrl Pts',(-0.306204172725652,1.99377431072008,
5.8809456550762));
#51636=CARTESIAN_POINT('Ctrl Pts',(-0.315788783613521,2.02704416444801,
5.87910369313275));
#51637=CARTESIAN_POINT('Ctrl Pts',(-0.320206132894077,2.06347018716599,
5.87692213068112));
#51638=CARTESIAN_POINT('Ctrl Pts',(-0.320457034050766,2.06574093252718,
5.87678560364946));
#51639=CARTESIAN_POINT('Ctrl Pts',(-0.320755003572805,2.06872831208986,
5.87660521435884));
#51640=CARTESIAN_POINT('Ctrl Pts',(-0.320823853346949,2.0694427440234,5.87656201615699));
#51641=CARTESIAN_POINT('Ctrl Pts',(-0.321121195060537,2.07263998764373,
5.8763684272592));
#51642=CARTESIAN_POINT('Ctrl Pts',(-0.321323251534889,2.07512511954268,
5.87621723427553));
#51643=CARTESIAN_POINT('Ctrl Pts',(-0.321548093505174,2.07835394040362,
5.87601978042419));
#51644=CARTESIAN_POINT('Ctrl Pts',(-0.321597171993456,2.07909575918394,
5.87597434615416));
#51645=CARTESIAN_POINT('Ctrl Pts',(-0.321671330922924,2.08027879852576,
5.875901775465));
#51646=CARTESIAN_POINT('Ctrl Pts',(-0.32169807158383,2.08071991541829,5.87587469119563));
#51647=CARTESIAN_POINT('Ctrl Pts',(-0.321746424284328,2.08154566461543,
5.87582394341814));
#51648=CARTESIAN_POINT('Ctrl Pts',(-0.321768254164313,2.08193028378087,
5.87580028679091));
#51649=CARTESIAN_POINT('Ctrl Pts',(-0.32181009389795,2.08269158074132,5.87575342358687));
#51650=CARTESIAN_POINT('Ctrl Pts',(-0.321830132164343,2.08306825641006,
5.87573021794098));
#51651=CARTESIAN_POINT('Ctrl Pts',(-0.321873936934282,2.0839198730813,5.87567771046431));
#51652=CARTESIAN_POINT('Ctrl Pts',(-0.321897313598774,2.08439483248053,
5.875648396445));
#51653=CARTESIAN_POINT('Ctrl Pts',(-0.321953706390739,2.08559468410446,
5.87557426672389));
#51654=CARTESIAN_POINT('Ctrl Pts',(-0.321985325483628,2.0863196365478,5.87552940728699));
#51655=CARTESIAN_POINT('Ctrl Pts',(-0.322189741514093,2.09140055695314,
5.87521450568765));
#51656=CARTESIAN_POINT('Ctrl Pts',(-0.32227657842632,2.09575931995697,5.87494178447891));
#51657=CARTESIAN_POINT('Ctrl Pts',(-0.322274978285881,2.10011830399491,
5.87466631836037));
#51658=CARTESIAN_POINT('',(-0.322274906241924,2.09975417128097,5.62420562594364));
#51659=CARTESIAN_POINT('Ctrl Pts',(-0.322274978376309,2.10011805739837,
5.87466633394405));
#51660=CARTESIAN_POINT('Ctrl Pts',(-0.322261304025871,2.13744651840769,
5.8723073616825));
#51661=CARTESIAN_POINT('Ctrl Pts',(-0.315761043457354,2.17448876595038,
5.86971828307802));
#51662=CARTESIAN_POINT('Ctrl Pts',(-0.300912371558147,2.21555646760403,
5.86682882722654));
#51663=CARTESIAN_POINT('Ctrl Pts',(-0.29857535205361,2.22146737439975,5.86641374952161));
#51664=CARTESIAN_POINT('Ctrl Pts',(-0.294885459834669,2.23004866868408,
5.86581614266381));
#51665=CARTESIAN_POINT('Ctrl Pts',(-0.293667886671735,2.23277524073928,
5.86562702548014));
#51666=CARTESIAN_POINT('Ctrl Pts',(-0.292200300874887,2.2359426889284,5.86540856071013));
#51667=CARTESIAN_POINT('Ctrl Pts',(-0.291986981329614,2.23640026849944,
5.8653770309333));
#51668=CARTESIAN_POINT('Ctrl Pts',(-0.291659704673618,2.23709800491725,
5.86532900151759));
#51669=CARTESIAN_POINT('Ctrl Pts',(-0.291546525466425,2.23733852253563,
5.86531245405373));
#51670=CARTESIAN_POINT('Ctrl Pts',(-0.291349071535339,2.23775678871357,
5.86528369330924));
#51671=CARTESIAN_POINT('Ctrl Pts',(-0.291264931875615,2.23793459965273,
5.86527147167055));
#51672=CARTESIAN_POINT('Ctrl Pts',(-0.291074185448169,2.23833674812616,
5.86524384172069));
#51673=CARTESIAN_POINT('Ctrl Pts',(-0.290967482330296,2.23856103905428,
5.86522843953113));
#51674=CARTESIAN_POINT('Ctrl Pts',(-0.290677546210389,2.23916867564697,
5.86518673361925));
#51675=CARTESIAN_POINT('Ctrl Pts',(-0.290493813421313,2.23955178437082,
5.86516046098384));
#51676=CARTESIAN_POINT('Ctrl Pts',(-0.289664334448925,2.24127262822696,
5.8650425462129));
#51677=CARTESIAN_POINT('Ctrl Pts',(-0.28901008841467,2.24260628012699,5.8649514246738));
#51678=CARTESIAN_POINT('Ctrl Pts',(-0.274952990325081,2.27076694888698,
5.86303192766152));
#51679=CARTESIAN_POINT('Ctrl Pts',(-0.257877352000274,2.29560280651141,
5.86141750102764));
#51680=CARTESIAN_POINT('Ctrl Pts',(-0.229374123297901,2.32670972971249,
5.85903797497653));
#51681=CARTESIAN_POINT('Ctrl Pts',(-0.220635648190775,2.33522258016575,
5.85834120709332));
#51682=CARTESIAN_POINT('Ctrl Pts',(-0.207655895312586,2.34650618596164,
5.85732981479167));
#51683=CARTESIAN_POINT('Ctrl Pts',(-0.203799303392252,2.3497040458331,5.8570320585353));
#51684=CARTESIAN_POINT('Ctrl Pts',(-0.198360977815014,2.35400353941477,
5.85661499626325));
#51685=CARTESIAN_POINT('Ctrl Pts',(-0.196841436312936,2.35518292313665,
5.85649875984245));
#51686=CARTESIAN_POINT('Ctrl Pts',(-0.194558575559887,2.35692222978957,
5.85632452821828));
#51687=CARTESIAN_POINT('Ctrl Pts',(-0.19380318130861,2.35749252099592,5.85626693894956));
#51688=CARTESIAN_POINT('Ctrl Pts',(-0.19259033178475,2.35839981143192,5.85617457089869));
#51689=CARTESIAN_POINT('Ctrl Pts',(-0.192134474652336,2.35873894582878,
5.85613987542671));
#51690=CARTESIAN_POINT('Ctrl Pts',(-0.191264902430163,2.35938229783766,
5.85607373182171));
#51691=CARTESIAN_POINT('Ctrl Pts',(-0.190851351972392,2.35968673585428,
5.85604229238287));
#51692=CARTESIAN_POINT('Ctrl Pts',(-0.190123106767869,2.36022015941282,
5.85598695801521));
#51693=CARTESIAN_POINT('Ctrl Pts',(-0.189808720779931,2.36044956633796,
5.85596307949456));
#51694=CARTESIAN_POINT('Ctrl Pts',(-0.189193410125803,2.36089685168069,
5.85591636308976));
#51695=CARTESIAN_POINT('Ctrl Pts',(-0.188892522613072,2.36111478041467,
5.85589352720101));
#51696=CARTESIAN_POINT('Ctrl Pts',(-0.188176397368744,2.36163157462699,
5.85583919655527));
#51697=CARTESIAN_POINT('Ctrl Pts',(-0.187760824427964,2.36192997188904,
5.85580768380528));
#51698=CARTESIAN_POINT('Ctrl Pts',(-0.186287929131073,2.36298226056254,
5.85569604886561));
#51699=CARTESIAN_POINT('Ctrl Pts',(-0.185226773365365,2.36373074196993,
5.85561571928685));
#51700=CARTESIAN_POINT('Ctrl Pts',(-0.167208512562438,2.37627745227219,
5.85425329440143));
#51701=CARTESIAN_POINT('Ctrl Pts',(-0.149163590855082,2.38642249401514,
5.85290726901761));
#51702=CARTESIAN_POINT('Ctrl Pts',(-0.119196983541462,2.39966641443426,
5.8507111766504));
#51703=CARTESIAN_POINT('Ctrl Pts',(-0.107851513131334,2.40393406844556,
5.84988898399211));
#51704=CARTESIAN_POINT('Ctrl Pts',(-0.0796365509684504,2.41276802243173,
5.84789180397521));
#51705=CARTESIAN_POINT('Ctrl Pts',(-0.0625813333070764,2.41662211195314,
5.84672370025639));
#51706=CARTESIAN_POINT('Ctrl Pts',(-0.0445963477278461,2.4191752505305,
5.84558405003193));
#51707=CARTESIAN_POINT('Ctrl Pts',(-0.0438965180187346,2.41927225139381,
5.84553984943952));
#51708=CARTESIAN_POINT('Ctrl Pts',(-0.0428942013346234,2.41940782096155,
5.84547675754714));
#51709=CARTESIAN_POINT('Ctrl Pts',(-0.0425919761426849,2.41944826211711,
5.84545776142461));
#51710=CARTESIAN_POINT('Ctrl Pts',(-0.0420689847243433,2.41951748890268,
5.84542493778293));
#51711=CARTESIAN_POINT('Ctrl Pts',(-0.0418482455951119,2.41954647476104,
5.8454110988658));
#51712=CARTESIAN_POINT('Ctrl Pts',(-0.0414225881143066,2.41960192037887,
5.8453844419481));
#51713=CARTESIAN_POINT('Ctrl Pts',(-0.041217674813951,2.4196284117526,5.84537162214842));
#51714=CARTESIAN_POINT('Ctrl Pts',(-0.0407306568584338,2.41969089773571,
5.8453411837737));
#51715=CARTESIAN_POINT('Ctrl Pts',(-0.0404485291875026,2.41972671610486,
5.84532357522967));
#51716=CARTESIAN_POINT('Ctrl Pts',(-0.0396021032452422,2.41983303838904,
5.84527081878165));
#51717=CARTESIAN_POINT('Ctrl Pts',(-0.0390376615991512,2.41990242264648,
5.84523573376646));
#51718=CARTESIAN_POINT('Ctrl Pts',(-0.0335322403891745,2.42056439111605,
5.84489443119215));
#51719=CARTESIAN_POINT('Ctrl Pts',(-0.0285780148947758,2.4210439903006,
5.84459442491015));
#51720=CARTESIAN_POINT('Ctrl Pts',(0.00366040774643581,2.4234125922658,
5.84267688648764));
#51721=CARTESIAN_POINT('Ctrl Pts',(0.0310824640225515,2.42193690608769,
5.84119878978093));
#51722=CARTESIAN_POINT('Ctrl Pts',(0.06909416337172,2.41498344560778,5.83901318761309));
#51723=CARTESIAN_POINT('Ctrl Pts',(0.0800818088619208,2.41237068676662,
5.83836585722197));
#51724=CARTESIAN_POINT('Ctrl Pts',(0.0955263338179536,2.40782958993038,
5.83741794104472));
#51725=CARTESIAN_POINT('Ctrl Pts',(0.100112324772235,2.40636882306435,5.83713161345061));
#51726=CARTESIAN_POINT('Ctrl Pts',(0.106429837464705,2.40419952707458,5.8367295806874));
#51727=CARTESIAN_POINT('Ctrl Pts',(0.108190622132576,2.40357775220463,5.83661669953718));
#51728=CARTESIAN_POINT('Ctrl Pts',(0.110816384508129,2.40262478772874,5.83644708202482));
#51729=CARTESIAN_POINT('Ctrl Pts',(0.111685519990436,2.40230510716807,5.8363907263837));
#51730=CARTESIAN_POINT('Ctrl Pts',(0.113077698801771,2.40178622053309,5.83630011110342));
#51731=CARTESIAN_POINT('Ctrl Pts',(0.113601626366577,2.40158938865717,5.83626593061311));
#51732=CARTESIAN_POINT('Ctrl Pts',(0.114594248785267,2.40121352144043,5.83620102246938));
#51733=CARTESIAN_POINT('Ctrl Pts',(0.115063043956052,2.40103475424653,5.83617030385437));
#51734=CARTESIAN_POINT('Ctrl Pts',(0.115894291816953,2.40071554639659,5.8361157207648));
#51735=CARTESIAN_POINT('Ctrl Pts',(0.116256912283089,2.40057554302473,5.83609187100535));
#51736=CARTESIAN_POINT('Ctrl Pts',(0.116966409613619,2.40030013870184,5.83604513088461));
#51737=CARTESIAN_POINT('Ctrl Pts',(0.1173133069793,2.40016479188276,5.8360222423727));
#51738=CARTESIAN_POINT('Ctrl Pts',(0.118139263257588,2.39984088306227,5.83596765980315));
#51739=CARTESIAN_POINT('Ctrl Pts',(0.118618105321567,2.39965177417065,5.83593594736216));
#51740=CARTESIAN_POINT('Ctrl Pts',(0.120320944671766,2.39897455130106,5.83582292698947));
#51741=CARTESIAN_POINT('Ctrl Pts',(0.121542386263503,2.39848008360864,5.8357414048548));
#51742=CARTESIAN_POINT('Ctrl Pts',(0.143245994100601,2.38953865233255,5.83428465426995));
#51743=CARTESIAN_POINT('Ctrl Pts',(0.162802085095929,2.37901105030961,5.83283527933183));
#51744=CARTESIAN_POINT('Ctrl Pts',(0.193887921975575,2.35788930853296,5.83030858301476));
#51745=CARTESIAN_POINT('Ctrl Pts',(0.206015010521904,2.34830874488463,5.82925655906084));
#51746=CARTESIAN_POINT('Ctrl Pts',(0.225902593486314,2.33013385407039,5.82745271371526));
#51747=CARTESIAN_POINT('Ctrl Pts',(0.23397556887387,2.32192130692495,5.82669426692387));
#51748=CARTESIAN_POINT('Ctrl Pts',(0.242633451848495,2.31211472515133,5.82586658072961));
#51749=CARTESIAN_POINT('Ctrl Pts',(0.243665615974822,2.31092822573732,5.82576766251313));
#51750=CARTESIAN_POINT('Ctrl Pts',(0.244958754286601,2.3094195693691,5.82564347571607));
#51751=CARTESIAN_POINT('Ctrl Pts',(0.245227824942748,2.30910442657871,5.82561762117162));
#51752=CARTESIAN_POINT('Ctrl Pts',(0.245655682344363,2.30860134680361,5.82557648749072));
#51753=CARTESIAN_POINT('Ctrl Pts',(0.245814861851628,2.30841374678795,5.8255611793846));
#51754=CARTESIAN_POINT('Ctrl Pts',(0.246115311936696,2.30805883015864,5.82553227670477));
#51755=CARTESIAN_POINT('Ctrl Pts',(0.246256625647555,2.30789155322347,5.82551867898451));
#51756=CARTESIAN_POINT('Ctrl Pts',(0.246578369036147,2.30750990833154,5.82548771117498));
#51757=CARTESIAN_POINT('Ctrl Pts',(0.246758689403117,2.30729544938994,5.82547034920103));
#51758=CARTESIAN_POINT('Ctrl Pts',(0.247295786657503,2.30665497406178,5.82541861603386));
#51759=CARTESIAN_POINT('Ctrl Pts',(0.247651743972001,2.30622826702841,5.82538430480438));
#51760=CARTESIAN_POINT('Ctrl Pts',(0.250141567183451,2.30322782643884,5.8251441107708));
#51761=CARTESIAN_POINT('Ctrl Pts',(0.252236472670122,2.30062182596584,5.82494099781612));
#51762=CARTESIAN_POINT('Ctrl Pts',(0.263409233166643,2.28627150758317,5.82384917322398));
#51763=CARTESIAN_POINT('Ctrl Pts',(0.271709004216018,2.27394199857122,5.82300602424876));
#51764=CARTESIAN_POINT('Ctrl Pts',(0.294231852242305,2.23491364438417,5.8204757104639));
#51765=CARTESIAN_POINT('Ctrl Pts',(0.305577187209028,2.20675435279571,5.81881562637419));
#51766=CARTESIAN_POINT('Ctrl Pts',(0.313304003825081,2.17553527465924,5.81688125887405));
#51767=CARTESIAN_POINT('Ctrl Pts',(0.313755209807903,2.17363860804277,5.81676346614677));
#51768=CARTESIAN_POINT('Ctrl Pts',(0.314401961195652,2.17080604656007,5.81658709669652));
#51769=CARTESIAN_POINT('Ctrl Pts',(0.314610601277312,2.16987316342066,5.81652893788738));
#51770=CARTESIAN_POINT('Ctrl Pts',(0.314937463478552,2.16838053088484,5.81643576101691));
#51771=CARTESIAN_POINT('Ctrl Pts',(0.315058352039031,2.16782136617775,5.81640082822223));
#51772=CARTESIAN_POINT('Ctrl Pts',(0.315285697474311,2.16675606414996,5.8163342223953));
#51773=CARTESIAN_POINT('Ctrl Pts',(0.315392426134213,2.16624998615022,5.81630255815529));
#51774=CARTESIAN_POINT('Ctrl Pts',(0.315577289248719,2.16536284456467,5.81624701091446));
#51775=CARTESIAN_POINT('Ctrl Pts',(0.315655953106971,2.16498189136318,5.81622314489794));
#51776=CARTESIAN_POINT('Ctrl Pts',(0.315808246711858,2.1642375622006,5.81617648806905));
#51777=CARTESIAN_POINT('Ctrl Pts',(0.315881939513622,2.16387419961159,5.81615369931177));
#51778=CARTESIAN_POINT('Ctrl Pts',(0.316055254684422,2.16301198607233,5.81609959545455));
#51779=CARTESIAN_POINT('Ctrl Pts',(0.316154323053205,2.16251302594218,5.81606826271168));
#51780=CARTESIAN_POINT('Ctrl Pts',(0.316498792268631,2.16075633488615,5.81595786705889));
#51781=CARTESIAN_POINT('Ctrl Pts',(0.316737870023572,2.15949738946507,5.81587860275574));
#51782=CARTESIAN_POINT('Ctrl Pts',(0.32019614432247,2.14067488846429,5.81469122353853));
#51783=CARTESIAN_POINT('Ctrl Pts',(0.321957166955455,2.12287806459793,5.81353600795519));
#51784=CARTESIAN_POINT('Ctrl Pts',(0.322543264728459,2.08532755459188,5.81103578064756));
#51785=CARTESIAN_POINT('Ctrl Pts',(0.321043150392427,2.0656391107074,5.80968829375565));
#51786=CARTESIAN_POINT('Ctrl Pts',(0.315822081177455,2.034795042447,5.8075933327428));
#51787=CARTESIAN_POINT('Ctrl Pts',(0.313275154605378,2.0234884802853,5.80682981808345));
#51788=CARTESIAN_POINT('Ctrl Pts',(0.309695503342594,2.01082399009489,5.80599708944635));
#51789=CARTESIAN_POINT('Ctrl Pts',(0.309255151750428,2.00930867246203,5.80589782989202));
#51790=CARTESIAN_POINT('Ctrl Pts',(0.30868498209923,2.00739908440096,5.80577327516655));
#51791=CARTESIAN_POINT('Ctrl Pts',(0.308565518394969,2.00700178170726,5.80574738985197));
#51792=CARTESIAN_POINT('Ctrl Pts',(0.308373955367174,2.00636912976164,5.8057062186117));
#51793=CARTESIAN_POINT('Ctrl Pts',(0.308302353557446,2.00613363220885,5.80569090362502));
#51794=CARTESIAN_POINT('Ctrl Pts',(0.308166547635754,2.00568879978513,5.80566199531376));
#51795=CARTESIAN_POINT('Ctrl Pts',(0.308102400514926,2.00547945003885,5.80564839882585));
#51796=CARTESIAN_POINT('Ctrl Pts',(0.307955734082109,2.00500252700914,5.80561744366719));
#51797=CARTESIAN_POINT('Ctrl Pts',(0.307873079518545,2.00473499625837,5.80560009308697));
#51798=CARTESIAN_POINT('Ctrl Pts',(0.307619976798715,2.0039195401112,5.80554724809682));
#51799=CARTESIAN_POINT('Ctrl Pts',(0.307448412649413,2.00337195816212,5.80551181901625));
#51800=CARTESIAN_POINT('Ctrl Pts',(0.30620032716099,1.99942541545164,5.80525686241967));
#51801=CARTESIAN_POINT('Ctrl Pts',(0.30506887653216,1.99604390088875,5.80504048894138));
#51802=CARTESIAN_POINT('Ctrl Pts',(0.294493729131883,1.96609941553954,5.80313725717975));
#51803=CARTESIAN_POINT('Ctrl Pts',(0.281657366288508,1.94086001307461,5.80161516039086));
#51804=CARTESIAN_POINT('Ctrl Pts',(0.256043267149803,1.90354633831779,5.79905942270686));
#51805=CARTESIAN_POINT('Ctrl Pts',(0.245288537666633,1.89027252831746,5.79807636470842));
#51806=CARTESIAN_POINT('Ctrl Pts',(0.232357792902995,1.87667523740651,5.79694543064981));
#51807=CARTESIAN_POINT('Ctrl Pts',(0.231170841441897,1.87544680940788,5.7968420653537));
#51808=CARTESIAN_POINT('Ctrl Pts',(0.229366525954607,1.87360891183762,5.79668557377957));
#51809=CARTESIAN_POINT('Ctrl Pts',(0.228756362602426,1.87299239093416,5.79663276124689));
#51810=CARTESIAN_POINT('Ctrl Pts',(0.22776571596125,1.87199947216841,5.79654718615519));
#51811=CARTESIAN_POINT('Ctrl Pts',(0.227386768211736,1.87162154283818,5.79651449137108));
#51812=CARTESIAN_POINT('Ctrl Pts',(0.226658546021859,1.87089888701902,5.79645173718722));
#51813=CARTESIAN_POINT('Ctrl Pts',(0.226309421870168,1.87055401066385,5.79642168450598));
#51814=CARTESIAN_POINT('Ctrl Pts',(0.225684599339732,1.86993960379489,5.79636795759394));
#51815=CARTESIAN_POINT('Ctrl Pts',(0.225409201855043,1.86966976751159,5.79634429684534));
#51816=CARTESIAN_POINT('Ctrl Pts',(0.224861531588896,1.86913507950386,5.79629728304853));
#51817=CARTESIAN_POINT('Ctrl Pts',(0.224589273431859,1.86887021359933,5.796273930675));
#51818=CARTESIAN_POINT('Ctrl Pts',(0.223927009818201,1.8682282065497,5.79621717241763));
#51819=CARTESIAN_POINT('Ctrl Pts',(0.223536520056469,1.86785156868807,5.79618374470276));
#51820=CARTESIAN_POINT('Ctrl Pts',(0.2220696412247,1.86644385728311,5.79605831566568));
#51821=CARTESIAN_POINT('Ctrl Pts',(0.220987067153297,1.86541928172667,5.79596603380541));
#51822=CARTESIAN_POINT('Ctrl Pts',(0.20146644999483,1.84719952360078,5.79430697774524));
#51823=CARTESIAN_POINT('Ctrl Pts',(0.181084603971428,1.8322227460614,5.79264247960456));
#51824=CARTESIAN_POINT('Ctrl Pts',(0.145501682547115,1.81201113453771,5.78987848022741));
#51825=CARTESIAN_POINT('Ctrl Pts',(0.131281770755558,1.80525697047362,5.78880830785901));
#51826=CARTESIAN_POINT('Ctrl Pts',(0.110701385478685,1.79726784032876,5.78734757530022));
#51827=CARTESIAN_POINT('Ctrl Pts',(0.104710271454859,1.79514375906814,5.78693247221359));
#51828=CARTESIAN_POINT('Ctrl Pts',(0.0958170873609895,1.79228393199961,
5.78633481790563));
#51829=CARTESIAN_POINT('Ctrl Pts',(0.0929616102911164,1.79140927862978,
5.78614567828058));
#51830=CARTESIAN_POINT('Ctrl Pts',(0.0896095238059031,1.79043326444257,
5.7859271905957));
#51831=CARTESIAN_POINT('Ctrl Pts',(0.0891244469151923,1.79029326211606,
5.78589565982756));
#51832=CARTESIAN_POINT('Ctrl Pts',(0.0883834728138306,1.7900812880484,5.78584762921457));
#51833=CARTESIAN_POINT('Ctrl Pts',(0.0881278150405387,1.79000849285541,
5.78583108154108));
#51834=CARTESIAN_POINT('Ctrl Pts',(0.0876828061165472,1.78988237742296,
5.78580232056664));
#51835=CARTESIAN_POINT('Ctrl Pts',(0.0874934967323825,1.78982891438509,
5.78579009890715));
#51836=CARTESIAN_POINT('Ctrl Pts',(0.0870650490739941,1.78970833954978,
5.78576246908865));
#51837=CARTESIAN_POINT('Ctrl Pts',(0.0868258825953968,1.78964133099309,
5.78574706705088));
#51838=CARTESIAN_POINT('Ctrl Pts',(0.0861773860394172,1.78946044651568,
5.78570536197318));
#51839=CARTESIAN_POINT('Ctrl Pts',(0.0857679060335804,1.78934710295515,
5.78567909001801));
#51840=CARTESIAN_POINT('Ctrl Pts',(0.0839259139530756,1.78884116145351,
5.78556118213063));
#51841=CARTESIAN_POINT('Ctrl Pts',(0.0824908926259773,1.7884576518811,5.78547006672072));
#51842=CARTESIAN_POINT('Ctrl Pts',(0.0497483552854235,1.77994930577037,
5.78340689894929));
#51843=CARTESIAN_POINT('Ctrl Pts',(0.0173913404426572,1.77657191857647,
5.78168207786853));
#51844=CARTESIAN_POINT('Ctrl Pts',(-0.0303441735639067,1.77878594144837,
5.77897111280782));
#51845=CARTESIAN_POINT('Ctrl Pts',(-0.0456837672685981,1.78060660481738,
5.77807696802879));
#51846=CARTESIAN_POINT('Ctrl Pts',(-0.0632378049101153,1.7839807704066,
5.77699870942219));
#51847=CARTESIAN_POINT('Ctrl Pts',(-0.0656374223046792,1.78447044239117,
5.77685013519579));
#51848=CARTESIAN_POINT('Ctrl Pts',(-0.0687225653146081,1.78513672021664,
5.77665752061109));
#51849=CARTESIAN_POINT('Ctrl Pts',(-0.0694134569845473,1.78528830985131,
5.77661428275099));
#51850=CARTESIAN_POINT('Ctrl Pts',(-0.0705272969504663,1.78553654547421,
5.77654440665554));
#51851=CARTESIAN_POINT('Ctrl Pts',(-0.0709505615512972,1.78563177377465,
5.77651781396503));
#51852=CARTESIAN_POINT('Ctrl Pts',(-0.0717572715552396,1.7858149838466,
5.77646705459217));
#51853=CARTESIAN_POINT('Ctrl Pts',(-0.0721407509518494,1.7859028136925,
5.77644289283263));
#51854=CARTESIAN_POINT('Ctrl Pts',(-0.0730159541299354,1.78610495236971,
5.77638767412367));
#51855=CARTESIAN_POINT('Ctrl Pts',(-0.0735075711692978,1.78621971467205,
5.77635660263584));
#51856=CARTESIAN_POINT('Ctrl Pts',(-0.0750105998791512,1.78657430545039,
5.77626144031217));
#51857=CARTESIAN_POINT('Ctrl Pts',(-0.0760211151709312,1.78681787071138,
5.77619722929066));
#51858=CARTESIAN_POINT('Ctrl Pts',(-0.0834826362918392,1.78865456703679,
5.77572136646752));
#51859=CARTESIAN_POINT('Ctrl Pts',(-0.0898837597899971,1.79044188215846,
5.77530346964419));
#51860=CARTESIAN_POINT('Ctrl Pts',(-0.098280069351014,1.7930686696114,5.77474183467616));
#51861=CARTESIAN_POINT('Ctrl Pts',(-0.100328892964028,1.79373226337854,
5.7746037123669));
#51862=CARTESIAN_POINT('Ctrl Pts',(-0.125783321773736,1.80225952572849,
5.77287423433374));
#51863=CARTESIAN_POINT('Ctrl Pts',(-0.148213958143662,1.8127664696498,5.77119840547065));
#51864=CARTESIAN_POINT('Ctrl Pts',(-0.176095641517313,1.82996899155539,
5.7689860278859));
#51865=CARTESIAN_POINT('Ctrl Pts',(-0.182808363734286,1.83446745241382,
5.76844314366138));
#51866=CARTESIAN_POINT('Ctrl Pts',(-0.194476692814756,1.84293929765491,
5.76748885006993));
#51867=CARTESIAN_POINT('Ctrl Pts',(-0.199497454972586,1.84681594557394,
5.76707448466603));
#51868=CARTESIAN_POINT('Ctrl Pts',(-0.206758363059428,1.8527724671951,5.76647337023529));
#51869=CARTESIAN_POINT('Ctrl Pts',(-0.209088395308526,1.85473989667044,
5.76628017755105));
#51870=CARTESIAN_POINT('Ctrl Pts',(-0.211773465900188,1.85707319515596,
5.76605755460009));
#51871=CARTESIAN_POINT('Ctrl Pts',(-0.212155894223305,1.85740711072704,
5.76602584713515));
#51872=CARTESIAN_POINT('Ctrl Pts',(-0.212737801821815,1.85791762914752,
5.76597760315692));
#51873=CARTESIAN_POINT('Ctrl Pts',(-0.212937851584951,1.85809357601512,
5.76596101816218));
#51874=CARTESIAN_POINT('Ctrl Pts',(-0.213285277486079,1.85839990738428,
5.76593221618894));
#51875=CARTESIAN_POINT('Ctrl Pts',(-0.213432752010577,1.85853017846088,
5.7659199907723));
#51876=CARTESIAN_POINT('Ctrl Pts',(-0.213742046386848,1.85880389722575,
5.76589435156682));
#51877=CARTESIAN_POINT('Ctrl Pts',(-0.213903840662034,1.85894737226529,
5.76588093994674));
#51878=CARTESIAN_POINT('Ctrl Pts',(-0.214355879565443,1.85934904233171,
5.76584346990755));
#51879=CARTESIAN_POINT('Ctrl Pts',(-0.214645803189693,1.8596076005616,5.76581943876788));
#51880=CARTESIAN_POINT('Ctrl Pts',(-0.215816446257672,1.86065540382703,
5.76572240723123));
#51881=CARTESIAN_POINT('Ctrl Pts',(-0.216693300071115,1.86144898239885,
5.7656497283223));
#51882=CARTESIAN_POINT('Ctrl Pts',(-0.232351593842768,1.87577777920176,
5.76435146915702));
#51883=CARTESIAN_POINT('Ctrl Pts',(-0.245845552949346,1.8906603371769,5.76322472049651));
#51884=CARTESIAN_POINT('Ctrl Pts',(-0.267613271164562,1.91969980399066,
5.76119407952408));
#51885=CARTESIAN_POINT('Ctrl Pts',(-0.276359105662823,1.93341477003469,
5.76029130180693));
#51886=CARTESIAN_POINT('Ctrl Pts',(-0.287695880101525,1.95456155558771,
5.75891464476735));
#51887=CARTESIAN_POINT('Ctrl Pts',(-0.291110440996095,1.961522712429,5.75846398847595));
#51888=CARTESIAN_POINT('Ctrl Pts',(-0.296761521501842,1.97417830515831,
5.75764347977848));
#51889=CARTESIAN_POINT('Ctrl Pts',(-0.299093192359397,1.97982614996347,
5.75727691812598));
#51890=CARTESIAN_POINT('Ctrl Pts',(-0.301595178384437,1.98641127018502,
5.75684785907323));
#51891=CARTESIAN_POINT('Ctrl Pts',(-0.301923701285814,1.98728740204127,
5.75679074127736));
#51892=CARTESIAN_POINT('Ctrl Pts',(-0.302416253927785,1.98861858794343,
5.75670390317121));
#51893=CARTESIAN_POINT('Ctrl Pts',(-0.302583084296901,1.98907260624739,
5.75667427642645));
#51894=CARTESIAN_POINT('Ctrl Pts',(-0.302870211292634,1.98985947160632,
5.75662291286098));
#51895=CARTESIAN_POINT('Ctrl Pts',(-0.302990983253272,1.99019214532241,
5.75660119192561));
#51896=CARTESIAN_POINT('Ctrl Pts',(-0.303240432305109,1.9908828127287,5.75655608565085));
#51897=CARTESIAN_POINT('Ctrl Pts',(-0.303369023960181,1.99124083651432,
5.75653269750685));
#51898=CARTESIAN_POINT('Ctrl Pts',(-0.303718044853324,1.9922180126599,5.75646884535007));
#51899=CARTESIAN_POINT('Ctrl Pts',(-0.303937213615156,1.99283761044965,
5.75642833952462));
#51900=CARTESIAN_POINT('Ctrl Pts',(-0.304760638896118,1.99518830958862,
5.75627458855151));
#51901=CARTESIAN_POINT('Ctrl Pts',(-0.305352004565568,1.99692386041463,
5.75616091720134));
#51902=CARTESIAN_POINT('Ctrl Pts',(-0.306527066306351,2.0004713271078,5.75592822628535));
#51903=CARTESIAN_POINT('Ctrl Pts',(-0.307109581823367,2.00228355507947,
5.75580917301125));
#51904=CARTESIAN_POINT('Ctrl Pts',(-0.317379047921046,2.03523136330209,
5.75364114179909));
#51905=CARTESIAN_POINT('Ctrl Pts',(-0.322299305162623,2.06764903880524,
5.75142184182319));
#51906=CARTESIAN_POINT('Ctrl Pts',(-0.322263896032269,2.1149554738878,5.74823733516237));
#51907=CARTESIAN_POINT('Ctrl Pts',(-0.321245161097404,2.12965378289162,
5.74726038670472));
#51908=CARTESIAN_POINT('Ctrl Pts',(-0.319099916130951,2.14513591319983,
5.74627740594293));
#51909=CARTESIAN_POINT('Ctrl Pts',(-0.318970925718339,2.14603863300754,
5.7462202615247));
#51910=CARTESIAN_POINT('Ctrl Pts',(-0.3187923292569,2.14725172161703,5.74614371042351));
#51911=CARTESIAN_POINT('Ctrl Pts',(-0.318746099839393,2.14756257171382,
5.74612411569842));
#51912=CARTESIAN_POINT('Ctrl Pts',(-0.318667512481556,2.148085738408,5.74609117375295));
#51913=CARTESIAN_POINT('Ctrl Pts',(-0.318635397000124,2.1482980903206,5.74607781279605));
#51914=CARTESIAN_POINT('Ctrl Pts',(-0.318573404021619,2.14870524319618,
5.74605221472523));
#51915=CARTESIAN_POINT('Ctrl Pts',(-0.318543560327155,2.1489000474343,5.74603997582303));
#51916=CARTESIAN_POINT('Ctrl Pts',(-0.318472514974431,2.14936096986873,
5.74601103786525));
#51917=CARTESIAN_POINT('Ctrl Pts',(-0.318431158500563,2.14962706356191,
5.74599434774502));
#51918=CARTESIAN_POINT('Ctrl Pts',(-0.318308755056396,2.15040817282588,
5.74594540049678));
#51919=CARTESIAN_POINT('Ctrl Pts',(-0.318226791334156,2.15092304703549,
5.74591319533897));
#51920=CARTESIAN_POINT('Ctrl Pts',(-0.317604053859782,2.15477469348178,
5.74567270147593));
#51921=CARTESIAN_POINT('Ctrl Pts',(-0.317012035522829,2.15810312910951,
5.74546726430517));
#51922=CARTESIAN_POINT('Ctrl Pts',(-0.314828137706103,2.16935182067675,
5.74477920737608));
#51923=CARTESIAN_POINT('Ctrl Pts',(-0.312990804308368,2.17722181463584,
5.74430832166821));
#51924=CARTESIAN_POINT('Ctrl Pts',(-0.3065353621125,2.20082629505893,5.74290562928294));
#51925=CARTESIAN_POINT('Ctrl Pts',(-0.301011042283634,2.2162853098696,5.74199920625989));
#51926=CARTESIAN_POINT('Ctrl Pts',(-0.288524885160847,2.24428450557417,
5.7402806638351));
#51927=CARTESIAN_POINT('Ctrl Pts',(-0.281857469217187,2.25691062747346,
5.73947357164822));
#51928=CARTESIAN_POINT('Ctrl Pts',(-0.273236127553258,2.27090324172775,
5.7385126180049));
#51929=CARTESIAN_POINT('Ctrl Pts',(-0.272077359460871,2.27274203193797,
5.73838496581106));
#51930=CARTESIAN_POINT('Ctrl Pts',(-0.267308184362823,2.2801429479829,5.73786533392497));
#51931=CARTESIAN_POINT('Ctrl Pts',(-0.263545307615271,2.28560444058553,
5.73746830524277));
#51932=CARTESIAN_POINT('Ctrl Pts',(-0.259001353804761,2.2917825683549,5.73700155967361));
#51933=CARTESIAN_POINT('Ctrl Pts',(-0.258381815859376,2.29261643748937,
5.73693818130351));
#51934=CARTESIAN_POINT('Ctrl Pts',(-0.257455306763621,2.29385096176754,
5.7368437767394));
#51935=CARTESIAN_POINT('Ctrl Pts',(-0.257151404350395,2.29425392041086,
5.73681287076288));
#51936=CARTESIAN_POINT('Ctrl Pts',(-0.256608945193304,2.29496968900571,
5.73675780901302));
#51937=CARTESIAN_POINT('Ctrl Pts',(-0.256370759386077,2.2952827798702,5.73673366786242));
#51938=CARTESIAN_POINT('Ctrl Pts',(-0.255868651698765,2.29594028932859,
5.73668285148313));
#51939=CARTESIAN_POINT('Ctrl Pts',(-0.255604606480336,2.29628461235516,
5.73665617141489));
#51940=CARTESIAN_POINT('Ctrl Pts',(-0.254908129074403,2.29718905163722,
5.73658590883799));
#51941=CARTESIAN_POINT('Ctrl Pts',(-0.254474547850597,2.29774827644576,
5.73654228085897));
#51942=CARTESIAN_POINT('Ctrl Pts',(-0.252530425392199,2.30023878615156,
5.73634715598701));
#51943=CARTESIAN_POINT('Ctrl Pts',(-0.250999747460072,2.30215418241752,
5.73619485801041));
#51944=CARTESIAN_POINT('Ctrl Pts',(-0.239658860514293,2.31601808140309,
5.73507579900811));
#51945=CARTESIAN_POINT('Ctrl Pts',(-0.229023482401768,2.32726262403565,
5.73407491891449));
#51946=CARTESIAN_POINT('Ctrl Pts',(-0.193787644780856,2.35952250849864,
5.73090250949542));
#51947=CARTESIAN_POINT('Ctrl Pts',(-0.166806463493108,2.37763484528071,
5.72864542612765));
#51948=CARTESIAN_POINT('Ctrl Pts',(-0.136239208305723,2.39206551130925,
5.72650776889335));
#51949=CARTESIAN_POINT('Ctrl Pts',(-0.134890734018903,2.39269074951912,
5.72641429385069));
#51950=CARTESIAN_POINT('Ctrl Pts',(-0.133151169938138,2.39348274596487,
5.7262948155963));
#51951=CARTESIAN_POINT('Ctrl Pts',(-0.132764037430547,2.39365807771122,
5.72626829636387));
#51952=CARTESIAN_POINT('Ctrl Pts',(-0.132150079737725,2.39393467599542,
5.72622635159065));
#51953=CARTESIAN_POINT('Ctrl Pts',(-0.131923484073053,2.39403644617334,
5.72621089508165));
#51954=CARTESIAN_POINT('Ctrl Pts',(-0.131517233199071,2.39421834016929,
5.72618322761232));
#51955=CARTESIAN_POINT('Ctrl Pts',(-0.131337623600715,2.39429856089954,
5.72617101070704));
#51956=CARTESIAN_POINT('Ctrl Pts',(-0.130915160230054,2.39448678593252,
5.72614231092519));
#51957=CARTESIAN_POINT('Ctrl Pts',(-0.130672246577873,2.39459465413079,
5.72612583653074));
#51958=CARTESIAN_POINT('Ctrl Pts',(-0.12996766376257,2.39490648812835,5.72607813148965));
#51959=CARTESIAN_POINT('Ctrl Pts',(-0.12950564588863,2.395109671233,5.72604694887368));
#51960=CARTESIAN_POINT('Ctrl Pts',(-0.126309968800665,2.39650609452702,
5.72583193699005));
#51961=CARTESIAN_POINT('Ctrl Pts',(-0.123560221627717,2.39766246904118,
5.72565031854719));
#51962=CARTESIAN_POINT('Ctrl Pts',(-0.114906770022824,2.40116099357221,
5.72508811778198));
#51963=CARTESIAN_POINT('Ctrl Pts',(-0.108949348527835,2.4033670390686,5.72471453610812));
#51964=CARTESIAN_POINT('Ctrl Pts',(-0.0880497203013235,2.41041102638192,
5.7234375654925));
#51965=CARTESIAN_POINT('Ctrl Pts',(-0.072821567161345,2.41433237614209,
5.72256489550529));
#51966=CARTESIAN_POINT('Ctrl Pts',(-0.0428376489126385,2.41975636438826,
5.7208611762729));
#51967=CARTESIAN_POINT('Ctrl Pts',(-0.0281451870300529,2.42138295424324,
5.72003266554318));
#51968=CARTESIAN_POINT('Ctrl Pts',(-0.0101383473961594,2.42213196985804,
5.71898884402014));
#51969=CARTESIAN_POINT('Ctrl Pts',(-0.0068810812781981,2.4222180036148,
5.71879894727686));
#51970=CARTESIAN_POINT('Ctrl Pts',(-0.00189330594087092,2.42227408169016,
5.71850615882642));
#51971=CARTESIAN_POINT('Ctrl Pts',(-0.00016336432746312,2.42227960142166,
5.71840424076998));
#51972=CARTESIAN_POINT('Ctrl Pts',(0.00216887711405079,2.42226826471898,
5.71826630085771));
#51973=CARTESIAN_POINT('Ctrl Pts',(0.00277122632638494,2.42226364792002,
5.71823062669442));
#51974=CARTESIAN_POINT('Ctrl Pts',(0.0090042002405497,2.42219839793129,
5.71786096559003));
#51975=CARTESIAN_POINT('Ctrl Pts',(0.0146320439378032,2.42199189519972,
5.71752283598708));
#51976=CARTESIAN_POINT('Ctrl Pts',(0.0212262050221727,2.42157670620926,
5.71712057188143));
#51977=CARTESIAN_POINT('Ctrl Pts',(0.0222007782505227,2.42151089432266,
5.71706096458906));
#51978=CARTESIAN_POINT('Ctrl Pts',(0.0236726425540074,2.4214047767629,5.71697070201268));
#51979=CARTESIAN_POINT('Ctrl Pts',(0.0241701700143458,2.42136774481667,
5.71694014956498));
#51980=CARTESIAN_POINT('Ctrl Pts',(0.0250591603829457,2.42129949941332,
5.71688548318985));
#51981=CARTESIAN_POINT('Ctrl Pts',(0.0254506568367829,2.42126872537917,
5.7168613831145));
#51982=CARTESIAN_POINT('Ctrl Pts',(0.02627779308269,2.42120218597838,5.71681041036384));
#51983=CARTESIAN_POINT('Ctrl Pts',(0.0267134179922768,2.42116624975666,
5.71678353236454));
#51984=CARTESIAN_POINT('Ctrl Pts',(0.0278682913960577,2.42106861429587,
5.71671219033035));
#51985=CARTESIAN_POINT('Ctrl Pts',(0.0285874049610076,2.42100538471379,
5.7166676782597));
#51986=CARTESIAN_POINT('Ctrl Pts',(0.031888081136572,2.42070398672882,5.7164629575731));
#51987=CARTESIAN_POINT('Ctrl Pts',(0.0344668651606478,2.42043709428932,
5.71630184783613));
#51988=CARTESIAN_POINT('Ctrl Pts',(0.0539605705825171,2.41818155123755,
5.71507485044191));
#51989=CARTESIAN_POINT('Ctrl Pts',(0.0706944722030677,2.41488628021309,
5.71396726861259));
#51990=CARTESIAN_POINT('Ctrl Pts',(0.116455667525205,2.40204251772472,5.71079617487498));
#51991=CARTESIAN_POINT('Ctrl Pts',(0.144504017689707,2.38967261991231,5.70867399907795));
#51992=CARTESIAN_POINT('Ctrl Pts',(0.171703673604288,2.37272953769918,5.70664647082098));
#51993=CARTESIAN_POINT('Ctrl Pts',(0.173006367511029,2.37190503726226,5.70654948694459));
#51994=CARTESIAN_POINT('Ctrl Pts',(0.174661350557042,2.37084085664952,5.7064264827988));
#51995=CARTESIAN_POINT('Ctrl Pts',(0.175019121405607,2.37060980055503,5.70639990446393));
#51996=CARTESIAN_POINT('Ctrl Pts',(0.175587083565339,2.37024140088314,5.70635773244519));
#51997=CARTESIAN_POINT('Ctrl Pts',(0.175797572632388,2.37010452073939,5.70634210795698));
#51998=CARTESIAN_POINT('Ctrl Pts',(0.176190726465049,2.3698482002248,5.70631293335261));
#51999=CARTESIAN_POINT('Ctrl Pts',(0.176373428488565,2.36972882118984,5.70629937933357));
#52000=CARTESIAN_POINT('Ctrl Pts',(0.176779354126597,2.36946299718756,5.70626927317869));
#52001=CARTESIAN_POINT('Ctrl Pts',(0.177002516546941,2.36931646075946,5.70625272734086));
#52002=CARTESIAN_POINT('Ctrl Pts',(0.177656931566837,2.3688855836936,5.70620422231186));
#52003=CARTESIAN_POINT('Ctrl Pts',(0.178087685506707,2.36860048162954,5.70617231410561));
#52004=CARTESIAN_POINT('Ctrl Pts',(0.179065201088069,2.36795011055405,5.7060999434479));
#52005=CARTESIAN_POINT('Ctrl Pts',(0.179611536075753,2.36758420004302,5.70605952325958));
#52006=CARTESIAN_POINT('Ctrl Pts',(0.194256997427316,2.35771026780845,5.70497663031193));
#52007=CARTESIAN_POINT('Ctrl Pts',(0.207584995705116,2.3471012168304,5.70400651664046));
#52008=CARTESIAN_POINT('Ctrl Pts',(0.236745396534201,2.31985686052574,5.70176307995427));
#52009=CARTESIAN_POINT('Ctrl Pts',(0.25176159907065,2.30248821601408,5.70050360685446));
#52010=CARTESIAN_POINT('Ctrl Pts',(0.265845525614916,2.28218295774062,5.69906802154962));
#52011=CARTESIAN_POINT('Ctrl Pts',(0.266867894727869,2.28068204165686,5.69896214191502));
#52012=CARTESIAN_POINT('Ctrl Pts',(0.268921924470235,2.27761110098055,5.69874590259292));
#52013=CARTESIAN_POINT('Ctrl Pts',(0.26995264991046,2.27604053868806,5.69863551855942));
#52014=CARTESIAN_POINT('Ctrl Pts',(0.27458400159836,2.26884721277617,5.69813070058535));
#52015=CARTESIAN_POINT('Ctrl Pts',(0.278022881426385,2.26312272313235,5.69773098904845));
#52016=CARTESIAN_POINT('Ctrl Pts',(0.281789380921575,2.25638735221986,5.69726134366988));
#52017=CARTESIAN_POINT('Ctrl Pts',(0.282293022279623,2.2554763926353,5.69719783875217));
#52018=CARTESIAN_POINT('Ctrl Pts',(0.283034495028333,2.25411977615095,5.69710328187821));
#52019=CARTESIAN_POINT('Ctrl Pts',(0.283275709579579,2.25367596797924,5.69707235071068));
#52020=CARTESIAN_POINT('Ctrl Pts',(0.283702949854325,2.25288546912238,5.69701726063319));
#52021=CARTESIAN_POINT('Ctrl Pts',(0.283889386385399,2.25253900065347,5.69699311640096));
#52022=CARTESIAN_POINT('Ctrl Pts',(0.284279996250785,2.2518099056283,5.69694231041289));
#52023=CARTESIAN_POINT('Ctrl Pts',(0.284484032478655,2.25142720685853,5.69691564385094));
#52024=CARTESIAN_POINT('Ctrl Pts',(0.285018487177012,2.25041986884669,5.69684545494302));
#52025=CARTESIAN_POINT('Ctrl Pts',(0.285347623420708,2.2497945552147,5.69680188729975));
#52026=CARTESIAN_POINT('Ctrl Pts',(0.286805243635251,2.24700303997135,5.69660740087385));
#52027=CARTESIAN_POINT('Ctrl Pts',(0.287911112270531,2.24482517888968,5.69645568744047));
#52028=CARTESIAN_POINT('Ctrl Pts',(0.295790421240226,2.22886094905362,5.69534348006815));
#52029=CARTESIAN_POINT('Ctrl Pts',(0.301594294018066,2.21462057602891,5.69434931830765));
#52030=CARTESIAN_POINT('Ctrl Pts',(0.315851898834108,2.17095075528838,5.69129971299677));
#52031=CARTESIAN_POINT('Ctrl Pts',(0.321156656626979,2.14067834545877,5.68917083618267));
#52032=CARTESIAN_POINT('Ctrl Pts',(0.322213828142119,2.1070062285022,5.68701272220404));
#52033=CARTESIAN_POINT('Ctrl Pts',(0.322266421657823,2.10389788555366,5.68681563153696));
#52034=CARTESIAN_POINT('Ctrl Pts',(0.322275363907552,2.10024594927253,5.68658695262188));
#52035=CARTESIAN_POINT('Ctrl Pts',(0.322275320699256,2.09970276066507,5.68655301379168));
#52036=CARTESIAN_POINT('Ctrl Pts',(0.32227318046278,2.09888205885579,5.68650185146313));
#52037=CARTESIAN_POINT('Ctrl Pts',(0.322272098313735,2.09860454743895,5.68648457146989));
#52038=CARTESIAN_POINT('Ctrl Pts',(0.322269522440866,2.09810834518969,5.68645371027364));
#52039=CARTESIAN_POINT('Ctrl Pts',(0.322268164571216,2.09788965473951,5.68644012144861));
#52040=CARTESIAN_POINT('Ctrl Pts',(0.322264830529612,2.0974283264848,5.68641148240982));
#52041=CARTESIAN_POINT('Ctrl Pts',(0.322262802945875,2.09718569025376,5.68639643516188));
#52042=CARTESIAN_POINT('Ctrl Pts',(0.322256634683385,2.09653543722573,5.68635615025939));
#52043=CARTESIAN_POINT('Ctrl Pts',(0.322251994639805,2.09612782390828,5.68633094068118));
#52044=CARTESIAN_POINT('Ctrl Pts',(0.322240059481081,2.09522916506435,5.68627545449753));
#52045=CARTESIAN_POINT('Ctrl Pts',(0.322232415299115,2.09473812407397,5.68624519720929));
#52046=CARTESIAN_POINT('Ctrl Pts',(0.322206194250205,2.09326946650015,5.68615487849985));
#52047=CARTESIAN_POINT('Ctrl Pts',(0.322184290450685,2.09229190442848,5.686094996838));
#52048=CARTESIAN_POINT('Ctrl Pts',(0.321879876659181,2.08100082454766,5.68540591922533));
#52049=CARTESIAN_POINT('Ctrl Pts',(0.321106669114624,2.07070533127981,5.6848023135118));
#52050=CARTESIAN_POINT('Ctrl Pts',(0.317805879462329,2.04400264937664,5.683260948556));
#52051=CARTESIAN_POINT('Ctrl Pts',(0.314503274945983,2.02772260956309,5.68234428644838));
#52052=CARTESIAN_POINT('Ctrl Pts',(0.306141697334235,1.99834792465086,5.68063145552539));
#52053=CARTESIAN_POINT('Ctrl Pts',(0.3014541483753,1.9851904535678,5.67984122179284));
#52054=CARTESIAN_POINT('Ctrl Pts',(0.295082760294708,1.97041640453826,5.67890042506923));
#52055=CARTESIAN_POINT('Ctrl Pts',(0.29421690389079,1.96846233690817,5.67877489485736));
#52056=CARTESIAN_POINT('Ctrl Pts',(0.29057838128421,1.96046660387529,5.67825647078186));
#52057=CARTESIAN_POINT('Ctrl Pts',(0.287638700329508,1.95450315225564,5.67785848172221));
#52058=CARTESIAN_POINT('Ctrl Pts',(0.284028625272619,1.94771737992242,5.67739069810518));
#52059=CARTESIAN_POINT('Ctrl Pts',(0.283535926000011,1.94680197462252,5.6773272743492));
#52060=CARTESIAN_POINT('Ctrl Pts',(0.282797387978917,1.94544558284828,5.67723281515676));
#52061=CARTESIAN_POINT('Ctrl Pts',(0.282554924747071,1.94500275807164,5.67720190014253));
#52062=CARTESIAN_POINT('Ctrl Pts',(0.282121672355839,1.94421587890324,5.6771468282319));
#52063=CARTESIAN_POINT('Ctrl Pts',(0.281931291430644,1.94387159992873,5.67712268597798));
#52064=CARTESIAN_POINT('Ctrl Pts',(0.281529644656134,1.94314840448331,5.67707187333779));
#52065=CARTESIAN_POINT('Ctrl Pts',(0.281318243272473,1.94276956453823,5.67704519812398));
#52066=CARTESIAN_POINT('Ctrl Pts',(0.280760186501039,1.94177423239412,5.6769749620248));
#52067=CARTESIAN_POINT('Ctrl Pts',(0.280412266902401,1.94115845500474,5.67693135573131));
#52068=CARTESIAN_POINT('Ctrl Pts',(0.27885085025985,1.93841604635052,5.67673646056181));
#52069=CARTESIAN_POINT('Ctrl Pts',(0.277615193542763,1.93630218526276,5.6765843729198));
#52070=CARTESIAN_POINT('Ctrl Pts',(0.268420593048042,1.92097637102988,5.67546778310713));
#52071=CARTESIAN_POINT('Ctrl Pts',(0.259547549768732,1.90833878953515,5.67446932488594));
#52072=CARTESIAN_POINT('Ctrl Pts',(0.234428682747998,1.87752148863825,5.67182949265537));
#52073=CARTESIAN_POINT('Ctrl Pts',(0.216966076158849,1.86046062677746,5.67015409278839));
#52074=CARTESIAN_POINT('Ctrl Pts',(0.19065567285789,1.84001475944158,5.66794946908287));
#52075=CARTESIAN_POINT('Ctrl Pts',(0.183332522709492,1.8347998270432,5.6673657281234));
#52076=CARTESIAN_POINT('Ctrl Pts',(0.175200675990513,1.82950709714011,5.66675684453527));
#52077=CARTESIAN_POINT('Ctrl Pts',(0.174599819420961,1.82911886288199,5.66671207939098));
#52078=CARTESIAN_POINT('Ctrl Pts',(0.173758823435224,1.82857942704932,5.66664974227395));
#52079=CARTESIAN_POINT('Ctrl Pts',(0.173519775156533,1.82842654074152,5.66663205915881));
#52080=CARTESIAN_POINT('Ctrl Pts',(0.173106454217469,1.82816296470914,5.66660154689277));
#52081=CARTESIAN_POINT('Ctrl Pts',(0.17293227707968,1.82805212670063,5.66658870783007));
#52082=CARTESIAN_POINT('Ctrl Pts',(0.172569949440291,1.82782204756103,5.66656203953184));
#52083=CARTESIAN_POINT('Ctrl Pts',(0.172381782056957,1.82770283428058,5.66654821222607));
#52084=CARTESIAN_POINT('Ctrl Pts',(0.17194038258395,1.82742382693615,5.66651582835683));
#52085=CARTESIAN_POINT('Ctrl Pts',(0.171687050280323,1.8272641900061,5.66649728230814));
#52086=CARTESIAN_POINT('Ctrl Pts',(0.170857353911134,1.82674297232584,5.66643667115047));
#52087=CARTESIAN_POINT('Ctrl Pts',(0.170280062281923,1.82638286061004,5.66639470298465));
#52088=CARTESIAN_POINT('Ctrl Pts',(0.168914776155318,1.82553719615057,5.66629591939255));
#52089=CARTESIAN_POINT('Ctrl Pts',(0.168125817008921,1.82505320150365,5.66623920336197));
#52090=CARTESIAN_POINT('Ctrl Pts',(0.165355068736371,1.82336984486522,5.66604126825538));
#52091=CARTESIAN_POINT('Ctrl Pts',(0.163362391365875,1.82218842490433,5.6659011388293));
#52092=CARTESIAN_POINT('Ctrl Pts',(0.157188250784807,1.81861730192732,5.66547320866404));
#52093=CARTESIAN_POINT('Ctrl Pts',(0.152965666118957,1.81629966716277,5.66518925467874));
#52094=CARTESIAN_POINT('Ctrl Pts',(0.137022174412028,1.80800833944024,5.66414330429391));
#52095=CARTESIAN_POINT('Ctrl Pts',(0.124990367536039,1.80265901351004,5.66340536470217));
#52096=CARTESIAN_POINT('Ctrl Pts',(0.0906877087635088,1.78985948056676,
5.66135753819177));
#52097=CARTESIAN_POINT('Ctrl Pts',(0.0678837871972534,1.78408377177473,
5.66005336241542));
#52098=CARTESIAN_POINT('Ctrl Pts',(0.0443095014057243,1.78078539184679,
5.65864459449509));
#52099=CARTESIAN_POINT('Ctrl Pts',(0.0439630147846903,1.78073748841599,
5.65862387743868));
#52100=CARTESIAN_POINT('Ctrl Pts',(0.0379381935890465,1.77991452187501,
5.65826343896273));
#52101=CARTESIAN_POINT('Ctrl Pts',(0.0322405523750295,1.77929053593703,
5.65791940293965));
#52102=CARTESIAN_POINT('Ctrl Pts',(0.0255509796251701,1.77873797730927,
5.65751075412378));
#52103=CARTESIAN_POINT('Ctrl Pts',(0.0245720410303623,1.77866161986268,
5.65745083609663));
#52104=CARTESIAN_POINT('Ctrl Pts',(0.0230941122956186,1.77855313408154,
5.65736019443623));
#52105=CARTESIAN_POINT('Ctrl Pts',(0.0225953651323818,1.77851769084193,
5.65732957494025));
#52106=CARTESIAN_POINT('Ctrl Pts',(0.021704633475605,1.77845647444453,5.65727483390327));
#52107=CARTESIAN_POINT('Ctrl Pts',(0.0213126797007923,1.77843025698497,
5.65725072636035));
#52108=CARTESIAN_POINT('Ctrl Pts',(0.0204851209619876,1.77837642194798,
5.65719978482904));
#52109=CARTESIAN_POINT('Ctrl Pts',(0.0200495061849004,1.77834897258276,
5.65717294561072));
#52110=CARTESIAN_POINT('Ctrl Pts',(0.0188960766874535,1.77827864384153,
5.65710181507925));
#52111=CARTESIAN_POINT('Ctrl Pts',(0.0181781749182886,1.77823728204488,
5.6570574762374));
#52112=CARTESIAN_POINT('Ctrl Pts',(0.0148995316412332,1.77805939115009,
5.65685467200544));
#52113=CARTESIAN_POINT('Ctrl Pts',(0.0123374126655923,1.77795102964437,
5.65669532597675));
#52114=CARTESIAN_POINT('Ctrl Pts',(0.00118108329803457,1.7776125117645,
5.65599755231745));
#52115=CARTESIAN_POINT('Ctrl Pts',(-0.00741842862448786,1.77769574626325,
5.65544942371332));
#52116=CARTESIAN_POINT('Ctrl Pts',(-0.0259853736189691,1.77861889337533,
5.65424301074626));
#52117=CARTESIAN_POINT('Ctrl Pts',(-0.0359377725378343,1.77957917692732,
5.65358189662956));
#52118=CARTESIAN_POINT('Ctrl Pts',(-0.0479490571053053,1.78130476658852,
5.65276933209553));
#52119=CARTESIAN_POINT('Ctrl Pts',(-0.0500661985594481,1.78163049853652,
5.65262555965485));
#52120=CARTESIAN_POINT('Ctrl Pts',(-0.0680565248867953,1.78458228068209,
5.65139954966809));
#52121=CARTESIAN_POINT('Ctrl Pts',(-0.0837155960282453,1.78837245570623,
5.65030229063019));
#52122=CARTESIAN_POINT('Ctrl Pts',(-0.103015365814818,1.79460421848962,
5.64894747261536));
#52123=CARTESIAN_POINT('Ctrl Pts',(-0.106979244317688,1.79597007938088,
5.64866917297206));
#52124=CARTESIAN_POINT('Ctrl Pts',(-0.118058533405901,1.80003127274252,
5.6478931331338));
#52125=CARTESIAN_POINT('Ctrl Pts',(-0.125107350737989,1.80290198987303,
5.64740152884588));
#52126=CARTESIAN_POINT('Ctrl Pts',(-0.132677236532066,1.80630219356559,
5.64688091896572));
#52127=CARTESIAN_POINT('Ctrl Pts',(-0.133305010669028,1.80658659752932,
5.64683780089367));
#52128=CARTESIAN_POINT('Ctrl Pts',(-0.134185856272308,1.80698906236297,
5.64677738515823));
#52129=CARTESIAN_POINT('Ctrl Pts',(-0.134439688324284,1.80710543910276,
5.64675998510387));
#52130=CARTESIAN_POINT('Ctrl Pts',(-0.134879864890374,1.80730794371257,
5.6467298287704));
#52131=CARTESIAN_POINT('Ctrl Pts',(-0.13506627841259,1.80739391974376,5.64671706311545));
#52132=CARTESIAN_POINT('Ctrl Pts',(-0.135440761480162,1.8075670697001,5.64669142958255));
#52133=CARTESIAN_POINT('Ctrl Pts',(-0.135628828869128,1.80765424686864,
5.6466785619821));
#52134=CARTESIAN_POINT('Ctrl Pts',(-0.13601515772189,1.80783377961885,5.64665214076689));
#52135=CARTESIAN_POINT('Ctrl Pts',(-0.136213409869735,1.80792615585394,
5.64663858841847));
#52136=CARTESIAN_POINT('Ctrl Pts',(-0.136881209538189,1.80823814710439,
5.64659295863402));
#52137=CARTESIAN_POINT('Ctrl Pts',(-0.137350324358735,1.80845869462952,
5.64656093877155));
#52138=CARTESIAN_POINT('Ctrl Pts',(-0.140844570835779,1.8101117697925,5.64632267520406));
#52139=CARTESIAN_POINT('Ctrl Pts',(-0.143847894497632,1.81159028355928,
5.64611922646788));
#52140=CARTESIAN_POINT('Ctrl Pts',(-0.153875716861637,1.81672253129519,
5.64544265856876));
#52141=CARTESIAN_POINT('Ctrl Pts',(-0.160788909888938,1.82058846334748,
5.64498077928952));
#52142=CARTESIAN_POINT('Ctrl Pts',(-0.173169909667254,1.8281239401837,5.64414930288855));
#52143=CARTESIAN_POINT('Ctrl Pts',(-0.17868089602663,1.83171367394219,5.64377754599345));
#52144=CARTESIAN_POINT('Ctrl Pts',(-0.200957885193175,1.84721552893903,
5.64225239834952));
#52145=CARTESIAN_POINT('Ctrl Pts',(-0.216673699879071,1.86054950013115,
5.64111892226011));
#52146=CARTESIAN_POINT('Ctrl Pts',(-0.232104167997648,1.87641269064684,
5.63984383717069));
#52147=CARTESIAN_POINT('Ctrl Pts',(-0.233188251522048,1.87754355716099,
5.63975331795452));
#52148=CARTESIAN_POINT('Ctrl Pts',(-0.235631762213985,1.88013000462552,
5.63954708109624));
#52149=CARTESIAN_POINT('Ctrl Pts',(-0.236986019245782,1.88159036491894,
5.63943119594179));
#52150=CARTESIAN_POINT('Ctrl Pts',(-0.240049828766292,1.88495626362243,
5.6391652458099));
#52151=CARTESIAN_POINT('Ctrl Pts',(-0.241750371143206,1.88686979003219,
5.63901487373053));
#52152=CARTESIAN_POINT('Ctrl Pts',(-0.247630908661074,1.89364777083966,
5.63848472424336));
#52153=CARTESIAN_POINT('Ctrl Pts',(-0.251688118290092,1.89861630702277,
5.63810047831109));
#52154=CARTESIAN_POINT('Ctrl Pts',(-0.25622079890972,1.90451819496466,5.63764755046925));
#52155=CARTESIAN_POINT('Ctrl Pts',(-0.256843477510074,1.90533705561698,
5.63758478566282));
#52156=CARTESIAN_POINT('Ctrl Pts',(-0.257764581652727,1.90656047772691,
5.63749111992739));
#52157=CARTESIAN_POINT('Ctrl Pts',(-0.258066002635016,1.90696278438782,
5.63746033646461));
#52158=CARTESIAN_POINT('Ctrl Pts',(-0.25860147708555,1.90768097795702,5.63740541219685));
#52159=CARTESIAN_POINT('Ctrl Pts',(-0.25883589664019,1.90799659170032,5.63738128574731));
#52160=CARTESIAN_POINT('Ctrl Pts',(-0.259328466589158,1.90866231093329,
5.63733041744136));
#52161=CARTESIAN_POINT('Ctrl Pts',(-0.259586486668148,1.90901251146422,
5.63730367058066));
#52162=CARTESIAN_POINT('Ctrl Pts',(-0.26026522713061,1.90993765565348,5.63723304372362));
#52163=CARTESIAN_POINT('Ctrl Pts',(-0.260684749652259,1.91051347151432,
5.63718911739745));
#52164=CARTESIAN_POINT('Ctrl Pts',(-0.262566917867694,1.91311492352801,
5.63699080517989));
#52165=CARTESIAN_POINT('Ctrl Pts',(-0.26400785492566,1.91515609250337,5.63683558567408));
#52166=CARTESIAN_POINT('Ctrl Pts',(-0.274479668810285,1.93036227005474,
5.63568176394858));
#52167=CARTESIAN_POINT('Ctrl Pts',(-0.282543538091337,1.94416335497829,
5.63464669965837));
#52168=CARTESIAN_POINT('Ctrl Pts',(-0.297615383437988,1.97500551822084,
5.6323635337471));
#52169=CARTESIAN_POINT('Ctrl Pts',(-0.304253923772735,1.99216668078398,
5.63111042013613));
#52170=CARTESIAN_POINT('Ctrl Pts',(-0.309886064193154,2.01148508737114,
5.62975751988349));
#52171=CARTESIAN_POINT('Ctrl Pts',(-0.310364023576022,2.01317583560878,
5.62963960736586));
#52172=CARTESIAN_POINT('Ctrl Pts',(-0.312726390681261,2.02180139433576,
5.62904080334086));
#52173=CARTESIAN_POINT('Ctrl Pts',(-0.31439240951314,2.02879436228716,5.62856428317902));
#52174=CARTESIAN_POINT('Ctrl Pts',(-0.316104906935959,2.03722369826351,
5.62800471248308));
#52175=CARTESIAN_POINT('Ctrl Pts',(-0.31637738612899,2.03861167919357,5.62791305117686));
#52176=CARTESIAN_POINT('Ctrl Pts',(-0.317417728464741,2.04410205608408,
5.62755247136607));
#52177=CARTESIAN_POINT('Ctrl Pts',(-0.318115050190996,2.04821763397942,
5.62728658232325));
#52178=CARTESIAN_POINT('Ctrl Pts',(-0.31881229817931,2.0528811384461,5.62699112419491));
#52179=CARTESIAN_POINT('Ctrl Pts',(-0.318890984834883,2.05341665119765,
5.62695728313937));
#52180=CARTESIAN_POINT('Ctrl Pts',(-0.319007959322328,2.05422692419948,
5.62690621245451));
#52181=CARTESIAN_POINT('Ctrl Pts',(-0.319047241641721,2.05450153649332,
5.62688892709596));
#52182=CARTESIAN_POINT('Ctrl Pts',(-0.319114910939878,2.05497899166809,
5.62685891456161));
#52183=CARTESIAN_POINT('Ctrl Pts',(-0.319143459130584,2.05518181094585,
5.62684617822489));
#52184=CARTESIAN_POINT('Ctrl Pts',(-0.319200470052503,2.05558965897626,
5.62682059263921));
#52185=CARTESIAN_POINT('Ctrl Pts',(-0.319228928580053,2.0557946877686,5.62680774368089));
#52186=CARTESIAN_POINT('Ctrl Pts',(-0.319287117427322,2.05621689458369,
5.62678131118779));
#52187=CARTESIAN_POINT('Ctrl Pts',(-0.319316823792063,2.05643407617212,
5.62676772900798));
#52188=CARTESIAN_POINT('Ctrl Pts',(-0.319385575835655,2.05694056669194,
5.62673608759647));
#52189=CARTESIAN_POINT('Ctrl Pts',(-0.319424450120711,2.05722989928284,
5.62671803805719));
#52190=CARTESIAN_POINT('Ctrl Pts',(-0.319524800616196,2.05798455381116,
5.62667102601109));
#52191=CARTESIAN_POINT('Ctrl Pts',(-0.3195856537926,2.05844996000358,5.62664209826355));
#52192=CARTESIAN_POINT('Ctrl Pts',(-0.321386042602537,2.07245733934876,
5.62577337477581));
#52193=CARTESIAN_POINT('Ctrl Pts',(-0.322264489247042,2.08609776830945,
5.62498113170366));
#52194=CARTESIAN_POINT('Ctrl Pts',(-0.322274906241924,2.09975417128097,
5.62420562594364));
#52195=CARTESIAN_POINT('',(-0.32227484120197,2.10029389008051,5.37446215688076));
#52196=CARTESIAN_POINT('Ctrl Pts',(-0.322274905917569,2.09975374642723,
5.62420565006981));
#52197=CARTESIAN_POINT('Ctrl Pts',(-0.322293894667884,2.12460454413308,
5.62279444786394));
#52198=CARTESIAN_POINT('Ctrl Pts',(-0.319438607195465,2.14937501801755,
5.62143993016761));
#52199=CARTESIAN_POINT('Ctrl Pts',(-0.311278981273533,2.18417309598891,
5.61937801561696));
#52200=CARTESIAN_POINT('Ctrl Pts',(-0.308258119663738,2.19463935704238,
5.6187372750986));
#52201=CARTESIAN_POINT('Ctrl Pts',(-0.304069280760107,2.20680339728441,
5.61795911815928));
#52202=CARTESIAN_POINT('Ctrl Pts',(-0.303407616867518,2.20866881304729,
5.61783884301304));
#52203=CARTESIAN_POINT('Ctrl Pts',(-0.302504689623937,2.21114187092898,
5.617678094228));
#52204=CARTESIAN_POINT('Ctrl Pts',(-0.302278690593447,2.21175507112102,
5.61763812973989));
#52205=CARTESIAN_POINT('Ctrl Pts',(-0.301903736363279,2.21276297073116,
5.61757226429109));
#52206=CARTESIAN_POINT('Ctrl Pts',(-0.301755867778648,2.21315807464206,
5.61754639969638));
#52207=CARTESIAN_POINT('Ctrl Pts',(-0.301467219349389,2.21392475222246,
5.61749612320407));
#52208=CARTESIAN_POINT('Ctrl Pts',(-0.301326527198473,2.21429635827734,
5.61747171428079));
#52209=CARTESIAN_POINT('Ctrl Pts',(-0.300999190531556,2.21515613780619,
5.6174151464042));
#52210=CARTESIAN_POINT('Ctrl Pts',(-0.300812045404396,2.21564411835274,
5.61738297070147));
#52211=CARTESIAN_POINT('Ctrl Pts',(-0.300304982880674,2.21695672377719,
5.61729623299978));
#52212=CARTESIAN_POINT('Ctrl Pts',(-0.2999828579708,2.21778048598279,5.61724159689273));
#52213=CARTESIAN_POINT('Ctrl Pts',(-0.297626458039936,2.22373407164333,
5.61684525043928));
#52214=CARTESIAN_POINT('Ctrl Pts',(-0.295464217979859,2.22881195138932,
5.61649923736257));
#52215=CARTESIAN_POINT('Ctrl Pts',(-0.280736314402415,2.26107504369753,
5.61424720354848));
#52216=CARTESIAN_POINT('Ctrl Pts',(-0.264564745827502,2.28644791314324,
5.61220782711879));
#52217=CARTESIAN_POINT('Ctrl Pts',(-0.241056891363572,2.31399095526909,
5.60976901817959));
#52218=CARTESIAN_POINT('Ctrl Pts',(-0.236844384934662,2.31864422515869,
5.6093487271038));
#52219=CARTESIAN_POINT('Ctrl Pts',(-0.226727449209503,2.32918397084104,
5.60838209454529));
#52220=CARTESIAN_POINT('Ctrl Pts',(-0.220724721958581,2.33497074926955,
5.60783993687223));
#52221=CARTESIAN_POINT('Ctrl Pts',(-0.213590463087684,2.34133335337852,
5.60723698184769));
#52222=CARTESIAN_POINT('Ctrl Pts',(-0.212672452975688,2.34214272905507,
5.60716014800779));
#52223=CARTESIAN_POINT('Ctrl Pts',(-0.211536672999875,2.34313266246771,
5.60706603358822));
#52224=CARTESIAN_POINT('Ctrl Pts',(-0.211323263392496,2.34331817427618,
5.60704839058749));
#52225=CARTESIAN_POINT('Ctrl Pts',(-0.210946452236227,2.34364485741056,
5.60701731118726));
#52226=CARTESIAN_POINT('Ctrl Pts',(-0.210783152840374,2.34378614549024,
5.60700386613649));
#52227=CARTESIAN_POINT('Ctrl Pts',(-0.210461243165171,2.34406409933609,
5.60697740933828));
#52228=CARTESIAN_POINT('Ctrl Pts',(-0.210302641353411,2.34420077497864,
5.60696439685787));
#52229=CARTESIAN_POINT('Ctrl Pts',(-0.209985884796363,2.34447320354668,
5.60693845365359));
#52230=CARTESIAN_POINT('Ctrl Pts',(-0.209827731937787,2.34460895726968,
5.60692552285198));
#52231=CARTESIAN_POINT('Ctrl Pts',(-0.209448290020109,2.34493402017479,
5.60689455233638));
#52232=CARTESIAN_POINT('Ctrl Pts',(-0.209226875373001,2.34512318342933,
5.60687652348263));
#52233=CARTESIAN_POINT('Ctrl Pts',(-0.208551515742056,2.3456985880163,5.60682166245034));
#52234=CARTESIAN_POINT('Ctrl Pts',(-0.208096752161335,2.34608387315052,
5.60678490034494));
#52235=CARTESIAN_POINT('Ctrl Pts',(-0.203094589444473,2.35029802707084,
5.60638246695065));
#52236=CARTESIAN_POINT('Ctrl Pts',(-0.198442798180099,2.35400193197372,
5.60602567825957));
#52237=CARTESIAN_POINT('Ctrl Pts',(-0.192125087800912,2.35875270851616,
5.60555980390401));
#52238=CARTESIAN_POINT('Ctrl Pts',(-0.190548595769804,2.35991584499391,
5.60544504616141));
#52239=CARTESIAN_POINT('Ctrl Pts',(-0.186044019973122,2.36317630939819,
5.60512105640865));
#52240=CARTESIAN_POINT('Ctrl Pts',(-0.183091193228606,2.36523906889371,
5.60491330171789));
#52241=CARTESIAN_POINT('Ctrl Pts',(-0.170188558587899,2.3739343105364,5.60402245979363));
#52242=CARTESIAN_POINT('Ctrl Pts',(-0.159908145039865,2.38005992486704,
5.60335515927367));
#52243=CARTESIAN_POINT('Ctrl Pts',(-0.138919793281672,2.39103255459073,
5.60203139366968));
#52244=CARTESIAN_POINT('Ctrl Pts',(-0.128240444816175,2.39589361271516,
5.60137591776683));
#52245=CARTESIAN_POINT('Ctrl Pts',(-0.104445479932888,2.40519404126875,
5.59991886336068));
#52246=CARTESIAN_POINT('Ctrl Pts',(-0.0912616916947774,2.40939213591887,
5.59911337662482));
#52247=CARTESIAN_POINT('Ctrl Pts',(-0.075625730148757,2.41328450242906,
5.59814054523436));
#52248=CARTESIAN_POINT('Ctrl Pts',(-0.0733954634364382,2.41381449305269,
5.59800140145558));
#52249=CARTESIAN_POINT('Ctrl Pts',(-0.070486325258787,2.41447309957748,
5.59781934661265));
#52250=CARTESIAN_POINT('Ctrl Pts',(-0.0698123903187466,2.41462339797391,
5.59777713284705));
#52251=CARTESIAN_POINT('Ctrl Pts',(-0.0687179137772091,2.41486379423668,
5.5977085127213));
#52252=CARTESIAN_POINT('Ctrl Pts',(-0.068297663235841,2.4149552187037,5.59768214894994));
#52253=CARTESIAN_POINT('Ctrl Pts',(-0.0674916840483304,2.41512886849212,
5.59763155702704));
#52254=CARTESIAN_POINT('Ctrl Pts',(-0.0671059847544436,2.41521122756137,
5.59760733321087));
#52255=CARTESIAN_POINT('Ctrl Pts',(-0.0662272027631062,2.41539718943548,
5.59755211092834));
#52256=CARTESIAN_POINT('Ctrl Pts',(-0.065734027222259,2.41550034413637,
5.59752109818129));
#52257=CARTESIAN_POINT('Ctrl Pts',(-0.0642004364224219,2.41581736461536,
5.59742459124282));
#52258=CARTESIAN_POINT('Ctrl Pts',(-0.0631592122802672,2.41602724200659,
5.59735896976916));
#52259=CARTESIAN_POINT('Ctrl Pts',(-0.0550916063346578,2.41761194996385,
5.59684973442431));
#52260=CARTESIAN_POINT('Ctrl Pts',(-0.0480226978021161,2.41875734205157,
5.5963988513845));
#52261=CARTESIAN_POINT('Ctrl Pts',(-0.0166224788965305,2.42277702701247,
5.59437311177226));
#52262=CARTESIAN_POINT('Ctrl Pts',(0.00794889355132273,2.42310640497271,
5.59271906379305));
#52263=CARTESIAN_POINT('Ctrl Pts',(0.0452498315668607,2.41934718794867,
5.59018347818709));
#52264=CARTESIAN_POINT('Ctrl Pts',(0.0580944713752727,2.41726212211376,
5.58930776522828));
#52265=CARTESIAN_POINT('Ctrl Pts',(0.0748610267401189,2.41348765742933,
5.58818655603967));
#52266=CARTESIAN_POINT('Ctrl Pts',(0.0789251841231117,2.41248920574225,
5.58791656508703));
#52267=CARTESIAN_POINT('Ctrl Pts',(0.0843454038256706,2.41104510540197,
5.5875599138755));
#52268=CARTESIAN_POINT('Ctrl Pts',(0.085719441284082,2.41066924903883,5.58746980004196));
#52269=CARTESIAN_POINT('Ctrl Pts',(0.0880120566407711,2.41002575497828,
5.58731999396892));
#52270=CARTESIAN_POINT('Ctrl Pts',(0.0889320012921847,2.40976311927848,
5.58726003111411));
#52271=CARTESIAN_POINT('Ctrl Pts',(0.0901817069604152,2.40940031367109,
5.58717878998671));
#52272=CARTESIAN_POINT('Ctrl Pts',(0.0905124849656022,2.40930370905965,
5.58715730731663));
#52273=CARTESIAN_POINT('Ctrl Pts',(0.091038990828018,2.40914902467175,5.5871231464867));
#52274=CARTESIAN_POINT('Ctrl Pts',(0.0912348183551359,2.40909128947083,
5.5871104481771));
#52275=CARTESIAN_POINT('Ctrl Pts',(0.0916422497778111,2.40897074683744,
5.58708404414975));
#52276=CARTESIAN_POINT('Ctrl Pts',(0.0918538434674642,2.40890790826087,
5.58707034039601));
#52277=CARTESIAN_POINT('Ctrl Pts',(0.0923416882031542,2.40876248376283,
5.58703876541266));
#52278=CARTESIAN_POINT('Ctrl Pts',(0.0926178939513587,2.4086797442029,5.587020903232));
#52279=CARTESIAN_POINT('Ctrl Pts',(0.0934999868431434,2.4084142159406,5.58696390463703));
#52280=CARTESIAN_POINT('Ctrl Pts',(0.094105451527379,2.40823001174897,5.58692485075662));
#52281=CARTESIAN_POINT('Ctrl Pts',(0.0995025782770252,2.40657062587088,
5.58657731345047));
#52282=CARTESIAN_POINT('Ctrl Pts',(0.104260072483303,2.40498550097454,5.58627511605419));
#52283=CARTESIAN_POINT('Ctrl Pts',(0.10925247496056,2.40319161732123,5.58596050949557));
#52284=CARTESIAN_POINT('Ctrl Pts',(0.109525864949491,2.40309296429817,5.58594328930999));
#52285=CARTESIAN_POINT('Ctrl Pts',(0.110096305234112,2.4028862478135,5.58590737471497));
#52286=CARTESIAN_POINT('Ctrl Pts',(0.110393330904645,2.40277811683474,5.58588868326479));
#52287=CARTESIAN_POINT('Ctrl Pts',(0.111022508505319,2.40254801838721,5.58584910829398));
#52288=CARTESIAN_POINT('Ctrl Pts',(0.111354619825424,2.40242594047179,5.58582822952333));
#52289=CARTESIAN_POINT('Ctrl Pts',(0.115022333895595,2.40107089658345,5.58559776541093));
#52290=CARTESIAN_POINT('Ctrl Pts',(0.118337623895132,2.3997833059733,5.58539048105336));
#52291=CARTESIAN_POINT('Ctrl Pts',(0.144040852626672,2.38930783664311,5.58378662377446));
#52292=CARTESIAN_POINT('Ctrl Pts',(0.16535174501644,2.37767921977826,5.58247038806492));
#52293=CARTESIAN_POINT('Ctrl Pts',(0.194784497416539,2.35701832717525,5.5804287686262));
#52294=CARTESIAN_POINT('Ctrl Pts',(0.204030193583439,2.3497419894129,5.57975023669485));
#52295=CARTESIAN_POINT('Ctrl Pts',(0.216969935110882,2.33835944860819,5.5787269029175));
#52296=CARTESIAN_POINT('Ctrl Pts',(0.220989615412571,2.33463751585345,5.57839765457339));
#52297=CARTESIAN_POINT('Ctrl Pts',(0.225564157568056,2.33017996168354,5.57800854652139));
#52298=CARTESIAN_POINT('Ctrl Pts',(0.226213290341575,2.32954204666287,5.57795298260532));
#52299=CARTESIAN_POINT('Ctrl Pts',(0.227199444637828,2.32856468838087,5.577868031874));
#52300=CARTESIAN_POINT('Ctrl Pts',(0.227538430694672,2.32822722662175,5.57783873249537));
#52301=CARTESIAN_POINT('Ctrl Pts',(0.228126478642944,2.3276392105419,5.57778773479919));
#52302=CARTESIAN_POINT('Ctrl Pts',(0.228375882803651,2.32738899838434,5.57776605167804));
#52303=CARTESIAN_POINT('Ctrl Pts',(0.228894762443821,2.32686672295988,5.57772082770776));
#52304=CARTESIAN_POINT('Ctrl Pts',(0.229164165321277,2.32659458861897,5.57769728370942));
#52305=CARTESIAN_POINT('Ctrl Pts',(0.22982192464791,2.32592778748829,5.57763964355417));
#52306=CARTESIAN_POINT('Ctrl Pts',(0.230209749182459,2.3255325998242,5.57760552412588));
#52307=CARTESIAN_POINT('Ctrl Pts',(0.231689606007087,2.32401685268078,5.57747481587128));
#52308=CARTESIAN_POINT('Ctrl Pts',(0.232774476901877,2.32288935950636,5.57737791535311));
#52309=CARTESIAN_POINT('Ctrl Pts',(0.250818142789262,2.30386138151041,5.5757478669752));
#52310=CARTESIAN_POINT('Ctrl Pts',(0.265671981487004,2.28408453242568,5.57412163651124));
#52311=CARTESIAN_POINT('Ctrl Pts',(0.286088100268379,2.2492088093593,5.57139342084446));
#52312=CARTESIAN_POINT('Ctrl Pts',(0.293043198854065,2.23503843736152,5.57031988158593));
#52313=CARTESIAN_POINT('Ctrl Pts',(0.302155152959246,2.21241789438034,5.5687037257685));
#52314=CARTESIAN_POINT('Ctrl Pts',(0.305054877336514,2.20429319618573,5.56814183355806));
#52315=CARTESIAN_POINT('Ctrl Pts',(0.307888536123916,2.19521871648552,5.567541627799));
#52316=CARTESIAN_POINT('Ctrl Pts',(0.308148162451034,2.19437512736893,5.56748608841484));
#52317=CARTESIAN_POINT('Ctrl Pts',(0.308536607966969,2.19309427979843,5.56740216243215));
#52318=CARTESIAN_POINT('Ctrl Pts',(0.308667968053393,2.19265780534169,5.56737363343976));
#52319=CARTESIAN_POINT('Ctrl Pts',(0.308905036577128,2.19186399112005,5.56732187775726));
#52320=CARTESIAN_POINT('Ctrl Pts',(0.309011051793809,2.19150674488712,5.56729863348237));
#52321=CARTESIAN_POINT('Ctrl Pts',(0.309184255345128,2.19091935629904,5.56726049428884));
#52322=CARTESIAN_POINT('Ctrl Pts',(0.309251806556559,2.19068932266567,5.56724557815371));
#52323=CARTESIAN_POINT('Ctrl Pts',(0.309380640668503,2.19024878321796,5.56721705063938));
#52324=CARTESIAN_POINT('Ctrl Pts',(0.309441964945319,2.19003829198646,5.56720343695138));
#52325=CARTESIAN_POINT('Ctrl Pts',(0.309581812423942,2.18955644499399,5.56717231145856));
#52326=CARTESIAN_POINT('Ctrl Pts',(0.309660193554651,2.18928504887613,5.56715480807657));
#52327=CARTESIAN_POINT('Ctrl Pts',(0.309900162912094,2.1884500335086,5.56710103912815));
#52328=CARTESIAN_POINT('Ctrl Pts',(0.310060571095411,2.18788607207843,5.56706484228345));
#52329=CARTESIAN_POINT('Ctrl Pts',(0.311258294179271,2.18363103456128,5.56679260890275));
#52330=CARTESIAN_POINT('Ctrl Pts',(0.31223126041805,2.17992195449762,5.56656022714857));
#52331=CARTESIAN_POINT('Ctrl Pts',(0.319877979054682,2.14849680332227,5.56462585872826));
#52332=CARTESIAN_POINT('Ctrl Pts',(0.322914036391696,2.1200217707311,5.56308899038667));
#52333=CARTESIAN_POINT('Ctrl Pts',(0.321681648631028,2.07322696637732,5.56044175154729));
#52334=CARTESIAN_POINT('Ctrl Pts',(0.319643736414476,2.05501544886811,5.55938282200033));
#52335=CARTESIAN_POINT('Ctrl Pts',(0.31584226296129,2.03592011826925,5.55819908850671));
#52336=CARTESIAN_POINT('Ctrl Pts',(0.315605668634554,2.03476482403635,5.55812719148735));
#52337=CARTESIAN_POINT('Ctrl Pts',(0.31525323014185,2.03309066498481,5.55802258961092));
#52338=CARTESIAN_POINT('Ctrl Pts',(0.315142432624692,2.03257073794644,5.55799004631638));
#52339=CARTESIAN_POINT('Ctrl Pts',(0.314946580069697,2.03166271015351,5.55793310850854));
#52340=CARTESIAN_POINT('Ctrl Pts',(0.314862092590016,2.03127448706113,5.55790873222972));
#52341=CARTESIAN_POINT('Ctrl Pts',(0.314697279025021,2.03052384582689,5.55786153612446));
#52342=CARTESIAN_POINT('Ctrl Pts',(0.314617044201586,2.03016140808618,5.55783871925944));
#52343=CARTESIAN_POINT('Ctrl Pts',(0.31442499543357,2.02930093057116,5.55778448001617));
#52344=CARTESIAN_POINT('Ctrl Pts',(0.314312624355159,2.02880301735542,5.55775303978618));
#52345=CARTESIAN_POINT('Ctrl Pts',(0.313911724398085,2.02704608794736,5.55764190520414));
#52346=CARTESIAN_POINT('Ctrl Pts',(0.31361681275725,2.02578855427604,5.55756200589506));
#52347=CARTESIAN_POINT('Ctrl Pts',(0.308828687669785,2.00590986330908,5.5562932808023));
#52348=CARTESIAN_POINT('Ctrl Pts',(0.302692483323738,1.9877274079924,5.55504991078165));
#52349=CARTESIAN_POINT('Ctrl Pts',(0.286572249620751,1.95109304796924,5.55237630930414));
#52350=CARTESIAN_POINT('Ctrl Pts',(0.276328586488783,1.93284914620568,5.55094532589311));
#52351=CARTESIAN_POINT('Ctrl Pts',(0.259065692322445,1.90808089219873,5.54893886601025));
#52352=CARTESIAN_POINT('Ctrl Pts',(0.253408900484507,1.90067127131184,5.54832998675162));
#52353=CARTESIAN_POINT('Ctrl Pts',(0.246847091766642,1.89280796198838,5.54768301353209));
#52354=CARTESIAN_POINT('Ctrl Pts',(0.246252749083555,1.89210192173584,5.54762491577301));
#52355=CARTESIAN_POINT('Ctrl Pts',(0.245350611575097,1.89103953792361,5.54753749858085));
#52356=CARTESIAN_POINT('Ctrl Pts',(0.245045061366366,1.8906813070507,5.54750802241737));
#52357=CARTESIAN_POINT('Ctrl Pts',(0.24448245293286,1.89002461814585,5.54745399137531));
#52358=CARTESIAN_POINT('Ctrl Pts',(0.244225631133095,1.88972596004632,5.54742941954106));
#52359=CARTESIAN_POINT('Ctrl Pts',(0.243811762763354,1.88924645357406,5.54738997149742));
#52360=CARTESIAN_POINT('Ctrl Pts',(0.243655062029273,1.88906530929861,5.54737506979359));
#52361=CARTESIAN_POINT('Ctrl Pts',(0.243354499688415,1.88871864445932,5.54734655324297));
#52362=CARTESIAN_POINT('Ctrl Pts',(0.243210672265955,1.88855309741232,5.54733293612317));
#52363=CARTESIAN_POINT('Ctrl Pts',(0.242880878483438,1.88817428258693,5.54730177806359));
#52364=CARTESIAN_POINT('Ctrl Pts',(0.242694800429434,1.88796111315036,5.54728424560988));
#52365=CARTESIAN_POINT('Ctrl Pts',(0.242120708284581,1.88730518380969,5.54723029986725));
#52366=CARTESIAN_POINT('Ctrl Pts',(0.24173175877594,1.88686323867884,5.54719395595913));
#52367=CARTESIAN_POINT('Ctrl Pts',(0.23876515558105,1.88351099288898,5.54691828101456));
#52368=CARTESIAN_POINT('Ctrl Pts',(0.236136103796485,1.88064632784557,5.54668270907939));
#52369=CARTESIAN_POINT('Ctrl Pts',(0.218386483405086,1.86199508612996,5.54514339696968));
#52370=CARTESIAN_POINT('Ctrl Pts',(0.201743263827784,1.84773247586465,5.54393662698129));
#52371=CARTESIAN_POINT('Ctrl Pts',(0.171893058436623,1.82701021600114,5.54190381826153));
#52372=CARTESIAN_POINT('Ctrl Pts',(0.1594621487787,1.81956743111643,5.54108988203961));
#52373=CARTESIAN_POINT('Ctrl Pts',(0.138923495294645,1.80907865097454,5.53975132959784));
#52374=CARTESIAN_POINT('Ctrl Pts',(0.131120492790419,1.80547943019854,5.53924433937148));
#52375=CARTESIAN_POINT('Ctrl Pts',(0.120817149001653,1.80121755419973,5.53857218626622));
#52376=CARTESIAN_POINT('Ctrl Pts',(0.118439254674684,1.80026699250859,5.53841689000507));
#52377=CARTESIAN_POINT('Ctrl Pts',(0.115379813999428,1.79908607421293,5.53821677982533));
#52378=CARTESIAN_POINT('Ctrl Pts',(0.114708431897085,1.79882950368659,5.53817284795284));
#52379=CARTESIAN_POINT('Ctrl Pts',(0.113628034736405,1.79842076365864,5.5381021204522));
#52380=CARTESIAN_POINT('Ctrl Pts',(0.113219556454756,1.7982671743023,5.53807537241661));
#52381=CARTESIAN_POINT('Ctrl Pts',(0.112442776375343,1.79797690155428,5.5380244928686));
#52382=CARTESIAN_POINT('Ctrl Pts',(0.112074533865669,1.79784006087773,5.53800036666766));
#52383=CARTESIAN_POINT('Ctrl Pts',(0.111236901310936,1.79753053450036,5.53794547307336));
#52384=CARTESIAN_POINT('Ctrl Pts',(0.11076735845625,1.79735826779999,5.53791469176346));
#52385=CARTESIAN_POINT('Ctrl Pts',(0.109374182318071,1.79685081342981,5.53782332954755));
#52386=CARTESIAN_POINT('Ctrl Pts',(0.108449421256802,1.79651875828853,5.5377626445148));
#52387=CARTESIAN_POINT('Ctrl Pts',(0.102108813984313,1.79427471014231,5.53734626252508));
#52388=CARTESIAN_POINT('Ctrl Pts',(0.0966445109294405,1.7925036676583,5.5369859225265));
#52389=CARTESIAN_POINT('Ctrl Pts',(0.0907289859771921,1.79075962932198,
5.53659388296296));
#52390=CARTESIAN_POINT('Ctrl Pts',(0.0903216591450512,1.79064041369291,
5.53656687854313));
#52391=CARTESIAN_POINT('Ctrl Pts',(0.0886600624377844,1.79015766217774,
5.536456680646));
#52392=CARTESIAN_POINT('Ctrl Pts',(0.087403837090714,1.78980095074159,5.53637327533756));
#52393=CARTESIAN_POINT('Ctrl Pts',(0.0821430834479778,1.78834162705317,
5.5360236078192));
#52394=CARTESIAN_POINT('Ctrl Pts',(0.0781197320298171,1.78730888621358,
5.53575524436712));
#52395=CARTESIAN_POINT('Ctrl Pts',(0.0733754512296643,1.78618836953102,
5.5354377312728));
#52396=CARTESIAN_POINT('Ctrl Pts',(0.0726726695424535,1.78602487463092,
5.53539067033124));
#52397=CARTESIAN_POINT('Ctrl Pts',(0.0452782300744373,1.77974874471338,
5.53355520272233));
#52398=CARTESIAN_POINT('Ctrl Pts',(0.0179176133821994,1.77706098853155,
5.53167013730327));
#52399=CARTESIAN_POINT('Ctrl Pts',(-0.0204371709266751,1.77818579322911,
5.52911314851227));
#52400=CARTESIAN_POINT('Ctrl Pts',(-0.0314049840513607,1.77907033868226,
5.52839368869949));
#52401=CARTESIAN_POINT('Ctrl Pts',(-0.0430107190615122,1.78060720556087,
5.52765918893693));
#52402=CARTESIAN_POINT('Ctrl Pts',(-0.0437138321390117,1.7807026777497,
5.52761479679176));
#52403=CARTESIAN_POINT('Ctrl Pts',(-0.0447191707553591,1.78084257067414,
5.52755148077596));
#52404=CARTESIAN_POINT('Ctrl Pts',(-0.0450216509713219,1.78088509926265,
5.52753245106234));
#52405=CARTESIAN_POINT('Ctrl Pts',(-0.045544585611618,1.78095938196836,
5.5274995879323));
#52406=CARTESIAN_POINT('Ctrl Pts',(-0.0457650680545207,1.7809909346434,
5.52748574304313));
#52407=CARTESIAN_POINT('Ctrl Pts',(-0.0461898915057663,1.78105217952795,
5.52745908831937));
#52408=CARTESIAN_POINT('Ctrl Pts',(-0.046394236240263,1.78108183948626,
5.52744627665958));
#52409=CARTESIAN_POINT('Ctrl Pts',(-0.0468794533654436,1.78115274335968,
5.52741587773129));
#52410=CARTESIAN_POINT('Ctrl Pts',(-0.0471603006068751,1.78119416212528,
5.52739830043288));
#52411=CARTESIAN_POINT('Ctrl Pts',(-0.0480015937746501,1.78131937031146,
5.52734569911124));
#52412=CARTESIAN_POINT('Ctrl Pts',(-0.0485618775625521,1.78140426744435,
5.52731073746318));
#52413=CARTESIAN_POINT('Ctrl Pts',(-0.0539781445485369,1.78223958839544,
5.52697341238737));
#52414=CARTESIAN_POINT('Ctrl Pts',(-0.0588169111640388,1.78309954773733,
5.52667710352944));
#52415=CARTESIAN_POINT('Ctrl Pts',(-0.084332624892313,1.78823890566646,
5.52513244071494));
#52416=CARTESIAN_POINT('Ctrl Pts',(-0.104573500604656,1.79443238944892,
5.52396705467592));
#52417=CARTESIAN_POINT('Ctrl Pts',(-0.146746379755469,1.81202319796713,
5.52141013587774));
#52418=CARTESIAN_POINT('Ctrl Pts',(-0.168267518248396,1.82404543989153,
5.52001706245288));
#52419=CARTESIAN_POINT('Ctrl Pts',(-0.189148382601726,1.83906821850734,
5.51845284771341));
#52420=CARTESIAN_POINT('Ctrl Pts',(-0.190080764579235,1.83974664629125,
5.51838253856672));
#52421=CARTESIAN_POINT('Ctrl Pts',(-0.191433725550719,1.84074224833561,
5.5182798290341));
#52422=CARTESIAN_POINT('Ctrl Pts',(-0.191857206859456,1.84105547843758,
5.51824758205778));
#52423=CARTESIAN_POINT('Ctrl Pts',(-0.192598136206746,1.8416063259489,5.51819098835226));
#52424=CARTESIAN_POINT('Ctrl Pts',(-0.192915917994448,1.84184349428685,
5.51816665919711));
#52425=CARTESIAN_POINT('Ctrl Pts',(-0.193531428825687,1.84230463626849,
5.51811942631984));
#52426=CARTESIAN_POINT('Ctrl Pts',(-0.193829208934796,1.84252854101099,
5.51809652532178));
#52427=CARTESIAN_POINT('Ctrl Pts',(-0.194538159041054,1.8430635367628,5.51804188316562));
#52428=CARTESIAN_POINT('Ctrl Pts',(-0.194948971105843,1.84337509839502,
5.51801012353151));
#52429=CARTESIAN_POINT('Ctrl Pts',(-0.196185715622039,1.8443177342251,5.51791421909141));
#52430=CARTESIAN_POINT('Ctrl Pts',(-0.197009338338682,1.84495181511588,
5.51784995568372));
#52431=CARTESIAN_POINT('Ctrl Pts',(-0.205529952321285,1.85157746294606,
5.5171809854742));
#52432=CARTESIAN_POINT('Ctrl Pts',(-0.212953473613203,1.85791096027722,
5.51656261252825));
#52433=CARTESIAN_POINT('Ctrl Pts',(-0.24124684114183,1.88435942972498,5.51405591492634));
#52434=CARTESIAN_POINT('Ctrl Pts',(-0.259648439283121,1.90691170300002,
5.51206297579435));
#52435=CARTESIAN_POINT('Ctrl Pts',(-0.280391262687232,1.94076103499131,
5.50941123382913));
#52436=CARTESIAN_POINT('Ctrl Pts',(-0.285537899331651,1.95018522254025,
5.50870605616307));
#52437=CARTESIAN_POINT('Ctrl Pts',(-0.290863299134398,1.96121236700717,
5.50793165752933));
#52438=CARTESIAN_POINT('Ctrl Pts',(-0.291511830774746,1.96257977373401,
5.50783649470384));
#52439=CARTESIAN_POINT('Ctrl Pts',(-0.292323324783649,1.96432237993624,
5.50771636381122));
#52440=CARTESIAN_POINT('Ctrl Pts',(-0.292495224231355,1.96469336082445,
5.50769085481153));
#52441=CARTESIAN_POINT('Ctrl Pts',(-0.292768914117127,1.96528697732778,
5.50765014298082));
#52442=CARTESIAN_POINT('Ctrl Pts',(-0.292871156985432,1.96550940197255,
5.50763491219748));
#52443=CARTESIAN_POINT('Ctrl Pts',(-0.293064481410822,1.96593123622593,
5.5076060718226));
#52444=CARTESIAN_POINT('Ctrl Pts',(-0.293155612172093,1.96613062061551,
5.50759245927366));
#52445=CARTESIAN_POINT('Ctrl Pts',(-0.293363641502988,1.96658699771594,
5.50756134468426));
#52446=CARTESIAN_POINT('Ctrl Pts',(-0.293480405678589,1.96684405075803,
5.50754385104543));
#52447=CARTESIAN_POINT('Ctrl Pts',(-0.29383828833047,1.96763467685022,5.50749014127575));
#52448=CARTESIAN_POINT('Ctrl Pts',(-0.2940782923008,1.96816875760393,5.50745399364673));
#52449=CARTESIAN_POINT('Ctrl Pts',(-0.295871612673212,1.97218869999091,
5.50718290196735));
#52450=CARTESIAN_POINT('Ctrl Pts',(-0.297364438556444,1.97570143447405,
5.5069515784283));
#52451=CARTESIAN_POINT('Ctrl Pts',(-0.299015871428391,1.97978755060825,
5.50668794942587));
#52452=CARTESIAN_POINT('Ctrl Pts',(-0.299235647092606,1.98033567000145,
5.50665269797099));
#52453=CARTESIAN_POINT('Ctrl Pts',(-0.299524662214626,1.98106224742794,
5.5066061138241));
#52454=CARTESIAN_POINT('Ctrl Pts',(-0.299595249622022,1.98124016391923,
5.50659471825437));
#52455=CARTESIAN_POINT('Ctrl Pts',(-0.309405440580394,2.00603128812938,
5.5050084255159));
#52456=CARTESIAN_POINT('Ctrl Pts',(-0.316076986674191,2.03175368944994,
5.50357282733193));
#52457=CARTESIAN_POINT('Ctrl Pts',(-0.321352720171683,2.07189531632057,
5.50129002417703));
#52458=CARTESIAN_POINT('Ctrl Pts',(-0.322270453599861,2.08588834095574,
5.50048798708834));
#52459=CARTESIAN_POINT('Ctrl Pts',(-0.322276865982724,2.10571836699165,
5.49931308438835));
#52460=CARTESIAN_POINT('Ctrl Pts',(-0.322120953444255,2.11153962048963,
5.49896364380085));
#52461=CARTESIAN_POINT('Ctrl Pts',(-0.321754330544614,2.11833848495581,
5.49854914231889));
#52462=CARTESIAN_POINT('Ctrl Pts',(-0.321696675001192,2.11932352229539,
5.49848893226455));
#52463=CARTESIAN_POINT('Ctrl Pts',(-0.32160292400506,2.12080831412132,5.49839793447864));
#52464=CARTESIAN_POINT('Ctrl Pts',(-0.321570184916,2.1213082808735,5.49836725211402));
#52465=CARTESIAN_POINT('Ctrl Pts',(-0.321509689437627,2.12220021695701,
5.49831244092881));
#52466=CARTESIAN_POINT('Ctrl Pts',(-0.321482381764131,2.12259221654261,
5.49828832624326));
#52467=CARTESIAN_POINT('Ctrl Pts',(-0.321423269456043,2.12341895573335,
5.49823741330481));
#52468=CARTESIAN_POINT('Ctrl Pts',(-0.321391299615117,2.12385368240307,
5.49821060990921));
#52469=CARTESIAN_POINT('Ctrl Pts',(-0.321304447842629,2.12500281608028,
5.49813967473842));
#52470=CARTESIAN_POINT('Ctrl Pts',(-0.321248065443725,2.12571710424626,
5.49809549590099));
#52471=CARTESIAN_POINT('Ctrl Pts',(-0.320981096913841,2.12896127990309,
5.49789444588954));
#52472=CARTESIAN_POINT('Ctrl Pts',(-0.320743009109898,2.13148875709897,
5.497736712605));
#52473=CARTESIAN_POINT('Ctrl Pts',(-0.319573011103134,2.14251260403641,
5.49704377104744));
#52474=CARTESIAN_POINT('Ctrl Pts',(-0.318333237040021,2.15097213975549,
5.49649896493205));
#52475=CARTESIAN_POINT('Ctrl Pts',(-0.314107253280467,2.17351849097337,
5.49501078221769));
#52476=CARTESIAN_POINT('Ctrl Pts',(-0.310511220005795,2.18747022524484,
5.49405068676668));
#52477=CARTESIAN_POINT('Ctrl Pts',(-0.298216336676489,2.22467027582034,
5.49140730119232));
#52478=CARTESIAN_POINT('Ctrl Pts',(-0.287747183095027,2.24723255818079,
5.48970685774586));
#52479=CARTESIAN_POINT('Ctrl Pts',(-0.274057626765783,2.26957470275187,
5.48805096014037));
#52480=CARTESIAN_POINT('Ctrl Pts',(-0.273313285612628,2.27077180880458,
5.48796234884667));
#52481=CARTESIAN_POINT('Ctrl Pts',(-0.272338916771984,2.27231617281539,
5.48784821907437));
#52482=CARTESIAN_POINT('Ctrl Pts',(-0.272116051929462,2.27266789883835,
5.4878222388131));
#52483=CARTESIAN_POINT('Ctrl Pts',(-0.271773386558472,2.27320638328987,
5.48778248415051));
#52484=CARTESIAN_POINT('Ctrl Pts',(-0.271654074864119,2.2733934498885,5.48776867740044));
#52485=CARTESIAN_POINT('Ctrl Pts',(-0.271418329197102,2.27376223058336,
5.48774146669893));
#52486=CARTESIAN_POINT('Ctrl Pts',(-0.2713019065783,2.27394394984873,5.48772806218924));
#52487=CARTESIAN_POINT('Ctrl Pts',(-0.27104168059063,2.27434922903433,5.48769817509327));
#52488=CARTESIAN_POINT('Ctrl Pts',(-0.270897783503091,2.27457272747079,
5.48768169892199));
#52489=CARTESIAN_POINT('Ctrl Pts',(-0.270479786466916,2.27522019179964,
5.48763398370626));
#52490=CARTESIAN_POINT('Ctrl Pts',(-0.2702049650226,2.27564369441235,5.48760279272412));
#52491=CARTESIAN_POINT('Ctrl Pts',(-0.268297965560087,2.27856733169868,
5.48738758729749));
#52492=CARTESIAN_POINT('Ctrl Pts',(-0.266632038985412,2.28104542965493,
5.48720578822395));
#52493=CARTESIAN_POINT('Ctrl Pts',(-0.261313809145535,2.28872372658117,
5.48664322048206));
#52494=CARTESIAN_POINT('Ctrl Pts',(-0.257541824439113,2.29383955116145,
5.48626945668818));
#52495=CARTESIAN_POINT('Ctrl Pts',(-0.243925213799659,2.3112074908391,5.48499168185766));
#52496=CARTESIAN_POINT('Ctrl Pts',(-0.233337482866846,2.32284927202884,
5.48411842030749));
#52497=CARTESIAN_POINT('Ctrl Pts',(-0.203686367941892,2.35101186068546,
5.48183186884205));
#52498=CARTESIAN_POINT('Ctrl Pts',(-0.183465026390983,2.36614924189718,
5.48041133467795));
#52499=CARTESIAN_POINT('Ctrl Pts',(-0.160376112338425,2.37954066762215,
5.47879259165192));
#52500=CARTESIAN_POINT('Ctrl Pts',(-0.159056980070522,2.3802933449642,5.47870015395734));
#52501=CARTESIAN_POINT('Ctrl Pts',(-0.157255744966577,2.38130429309308,
5.47857397689779));
#52502=CARTESIAN_POINT('Ctrl Pts',(-0.156778217671602,2.3815707106492,5.47854053014247));
#52503=CARTESIAN_POINT('Ctrl Pts',(-0.155966804355902,2.38202070268487,
5.4784837036182));
#52504=CARTESIAN_POINT('Ctrl Pts',(-0.155633265448059,2.38220490337309,
5.4784603463042));
#52505=CARTESIAN_POINT('Ctrl Pts',(-0.154989430400462,2.38255898009255,
5.47841526236468));
#52506=CARTESIAN_POINT('Ctrl Pts',(-0.15467917950265,2.38272893766578,5.47839353869087));
#52507=CARTESIAN_POINT('Ctrl Pts',(-0.153945226617312,2.38312943241208,
5.47834215039444));
#52508=CARTESIAN_POINT('Ctrl Pts',(-0.153521286518485,2.38335952935793,
5.47831247013925));
#52509=CARTESIAN_POINT('Ctrl Pts',(-0.152279091326095,2.38403013495172,
5.47822550902477));
#52510=CARTESIAN_POINT('Ctrl Pts',(-0.151459450707467,2.38446805440722,
5.47816813632279));
#52511=CARTESIAN_POINT('Ctrl Pts',(-0.145384368524918,2.3876801641316,5.47774293194926));
#52512=CARTESIAN_POINT('Ctrl Pts',(-0.140055283043021,2.39031190389838,
5.47737010451449));
#52513=CARTESIAN_POINT('Ctrl Pts',(-0.121897577070789,2.39866266305496,
5.47609912247734));
#52514=CARTESIAN_POINT('Ctrl Pts',(-0.108770068955668,2.40368962877323,
5.47517832157192));
#52515=CARTESIAN_POINT('Ctrl Pts',(-0.0668677783807147,2.4166693127497,
5.47224630628456));
#52516=CARTESIAN_POINT('Ctrl Pts',(-0.0372908192370373,2.42149684376432,
5.47017445976105));
#52517=CARTESIAN_POINT('Ctrl Pts',(-0.00598221325780764,2.42222291804165,
5.46819391060895));
#52518=CARTESIAN_POINT('Ctrl Pts',(-0.00449233699372369,2.42224713326685,
5.46810020094994));
#52519=CARTESIAN_POINT('Ctrl Pts',(-0.00257694369039802,2.42226497783755,
5.46798046537174));
#52520=CARTESIAN_POINT('Ctrl Pts',(-0.00215156442677821,2.4222680985684,
5.46795392074176));
#52521=CARTESIAN_POINT('Ctrl Pts',(-0.00147769125543491,2.42227170803633,
5.46791194498887));
#52522=CARTESIAN_POINT('Ctrl Pts',(-0.00122920271492537,2.42227275161544,
5.46789648282019));
#52523=CARTESIAN_POINT('Ctrl Pts',(-0.000784013611597522,2.42227410637275,
5.46786881040482));
#52524=CARTESIAN_POINT('Ctrl Pts',(-0.000587315399775385,2.42227452486449,
5.46785659420002));
#52525=CARTESIAN_POINT('Ctrl Pts',(-0.000124952233957228,2.42227508527478,
5.46782790266901));
#52526=CARTESIAN_POINT('Ctrl Pts',(0.000140712203431249,2.42227507878088,
5.46781143580907));
#52527=CARTESIAN_POINT('Ctrl Pts',(0.000910516995918739,2.42227410808326,
5.46776377390247));
#52528=CARTESIAN_POINT('Ctrl Pts',(0.00141465837598556,2.42227228942604,
5.46773262675243));
#52529=CARTESIAN_POINT('Ctrl Pts',(0.00488875817467803,2.42225160456992,
5.46751843280818));
#52530=CARTESIAN_POINT('Ctrl Pts',(0.00785846043961619,2.42219286571755,
5.46733757767998));
#52531=CARTESIAN_POINT('Ctrl Pts',(0.0171581674030124,2.42188025914563,
5.46677706451395));
#52532=CARTESIAN_POINT('Ctrl Pts',(0.0234820758094596,2.42148080358666,
5.46640438284897));
#52533=CARTESIAN_POINT('Ctrl Pts',(0.0453706828055154,2.4194487605064,5.46513138912766));
#52534=CARTESIAN_POINT('Ctrl Pts',(0.0608258639922243,2.41686951295002,
5.46426163966309));
#52535=CARTESIAN_POINT('Ctrl Pts',(0.100621616762986,2.40720788631713,5.4619719672567));
#52536=CARTESIAN_POINT('Ctrl Pts',(0.124417202303798,2.39836470541229,5.46054490197707));
#52537=CARTESIAN_POINT('Ctrl Pts',(0.148270629436193,2.38614551669515,5.45891934622149));
#52538=CARTESIAN_POINT('Ctrl Pts',(0.149603983702544,2.38545066862605,5.45882782870796));
#52539=CARTESIAN_POINT('Ctrl Pts',(0.151413515484319,2.3844915103285,5.4587027185203));
#52540=CARTESIAN_POINT('Ctrl Pts',(0.151893972011068,2.38423527821379,5.45866941211837));
#52541=CARTESIAN_POINT('Ctrl Pts',(0.152708958603905,2.38379798146093,5.45861276491664));
#52542=CARTESIAN_POINT('Ctrl Pts',(0.153043822841717,2.38361753931514,5.45858944627565));
#52543=CARTESIAN_POINT('Ctrl Pts',(0.153689639730539,2.38326806302306,5.45854439016439));
#52544=CARTESIAN_POINT('Ctrl Pts',(0.154000635106508,2.38309910857253,5.45852265555732));
#52545=CARTESIAN_POINT('Ctrl Pts',(0.154727533717985,2.38270265415583,5.45847176607049));
#52546=CARTESIAN_POINT('Ctrl Pts',(0.155143213740165,2.38247474857724,5.45844259673226));
#52547=CARTESIAN_POINT('Ctrl Pts',(0.156347308056751,2.38181111820341,5.45835790403401));
#52548=CARTESIAN_POINT('Ctrl Pts',(0.157134395470455,2.38137300654721,5.45830229526224));
#52549=CARTESIAN_POINT('Ctrl Pts',(0.158906659632299,2.38037676655368,5.45817651863588));
#52550=CARTESIAN_POINT('Ctrl Pts',(0.159890748660483,2.37981673670239,5.45810628272576));
#52551=CARTESIAN_POINT('Ctrl Pts',(0.16814507790996,2.37506156408967,5.4575137902397));
#52552=CARTESIAN_POINT('Ctrl Pts',(0.175251222535629,2.37058939213237,5.45698151285667));
#52553=CARTESIAN_POINT('Ctrl Pts',(0.188682598976473,2.3613853523159,5.45593029768668));
#52554=CARTESIAN_POINT('Ctrl Pts',(0.195024559863242,2.3566881992054,5.4554128409537));
#52555=CARTESIAN_POINT('Ctrl Pts',(0.219139782126374,2.33741740679355,5.45336369861132));
#52556=CARTESIAN_POINT('Ctrl Pts',(0.235504789198929,2.32119371898361,5.45178545924755));
#52557=CARTESIAN_POINT('Ctrl Pts',(0.256564615673412,2.29530446054654,5.44956552267682));
#52558=CARTESIAN_POINT('Ctrl Pts',(0.262731164915596,2.286926777387,5.44888656224427));
#52559=CARTESIAN_POINT('Ctrl Pts',(0.268890207525898,2.27765071101888,5.44818763724594));
#52560=CARTESIAN_POINT('Ctrl Pts',(0.269295785543312,2.27703530366225,5.44814150860983));
#52561=CARTESIAN_POINT('Ctrl Pts',(0.269856616078544,2.27617793567686,5.44807758319661));
#52562=CARTESIAN_POINT('Ctrl Pts',(0.270013657456531,2.27593715653396,5.44805966777851));
#52563=CARTESIAN_POINT('Ctrl Pts',(0.270283460928864,2.27552227607668,5.44802886242149));
#52564=CARTESIAN_POINT('Ctrl Pts',(0.270396377122332,2.27534827598381,5.44801596212548));
#52565=CARTESIAN_POINT('Ctrl Pts',(0.270629843543588,2.27498775023522,5.44798927327071));
#52566=CARTESIAN_POINT('Ctrl Pts',(0.270750368744672,2.27480120930266,5.44797548646491));
#52567=CARTESIAN_POINT('Ctrl Pts',(0.271034207450663,2.27436090468765,5.44794299698494));
#52568=CARTESIAN_POINT('Ctrl Pts',(0.271197358059685,2.27410703511096,5.44792430527646));
#52569=CARTESIAN_POINT('Ctrl Pts',(0.27173174612678,2.27327292996899,5.44786302555611));
#52570=CARTESIAN_POINT('Ctrl Pts',(0.272101483134963,2.27269172826021,5.44782053713983));
#52571=CARTESIAN_POINT('Ctrl Pts',(0.276846170942745,2.26518032855535,5.44727407700903));
#52572=CARTESIAN_POINT('Ctrl Pts',(0.280957525559753,2.25808617571687,5.44678705146307));
#52573=CARTESIAN_POINT('Ctrl Pts',(0.288506293656836,2.24383389999406,5.44584906930945));
#52574=CARTESIAN_POINT('Ctrl Pts',(0.291958547138894,2.23669049726903,5.44539777012987));
#52575=CARTESIAN_POINT('Ctrl Pts',(0.305341723786479,2.20617157126901,5.44351906431897));
#52576=CARTESIAN_POINT('Ctrl Pts',(0.312754930339056,2.18179421653629,5.44212900298032));
#52577=CARTESIAN_POINT('Ctrl Pts',(0.318819265534685,2.14792436198608,5.44012015199074));
#52578=CARTESIAN_POINT('Ctrl Pts',(0.32003506716393,2.13898719208069,5.43958401303356));
#52579=CARTESIAN_POINT('Ctrl Pts',(0.320979968617445,2.12888453377995,5.43896690539494));
#52580=CARTESIAN_POINT('Ctrl Pts',(0.321079425939802,2.12775713840329,5.438897888472));
#52581=CARTESIAN_POINT('Ctrl Pts',(0.321215667525561,2.1261139413605,5.43879706703203));
#52582=CARTESIAN_POINT('Ctrl Pts',(0.321257152896059,2.12559852936139,5.43876541029212));
#52583=CARTESIAN_POINT('Ctrl Pts',(0.32132825154408,2.12468780136103,5.43870941461969));
#52584=CARTESIAN_POINT('Ctrl Pts',(0.321358376244884,2.1242925254233,5.43868509180328));
#52585=CARTESIAN_POINT('Ctrl Pts',(0.321419218459153,2.12347427279631,5.4386347009419));
#52586=CARTESIAN_POINT('Ctrl Pts',(0.321449830517269,2.12305128924576,5.43860862963398));
#52587=CARTESIAN_POINT('Ctrl Pts',(0.321525268835573,2.12197953676884,5.43854251276637));
#52588=CARTESIAN_POINT('Ctrl Pts',(0.32156896629203,2.12133069254226,5.43850243184295));
#52589=CARTESIAN_POINT('Ctrl Pts',(0.32173675741375,2.11872146038745,5.43834103422671));
#52590=CARTESIAN_POINT('Ctrl Pts',(0.321844888455715,2.11676012083946,5.43821921782391));
#52591=CARTESIAN_POINT('Ctrl Pts',(0.322432636351808,2.10397343947409,5.43742170571779));
#52592=CARTESIAN_POINT('Ctrl Pts',(0.322383897912865,2.09313189967414,5.43672953335399));
#52593=CARTESIAN_POINT('Ctrl Pts',(0.32069052230028,2.06232102646898,5.43471541949836));
#52594=CARTESIAN_POINT('Ctrl Pts',(0.317730829991121,2.04247546417565,5.43335878411516));
#52595=CARTESIAN_POINT('Ctrl Pts',(0.309637878474823,2.00956831758908,5.43106752834243));
#52596=CARTESIAN_POINT('Ctrl Pts',(0.305459779482496,1.99632795488765,5.43013475321236));
#52597=CARTESIAN_POINT('Ctrl Pts',(0.300326460690109,1.98310135483789,5.42921594308472));
#52598=CARTESIAN_POINT('Ctrl Pts',(0.300211262406068,1.98280582711797,5.42919542084632));
#52599=CARTESIAN_POINT('Ctrl Pts',(0.299908418836599,1.98203229410519,5.42914172420527));
#52600=CARTESIAN_POINT('Ctrl Pts',(0.299720066270474,1.98155456444091,5.4291085810546));
#52601=CARTESIAN_POINT('Ctrl Pts',(0.298067112133717,1.97739126987797,5.42881993011546));
#52602=CARTESIAN_POINT('Ctrl Pts',(0.296535653133009,1.97373237148994,5.42856750226994));
#52603=CARTESIAN_POINT('Ctrl Pts',(0.294698281108808,1.96956055280517,5.42828190275605));
#52604=CARTESIAN_POINT('Ctrl Pts',(0.294458109043916,1.9690192826997,5.42824489116837));
#52605=CARTESIAN_POINT('Ctrl Pts',(0.294101931190119,1.9682225040807,5.42819047543847));
#52606=CARTESIAN_POINT('Ctrl Pts',(0.29398708312257,1.96796648410711,5.42817300090714));
#52607=CARTESIAN_POINT('Ctrl Pts',(0.293781759611228,1.96751037185233,5.42814188790965));
#52608=CARTESIAN_POINT('Ctrl Pts',(0.29369141400204,1.96731022198528,5.4281282414526));
#52609=CARTESIAN_POINT('Ctrl Pts',(0.29350059098803,1.96688862615203,5.4280995103009));
#52610=CARTESIAN_POINT('Ctrl Pts',(0.293400067767213,1.96666720211009,5.4280844285301));
#52611=CARTESIAN_POINT('Ctrl Pts',(0.293132859331976,1.96608038343414,5.42804447934433));
#52612=CARTESIAN_POINT('Ctrl Pts',(0.292965740870769,1.96571518476953,5.42801963867957));
#52613=CARTESIAN_POINT('Ctrl Pts',(0.292211652667885,1.96407540787467,5.42790819275321));
#52614=CARTESIAN_POINT('Ctrl Pts',(0.291617033324823,1.96280433409578,5.42782205288824));
#52615=CARTESIAN_POINT('Ctrl Pts',(0.28814752068478,1.95551228993735,5.42732907534745));
#52616=CARTESIAN_POINT('Ctrl Pts',(0.285094280581425,1.94957740358488,5.42693256799952));
#52617=CARTESIAN_POINT('Ctrl Pts',(0.278329834024467,1.93737573789517,5.42611854041927));
#52618=CARTESIAN_POINT('Ctrl Pts',(0.274586127028144,1.93113136192336,5.42570260439875));
#52619=CARTESIAN_POINT('Ctrl Pts',(0.259828133912047,1.90830596581136,5.424165114902));
#52620=CARTESIAN_POINT('Ctrl Pts',(0.247497502241578,1.89263012271813,5.42307156284944));
#52621=CARTESIAN_POINT('Ctrl Pts',(0.230500844902445,1.874714609338,5.42166477066251));
#52622=CARTESIAN_POINT('Ctrl Pts',(0.227125089732386,1.87131170155389,5.42138976452423));
#52623=CARTESIAN_POINT('Ctrl Pts',(0.221613274881717,1.86599800912481,5.420946238249));
#52624=CARTESIAN_POINT('Ctrl Pts',(0.219525398845091,1.86403819387262,5.42077943457096));
#52625=CARTESIAN_POINT('Ctrl Pts',(0.216101694065897,1.86090925778488,5.42050758014579));
#52626=CARTESIAN_POINT('Ctrl Pts',(0.214781814587858,1.85972287427596,5.42040316875304));
#52627=CARTESIAN_POINT('Ctrl Pts',(0.208613695126754,1.85427004763613,5.41991687675334));
#52628=CARTESIAN_POINT('Ctrl Pts',(0.203647973641547,1.85013928436124,5.41953000971795));
#52629=CARTESIAN_POINT('Ctrl Pts',(0.197749845275552,1.84552556728034,5.41907424830028));
#52630=CARTESIAN_POINT('Ctrl Pts',(0.196934886912207,1.84489435817163,5.41901135617647));
#52631=CARTESIAN_POINT('Ctrl Pts',(0.195717685494316,1.84396090857565,5.41891753708184));
#52632=CARTESIAN_POINT('Ctrl Pts',(0.195317734763219,1.84365567836387,5.41888672814565));
#52633=CARTESIAN_POINT('Ctrl Pts',(0.194603942961369,1.84311357448462,5.41883177533185));
#52634=CARTESIAN_POINT('Ctrl Pts',(0.194290379361589,1.84287633575352,5.41880764586522));
#52635=CARTESIAN_POINT('Ctrl Pts',(0.193629193260876,1.84237798975837,5.41875678854835));
#52636=CARTESIAN_POINT('Ctrl Pts',(0.193281475228625,1.84211701108004,5.41873005572834));
#52637=CARTESIAN_POINT('Ctrl Pts',(0.192374762481449,1.84143934465985,5.41866038028493));
#52638=CARTESIAN_POINT('Ctrl Pts',(0.191814943975307,1.84102376752825,5.418617394429));
#52639=CARTESIAN_POINT('Ctrl Pts',(0.18934745219006,1.83920443306523,5.41842806699322));
#52640=CARTESIAN_POINT('Ctrl Pts',(0.187425724830139,1.83781994245557,5.4182809805374));
#52641=CARTESIAN_POINT('Ctrl Pts',(0.182377334847451,1.83426674689942,5.41789544473136));
#52642=CARTESIAN_POINT('Ctrl Pts',(0.179227288298967,1.83213206386712,5.41765572453062));
#52643=CARTESIAN_POINT('Ctrl Pts',(0.164918298418156,1.82280073036235,5.41657019185037));
#52644=CARTESIAN_POINT('Ctrl Pts',(0.153360034625548,1.81624287598682,5.41570166793357));
#52645=CARTESIAN_POINT('Ctrl Pts',(0.131207925591312,1.80542384758623,5.41405770742067));
#52646=CARTESIAN_POINT('Ctrl Pts',(0.120727461197904,1.80097577056267,5.41328801707458));
#52647=CARTESIAN_POINT('Ctrl Pts',(0.102037788519311,1.79418658305347,5.41194242963219));
#52648=CARTESIAN_POINT('Ctrl Pts',(0.0939292555898534,1.79159951559482,
5.4113672259582));
#52649=CARTESIAN_POINT('Ctrl Pts',(0.0815339107971464,1.78817901947045,
5.41050804362356));
#52650=CARTESIAN_POINT('Ctrl Pts',(0.0773169957283992,1.78710674767852,
5.41021921162116));
#52651=CARTESIAN_POINT('Ctrl Pts',(0.0657471137855053,1.78441297344845,
5.40943825748318));
#52652=CARTESIAN_POINT('Ctrl Pts',(0.0583564098576204,1.78296308528809,
5.40895193056711));
#52653=CARTESIAN_POINT('Ctrl Pts',(0.0502422525964148,1.78166469841884,
5.40843641833261));
#52654=CARTESIAN_POINT('Ctrl Pts',(0.0495631091928234,1.78155825272675,
5.40839341082757));
#52655=CARTESIAN_POINT('Ctrl Pts',(0.0486079203664809,1.78141167079654,
5.40833312432616));
#52656=CARTESIAN_POINT('Ctrl Pts',(0.0483321616095003,1.78136971960813,
5.40831574351391));
#52657=CARTESIAN_POINT('Ctrl Pts',(0.0478534361076003,1.78129752685762,
5.40828561132349));
#52658=CARTESIAN_POINT('Ctrl Pts',(0.0476504948933998,1.78126712113224,
5.40827285060569));
#52659=CARTESIAN_POINT('Ctrl Pts',(0.0472262335667353,1.78120397031555,
5.40824620071383));
#52660=CARTESIAN_POINT('Ctrl Pts',(0.0470049085337124,1.78117126187632,
5.4082323137085));
#52661=CARTESIAN_POINT('Ctrl Pts',(0.0464758713151132,1.7810936411515,5.40819915598401));
#52662=CARTESIAN_POINT('Ctrl Pts',(0.0461681267694432,1.78104894356492,
5.40817989751453));
#52663=CARTESIAN_POINT('Ctrl Pts',(0.0451264751319401,1.78089919066125,
5.40811481027743));
#52664=CARTESIAN_POINT('Ctrl Pts',(0.0443922633853062,1.78079622142647,
5.4080690990508));
#52665=CARTESIAN_POINT('Ctrl Pts',(0.0381647343763009,1.77994474642084,
5.40768273457114));
#52666=CARTESIAN_POINT('Ctrl Pts',(0.0326529046138534,1.77933551948599,
5.40734970187929));
#52667=CARTESIAN_POINT('Ctrl Pts',(0.0192642221008671,1.77820450425854,
5.4065563883369));
#52668=CARTESIAN_POINT('Ctrl Pts',(0.0113784577495407,1.77782924057204,
5.40610215871798));
#52669=CARTESIAN_POINT('Ctrl Pts',(-0.0137561572696534,1.77755731632922,
5.40467413229642));
#52670=CARTESIAN_POINT('Ctrl Pts',(-0.0309861760079501,1.77875491439723,
5.40372344898987));
#52671=CARTESIAN_POINT('Ctrl Pts',(-0.0673168322274205,1.78423151182528,
5.40165246160266));
#52672=CARTESIAN_POINT('Ctrl Pts',(-0.0862891222075503,1.78888055311415,
5.40052931994267));
#52673=CARTESIAN_POINT('Ctrl Pts',(-0.105946983831741,1.79563494649698,
5.39926681692344));
#52674=CARTESIAN_POINT('Ctrl Pts',(-0.107167880059132,1.79606267984282,
5.39918800208811));
#52675=CARTESIAN_POINT('Ctrl Pts',(-0.108867178257717,1.79666953002278,
5.39907772802283));
#52676=CARTESIAN_POINT('Ctrl Pts',(-0.109347791099799,1.79684245499204,
5.3990464746756));
#52677=CARTESIAN_POINT('Ctrl Pts',(-0.110177064598686,1.79714305699424,
5.39899243630339));
#52678=CARTESIAN_POINT('Ctrl Pts',(-0.110525920453564,1.79727019572497,
5.39896966924437));
#52679=CARTESIAN_POINT('Ctrl Pts',(-0.111247561928675,1.79753460792449,
5.39892250185479));
#52680=CARTESIAN_POINT('Ctrl Pts',(-0.111620314866197,1.79767196831019,
5.39889809865401));
#52681=CARTESIAN_POINT('Ctrl Pts',(-0.112358354758705,1.79794548883466,
5.39884970212577));
#52682=CARTESIAN_POINT('Ctrl Pts',(-0.112723650539264,1.79808162327148,
5.3988257096936));
#52683=CARTESIAN_POINT('Ctrl Pts',(-0.113569732243776,1.79839868131572,
5.39877005007774));
#52684=CARTESIAN_POINT('Ctrl Pts',(-0.114050333417659,1.79858009197061,
5.39873836661556));
#52685=CARTESIAN_POINT('Ctrl Pts',(-0.116681519290509,1.79958046932987,
5.3985645368132));
#52686=CARTESIAN_POINT('Ctrl Pts',(-0.11882367432071,1.80042128691901,5.39842165866004));
#52687=CARTESIAN_POINT('Ctrl Pts',(-0.124354549868803,1.8026608657438,5.39804915134871));
#52688=CARTESIAN_POINT('Ctrl Pts',(-0.127728659690684,1.80409460541302,
5.39781835464009));
#52689=CARTESIAN_POINT('Ctrl Pts',(-0.140983777014739,1.80999597066668,
5.39689724830606));
#52690=CARTESIAN_POINT('Ctrl Pts',(-0.150660181207837,1.81490312124893,
5.39619236826437));
#52691=CARTESIAN_POINT('Ctrl Pts',(-0.167392974965766,1.82447876040177,
5.39491636639438));
#52692=CARTESIAN_POINT('Ctrl Pts',(-0.174548114375526,1.82895516076368,
5.39435082867938));
#52693=CARTESIAN_POINT('Ctrl Pts',(-0.202201408697887,1.84780506988692,
5.39209362140023));
#52694=CARTESIAN_POINT('Ctrl Pts',(-0.221172382961298,1.86426567315857,
5.39037543405836));
#52695=CARTESIAN_POINT('Ctrl Pts',(-0.239011923323253,1.88381368773901,
5.38870266575288));
#52696=CARTESIAN_POINT('Ctrl Pts',(-0.239968987558174,1.88487653245071,
5.38861274888465));
#52697=CARTESIAN_POINT('Ctrl Pts',(-0.241197085918644,1.88625876227192,
5.38849718074833));
#52698=CARTESIAN_POINT('Ctrl Pts',(-0.241474597981206,1.88657233193487,
5.3884710534253));
#52699=CARTESIAN_POINT('Ctrl Pts',(-0.241898533777412,1.88705323571404,
5.38843112256323));
#52700=CARTESIAN_POINT('Ctrl Pts',(-0.242045395451564,1.88722018045661,
5.38841728622338));
#52701=CARTESIAN_POINT('Ctrl Pts',(-0.242334442985935,1.8875494412091,5.38839004776032));
#52702=CARTESIAN_POINT('Ctrl Pts',(-0.242476637769516,1.88771174708801,
5.38837664501733));
#52703=CARTESIAN_POINT('Ctrl Pts',(-0.242793148449044,1.88807375585528,
5.38834680518022));
#52704=CARTESIAN_POINT('Ctrl Pts',(-0.242967380559522,1.88827353052501,
5.38833037440161));
#52705=CARTESIAN_POINT('Ctrl Pts',(-0.24347045005203,1.88885178911672,5.38828291883063));
#52706=CARTESIAN_POINT('Ctrl Pts',(-0.243798652803775,1.88923082790208,
5.38825194129602));
#52707=CARTESIAN_POINT('Ctrl Pts',(-0.245989326017422,1.89177278255795,
5.38804504422895));
#52708=CARTESIAN_POINT('Ctrl Pts',(-0.247823950678534,1.8939596801155,5.38787114475938));
#52709=CARTESIAN_POINT('Ctrl Pts',(-0.259167885967184,1.90785257956498,
5.38678976192762));
#52710=CARTESIAN_POINT('Ctrl Pts',(-0.267875889781211,1.92019108893208,
5.38593158015138));
#52711=CARTESIAN_POINT('Ctrl Pts',(-0.278556747133182,1.93783345257043,
5.38477274522406));
#52712=CARTESIAN_POINT('Ctrl Pts',(-0.281302513158801,1.94264451823446,
5.38446322460756));
#52713=CARTESIAN_POINT('Ctrl Pts',(-0.286700075641271,1.95269522624271,
5.38382556971354));
#52714=CARTESIAN_POINT('Ctrl Pts',(-0.289335382443309,1.95794133189071,
5.38349754836957));
#52715=CARTESIAN_POINT('Ctrl Pts',(-0.300817000593729,1.98244437719901,
5.38197729242602));
#52716=CARTESIAN_POINT('Ctrl Pts',(-0.30789236213191,2.00246906532676,5.38076338816379));
#52717=CARTESIAN_POINT('Ctrl Pts',(-0.31326175076767,2.02430362820246,5.37939773793129));
#52718=CARTESIAN_POINT('Ctrl Pts',(-0.313564505880587,2.025567710153,5.37931854899921));
#52719=CARTESIAN_POINT('Ctrl Pts',(-0.313975801721425,2.02733203236149,
5.37920783503972));
#52720=CARTESIAN_POINT('Ctrl Pts',(-0.314090813183097,2.02783076378029,
5.37917651807404));
#52721=CARTESIAN_POINT('Ctrl Pts',(-0.314287269731863,2.0286920356617,5.37912239936116));
#52722=CARTESIAN_POINT('Ctrl Pts',(-0.314369277024154,2.02905444795468,
5.3790996157061));
#52723=CARTESIAN_POINT('Ctrl Pts',(-0.314537626595867,2.02980445338761,
5.37905244188346));
#52724=CARTESIAN_POINT('Ctrl Pts',(-0.314623879614969,2.03019206576184,
5.37902804889419));
#52725=CARTESIAN_POINT('Ctrl Pts',(-0.314793323414977,2.03096022238409,
5.37897968168066));
#52726=CARTESIAN_POINT('Ctrl Pts',(-0.314876541083524,2.0313407600315,5.37895570836762));
#52727=CARTESIAN_POINT('Ctrl Pts',(-0.315067720504291,2.0322226429798,5.37890012134462));
#52728=CARTESIAN_POINT('Ctrl Pts',(-0.315175175672819,2.0327240959693,5.37886849145033));
#52729=CARTESIAN_POINT('Ctrl Pts',(-0.315450125074151,2.03402229860653,
5.37878654695159));
#52730=CARTESIAN_POINT('Ctrl Pts',(-0.315615797025389,2.03481942667491,
5.37873617413641));
#52731=CARTESIAN_POINT('Ctrl Pts',(-0.320119133983381,2.05690694135706,
5.3773387870345));
#52732=CARTESIAN_POINT('Ctrl Pts',(-0.322294686399018,2.07857588294554,
5.37592050230308));
#52733=CARTESIAN_POINT('Ctrl Pts',(-0.322274865791103,2.1002941161782,5.37446218470553));
#52734=CARTESIAN_POINT('',(-0.322274887569339,2.09973080273101,5.12450080716969));
#52735=CARTESIAN_POINT('Ctrl Pts',(-0.322274865994725,2.10029389297751,
5.37446219969282));
#52736=CARTESIAN_POINT('Ctrl Pts',(-0.322249612424585,2.12798625569297,
5.37260273655975));
#52737=CARTESIAN_POINT('Ctrl Pts',(-0.3186553232017,2.15556189805677,5.37068861547277));
#52738=CARTESIAN_POINT('Ctrl Pts',(-0.31132187915047,2.18331190230028,5.36887336880326));
#52739=CARTESIAN_POINT('Ctrl Pts',(-0.311060576370121,2.18428228397896,
5.36881005137164));
#52740=CARTESIAN_POINT('Ctrl Pts',(-0.310662201973125,2.18573460738666,
5.36871554284536));
#52741=CARTESIAN_POINT('Ctrl Pts',(-0.310528541506869,2.18621746665312,
5.36868416370155));
#52742=CARTESIAN_POINT('Ctrl Pts',(-0.310281228126122,2.18710287051207,
5.36862670520916));
#52743=CARTESIAN_POINT('Ctrl Pts',(-0.310167916801625,2.18750550822975,
5.36860060652096));
#52744=CARTESIAN_POINT('Ctrl Pts',(-0.309986472970255,2.188145465913,5.36855917485648));
#52745=CARTESIAN_POINT('Ctrl Pts',(-0.309918851561226,2.18838292840539,
5.36854381218281));
#52746=CARTESIAN_POINT('Ctrl Pts',(-0.309790784513868,2.18883070042786,
5.368514864467));
#52747=CARTESIAN_POINT('Ctrl Pts',(-0.309730398063365,2.18904102438796,
5.36850127614593));
#52748=CARTESIAN_POINT('Ctrl Pts',(-0.309592600187295,2.18951913334254,
5.36847040690646));
#52749=CARTESIAN_POINT('Ctrl Pts',(-0.309515055665193,2.18978687901418,
5.36845313390995));
#52750=CARTESIAN_POINT('Ctrl Pts',(-0.309278576337156,2.19059944776114,
5.36840075471699));
#52751=CARTESIAN_POINT('Ctrl Pts',(-0.309118548590051,2.19114395561384,
5.36836571217274));
#52752=CARTESIAN_POINT('Ctrl Pts',(-0.307978461256816,2.19498565672157,
5.36811885925182));
#52753=CARTESIAN_POINT('Ctrl Pts',(-0.306947060434243,2.19826755304104,
5.36790998148493));
#52754=CARTESIAN_POINT('Ctrl Pts',(-0.298003267217911,2.22521044057296,
5.36620698149002));
#52755=CARTESIAN_POINT('Ctrl Pts',(-0.287419251519737,2.24789908411726,
5.36484361909228));
#52756=CARTESIAN_POINT('Ctrl Pts',(-0.27018353699954,2.27585276902655,5.36300116544574));
#52757=CARTESIAN_POINT('Ctrl Pts',(-0.265800737583564,2.28240970523873,
5.36255631173721));
#52758=CARTESIAN_POINT('Ctrl Pts',(-0.253638006223584,2.29923545591094,
5.36136871451682));
#52759=CARTESIAN_POINT('Ctrl Pts',(-0.245476064301503,2.30920910116654,
5.36061641797045));
#52760=CARTESIAN_POINT('Ctrl Pts',(-0.235177163180014,2.32035921496239,
5.35970010914322));
#52761=CARTESIAN_POINT('Ctrl Pts',(-0.233596154298098,2.32203449725558,
5.35956030178224));
#52762=CARTESIAN_POINT('Ctrl Pts',(-0.231640788146569,2.32406245733014,
5.35938836825748));
#52763=CARTESIAN_POINT('Ctrl Pts',(-0.231283340830812,2.32443140548356,
5.35935697761181));
#52764=CARTESIAN_POINT('Ctrl Pts',(-0.230653085546425,2.32507883447451,
5.35930169749402));
#52765=CARTESIAN_POINT('Ctrl Pts',(-0.230380650887815,2.32535767857982,
5.35927782435349));
#52766=CARTESIAN_POINT('Ctrl Pts',(-0.22982957748871,2.3259196732258,5.35922957893271));
#52767=CARTESIAN_POINT('Ctrl Pts',(-0.229550919851689,2.32620280420907,
5.35920520584389));
#52768=CARTESIAN_POINT('Ctrl Pts',(-0.22901080095871,2.32674956787981,5.35915800750745));
#52769=CARTESIAN_POINT('Ctrl Pts',(-0.228749406054928,2.32701326550921,
5.35913518520563));
#52770=CARTESIAN_POINT('Ctrl Pts',(-0.228127347089528,2.32763863912682,
5.35908091982183));
#52771=CARTESIAN_POINT('Ctrl Pts',(-0.227766278580647,2.32799990975951,
5.35904945884774));
#52772=CARTESIAN_POINT('Ctrl Pts',(-0.226487702539206,2.32927313341205,
5.35893818128994));
#52773=CARTESIAN_POINT('Ctrl Pts',(-0.225565573772758,2.33018040958424,
5.35885815905579));
#52774=CARTESIAN_POINT('Ctrl Pts',(-0.210661457314349,2.3446689017759,5.3575684080615));
#52775=CARTESIAN_POINT('Ctrl Pts',(-0.19548378910435,2.35695711567857,5.35630210574563));
#52776=CARTESIAN_POINT('Ctrl Pts',(-0.169831299662873,2.37413158589911,
5.354238262045));
#52777=CARTESIAN_POINT('Ctrl Pts',(-0.160042000334104,2.37995953000421,
5.35346699606518));
#52778=CARTESIAN_POINT('Ctrl Pts',(-0.138994731187167,2.3910244937118,5.35185843227491));
#52779=CARTESIAN_POINT('Ctrl Pts',(-0.127699926459639,2.39615461849474,
5.35102261132419));
#52780=CARTESIAN_POINT('Ctrl Pts',(-0.111575249428453,2.40238395362104,
5.34988925278753));
#52781=CARTESIAN_POINT('Ctrl Pts',(-0.106973623711378,2.40404233455917,
5.34957240594026));
#52782=CARTESIAN_POINT('Ctrl Pts',(-0.100043522698501,2.40636304091178,
5.34910679245209));
#52783=CARTESIAN_POINT('Ctrl Pts',(-0.0977426235781468,2.40710486751691,
5.34895407842226));
#52784=CARTESIAN_POINT('Ctrl Pts',(-0.0949763744272689,2.40796248633253,
5.3487729011738));
#52785=CARTESIAN_POINT('Ctrl Pts',(-0.0945189167901363,2.40810319547728,
5.34874301868718));
#52786=CARTESIAN_POINT('Ctrl Pts',(-0.0938122788012034,2.40831882795594,
5.3486969827086));
#52787=CARTESIAN_POINT('Ctrl Pts',(-0.0935633207715556,2.40839446871393,
5.34868078728533));
#52788=CARTESIAN_POINT('Ctrl Pts',(-0.0931264173473537,2.4085266350497,
5.34865240732878));
#52789=CARTESIAN_POINT('Ctrl Pts',(-0.0929385127266302,2.4085832902083,
5.3486402151869));
#52790=CARTESIAN_POINT('Ctrl Pts',(-0.0925399413783279,2.40870306645484,
5.34861438279622));
#52791=CARTESIAN_POINT('Ctrl Pts',(-0.0923292624639065,2.40876614335528,
5.34860074519627));
#52792=CARTESIAN_POINT('Ctrl Pts',(-0.0917288138277761,2.40894524712427,
5.34856192518865));
#52793=CARTESIAN_POINT('Ctrl Pts',(-0.0913388870502348,2.40906075248026,
5.34853677341013));
#52794=CARTESIAN_POINT('Ctrl Pts',(-0.089675797757754,2.40954997580492,
5.34842973918893));
#52795=CARTESIAN_POINT('Ctrl Pts',(-0.0884005291084146,2.40991657396879,
5.34834826720676));
#52796=CARTESIAN_POINT('Ctrl Pts',(-0.0634419699234283,2.41692475275216,
5.34676485715235));
#52797=CARTESIAN_POINT('Ctrl Pts',(-0.0390731478370692,2.42084248359268,
5.34540985040712));
#52798=CARTESIAN_POINT('Ctrl Pts',(0.000772688522043308,2.42263613487547,
5.3431787682995));
#52799=CARTESIAN_POINT('Ctrl Pts',(0.0160665099609959,2.42223669669883,
5.3423194570174));
#52800=CARTESIAN_POINT('Ctrl Pts',(0.0408147933276175,2.41982375321389,
5.34087234814208));
#52801=CARTESIAN_POINT('Ctrl Pts',(0.0503091647327236,2.41846827311348,
5.34030369557085));
#52802=CARTESIAN_POINT('Ctrl Pts',(0.0609655111849718,2.41645847596923,
5.3396448103054));
#52803=CARTESIAN_POINT('Ctrl Pts',(0.0622012537301906,2.41621790672081,
5.33956809042691));
#52804=CARTESIAN_POINT('Ctrl Pts',(0.0638551262898368,2.41588586802663,
5.33946498103141));
#52805=CARTESIAN_POINT('Ctrl Pts',(0.0642745413199586,2.41580079497644,
5.33943879577942));
#52806=CARTESIAN_POINT('Ctrl Pts',(0.065106305784319,2.41563035641668,5.33938679214317));
#52807=CARTESIAN_POINT('Ctrl Pts',(0.0655186598730812,2.41554501762882,
5.33936097465887));
#52808=CARTESIAN_POINT('Ctrl Pts',(0.0663201302861099,2.41537751046522,
5.33931072361489));
#52809=CARTESIAN_POINT('Ctrl Pts',(0.0667092642640448,2.41529542947449,
5.33928629289381));
#52810=CARTESIAN_POINT('Ctrl Pts',(0.0676114193297003,2.4151033907833,5.33922957749078));
#52811=CARTESIAN_POINT('Ctrl Pts',(0.0681243247611521,2.41499290036056,
5.33919727578923));
#52812=CARTESIAN_POINT('Ctrl Pts',(0.0697829381395514,2.41463136023694,
5.33909263361659));
#52813=CARTESIAN_POINT('Ctrl Pts',(0.0709275360287182,2.41437531053588,
5.33902013296391));
#52814=CARTESIAN_POINT('Ctrl Pts',(0.0821855812576749,2.41179224287829,
5.33830414991492));
#52815=CARTESIAN_POINT('Ctrl Pts',(0.0921813998309867,2.4089845015729,5.33764520773177));
#52816=CARTESIAN_POINT('Ctrl Pts',(0.108425904298832,2.40356309824571,5.33653397192166));
#52817=CARTESIAN_POINT('Ctrl Pts',(0.114759211500483,2.40122590454839,5.33609029475168));
#52818=CARTESIAN_POINT('Ctrl Pts',(0.138697953576414,2.39152718591101,5.3343751204751));
#52819=CARTESIAN_POINT('Ctrl Pts',(0.155710020005394,2.38280653710142,5.33307276752409));
#52820=CARTESIAN_POINT('Ctrl Pts',(0.177895806852452,2.36882213886011,5.33131010566852));
#52821=CARTESIAN_POINT('Ctrl Pts',(0.183814092717787,2.36481059334195,5.33083337026686));
#52822=CARTESIAN_POINT('Ctrl Pts',(0.193003447917024,2.35812519800486,5.33008784690319));
#52823=CARTESIAN_POINT('Ctrl Pts',(0.196363719129032,2.35557825044378,5.32981405686595));
#52824=CARTESIAN_POINT('Ctrl Pts',(0.202151279633928,2.35100996515424,5.32934174934064));
#52825=CARTESIAN_POINT('Ctrl Pts',(0.204600594071199,2.34901755201746,5.32914162588617));
#52826=CARTESIAN_POINT('Ctrl Pts',(0.207414925368038,2.3466586496251,5.32891178695415));
#52827=CARTESIAN_POINT('Ctrl Pts',(0.207808716636984,2.34632697375386,5.32887962960817));
#52828=CARTESIAN_POINT('Ctrl Pts',(0.208406223419608,2.3458212632155,5.32883084280319));
#52829=CARTESIAN_POINT('Ctrl Pts',(0.208610517190153,2.34564791781694,5.32881416318259));
#52830=CARTESIAN_POINT('Ctrl Pts',(0.208964593694375,2.34534671994476,5.32878525677634));
#52831=CARTESIAN_POINT('Ctrl Pts',(0.209114475085133,2.34521898522771,5.32877302135175));
#52832=CARTESIAN_POINT('Ctrl Pts',(0.209428092491563,2.34495121171352,5.32874742106021));
#52833=CARTESIAN_POINT('Ctrl Pts',(0.20959180464835,2.34481114653845,5.32873405825423));
#52834=CARTESIAN_POINT('Ctrl Pts',(0.210047309458551,2.34442064412672,5.32869688022941));
#52835=CARTESIAN_POINT('Ctrl Pts',(0.210338795768285,2.34416984761533,5.32867309158664));
#52836=CARTESIAN_POINT('Ctrl Pts',(0.211502660477131,2.34316482092742,5.32857811271753));
#52837=CARTESIAN_POINT('Ctrl Pts',(0.212371450319303,2.34240642052001,5.32850722716675));
#52838=CARTESIAN_POINT('Ctrl Pts',(0.227537661166986,2.32902312433443,5.32726964584599));
#52839=CARTESIAN_POINT('Ctrl Pts',(0.240692974549557,2.31515599939262,5.32619265042133));
#52840=CARTESIAN_POINT('Ctrl Pts',(0.262322574185994,2.28787157662924,5.32424252485281));
#52841=CARTESIAN_POINT('Ctrl Pts',(0.27118275332493,2.27483923363588,5.32336922655604));
#52842=CARTESIAN_POINT('Ctrl Pts',(0.283417572359509,2.25366101669827,5.32197298481332));
#52843=CARTESIAN_POINT('Ctrl Pts',(0.287471425119374,2.24593625729544,5.32146829131679));
#52844=CARTESIAN_POINT('Ctrl Pts',(0.293947789745559,2.2322755120116,5.32057544604335));
#52845=CARTESIAN_POINT('Ctrl Pts',(0.296515779054099,2.22641399569016,5.32019228033022));
#52846=CARTESIAN_POINT('Ctrl Pts',(0.299303639607894,2.21949740504755,5.31973861473266));
#52847=CARTESIAN_POINT('Ctrl Pts',(0.299694930942479,2.21851264413984,5.3196739889381));
#52848=CARTESIAN_POINT('Ctrl Pts',(0.300271460621285,2.21704057978066,5.31957732579565));
#52849=CARTESIAN_POINT('Ctrl Pts',(0.300460387458403,2.21655472080673,5.31954541252896));
#52850=CARTESIAN_POINT('Ctrl Pts',(0.300791250263799,2.21569769789381,5.31948910239449));
#52851=CARTESIAN_POINT('Ctrl Pts',(0.300933680490832,2.21532672490426,5.31946472217123));
#52852=CARTESIAN_POINT('Ctrl Pts',(0.30120779724125,2.21460879645887,5.3194175287764));
#52853=CARTESIAN_POINT('Ctrl Pts',(0.301339571386652,2.21426187491633,5.31939471858546));
#52854=CARTESIAN_POINT('Ctrl Pts',(0.301651024765338,2.21343762607498,5.31934051145211));
#52855=CARTESIAN_POINT('Ctrl Pts',(0.30183017027645,2.21296009940515,5.31930909670753));
#52856=CARTESIAN_POINT('Ctrl Pts',(0.302363244962233,2.21152882418844,5.31921490732196));
#52857=CARTESIAN_POINT('Ctrl Pts',(0.302713790020077,2.21057382973645,5.31915201987342));
#52858=CARTESIAN_POINT('Ctrl Pts',(0.306110819346862,2.20118202771201,5.31853312797519));
#52859=CARTESIAN_POINT('Ctrl Pts',(0.308808064651436,2.19262391592803,5.31796559361946));
#52860=CARTESIAN_POINT('Ctrl Pts',(0.312328872844876,2.17957705695229,5.31709386886126));
#52861=CARTESIAN_POINT('Ctrl Pts',(0.31342002107324,2.17516462048126,5.31679798738802));
#52862=CARTESIAN_POINT('Ctrl Pts',(0.32011092718653,2.14542171626322,5.31479710262097));
#52863=CARTESIAN_POINT('Ctrl Pts',(0.322727303865083,2.11951854011185,5.31301276868194));
#52864=CARTESIAN_POINT('Ctrl Pts',(0.322010409968627,2.0834992474377,5.31061157037432));
#52865=CARTESIAN_POINT('Ctrl Pts',(0.321335976284749,2.07342532414392,5.30995012578004));
#52866=CARTESIAN_POINT('Ctrl Pts',(0.320080146487538,2.06243927694061,5.3092511849257));
#52867=CARTESIAN_POINT('Ctrl Pts',(0.319966163625463,2.0614803649815,5.3091903674611));
#52868=CARTESIAN_POINT('Ctrl Pts',(0.319761017517982,2.05981828765076,5.30908529815983));
#52869=CARTESIAN_POINT('Ctrl Pts',(0.319671841332871,2.05911489008313,5.30904093982269));
#52870=CARTESIAN_POINT('Ctrl Pts',(0.31954093823942,2.05810897878717,5.30897766335618));
#52871=CARTESIAN_POINT('Ctrl Pts',(0.319501102404894,2.05780622755562,5.30895863956429));
#52872=CARTESIAN_POINT('Ctrl Pts',(0.319431468599835,2.05728276585201,5.30892578339778));
#52873=CARTESIAN_POINT('Ctrl Pts',(0.319401872079469,2.05706202917679,5.30891193956358));
#52874=CARTESIAN_POINT('Ctrl Pts',(0.319344391188762,2.05663667347782,5.30888528446205));
#52875=CARTESIAN_POINT('Ctrl Pts',(0.319316539022994,2.05643205102634,5.3088724713741));
#52876=CARTESIAN_POINT('Ctrl Pts',(0.319249919914511,2.05594611367809,5.30884206552016));
#52877=CARTESIAN_POINT('Ctrl Pts',(0.319210977716427,2.05566482240652,5.30882448273496));
#52878=CARTESIAN_POINT('Ctrl Pts',(0.319093163325193,2.05482201572913,5.30877185418631));
#52879=CARTESIAN_POINT('Ctrl Pts',(0.31901318041588,2.05426065286748,5.308736870888));
#52880=CARTESIAN_POINT('Ctrl Pts',(0.318224209638734,2.04882598589505,5.30839884974354));
#52881=CARTESIAN_POINT('Ctrl Pts',(0.317405042719753,2.04396900297328,5.30810189374493));
#52882=CARTESIAN_POINT('Ctrl Pts',(0.314775937110119,2.03029924143429,5.30727584509019));
#52883=CARTESIAN_POINT('Ctrl Pts',(0.31270785295563,2.02154039527352,5.30675802724983));
#52884=CARTESIAN_POINT('Ctrl Pts',(0.304776102839767,1.99329199207191,5.30509291737144));
#52885=CARTESIAN_POINT('Ctrl Pts',(0.297434050760179,1.97426976662998,5.3039766664098));
#52886=CARTESIAN_POINT('Ctrl Pts',(0.281782076944971,1.94291360431153,5.30198390196496));
#52887=CARTESIAN_POINT('Ctrl Pts',(0.274325263971722,1.93022708835698,5.30112987465177));
#52888=CARTESIAN_POINT('Ctrl Pts',(0.26469148913167,1.91613806921593,5.30009992070704));
#52889=CARTESIAN_POINT('Ctrl Pts',(0.26333206950508,1.91419630058332,5.2999560914321));
#52890=CARTESIAN_POINT('Ctrl Pts',(0.261545026737307,1.91170273172328,5.29976887078169));
#52891=CARTESIAN_POINT('Ctrl Pts',(0.261136834419148,1.91113704452967,5.29972622835768));
#52892=CARTESIAN_POINT('Ctrl Pts',(0.260471215042895,1.91022088931447,5.29965688883998));
#52893=CARTESIAN_POINT('Ctrl Pts',(0.260214908131131,1.90986960710637,5.29963023516774));
#52894=CARTESIAN_POINT('Ctrl Pts',(0.259725502714694,1.90920169430879,5.29957942920904));
#52895=CARTESIAN_POINT('Ctrl Pts',(0.259492534028964,1.90888496920418,5.29955528199885));
#52896=CARTESIAN_POINT('Ctrl Pts',(0.258960229520762,1.90816405936498,5.29950019376614));
#52897=CARTESIAN_POINT('Ctrl Pts',(0.258660526480865,1.90776014817723,5.29946923845431));
#52898=CARTESIAN_POINT('Ctrl Pts',(0.257744174232607,1.90653119832636,5.29937477563744));
#52899=CARTESIAN_POINT('Ctrl Pts',(0.257124518588222,1.9057084189338,5.29931115051362));
#52900=CARTESIAN_POINT('Ctrl Pts',(0.252601311168233,1.89976203588523,5.29884851375601));
#52901=CARTESIAN_POINT('Ctrl Pts',(0.248549117561542,1.89475382785139,5.29844364065612));
#52902=CARTESIAN_POINT('Ctrl Pts',(0.243214854860084,1.88855085709718,5.29792185703795));
#52903=CARTESIAN_POINT('Ctrl Pts',(0.242069229697573,1.88724029162431,5.29781041887751));
#52904=CARTESIAN_POINT('Ctrl Pts',(0.219034718236723,1.86131629323071,5.2955820744102));
#52905=CARTESIAN_POINT('Ctrl Pts',(0.193511546820579,1.84019504360487,5.29330279454498));
#52906=CARTESIAN_POINT('Ctrl Pts',(0.157726692849757,1.81882371590439,5.29053899782507));
#52907=CARTESIAN_POINT('Ctrl Pts',(0.15003021819437,1.81464272094027,5.28996819446978));
#52908=CARTESIAN_POINT('Ctrl Pts',(0.14137323322767,1.81038719406892,5.28935909655454));
#52909=CARTESIAN_POINT('Ctrl Pts',(0.140572526422557,1.80999770123157,5.28930306313519));
#52910=CARTESIAN_POINT('Ctrl Pts',(0.139171354433488,1.80932328708003,5.28920555173677));
#52911=CARTESIAN_POINT('Ctrl Pts',(0.138571607514859,1.80903689763439,5.28916398643176));
#52912=CARTESIAN_POINT('Ctrl Pts',(0.137702223020234,1.80862504940321,5.28910398825334));
#52913=CARTESIAN_POINT('Ctrl Pts',(0.13743329600494,1.80849810770611,5.28908546411602));
#52914=CARTESIAN_POINT('Ctrl Pts',(0.136963882545658,1.80827732432458,5.28905319186774));
#52915=CARTESIAN_POINT('Ctrl Pts',(0.136763474773593,1.80818331679928,5.28903943340415));
#52916=CARTESIAN_POINT('Ctrl Pts',(0.13637397469899,1.80800109899868,5.28901273155151));
#52917=CARTESIAN_POINT('Ctrl Pts',(0.136184894151664,1.80791286613973,5.28899978674329));
#52918=CARTESIAN_POINT('Ctrl Pts',(0.135730940285783,1.80770156898069,5.28896874975771));
#52919=CARTESIAN_POINT('Ctrl Pts',(0.135465984535476,1.80757868073171,5.28895066854508));
#52920=CARTESIAN_POINT('Ctrl Pts',(0.13465669417487,1.80720466242878,5.28889554297786));
#52921=CARTESIAN_POINT('Ctrl Pts',(0.134111821689195,1.80695468902177,5.28885856962816));
#52922=CARTESIAN_POINT('Ctrl Pts',(0.128033224497069,1.80418649028142,5.28844763106513));
#52923=CARTESIAN_POINT('Ctrl Pts',(0.122429560912719,1.8018236202934,5.28808295895694));
#52924=CARTESIAN_POINT('Ctrl Pts',(0.0915041114146103,1.78980243769835,
5.28612915597707));
#52925=CARTESIAN_POINT('Ctrl Pts',(0.0651063897897951,1.78320823665236,
5.28466480923543));
#52926=CARTESIAN_POINT('Ctrl Pts',(0.0226599989319834,1.77814228589429,
5.28224129324522));
#52927=CARTESIAN_POINT('Ctrl Pts',(0.00701535455697281,1.77742202085685,
5.28133545919211));
#52928=CARTESIAN_POINT('Ctrl Pts',(-0.0110865448487909,1.77790628727999,
5.28024326934254));
#52929=CARTESIAN_POINT('Ctrl Pts',(-0.0135536986956862,1.77800067084132,
5.280093498751));
#52930=CARTESIAN_POINT('Ctrl Pts',(-0.0167279902989963,1.77815865211877,
5.27989954829253));
#52931=CARTESIAN_POINT('Ctrl Pts',(-0.0174363849161661,1.77819625338751,
5.27985618480338));
#52932=CARTESIAN_POINT('Ctrl Pts',(-0.0185782646566136,1.7782606453492,
5.27978615459769));
#52933=CARTESIAN_POINT('Ctrl Pts',(-0.0190118325690887,1.77828597408847,
5.279759533794));
#52934=CARTESIAN_POINT('Ctrl Pts',(-0.0198379317653035,1.77833591003223,
5.27970875304202));
#52935=CARTESIAN_POINT('Ctrl Pts',(-0.0202304720858855,1.77836035955044,
5.27968459808741));
#52936=CARTESIAN_POINT('Ctrl Pts',(-0.0211258969829911,1.77841777710515,
5.27962944000043));
#52937=CARTESIAN_POINT('Ctrl Pts',(-0.0216287500443039,1.77845120623419,
5.27959842244529));
#52938=CARTESIAN_POINT('Ctrl Pts',(-0.0231641490497526,1.77855689586124,
5.27950358520647));
#52939=CARTESIAN_POINT('Ctrl Pts',(-0.0241964195077273,1.77863295090733,
5.27943964653354));
#52940=CARTESIAN_POINT('Ctrl Pts',(-0.031757648939175,1.77922668023667,
5.27896997619658));
#52941=CARTESIAN_POINT('Ctrl Pts',(-0.0382694330121295,1.77993826956598,
5.27855818066542));
#52942=CARTESIAN_POINT('Ctrl Pts',(-0.0465582409532081,1.78110060722995,
5.27802408779569));
#52943=CARTESIAN_POINT('Ctrl Pts',(-0.0483596200392123,1.78136880339758,
5.27790741584851));
#52944=CARTESIAN_POINT('Ctrl Pts',(-0.0528260305989383,1.78207252724776,
5.27761664216174));
#52945=CARTESIAN_POINT('Ctrl Pts',(-0.055488010078569,1.78252630421174,
5.27744201681422));
#52946=CARTESIAN_POINT('Ctrl Pts',(-0.0853118551029541,1.78799680503545,
5.27547079466282));
#52947=CARTESIAN_POINT('Ctrl Pts',(-0.111724677724404,1.79645213079262,
5.27357269031489));
#52948=CARTESIAN_POINT('Ctrl Pts',(-0.142482069614941,1.81086269517012,
5.27130249284765));
#52949=CARTESIAN_POINT('Ctrl Pts',(-0.148153283664967,1.81372716738078,
5.27088187763395));
#52950=CARTESIAN_POINT('Ctrl Pts',(-0.158837942588785,1.81952651390357,
5.27009017637544));
#52951=CARTESIAN_POINT('Ctrl Pts',(-0.16386414149897,1.82243303133076,5.26971808846018));
#52952=CARTESIAN_POINT('Ctrl Pts',(-0.169308452348046,1.8257808052959,5.26931769588774));
#52953=CARTESIAN_POINT('Ctrl Pts',(-0.169806621729595,1.82608901078952,
5.26928108388257));
#52954=CARTESIAN_POINT('Ctrl Pts',(-0.170543686301537,1.82654779864226,
5.26922695512034));
#52955=CARTESIAN_POINT('Ctrl Pts',(-0.1707832248588,1.82669733723763,5.26920937016122));
#52956=CARTESIAN_POINT('Ctrl Pts',(-0.1711911297326,1.82695272885954,5.26917943636585));
#52957=CARTESIAN_POINT('Ctrl Pts',(-0.171359594702472,1.82705842295344,
5.26916707697144));
#52958=CARTESIAN_POINT('Ctrl Pts',(-0.171705179644935,1.82727568731986,
5.26914173007303));
#52959=CARTESIAN_POINT('Ctrl Pts',(-0.171882288340938,1.8273872739598,5.26912874372687));
#52960=CARTESIAN_POINT('Ctrl Pts',(-0.17230836727104,1.82765630360265,5.2690975103848));
#52961=CARTESIAN_POINT('Ctrl Pts',(-0.172557231150622,1.82781391589904,
5.26907927466371));
#52962=CARTESIAN_POINT('Ctrl Pts',(-0.17332050737381,1.82829878714813,5.2690233653839));
#52963=CARTESIAN_POINT('Ctrl Pts',(-0.173834211218235,1.82862716722948,
5.26898576562825));
#52964=CARTESIAN_POINT('Ctrl Pts',(-0.179812731395174,1.8324728189962,5.26854847287769));
#52965=CARTESIAN_POINT('Ctrl Pts',(-0.185171341773247,1.83615345516246,
5.26815940535848));
#52966=CARTESIAN_POINT('Ctrl Pts',(-0.194766520107832,1.84318048240553,
5.26746092743591));
#52967=CARTESIAN_POINT('Ctrl Pts',(-0.199037172804504,1.84647589638866,
5.26714934813183));
#52968=CARTESIAN_POINT('Ctrl Pts',(-0.208905315525695,1.85449369999891,
5.26642258027478));
#52969=CARTESIAN_POINT('Ctrl Pts',(-0.214428571849699,1.85930274472875,
5.26601035317778));
#52970=CARTESIAN_POINT('Ctrl Pts',(-0.229754959315943,1.87359390527383,
5.26483586848309));
#52971=CARTESIAN_POINT('Ctrl Pts',(-0.23912639425859,1.88351530880313,5.26407894679034));
#52972=CARTESIAN_POINT('Ctrl Pts',(-0.254054086170672,1.90147501058507,
5.26275597177458));
#52973=CARTESIAN_POINT('Ctrl Pts',(-0.259925289851452,1.90922664493999,
5.26219835814575));
#52974=CARTESIAN_POINT('Ctrl Pts',(-0.269607873615735,1.92328876929516,
5.26119714312606));
#52975=CARTESIAN_POINT('Ctrl Pts',(-0.273569922982116,1.92948680676459,
5.26075916025585));
#52976=CARTESIAN_POINT('Ctrl Pts',(-0.278110585263648,1.93715618296798,
5.26021866404168));
#52977=CARTESIAN_POINT('Ctrl Pts',(-0.278895117424574,1.93850349934175,
5.26012376867364));
#52978=CARTESIAN_POINT('Ctrl Pts',(-0.279965657936536,1.94037305862732,
5.25999214802981));
#52979=CARTESIAN_POINT('Ctrl Pts',(-0.280260050307567,1.94089049610431,
5.25995572550803));
#52980=CARTESIAN_POINT('Ctrl Pts',(-0.28075445283489,1.94176510999046,5.25989417032823));
#52981=CARTESIAN_POINT('Ctrl Pts',(-0.280955220029378,1.94212185857839,
5.2598690649564));
#52982=CARTESIAN_POINT('Ctrl Pts',(-0.281351054551799,1.94282837369371,
5.25981935012885));
#52983=CARTESIAN_POINT('Ctrl Pts',(-0.281546150732992,1.94317812327897,
5.25979474176635));
#52984=CARTESIAN_POINT('Ctrl Pts',(-0.281974613811734,1.94394960714206,
5.25974046462356));
#52985=CARTESIAN_POINT('Ctrl Pts',(-0.282207687216855,1.9443715025547,5.2597107854053));
#52986=CARTESIAN_POINT('Ctrl Pts',(-0.283018088563132,1.94584624890688,
5.25960704989086));
#52987=CARTESIAN_POINT('Ctrl Pts',(-0.28359047269195,1.94690179241485,5.25953281749829));
#52988=CARTESIAN_POINT('Ctrl Pts',(-0.289547709250379,1.95803567596174,
5.25874993066847));
#52989=CARTESIAN_POINT('Ctrl Pts',(-0.294398205576087,1.96838925223525,
5.25802246766615));
#52990=CARTESIAN_POINT('Ctrl Pts',(-0.299235365124926,1.98032755660327,
5.25718312586535));
#52991=CARTESIAN_POINT('Ctrl Pts',(-0.299773208131224,1.9816812735016,5.2570879503773));
#52992=CARTESIAN_POINT('Ctrl Pts',(-0.309387489097007,2.0063662185636,5.2553525046248));
#52993=CARTESIAN_POINT('Ctrl Pts',(-0.315723424834338,2.0306719952212,5.2536352899542));
#52994=CARTESIAN_POINT('Ctrl Pts',(-0.320758028711347,2.06675206657146,
5.25119692420123));
#52995=CARTESIAN_POINT('Ctrl Pts',(-0.321733513965345,2.07811979239006,
5.25044578398571));
#52996=CARTESIAN_POINT('Ctrl Pts',(-0.322138027217224,2.09054838527785,
5.24965905090197));
#52997=CARTESIAN_POINT('Ctrl Pts',(-0.322166654395369,2.09158047134321,
5.24959398025463));
#52998=CARTESIAN_POINT('Ctrl Pts',(-0.322207461487357,2.09336023363765,
5.24948224026227));
#52999=CARTESIAN_POINT('Ctrl Pts',(-0.322221999895217,2.09410784033823,
5.24943544570146));
#53000=CARTESIAN_POINT('Ctrl Pts',(-0.32223891769658,2.09516751365462,5.24936932714181));
#53001=CARTESIAN_POINT('Ctrl Pts',(-0.322243445879631,2.0954795362922,5.24934988410092));
#53002=CARTESIAN_POINT('Ctrl Pts',(-0.322250445061775,2.09601547659921,
5.24931653278148));
#53003=CARTESIAN_POINT('Ctrl Pts',(-0.322253135886101,2.09623939074842,
5.24930261210553));
#53004=CARTESIAN_POINT('Ctrl Pts',(-0.322257842731121,2.09666826821539,
5.2492759748053));
#53005=CARTESIAN_POINT('Ctrl Pts',(-0.322259896590546,2.09687323035054,
5.24926325604357));
#53006=CARTESIAN_POINT('Ctrl Pts',(-0.322264275426226,2.09735619594281,
5.24923331234097));
#53007=CARTESIAN_POINT('Ctrl Pts',(-0.322266436219366,2.09763420125487,
5.24921609667152));
#53008=CARTESIAN_POINT('Ctrl Pts',(-0.322272656705628,2.09859438660008,
5.24915670649722));
#53009=CARTESIAN_POINT('Ctrl Pts',(-0.322274910125506,2.09927658260931,
5.24911463271193));
#53010=CARTESIAN_POINT('Ctrl Pts',(-0.322276774331859,2.11385452741531,
5.2482180605504));
#53011=CARTESIAN_POINT('Ctrl Pts',(-0.321379814763137,2.12773790983263,
5.24741269427191));
#53012=CARTESIAN_POINT('Ctrl Pts',(-0.315022139962535,2.17667233039282,
5.24461296763276));
#53013=CARTESIAN_POINT('Ctrl Pts',(-0.304688950478254,2.21082538500583,
5.24269992718813));
#53014=CARTESIAN_POINT('Ctrl Pts',(-0.288117487796207,2.2444073956663,5.24043568955618));
#53015=CARTESIAN_POINT('Ctrl Pts',(-0.287214981102895,2.24619417583121,
5.2403140875302));
#53016=CARTESIAN_POINT('Ctrl Pts',(-0.285983113701354,2.24857758372335,
5.24015031821767));
#53017=CARTESIAN_POINT('Ctrl Pts',(-0.28566840838782,2.24918176881018,5.24010866763992));
#53018=CARTESIAN_POINT('Ctrl Pts',(-0.285172753450314,2.25012602940811,
5.24004335892914));
#53019=CARTESIAN_POINT('Ctrl Pts',(-0.28499310445422,2.25046678845427,5.24001974684825));
#53020=CARTESIAN_POINT('Ctrl Pts',(-0.284647751100432,2.25111901895891,
5.23997446761668));
#53021=CARTESIAN_POINT('Ctrl Pts',(-0.284482145272294,2.25143054222098,
5.2399528039837));
#53022=CARTESIAN_POINT('Ctrl Pts',(-0.284092931409167,2.25215980565254,
5.23990200314286));
#53023=CARTESIAN_POINT('Ctrl Pts',(-0.283868913422423,2.2525773250567,5.23987285139383));
#53024=CARTESIAN_POINT('Ctrl Pts',(-0.28322197266807,2.25377672131862,5.23978891371425));
#53025=CARTESIAN_POINT('Ctrl Pts',(-0.282796737115337,2.25455733975803,
5.23973404543842));
#53026=CARTESIAN_POINT('Ctrl Pts',(-0.279950793237332,2.25973066297264,
5.23936882408137));
#53027=CARTESIAN_POINT('Ctrl Pts',(-0.277431166943849,2.26406789559316,
5.23905493689193));
#53028=CARTESIAN_POINT('Ctrl Pts',(-0.269694283233309,2.27669786509595,
5.23811719803429));
#53029=CARTESIAN_POINT('Ctrl Pts',(-0.264199350090646,2.28481291543802,
5.23748343956776));
#53030=CARTESIAN_POINT('Ctrl Pts',(-0.248373357684495,2.30603398755055,
5.23574056374043));
#53031=CARTESIAN_POINT('Ctrl Pts',(-0.23738077891124,2.31860835147005,5.23461170913222));
#53032=CARTESIAN_POINT('Ctrl Pts',(-0.212025472155604,2.34343415760863,
5.2322111602948));
#53033=CARTESIAN_POINT('Ctrl Pts',(-0.197457119170619,2.35539353284754,
5.23094415646567));
#53034=CARTESIAN_POINT('Ctrl Pts',(-0.181324923253764,2.36642631196949,
5.22971237406465));
#53035=CARTESIAN_POINT('Ctrl Pts',(-0.180721536970899,2.36683596759337,
5.22966653748616));
#53036=CARTESIAN_POINT('Ctrl Pts',(-0.17961065180931,2.36758468169668,5.22958258743724));
#53037=CARTESIAN_POINT('Ctrl Pts',(-0.179103572209121,2.36792435230583,
5.22954443419822));
#53038=CARTESIAN_POINT('Ctrl Pts',(-0.178359051491941,2.36842001617057,
5.22948866349852));
#53039=CARTESIAN_POINT('Ctrl Pts',(-0.178122368004778,2.36857713668139,
5.22947097054284));
#53040=CARTESIAN_POINT('Ctrl Pts',(-0.177701956653994,2.36885542334633,
5.22943960855945));
#53041=CARTESIAN_POINT('Ctrl Pts',(-0.177518312275474,2.36897671436283,
5.22942593107253));
#53042=CARTESIAN_POINT('Ctrl Pts',(-0.177133014027207,2.36923062459127,
5.22939728119826));
#53043=CARTESIAN_POINT('Ctrl Pts',(-0.176931335883847,2.36936320509573,
5.22938231144218));
#53044=CARTESIAN_POINT('Ctrl Pts',(-0.176400456138511,2.36971134484431,
5.22934297565138));
#53045=CARTESIAN_POINT('Ctrl Pts',(-0.176071007067762,2.3699265287771,5.22931863491561));
#53046=CARTESIAN_POINT('Ctrl Pts',(-0.174601822260692,2.37088231164919,
5.2292103942187));
#53047=CARTESIAN_POINT('Ctrl Pts',(-0.173457780487889,2.37161631328595,
5.22912693029752));
#53048=CARTESIAN_POINT('Ctrl Pts',(-0.164773010845749,2.37711109193931,
5.2284992483708));
#53049=CARTESIAN_POINT('Ctrl Pts',(-0.15704147785986,2.38156475021108,5.22797398682604));
#53050=CARTESIAN_POINT('Ctrl Pts',(-0.134542901634906,2.39330924399824,
5.22650989287571));
#53051=CARTESIAN_POINT('Ctrl Pts',(-0.119388451271401,2.3997975442745,5.2255981322386));
#53052=CARTESIAN_POINT('Ctrl Pts',(-0.0813040140909026,2.41275497846031,
5.22334645200766));
#53053=CARTESIAN_POINT('Ctrl Pts',(-0.0580303231001466,2.41789661871543,
5.22199832453671));
#53054=CARTESIAN_POINT('Ctrl Pts',(-0.0329478271526801,2.42058971188798,
5.22046787271104));
#53055=CARTESIAN_POINT('Ctrl Pts',(-0.0314898860301568,2.42073619946888,
5.22037866963294));
#53056=CARTESIAN_POINT('Ctrl Pts',(-0.0294947155725804,2.42092293080252,
5.22025624673776));
#53057=CARTESIAN_POINT('Ctrl Pts',(-0.0289582935937396,2.42097177911488,
5.22022329755897));
#53058=CARTESIAN_POINT('Ctrl Pts',(-0.0280444559599168,2.42105268661818,
5.2201671062988));
#53059=CARTESIAN_POINT('Ctrl Pts',(-0.0276671003772481,2.42108542578194,
5.22014388562807));
#53060=CARTESIAN_POINT('Ctrl Pts',(-0.0269365572402991,2.42114750989516,
5.2200988975896));
#53061=CARTESIAN_POINT('Ctrl Pts',(-0.0265833770888911,2.42117693766646,
5.22007713285717));
#53062=CARTESIAN_POINT('Ctrl Pts',(-0.0257442744628854,2.42124546005649,
5.22002538641883));
#53063=CARTESIAN_POINT('Ctrl Pts',(-0.0252583114557175,2.42128403473062,
5.2199953884227));
#53064=CARTESIAN_POINT('Ctrl Pts',(-0.0238211524478474,2.42139483242993,
5.21990658658014));
#53065=CARTESIAN_POINT('Ctrl Pts',(-0.0228697274119282,2.42146393445204,
5.21984768486017));
#53066=CARTESIAN_POINT('Ctrl Pts',(-0.0153149981860956,2.42197892621476,
5.21937906127795));
#53067=CARTESIAN_POINT('Ctrl Pts',(-0.00870011223477689,2.42222550437639,
5.2189631198275));
#53068=CARTESIAN_POINT('Ctrl Pts',(0.00663077826136184,2.42232458213162,
5.21798507903022));
#53069=CARTESIAN_POINT('Ctrl Pts',(0.0153422657119557,2.42202747812151,
5.21741875745424));
#53070=CARTESIAN_POINT('Ctrl Pts',(0.0506838314702809,2.41938487875055,
5.21508064263407));
#53071=CARTESIAN_POINT('Ctrl Pts',(0.0769825413879906,2.41408443930217,
5.21323589837396));
#53072=CARTESIAN_POINT('Ctrl Pts',(0.11058169555953,2.40283444883238,5.21089423798737));
#53073=CARTESIAN_POINT('Ctrl Pts',(0.118725096218756,2.39973554721936,5.21032907812232));
#53074=CARTESIAN_POINT('Ctrl Pts',(0.127386948997826,2.39603081867868,5.20973790664558));
#53075=CARTESIAN_POINT('Ctrl Pts',(0.128039253576035,2.39574926872082,5.20969344966995));
#53076=CARTESIAN_POINT('Ctrl Pts',(0.128950012247246,2.3953525859196,5.20963147151242));
#53077=CARTESIAN_POINT('Ctrl Pts',(0.12920924777632,2.39523926899812,5.20961384085194));
#53078=CARTESIAN_POINT('Ctrl Pts',(0.129657195091897,2.39504275947453,5.20958339464927));
#53079=CARTESIAN_POINT('Ctrl Pts',(0.129845976284511,2.39495972708272,5.20957056929516));
#53080=CARTESIAN_POINT('Ctrl Pts',(0.130238639513694,2.39478657040735,5.20954390489615));
#53081=CARTESIAN_POINT('Ctrl Pts',(0.130442507511382,2.39469641590852,5.20953006782174));
#53082=CARTESIAN_POINT('Ctrl Pts',(0.130926456770839,2.39448180330434,5.20949723690781));
#53083=CARTESIAN_POINT('Ctrl Pts',(0.131206455293395,2.39435715661615,5.20947825468813));
#53084=CARTESIAN_POINT('Ctrl Pts',(0.132139473440044,2.39394021000074,5.20941504285569));
#53085=CARTESIAN_POINT('Ctrl Pts',(0.132791703429462,2.39364613230832,5.20937092174894));
#53086=CARTESIAN_POINT('Ctrl Pts',(0.14409488731944,2.38850438736617,5.20860737997982));
#53087=CARTESIAN_POINT('Ctrl Pts',(0.154476405955145,2.38308166319921,5.20792267004324));
#53088=CARTESIAN_POINT('Ctrl Pts',(0.196767554430835,2.35796981334613,5.205109754711));
#53089=CARTESIAN_POINT('Ctrl Pts',(0.225407533320787,2.33336145887135,5.20310698965065));
#53090=CARTESIAN_POINT('Ctrl Pts',(0.250519689444358,2.3027449991922,5.20071440985734));
#53091=CARTESIAN_POINT('Ctrl Pts',(0.251844919147699,2.30109645910873,5.20058597431179));
#53092=CARTESIAN_POINT('Ctrl Pts',(0.253584947958278,2.29888774520995,5.20041436526582));
#53093=CARTESIAN_POINT('Ctrl Pts',(0.254014316084633,2.29833907390565,5.20037177352289));
#53094=CARTESIAN_POINT('Ctrl Pts',(0.254680224637519,2.29748242858476,5.2003053319119));
#53095=CARTESIAN_POINT('Ctrl Pts',(0.254917995071817,2.29717540974369,5.2002815308521));
#53096=CARTESIAN_POINT('Ctrl Pts',(0.255392048046833,2.29656100258383,5.20023392244234));
#53097=CARTESIAN_POINT('Ctrl Pts',(0.255628331962342,2.29625361611552,5.20021011520046));
#53098=CARTESIAN_POINT('Ctrl Pts',(0.256152469940571,2.29556920201964,5.20015713128669));
#53099=CARTESIAN_POINT('Ctrl Pts',(0.256440047003135,2.29519196429271,5.20012794377593));
#53100=CARTESIAN_POINT('Ctrl Pts',(0.257270249870077,2.29409791965185,5.20004334203526));
#53101=CARTESIAN_POINT('Ctrl Pts',(0.257810707154714,2.29337947960308,5.199987842899));
#53102=CARTESIAN_POINT('Ctrl Pts',(0.259024672913913,2.29175159748644,5.19986221435802));
#53103=CARTESIAN_POINT('Ctrl Pts',(0.259696408763728,2.29084085395812,5.19979201662996));
#53104=CARTESIAN_POINT('Ctrl Pts',(0.265305360104281,2.28315175075807,5.19920005998425));
#53105=CARTESIAN_POINT('Ctrl Pts',(0.269980670352369,2.27618715750858,5.19866829940312));
#53106=CARTESIAN_POINT('Ctrl Pts',(0.280621370836128,2.25891649681372,5.19735868871463));
#53107=CARTESIAN_POINT('Ctrl Pts',(0.286297344025724,2.24844726078929,5.19657190175394));
#53108=CARTESIAN_POINT('Ctrl Pts',(0.303532352297848,2.21197410479837,5.19386710466406));
#53109=CARTESIAN_POINT('Ctrl Pts',(0.312226477123553,2.18476347292928,5.19189781300503));
#53110=CARTESIAN_POINT('Ctrl Pts',(0.317495769911637,2.15531527051852,5.19000617503632));
#53111=CARTESIAN_POINT('Ctrl Pts',(0.317745154876764,2.15386427214024,5.18991359406522));
#53112=CARTESIAN_POINT('Ctrl Pts',(0.318053455842723,2.15199378948639,5.18979509697316));
#53113=CARTESIAN_POINT('Ctrl Pts',(0.318121495402431,2.15157585759306,5.18976867502074));
#53114=CARTESIAN_POINT('Ctrl Pts',(0.318228087398852,2.15091288192473,5.18972684891775));
#53115=CARTESIAN_POINT('Ctrl Pts',(0.318267180650818,2.15066792749847,5.18971141409486));
#53116=CARTESIAN_POINT('Ctrl Pts',(0.318336775715639,2.15022859310585,5.18968376550876));
#53117=CARTESIAN_POINT('Ctrl Pts',(0.318367382107366,2.15003423177019,5.18967154585157));
#53118=CARTESIAN_POINT('Ctrl Pts',(0.318438987579735,2.14957678597483,5.18964281413764));
#53119=CARTESIAN_POINT('Ctrl Pts',(0.318479838577145,2.14931367903029,5.18962631062424));
#53120=CARTESIAN_POINT('Ctrl Pts',(0.318597521700832,2.14854947773591,5.18957843872311));
#53121=CARTESIAN_POINT('Ctrl Pts',(0.318673498044471,2.14804824944509,5.18954711888645));
#53122=CARTESIAN_POINT('Ctrl Pts',(0.31919570227801,2.14454745511765,5.18932890338729));
#53123=CARTESIAN_POINT('Ctrl Pts',(0.319600774120806,2.14154177296956,5.18914429442933));
#53124=CARTESIAN_POINT('Ctrl Pts',(0.320724483842525,2.13221035566627,5.18857840517347));
#53125=CARTESIAN_POINT('Ctrl Pts',(0.321298207093124,2.12586841299972,5.18820408300118));
#53126=CARTESIAN_POINT('Ctrl Pts',(0.323437308828386,2.09060441953885,5.18615925515112));
#53127=CARTESIAN_POINT('Ctrl Pts',(0.321286329393357,2.06159019594428,5.18460093381483));
#53128=CARTESIAN_POINT('Ctrl Pts',(0.314320926572631,2.02868880014485,5.18266388569069));
#53129=CARTESIAN_POINT('Ctrl Pts',(0.313255941796059,2.02414721942819,5.18239296153203));
#53130=CARTESIAN_POINT('Ctrl Pts',(0.310131184234953,2.01201308664056,5.18165767523588));
#53131=CARTESIAN_POINT('Ctrl Pts',(0.307891485164788,2.0044706013569,5.18118838902889));
#53132=CARTESIAN_POINT('Ctrl Pts',(0.305034123103405,1.9959975034611,5.18064439610691));
#53133=CARTESIAN_POINT('Ctrl Pts',(0.304684862442675,1.99497871597641,5.18057870884673));
#53134=CARTESIAN_POINT('Ctrl Pts',(0.304161260477422,1.99347597534082,5.18048139913861));
#53135=CARTESIAN_POINT('Ctrl Pts',(0.303990854150602,1.99299065090963,5.18044990722909));
#53136=CARTESIAN_POINT('Ctrl Pts',(0.303687206633742,1.99213242860905,5.18039410298152));
#53137=CARTESIAN_POINT('Ctrl Pts',(0.303554438369028,1.9917593635688,5.18036980640283));
#53138=CARTESIAN_POINT('Ctrl Pts',(0.303297615875805,1.99104190794798,5.18032300573338));
#53139=CARTESIAN_POINT('Ctrl Pts',(0.303173661739258,1.99069748198044,5.18030050500655));
#53140=CARTESIAN_POINT('Ctrl Pts',(0.302843669466593,1.98978542680583,5.18024083334214));
#53141=CARTESIAN_POINT('Ctrl Pts',(0.3026366229957,1.9892181662266,5.18020362882756));
#53142=CARTESIAN_POINT('Ctrl Pts',(0.301866260114837,1.98712582299045,5.18006606031803));
#53143=CARTESIAN_POINT('Ctrl Pts',(0.301293007276265,1.98560444745442,5.17996536477824));
#53144=CARTESIAN_POINT('Ctrl Pts',(0.299861883024081,1.9818917254122,5.17971796541122));
#53145=CARTESIAN_POINT('Ctrl Pts',(0.298991484020115,1.97970533915752,5.17957084452875));
#53146=CARTESIAN_POINT('Ctrl Pts',(0.294414519943299,1.96856492793829,5.17881373382568));
#53147=CARTESIAN_POINT('Ctrl Pts',(0.290329716441638,1.95977264181296,5.17819109231995));
#53148=CARTESIAN_POINT('Ctrl Pts',(0.278273027649334,1.93661424644853,5.17648211320755));
#53149=CARTESIAN_POINT('Ctrl Pts',(0.269589359543073,1.92265213197186,5.17537538829992));
#53150=CARTESIAN_POINT('Ctrl Pts',(0.24973663878972,1.89558124762562,5.17310361924909));
#53151=CARTESIAN_POINT('Ctrl Pts',(0.238503461464012,1.88257964314422,5.17194188848285));
#53152=CARTESIAN_POINT('Ctrl Pts',(0.223212478551798,1.86750049358797,5.17055485455683));
#53153=CARTESIAN_POINT('Ctrl Pts',(0.220076270264897,1.86452968156225,5.17027951536881));
#53154=CARTESIAN_POINT('Ctrl Pts',(0.216476857875146,1.86125485489575,5.1699745801794));
#53155=CARTESIAN_POINT('Ctrl Pts',(0.216071676525542,1.8608880912205,5.16994040845716));
#53156=CARTESIAN_POINT('Ctrl Pts',(0.215458420729558,1.8603358135493,5.16988892377945));
#53157=CARTESIAN_POINT('Ctrl Pts',(0.215251037898026,1.86014953822097,5.16987155382379));
#53158=CARTESIAN_POINT('Ctrl Pts',(0.214890604653809,1.85982663397509,5.16984143525201));
#53159=CARTESIAN_POINT('Ctrl Pts',(0.214737665422739,1.8596898820991,5.16982867731664));
#53160=CARTESIAN_POINT('Ctrl Pts',(0.214417645089925,1.85940428272639,5.16980202789545));
#53161=CARTESIAN_POINT('Ctrl Pts',(0.214250539649334,1.85925546328813,5.16978813858713));
#53162=CARTESIAN_POINT('Ctrl Pts',(0.213850683036311,1.85890010821325,5.16975496603623));
#53163=CARTESIAN_POINT('Ctrl Pts',(0.213617786657616,1.8586937346853,5.16973569507197));
#53164=CARTESIAN_POINT('Ctrl Pts',(0.212828107042354,1.85799602504557,5.16967052210728));
#53165=CARTESIAN_POINT('Ctrl Pts',(0.212269919344827,1.8575062714047,5.16962473806997));
#53166=CARTESIAN_POINT('Ctrl Pts',(0.210938372532199,1.85634609352077,5.16951617972235));
#53167=CARTESIAN_POINT('Ctrl Pts',(0.21016349735812,1.85567741080384,5.16945353020245));
#53168=CARTESIAN_POINT('Ctrl Pts',(0.200860187725624,1.84772607887438,5.16870740876328));
#53169=CARTESIAN_POINT('Ctrl Pts',(0.191959386419483,1.84088882988374,5.16805408888592));
#53170=CARTESIAN_POINT('Ctrl Pts',(0.163751671426793,1.82147393900853,5.16610015139519));
#53171=CARTESIAN_POINT('Ctrl Pts',(0.143439508798616,1.81048910865807,5.16484352497725));
#53172=CARTESIAN_POINT('Ctrl Pts',(0.108262271223417,1.79608389172537,5.16267438403878));
#53173=CARTESIAN_POINT('Ctrl Pts',(0.0940177835226997,1.79138003211136,
5.16179884426182));
#53174=CARTESIAN_POINT('Ctrl Pts',(0.0782914478583242,1.78737694015411,
5.1608128646853));
#53175=CARTESIAN_POINT('Ctrl Pts',(0.0770821108106107,1.787076564508,5.16073693143421));
#53176=CARTESIAN_POINT('Ctrl Pts',(0.0753825691881916,1.78666488143178,
5.16063005100006));
#53177=CARTESIAN_POINT('Ctrl Pts',(0.0748937891579322,1.78654769325044,
5.16059929329663));
#53178=CARTESIAN_POINT('Ctrl Pts',(0.0740455195771288,1.78634641248727,
5.160545879437));
#53179=CARTESIAN_POINT('Ctrl Pts',(0.0736861549897506,1.78626179306619,
5.16052324027157));
#53180=CARTESIAN_POINT('Ctrl Pts',(0.0729384689520039,1.78608709124875,
5.16047611516627));
#53181=CARTESIAN_POINT('Ctrl Pts',(0.0725501243478201,1.78599711149637,
5.1604516259688));
#53182=CARTESIAN_POINT('Ctrl Pts',(0.0717792064542373,1.78581999570137,
5.1604029860534));
#53183=CARTESIAN_POINT('Ctrl Pts',(0.0713966389815536,1.78573283734973,
5.16037883610215));
#53184=CARTESIAN_POINT('Ctrl Pts',(0.0700956251357066,1.78543893239755,
5.16029666547259));
#53185=CARTESIAN_POINT('Ctrl Pts',(0.0691764389663697,1.78523551315915,
5.16023853812906));
#53186=CARTESIAN_POINT('Ctrl Pts',(0.06214162405785,1.78371098588337,5.15979309984281));
#53187=CARTESIAN_POINT('Ctrl Pts',(0.0559899499688998,1.78256427652382,
5.15940024114404));
#53188=CARTESIAN_POINT('Ctrl Pts',(0.0425768557792685,1.78046600683525,
5.15853558189868));
#53189=CARTESIAN_POINT('Ctrl Pts',(0.0353086189814152,1.77958144606202,
5.15806195471429));
#53190=CARTESIAN_POINT('Ctrl Pts',(0.0167504593464377,1.7779619599821,5.15684028680054));
#53191=CARTESIAN_POINT('Ctrl Pts',(0.00544077935704302,1.77757257982312,
5.15608399689353));
#53192=CARTESIAN_POINT('Ctrl Pts',(-0.0308161556875546,1.77823254335554,
5.15363793883813));
#53193=CARTESIAN_POINT('Ctrl Pts',(-0.0556317085551485,1.781583215079,5.15192527646117));
#53194=CARTESIAN_POINT('Ctrl Pts',(-0.0811939182771575,1.78811740388909,
5.15025767293304));
#53195=CARTESIAN_POINT('Ctrl Pts',(-0.0825721580369343,1.78847946292789,
5.1501680885667));
#53196=CARTESIAN_POINT('Ctrl Pts',(-0.0843516828851688,1.78895957809642,
5.15005288656102));
#53197=CARTESIAN_POINT('Ctrl Pts',(-0.0847551751763398,1.78906928304034,
5.1500267965216));
#53198=CARTESIAN_POINT('Ctrl Pts',(-0.0853727848581228,1.7892384956017,
5.14998691032801));
#53199=CARTESIAN_POINT('Ctrl Pts',(-0.0855870541616043,1.78929743938782,
5.14997308148789));
#53200=CARTESIAN_POINT('Ctrl Pts',(-0.0860092666069014,1.78941405658195,
5.14994585008614));
#53201=CARTESIAN_POINT('Ctrl Pts',(-0.0862172115706606,1.78947171687481,
5.14993244692034));
#53202=CARTESIAN_POINT('Ctrl Pts',(-0.0866806469675839,1.7896007225675,
5.14990259522211));
#53203=CARTESIAN_POINT('Ctrl Pts',(-0.0869361066297151,1.78967217437906,
5.14988615303021));
#53204=CARTESIAN_POINT('Ctrl Pts',(-0.087675000769768,1.78987982632045,
5.14983863223153));
#53205=CARTESIAN_POINT('Ctrl Pts',(-0.0881582082064824,1.79001684204315,
5.14980760108401));
#53206=CARTESIAN_POINT('Ctrl Pts',(-0.0914570078763413,1.79096056942568,
5.14959605418239));
#53207=CARTESIAN_POINT('Ctrl Pts',(-0.0942619255837974,1.79180453478371,
5.14941766869033));
#53208=CARTESIAN_POINT('Ctrl Pts',(-0.1030276472398,1.7945729068964,5.14886375076047));
#53209=CARTESIAN_POINT('Ctrl Pts',(-0.108944388198496,1.79663300065862,
5.14849506348126));
#53210=CARTESIAN_POINT('Ctrl Pts',(-0.126172558665861,1.80320065429629,
5.14742673492484));
#53211=CARTESIAN_POINT('Ctrl Pts',(-0.137293301619349,1.80817821944364,
5.14674363169106));
#53212=CARTESIAN_POINT('Ctrl Pts',(-0.158877418228624,1.81934679470042,
5.14538422246422));
#53213=CARTESIAN_POINT('Ctrl Pts',(-0.169325183009241,1.82552371975195,
5.14470891064443));
#53214=CARTESIAN_POINT('Ctrl Pts',(-0.19357989509715,1.84177652286455,5.14305326335965));
#53215=CARTESIAN_POINT('Ctrl Pts',(-0.206980719399404,1.85238862119319,
5.14206231232925));
#53216=CARTESIAN_POINT('Ctrl Pts',(-0.220409938129574,1.86487820780833,
5.14094825134968));
#53217=CARTESIAN_POINT('Ctrl Pts',(-0.221337472170128,1.8657511551132,5.14087064406197));
#53218=CARTESIAN_POINT('Ctrl Pts',(-0.222627211277037,1.8669794904672,5.14076179099068));
#53219=CARTESIAN_POINT('Ctrl Pts',(-0.222993797243992,1.86733027818391,
5.14073074414034));
#53220=CARTESIAN_POINT('Ctrl Pts',(-0.223626575105206,1.86793865521845,
5.14067696626749));
#53221=CARTESIAN_POINT('Ctrl Pts',(-0.223893154864485,1.86819584119763,
5.14065425280302));
#53222=CARTESIAN_POINT('Ctrl Pts',(-0.224445104716863,1.86873018172551,
5.14060710475687));
#53223=CARTESIAN_POINT('Ctrl Pts',(-0.224730406115604,1.86900740609062,
5.14058266714561));
#53224=CARTESIAN_POINT('Ctrl Pts',(-0.225295009539006,1.86955806137732,
5.14053417251841));
#53225=CARTESIAN_POINT('Ctrl Pts',(-0.225574328879594,1.86983147359438,
5.14051011634514));
#53226=CARTESIAN_POINT('Ctrl Pts',(-0.226221638295365,1.87046740356031,
5.14045421566478));
#53227=CARTESIAN_POINT('Ctrl Pts',(-0.226589254792265,1.87083029853602,
5.14042235456631));
#53228=CARTESIAN_POINT('Ctrl Pts',(-0.22862195168902,1.87284656077199,5.1402455448671));
#53229=CARTESIAN_POINT('Ctrl Pts',(-0.230269773698166,1.8745171567504,5.14009983432692));
#53230=CARTESIAN_POINT('Ctrl Pts',(-0.239768937849669,1.88436033395053,
5.13924566302208));
#53231=CARTESIAN_POINT('Ctrl Pts',(-0.247202200108863,1.89292361167454,
5.13851938866038));
#53232=CARTESIAN_POINT('Ctrl Pts',(-0.258682140403213,1.9076497373701,5.13729632073514));
#53233=CARTESIAN_POINT('Ctrl Pts',(-0.262996425928488,1.91359199897851,
5.13680922056989));
#53234=CARTESIAN_POINT('Ctrl Pts',(-0.283414113068759,1.94383559384086,
5.13436664918898));
#53235=CARTESIAN_POINT('Ctrl Pts',(-0.296371318743832,1.97009610528975,
5.13234483393486));
#53236=CARTESIAN_POINT('Ctrl Pts',(-0.306105558473916,1.99918882369695,
5.13040406135502));
#53237=CARTESIAN_POINT('Ctrl Pts',(-0.306579678693467,2.00064001294697,
5.13030803007201));
#53238=CARTESIAN_POINT('Ctrl Pts',(-0.307172383800047,2.00249880874143,
5.13018606628796));
#53239=CARTESIAN_POINT('Ctrl Pts',(-0.307300490132461,2.0029033242819,5.13015958699455));
#53240=CARTESIAN_POINT('Ctrl Pts',(-0.307503018739293,2.00354725536647,
5.13011753683545));
#53241=CARTESIAN_POINT('Ctrl Pts',(-0.307577960626679,2.00378650500642,
5.13010193546454));
#53242=CARTESIAN_POINT('Ctrl Pts',(-0.307717629983874,2.00423422599131,
5.13007278154937));
#53243=CARTESIAN_POINT('Ctrl Pts',(-0.307782424342285,2.00444267406015,
5.13005922515666));
#53244=CARTESIAN_POINT('Ctrl Pts',(-0.307927771702084,2.0049119483978,5.1300287439884));
#53245=CARTESIAN_POINT('Ctrl Pts',(-0.308008204937849,2.00517281067543,
5.13001182636143));
#53246=CARTESIAN_POINT('Ctrl Pts',(-0.30824651265352,2.0059491959169,5.12996155324783));
#53247=CARTESIAN_POINT('Ctrl Pts',(-0.308403426009957,2.00646501645366,
5.12992825410458));
#53248=CARTESIAN_POINT('Ctrl Pts',(-0.309680047697135,2.01069978735975,
5.12965569059996));
#53249=CARTESIAN_POINT('Ctrl Pts',(-0.310733799261558,2.01443850629147,
5.12942020549679));
#53250=CARTESIAN_POINT('Ctrl Pts',(-0.313968565525912,2.02676473925569,
5.12865788095341));
#53251=CARTESIAN_POINT('Ctrl Pts',(-0.315863253984758,2.03542373370896,
5.12814448466333));
#53252=CARTESIAN_POINT('Ctrl Pts',(-0.320627858892563,2.06250148667257,
5.12657688193106));
#53253=CARTESIAN_POINT('Ctrl Pts',(-0.322259323361285,2.08109780017599,
5.12555199586756));
#53254=CARTESIAN_POINT('Ctrl Pts',(-0.322274887569339,2.09973080273101,
5.12450080716969));
#53255=CARTESIAN_POINT('',(-0.322275001354959,2.10019426933339,4.8741705987911));
#53256=CARTESIAN_POINT('Ctrl Pts',(-0.322274887825424,2.09973110948229,
5.12450078986419));
#53257=CARTESIAN_POINT('Ctrl Pts',(-0.322290989735653,2.11902982390781,
5.12341204450041));
#53258=CARTESIAN_POINT('Ctrl Pts',(-0.320573677161122,2.1382886947902,5.12229858258352));
#53259=CARTESIAN_POINT('Ctrl Pts',(-0.31699887790656,2.15808232175565,5.12107578042294));
#53260=CARTESIAN_POINT('Ctrl Pts',(-0.316850439140216,2.1588867038636,5.12102595671167));
#53261=CARTESIAN_POINT('Ctrl Pts',(-0.316603658603497,2.16019604330961,
5.12094463904795));
#53262=CARTESIAN_POINT('Ctrl Pts',(-0.316507166573223,2.16070134903135,
5.12091320393642));
#53263=CARTESIAN_POINT('Ctrl Pts',(-0.316335377410049,2.16158942119691,
5.12085786342632));
#53264=CARTESIAN_POINT('Ctrl Pts',(-0.316260594212975,2.16197228695529,
5.12083397443929));
#53265=CARTESIAN_POINT('Ctrl Pts',(-0.316108226223457,2.16274490309125,
5.12078570474398));
#53266=CARTESIAN_POINT('Ctrl Pts',(-0.316030615326477,2.16313464757288,
5.1207613232407));
#53267=CARTESIAN_POINT('Ctrl Pts',(-0.31587914143663,2.16388803741071,5.12071413071407));
#53268=CARTESIAN_POINT('Ctrl Pts',(-0.315805370834198,2.16425170090682,
5.12069132267755));
#53269=CARTESIAN_POINT('Ctrl Pts',(-0.315628740425976,2.16511477430685,
5.12063712591431));
#53270=CARTESIAN_POINT('Ctrl Pts',(-0.315525323381796,2.16561406797299,
5.12060571940141));
#53271=CARTESIAN_POINT('Ctrl Pts',(-0.31515640359698,2.16737415673281,5.12049481695449));
#53272=CARTESIAN_POINT('Ctrl Pts',(-0.314884527945459,2.16863359022284,
5.12041511718659));
#53273=CARTESIAN_POINT('Ctrl Pts',(-0.310551897787788,2.18813625666248,
5.11917552545883));
#53274=CARTESIAN_POINT('Ctrl Pts',(-0.304920064847378,2.2059906293523,5.11796382874564));
#53275=CARTESIAN_POINT('Ctrl Pts',(-0.2961155258687,2.22726187992745,5.11642780074655));
#53276=CARTESIAN_POINT('Ctrl Pts',(-0.294375885379781,2.23123576994947,
5.11613682321052));
#53277=CARTESIAN_POINT('Ctrl Pts',(-0.284204516917543,2.25324974741796,
5.1145041546049));
#53278=CARTESIAN_POINT('Ctrl Pts',(-0.274194972971028,2.27051348535402,
5.11314156421886));
#53279=CARTESIAN_POINT('Ctrl Pts',(-0.259912167036294,2.29060236542015,
5.11152282370122));
#53280=CARTESIAN_POINT('Ctrl Pts',(-0.25708355519201,2.29440073802936,5.11121531763284));
#53281=CARTESIAN_POINT('Ctrl Pts',(-0.252400458770424,2.30040830318866,
5.11072835750816));
#53282=CARTESIAN_POINT('Ctrl Pts',(-0.250598328203254,2.30265724484829,
5.11054592357357));
#53283=CARTESIAN_POINT('Ctrl Pts',(-0.248448301231652,2.30526779408155,
5.11033429227091));
#53284=CARTESIAN_POINT('Ctrl Pts',(-0.248129502894311,2.30565304635097,
5.11030306429527));
#53285=CARTESIAN_POINT('Ctrl Pts',(-0.247640518010151,2.30624116849087,
5.11025539952218));
#53286=CARTESIAN_POINT('Ctrl Pts',(-0.247470977779101,2.30644457100898,
5.11023891600546));
#53287=CARTESIAN_POINT('Ctrl Pts',(-0.247162829367344,2.30681334087063,
5.11020903418381));
#53288=CARTESIAN_POINT('Ctrl Pts',(-0.247024306381369,2.30697877727075,
5.11019562977755));
#53289=CARTESIAN_POINT('Ctrl Pts',(-0.246742582205981,2.30731455151985,
5.1101684260331));
#53290=CARTESIAN_POINT('Ctrl Pts',(-0.24659937135742,2.30748487943079,5.11015462753255));
#53291=CARTESIAN_POINT('Ctrl Pts',(-0.246185586894886,2.30797598066852,
5.11011484551426));
#53292=CARTESIAN_POINT('Ctrl Pts',(-0.245914561730789,2.30829637554048,
5.11008889511359));
#53293=CARTESIAN_POINT('Ctrl Pts',(-0.244711850989432,2.30971255178271,
5.10997420230622));
#53294=CARTESIAN_POINT('Ctrl Pts',(-0.243773443036006,2.31080264002487,
5.10988594642229));
#53295=CARTESIAN_POINT('Ctrl Pts',(-0.226104844866034,2.33105134517014,
5.10824628988625));
#53296=CARTESIAN_POINT('Ctrl Pts',(-0.207168815676109,2.34817265410367,
5.10685067631635));
#53297=CARTESIAN_POINT('Ctrl Pts',(-0.181621330405773,2.36628814159831,
5.10509742295786));
#53298=CARTESIAN_POINT('Ctrl Pts',(-0.176737616443746,2.36955425195539,
5.10476767319525));
#53299=CARTESIAN_POINT('Ctrl Pts',(-0.16087948564072,2.37954347251795,5.10370741742335));
#53300=CARTESIAN_POINT('Ctrl Pts',(-0.149591541705932,2.38574303696075,
5.1029676859577));
#53301=CARTESIAN_POINT('Ctrl Pts',(-0.134580793271711,2.39285354717694,
5.10198241911863));
#53302=CARTESIAN_POINT('Ctrl Pts',(-0.131170035778878,2.39439702783201,
5.10175849753345));
#53303=CARTESIAN_POINT('Ctrl Pts',(-0.125586000347327,2.39680768554956,
5.10139140383402));
#53304=CARTESIAN_POINT('Ctrl Pts',(-0.123428751275179,2.39771125037125,
5.10124947023267));
#53305=CARTESIAN_POINT('Ctrl Pts',(-0.120783640941969,2.39878546511438,
5.10107523573262));
#53306=CARTESIAN_POINT('Ctrl Pts',(-0.120304916509685,2.39897854294505,
5.101043693943));
#53307=CARTESIAN_POINT('Ctrl Pts',(-0.119463012927586,2.39931574772912,
5.10098820840468));
#53308=CARTESIAN_POINT('Ctrl Pts',(-0.119100030774898,2.39946036626518,
5.10096428125955));
#53309=CARTESIAN_POINT('Ctrl Pts',(-0.118367030246989,2.39975086316793,
5.10091595295899));
#53310=CARTESIAN_POINT('Ctrl Pts',(-0.117997003079354,2.39989671735684,
5.10089155104111));
#53311=CARTESIAN_POINT('Ctrl Pts',(-0.117281740319008,2.40017712488663,
5.10084437163062));
#53312=CARTESIAN_POINT('Ctrl Pts',(-0.116936540622828,2.40031176863861,
5.10082159722263));
#53313=CARTESIAN_POINT('Ctrl Pts',(-0.116117694219233,2.40062953046593,
5.10076756264189));
#53314=CARTESIAN_POINT('Ctrl Pts',(-0.115643846450979,2.40081212454332,
5.10073628493291));
#53315=CARTESIAN_POINT('Ctrl Pts',(-0.113977614955863,2.4014496768659,5.10062626705278));
#53316=CARTESIAN_POINT('Ctrl Pts',(-0.112782974021728,2.40189866692113,
5.10054732729816));
#53317=CARTESIAN_POINT('Ctrl Pts',(-0.0953332341643595,2.40833889359271,
5.09939332566543));
#53318=CARTESIAN_POINT('Ctrl Pts',(-0.0786263957461685,2.41301599125315,
5.09827403538385));
#53319=CARTESIAN_POINT('Ctrl Pts',(-0.0429353249489763,2.4199693352295,
5.09585681100981));
#53320=CARTESIAN_POINT('Ctrl Pts',(-0.0239580382526524,2.42194682999478,
5.09455651042902));
#53321=CARTESIAN_POINT('Ctrl Pts',(0.00347129750252263,2.42236553399417,
5.0927140680452));
#53322=CARTESIAN_POINT('Ctrl Pts',(0.0118638808303338,2.42216588041121,
5.09215580736258));
#53323=CARTESIAN_POINT('Ctrl Pts',(0.0259063952551296,2.42128223414555,
5.09124015626121));
#53324=CARTESIAN_POINT('Ctrl Pts',(0.0315632208922404,2.4207759160237,5.09087636766627));
#53325=CARTESIAN_POINT('Ctrl Pts',(0.0377836730736761,2.42005298012418,
5.09048406385771));
#53326=CARTESIAN_POINT('Ctrl Pts',(0.0383630423190885,2.41998405121819,
5.09044759924346));
#53327=CARTESIAN_POINT('Ctrl Pts',(0.0392220794861484,2.41987948290555,
5.09039364626036));
#53328=CARTESIAN_POINT('Ctrl Pts',(0.0395018888889973,2.41984504979568,
5.09037609032723));
#53329=CARTESIAN_POINT('Ctrl Pts',(0.039978935907294,2.41978570923523,5.09034619011822));
#53330=CARTESIAN_POINT('Ctrl Pts',(0.0401761957510601,2.41976098643082,
5.09033383534596));
#53331=CARTESIAN_POINT('Ctrl Pts',(0.0405812749875582,2.41970983662066,
5.09030848308549));
#53332=CARTESIAN_POINT('Ctrl Pts',(0.0407890909996474,2.41968338957112,
5.09029548678114));
#53333=CARTESIAN_POINT('Ctrl Pts',(0.0412896568049494,2.4196191905895,5.09026420652612));
#53334=CARTESIAN_POINT('Ctrl Pts',(0.0415823814510605,2.41958123897786,
5.09024593392468));
#53335=CARTESIAN_POINT('Ctrl Pts',(0.042652740496143,2.41944097190929,5.09017919016142));
#53336=CARTESIAN_POINT('Ctrl Pts',(0.0434300610083019,2.4193362187996,5.09013085577881));
#53337=CARTESIAN_POINT('Ctrl Pts',(0.0580704337395859,2.41730880987055,
5.0892229496975));
#53338=CARTESIAN_POINT('Ctrl Pts',(0.0717961418628959,2.41448764813134,
5.08841284188422));
#53339=CARTESIAN_POINT('Ctrl Pts',(0.0955639431645579,2.40796439391599,
5.08701557993845));
#53340=CARTESIAN_POINT('Ctrl Pts',(0.105685601139688,2.40463929526679,5.08642237373804));
#53341=CARTESIAN_POINT('Ctrl Pts',(0.130589283256337,2.3950671973472,5.08493056501713));
#53342=CARTESIAN_POINT('Ctrl Pts',(0.145103345660951,2.38820682651836,5.08403042934113));
#53343=CARTESIAN_POINT('Ctrl Pts',(0.164794450155189,2.37703366540393,5.08271226016531));
#53344=CARTESIAN_POINT('Ctrl Pts',(0.170441066592464,2.37359586367385,5.08232232142532));
#53345=CARTESIAN_POINT('Ctrl Pts',(0.178990390496495,2.36802340895069,5.08171059857379));
#53346=CARTESIAN_POINT('Ctrl Pts',(0.181969868958167,2.36600953522321,5.08149324894688));
#53347=CARTESIAN_POINT('Ctrl Pts',(0.185573031637483,2.36348523907211,5.08122501707319));
#53348=CARTESIAN_POINT('Ctrl Pts',(0.186229396230823,2.36302173530172,5.08117593287879));
#53349=CARTESIAN_POINT('Ctrl Pts',(0.187192887261557,2.36233593409902,5.08110355070279));
#53350=CARTESIAN_POINT('Ctrl Pts',(0.187501369377192,2.3621155391057,5.08108032589258));
#53351=CARTESIAN_POINT('Ctrl Pts',(0.188098286130516,2.36168747906486,5.08103528801968));
#53352=CARTESIAN_POINT('Ctrl Pts',(0.188386767670128,2.36147988012407,5.0810134775277));
#53353=CARTESIAN_POINT('Ctrl Pts',(0.188979644095424,2.3610517401541,5.08096856183576));
#53354=CARTESIAN_POINT('Ctrl Pts',(0.189283997651864,2.36083114298524,5.08094545448292));
#53355=CARTESIAN_POINT('Ctrl Pts',(0.190014969379065,2.36029937738361,5.0808898366956));
#53356=CARTESIAN_POINT('Ctrl Pts',(0.190441209035269,2.35998769269007,5.08085730625504));
#53357=CARTESIAN_POINT('Ctrl Pts',(0.191744645700283,2.35902963872904,5.08075752350956));
#53358=CARTESIAN_POINT('Ctrl Pts',(0.192619325452803,2.35837987210721,5.0806901389415));
#53359=CARTESIAN_POINT('Ctrl Pts',(0.20295330518261,2.35062151156219,5.07988892164561));
#53360=CARTESIAN_POINT('Ctrl Pts',(0.212016359303991,2.34300245051973,5.0791348521145));
#53361=CARTESIAN_POINT('Ctrl Pts',(0.222891291432097,2.33278787375085,5.07816112957286));
#53362=CARTESIAN_POINT('Ctrl Pts',(0.225112764582052,2.3306403353714,5.07795833917096));
#53363=CARTESIAN_POINT('Ctrl Pts',(0.246123641354727,2.30973598119556,5.07600306976637));
#53364=CARTESIAN_POINT('Ctrl Pts',(0.262556194573822,2.28875929145849,5.07417133286359));
#53365=CARTESIAN_POINT('Ctrl Pts',(0.280223431444274,2.25936157118612,5.07190287044791));
#53366=CARTESIAN_POINT('Ctrl Pts',(0.283976264665861,2.25257386622189,5.07139816912015));
#53367=CARTESIAN_POINT('Ctrl Pts',(0.288220675237953,2.24419673066484,5.07080365825575));
#53368=CARTESIAN_POINT('Ctrl Pts',(0.288949339107641,2.24273098636042,5.07070066325066));
#53369=CARTESIAN_POINT('Ctrl Pts',(0.289850976365465,2.24088209126622,5.07057208967466));
#53370=CARTESIAN_POINT('Ctrl Pts',(0.290034393342297,2.24050410251269,5.07054587427993));
#53371=CARTESIAN_POINT('Ctrl Pts',(0.290324606086949,2.23990303746364,5.07050430019729));
#53372=CARTESIAN_POINT('Ctrl Pts',(0.290431884340066,2.23968019670218,5.07048891146154));
#53373=CARTESIAN_POINT('Ctrl Pts',(0.290633566586655,2.2392600210066,5.07045994194081));
#53374=CARTESIAN_POINT('Ctrl Pts',(0.290728025414564,2.23906271504799,5.07044635781396));
#53375=CARTESIAN_POINT('Ctrl Pts',(0.290942104253013,2.23861437488134,5.07041553426673));
#53376=CARTESIAN_POINT('Ctrl Pts',(0.291061600065896,2.23836328241044,5.07039830267819));
#53377=CARTESIAN_POINT('Ctrl Pts',(0.29142255528913,2.23760228268504,5.07034617118902));
#53378=CARTESIAN_POINT('Ctrl Pts',(0.291663002460461,2.23709189231505,5.07031133405769));
#53379=CARTESIAN_POINT('Ctrl Pts',(0.293331380298038,2.23352621714782,5.07006882028422));
#53380=CARTESIAN_POINT('Ctrl Pts',(0.294712682314785,2.23044917169992,5.06986396089299));
#53381=CARTESIAN_POINT('Ctrl Pts',(0.301917961958978,2.21369945770151,5.06876957093372));
#53382=CARTESIAN_POINT('Ctrl Pts',(0.306839867066766,2.19965651831783,5.06792559619228));
#53383=CARTESIAN_POINT('Ctrl Pts',(0.315357967151924,2.16863054863798,5.06611908227535));
#53384=CARTESIAN_POINT('Ctrl Pts',(0.318588355039654,2.1515969625496,5.06516194281945));
#53385=CARTESIAN_POINT('Ctrl Pts',(0.321174776211667,2.12749505029734,5.06377860383119));
#53386=CARTESIAN_POINT('Ctrl Pts',(0.321691767704263,2.12058186235698,5.06337877322469));
#53387=CARTESIAN_POINT('Ctrl Pts',(0.322307005562279,2.10607735327945,5.06252841579754));
#53388=CARTESIAN_POINT('Ctrl Pts',(0.322360732275647,2.09848857118847,5.06207693490839));
#53389=CARTESIAN_POINT('Ctrl Pts',(0.32210207847004,2.08932661322413,5.06152120832134));
#53390=CARTESIAN_POINT('Ctrl Pts',(0.322045903016981,2.08774821026855,5.06142508999017));
#53391=CARTESIAN_POINT('Ctrl Pts',(0.321952508226176,2.08557382528188,5.06129213622317));
#53392=CARTESIAN_POINT('Ctrl Pts',(0.321925230711765,2.08497742053659,5.06125561252182));
#53393=CARTESIAN_POINT('Ctrl Pts',(0.321878554959674,2.08401546098945,5.06119661039005));
#53394=CARTESIAN_POINT('Ctrl Pts',(0.321860190771092,2.08364985549447,5.06117416441928));
#53395=CARTESIAN_POINT('Ctrl Pts',(0.321820619027484,2.08288794873296,5.06112734294976));
#53396=CARTESIAN_POINT('Ctrl Pts',(0.321799302278504,2.08249165397225,5.0611029640643));
#53397=CARTESIAN_POINT('Ctrl Pts',(0.321748376033813,2.08157641944752,5.06104660246538));
#53398=CARTESIAN_POINT('Ctrl Pts',(0.321718243039881,2.08105751095941,5.06101460338021));
#53399=CARTESIAN_POINT('Ctrl Pts',(0.321617631892016,2.07939445399211,5.06091190707832));
#53400=CARTESIAN_POINT('Ctrl Pts',(0.321542305108791,2.07825061745658,5.06084105790569));
#53401=CARTESIAN_POINT('Ctrl Pts',(0.320787889792605,2.06765710290873,5.06018286091458));
#53402=CARTESIAN_POINT('Ctrl Pts',(0.319698585932033,2.0582421626526,5.05958266785852));
#53403=CARTESIAN_POINT('Ctrl Pts',(0.313367349693663,2.01882599424673,5.05700191373256));
#53404=CARTESIAN_POINT('Ctrl Pts',(0.304301913772158,1.98960031671679,5.05490147069499));
#53405=CARTESIAN_POINT('Ctrl Pts',(0.287140701440011,1.95335495075952,5.05223271992611));
#53406=CARTESIAN_POINT('Ctrl Pts',(0.282614343617413,1.94481067941096,5.05160031452623));
#53407=CARTESIAN_POINT('Ctrl Pts',(0.276987258086444,1.93525393670418,5.05089953091354));
#53408=CARTESIAN_POINT('Ctrl Pts',(0.27625603161004,1.93403069051291,5.0508099618198));
#53409=CARTESIAN_POINT('Ctrl Pts',(0.275309056415208,1.93247012419787,5.0506959006802));
#53410=CARTESIAN_POINT('Ctrl Pts',(0.27510077520371,1.93212832485211,5.05067093153232));
#53411=CARTESIAN_POINT('Ctrl Pts',(0.27476509024119,1.93157975242092,5.05063087893878));
#53412=CARTESIAN_POINT('Ctrl Pts',(0.274638089424235,1.93137273515771,5.05061576910076));
#53413=CARTESIAN_POINT('Ctrl Pts',(0.274395771665549,1.9309787457948,5.05058702229763));
#53414=CARTESIAN_POINT('Ctrl Pts',(0.27428049853325,1.93079174959348,5.0505733826751));
#53415=CARTESIAN_POINT('Ctrl Pts',(0.274017247596186,1.93036567948253,5.05054231432302));
#53416=CARTESIAN_POINT('Ctrl Pts',(0.273869148267887,1.93012668159456,5.0505248937666));
#53417=CARTESIAN_POINT('Ctrl Pts',(0.273406626589571,1.92938245612943,5.05047066734592));
#53418=CARTESIAN_POINT('Ctrl Pts',(0.27309111526163,1.92887790172505,5.05043393307344));
#53419=CARTESIAN_POINT('Ctrl Pts',(0.270626167724756,1.92496022628656,5.05014890777184));
#53420=CARTESIAN_POINT('Ctrl Pts',(0.268414104928647,1.92158666819795,5.04990466695142));
#53421=CARTESIAN_POINT('Ctrl Pts',(0.265882829269675,1.91787997546941,5.04963660728115));
#53422=CARTESIAN_POINT('Ctrl Pts',(0.265625697060738,1.91750514719308,5.04960950401381));
#53423=CARTESIAN_POINT('Ctrl Pts',(0.26528888002001,1.91701638026136,5.04957416479857));
#53424=CARTESIAN_POINT('Ctrl Pts',(0.265209914550773,1.91690194927554,5.04956589131828));
#53425=CARTESIAN_POINT('Ctrl Pts',(0.264484257771594,1.91585183484934,5.04948996842644));
#53426=CARTESIAN_POINT('Ctrl Pts',(0.263832683031667,1.91491951813147,5.04942257307185));
#53427=CARTESIAN_POINT('Ctrl Pts',(0.262764931387842,1.91340880477609,5.04931335011777));
#53428=CARTESIAN_POINT('Ctrl Pts',(0.26235175342893,1.91282831199514,5.04927137713442));
#53429=CARTESIAN_POINT('Ctrl Pts',(0.258297495786963,1.90717209849313,5.04886231118013));
#53430=CARTESIAN_POINT('Ctrl Pts',(0.254511303215902,1.90220161647403,5.04850212272989));
#53431=CARTESIAN_POINT('Ctrl Pts',(0.236216575068306,1.87958029254415,5.04684375314817));
#53432=CARTESIAN_POINT('Ctrl Pts',(0.220002117708237,1.86339431269344,5.04559632204089));
#53433=CARTESIAN_POINT('Ctrl Pts',(0.198119025756772,1.84576063487912,5.04399216206107));
#53434=CARTESIAN_POINT('Ctrl Pts',(0.193946331663507,1.84256336681153,5.04368965737329));
#53435=CARTESIAN_POINT('Ctrl Pts',(0.182445540975262,1.83418940689309,5.04286188740506));
#53436=CARTESIAN_POINT('Ctrl Pts',(0.174976916742463,1.8292146549316,5.04233055739251));
#53437=CARTESIAN_POINT('Ctrl Pts',(0.166305791173099,1.82394757245131,5.04171607259803));
#53438=CARTESIAN_POINT('Ctrl Pts',(0.165297242854236,1.82334248540625,5.04164463942759));
#53439=CARTESIAN_POINT('Ctrl Pts',(0.163485821014944,1.82226914867095,5.04151639750932));
#53440=CARTESIAN_POINT('Ctrl Pts',(0.162684187691023,1.82179882369085,5.04145966466839));
#53441=CARTESIAN_POINT('Ctrl Pts',(0.161465443017888,1.82109084492593,5.04137343785837));
#53442=CARTESIAN_POINT('Ctrl Pts',(0.161049811954038,1.82085064188017,5.04134403625283));
#53443=CARTESIAN_POINT('Ctrl Pts',(0.160326126028349,1.8204345608476,5.04129285013193));
#53444=CARTESIAN_POINT('Ctrl Pts',(0.160018313801099,1.82025826070757,5.04127108090512));
#53445=CARTESIAN_POINT('Ctrl Pts',(0.159382076798349,1.81989524826401,5.04122608903721));
#53446=CARTESIAN_POINT('Ctrl Pts',(0.159053613638527,1.81970860459823,5.04120286396458));
#53447=CARTESIAN_POINT('Ctrl Pts',(0.158259178424362,1.81925902626332,5.04114669616668));
#53448=CARTESIAN_POINT('Ctrl Pts',(0.157792879472626,1.81899667426808,5.04111373256036));
#53449=CARTESIAN_POINT('Ctrl Pts',(0.156067027424413,1.81803131508584,5.04099174339158));
#53450=CARTESIAN_POINT('Ctrl Pts',(0.154803426542772,1.81733561359209,5.04090245662954));
#53451=CARTESIAN_POINT('Ctrl Pts',(0.132123422029216,1.80504635994124,5.03930024905909));
#53452=CARTESIAN_POINT('Ctrl Pts',(0.109470280984165,1.79591114036698,5.03769662236508));
#53453=CARTESIAN_POINT('Ctrl Pts',(0.0712673969030711,1.78533169691852,
5.03502197105733));
#53454=CARTESIAN_POINT('Ctrl Pts',(0.056252799806753,1.78230388280608,5.03398014918179));
#53455=CARTESIAN_POINT('Ctrl Pts',(0.0316871621711188,1.77914679892424,
5.03233312175335));
#53456=CARTESIAN_POINT('Ctrl Pts',(0.0222449271769151,1.77835414866932,
5.03171385417739));
#53457=CARTESIAN_POINT('Ctrl Pts',(0.0118497940664607,1.77794158022964,
5.03105658110516));
#53458=CARTESIAN_POINT('Ctrl Pts',(0.0109188324510574,1.77790867364718,
5.03099793357717));
#53459=CARTESIAN_POINT('Ctrl Pts',(0.00929906813292923,1.77785845088637,
5.03089628498103));
#53460=CARTESIAN_POINT('Ctrl Pts',(0.00861033391947493,1.77783930639503,
5.03085318635514));
#53461=CARTESIAN_POINT('Ctrl Pts',(0.00761982568529739,1.77781495229335,
5.03079138576122));
#53462=CARTESIAN_POINT('Ctrl Pts',(0.0073181035060271,1.77780795777662,
5.03077258474916));
#53463=CARTESIAN_POINT('Ctrl Pts',(0.00679432966799497,1.77779655179551,
5.03073998985571));
#53464=CARTESIAN_POINT('Ctrl Pts',(0.00657228282530661,1.77779194601909,
5.03072618500951));
#53465=CARTESIAN_POINT('Ctrl Pts',(0.00614285113018282,1.77778348268963,
5.03069951281746));
#53466=CARTESIAN_POINT('Ctrl Pts',(0.00593546784611308,1.77777959582036,
5.03068664382648));
#53467=CARTESIAN_POINT('Ctrl Pts',(0.00544069010948374,1.77777080030617,
5.03065596837073));
#53468=CARTESIAN_POINT('Ctrl Pts',(0.00515329196500484,1.7777660759206,
5.03063817230475));
#53469=CARTESIAN_POINT('Ctrl Pts',(0.00412911766850792,1.77775061060648,
5.03057483190725));
#53470=CARTESIAN_POINT('Ctrl Pts',(0.00339230423775913,1.77774201193097,
5.03052940691464));
#53471=CARTESIAN_POINT('Ctrl Pts',(-0.00772679117763137,1.77765039046605,
5.02984598613993));
#53472=CARTESIAN_POINT('Ctrl Pts',(-0.0181083723695242,1.7780666037564,
5.02923518388131));
#53473=CARTESIAN_POINT('Ctrl Pts',(-0.0379549990749316,1.77982568252373,
5.02808944697103));
#53474=CARTESIAN_POINT('Ctrl Pts',(-0.0474154973559427,1.78108941310515,
5.02755293200982));
#53475=CARTESIAN_POINT('Ctrl Pts',(-0.0730233954084606,1.78567503326315,
5.02609632587077));
#53476=CARTESIAN_POINT('Ctrl Pts',(-0.0889936083421476,1.78981825803421,
5.02518197589592));
#53477=CARTESIAN_POINT('Ctrl Pts',(-0.113676190606082,1.79828581146635,
5.0236872321499));
#53478=CARTESIAN_POINT('Ctrl Pts',(-0.122630978739701,1.80181323493596,
5.02312726758484));
#53479=CARTESIAN_POINT('Ctrl Pts',(-0.135807048012492,1.80769747134277,
5.02226758582056));
#53480=CARTESIAN_POINT('Ctrl Pts',(-0.14015533842918,1.80975734309257,5.02197783998102));
#53481=CARTESIAN_POINT('Ctrl Pts',(-0.145241276963538,1.81230759595482,
5.02163114716792));
#53482=CARTESIAN_POINT('Ctrl Pts',(-0.146025210563177,1.81270470638167,
5.02157748690999));
#53483=CARTESIAN_POINT('Ctrl Pts',(-0.147227376879879,1.81331986888282,
5.02149485324341));
#53484=CARTESIAN_POINT('Ctrl Pts',(-0.147646775706,1.81353564322915,5.02146596002464));
#53485=CARTESIAN_POINT('Ctrl Pts',(-0.148378877217293,1.81391433320574,
5.02141540998837));
#53486=CARTESIAN_POINT('Ctrl Pts',(-0.148691789796554,1.81407684319918,
5.02139376751383));
#53487=CARTESIAN_POINT('Ctrl Pts',(-0.149396932487417,1.81444452705379,
5.02134491381824));
#53488=CARTESIAN_POINT('Ctrl Pts',(-0.149789007239939,1.81464999584169,
5.02131769219879));
#53489=CARTESIAN_POINT('Ctrl Pts',(-0.150841311059495,1.81520422748594,
5.0212444746596));
#53490=CARTESIAN_POINT('Ctrl Pts',(-0.15150075046947,1.81555447664586,5.02119842611181));
#53491=CARTESIAN_POINT('Ctrl Pts',(-0.154381731918961,1.81709751771464,
5.02099651516158));
#53492=CARTESIAN_POINT('Ctrl Pts',(-0.156590400355959,1.81831404087424,
5.02083980967736));
#53493=CARTESIAN_POINT('Ctrl Pts',(-0.159360322513527,1.81988234423476,
5.02064080561667));
#53494=CARTESIAN_POINT('Ctrl Pts',(-0.15993511903893,1.82021013036475,5.02059937358226));
#53495=CARTESIAN_POINT('Ctrl Pts',(-0.161492626099176,1.82110468936661,
5.02048673536953));
#53496=CARTESIAN_POINT('Ctrl Pts',(-0.162473353175811,1.82167488070132,
5.02041540692031));
#53497=CARTESIAN_POINT('Ctrl Pts',(-0.174844416360484,1.82895504209535,
5.01951051788355));
#53498=CARTESIAN_POINT('Ctrl Pts',(-0.185813026579996,1.83635368112237,
5.01865207491566));
#53499=CARTESIAN_POINT('Ctrl Pts',(-0.202048255611407,1.848822185792,5.01729387039441));
#53500=CARTESIAN_POINT('Ctrl Pts',(-0.20765013893108,1.85343316513334,5.01680758028215));
#53501=CARTESIAN_POINT('Ctrl Pts',(-0.222879251480175,1.86685576212933,
5.01543908957125));
#53502=CARTESIAN_POINT('Ctrl Pts',(-0.232134107363772,1.87606886180473,
5.01455169401613));
#53503=CARTESIAN_POINT('Ctrl Pts',(-0.247318841527261,1.89314104138514,
5.01301926106832));
#53504=CARTESIAN_POINT('Ctrl Pts',(-0.253495756304145,1.90075850562912,
5.01236980037025));
#53505=CARTESIAN_POINT('Ctrl Pts',(-0.261543922447949,1.91166511778105,
5.01149801481006));
#53506=CARTESIAN_POINT('Ctrl Pts',(-0.263718793678523,1.91472276953452,
5.0112595741256));
#53507=CARTESIAN_POINT('Ctrl Pts',(-0.266142202101732,1.91825900329253,
5.01099118635538));
#53508=CARTESIAN_POINT('Ctrl Pts',(-0.266443422265544,1.91870089805796,
5.01095777764401));
#53509=CARTESIAN_POINT('Ctrl Pts',(-0.266896231026274,1.91936874158604,
5.01090748411884));
#53510=CARTESIAN_POINT('Ctrl Pts',(-0.267048633852031,1.91959413310173,
5.01089054433338));
#53511=CARTESIAN_POINT('Ctrl Pts',(-0.267322754595842,1.9200006441147,5.01086005347034));
#53512=CARTESIAN_POINT('Ctrl Pts',(-0.26744457369719,1.92018169379983,5.01084649551848));
#53513=CARTESIAN_POINT('Ctrl Pts',(-0.26770631802739,1.9205715571758,5.01081734765906));
#53514=CARTESIAN_POINT('Ctrl Pts',(-0.267846182451296,1.92078041024095,
5.01080176191374));
#53515=CARTESIAN_POINT('Ctrl Pts',(-0.268223030692836,1.92134456674432,
5.01075973911796));
#53516=CARTESIAN_POINT('Ctrl Pts',(-0.268459553859299,1.92170017955008,
5.01073333323974));
#53517=CARTESIAN_POINT('Ctrl Pts',(-0.26955288541927,1.92335111223036,5.01061112281839));
#53518=CARTESIAN_POINT('Ctrl Pts',(-0.270401048950577,1.92465217269202,
5.01051589088028));
#53519=CARTESIAN_POINT('Ctrl Pts',(-0.288387925022203,1.95268445361817,
5.00848592897194));
#53520=CARTESIAN_POINT('Ctrl Pts',(-0.301495468974115,1.98180211353624,
5.00678883480819));
#53521=CARTESIAN_POINT('Ctrl Pts',(-0.31445233744858,2.0276586973579,5.00408923342287));
#53522=CARTESIAN_POINT('Ctrl Pts',(-0.317635051215339,2.0432425206578,5.00317007649653));
#53523=CARTESIAN_POINT('Ctrl Pts',(-0.319972831598253,2.06146729296592,
5.00206200044817));
#53524=CARTESIAN_POINT('Ctrl Pts',(-0.320261140377203,2.0639419371161,5.00191088117988));
#53525=CARTESIAN_POINT('Ctrl Pts',(-0.320594881149092,2.06712745325744,
5.00171542574204));
#53526=CARTESIAN_POINT('Ctrl Pts',(-0.320666693853842,2.06783552288016,
5.00167192174122));
#53527=CARTESIAN_POINT('Ctrl Pts',(-0.320778601919084,2.0689765693541,5.00160171916253));
#53528=CARTESIAN_POINT('Ctrl Pts',(-0.320820167742375,2.06940940234282,
5.0015750669105));
#53529=CARTESIAN_POINT('Ctrl Pts',(-0.320897650528802,2.07023377578126,
5.00152426204562));
#53530=CARTESIAN_POINT('Ctrl Pts',(-0.320933727207909,2.0706253007265,5.00150011450546));
#53531=CARTESIAN_POINT('Ctrl Pts',(-0.321014323595677,2.0715178532656,5.00144502327685));
#53532=CARTESIAN_POINT('Ctrl Pts',(-0.321058386903391,2.07201892013148,
5.00141406529338));
#53533=CARTESIAN_POINT('Ctrl Pts',(-0.321189123749972,2.07354657295185,
5.001319586422));
#53534=CARTESIAN_POINT('Ctrl Pts',(-0.321272047231104,2.07457346570365,
5.0012559478567));
#53535=CARTESIAN_POINT('Ctrl Pts',(-0.321838053196802,2.08202803440889,
5.00079301173939));
#53536=CARTESIAN_POINT('Ctrl Pts',(-0.322133093955582,2.08846812520689,
5.00038784417965));
#53537=CARTESIAN_POINT('Ctrl Pts',(-0.322262523999165,2.09666583735707,
4.99986492775648));
#53538=CARTESIAN_POINT('Ctrl Pts',(-0.322275895377875,2.0984194669757,4.99975265313351));
#53539=CARTESIAN_POINT('Ctrl Pts',(-0.322271485723973,2.10662967802178,
4.99922505759846));
#53540=CARTESIAN_POINT('Ctrl Pts',(-0.322073989251974,2.11308433849747,
4.99880460416471));
#53541=CARTESIAN_POINT('Ctrl Pts',(-0.32066990953947,2.13621314073731,4.99727868082112));
#53542=CARTESIAN_POINT('Ctrl Pts',(-0.318360545268536,2.15279263742777,
4.99614703720909));
#53543=CARTESIAN_POINT('Ctrl Pts',(-0.31074640657444,2.18746947234569,4.99374543018148));
#53544=CARTESIAN_POINT('Ctrl Pts',(-0.3051187256686,2.20543710589109,4.99248024458738));
#53545=CARTESIAN_POINT('Ctrl Pts',(-0.297555743970668,2.22378553987144,
4.99123033162662));
#53546=CARTESIAN_POINT('Ctrl Pts',(-0.297150388856748,2.2247554693234,4.99116439414858));
#53547=CARTESIAN_POINT('Ctrl Pts',(-0.296595765151285,2.22606452698728,
4.99107560225768));
#53548=CARTESIAN_POINT('Ctrl Pts',(-0.2964506528227,2.22640539274288,4.99105250013645));
#53549=CARTESIAN_POINT('Ctrl Pts',(-0.296221327926977,2.22694150510257,
4.99101619508998));
#53550=CARTESIAN_POINT('Ctrl Pts',(-0.296137509920641,2.22713691853733,
4.99100296812664));
#53551=CARTESIAN_POINT('Ctrl Pts',(-0.295975409014389,2.2275138108057,4.99097746967704));
#53552=CARTESIAN_POINT('Ctrl Pts',(-0.295897153164332,2.22769529919646,
4.99096519670665));
#53553=CARTESIAN_POINT('Ctrl Pts',(-0.295710049611672,2.22812812806948,
4.99093594013195));
#53554=CARTESIAN_POINT('Ctrl Pts',(-0.295601048504267,2.22837940165166,
4.99091896605956));
#53555=CARTESIAN_POINT('Ctrl Pts',(-0.29527475277289,2.22912897240887,4.99086836135098));
#53556=CARTESIAN_POINT('Ctrl Pts',(-0.295056516169467,2.22962686224932,
4.99083478817932));
#53557=CARTESIAN_POINT('Ctrl Pts',(-0.293211738371326,2.23380678250297,
4.99055325076726));
#53558=CARTESIAN_POINT('Ctrl Pts',(-0.291517514121243,2.23745879807833,
4.99030934973404));
#53559=CARTESIAN_POINT('Ctrl Pts',(-0.28592472370122,2.24894561104576,4.98954588004797));
#53560=CARTESIAN_POINT('Ctrl Pts',(-0.281775085198949,2.25665429690691,
4.98903901052657));
#53561=CARTESIAN_POINT('Ctrl Pts',(-0.265187406427254,2.28467168360347,
4.98718285014188));
#53562=CARTESIAN_POINT('Ctrl Pts',(-0.250825608139067,2.30375125909199,
4.98588500129471));
#53563=CARTESIAN_POINT('Ctrl Pts',(-0.230231663522013,2.32559508367137,
4.98416616410154));
#53564=CARTESIAN_POINT('Ctrl Pts',(-0.225840953701362,2.32999047411652,
4.98380685017447));
#53565=CARTESIAN_POINT('Ctrl Pts',(-0.220106859677583,2.33540807054301,
4.98334423219237));
#53566=CARTESIAN_POINT('Ctrl Pts',(-0.218878614581359,2.33655050473622,
4.98324551208478));
#53567=CARTESIAN_POINT('Ctrl Pts',(-0.212895445199329,2.34202916553444,
4.982766268601));
#53568=CARTESIAN_POINT('Ctrl Pts',(-0.208020543743614,2.3462316635459,4.98238074990235));
#53569=CARTESIAN_POINT('Ctrl Pts',(-0.202223643370219,2.35093392368583,
4.9819264460974));
#53570=CARTESIAN_POINT('Ctrl Pts',(-0.201420827684218,2.35157878712385,
4.98186361936357));
#53571=CARTESIAN_POINT('Ctrl Pts',(-0.200221358958731,2.35253284133606,
4.98176987903078));
#53572=CARTESIAN_POINT('Ctrl Pts',(-0.199827045020115,2.35284497347296,
4.98173908317434));
#53573=CARTESIAN_POINT('Ctrl Pts',(-0.199123155569262,2.35339948525176,
4.98168414502061));
#53574=CARTESIAN_POINT('Ctrl Pts',(-0.198813863387272,2.35364222426988,
4.98166001710579));
#53575=CARTESIAN_POINT('Ctrl Pts',(-0.198161536298619,2.35415225805923,
4.98160915415914));
#53576=CARTESIAN_POINT('Ctrl Pts',(-0.197818403251213,2.35441942551036,
4.98158241413985));
#53577=CARTESIAN_POINT('Ctrl Pts',(-0.196912100179739,2.35512214190885,
4.98151182459335));
#53578=CARTESIAN_POINT('Ctrl Pts',(-0.196348028149831,2.35555651883297,
4.98146792882462));
#53579=CARTESIAN_POINT('Ctrl Pts',(-0.193801739109052,2.35750394180115,
4.98126994540544));
#53580=CARTESIAN_POINT('Ctrl Pts',(-0.191803483185973,2.35899578645299,
4.98111502752843));
#53581=CARTESIAN_POINT('Ctrl Pts',(-0.176928058707613,2.3698348146456,4.97996483696135));
#53582=CARTESIAN_POINT('Ctrl Pts',(-0.163393651115211,2.37823864586887,
4.97893335115944));
#53583=CARTESIAN_POINT('Ctrl Pts',(-0.121165639349065,2.40031250055532,
4.97576467543245));
#53584=CARTESIAN_POINT('Ctrl Pts',(-0.0910191242563905,2.41077996187976,
4.97355041953272));
#53585=CARTESIAN_POINT('Ctrl Pts',(-0.0583117413782876,2.41695946677943,
4.97144431421122));
#53586=CARTESIAN_POINT('Ctrl Pts',(-0.056791483864932,2.41723538634693,
4.97134711446894));
#53587=CARTESIAN_POINT('Ctrl Pts',(-0.0548493320747358,2.41757346879647,
4.97122387469924));
#53588=CARTESIAN_POINT('Ctrl Pts',(-0.0544292514864776,2.41764573647393,
4.97119727403627));
#53589=CARTESIAN_POINT('Ctrl Pts',(-0.053761414671408,2.41775926265107,
4.97115507454749));
#53590=CARTESIAN_POINT('Ctrl Pts',(-0.0535137533180082,2.41780106499959,
4.97113944484968));
#53591=CARTESIAN_POINT('Ctrl Pts',(-0.0530508054601922,2.41787864869009,
4.97111026556675));
#53592=CARTESIAN_POINT('Ctrl Pts',(-0.0528355330996498,2.41791450060592,
4.9710967120665));
#53593=CARTESIAN_POINT('Ctrl Pts',(-0.0523515286224808,2.41799460254804,
4.97106627275392));
#53594=CARTESIAN_POINT('Ctrl Pts',(-0.0520827773663643,2.41803873050608,
4.97104939400537));
#53595=CARTESIAN_POINT('Ctrl Pts',(-0.0512848511968853,2.41816870848262,
4.97099934866596));
#53596=CARTESIAN_POINT('Ctrl Pts',(-0.0507555143419635,2.4182535793883,
4.97096623765473));
#53597=CARTESIAN_POINT('Ctrl Pts',(-0.0464817112175732,2.41892788301294,
4.97069960020094));
#53598=CARTESIAN_POINT('Ctrl Pts',(-0.0427271268090138,2.41945256258654,
4.97046967135441));
#53599=CARTESIAN_POINT('Ctrl Pts',(-0.0290514684207105,2.42111820708981,
4.96964497791762));
#53600=CARTESIAN_POINT('Ctrl Pts',(-0.019087289661456,2.42186426015096,
4.9690684034992));
#53601=CARTESIAN_POINT('Ctrl Pts',(0.0225361987648381,2.42304052415228,
4.96670299882422));
#53602=CARTESIAN_POINT('Ctrl Pts',(0.0541331972883655,2.41926902255556,
4.96499186891994));
#53603=CARTESIAN_POINT('Ctrl Pts',(0.0900702326479179,2.40948312028369,
4.96278263195383));
#53604=CARTESIAN_POINT('Ctrl Pts',(0.0954265477058944,2.40787370250556,
4.96244678978236));
#53605=CARTESIAN_POINT('Ctrl Pts',(0.10166385252573,2.40582116776102,4.96204700758918));
#53606=CARTESIAN_POINT('Ctrl Pts',(0.102588264797286,2.40551231309757,4.96198753078389));
#53607=CARTESIAN_POINT('Ctrl Pts',(0.103983286084491,2.40503917827812,4.96189742744099));
#53608=CARTESIAN_POINT('Ctrl Pts',(0.104454944084816,2.40487798989324,4.96186690319567));
#53609=CARTESIAN_POINT('Ctrl Pts',(0.105297483412978,2.40458786874787,4.96181226817832));
#53610=CARTESIAN_POINT('Ctrl Pts',(0.105668507407683,2.40445935088537,4.96178817119696));
#53611=CARTESIAN_POINT('Ctrl Pts',(0.106452312766385,2.40418624562274,4.96173718508696));
#53612=CARTESIAN_POINT('Ctrl Pts',(0.10686503620849,2.40404149544515,4.96171029059445));
#53613=CARTESIAN_POINT('Ctrl Pts',(0.107959305193172,2.40365521054573,4.96163885860543));
#53614=CARTESIAN_POINT('Ctrl Pts',(0.108640331808949,2.40341222249637,4.96159427285685));
#53615=CARTESIAN_POINT('Ctrl Pts',(0.111770688938348,2.40228343089694,4.96138873156491));
#53616=CARTESIAN_POINT('Ctrl Pts',(0.114209986591381,2.40137026698525,4.9612268660532));
#53617=CARTESIAN_POINT('Ctrl Pts',(0.132647455058963,2.39421211295628,4.95999012594554));
#53618=CARTESIAN_POINT('Ctrl Pts',(0.148131934769037,2.3867278776924,4.9588728290175));
#53619=CARTESIAN_POINT('Ctrl Pts',(0.189113194512018,2.3627115362149,4.95570245111312));
#53620=CARTESIAN_POINT('Ctrl Pts',(0.212985217171318,2.34375908173166,4.95359301430377));
#53621=CARTESIAN_POINT('Ctrl Pts',(0.234924769645321,2.32062171719677,4.95157537334494));
#53622=CARTESIAN_POINT('Ctrl Pts',(0.235985663713025,2.31948657417719,4.95147762625543));
#53623=CARTESIAN_POINT('Ctrl Pts',(0.237327728052484,2.31802960252633,4.95135378925536));
#53624=CARTESIAN_POINT('Ctrl Pts',(0.237616501121513,2.31771485130814,4.95132713216683));
#53625=CARTESIAN_POINT('Ctrl Pts',(0.238074220426648,2.31721395991472,4.9512848632618));
#53626=CARTESIAN_POINT('Ctrl Pts',(0.238243574847161,2.31702819599921,4.95126922040223));
#53627=CARTESIAN_POINT('Ctrl Pts',(0.238558607954501,2.31668182483127,4.95124011530601));
#53628=CARTESIAN_POINT('Ctrl Pts',(0.238704340814863,2.31652126989736,4.95122664896153));
#53629=CARTESIAN_POINT('Ctrl Pts',(0.239028435933346,2.31616348709024,4.95119669555889));
#53630=CARTESIAN_POINT('Ctrl Pts',(0.239206715734693,2.31596618597456,4.95118021481238));
#53631=CARTESIAN_POINT('Ctrl Pts',(0.239727800298777,2.31538806820237,4.95113203208205));
#53632=CARTESIAN_POINT('Ctrl Pts',(0.240069943345522,2.31500665215448,4.95110038011802));
#53633=CARTESIAN_POINT('Ctrl Pts',(0.240844396508689,2.3141391497589,4.95102869557715));
#53634=CARTESIAN_POINT('Ctrl Pts',(0.241276149017725,2.31365256544504,4.95098870402498));
#53635=CARTESIAN_POINT('Ctrl Pts',(0.255837842019844,2.29714112953975,4.94963882967666));
#53636=CARTESIAN_POINT('Ctrl Pts',(0.268343427761699,2.27974911802647,4.94844310701638));
#53637=CARTESIAN_POINT('Ctrl Pts',(0.290487159757172,2.24142897747541,4.94596843700238));
#53638=CARTESIAN_POINT('Ctrl Pts',(0.299793301913102,2.22045244646608,4.94469378482681));
#53639=CARTESIAN_POINT('Ctrl Pts',(0.306907861206409,2.19833039312343,4.94331874786958));
#53640=CARTESIAN_POINT('Ctrl Pts',(0.307015917992102,2.19799248736597,4.94329773922019));
#53641=CARTESIAN_POINT('Ctrl Pts',(0.308869314849948,2.19216354830406,4.94293523702275));
#53642=CARTESIAN_POINT('Ctrl Pts',(0.310467557689133,2.18662714662972,4.94258938599066));
#53643=CARTESIAN_POINT('Ctrl Pts',(0.312163835300871,2.18009920665505,4.9421787714325));
#53644=CARTESIAN_POINT('Ctrl Pts',(0.31240683133674,2.17914616021652,4.94211875478632));
#53645=CARTESIAN_POINT('Ctrl Pts',(0.312766857644355,2.1777066196658,4.94202799284582));
#53646=CARTESIAN_POINT('Ctrl Pts',(0.312887125325678,2.177220934866,4.94199735210328));
#53647=CARTESIAN_POINT('Ctrl Pts',(0.313099805080128,2.17635340222543,4.94194258737468));
#53648=CARTESIAN_POINT('Ctrl Pts',(0.313192651098484,2.17597166095557,4.94191847743297));
#53649=CARTESIAN_POINT('Ctrl Pts',(0.313387129071949,2.17516563909467,4.94186754563762));
#53650=CARTESIAN_POINT('Ctrl Pts',(0.313488597887623,2.17474132029835,4.94184071858365));
#53651=CARTESIAN_POINT('Ctrl Pts',(0.313754825874647,2.17361793737006,4.94176965439154));
#53652=CARTESIAN_POINT('Ctrl Pts',(0.3139181096242,2.17291852918753,4.94172536988332));
#53653=CARTESIAN_POINT('Ctrl Pts',(0.314651739773671,2.16972796735458,4.94152316304693));
#53654=CARTESIAN_POINT('Ctrl Pts',(0.31519476699923,2.16723068514589,4.94136436641353));
#53655=CARTESIAN_POINT('Ctrl Pts',(0.317431347067279,2.15632173864572,4.94066822734824));
#53656=CARTESIAN_POINT('Ctrl Pts',(0.318818152565558,2.14785145346323,4.94012121866955));
#53657=CARTESIAN_POINT('Ctrl Pts',(0.321629972427538,2.12498712042102,4.93862639135604));
#53658=CARTESIAN_POINT('Ctrl Pts',(0.322426885125518,2.11053666742506,4.93766171497881));
#53659=CARTESIAN_POINT('Ctrl Pts',(0.322118612248737,2.08517567533685,4.93595025601389));
#53660=CARTESIAN_POINT('Ctrl Pts',(0.321432353448473,2.07428222323742,4.93520946009156));
#53661=CARTESIAN_POINT('Ctrl Pts',(0.318559899753805,2.04912194627197,4.93350583779406));
#53662=CARTESIAN_POINT('Ctrl Pts',(0.315965351473869,2.03492317229471,4.9325498529394));
#53663=CARTESIAN_POINT('Ctrl Pts',(0.312211581362928,2.02008827536237,4.93158776963432));
#53664=CARTESIAN_POINT('Ctrl Pts',(0.311991462736948,2.01923315968619,4.93153244718585));
#53665=CARTESIAN_POINT('Ctrl Pts',(0.311689306878116,2.01807901533772,4.9314579703632));
#53666=CARTESIAN_POINT('Ctrl Pts',(0.311610351183128,2.01777919492188,4.93143864047791));
#53667=CARTESIAN_POINT('Ctrl Pts',(0.311476273151781,2.01727302431225,4.93140603698993));
#53668=CARTESIAN_POINT('Ctrl Pts',(0.311421378339076,2.01706661494332,4.93139275020344));
#53669=CARTESIAN_POINT('Ctrl Pts',(0.311311329296443,2.01665447075513,4.93136623717617));
#53670=CARTESIAN_POINT('Ctrl Pts',(0.311256176734703,2.0164487376626,4.93135301103546));
#53671=CARTESIAN_POINT('Ctrl Pts',(0.311129591912441,2.01597840888347,4.93132279400105));
#53672=CARTESIAN_POINT('Ctrl Pts',(0.311058026175602,2.01571384994894,4.93130581100523));
#53673=CARTESIAN_POINT('Ctrl Pts',(0.310841818368519,2.01491861475394,4.93125480326497));
#53674=CARTESIAN_POINT('Ctrl Pts',(0.310696154181569,2.01438821372391,4.93122083776021));
#53675=CARTESIAN_POINT('Ctrl Pts',(0.310359140540996,2.01317324870739,4.93114315596628));
#53676=CARTESIAN_POINT('Ctrl Pts',(0.310166882007339,2.0124889367837,4.9310994913013));
#53677=CARTESIAN_POINT('Ctrl Pts',(0.3095296218116,2.01024919953733,4.93095685115454));
#53678=CARTESIAN_POINT('Ctrl Pts',(0.309075163547145,2.00869645962982,4.93085839574877));
#53679=CARTESIAN_POINT('Ctrl Pts',(0.307172379495514,2.00237229765838,4.93045891718404));
#53680=CARTESIAN_POINT('Ctrl Pts',(0.305625028726907,1.99763112468333,4.93016297582191));
#53681=CARTESIAN_POINT('Ctrl Pts',(0.298446854704317,1.97725300163685,4.92889879734349));
#53682=CARTESIAN_POINT('Ctrl Pts',(0.29172090269926,1.96202768642256,4.92797351204341));
#53683=CARTESIAN_POINT('Ctrl Pts',(0.271449038642051,1.92432310109351,4.92558069045999));
#53684=CARTESIAN_POINT('Ctrl Pts',(0.256285466088191,1.90285931328351,4.924108867789));
#53685=CARTESIAN_POINT('Ctrl Pts',(0.237656837394638,1.88232412738319,4.92242765980989));
#53686=CARTESIAN_POINT('Ctrl Pts',(0.236611623555963,1.88118844329193,4.92233372892197));
#53687=CARTESIAN_POINT('Ctrl Pts',(0.235182587814837,1.87965792707016,4.92220582218965));
#53688=CARTESIAN_POINT('Ctrl Pts',(0.234805840942989,1.87925649326101,4.92217214938553));
#53689=CARTESIAN_POINT('Ctrl Pts',(0.23416590652874,1.87857811804576,4.92211503384966));
#53690=CARTESIAN_POINT('Ctrl Pts',(0.233903250839194,1.87830067471143,4.92209161405256));
#53691=CARTESIAN_POINT('Ctrl Pts',(0.233396625760517,1.87776742888401,4.92204648407902));
#53692=CARTESIAN_POINT('Ctrl Pts',(0.233152727485863,1.87751155929903,4.92202477699577));
#53693=CARTESIAN_POINT('Ctrl Pts',(0.232576548693942,1.87690908766511,4.92197354183132));
#53694=CARTESIAN_POINT('Ctrl Pts',(0.232243914259228,1.87656282660576,4.92194399840028));
#53695=CARTESIAN_POINT('Ctrl Pts',(0.231272526633299,1.87555615803756,4.92185782447984));
#53696=CARTESIAN_POINT('Ctrl Pts',(0.230631725549644,1.8748977412103,4.9218011046692));
#53697=CARTESIAN_POINT('Ctrl Pts',(0.226008115444792,1.87018749492261,4.92139274397734));
#53698=CARTESIAN_POINT('Ctrl Pts',(0.221921805314116,1.86623909346406,4.92103654449244));
#53699=CARTESIAN_POINT('Ctrl Pts',(0.208276177960231,1.85373437244721,4.91986095935454));
#53700=CARTESIAN_POINT('Ctrl Pts',(0.198310988337186,1.84564117916157,4.919023077544));
#53701=CARTESIAN_POINT('Ctrl Pts',(0.166979342514135,1.82315787851648,4.91645524053457));
#53702=CARTESIAN_POINT('Ctrl Pts',(0.144346563418404,1.81071179923744,4.91467843008413));
#53703=CARTESIAN_POINT('Ctrl Pts',(0.119867772167208,1.80084565593393,4.9129509756304));
#53704=CARTESIAN_POINT('Ctrl Pts',(0.119259704409608,1.80060272664195,4.91290818688716));
#53705=CARTESIAN_POINT('Ctrl Pts',(0.118107154228722,1.80014633942668,4.91282732028419));
#53706=CARTESIAN_POINT('Ctrl Pts',(0.117562823543743,1.79993250731083,4.91278922782771));
#53707=CARTESIAN_POINT('Ctrl Pts',(0.116104641530133,1.79936425933894,4.91268745518606));
#53708=CARTESIAN_POINT('Ctrl Pts',(0.115189743210504,1.7990125260885,4.91262388522602));
#53709=CARTESIAN_POINT('Ctrl Pts',(0.114031636473136,1.79857334511165,4.91254378762926));
#53710=CARTESIAN_POINT('Ctrl Pts',(0.113789918209831,1.79848201229681,4.91252709016359));
#53711=CARTESIAN_POINT('Ctrl Pts',(0.109546616859029,1.79688451781218,4.9122343310971));
#53712=CARTESIAN_POINT('Ctrl Pts',(0.105515314470069,1.79545775395595,4.91196181916322));
#53713=CARTESIAN_POINT('Ctrl Pts',(0.100939315151927,1.79393999399408,4.91165971645277));
#53714=CARTESIAN_POINT('Ctrl Pts',(0.100421614059181,1.79376974013052,4.91162564187411));
#53715=CARTESIAN_POINT('Ctrl Pts',(0.0996388310344936,1.79351450856575,
4.91157427878358));
#53716=CARTESIAN_POINT('Ctrl Pts',(0.0993740700341939,1.79342856082816,
4.91155693364632));
#53717=CARTESIAN_POINT('Ctrl Pts',(0.0989140740047226,1.7932798936513,4.9115268461984));
#53718=CARTESIAN_POINT('Ctrl Pts',(0.0987188904218197,1.79321701750391,
4.9115140946151));
#53719=CARTESIAN_POINT('Ctrl Pts',(0.098326416285836,1.79309099981352,4.91148848412391));
#53720=CARTESIAN_POINT('Ctrl Pts',(0.0981291250528937,1.79302786225508,
4.91147562549983));
#53721=CARTESIAN_POINT('Ctrl Pts',(0.0976511473070049,1.7928754066882,4.91144450991313));
#53722=CARTESIAN_POINT('Ctrl Pts',(0.0973703980071717,1.79278628288943,
4.9114262644739));
#53723=CARTESIAN_POINT('Ctrl Pts',(0.0964694179139788,1.79250162610258,
4.91136780911793));
#53724=CARTESIAN_POINT('Ctrl Pts',(0.0958487122960348,1.79230758392387,
4.91132768655093));
#53725=CARTESIAN_POINT('Ctrl Pts',(0.0943896870109544,1.79185631348505,
4.91123371426582));
#53726=CARTESIAN_POINT('Ctrl Pts',(0.0935508916661377,1.79160062376468,
4.91117995205819));
#53727=CARTESIAN_POINT('Ctrl Pts',(0.0906499029710511,1.79072924102489,
4.91099488685064));
#53728=CARTESIAN_POINT('Ctrl Pts',(0.0885825422377806,1.79013076785538,
4.91086452117648));
#53729=CARTESIAN_POINT('Ctrl Pts',(0.0796508718086383,1.78764186488825,
4.91030720788724));
#53730=CARTESIAN_POINT('Ctrl Pts',(0.0727304956507097,1.78595835325802,
4.90989034566553));
#53731=CARTESIAN_POINT('Ctrl Pts',(0.0557793061854829,1.78242516294654,
4.90889292126009));
#53732=CARTESIAN_POINT('Ctrl Pts',(0.0457054754876024,1.78081958425325,
4.90831986355142));
#53733=CARTESIAN_POINT('Ctrl Pts',(0.0126161561991393,1.77714479862516,
4.9064563309362));
#53734=CARTESIAN_POINT('Ctrl Pts',(-0.0105450421554305,1.77707068013885,
4.90517593918929));
#53735=CARTESIAN_POINT('Ctrl Pts',(-0.0340603516362207,1.77952945658949,
4.9037844805471));
#53736=CARTESIAN_POINT('Ctrl Pts',(-0.0346059736006281,1.77958791637398,
4.90375214751362));
#53737=CARTESIAN_POINT('Ctrl Pts',(-0.0370285748449317,1.77985374229101,
4.9036083722892));
#53738=CARTESIAN_POINT('Ctrl Pts',(-0.0389038331065797,1.78007620713922,
4.90349650885488));
#53739=CARTESIAN_POINT('Ctrl Pts',(-0.0457185701542494,1.78094545235103,
4.90308777707625));
#53740=CARTESIAN_POINT('Ctrl Pts',(-0.0506446370890009,1.78169023169552,
4.90278806349461));
#53741=CARTESIAN_POINT('Ctrl Pts',(-0.0563944995492054,1.78269640900079,
4.9024325737323));
#53742=CARTESIAN_POINT('Ctrl Pts',(-0.0572371347822403,1.78284732569291,
4.90238033452974));
#53743=CARTESIAN_POINT('Ctrl Pts',(-0.0585849977047262,1.78309427563108,
4.90229654169261));
#53744=CARTESIAN_POINT('Ctrl Pts',(-0.0590906181149852,1.78318816477316,
4.90226505635006));
#53745=CARTESIAN_POINT('Ctrl Pts',(-0.0599851499888794,1.7833564872005,
4.90220925971586));
#53746=CARTESIAN_POINT('Ctrl Pts',(-0.0603741539823994,1.78343042795322,
4.90218496416936));
#53747=CARTESIAN_POINT('Ctrl Pts',(-0.061180671074282,1.78358526903079,
4.90213452710143));
#53748=CARTESIAN_POINT('Ctrl Pts',(-0.061598162073709,1.78366627920217,
4.90210838211758));
#53749=CARTESIAN_POINT('Ctrl Pts',(-0.0626719243003144,1.78387683886596,
4.90204104447265));
#53750=CARTESIAN_POINT('Ctrl Pts',(-0.0633279523224707,1.78400760524223,
4.90199981301688));
#53751=CARTESIAN_POINT('Ctrl Pts',(-0.0660465977404793,1.78455832027943,
4.90182856580469));
#53752=CARTESIAN_POINT('Ctrl Pts',(-0.0681054465392296,1.78499642193805,
4.9016979707848));
#53753=CARTESIAN_POINT('Ctrl Pts',(-0.0819021885258003,1.78807380619137,
4.90081656257755));
#53754=CARTESIAN_POINT('Ctrl Pts',(-0.0934872709603142,1.79134811145348,
4.90004535706683));
#53755=CARTESIAN_POINT('Ctrl Pts',(-0.118037164213278,1.79979579047846,
4.89834238871617));
#53756=CARTESIAN_POINT('Ctrl Pts',(-0.130904235254047,1.80517910128837,
4.8974060981435));
#53757=CARTESIAN_POINT('Ctrl Pts',(-0.156012751790007,1.81765248781097,
4.89551012055536));
#53758=CARTESIAN_POINT('Ctrl Pts',(-0.168218820636678,1.8247500149342,4.89455235768706));
#53759=CARTESIAN_POINT('Ctrl Pts',(-0.187449868611456,1.83769088207898,
4.89301814238897));
#53760=CARTESIAN_POINT('Ctrl Pts',(-0.19476223326193,1.84307348380651,4.89242838634614));
#53761=CARTESIAN_POINT('Ctrl Pts',(-0.202397233178494,1.84920715798605,
4.89181377737325));
#53762=CARTESIAN_POINT('Ctrl Pts',(-0.202954644578776,1.84965803014506,
4.89176891387104));
#53763=CARTESIAN_POINT('Ctrl Pts',(-0.203730781650267,1.85029011853364,
4.8917064622363));
#53764=CARTESIAN_POINT('Ctrl Pts',(-0.203950774068478,1.85046976525445,
4.89168876242783));
#53765=CARTESIAN_POINT('Ctrl Pts',(-0.20433031942275,1.85078054080631,4.89165822912815));
#53766=CARTESIAN_POINT('Ctrl Pts',(-0.204489983837239,1.85091153220795,
4.89164538569328));
#53767=CARTESIAN_POINT('Ctrl Pts',(-0.204810273912798,1.85117481914578,
4.89161962389364));
#53768=CARTESIAN_POINT('Ctrl Pts',(-0.204970897090989,1.85130711656083,
4.89160670577159));
#53769=CARTESIAN_POINT('Ctrl Pts',(-0.205299163985142,1.85157802792428,
4.89158030719383));
#53770=CARTESIAN_POINT('Ctrl Pts',(-0.205466795978473,1.8517166564306,4.89156682778007));
#53771=CARTESIAN_POINT('Ctrl Pts',(-0.206024825204633,1.85217908828728,
4.89152195981218));
#53772=CARTESIAN_POINT('Ctrl Pts',(-0.206414600923051,1.85250364564947,
4.89149062600046));
#53773=CARTESIAN_POINT('Ctrl Pts',(-0.209158625115843,1.85479952340239,
4.89127006377298));
#53774=CARTESIAN_POINT('Ctrl Pts',(-0.211485461943075,1.85680356655684,
4.89108318069101));
#53775=CARTESIAN_POINT('Ctrl Pts',(-0.218456199692757,1.86298299943317,
4.89052250082994));
#53776=CARTESIAN_POINT('Ctrl Pts',(-0.223007936643175,1.86726057393529,
4.89015525580672));
#53777=CARTESIAN_POINT('Ctrl Pts',(-0.231209344535718,1.87542968286756,
4.88948499572229));
#53778=CARTESIAN_POINT('Ctrl Pts',(-0.234892137846137,1.8792846267259,4.88918056091153));
#53779=CARTESIAN_POINT('Ctrl Pts',(-0.2588322070827,1.90562200977954,4.88716418725922));
#53780=CARTESIAN_POINT('Ctrl Pts',(-0.275930231567867,1.93076811539111,
4.88552213332932));
#53781=CARTESIAN_POINT('Ctrl Pts',(-0.289433127595241,1.95826159141789,
4.88370980546362));
#53782=CARTESIAN_POINT('Ctrl Pts',(-0.289595244123922,1.95859311757843,
4.88368795218456));
#53783=CARTESIAN_POINT('Ctrl Pts',(-0.292279880270452,1.96410714284778,
4.88332448532333));
#53784=CARTESIAN_POINT('Ctrl Pts',(-0.294663360651078,1.96935584767068,
4.8829785127219));
#53785=CARTESIAN_POINT('Ctrl Pts',(-0.297287267483676,1.97557161183215,
4.88256776650722));
#53786=CARTESIAN_POINT('Ctrl Pts',(-0.297665659860272,1.97647956405412,
4.88250774327529));
#53787=CARTESIAN_POINT('Ctrl Pts',(-0.298230257399003,1.97785197678372,
4.88241697330308));
#53788=CARTESIAN_POINT('Ctrl Pts',(-0.298419549601623,1.97831516768709,
4.88238633114226));
#53789=CARTESIAN_POINT('Ctrl Pts',(-0.298755537806978,1.97914281732393,
4.88233156483162));
#53790=CARTESIAN_POINT('Ctrl Pts',(-0.298902647857488,1.97950710777665,
4.88230745472925));
#53791=CARTESIAN_POINT('Ctrl Pts',(-0.299211711218769,1.98027649426032,
4.88225652358116));
#53792=CARTESIAN_POINT('Ctrl Pts',(-0.299373508694214,1.98068165167838,
4.88222969733709));
#53793=CARTESIAN_POINT('Ctrl Pts',(-0.29979946855865,1.98175461941225,4.88215863756179));
#53794=CARTESIAN_POINT('Ctrl Pts',(-0.300062221155235,1.9824229835366,4.88211435667104));
#53795=CARTESIAN_POINT('Ctrl Pts',(-0.301249592477169,1.98547320476046,
4.88191218954603));
#53796=CARTESIAN_POINT('Ctrl Pts',(-0.302148079004301,1.98786507437551,
4.88175342942669));
#53797=CARTESIAN_POINT('Ctrl Pts',(-0.30593919039407,1.99833392497667,4.88105739941803));
#53798=CARTESIAN_POINT('Ctrl Pts',(-0.30853685196925,2.00651327541375,4.8805104656047));
#53799=CARTESIAN_POINT('Ctrl Pts',(-0.318435690733512,2.04261773638176,
4.87808123122172));
#53800=CARTESIAN_POINT('Ctrl Pts',(-0.322292289400603,2.07134562550872,
4.87609432867143));
#53801=CARTESIAN_POINT('Ctrl Pts',(-0.322274941730377,2.10019379804403,
4.87417052639597));
#53802=CARTESIAN_POINT('',(-0.322274997047983,2.09995637979558,4.62467682828221));
#53803=CARTESIAN_POINT('Ctrl Pts',(-0.322274941450803,2.10019426240285,
4.87417049542921));
#53804=CARTESIAN_POINT('Ctrl Pts',(-0.322268128655327,2.11149646618101,
4.87341678409002));
#53805=CARTESIAN_POINT('Ctrl Pts',(-0.321666760855951,2.12279221049134,
4.87267666953879));
#53806=CARTESIAN_POINT('Ctrl Pts',(-0.320424902963008,2.13448569369698,
4.87193935096571));
#53807=CARTESIAN_POINT('Ctrl Pts',(-0.320376031233745,2.13493680187771,
4.87191095211947));
#53808=CARTESIAN_POINT('Ctrl Pts',(-0.320294868028792,2.13567148149227,
4.87186477682651));
#53809=CARTESIAN_POINT('Ctrl Pts',(-0.320263152514294,2.13595511396919,
4.87184696857217));
#53810=CARTESIAN_POINT('Ctrl Pts',(-0.320206675156625,2.13645418820485,
4.87181566618503));
#53811=CARTESIAN_POINT('Ctrl Pts',(-0.320182072613328,2.13666964726079,
4.87180216311917));
#53812=CARTESIAN_POINT('Ctrl Pts',(-0.320133378167099,2.1370923081101,4.87177569573478));
#53813=CARTESIAN_POINT('Ctrl Pts',(-0.320109302509417,2.13729951186743,
4.87176273048878));
#53814=CARTESIAN_POINT('Ctrl Pts',(-0.320060901577437,2.13771256916723,
4.87173690464753));
#53815=CARTESIAN_POINT('Ctrl Pts',(-0.320036578926151,2.13791842219309,
4.8717240439309));
#53816=CARTESIAN_POINT('Ctrl Pts',(-0.319978115060117,2.13840916341201,
4.87169340820454));
#53817=CARTESIAN_POINT('Ctrl Pts',(-0.319943791889473,2.13869403034452,
4.87167564353179));
#53818=CARTESIAN_POINT('Ctrl Pts',(-0.319820330693305,2.13970730693732,
4.87161252013109));
#53819=CARTESIAN_POINT('Ctrl Pts',(-0.319729084340935,2.14043546464048,
4.87156727967688));
#53820=CARTESIAN_POINT('Ctrl Pts',(-0.318336874951251,2.15124604585586,
4.87089733286547));
#53821=CARTESIAN_POINT('Ctrl Pts',(-0.316561887017375,2.16126289887626,
4.8702986931919));
#53822=CARTESIAN_POINT('Ctrl Pts',(-0.313962964170089,2.17273917804128,
4.86962136279284));
#53823=CARTESIAN_POINT('Ctrl Pts',(-0.313598303937198,2.17429559055922,
4.86952968879505));
#53824=CARTESIAN_POINT('Ctrl Pts',(-0.308532015426681,2.19521700439227,
4.86829915195087));
#53825=CARTESIAN_POINT('Ctrl Pts',(-0.302055595949303,2.21410856289424,
4.86720559521908));
#53826=CARTESIAN_POINT('Ctrl Pts',(-0.288420639419096,2.24439985878511,
4.86532880260235));
#53827=CARTESIAN_POINT('Ctrl Pts',(-0.282222028776344,2.25616804327379,
4.86456601735192));
#53828=CARTESIAN_POINT('Ctrl Pts',(-0.272308552442702,2.2724606763237,4.86343522251373));
#53829=CARTESIAN_POINT('Ctrl Pts',(-0.269169583373027,2.27731994114857,
4.86308784788229));
#53830=CARTESIAN_POINT('Ctrl Pts',(-0.265380204734901,2.282853423421,4.86267932171832));
#53831=CARTESIAN_POINT('Ctrl Pts',(-0.264855436120933,2.28361270503775,
4.86262297646148));
#53832=CARTESIAN_POINT('Ctrl Pts',(-0.264052222736889,2.28476425706182,
4.86253707624422));
#53833=CARTESIAN_POINT('Ctrl Pts',(-0.26377614634954,2.28515818003233,4.86250761177816));
#53834=CARTESIAN_POINT('Ctrl Pts',(-0.263295605950863,2.28584058905837,
4.86245643010016));
#53835=CARTESIAN_POINT('Ctrl Pts',(-0.263091546647212,2.28612936021965,
4.86243472843184));
#53836=CARTESIAN_POINT('Ctrl Pts',(-0.262666258801115,2.28672910260028,
4.86238956606743));
#53837=CARTESIAN_POINT('Ctrl Pts',(-0.262444952403878,2.28704001771347,
4.86236610239837));
#53838=CARTESIAN_POINT('Ctrl Pts',(-0.261903921812844,2.28779726515785,
4.86230883103157));
#53839=CARTESIAN_POINT('Ctrl Pts',(-0.26158360915885,2.28824317378112,4.86227500066798));
#53840=CARTESIAN_POINT('Ctrl Pts',(-0.260364349747404,2.28993138876847,
4.86214651446085));
#53841=CARTESIAN_POINT('Ctrl Pts',(-0.259457690959584,2.29116807665078,
4.86205156024783));
#53842=CARTESIAN_POINT('Ctrl Pts',(-0.258188081013857,2.29287416207649,
4.86191939145064));
#53843=CARTESIAN_POINT('Ctrl Pts',(-0.257832597204343,2.29334911270965,
4.86188247014929));
#53844=CARTESIAN_POINT('Ctrl Pts',(-0.236716853230922,2.32139940111636,
4.85969434212092));
#53845=CARTESIAN_POINT('Ctrl Pts',(-0.211666025758102,2.34545629989079,
4.85734672268934));
#53846=CARTESIAN_POINT('Ctrl Pts',(-0.175988098028588,2.37012624668841,
4.85442776457839));
#53847=CARTESIAN_POINT('Ctrl Pts',(-0.168479501207194,2.37487211219895,
4.85383542130252));
#53848=CARTESIAN_POINT('Ctrl Pts',(-0.157159769817998,2.38138846941071,
4.85298332544006));
#53849=CARTESIAN_POINT('Ctrl Pts',(-0.153495025439052,2.38340420751134,
4.85271349829144));
#53850=CARTESIAN_POINT('Ctrl Pts',(-0.148531186383487,2.38600994680659,
4.85235704602735));
#53851=CARTESIAN_POINT('Ctrl Pts',(-0.14726607644514,2.38666340174567,4.85226697134025));
#53852=CARTESIAN_POINT('Ctrl Pts',(-0.145143175727789,2.3877421600609,4.85211716236207));
#53853=CARTESIAN_POINT('Ctrl Pts',(-0.144287759498379,2.38817205737353,
4.85205715818387));
#53854=CARTESIAN_POINT('Ctrl Pts',(-0.143122279916794,2.3887512892182,4.85197590675229));
#53855=CARTESIAN_POINT('Ctrl Pts',(-0.142813885492725,2.38890394276794,
4.85195445467657));
#53856=CARTESIAN_POINT('Ctrl Pts',(-0.142322137422816,2.38914637556452,
4.85192032499414));
#53857=CARTESIAN_POINT('Ctrl Pts',(-0.142138943045734,2.38923647448601,
4.85190762732413));
#53858=CARTESIAN_POINT('Ctrl Pts',(-0.141757448412948,2.38942365174824,
4.85188122031524));
#53859=CARTESIAN_POINT('Ctrl Pts',(-0.141559134511655,2.38952070013796,
4.85186751294768));
#53860=CARTESIAN_POINT('Ctrl Pts',(-0.141101270043214,2.38974418125038,
4.85183591116737));
#53861=CARTESIAN_POINT('Ctrl Pts',(-0.1408416483862,2.38987046944743,4.85181802585306));
#53862=CARTESIAN_POINT('Ctrl Pts',(-0.140010570155516,2.39027335209213,
4.85176087975923));
#53863=CARTESIAN_POINT('Ctrl Pts',(-0.139438461309851,2.39054860903778,
4.85172170211838));
#53864=CARTESIAN_POINT('Ctrl Pts',(-0.134286039308753,2.39300885418631,
4.85137028360454));
#53865=CARTESIAN_POINT('Ctrl Pts',(-0.129655215699195,2.39508720923257,
4.85106448456639));
#53866=CARTESIAN_POINT('Ctrl Pts',(-0.124777432473551,2.39713938616822,
4.85075078170711));
#53867=CARTESIAN_POINT('Ctrl Pts',(-0.124577853788275,2.39722311621589,
4.85073796079745));
#53868=CARTESIAN_POINT('Ctrl Pts',(-0.120528645131049,2.39891710204929,
4.85047813139925));
#53869=CARTESIAN_POINT('Ctrl Pts',(-0.116648025050203,2.40045270722893,
4.8502344541806));
#53870=CARTESIAN_POINT('Ctrl Pts',(-0.0973425337813854,2.40766165707349,
4.84904328892021));
#53871=CARTESIAN_POINT('Ctrl Pts',(-0.0815283744665412,2.41222500997753,
4.84813226904585));
#53872=CARTESIAN_POINT('Ctrl Pts',(-0.0634174388931679,2.4159804528886,
4.84709737643731));
#53873=CARTESIAN_POINT('Ctrl Pts',(-0.0613966437774145,2.4163793138569,
4.84698203834633));
#53874=CARTESIAN_POINT('Ctrl Pts',(-0.0569698697425441,2.41720905310331,
4.84672946753446));
#53875=CARTESIAN_POINT('Ctrl Pts',(-0.0545625397841204,2.41763198598952,
4.84659217424934));
#53876=CARTESIAN_POINT('Ctrl Pts',(-0.049199147629875,2.41851148346717,
4.84628609520719));
#53877=CARTESIAN_POINT('Ctrl Pts',(-0.0462410873781094,2.41895435826742,
4.84611715067794));
#53878=CARTESIAN_POINT('Ctrl Pts',(-0.0394372929907041,2.41987637016344,
4.84572768648321));
#53879=CARTESIAN_POINT('Ctrl Pts',(-0.0355882665178808,2.42032743618227,
4.84550671726191));
#53880=CARTESIAN_POINT('Ctrl Pts',(-0.0197746804476762,2.4218920901358,
4.84459424930391));
#53881=CARTESIAN_POINT('Ctrl Pts',(-0.00776167628994374,2.4224054320035,
4.84388978840217));
#53882=CARTESIAN_POINT('Ctrl Pts',(0.00635418966876181,2.42221921712871,
4.84303653023704));
#53883=CARTESIAN_POINT('Ctrl Pts',(0.00845697275531886,2.42217088462533,
4.84290877476047));
#53884=CARTESIAN_POINT('Ctrl Pts',(0.0112274795880952,2.4220800623233,4.84273954849792));
#53885=CARTESIAN_POINT('Ctrl Pts',(0.0118957911237079,2.42205607118482,
4.84269865789764));
#53886=CARTESIAN_POINT('Ctrl Pts',(0.0129889325340823,2.42201342220907,
4.84263165915507));
#53887=CARTESIAN_POINT('Ctrl Pts',(0.0134138110157763,2.42199600327094,
4.84260558989657));
#53888=CARTESIAN_POINT('Ctrl Pts',(0.0142342726536967,2.42196073970551,
4.84255519348863));
#53889=CARTESIAN_POINT('Ctrl Pts',(0.0146298600493643,2.42194300679221,
4.84253086988713));
#53890=CARTESIAN_POINT('Ctrl Pts',(0.0155392175825932,2.4219005637038,4.84247489833979));
#53891=CARTESIAN_POINT('Ctrl Pts',(0.0160529622635845,2.42187535257235,
4.84244323473672));
#53892=CARTESIAN_POINT('Ctrl Pts',(0.0174218916145037,2.42180488919129,
4.84235874979769));
#53893=CARTESIAN_POINT('Ctrl Pts',(0.0182769556424048,2.42175745816472,
4.8423058602328));
#53894=CARTESIAN_POINT('Ctrl Pts',(0.0241106936887208,2.4214105271917,4.84194419742778));
#53895=CARTESIAN_POINT('Ctrl Pts',(0.0290817875505189,2.42099890603712,
4.84163192225173));
#53896=CARTESIAN_POINT('Ctrl Pts',(0.0354452542983857,2.42032296737841,
4.84122663125795));
#53897=CARTESIAN_POINT('Ctrl Pts',(0.0368483816991462,2.42016459227723,
4.84113691936874));
#53898=CARTESIAN_POINT('Ctrl Pts',(0.0615720046078876,2.41720928771899,
4.83955001167512));
#53899=CARTESIAN_POINT('Ctrl Pts',(0.0845152488114976,2.41188084254682,
4.83797290926765));
#53900=CARTESIAN_POINT('Ctrl Pts',(0.117922385920848,2.40016268419484,4.83557709613835));
#53901=CARTESIAN_POINT('Ctrl Pts',(0.12894585453008,2.39559485409365,4.83477050991965));
#53902=CARTESIAN_POINT('Ctrl Pts',(0.145281319472512,2.38773771426922,4.83357135995942));
#53903=CARTESIAN_POINT('Ctrl Pts',(0.150793000920482,2.38488793481828,4.83316613614821));
#53904=CARTESIAN_POINT('Ctrl Pts',(0.158002113638956,2.38089261685851,4.83263846629668));
#53905=CARTESIAN_POINT('Ctrl Pts',(0.159775532780996,2.37988767341365,4.83250885714809));
#53906=CARTESIAN_POINT('Ctrl Pts',(0.162268400156727,2.37844362410543,4.8323270738612));
#53907=CARTESIAN_POINT('Ctrl Pts',(0.162995802000475,2.37801844194476,4.83227408012897));
#53908=CARTESIAN_POINT('Ctrl Pts',(0.164265118212909,2.37726980511566,4.8321817040103));
#53909=CARTESIAN_POINT('Ctrl Pts',(0.164807761611215,2.37694760446531,4.83214224392933));
#53910=CARTESIAN_POINT('Ctrl Pts',(0.165598491076305,2.37647495284844,4.83208479351402));
#53911=CARTESIAN_POINT('Ctrl Pts',(0.165847321711147,2.37632576007698,4.83206672199443));
#53912=CARTESIAN_POINT('Ctrl Pts',(0.166274265406379,2.37606899062516,4.83203572781));
#53913=CARTESIAN_POINT('Ctrl Pts',(0.166452476047773,2.37596157728889,4.83202279440428));
#53914=CARTESIAN_POINT('Ctrl Pts',(0.166807339571422,2.37574722071598,4.83199704855406));
#53915=CARTESIAN_POINT('Ctrl Pts',(0.166983993388746,2.37564028047446,4.83198423595731));
#53916=CARTESIAN_POINT('Ctrl Pts',(0.167403304812929,2.37538589249596,4.83195383248506));
#53917=CARTESIAN_POINT('Ctrl Pts',(0.167645871068165,2.3752382934174,4.83193625158671));
#53918=CARTESIAN_POINT('Ctrl Pts',(0.168372146672137,2.37479504586338,4.83188363240171));
#53919=CARTESIAN_POINT('Ctrl Pts',(0.168855274556989,2.37449843947065,4.83184865654926));
#53920=CARTESIAN_POINT('Ctrl Pts',(0.173524394531838,2.37161493813981,4.83151087488642));
#53921=CARTESIAN_POINT('Ctrl Pts',(0.177651679100235,2.36893359304684,4.8312141415317));
#53922=CARTESIAN_POINT('Ctrl Pts',(0.1821138842968,2.36588708250768,4.83089351143413));
#53923=CARTESIAN_POINT('Ctrl Pts',(0.182510962329631,2.36561467604989,4.83086498117166));
#53924=CARTESIAN_POINT('Ctrl Pts',(0.183958819967914,2.36461662621113,4.83076095201303));
#53925=CARTESIAN_POINT('Ctrl Pts',(0.185005906809195,2.36388562076396,4.83068571870046));
#53926=CARTESIAN_POINT('Ctrl Pts',(0.208035144533708,2.34760371203934,4.82903042001129));
#53927=CARTESIAN_POINT('Ctrl Pts',(0.227988780203923,2.32936356013473,4.82757509403875));
#53928=CARTESIAN_POINT('Ctrl Pts',(0.255361709097943,2.29719496307759,4.82517797169339));
#53929=CARTESIAN_POINT('Ctrl Pts',(0.264436702590681,2.28484749174768,4.8242905871659));
#53930=CARTESIAN_POINT('Ctrl Pts',(0.273899678817082,2.26984134581946,4.82322038231216));
#53931=CARTESIAN_POINT('Ctrl Pts',(0.27517636809393,2.26776496280401,4.82307250538115));
#53932=CARTESIAN_POINT('Ctrl Pts',(0.276792354679387,2.26506867243317,4.82288066978062));
#53933=CARTESIAN_POINT('Ctrl Pts',(0.27715336030624,2.26446181649937,4.82283750557514));
#53934=CARTESIAN_POINT('Ctrl Pts',(0.277732808280146,2.26348042946233,4.82276771982976));
#53935=CARTESIAN_POINT('Ctrl Pts',(0.277952495676334,2.26310663308631,4.8227411436195));
#53936=CARTESIAN_POINT('Ctrl Pts',(0.278370111697928,2.26239276880576,4.82269039670057));
#53937=CARTESIAN_POINT('Ctrl Pts',(0.278568173299315,2.26205277927151,4.82266623087303));
#53938=CARTESIAN_POINT('Ctrl Pts',(0.279019188405874,2.26127530346146,4.82261097624568));
#53939=CARTESIAN_POINT('Ctrl Pts',(0.279271736067242,2.26083758402379,4.82257987283894));
#53940=CARTESIAN_POINT('Ctrl Pts',(0.280041894192321,2.2594954513706,4.82248451783246));
#53941=CARTESIAN_POINT('Ctrl Pts',(0.280556144690441,2.25858912682247,4.82242014533502));
#53942=CARTESIAN_POINT('Ctrl Pts',(0.284345061306474,2.25183536390115,4.82194057465915));
#53943=CARTESIAN_POINT('Ctrl Pts',(0.287440797539427,2.24588991967462,4.82151902166383));
#53944=CARTESIAN_POINT('Ctrl Pts',(0.291198620017513,2.23808828514821,4.82096605773868));
#53945=CARTESIAN_POINT('Ctrl Pts',(0.292032343852998,2.23631625243464,4.8208404768697));
#53946=CARTESIAN_POINT('Ctrl Pts',(0.303391096256598,2.21159134502695,4.81908849040367));
#53947=CARTESIAN_POINT('Ctrl Pts',(0.311197726987942,2.18748931346215,4.8173730224208));
#53948=CARTESIAN_POINT('Ctrl Pts',(0.318041263535512,2.15300241744209,4.8149999249504));
#53949=CARTESIAN_POINT('Ctrl Pts',(0.319521535311326,2.14319159989958,4.81433498082942));
#53950=CARTESIAN_POINT('Ctrl Pts',(0.321197690317714,2.12707023000438,4.81327295667407));
#53951=CARTESIAN_POINT('Ctrl Pts',(0.321664965062384,2.12079462817901,4.81286709042574));
#53952=CARTESIAN_POINT('Ctrl Pts',(0.321981371918348,2.11377365039208,4.81242432537052));
#53953=CARTESIAN_POINT('Ctrl Pts',(0.322011988022272,2.11303828601411,4.81237808949803));
#53954=CARTESIAN_POINT('Ctrl Pts',(0.322061679753676,2.1117375487786,4.81229655856279));
#53955=CARTESIAN_POINT('Ctrl Pts',(0.322081786338681,2.11117222169169,4.81226120791357));
#53956=CARTESIAN_POINT('Ctrl Pts',(0.322109531414066,2.11032968042448,4.81220865136003));
#53957=CARTESIAN_POINT('Ctrl Pts',(0.322118300630859,2.11005250842005,4.81219138250199));
#53958=CARTESIAN_POINT('Ctrl Pts',(0.322133135297717,2.10956366095423,4.81216096246701));
#53959=CARTESIAN_POINT('Ctrl Pts',(0.322139349874116,2.10935199076667,4.81214780288536));
#53960=CARTESIAN_POINT('Ctrl Pts',(0.322151364572573,2.10892853925314,4.81212150143145));
#53961=CARTESIAN_POINT('Ctrl Pts',(0.322157164473211,2.10871675905122,4.81210835960547));
#53962=CARTESIAN_POINT('Ctrl Pts',(0.322172430330033,2.10813849845567,4.81207250933764));
#53963=CARTESIAN_POINT('Ctrl Pts',(0.322181479834903,2.1077720059466,4.81204982436566));
#53964=CARTESIAN_POINT('Ctrl Pts',(0.322213438525605,2.10638158367025,4.81196389596481));
#53965=CARTESIAN_POINT('Ctrl Pts',(0.322232092321038,2.10535754809489,4.81190088861712));
#53966=CARTESIAN_POINT('Ctrl Pts',(0.322485255830175,2.08653158537324,4.81074738667012));
#53967=CARTESIAN_POINT('Ctrl Pts',(0.32124911896349,2.06873754545673,4.80973572988078));
#53968=CARTESIAN_POINT('Ctrl Pts',(0.313838026920968,2.02042553719714,4.8069925051278));
#53969=CARTESIAN_POINT('Ctrl Pts',(0.304712742059126,1.99056349005026,4.80528361107469));
#53970=CARTESIAN_POINT('Ctrl Pts',(0.290591778881093,1.96063826586778,4.80328269644488));
#53971=CARTESIAN_POINT('Ctrl Pts',(0.289710533985563,1.95881543603725,4.80315968384702));
#53972=CARTESIAN_POINT('Ctrl Pts',(0.288519695560239,1.95641032271227,4.80299582767971));
#53973=CARTESIAN_POINT('Ctrl Pts',(0.288225393876434,1.95582048528183,4.80295551871572));
#53974=CARTESIAN_POINT('Ctrl Pts',(0.287739218182699,1.95485353268535,4.80288923191766));
#53975=CARTESIAN_POINT('Ctrl Pts',(0.287548406463915,1.95447588312698,4.80286329137894));
#53976=CARTESIAN_POINT('Ctrl Pts',(0.28717720473359,1.95374479096842,4.80281297210186));
#53977=CARTESIAN_POINT('Ctrl Pts',(0.286996904477842,1.95339130344565,4.80278859655356));
#53978=CARTESIAN_POINT('Ctrl Pts',(0.286579069856641,1.95257584259151,4.80273225809954));
#53979=CARTESIAN_POINT('Ctrl Pts',(0.286341070946028,1.95211410969283,4.80270027886447));
#53980=CARTESIAN_POINT('Ctrl Pts',(0.285575090363893,1.95063684031922,4.80259770940755));
#53981=CARTESIAN_POINT('Ctrl Pts',(0.285042818939824,1.94962354897512,4.80252696775815));
#53982=CARTESIAN_POINT('Ctrl Pts',(0.280080937216537,1.94029855970708,4.80187233642857));
#53983=CARTESIAN_POINT('Ctrl Pts',(0.27529477503627,1.93218272322465,4.80127575448553));
#53984=CARTESIAN_POINT('Ctrl Pts',(0.254228450564688,1.89979271928812,4.79877854827676));
#53985=CARTESIAN_POINT('Ctrl Pts',(0.235039651075048,1.87757943941959,4.79676927091829));
#53986=CARTESIAN_POINT('Ctrl Pts',(0.205004019701675,1.85109880084923,4.79409378790848));
#53987=CARTESIAN_POINT('Ctrl Pts',(0.196523941432936,1.8443501457477,4.79338179226732));
#53988=CARTESIAN_POINT('Ctrl Pts',(0.186902877453307,1.83745572055375,4.79263323342299));
#53989=CARTESIAN_POINT('Ctrl Pts',(0.186083784810643,1.83687453684134,4.79256995503804));
#53990=CARTESIAN_POINT('Ctrl Pts',(0.184852203585605,1.83600930083761,4.79247549940798));
#53991=CARTESIAN_POINT('Ctrl Pts',(0.18444175719958,1.83572237207105,4.79244413435826));
#53992=CARTESIAN_POINT('Ctrl Pts',(0.183780242123295,1.83526222168505,4.79239376870911));
#53993=CARTESIAN_POINT('Ctrl Pts',(0.183529595407413,1.83508839913382,4.79237472791721));
#53994=CARTESIAN_POINT('Ctrl Pts',(0.183059261097417,1.83476321197031,4.79233907865184));
#53995=CARTESIAN_POINT('Ctrl Pts',(0.18283963189247,1.8346117639976,4.79232246452709));
#53996=CARTESIAN_POINT('Ctrl Pts',(0.182441750354263,1.83433812833652,4.79229242597892));
#53997=CARTESIAN_POINT('Ctrl Pts',(0.182263562946289,1.83421584706511,4.79227899513823));
#53998=CARTESIAN_POINT('Ctrl Pts',(0.181911687228781,1.83397489230373,4.79225251538646));
#53999=CARTESIAN_POINT('Ctrl Pts',(0.181738006293539,1.83385621002112,4.792239465858));
#54000=CARTESIAN_POINT('Ctrl Pts',(0.181317706356923,1.83356960758188,4.79220793583064));
#54001=CARTESIAN_POINT('Ctrl Pts',(0.181070969573557,1.83340185930513,4.792189467079));
#54002=CARTESIAN_POINT('Ctrl Pts',(0.180157314519947,1.832782548594,4.79212122799425));
#54003=CARTESIAN_POINT('Ctrl Pts',(0.179488929885066,1.83233313915921,4.79207160258001));
#54004=CARTESIAN_POINT('Ctrl Pts',(0.166933218304063,1.82395908937581,4.79114475263217));
#54005=CARTESIAN_POINT('Ctrl Pts',(0.154531818082685,1.81682987901813,4.79031900275228));
#54006=CARTESIAN_POINT('Ctrl Pts',(0.12489229302803,1.8023204021336,4.78845002941961));
#54007=CARTESIAN_POINT('Ctrl Pts',(0.107403620836295,1.79557313929471,4.78742062358528));
#54008=CARTESIAN_POINT('Ctrl Pts',(0.0744499114832903,1.78605502365687,
4.7854756855256));
#54009=CARTESIAN_POINT('Ctrl Pts',(0.0591794655796977,1.78282192188091,
4.78457270493879));
#54010=CARTESIAN_POINT('Ctrl Pts',(0.0412949831052748,1.78037213550469,
4.78348391645955));
#54011=CARTESIAN_POINT('Ctrl Pts',(0.0388499836119388,1.78006574793495,
4.78333443680278));
#54012=CARTESIAN_POINT('Ctrl Pts',(0.035697405382869,1.77970736286322,4.78314081112966));
#54013=CARTESIAN_POINT('Ctrl Pts',(0.0349927906499727,1.77962961631108,
4.7830974781047));
#54014=CARTESIAN_POINT('Ctrl Pts',(0.0338561977097987,1.7795080000561,4.78302748526975));
#54015=CARTESIAN_POINT('Ctrl Pts',(0.0334243746457255,1.77946267716843,
4.78300087128325));
#54016=CARTESIAN_POINT('Ctrl Pts',(0.0326012015240472,1.77937796084627,
4.78295009573004));
#54017=CARTESIAN_POINT('Ctrl Pts',(0.0322098680723235,1.77933841089321,
4.78292593913988));
#54018=CARTESIAN_POINT('Ctrl Pts',(0.0313167529035856,1.7792497999923,4.78287076642416));
#54019=CARTESIAN_POINT('Ctrl Pts',(0.0308149274061844,1.77920120003069,
4.78283973584789));
#54020=CARTESIAN_POINT('Ctrl Pts',(0.0292814555914005,1.77905632028465,
4.78274482018136));
#54021=CARTESIAN_POINT('Ctrl Pts',(0.0282494647856454,1.77896383865685,
4.78268081581378));
#54022=CARTESIAN_POINT('Ctrl Pts',(0.0206681939859864,1.77832128287119,
4.78220965879185));
#54023=CARTESIAN_POINT('Ctrl Pts',(0.0141043110404413,1.77796672617015,
4.78179639903181));
#54024=CARTESIAN_POINT('Ctrl Pts',(0.00703368274073614,1.77780137502898,
4.78134504303566));
#54025=CARTESIAN_POINT('Ctrl Pts',(0.00653279515968749,1.77779083003571,
4.78131303558347));
#54026=CARTESIAN_POINT('Ctrl Pts',(-0.0190737884633688,1.77731147828438,
4.77967504165991));
#54027=CARTESIAN_POINT('Ctrl Pts',(-0.0441447003268799,1.7797773806324,
4.7779777608863));
#54028=CARTESIAN_POINT('Ctrl Pts',(-0.0867273544029329,1.78906413278301,
4.77503097228658));
#54029=CARTESIAN_POINT('Ctrl Pts',(-0.104414975911622,1.79454878027021,
4.77378988504117));
#54030=CARTESIAN_POINT('Ctrl Pts',(-0.122191856685247,1.80178728036398,
4.77258567868829));
#54031=CARTESIAN_POINT('Ctrl Pts',(-0.122846121692588,1.80205620261458,
4.77254142421478));
#54032=CARTESIAN_POINT('Ctrl Pts',(-0.123781282844102,1.80244418555649,
4.77247826926928));
#54033=CARTESIAN_POINT('Ctrl Pts',(-0.124062897676875,1.80256149187852,
4.77245926368818));
#54034=CARTESIAN_POINT('Ctrl Pts',(-0.124549765577342,1.80276510787446,
4.77242642893027));
#54035=CARTESIAN_POINT('Ctrl Pts',(-0.12475509620438,1.8028512305688,4.77241258833444));
#54036=CARTESIAN_POINT('Ctrl Pts',(-0.125150757770159,1.80301766697324,
4.77238593204706));
#54037=CARTESIAN_POINT('Ctrl Pts',(-0.12534110031677,1.80309795071026,4.77237311454903));
#54038=CARTESIAN_POINT('Ctrl Pts',(-0.125793163755688,1.80328913674417,
4.77234268732114));
#54039=CARTESIAN_POINT('Ctrl Pts',(-0.126054815903675,1.80340020261198,
4.77232508760511));
#54040=CARTESIAN_POINT('Ctrl Pts',(-0.126838980215234,1.80373428906069,
4.77227237500421));
#54041=CARTESIAN_POINT('Ctrl Pts',(-0.127361053463563,1.80395834676073,
4.77223732486269));
#54042=CARTESIAN_POINT('Ctrl Pts',(-0.132434029451511,1.8061514146326,4.77189714943663));
#54043=CARTESIAN_POINT('Ctrl Pts',(-0.136939812009465,1.80822395961091,
4.77159819081554));
#54044=CARTESIAN_POINT('Ctrl Pts',(-0.151369038822595,1.81526897803176,
4.77064555783122));
#54045=CARTESIAN_POINT('Ctrl Pts',(-0.161084547826962,1.82065048447673,
4.77001141832463));
#54046=CARTESIAN_POINT('Ctrl Pts',(-0.17818285015979,1.83131070310796,4.76887503486144));
#54047=CARTESIAN_POINT('Ctrl Pts',(-0.185657024213084,1.83641976409258,
4.76837059430449));
#54048=CARTESIAN_POINT('Ctrl Pts',(-0.200010987435166,1.84714541917724,
4.76736856006734));
#54049=CARTESIAN_POINT('Ctrl Pts',(-0.206893265007696,1.8527450632355,4.76687145972178));
#54050=CARTESIAN_POINT('Ctrl Pts',(-0.224731240007123,1.86852542544296,
4.76551830727427));
#54051=CARTESIAN_POINT('Ctrl Pts',(-0.235222832762577,1.87919524049093,
4.76465064307751));
#54052=CARTESIAN_POINT('Ctrl Pts',(-0.2459659922425,1.89175874405818,4.7636532497755));
#54053=CARTESIAN_POINT('Ctrl Pts',(-0.246987604121375,1.89297146745341,
4.76355721978287));
#54054=CARTESIAN_POINT('Ctrl Pts',(-0.248762236370317,1.89510990937155,
4.76338828617161));
#54055=CARTESIAN_POINT('Ctrl Pts',(-0.249519147959675,1.89603236966802,
4.76331554166465));
#54056=CARTESIAN_POINT('Ctrl Pts',(-0.250607453805062,1.89737382927089,
4.76320993133883));
#54057=CARTESIAN_POINT('Ctrl Pts',(-0.250942962845622,1.89778948998671,
4.76317723151798));
#54058=CARTESIAN_POINT('Ctrl Pts',(-0.251526479257595,1.89851609480964,
4.76312011126511));
#54059=CARTESIAN_POINT('Ctrl Pts',(-0.251774947992806,1.89882666831957,
4.76309570941787));
#54060=CARTESIAN_POINT('Ctrl Pts',(-0.25225377927961,1.89942746010993,4.76304852996609));
#54061=CARTESIAN_POINT('Ctrl Pts',(-0.252484217631362,1.89971761743953,
4.76302575544581));
#54062=CARTESIAN_POINT('Ctrl Pts',(-0.253029288393582,1.90040638106119,
4.76297172032097));
#54063=CARTESIAN_POINT('Ctrl Pts',(-0.253343479359646,1.90080533398885,
4.76294044217932));
#54064=CARTESIAN_POINT('Ctrl Pts',(-0.254443992338109,1.90220955720428,
4.7628304213289));
#54065=CARTESIAN_POINT('Ctrl Pts',(-0.255225276624635,1.9032187443009,4.76275147902246));
#54066=CARTESIAN_POINT('Ctrl Pts',(-0.266526580048867,1.91799719448045,
4.76159722340893));
#54067=CARTESIAN_POINT('Ctrl Pts',(-0.27592353813765,1.93258595602232,4.76047766022678));
#54068=CARTESIAN_POINT('Ctrl Pts',(-0.293697794153064,1.96577640500607,
4.75797478464817));
#54069=CARTESIAN_POINT('Ctrl Pts',(-0.301576948587302,1.98456328165682,
4.75658403687646));
#54070=CARTESIAN_POINT('Ctrl Pts',(-0.3101888433781,2.01215023269976,4.75464910060457));
#54071=CARTESIAN_POINT('Ctrl Pts',(-0.312416526892854,2.02043470224888,
4.75408163622111));
#54072=CARTESIAN_POINT('Ctrl Pts',(-0.31525265901204,2.03295454173911,4.75325326273716));
#54073=CARTESIAN_POINT('Ctrl Pts',(-0.316111618806432,2.03712885140085,
4.75298185759566));
#54074=CARTESIAN_POINT('Ctrl Pts',(-0.3169878380855,2.04186060468506,4.75268052334854));
#54075=CARTESIAN_POINT('Ctrl Pts',(-0.317086705653594,2.04240225794249,
4.75264612206017));
#54076=CARTESIAN_POINT('Ctrl Pts',(-0.317232928903758,2.04321514068883,
4.75259463678681));
#54077=CARTESIAN_POINT('Ctrl Pts',(-0.317281325300182,2.04348617828385,
4.75257749387181));
#54078=CARTESIAN_POINT('Ctrl Pts',(-0.317363899786889,2.04395207519724,
4.75254806737087));
#54079=CARTESIAN_POINT('Ctrl Pts',(-0.31739824576466,2.044146903855,4.75253577416445));
#54080=CARTESIAN_POINT('Ctrl Pts',(-0.317469029612501,2.04455060131008,
4.75251032754907));
#54081=CARTESIAN_POINT('Ctrl Pts',(-0.3175054406621,2.0447594738552,4.75249717571326));
#54082=CARTESIAN_POINT('Ctrl Pts',(-0.317604386025712,2.0453304051715,4.75246126499654));
#54083=CARTESIAN_POINT('Ctrl Pts',(-0.317666507592022,2.04569253661826,
4.75243852972371));
#54084=CARTESIAN_POINT('Ctrl Pts',(-0.317900383443802,2.04707002479976,
4.75235220640011));
#54085=CARTESIAN_POINT('Ctrl Pts',(-0.318067892457474,2.04808611049339,
4.75228885722561));
#54086=CARTESIAN_POINT('Ctrl Pts',(-0.320907561612405,2.06584097587976,
4.7511873216208));
#54087=CARTESIAN_POINT('Ctrl Pts',(-0.322260290453718,2.08276679870848,
4.750220556137));
#54088=CARTESIAN_POINT('Ctrl Pts',(-0.32229447047123,2.12248874906482,4.74798769927676));
#54089=CARTESIAN_POINT('Ctrl Pts',(-0.3199017979713,2.14519145954743,4.74673518061688));
#54090=CARTESIAN_POINT('Ctrl Pts',(-0.314698395215594,2.16950171021866,
4.7452914527566));
#54091=CARTESIAN_POINT('Ctrl Pts',(-0.314239786475283,2.17154665620285,
4.74516924563928));
#54092=CARTESIAN_POINT('Ctrl Pts',(-0.313345478981616,2.17535981926996,
4.74493982652879));
#54093=CARTESIAN_POINT('Ctrl Pts',(-0.312914673320171,2.1771291034513,4.74483275304375));
#54094=CARTESIAN_POINT('Ctrl Pts',(-0.310863981700725,2.18525104352628,
4.74433818362047));
#54095=CARTESIAN_POINT('Ctrl Pts',(-0.309065572852634,2.1915566378076,4.74394557163244));
#54096=CARTESIAN_POINT('Ctrl Pts',(-0.306762017828688,2.19878923037657,
4.74348360007954));
#54097=CARTESIAN_POINT('Ctrl Pts',(-0.306443057872553,2.19977424448834,
4.74342043168156));
#54098=CARTESIAN_POINT('Ctrl Pts',(-0.305961779027517,2.20123645311741,
4.74332627989157));
#54099=CARTESIAN_POINT('Ctrl Pts',(-0.305803076107235,2.20171483817156,
4.7432954157721));
#54100=CARTESIAN_POINT('Ctrl Pts',(-0.305518534580197,2.20256585857512,
4.74324040104798));
#54101=CARTESIAN_POINT('Ctrl Pts',(-0.305393134550463,2.20293864038615,
4.74321626497472));
#54102=CARTESIAN_POINT('Ctrl Pts',(-0.305127837524803,2.20372254812007,
4.74316543111873));
#54103=CARTESIAN_POINT('Ctrl Pts',(-0.304987791397928,2.20413362241062,
4.74313872844051));
#54104=CARTESIAN_POINT('Ctrl Pts',(-0.304616837482741,2.20521530775314,
4.74306834254177));
#54105=CARTESIAN_POINT('Ctrl Pts',(-0.304384546993899,2.20588543904636,
4.74302461356063));
#54106=CARTESIAN_POINT('Ctrl Pts',(-0.303334191026098,2.20888357555696,
4.74282841531693));
#54107=CARTESIAN_POINT('Ctrl Pts',(-0.302491634034368,2.21120285637565,
4.74267513409293));
#54108=CARTESIAN_POINT('Ctrl Pts',(-0.296117965925828,2.22813885352821,
4.74154447449076));
#54109=CARTESIAN_POINT('Ctrl Pts',(-0.289557610523375,2.24234351633138,
4.74053220514915));
#54110=CARTESIAN_POINT('Ctrl Pts',(-0.266454111670279,2.28410269655956,
4.73736134912195));
#54111=CARTESIAN_POINT('Ctrl Pts',(-0.24680636084669,2.30970968101141,4.73512042852325));
#54112=CARTESIAN_POINT('Ctrl Pts',(-0.222612535317334,2.33303887158884,
4.73299451931738));
#54113=CARTESIAN_POINT('Ctrl Pts',(-0.221517979475821,2.33407956239844,
4.73289952506346));
#54114=CARTESIAN_POINT('Ctrl Pts',(-0.220104178893503,2.33540498909725,
4.73277838162719));
#54115=CARTESIAN_POINT('Ctrl Pts',(-0.219791650930607,2.33569681509194,
4.73275169888468));
#54116=CARTESIAN_POINT('Ctrl Pts',(-0.219296223276313,2.3361575831369,4.73270955468023));
#54117=CARTESIAN_POINT('Ctrl Pts',(-0.219113708422816,2.33632693540628,
4.73269406174996));
#54118=CARTESIAN_POINT('Ctrl Pts',(-0.218786697378166,2.33662965862673,
4.73266636232387));
#54119=CARTESIAN_POINT('Ctrl Pts',(-0.21864227641429,2.33676310788666,4.73265414979793));
#54120=CARTESIAN_POINT('Ctrl Pts',(-0.21830293274274,2.3370760962415,4.73262550251671));
#54121=CARTESIAN_POINT('Ctrl Pts',(-0.218107910957724,2.33725552687358,
4.73260907614257));
#54122=CARTESIAN_POINT('Ctrl Pts',(-0.21754352502898,2.33777350859236,4.73256164574526));
#54123=CARTESIAN_POINT('Ctrl Pts',(-0.217173590299353,2.33811144104149,
4.73253068890219));
#54124=CARTESIAN_POINT('Ctrl Pts',(-0.214655043948123,2.34040136125284,
4.73232081526259));
#54125=CARTESIAN_POINT('Ctrl Pts',(-0.212480843920028,2.34232518393617,
4.73214399038355));
#54126=CARTESIAN_POINT('Ctrl Pts',(-0.205576265880877,2.34827024933106,
4.73159484729011));
#54127=CARTESIAN_POINT('Ctrl Pts',(-0.200755281736487,2.35218454576287,
4.73122926383669));
#54128=CARTESIAN_POINT('Ctrl Pts',(-0.184258546457667,2.36480561303203,
4.73002521544727));
#54129=CARTESIAN_POINT('Ctrl Pts',(-0.172105993366381,2.37286041799107,
4.72921310604732));
#54130=CARTESIAN_POINT('Ctrl Pts',(-0.136465703089263,2.3931514549812,4.72692080766496));
#54131=CARTESIAN_POINT('Ctrl Pts',(-0.111962445982215,2.40335591723922,
4.72543634664687));
#54132=CARTESIAN_POINT('Ctrl Pts',(-0.0849414614765147,2.4108837508264,
4.72373618032123));
#54133=CARTESIAN_POINT('Ctrl Pts',(-0.0833901321576499,2.41130345985668,
4.72363840181915));
#54134=CARTESIAN_POINT('Ctrl Pts',(-0.0812339868929345,2.41186952732937,
4.72350224756173));
#54135=CARTESIAN_POINT('Ctrl Pts',(-0.0806317708512905,2.41202576852561,
4.72346419191757));
#54136=CARTESIAN_POINT('Ctrl Pts',(-0.0796672802145586,2.41227302094876,
4.72340319793779));
#54137=CARTESIAN_POINT('Ctrl Pts',(-0.0793052911839022,2.41236514840421,
4.72338029572481));
#54138=CARTESIAN_POINT('Ctrl Pts',(-0.0785591904951232,2.41255365306523,
4.72333307033914));
#54139=CARTESIAN_POINT('Ctrl Pts',(-0.0781750598429435,2.41264995197831,
4.72330874468141));
#54140=CARTESIAN_POINT('Ctrl Pts',(-0.0772827692325008,2.41287189585916,
4.72325221159709));
#54141=CARTESIAN_POINT('Ctrl Pts',(-0.0767744797801339,2.41299701098905,
4.72321998714346));
#54142=CARTESIAN_POINT('Ctrl Pts',(-0.0751624768244624,2.41338964158503,
4.72311772293767));
#54143=CARTESIAN_POINT('Ctrl Pts',(-0.0740576621192644,2.41365255937694,
4.72304753532863));
#54144=CARTESIAN_POINT('Ctrl Pts',(-0.0540452197870818,2.41830338047471,
4.72177430657084));
#54145=CARTESIAN_POINT('Ctrl Pts',(-0.0347843170496422,2.42097933122551,
4.72051511248661));
#54146=CARTESIAN_POINT('Ctrl Pts',(0.0145843283142795,2.42334155036074,
4.71721364217749));
#54147=CARTESIAN_POINT('Ctrl Pts',(0.0446242229580015,2.42057947129813,
4.71512719575121));
#54148=CARTESIAN_POINT('Ctrl Pts',(0.075351629882844,2.41334596602037,4.71312983752989));
#54149=CARTESIAN_POINT('Ctrl Pts',(0.0768529593083725,2.41298112629895,
4.71303264223228));
#54150=CARTESIAN_POINT('Ctrl Pts',(0.0787650941151597,2.41250186760287,
4.71290940731139));
#54151=CARTESIAN_POINT('Ctrl Pts',(0.0791783429142083,2.41239741888273,
4.71288280710551));
#54152=CARTESIAN_POINT('Ctrl Pts',(0.0798347677233625,2.41223012117625,
4.71284060817787));
#54153=CARTESIAN_POINT('Ctrl Pts',(0.0800780777510664,2.4121678077123,4.71282497858551));
#54154=CARTESIAN_POINT('Ctrl Pts',(0.080532667481871,2.41205081753032,4.71279579939799));
#54155=CARTESIAN_POINT('Ctrl Pts',(0.0807439629013194,2.41199621104831,
4.71278224588794));
#54156=CARTESIAN_POINT('Ctrl Pts',(0.0812188228869276,2.41187297511796,
4.71275180642207));
#54157=CARTESIAN_POINT('Ctrl Pts',(0.0814823554000284,2.41180422633416,
4.71273492753036));
#54158=CARTESIAN_POINT('Ctrl Pts',(0.0822643721400682,2.41159915935127,
4.71268488134413));
#54159=CARTESIAN_POINT('Ctrl Pts',(0.0827826069644153,2.41146188053434,
4.71265176963212));
#54160=CARTESIAN_POINT('Ctrl Pts',(0.086962590227864,2.41034344612227,4.71238511030734));
#54161=CARTESIAN_POINT('Ctrl Pts',(0.0906073014049481,2.40929899232091,
4.7121551609534));
#54162=CARTESIAN_POINT('Ctrl Pts',(0.10378384929359,2.40527010435142,4.71133034939099));
#54163=CARTESIAN_POINT('Ctrl Pts',(0.113194752466662,2.40190711793694,4.71075368353714));
#54164=CARTESIAN_POINT('Ctrl Pts',(0.151532163623229,2.38616189760132,4.70839939133914));
#54165=CARTESIAN_POINT('Ctrl Pts',(0.178721359323029,2.37001732351581,4.70669857777219));
#54166=CARTESIAN_POINT('Ctrl Pts',(0.20762171962464,2.34655161823008,4.70449235536249));
#54167=CARTESIAN_POINT('Ctrl Pts',(0.212003047743296,2.34279452269041,4.7041459639046));
#54168=CARTESIAN_POINT('Ctrl Pts',(0.21701046944905,2.33826162106833,4.70373476409637));
#54169=CARTESIAN_POINT('Ctrl Pts',(0.217736949909935,2.33759790515667,4.70367471820302));
#54170=CARTESIAN_POINT('Ctrl Pts',(0.218828301502073,2.3365916324509,4.70358392059871));
#54171=CARTESIAN_POINT('Ctrl Pts',(0.219195437626998,2.33625153164183,4.70355327356264));
#54172=CARTESIAN_POINT('Ctrl Pts',(0.219843467654706,2.33564841063624,4.70349899661171));
#54173=CARTESIAN_POINT('Ctrl Pts',(0.220124686106478,2.33538573930958,4.70347538166765));
#54174=CARTESIAN_POINT('Ctrl Pts',(0.220715455426778,2.33483194828122,4.70342564370211));
#54175=CARTESIAN_POINT('Ctrl Pts',(0.221024902104478,2.33454071894824,4.70339951598795));
#54176=CARTESIAN_POINT('Ctrl Pts',(0.221656081702871,2.33394433888966,4.70334606952108));
#54177=CARTESIAN_POINT('Ctrl Pts',(0.221977762518819,2.33363913456095,4.70331874848007));
#54178=CARTESIAN_POINT('Ctrl Pts',(0.222768752800128,2.33288555064095,4.70325136483833));
#54179=CARTESIAN_POINT('Ctrl Pts',(0.22323733803676,2.33243641672047,4.70321126953441));
#54180=CARTESIAN_POINT('Ctrl Pts',(0.224528197274878,2.33119163791149,4.7031003223998));
#54181=CARTESIAN_POINT('Ctrl Pts',(0.22534758975252,2.33039303060238,4.70302934137892));
#54182=CARTESIAN_POINT('Ctrl Pts',(0.232253276749586,2.3235904335203,4.7024263637213));
#54183=CARTESIAN_POINT('Ctrl Pts',(0.238102183101612,2.31735131611586,4.70188396789753));
#54184=CARTESIAN_POINT('Ctrl Pts',(0.24889836449907,2.30487554958358,4.7008180169498));
#54185=CARTESIAN_POINT('Ctrl Pts',(0.253876372178593,2.29867349867532,4.70029617891608));
#54186=CARTESIAN_POINT('Ctrl Pts',(0.277825862088175,2.26646341172295,4.69762991055377));
#54187=CARTESIAN_POINT('Ctrl Pts',(0.293052819310045,2.23790304731271,4.69538241483096));
#54188=CARTESIAN_POINT('Ctrl Pts',(0.304295683437239,2.2061487541136,4.69325189515312));
#54189=CARTESIAN_POINT('Ctrl Pts',(0.304785952355911,2.20473272846598,4.69315765127834));
#54190=CARTESIAN_POINT('Ctrl Pts',(0.305403001215232,2.20290949524154,4.69303733001132));
#54191=CARTESIAN_POINT('Ctrl Pts',(0.305538863947283,2.20250541441762,4.69301072775747));
#54192=CARTESIAN_POINT('Ctrl Pts',(0.305752715163683,2.2018651787608,4.69296868172219));
#54193=CARTESIAN_POINT('Ctrl Pts',(0.305831232171156,2.20162920300588,4.69295320671902));
#54194=CARTESIAN_POINT('Ctrl Pts',(0.305971352977167,2.20120644970894,4.69292552306731));
#54195=CARTESIAN_POINT('Ctrl Pts',(0.30603305850721,2.20101970800992,4.69291330843054));
#54196=CARTESIAN_POINT('Ctrl Pts',(0.306177627519708,2.20058084540187,4.69288463550763));
#54197=CARTESIAN_POINT('Ctrl Pts',(0.306260350424772,2.20032867892214,4.69286818565203));
#54198=CARTESIAN_POINT('Ctrl Pts',(0.306498909342499,2.19959842892441,4.69282062100725));
#54199=CARTESIAN_POINT('Ctrl Pts',(0.30665393894006,2.19912007976689,4.69278955381309));
#54200=CARTESIAN_POINT('Ctrl Pts',(0.307708205853703,2.19584095481054,4.6925771886934));
#54201=CARTESIAN_POINT('Ctrl Pts',(0.30857021693016,2.19302822832906,4.69239803991428));
#54202=CARTESIAN_POINT('Ctrl Pts',(0.311153591107174,2.18416742683443,4.69184193452161));
#54203=CARTESIAN_POINT('Ctrl Pts',(0.312736629787916,2.17808024210419,4.69147187046152));
#54204=CARTESIAN_POINT('Ctrl Pts',(0.317590849055811,2.15688632271318,4.69021227830414));
#54205=CARTESIAN_POINT('Ctrl Pts',(0.319953291456941,2.14159273671054,4.68935269184683));
#54206=CARTESIAN_POINT('Ctrl Pts',(0.323285875256329,2.10071660916601,4.68705991796746));
#54207=CARTESIAN_POINT('Ctrl Pts',(0.322325396691778,2.07509317366343,4.68562001907203));
#54208=CARTESIAN_POINT('Ctrl Pts',(0.318113695042522,2.04835551336149,4.68397845132261));
#54209=CARTESIAN_POINT('Ctrl Pts',(0.317867126552376,2.04685900162257,4.68388613893577));
#54210=CARTESIAN_POINT('Ctrl Pts',(0.317517356945999,2.04482570949266,4.68376010711967));
#54211=CARTESIAN_POINT('Ctrl Pts',(0.317423337497217,2.04428735241179,4.68372667943307));
#54212=CARTESIAN_POINT('Ctrl Pts',(0.317261459833271,2.04337415040534,4.68366987728087));
#54213=CARTESIAN_POINT('Ctrl Pts',(0.317194305312372,2.0429991805915,4.68364652522996));
#54214=CARTESIAN_POINT('Ctrl Pts',(0.317057959777484,2.04224557227749,4.68359953492941));
#54215=CARTESIAN_POINT('Ctrl Pts',(0.316988754933454,2.04186693691577,4.68357589627299));
#54216=CARTESIAN_POINT('Ctrl Pts',(0.316830292203949,2.04100864807557,4.68352224535904));
#54217=CARTESIAN_POINT('Ctrl Pts',(0.316740623250193,2.04052907232254,4.68349222004913));
#54218=CARTESIAN_POINT('Ctrl Pts',(0.316551036549072,2.03952769939121,4.68342942617512));
#54219=CARTESIAN_POINT('Ctrl Pts',(0.316450916901234,2.03900594235374,4.68339665124279));
#54220=CARTESIAN_POINT('Ctrl Pts',(0.316185721577719,2.03764215070368,4.68331083319887));
#54221=CARTESIAN_POINT('Ctrl Pts',(0.316018573161058,2.03680052774827,4.68325772399474));
#54222=CARTESIAN_POINT('Ctrl Pts',(0.315513609655335,2.03431004175316,4.68310011901254));
#54223=CARTESIAN_POINT('Ctrl Pts',(0.315166240409126,2.03266316590817,4.68299531862604));
#54224=CARTESIAN_POINT('Ctrl Pts',(0.312969347932007,2.02263727424979,4.68235369661809));
#54225=CARTESIAN_POINT('Ctrl Pts',(0.310798841185253,2.01433284144608,4.68180666570732));
#54226=CARTESIAN_POINT('Ctrl Pts',(0.304088306439989,1.99229431219967,4.68031177326691));
#54227=CARTESIAN_POINT('Ctrl Pts',(0.298951291259274,1.97876361516742,4.67934705270825));
#54228=CARTESIAN_POINT('Ctrl Pts',(0.282631438468832,1.94318806109096,4.67670590825821));
#54229=CARTESIAN_POINT('Ctrl Pts',(0.26979444527191,1.92200651886549,4.67501311919923));
#54230=CARTESIAN_POINT('Ctrl Pts',(0.253807897984132,1.90139315664724,4.67336477728538));
#54231=CARTESIAN_POINT('Ctrl Pts',(0.25294455753177,1.90029477150287,4.67327696293238));
#54232=CARTESIAN_POINT('Ctrl Pts',(0.251815549208849,1.89887745781029,4.67316371214626));
#54233=CARTESIAN_POINT('Ctrl Pts',(0.251556386683429,1.89855340131047,4.67313782253891));
#54234=CARTESIAN_POINT('Ctrl Pts',(0.251157867475305,1.89805706169818,4.67309817650121));
#54235=CARTESIAN_POINT('Ctrl Pts',(0.251018959006343,1.89788442181567,4.6730843879994));
#54236=CARTESIAN_POINT('Ctrl Pts',(0.250743084396651,1.89754227912291,4.67305706461617));
#54237=CARTESIAN_POINT('Ctrl Pts',(0.250606125232967,1.89737277302457,4.67304352945788));
#54238=CARTESIAN_POINT('Ctrl Pts',(0.250300828460356,1.89699570863196,4.67301342397207));
#54239=CARTESIAN_POINT('Ctrl Pts',(0.250132405010795,1.89678822128987,4.67299686001929));
#54240=CARTESIAN_POINT('Ctrl Pts',(0.249640806380492,1.89618413912813,4.67294864107108));
#54241=CARTESIAN_POINT('Ctrl Pts',(0.24931694279469,1.89578810172452,4.67291703571754));
#54242=CARTESIAN_POINT('Ctrl Pts',(0.246998859199979,1.8929671615086,4.67269195038114));
#54243=CARTESIAN_POINT('Ctrl Pts',(0.244970153439424,1.89057063633793,4.67250092433542));
#54244=CARTESIAN_POINT('Ctrl Pts',(0.240124849356564,1.88501360590962,4.6720573931713));
#54245=CARTESIAN_POINT('Ctrl Pts',(0.237280316945324,1.8818781359135,4.67180667961306));
#54246=CARTESIAN_POINT('Ctrl Pts',(0.224836253359085,1.86869293375816,4.67074576451726));
#54247=CARTESIAN_POINT('Ctrl Pts',(0.214653291626464,1.85921311260342,4.6699655944049));
#54248=CARTESIAN_POINT('Ctrl Pts',(0.189962177871301,1.83904222265235,4.66818205537132));
#54249=CARTESIAN_POINT('Ctrl Pts',(0.175107478445908,1.82885075209964,4.66718238465805));
#54250=CARTESIAN_POINT('Ctrl Pts',(0.149540783323748,1.81429107839264,4.66548187218267));
#54251=CARTESIAN_POINT('Ctrl Pts',(0.139307003016006,1.80916405371986,4.66480640465326));
#54252=CARTESIAN_POINT('Ctrl Pts',(0.127722463865901,1.804112200744,4.66403815130503));
#54253=CARTESIAN_POINT('Ctrl Pts',(0.126619117153392,1.80363836848408,4.6639649499326));
#54254=CARTESIAN_POINT('Ctrl Pts',(0.125069213822046,1.80298299761466,4.66386207025725));
#54255=CARTESIAN_POINT('Ctrl Pts',(0.124624849307177,1.802796273773,4.66383256826626));
#54256=CARTESIAN_POINT('Ctrl Pts',(0.123814248011677,1.8024577932902,4.66377873985155));
#54257=CARTESIAN_POINT('Ctrl Pts',(0.123448146313705,1.80230571393808,4.66375442442804));
#54258=CARTESIAN_POINT('Ctrl Pts',(0.122711693234474,1.8020013820337,4.66370550240214));
#54259=CARTESIAN_POINT('Ctrl Pts',(0.122341336872543,1.80184914345883,4.66368089537897));
#54260=CARTESIAN_POINT('Ctrl Pts',(0.121439686066852,1.8014804740226,4.6636209768788));
#54261=CARTESIAN_POINT('Ctrl Pts',(0.120908097023008,1.80126477139569,4.66358564085488));
#54262=CARTESIAN_POINT('Ctrl Pts',(0.119772473233747,1.80080749759525,4.66351013132357));
#54263=CARTESIAN_POINT('Ctrl Pts',(0.119168278073462,1.80056633400566,4.66346994422556));
#54264=CARTESIAN_POINT('Ctrl Pts',(0.117496005380549,1.79990471193144,4.66335867722148));
#54265=CARTESIAN_POINT('Ctrl Pts',(0.116426413159749,1.79948813090781,4.66328746718483));
#54266=CARTESIAN_POINT('Ctrl Pts',(0.113023060331444,1.7981835019318,4.6630607340252));
#54267=CARTESIAN_POINT('Ctrl Pts',(0.110681237370315,1.79731687559112,4.66290449843538));
#54268=CARTESIAN_POINT('Ctrl Pts',(0.100986540465924,1.79385675916467,4.66225668070163));
#54269=CARTESIAN_POINT('Ctrl Pts',(0.093551312552428,1.79150348360915,4.66175732456876));
#54270=CARTESIAN_POINT('Ctrl Pts',(0.0715980601253098,1.78542183067228,
4.66027533106316));
#54271=CARTESIAN_POINT('Ctrl Pts',(0.0568975592974022,1.78243379874549,
4.65927250163564));
#54272=CARTESIAN_POINT('Ctrl Pts',(0.0220662687796256,1.77785053960165,
4.65689884413128));
#54273=CARTESIAN_POINT('Ctrl Pts',(0.00188482287959766,1.77710102166971,
4.65552432948218));
#54274=CARTESIAN_POINT('Ctrl Pts',(-0.0193298806421376,1.77830335269784,
4.65415121043592));
#54275=CARTESIAN_POINT('Ctrl Pts',(-0.0204239669655363,1.77837096086944,
4.65408060692298));
#54276=CARTESIAN_POINT('Ctrl Pts',(-0.0248880044125756,1.77866968293866,
4.6537934517719));
#54277=CARTESIAN_POINT('Ctrl Pts',(-0.0282547203627233,1.77894819975883,
4.6535790181372));
#54278=CARTESIAN_POINT('Ctrl Pts',(-0.0321783322720964,1.77933498916711,
4.65333209109713));
#54279=CARTESIAN_POINT('Ctrl Pts',(-0.0327399281691189,1.7793918414088,
4.65329681918501));
#54280=CARTESIAN_POINT('Ctrl Pts',(-0.0335780185733662,1.7794789091958,
4.65324429105903));
#54281=CARTESIAN_POINT('Ctrl Pts',(-0.0338546242406436,1.77950800727545,
4.65322697233886));
#54282=CARTESIAN_POINT('Ctrl Pts',(-0.03434871986902,1.77956063144022,4.65319606846604));
#54283=CARTESIAN_POINT('Ctrl Pts',(-0.0345662233157622,1.77958402086294,
4.65318247560642));
#54284=CARTESIAN_POINT('Ctrl Pts',(-0.0350295433034604,1.77963432164187,
4.65315354438992));
#54285=CARTESIAN_POINT('Ctrl Pts',(-0.0352753520119601,1.77966129438462,
4.65313820959209));
#54286=CARTESIAN_POINT('Ctrl Pts',(-0.0359385536488279,1.77973484052807,
4.65309687371149));
#54287=CARTESIAN_POINT('Ctrl Pts',(-0.0363558887958978,1.77978194716013,
4.6530709027797));
#54288=CARTESIAN_POINT('Ctrl Pts',(-0.0383975142120484,1.78001643800371,
4.65294404529832));
#54289=CARTESIAN_POINT('Ctrl Pts',(-0.0400204918343865,1.78021537006362,
4.65284380076537));
#54290=CARTESIAN_POINT('Ctrl Pts',(-0.049325616557849,1.78142787200496,
4.65227214793176));
#54291=CARTESIAN_POINT('Ctrl Pts',(-0.0569713964816663,1.78270597476258,
4.6518145057367));
#54292=CARTESIAN_POINT('Ctrl Pts',(-0.0812282180897502,1.78766612484256,
4.65038024451293));
#54293=CARTESIAN_POINT('Ctrl Pts',(-0.0975973483235727,1.7923877288741,
4.64943805181323));
#54294=CARTESIAN_POINT('Ctrl Pts',(-0.122024625474658,1.80158120715939,
4.64797754801995));
#54295=CARTESIAN_POINT('Ctrl Pts',(-0.130391599172382,1.8051410389746,4.64746710085284));
#54296=CARTESIAN_POINT('Ctrl Pts',(-0.15237497237863,1.81561300539085,4.64607882133509));
#54297=CARTESIAN_POINT('Ctrl Pts',(-0.165667816522649,1.82314593541205,
4.64518785555756));
#54298=CARTESIAN_POINT('Ctrl Pts',(-0.17941734706603,1.83228344354583,4.64418482875963));
#54299=CARTESIAN_POINT('Ctrl Pts',(-0.18045466953299,1.83298155269204,4.64410863651903));
#54300=CARTESIAN_POINT('Ctrl Pts',(-0.181903857228763,1.83396914514694,
4.64400145070112));
#54301=CARTESIAN_POINT('Ctrl Pts',(-0.182319155955958,1.83425359009852,
4.64397064804889));
#54302=CARTESIAN_POINT('Ctrl Pts',(-0.183038048838936,1.83474845005943,
4.64391717769331));
#54303=CARTESIAN_POINT('Ctrl Pts',(-0.183341951638912,1.8349584167795,4.64389452706873));
#54304=CARTESIAN_POINT('Ctrl Pts',(-0.18396641346124,1.83539144598389,4.64384788783974));
#54305=CARTESIAN_POINT('Ctrl Pts',(-0.184286929253606,1.83561456953063,
4.64382389692861));
#54306=CARTESIAN_POINT('Ctrl Pts',(-0.185035784543128,1.83613790029041,
4.64376772094007));
#54307=CARTESIAN_POINT('Ctrl Pts',(-0.185463799363721,1.83643856817608,
4.64373551826451));
#54308=CARTESIAN_POINT('Ctrl Pts',(-0.186364826648522,1.83707479513318,
4.64366752627649));
#54309=CARTESIAN_POINT('Ctrl Pts',(-0.186837668654765,1.83741059135866,
4.64363172791377));
#54310=CARTESIAN_POINT('Ctrl Pts',(-0.188102954524015,1.83831430184366,
4.64353561749699));
#54311=CARTESIAN_POINT('Ctrl Pts',(-0.188893727364413,1.83888453540806,
4.64347521605263));
#54312=CARTESIAN_POINT('Ctrl Pts',(-0.191300675919869,1.8406368638681,4.64329033370659));
#54313=CARTESIAN_POINT('Ctrl Pts',(-0.192908409267721,1.84183042329919,
4.64316540885032));
#54314=CARTESIAN_POINT('Ctrl Pts',(-0.218547981896928,1.86123811387354,
4.64114973258302));
#54315=CARTESIAN_POINT('Ctrl Pts',(-0.239913090764258,1.88271828066298,
4.63911568429291));
#54316=CARTESIAN_POINT('Ctrl Pts',(-0.266864060205434,1.91871410395949,
4.63607667084967));
#54317=CARTESIAN_POINT('Ctrl Pts',(-0.274921624118765,1.93118296334252,
4.63508149240349));
#54318=CARTESIAN_POINT('Ctrl Pts',(-0.283702852571273,1.94707858855951,
4.63391632864756));
#54319=CARTESIAN_POINT('Ctrl Pts',(-0.28526802820553,1.95001859827816,4.63370495753369));
#54320=CARTESIAN_POINT('Ctrl Pts',(-0.287040612557722,1.95347638274788,
4.63346160636504));
#54321=CARTESIAN_POINT('Ctrl Pts',(-0.287292530313309,1.95397094225035,
4.63342692424446));
#54322=CARTESIAN_POINT('Ctrl Pts',(-0.287669637322058,1.95471602353945,
4.63337486265846));
#54323=CARTESIAN_POINT('Ctrl Pts',(-0.287795778063445,1.95496605851223,
4.63335742372047));
#54324=CARTESIAN_POINT('Ctrl Pts',(-0.28801996285247,1.95541187957668,4.63332638677494));
#54325=CARTESIAN_POINT('Ctrl Pts',(-0.288118133220805,1.95560760103276,
4.63331278079689));
#54326=CARTESIAN_POINT('Ctrl Pts',(-0.288326224425396,1.95602352794442,
4.63328390862952));
#54327=CARTESIAN_POINT('Ctrl Pts',(-0.288436092189978,1.9562437586742,4.63326864582177));
#54328=CARTESIAN_POINT('Ctrl Pts',(-0.288730431567737,1.956835459939,4.63322770477675));
#54329=CARTESIAN_POINT('Ctrl Pts',(-0.288914439332306,1.95720716266549,
4.63320205570511));
#54330=CARTESIAN_POINT('Ctrl Pts',(-0.289794484686172,1.95899355309227,
4.63307911712227));
#54331=CARTESIAN_POINT('Ctrl Pts',(-0.2904808675845,1.96041301196285,4.63298242273095));
#54332=CARTESIAN_POINT('Ctrl Pts',(-0.296113634762158,1.97228322572427,
4.6321815850503));
#54333=CARTESIAN_POINT('Ctrl Pts',(-0.300505323576294,1.98298943380868,
4.63150912491742));
#54334=CARTESIAN_POINT('Ctrl Pts',(-0.316198905427581,2.02800535365237,
4.62879278800612));
#54335=CARTESIAN_POINT('Ctrl Pts',(-0.322270110159706,2.06385104911035,
4.62685414642446));
#54336=CARTESIAN_POINT('Ctrl Pts',(-0.322274997047983,2.09995637979558,
4.62467682828221));
#54337=CARTESIAN_POINT('',(-0.322274981579892,2.09989103817067,4.37437734492394));
#54338=CARTESIAN_POINT('Ctrl Pts',(-0.322274997069199,2.09995653682505,
4.62467681881261));
#54339=CARTESIAN_POINT('Ctrl Pts',(-0.322275187530063,2.10136878465242,
4.62459165372713));
#54340=CARTESIAN_POINT('Ctrl Pts',(-0.32226609503044,2.10278100557306,4.62450620683319));
#54341=CARTESIAN_POINT('Ctrl Pts',(-0.322232983422061,2.10532569039139,
4.62435170814883));
#54342=CARTESIAN_POINT('Ctrl Pts',(-0.32221227553972,2.10645817494858,4.62428276038247));
#54343=CARTESIAN_POINT('Ctrl Pts',(-0.322173630227217,2.10809850660617,
4.62418261114945));
#54344=CARTESIAN_POINT('Ctrl Pts',(-0.322160460884536,2.10860646623495,
4.6241515587642));
#54345=CARTESIAN_POINT('Ctrl Pts',(-0.322135120840432,2.10950210443448,
4.62409673688665));
#54346=CARTESIAN_POINT('Ctrl Pts',(-0.322123451457929,2.10988979708164,
4.62407298312027));
#54347=CARTESIAN_POINT('Ctrl Pts',(-0.322099172786788,2.11065072674517,
4.62402631543877));
#54348=CARTESIAN_POINT('Ctrl Pts',(-0.322086614572444,2.11102396487159,
4.62400340315945));
#54349=CARTESIAN_POINT('Ctrl Pts',(-0.322060358722216,2.11176593015203,
4.62395781214256));
#54350=CARTESIAN_POINT('Ctrl Pts',(-0.322046676527055,2.11213465733939,
4.6239351339217));
#54351=CARTESIAN_POINT('Ctrl Pts',(-0.322012892473588,2.11300478819637,
4.62388156669676));
#54352=CARTESIAN_POINT('Ctrl Pts',(-0.321992252750884,2.11350616892771,
4.62385066087302));
#54353=CARTESIAN_POINT('Ctrl Pts',(-0.321916489087427,2.11524764065199,
4.62374317488986));
#54354=CARTESIAN_POINT('Ctrl Pts',(-0.321855371998147,2.11648744791126,
4.62366640705546));
#54355=CARTESIAN_POINT('Ctrl Pts',(-0.321651256538203,2.12019265743169,
4.62343623491896));
#54356=CARTESIAN_POINT('Ctrl Pts',(-0.321487083791414,2.12265675738753,
4.62328216975928));
#54357=CARTESIAN_POINT('Ctrl Pts',(-0.318546131365999,2.16027467452957,
4.62091450096085));
#54358=CARTESIAN_POINT('Ctrl Pts',(-0.310045951090214,2.19473598291975,
4.61849722897432));
#54359=CARTESIAN_POINT('Ctrl Pts',(-0.29159527079729,2.2377182288673,4.61536523362758));
#54360=CARTESIAN_POINT('Ctrl Pts',(-0.286481409072725,2.24806274287713,
4.61460517481756));
#54361=CARTESIAN_POINT('Ctrl Pts',(-0.28005108146272,2.25948368493022,4.61377588403408));
#54362=CARTESIAN_POINT('Ctrl Pts',(-0.279268660410145,2.26084983537447,
4.61367685685382));
#54363=CARTESIAN_POINT('Ctrl Pts',(-0.278267592175472,2.26256843055088,
4.61355255255379));
#54364=CARTESIAN_POINT('Ctrl Pts',(-0.27805825091827,2.26292623044731,4.61352668813877));
#54365=CARTESIAN_POINT('Ctrl Pts',(-0.277723546463401,2.2634957733816,4.61348554238852));
#54366=CARTESIAN_POINT('Ctrl Pts',(-0.277598631012643,2.26370777695252,
4.61347023205442));
#54367=CARTESIAN_POINT('Ctrl Pts',(-0.277362094851295,2.26410817138233,
4.61344132741317));
#54368=CARTESIAN_POINT('Ctrl Pts',(-0.277250525864528,2.2642965899917,4.61342772995435));
#54369=CARTESIAN_POINT('Ctrl Pts',(-0.276995786057336,2.26472579824611,
4.61339676581713));
#54370=CARTESIAN_POINT('Ctrl Pts',(-0.27685249350869,2.26496651460459,4.61337940724632));
#54371=CARTESIAN_POINT('Ctrl Pts',(-0.276424168679889,2.26568392521232,
4.61332769407639));
#54372=CARTESIAN_POINT('Ctrl Pts',(-0.276138215920658,2.26616007289104,
4.61329339937088));
#54373=CARTESIAN_POINT('Ctrl Pts',(-0.274125147743464,2.26949253799383,
4.61305355308458));
#54374=CARTESIAN_POINT('Ctrl Pts',(-0.272354899408359,2.27232274355462,
4.61285076224998));
#54375=CARTESIAN_POINT('Ctrl Pts',(-0.262479003959397,2.28757946177137,
4.61175965348516));
#54376=CARTESIAN_POINT('Ctrl Pts',(-0.253565700416985,2.29946383299502,
4.61091687257788));
#54377=CARTESIAN_POINT('Ctrl Pts',(-0.224126862767211,2.33353750605077,
4.60838825886458));
#54378=CARTESIAN_POINT('Ctrl Pts',(-0.201280413452453,2.35349289627581,
4.60672957473035));
#54379=CARTESIAN_POINT('Ctrl Pts',(-0.174341401341979,2.37105374395786,
4.6047957642201));
#54380=CARTESIAN_POINT('Ctrl Pts',(-0.172681322207265,2.37211434551246,
4.60467675632164));
#54381=CARTESIAN_POINT('Ctrl Pts',(-0.17019517415967,2.37367079901421,4.6044987185447));
#54382=CARTESIAN_POINT('Ctrl Pts',(-0.169376416229719,2.37417828713108,
4.60444011605323));
#54383=CARTESIAN_POINT('Ctrl Pts',(-0.16806520488208,2.37498289639412,4.6043463091766));
#54384=CARTESIAN_POINT('Ctrl Pts',(-0.167574205708521,2.37528238587998,
4.60431119159643));
#54385=CARTESIAN_POINT('Ctrl Pts',(-0.166638219094032,2.37584986749199,
4.60424426419851));
#54386=CARTESIAN_POINT('Ctrl Pts',(-0.166193379814277,2.37611810146945,
4.60421246334414));
#54387=CARTESIAN_POINT('Ctrl Pts',(-0.165413510654871,2.37658578803669,
4.60415672354022));
#54388=CARTESIAN_POINT('Ctrl Pts',(-0.165078762823075,2.37678571081919,
4.60413280181023));
#54389=CARTESIAN_POINT('Ctrl Pts',(-0.164425417875467,2.3771743037915,4.6040861195305));
#54390=CARTESIAN_POINT('Ctrl Pts',(-0.164106856655065,2.37736303344685,
4.60406336119257));
#54391=CARTESIAN_POINT('Ctrl Pts',(-0.163351497476454,2.37780878450867,
4.60400940486667));
#54392=CARTESIAN_POINT('Ctrl Pts',(-0.162914418063582,2.37806532480751,
4.60397818946346));
#54393=CARTESIAN_POINT('Ctrl Pts',(-0.161379668751497,2.37896127305236,
4.60386859936239));
#54394=CARTESIAN_POINT('Ctrl Pts',(-0.160278835930207,2.37959521460155,
4.6037900271237));
#54395=CARTESIAN_POINT('Ctrl Pts',(-0.144586359620438,2.38850898051737,
4.60267037159344));
#54396=CARTESIAN_POINT('Ctrl Pts',(-0.12937612332373,2.39564218873458,4.60158790867995));
#54397=CARTESIAN_POINT('Ctrl Pts',(-0.106102971298018,2.40441573548338,
4.59993711829214));
#54398=CARTESIAN_POINT('Ctrl Pts',(-0.0984192432931792,2.40698603034381,
4.59939331988942));
#54399=CARTESIAN_POINT('Ctrl Pts',(-0.0805222913351933,2.41223173500415,
4.59813452148875));
#54400=CARTESIAN_POINT('Ctrl Pts',(-0.0702577968750717,2.41470039527728,
4.59741815471573));
#54401=CARTESIAN_POINT('Ctrl Pts',(-0.0456798702669214,2.41934886356838,
4.59573493947132));
#54402=CARTESIAN_POINT('Ctrl Pts',(-0.0313022276549956,2.42107729352348,
4.59477528233938));
#54403=CARTESIAN_POINT('Ctrl Pts',(-0.0158851986191007,2.42188473097346,
4.59380395953406));
#54404=CARTESIAN_POINT('Ctrl Pts',(-0.0149147208572632,2.42193115836829,
4.59374306185069));
#54405=CARTESIAN_POINT('Ctrl Pts',(-0.013597795183024,2.42198819185932,
4.59366077112828));
#54406=CARTESIAN_POINT('Ctrl Pts',(-0.0132515311714041,2.42200262833551,
4.59363916663381));
#54407=CARTESIAN_POINT('Ctrl Pts',(-0.0126744555465138,2.42202575541378,
4.59360321600057));
#54408=CARTESIAN_POINT('Ctrl Pts',(-0.012443657731343,2.42203475644143,
4.59358885240479));
#54409=CARTESIAN_POINT('Ctrl Pts',(-0.0119906035835674,2.42205193760481,
4.59356068578388));
#54410=CARTESIAN_POINT('Ctrl Pts',(-0.0117683485032361,2.42206013578722,
4.5935468817782));
#54411=CARTESIAN_POINT('Ctrl Pts',(-0.0112795133407785,2.4220776604413,
4.59351655061084));
#54412=CARTESIAN_POINT('Ctrl Pts',(-0.0110129292292425,2.42208688605334,
4.59350002914122));
#54413=CARTESIAN_POINT('Ctrl Pts',(-0.0100878985711194,2.42211774857295,
4.5934427673555));
#54414=CARTESIAN_POINT('Ctrl Pts',(-0.00942939163363354,2.42213769763063,
4.59340212134454));
#54415=CARTESIAN_POINT('Ctrl Pts',(-0.00293933082998487,2.42231439224278,
4.59300264061024));
#54416=CARTESIAN_POINT('Ctrl Pts',(0.00289584677027582,2.42231480201296,
4.5926523374891));
#54417=CARTESIAN_POINT('Ctrl Pts',(0.0377133692223503,2.42137148476953,
4.59059807276249));
#54418=CARTESIAN_POINT('Ctrl Pts',(0.0664627189404521,2.41667813564588,
4.58903984646069));
#54419=CARTESIAN_POINT('Ctrl Pts',(0.101267702356863,2.40604029852649,4.58696676273227));
#54420=CARTESIAN_POINT('Ctrl Pts',(0.108259755867507,2.40363732871762,4.58654103316248));
#54421=CARTESIAN_POINT('Ctrl Pts',(0.120500130013859,2.39895409747222,4.58577381460868));
#54422=CARTESIAN_POINT('Ctrl Pts',(0.125782010324904,2.39677047322707,4.58543527649251));
#54423=CARTESIAN_POINT('Ctrl Pts',(0.132939740478171,2.39358592488311,4.58496475094986));
#54424=CARTESIAN_POINT('Ctrl Pts',(0.134868069820154,2.39270509613726,4.58483679810572));
#54425=CARTESIAN_POINT('Ctrl Pts',(0.137708281537022,2.39137371001142,4.58464650784085));
#54426=CARTESIAN_POINT('Ctrl Pts',(0.138626972506996,2.39093774616984,4.584584670991));
#54427=CARTESIAN_POINT('Ctrl Pts',(0.140081926274201,2.39023884345766,4.58448627741105));
#54428=CARTESIAN_POINT('Ctrl Pts',(0.140619553124763,2.38997874679325,4.58444981912336));
#54429=CARTESIAN_POINT('Ctrl Pts',(0.141637797910818,2.38948263596219,4.58438057640223));
#54430=CARTESIAN_POINT('Ctrl Pts',(0.142118557249825,2.38924691528244,4.58434780225779));
#54431=CARTESIAN_POINT('Ctrl Pts',(0.142950862924263,2.38883625223199,4.58429092024555));
#54432=CARTESIAN_POINT('Ctrl Pts',(0.143302682127653,2.38866186292447,4.58426683174087));
#54433=CARTESIAN_POINT('Ctrl Pts',(0.14398216390915,2.38832350987764,4.58422022273971));
#54434=CARTESIAN_POINT('Ctrl Pts',(0.14430986749189,2.38815962939814,4.58419770518633));
#54435=CARTESIAN_POINT('Ctrl Pts',(0.145076569375989,2.38777457545933,4.58414493149331));
#54436=CARTESIAN_POINT('Ctrl Pts',(0.145515341620354,2.38755295618641,4.58411465973887));
#54437=CARTESIAN_POINT('Ctrl Pts',(0.147031208403229,2.38678294970945,4.58400983302295));
#54438=CARTESIAN_POINT('Ctrl Pts',(0.148105713754767,2.3862295127654,4.58393510054501));
#54439=CARTESIAN_POINT('Ctrl Pts',(0.160238942053434,2.37989353379258,4.58308632162054));
#54440=CARTESIAN_POINT('Ctrl Pts',(0.170954556217832,2.37348012732697,4.58228975546083));
#54441=CARTESIAN_POINT('Ctrl Pts',(0.194569085765799,2.35741551657576,4.58042121090629));
#54442=CARTESIAN_POINT('Ctrl Pts',(0.207170680760043,2.34738653331393,4.57933814398522));
#54443=CARTESIAN_POINT('Ctrl Pts',(0.223237535552025,2.33250808194978,4.57785638931334));
#54444=CARTESIAN_POINT('Ctrl Pts',(0.227397372423332,2.32844133047175,4.57746259728413));
#54445=CARTESIAN_POINT('Ctrl Pts',(0.234344543051893,2.32127171913313,4.5767894830817));
#54446=CARTESIAN_POINT('Ctrl Pts',(0.237185938327672,2.31822321284495,4.57650943546035));
#54447=CARTESIAN_POINT('Ctrl Pts',(0.247158038847169,2.30709930416308,4.57551141629466));
#54448=CARTESIAN_POINT('Ctrl Pts',(0.253942762687946,2.29872177298631,4.57480334133327));
#54449=CARTESIAN_POINT('Ctrl Pts',(0.261189986599597,2.28879424474817,4.5740260321682));
#54450=CARTESIAN_POINT('Ctrl Pts',(0.262075612528277,2.28756292139651,4.57393065804701));
#54451=CARTESIAN_POINT('Ctrl Pts',(0.263189102947726,2.28599150287744,4.5738102988537));
#54452=CARTESIAN_POINT('Ctrl Pts',(0.26342503834332,2.28565719008773,4.57378477035259));
#54453=CARTESIAN_POINT('Ctrl Pts',(0.263801145807956,2.2851220976922,4.57374403487827));
#54454=CARTESIAN_POINT('Ctrl Pts',(0.263941725881553,2.28492160750756,4.57372879989495));
#54455=CARTESIAN_POINT('Ctrl Pts',(0.264207721919452,2.28454133237403,4.57369995646709));
#54456=CARTESIAN_POINT('Ctrl Pts',(0.264333181912522,2.28436158118365,4.57368634505427));
#54457=CARTESIAN_POINT('Ctrl Pts',(0.26461973645995,2.28395013002444,4.57365523971034));
#54458=CARTESIAN_POINT('Ctrl Pts',(0.264780709897111,2.28371834673756,4.57363775416373));
#54459=CARTESIAN_POINT('Ctrl Pts',(0.265274374010635,2.28300553049639,4.57358409266247));
#54460=CARTESIAN_POINT('Ctrl Pts',(0.265606062165876,2.28252379968764,4.57354798503256));
#54461=CARTESIAN_POINT('Ctrl Pts',(0.268084063511809,2.27890378956677,4.57327780876737));
#54462=CARTESIAN_POINT('Ctrl Pts',(0.270176114122937,2.27572848792521,4.57304733335643));
#54463=CARTESIAN_POINT('Ctrl Pts',(0.285609168738636,2.25137690133295,4.57132259907083));
#54464=CARTESIAN_POINT('Ctrl Pts',(0.296500475998486,2.22874542623796,4.56995645758664));
#54465=CARTESIAN_POINT('Ctrl Pts',(0.311093954214909,2.18643339276941,4.56744356382087));
#54466=CARTESIAN_POINT('Ctrl Pts',(0.315798718087328,2.16723981550127,4.56631753744043));
#54467=CARTESIAN_POINT('Ctrl Pts',(0.318992085717201,2.14591956323552,4.56501967609921));
#54468=CARTESIAN_POINT('Ctrl Pts',(0.319248899449333,2.1440987190766,4.56490849628523));
#54469=CARTESIAN_POINT('Ctrl Pts',(0.31961022762356,2.14136806075941,4.56474122114416));
#54470=CARTESIAN_POINT('Ctrl Pts',(0.319726472657586,2.14045981596039,4.5646854940741));
#54471=CARTESIAN_POINT('Ctrl Pts',(0.319906999619618,2.13899994400357,4.56459577232617));
#54472=CARTESIAN_POINT('Ctrl Pts',(0.319973729609344,2.13844862015373,4.56456185471717));
#54473=CARTESIAN_POINT('Ctrl Pts',(0.32009838123621,2.1373959444762,4.56449702778116));
#54474=CARTESIAN_POINT('Ctrl Pts',(0.320156550933138,2.13689462323059,4.56446612635752));
#54475=CARTESIAN_POINT('Ctrl Pts',(0.32025731941996,2.13600798888557,4.56441142301896));
#54476=CARTESIAN_POINT('Ctrl Pts',(0.320300401116058,2.13562273078256,4.56438763637306));
#54477=CARTESIAN_POINT('Ctrl Pts',(0.320383726791296,2.13486521799335,4.56434083198357));
#54478=CARTESIAN_POINT('Ctrl Pts',(0.320424017374704,2.13449296893601,4.56431781574675));
#54479=CARTESIAN_POINT('Ctrl Pts',(0.320518986771833,2.13360100940536,4.56426262672786));
#54480=CARTESIAN_POINT('Ctrl Pts',(0.3205730502568,2.13308123574199,4.56423043461548));
#54481=CARTESIAN_POINT('Ctrl Pts',(0.320733701462322,2.13149933104821,4.564132361899));
#54482=CARTESIAN_POINT('Ctrl Pts',(0.320836275679614,2.13043680788569,4.56406635515123));
#54483=CARTESIAN_POINT('Ctrl Pts',(0.321923602454403,2.11855684670442,4.56332680818932));
#54484=CARTESIAN_POINT('Ctrl Pts',(0.322366031817001,2.1076979461868,4.5626362645731));
#54485=CARTESIAN_POINT('Ctrl Pts',(0.321975340975053,2.06787519781979,4.56004703924851));
#54486=CARTESIAN_POINT('Ctrl Pts',(0.317787518208194,2.03908385862853,4.55805023089022));
#54487=CARTESIAN_POINT('Ctrl Pts',(0.307144261411345,2.00193127254364,4.55547810368107));
#54488=CARTESIAN_POINT('Ctrl Pts',(0.304056578824144,1.99273999194857,4.55484387331992));
#54489=CARTESIAN_POINT('Ctrl Pts',(0.300043891779038,1.98236974819069,4.55414123143897));
#54490=CARTESIAN_POINT('Ctrl Pts',(0.299519932477342,1.98104192602815,4.55405151534968));
#54491=CARTESIAN_POINT('Ctrl Pts',(0.298837680397546,1.97934604525443,4.55393729392506));
#54492=CARTESIAN_POINT('Ctrl Pts',(0.298687510632921,1.97897476702282,4.55391230986944));
#54493=CARTESIAN_POINT('Ctrl Pts',(0.29844514215234,1.97837873638653,4.55387223888141));
#54494=CARTESIAN_POINT('Ctrl Pts',(0.298353381346516,1.97815380811325,4.55385712551486));
#54495=CARTESIAN_POINT('Ctrl Pts',(0.298178157377616,1.97772567585418,4.55382837498));
#54496=CARTESIAN_POINT('Ctrl Pts',(0.298094741464879,1.97752245514518,4.55381473514727));
#54497=CARTESIAN_POINT('Ctrl Pts',(0.297904112858937,1.97705938758681,4.55378367084896));
#54498=CARTESIAN_POINT('Ctrl Pts',(0.297796768091028,1.97679959596341,4.55376625454502));
#54499=CARTESIAN_POINT('Ctrl Pts',(0.297461283843121,1.97599067037787,4.5537120593778));
#54500=CARTESIAN_POINT('Ctrl Pts',(0.29723196268716,1.97544202318043,4.553675351975));
#54501=CARTESIAN_POINT('Ctrl Pts',(0.295439620695161,1.9711870104725,4.55339103449133));
#54502=CARTESIAN_POINT('Ctrl Pts',(0.293808765264527,1.96750936326479,4.55314745171547));
#54503=CARTESIAN_POINT('Ctrl Pts',(0.285988003195334,1.95072833928226,4.55204168513106));
#54504=CARTESIAN_POINT('Ctrl Pts',(0.278986976188894,1.93801998498287,4.55122006229704));
#54505=CARTESIAN_POINT('Ctrl Pts',(0.254900776914848,1.90052289926077,4.54871910649744));
#54506=CARTESIAN_POINT('Ctrl Pts',(0.235189227775424,1.87762336639573,4.54706431017389));
#54507=CARTESIAN_POINT('Ctrl Pts',(0.211223847348802,1.85658889443726,4.54514425815119));
#54508=CARTESIAN_POINT('Ctrl Pts',(0.209847550212254,1.85540137886105,4.54503433727265));
#54509=CARTESIAN_POINT('Ctrl Pts',(0.207768880582198,1.85363828979879,4.54486879580796));
#54510=CARTESIAN_POINT('Ctrl Pts',(0.20707398633711,1.8530539246155,4.54481353435915));
#54511=CARTESIAN_POINT('Ctrl Pts',(0.205952554088424,1.85211892779933,4.54472447403346));
#54512=CARTESIAN_POINT('Ctrl Pts',(0.20552756483114,1.85176643945768,4.54469075069432));
#54513=CARTESIAN_POINT('Ctrl Pts',(0.204713720689455,1.85109495555024,4.54462622330877));
#54514=CARTESIAN_POINT('Ctrl Pts',(0.204325020442008,1.85077577443616,4.54459542690181));
#54515=CARTESIAN_POINT('Ctrl Pts',(0.203635702488499,1.85021243769995,4.54454085184358));
#54516=CARTESIAN_POINT('Ctrl Pts',(0.203335388177042,1.8499679110183,4.54451708824976));
#54517=CARTESIAN_POINT('Ctrl Pts',(0.20274315640915,1.84948746732515,4.54447025080113));
#54518=CARTESIAN_POINT('Ctrl Pts',(0.202451266054904,1.84925151771381,4.54444717831058));
#54519=CARTESIAN_POINT('Ctrl Pts',(0.201749397842952,1.84868618687107,4.54439172760249));
#54520=CARTESIAN_POINT('Ctrl Pts',(0.201339025612784,1.84835729901414,4.54435932964721));
#54521=CARTESIAN_POINT('Ctrl Pts',(0.19984501305444,1.84716593479695,4.54424146359948));
#54522=CARTESIAN_POINT('Ctrl Pts',(0.198756632859906,1.84630945116549,4.54415575655851));
#54523=CARTESIAN_POINT('Ctrl Pts',(0.180772483103976,1.83234387677761,4.54274201784886));
#54524=CARTESIAN_POINT('Ctrl Pts',(0.162622125117904,1.82094407394239,4.5413452554332));
#54525=CARTESIAN_POINT('Ctrl Pts',(0.129714878429536,1.80458240197122,4.53887761804258));
#54526=CARTESIAN_POINT('Ctrl Pts',(0.115477669790181,1.79873200633156,4.5378300129434));
#54527=CARTESIAN_POINT('Ctrl Pts',(0.0915294864427441,1.79083919181348,
4.53613860571807));
#54528=CARTESIAN_POINT('Ctrl Pts',(0.0820444181801044,1.78818787806282,
4.53548629660424));
#54529=CARTESIAN_POINT('Ctrl Pts',(0.0687877575405258,1.78512929270441,
4.53461122360926));
#54530=CARTESIAN_POINT('Ctrl Pts',(0.0651086824127195,1.78434800739767,
4.53437220990488));
#54531=CARTESIAN_POINT('Ctrl Pts',(0.0608912901534426,1.78352928612848,
4.53410324614969));
#54532=CARTESIAN_POINT('Ctrl Pts',(0.0603657410783373,1.78342861899918,
4.53406981803239));
#54533=CARTESIAN_POINT('Ctrl Pts',(0.0595725244416208,1.78327872818386,
4.53401950093834));
#54534=CARTESIAN_POINT('Ctrl Pts',(0.0593050445592811,1.78322853446007,
4.53400255691538));
#54535=CARTESIAN_POINT('Ctrl Pts',(0.0588229788532426,1.78313870479148,
4.53397206202357));
#54536=CARTESIAN_POINT('Ctrl Pts',(0.058608416822605,1.78309894805966,4.53395850426682));
#54537=CARTESIAN_POINT('Ctrl Pts',(0.0581466913976274,1.78301387877959,
4.53392936144607));
#54538=CARTESIAN_POINT('Ctrl Pts',(0.0578995160846108,1.78296863750561,
4.53391378053407));
#54539=CARTESIAN_POINT('Ctrl Pts',(0.0572323372415175,1.782847327952,4.53387177795912));
#54540=CARTESIAN_POINT('Ctrl Pts',(0.0568122332340528,1.78277180457398,
4.53384538742762));
#54541=CARTESIAN_POINT('Ctrl Pts',(0.0548649124117083,1.78242572113924,
4.53372331894553));
#54542=CARTESIAN_POINT('Ctrl Pts',(0.0533358720597281,1.7821653477266,4.53362821210427));
#54543=CARTESIAN_POINT('Ctrl Pts',(0.0204327649374402,1.77680655960813,
4.53159639272886));
#54544=CARTESIAN_POINT('Ctrl Pts',(-0.0115285967771731,1.77636535368129,
4.52989783877908));
#54545=CARTESIAN_POINT('Ctrl Pts',(-0.055322460813225,1.782267164628,4.52739423577715));
#54546=CARTESIAN_POINT('Ctrl Pts',(-0.0674963361952112,1.78462890314258,
4.52668068021975));
#54547=CARTESIAN_POINT('Ctrl Pts',(-0.0849204757361831,1.78906441778081,
4.52561362809984));
#54548=CARTESIAN_POINT('Ctrl Pts',(-0.0903006157187279,1.79058407210571,
4.52527773327316));
#54549=CARTESIAN_POINT('Ctrl Pts',(-0.0965119185732252,1.79251428951246,
4.5248815070195));
#54550=CARTESIAN_POINT('Ctrl Pts',(-0.0973843920833234,1.79278949768575,
4.52482565573068));
#54551=CARTESIAN_POINT('Ctrl Pts',(-0.0987121433231434,1.7932145405961,
4.52474035793878));
#54552=CARTESIAN_POINT('Ctrl Pts',(-0.0991682831903105,1.79336168382565,
4.52471100000876));
#54553=CARTESIAN_POINT('Ctrl Pts',(-0.0999601383356593,1.79361907496038,
4.52465993957367));
#54554=CARTESIAN_POINT('Ctrl Pts',(-0.100296004564026,1.7937288587687,4.52463825239425));
#54555=CARTESIAN_POINT('Ctrl Pts',(-0.100994954344315,1.7939585958718,4.52459305813245));
#54556=CARTESIAN_POINT('Ctrl Pts',(-0.101358006145582,1.7940786433869,4.52456954796843));
#54557=CARTESIAN_POINT('Ctrl Pts',(-0.102244476148977,1.79437351676707,
4.52451205644772));
#54558=CARTESIAN_POINT('Ctrl Pts',(-0.10276765921128,1.79454904097303,4.5244780520548));
#54559=CARTESIAN_POINT('Ctrl Pts',(-0.104760965577773,1.79522348203908,
4.52434821375438));
#54560=CARTESIAN_POINT('Ctrl Pts',(-0.1062279091361,1.79573166941937,4.5242520733434));
#54561=CARTESIAN_POINT('Ctrl Pts',(-0.130484381856795,1.80433153773056,
4.52265242544909));
#54562=CARTESIAN_POINT('Ctrl Pts',(-0.152290713152085,1.81495072102985,
4.52105963881474));
#54563=CARTESIAN_POINT('Ctrl Pts',(-0.184708505815811,1.83552652170552,
4.51846897725457));
#54564=CARTESIAN_POINT('Ctrl Pts',(-0.196198824550928,1.84393460792379,
4.51750103030015));
#54565=CARTESIAN_POINT('Ctrl Pts',(-0.215112060873255,1.85979711464196,
4.51585364986379));
#54566=CARTESIAN_POINT('Ctrl Pts',(-0.22279666352885,1.86690705752968,4.51516680767203));
#54567=CARTESIAN_POINT('Ctrl Pts',(-0.230812284088111,1.87508260176963,
4.51444289900769));
#54568=CARTESIAN_POINT('Ctrl Pts',(-0.231498886629132,1.87578935783409,
4.514380828236));
#54569=CARTESIAN_POINT('Ctrl Pts',(-0.232681906574711,1.8770183301956,4.51427378975466));
#54570=CARTESIAN_POINT('Ctrl Pts',(-0.233179829686016,1.87753907811186,
4.51422871017536));
#54571=CARTESIAN_POINT('Ctrl Pts',(-0.233887663234675,1.87828434635492,
4.51416459206058));
#54572=CARTESIAN_POINT('Ctrl Pts',(-0.234099000715582,1.87850749911003,
4.51414544396624));
#54573=CARTESIAN_POINT('Ctrl Pts',(-0.234463158984647,1.87889311984239,
4.51411244261688));
#54574=CARTESIAN_POINT('Ctrl Pts',(-0.234616130666335,1.87905544449699,
4.51409857762197));
#54575=CARTESIAN_POINT('Ctrl Pts',(-0.234910064101439,1.87936799904045,
4.51407193226462));
#54576=CARTESIAN_POINT('Ctrl Pts',(-0.235051050040951,1.87951820497192,
4.5140591499858));
#54577=CARTESIAN_POINT('Ctrl Pts',(-0.235384741871708,1.87987440292686,
4.5140288918353));
#54578=CARTESIAN_POINT('Ctrl Pts',(-0.235577321912191,1.88008051338068,
4.51401142571908));
#54579=CARTESIAN_POINT('Ctrl Pts',(-0.236250706344075,1.88080310836149,
4.51395033929737));
#54580=CARTESIAN_POINT('Ctrl Pts',(-0.236730089302662,1.88132092374223,
4.51390682752149));
#54581=CARTESIAN_POINT('Ctrl Pts',(-0.242925121458277,1.88805686023063,
4.51334414602258));
#54582=CARTESIAN_POINT('Ctrl Pts',(-0.2483964780876,1.89449640429394,4.51284294273553));
#54583=CARTESIAN_POINT('Ctrl Pts',(-0.269186200550787,1.92101038419349,
4.51088651071572));
#54584=CARTESIAN_POINT('Ctrl Pts',(-0.282376156885098,1.94263926276705,
4.50951674486301));
#54585=CARTESIAN_POINT('Ctrl Pts',(-0.297782674136048,1.97621260265667,
4.50741908689142));
#54586=CARTESIAN_POINT('Ctrl Pts',(-0.302076273279367,1.98709416902304,
4.50674429327485));
#54587=CARTESIAN_POINT('Ctrl Pts',(-0.307496400373257,2.00337167708153,
4.50572550675659));
#54588=CARTESIAN_POINT('Ctrl Pts',(-0.309091358748421,2.00860199404576,
4.5053968543759));
#54589=CARTESIAN_POINT('Ctrl Pts',(-0.310795565517467,2.01474673239587,
4.50500838373934));
#54590=CARTESIAN_POINT('Ctrl Pts',(-0.311034973908767,2.0156243627495,4.50495284492084));
#54591=CARTESIAN_POINT('Ctrl Pts',(-0.311394568008039,2.01696490285246,
4.50486792407217));
#54592=CARTESIAN_POINT('Ctrl Pts',(-0.311517445796499,2.01742709098192,
4.50483862937747));
#54593=CARTESIAN_POINT('Ctrl Pts',(-0.311729305006143,2.01823117442838,
4.50478763621584));
#54594=CARTESIAN_POINT('Ctrl Pts',(-0.311818754102739,2.01857294661352,
4.50476595293384));
#54595=CARTESIAN_POINT('Ctrl Pts',(-0.312004001758485,2.01928553294174,
4.50472072509327));
#54596=CARTESIAN_POINT('Ctrl Pts',(-0.312099701600884,2.01965637197343,
4.5046971773791));
#54597=CARTESIAN_POINT('Ctrl Pts',(-0.31233218626508,2.02056393869788,4.50463952201286));
#54598=CARTESIAN_POINT('Ctrl Pts',(-0.312468248508577,2.02110084867259,
4.50460539106698));
#54599=CARTESIAN_POINT('Ctrl Pts',(-0.312983662586338,2.02315694936466,
4.50447459862682));
#54600=CARTESIAN_POINT('Ctrl Pts',(-0.3133533198935,2.02467852729999,4.50437762494992));
#54601=CARTESIAN_POINT('Ctrl Pts',(-0.319425494415398,2.05049130998662,
4.50272925164632));
#54602=CARTESIAN_POINT('Ctrl Pts',(-0.322297879207263,2.07535592345029,
4.50108236478238));
#54603=CARTESIAN_POINT('Ctrl Pts',(-0.322252709050149,2.12430402355982,
4.49777687468305));
#54604=CARTESIAN_POINT('Ctrl Pts',(-0.319548251603004,2.14823505406213,
4.49613367791463));
#54605=CARTESIAN_POINT('Ctrl Pts',(-0.313902454782349,2.17299549645883,
4.49452912794629));
#54606=CARTESIAN_POINT('Ctrl Pts',(-0.31358586537667,2.17434378805043,4.49444208125366));
#54607=CARTESIAN_POINT('Ctrl Pts',(-0.313163453274868,2.17609203773674,
4.49432967518207));
#54608=CARTESIAN_POINT('Ctrl Pts',(-0.313065544632058,2.17649386539296,
4.49430387092083));
#54609=CARTESIAN_POINT('Ctrl Pts',(-0.312914051216105,2.17711044783589,
4.49426432571514));
#54610=CARTESIAN_POINT('Ctrl Pts',(-0.312861018745365,2.17732533584948,
4.49425055296658));
#54611=CARTESIAN_POINT('Ctrl Pts',(-0.312755303230623,2.17775180685073,
4.49422323806932));
#54612=CARTESIAN_POINT('Ctrl Pts',(-0.312702627192136,2.17796338958157,
4.49420969569517));
#54613=CARTESIAN_POINT('Ctrl Pts',(-0.312584755136581,2.1784348024938,4.49417954329042));
#54614=CARTESIAN_POINT('Ctrl Pts',(-0.31251945003005,2.17869460426357,4.4941629397082));
#54615=CARTESIAN_POINT('Ctrl Pts',(-0.312327854277337,2.17945282523058,
4.4941145223147));
#54616=CARTESIAN_POINT('Ctrl Pts',(-0.312200693939053,2.1799510269304,4.49408275870935));
#54617=CARTESIAN_POINT('Ctrl Pts',(-0.31127472970468,2.18354296829767,4.49385409476724));
#54618=CARTESIAN_POINT('Ctrl Pts',(-0.310431112203309,2.18662511963994,
4.49365973584894));
#54619=CARTESIAN_POINT('Ctrl Pts',(-0.307942611817073,2.19521311597016,
4.49312207033707));
#54620=CARTESIAN_POINT('Ctrl Pts',(-0.306196062322751,2.20068847643272,
4.49278378386813));
#54621=CARTESIAN_POINT('Ctrl Pts',(-0.301532736499007,2.21406146455074,
4.49196212952329));
#54622=CARTESIAN_POINT('Ctrl Pts',(-0.298451155384507,2.22189721584668,
4.49148466461904));
#54623=CARTESIAN_POINT('Ctrl Pts',(-0.28515399750154,2.25217059518616,4.48962451458178));
#54624=CARTESIAN_POINT('Ctrl Pts',(-0.272686498978403,2.2735243920923,4.48827108571912));
#54625=CARTESIAN_POINT('Ctrl Pts',(-0.256379259867567,2.29528785044138,
4.48668170716075));
#54626=CARTESIAN_POINT('Ctrl Pts',(-0.254827101037764,2.29730893924557,
4.48653199021396));
#54627=CARTESIAN_POINT('Ctrl Pts',(-0.249302626687654,2.30432850648377,
4.48600415617149));
#54628=CARTESIAN_POINT('Ctrl Pts',(-0.245206098789032,2.30922690733415,
4.4856216105108));
#54629=CARTESIAN_POINT('Ctrl Pts',(-0.240284634971525,2.3147685401397,4.48517050701104));
#54630=CARTESIAN_POINT('Ctrl Pts',(-0.239598596882237,2.31553362607924,
4.48510780838867));
#54631=CARTESIAN_POINT('Ctrl Pts',(-0.238571596637828,2.316667998351,4.48501421506202));
#54632=CARTESIAN_POINT('Ctrl Pts',(-0.238233406189017,2.3170397945143,4.4849834374572));
#54633=CARTESIAN_POINT('Ctrl Pts',(-0.237629043917199,2.31770109731778,
4.48492851142747));
#54634=CARTESIAN_POINT('Ctrl Pts',(-0.237363208713023,2.31799091135561,
4.48490437732318));
#54635=CARTESIAN_POINT('Ctrl Pts',(-0.236801991521736,2.31860050765711,
4.48485348030516));
#54636=CARTESIAN_POINT('Ctrl Pts',(-0.236506490945261,2.31892017923071,
4.48482671236027));
#54637=CARTESIAN_POINT('Ctrl Pts',(-0.23572498777887,2.31976217778918,4.48475600111385));
#54638=CARTESIAN_POINT('Ctrl Pts',(-0.235237898824132,2.32028348915368,
4.48471201133277));
#54639=CARTESIAN_POINT('Ctrl Pts',(-0.233031629605031,2.32262910615578,
4.48451312617098));
#54640=CARTESIAN_POINT('Ctrl Pts',(-0.231292968485754,2.32443489359354,
4.48435739175576));
#54641=CARTESIAN_POINT('Ctrl Pts',(-0.223579583352869,2.3322612510759,4.48367065009848));
#54642=CARTESIAN_POINT('Ctrl Pts',(-0.217390038820479,2.33806442041225,
4.48313018379167));
#54643=CARTESIAN_POINT('Ctrl Pts',(-0.200214722962118,2.35293877490139,
4.48165676651));
#54644=CARTESIAN_POINT('Ctrl Pts',(-0.188845205068137,2.36153656040124,
4.48070746905897));
#54645=CARTESIAN_POINT('Ctrl Pts',(-0.155942505368941,2.38315121774945,
4.47805228586352));
#54646=CARTESIAN_POINT('Ctrl Pts',(-0.13339620331319,2.39444581406517,4.47632715146045));
#54647=CARTESIAN_POINT('Ctrl Pts',(-0.108498678045123,2.4034650340022,4.47465463986337));
#54648=CARTESIAN_POINT('Ctrl Pts',(-0.107229336516695,2.40391587576309,
4.47456999580508));
#54649=CARTESIAN_POINT('Ctrl Pts',(-0.105570817886753,2.40449326002815,
4.47446024770178));
#54650=CARTESIAN_POINT('Ctrl Pts',(-0.105184198018649,2.40462703012608,
4.47443472398899));
#54651=CARTESIAN_POINT('Ctrl Pts',(-0.104588877874785,2.40483174184533,
4.47439551556005));
#54652=CARTESIAN_POINT('Ctrl Pts',(-0.104380359588049,2.40490320553337,
4.47438179988561));
#54653=CARTESIAN_POINT('Ctrl Pts',(-0.103965557906558,2.4050448915779,4.47435455069314));
#54654=CARTESIAN_POINT('Ctrl Pts',(-0.103759277718189,2.40511511826951,
4.47434101701871));
#54655=CARTESIAN_POINT('Ctrl Pts',(-0.103298268426545,2.40527154417185,
4.4743108096053));
#54656=CARTESIAN_POINT('Ctrl Pts',(-0.103043503258766,2.40535763356827,
4.47429414248433));
#54657=CARTESIAN_POINT('Ctrl Pts',(-0.102295414053347,2.40560938254398,
4.47424527754099));
#54658=CARTESIAN_POINT('Ctrl Pts',(-0.101801793203356,2.40577416722936,
4.4742131315385));
#54659=CARTESIAN_POINT('Ctrl Pts',(-0.0981122153388935,2.40699592852565,
4.47397356550991));
#54660=CARTESIAN_POINT('Ctrl Pts',(-0.0949001221484285,2.40800401933534,
4.47376897620937));
#54661=CARTESIAN_POINT('Ctrl Pts',(-0.0839914687636972,2.41124074924305,
4.47308567521436));
#54662=CARTESIAN_POINT('Ctrl Pts',(-0.0762273130646911,2.4132328016951,
4.47261850980601));
#54663=CARTESIAN_POINT('Ctrl Pts',(-0.0391905778975258,2.4212763381231,
4.47044554647348));
#54664=CARTESIAN_POINT('Ctrl Pts',(-0.00924472785627596,2.42352602791262,
4.46883609786955));
#54665=CARTESIAN_POINT('Ctrl Pts',(0.0301083332534404,2.42100740481181,
4.46653927602263));
#54666=CARTESIAN_POINT('Ctrl Pts',(0.0396003521912912,2.41997507797706,
4.46597263872235));
#54667=CARTESIAN_POINT('Ctrl Pts',(0.0501516498871189,2.41835086161297,
4.465323462058));
#54668=CARTESIAN_POINT('Ctrl Pts',(0.0512704282328862,2.41817259815009,
4.46525438655756));
#54669=CARTESIAN_POINT('Ctrl Pts',(0.0528597967512131,2.41791075150287,
4.46515590436989));
#54670=CARTESIAN_POINT('Ctrl Pts',(0.0533311857580323,2.41783201326401,
4.46512665161407));
#54671=CARTESIAN_POINT('Ctrl Pts',(0.0541959564767994,2.41768558868351,
4.465072905447));
#54672=CARTESIAN_POINT('Ctrl Pts',(0.0545893915174747,2.41761821938784,
4.46504842215948));
#54673=CARTESIAN_POINT('Ctrl Pts',(0.055386815898049,2.41748014812923,4.4649987355163));
#54674=CARTESIAN_POINT('Ctrl Pts',(0.0557907973796482,2.41740940558961,
4.46497353091056));
#54675=CARTESIAN_POINT('Ctrl Pts',(0.0567857764561705,2.4172332132924,4.46491137191246));
#54676=CARTESIAN_POINT('Ctrl Pts',(0.0573766148008803,2.41712688326559,
4.46487438953699));
#54677=CARTESIAN_POINT('Ctrl Pts',(0.0595356592593219,2.41673210033206,
4.4647389858631));
#54678=CARTESIAN_POINT('Ctrl Pts',(0.0611019957969733,2.41643366456019,
4.4646402467365));
#54679=CARTESIAN_POINT('Ctrl Pts',(0.0701600580862758,2.41463806064984,
4.46406624199894));
#54680=CARTESIAN_POINT('Ctrl Pts',(0.0775983221806385,2.41288660461245,
4.46358288508447));
#54681=CARTESIAN_POINT('Ctrl Pts',(0.0919936168366696,2.40895212227722,
4.46262287294023));
#54682=CARTESIAN_POINT('Ctrl Pts',(0.0989527974004637,2.40679402052957,
4.46214723261885));
#54683=CARTESIAN_POINT('Ctrl Pts',(0.128649744806816,2.39646918363126,4.46006939889688));
#54684=CARTESIAN_POINT('Ctrl Pts',(0.150500257436267,2.38599694141076,4.45840914776875));
#54685=CARTESIAN_POINT('Ctrl Pts',(0.180046294304361,2.36750521033777,4.45608800343556));
#54686=CARTESIAN_POINT('Ctrl Pts',(0.188830652553895,2.36137854744795,4.45538816864679));
#54687=CARTESIAN_POINT('Ctrl Pts',(0.197880281213324,2.35437200776909,4.45466971185274));
#54688=CARTESIAN_POINT('Ctrl Pts',(0.198464277207677,2.3539166294824,4.45462336044449));
#54689=CARTESIAN_POINT('Ctrl Pts',(0.199273157668604,2.35328139916858,4.45455918361392));
#54690=CARTESIAN_POINT('Ctrl Pts',(0.199499372824427,2.35310325714273,4.45454123819974));
#54691=CARTESIAN_POINT('Ctrl Pts',(0.199888149776683,2.35279625439183,4.45451040179857));
#54692=CARTESIAN_POINT('Ctrl Pts',(0.200050825934099,2.35266753986083,4.45449750037733));
#54693=CARTESIAN_POINT('Ctrl Pts',(0.200383778747172,2.35240357391829,4.45447109797611));
#54694=CARTESIAN_POINT('Ctrl Pts',(0.20055404256886,2.35226830740556,4.4544575981957));
#54695=CARTESIAN_POINT('Ctrl Pts',(0.200952656417856,2.35195096903396,4.45442599692546));
#54696=CARTESIAN_POINT('Ctrl Pts',(0.201180896832849,2.35176875832733,4.45440790542132));
#54697=CARTESIAN_POINT('Ctrl Pts',(0.201662895029652,2.35138289174255,4.45436970519287));
#54698=CARTESIAN_POINT('Ctrl Pts',(0.201916592956766,2.3511791611251,4.45434960183096));
#54699=CARTESIAN_POINT('Ctrl Pts',(0.202598398843979,2.35062994044679,4.4542955818674));
#54700=CARTESIAN_POINT('Ctrl Pts',(0.203025933783631,2.3502837359561,4.45426171567616));
#54701=CARTESIAN_POINT('Ctrl Pts',(0.213880728340614,2.34144774533698,4.45340201371961));
#54702=CARTESIAN_POINT('Ctrl Pts',(0.223768893485688,2.33231349890859,4.45262186816909));
#54703=CARTESIAN_POINT('Ctrl Pts',(0.255183806318814,2.29942066912169,4.45003877443414));
#54704=CARTESIAN_POINT('Ctrl Pts',(0.273730340374863,2.27308705072218,4.44830741820548));
#54705=CARTESIAN_POINT('Ctrl Pts',(0.290429522192716,2.23978244713345,4.44609339193743));
#54706=CARTESIAN_POINT('Ctrl Pts',(0.292656017105525,2.23505884182629,4.44577945773601));
#54707=CARTESIAN_POINT('Ctrl Pts',(0.295118138897196,2.22948828324147,4.44540858022175));
#54708=CARTESIAN_POINT('Ctrl Pts',(0.295466364161317,2.22869172090325,4.44535553171109));
#54709=CARTESIAN_POINT('Ctrl Pts',(0.296017055693599,2.22741800118514,4.44527067863244));
#54710=CARTESIAN_POINT('Ctrl Pts',(0.296221602870952,2.22694174362727,4.44523894506001));
#54711=CARTESIAN_POINT('Ctrl Pts',(0.29658070369808,2.22610003671187,4.44518284962745));
#54712=CARTESIAN_POINT('Ctrl Pts',(0.2967357334264,2.22573479061281,4.4451585040221));
#54713=CARTESIAN_POINT('Ctrl Pts',(0.297054992033892,2.22497874630301,4.44510810129153));
#54714=CARTESIAN_POINT('Ctrl Pts',(0.297219125100246,2.22458790868957,4.44508204097011));
#54715=CARTESIAN_POINT('Ctrl Pts',(0.29763764068907,2.22358579545913,4.44501520957049));
#54716=CARTESIAN_POINT('Ctrl Pts',(0.297890910535101,2.22297405988396,4.44497440087338));
#54717=CARTESIAN_POINT('Ctrl Pts',(0.298919354571821,2.22046818563054,4.44480718324378));
#54718=CARTESIAN_POINT('Ctrl Pts',(0.299678348858594,2.21856749639668,4.44468022919748));
#54719=CARTESIAN_POINT('Ctrl Pts',(0.304579666821558,2.20594574807542,4.44383624186085));
#54720=CARTESIAN_POINT('Ctrl Pts',(0.308163565718999,2.1950180963027,4.44310064696179));
#54721=CARTESIAN_POINT('Ctrl Pts',(0.319705909018979,2.1522235003017,4.44019971276318));
#54722=CARTESIAN_POINT('Ctrl Pts',(0.323360473012411,2.11940908314164,4.43790971082713));
#54723=CARTESIAN_POINT('Ctrl Pts',(0.321786569198625,2.08155592580723,4.43545177812395));
#54724=CARTESIAN_POINT('Ctrl Pts',(0.321457300508331,2.07650551018429,4.43512820494653));
#54725=CARTESIAN_POINT('Ctrl Pts',(0.320952975646236,2.07083210197153,4.43477118094128));
#54726=CARTESIAN_POINT('Ctrl Pts',(0.320894880489813,2.07019975598632,4.43473147849955));
#54727=CARTESIAN_POINT('Ctrl Pts',(0.320807628880947,2.06927990268041,4.43467386070206));
#54728=CARTESIAN_POINT('Ctrl Pts',(0.32077995459967,2.06899226135075,4.4346558627857));
#54729=CARTESIAN_POINT('Ctrl Pts',(0.320730832246723,2.06848879707,4.43462439505245));
#54730=CARTESIAN_POINT('Ctrl Pts',(0.320709553215465,2.06827295883453,4.43461091572398));
#54731=CARTESIAN_POINT('Ctrl Pts',(0.320664846116422,2.06782412511059,4.43458290871706));
#54732=CARTESIAN_POINT('Ctrl Pts',(0.320641382065921,2.06759113443115,4.43456838313801));
#54733=CARTESIAN_POINT('Ctrl Pts',(0.320580442822337,2.06699257126501,4.43453109903687));
#54734=CARTESIAN_POINT('Ctrl Pts',(0.320542596118838,2.06662703566607,4.43450836145497));
#54735=CARTESIAN_POINT('Ctrl Pts',(0.320458871388904,2.06583167808654,4.43445895422118));
#54736=CARTESIAN_POINT('Ctrl Pts',(0.320412753586477,2.0654018812878,4.43443229790286));
#54737=CARTESIAN_POINT('Ctrl Pts',(0.320276748932008,2.06415797771096,4.43435526963409));
#54738=CARTESIAN_POINT('Ctrl Pts',(0.320184622327838,2.06334411198364,4.43430501961294));
#54739=CARTESIAN_POINT('Ctrl Pts',(0.319210546791,2.05502288943818,4.43379268426282));
#54740=CARTESIAN_POINT('Ctrl Pts',(0.318067751716315,2.04754774194699,4.4333443976989));
#54741=CARTESIAN_POINT('Ctrl Pts',(0.31512367707776,2.03197885260587,4.43242301783707));
#54742=CARTESIAN_POINT('Ctrl Pts',(0.313270967515525,2.023900567361,4.43195199141336));
#54743=CARTESIAN_POINT('Ctrl Pts',(0.304536883868285,1.991589926744,4.43006592967774));
#54744=CARTESIAN_POINT('Ctrl Pts',(0.295138258999131,1.96813331643806,4.4286841869479));
#54745=CARTESIAN_POINT('Ctrl Pts',(0.28169330484156,1.94341525150783,4.42703826527747));
#54746=CARTESIAN_POINT('Ctrl Pts',(0.280246266328384,1.94083992054523,4.42686441923744));
#54747=CARTESIAN_POINT('Ctrl Pts',(0.275827611325756,1.93322305471463,4.42634269655314));
#54748=CARTESIAN_POINT('Ctrl Pts',(0.272753991311786,1.92824239691003,4.42599149944224));
#54749=CARTESIAN_POINT('Ctrl Pts',(0.269004041470019,1.9225204767946,4.42557501257402));
#54750=CARTESIAN_POINT('Ctrl Pts',(0.268457643341898,1.92169506686144,4.4255146091281));
#54751=CARTESIAN_POINT('Ctrl Pts',(0.267628188795722,1.92045451653725,4.42542333125281));
#54752=CARTESIAN_POINT('Ctrl Pts',(0.267347946596122,1.92003749413758,4.42539256259399));
#54753=CARTESIAN_POINT('Ctrl Pts',(0.266846234064971,1.9192946647454,4.42533760309664));
#54754=CARTESIAN_POINT('Ctrl Pts',(0.266625138903693,1.91896860458324,4.42531342644442));
#54755=CARTESIAN_POINT('Ctrl Pts',(0.26615757632399,1.91828178108096,4.42526238862274));
#54756=CARTESIAN_POINT('Ctrl Pts',(0.265910972184482,1.91792111217748,4.42523552231068));
#54757=CARTESIAN_POINT('Ctrl Pts',(0.265257198688153,1.91696910194844,4.42516443405522));
#54758=CARTESIAN_POINT('Ctrl Pts',(0.264848787064476,1.91637862032262,4.42512016499919));
#54759=CARTESIAN_POINT('Ctrl Pts',(0.26298561063822,1.91370398754606,4.42491883559167));
#54760=CARTESIAN_POINT('Ctrl Pts',(0.261508226866333,1.91163577211601,4.42476091336106));
#54761=CARTESIAN_POINT('Ctrl Pts',(0.254956597043167,1.90268968375777,4.42406779465087));
#54762=CARTESIAN_POINT('Ctrl Pts',(0.249634736505242,1.89599827562939,4.42352302341793));
#54763=CARTESIAN_POINT('Ctrl Pts',(0.24050585607852,1.88541291029464,4.42261623387618));
#54764=CARTESIAN_POINT('Ctrl Pts',(0.236854784251018,1.88138963388034,4.42226012244768));
#54765=CARTESIAN_POINT('Ctrl Pts',(0.230367087010454,1.87459394533332,4.42163880562299));
#54766=CARTESIAN_POINT('Ctrl Pts',(0.227577665743222,1.87177798354352,4.42137510890594));
#54767=CARTESIAN_POINT('Ctrl Pts',(0.211598483321895,1.85623107254909,4.41988460608222));
#54768=CARTESIAN_POINT('Ctrl Pts',(0.197393770619289,1.84459272900576,4.41863209166605));
#54769=CARTESIAN_POINT('Ctrl Pts',(0.172130132608163,1.8272660942492,4.41658197186032));
#54770=CARTESIAN_POINT('Ctrl Pts',(0.161591580632492,1.82089284451229,4.41577255006289));
#54771=CARTESIAN_POINT('Ctrl Pts',(0.150023218241999,1.8147723387325,4.41495063754112));
#54772=CARTESIAN_POINT('Ctrl Pts',(0.149332016418205,1.81440985019381,4.41490177406642));
#54773=CARTESIAN_POINT('Ctrl Pts',(0.14837827955385,1.81391408903499,4.41483469532006));
#54774=CARTESIAN_POINT('Ctrl Pts',(0.148116875795505,1.81377866361448,4.41481634562381));
#54775=CARTESIAN_POINT('Ctrl Pts',(0.147669296514933,1.81354756362365,4.4147849881801));
#54776=CARTESIAN_POINT('Ctrl Pts',(0.14748321332103,1.81345171222247,4.41477196923512));
#54777=CARTESIAN_POINT('Ctrl Pts',(0.147105261952016,1.81325749526824,4.41474556345939));
#54778=CARTESIAN_POINT('Ctrl Pts',(0.146913388685245,1.81315914109081,4.41473217740209));
#54779=CARTESIAN_POINT('Ctrl Pts',(0.14646853124635,1.81293167076412,4.41470118658725));
#54780=CARTESIAN_POINT('Ctrl Pts',(0.146215475433979,1.81280269666855,4.41468359095198));
#54781=CARTESIAN_POINT('Ctrl Pts',(0.145681391537066,1.81253138080525,4.41464652438819));
#54782=CARTESIAN_POINT('Ctrl Pts',(0.145400324331815,1.81238911608194,4.41462705834358));
#54783=CARTESIAN_POINT('Ctrl Pts',(0.144648598620156,1.81201000684936,4.41457510288657));
#54784=CARTESIAN_POINT('Ctrl Pts',(0.144177564655171,1.81177390281764,4.41454265961742));
#54785=CARTESIAN_POINT('Ctrl Pts',(0.142739533054601,1.81105750211353,4.41444394800241));
#54786=CARTESIAN_POINT('Ctrl Pts',(0.141770687159321,1.81058090298048,4.41437790410398));
#54787=CARTESIAN_POINT('Ctrl Pts',(0.138221168679432,1.80885690828808,4.41413755668986));
#54788=CARTESIAN_POINT('Ctrl Pts',(0.135626197375761,1.80763904643118,4.41396495003369));
#54789=CARTESIAN_POINT('Ctrl Pts',(0.126642533147847,1.80356822979324,4.41337684640274));
#54790=CARTESIAN_POINT('Ctrl Pts',(0.120177050737953,1.80088862382197,4.41296984152715));
#54791=CARTESIAN_POINT('Ctrl Pts',(0.0847615380862129,1.78754473360271,
4.41080099533721));
#54792=CARTESIAN_POINT('Ctrl Pts',(0.0544823634979874,1.78086887746603,
4.40914501070586));
#54793=CARTESIAN_POINT('Ctrl Pts',(0.0209445314662134,1.7783943163197,4.40718131347243));
#54794=CARTESIAN_POINT('Ctrl Pts',(0.0181722671549749,1.7782257666651,4.40701819627046));
#54795=CARTESIAN_POINT('Ctrl Pts',(0.0141491157124072,1.7780333216021,4.40678013542227));
#54796=CARTESIAN_POINT('Ctrl Pts',(0.0128996799294585,1.77798084269795,
4.4067060155409));
#54797=CARTESIAN_POINT('Ctrl Pts',(0.00656572131066864,1.77775172542638,
4.40632926464961));
#54798=CARTESIAN_POINT('Ctrl Pts',(0.00147805479965953,1.77768824091122,
4.40602335184442));
#54799=CARTESIAN_POINT('Ctrl Pts',(-0.00446655842054763,1.77775481172251,
4.40566137815842));
#54800=CARTESIAN_POINT('Ctrl Pts',(-0.00532429485811365,1.7777678424274,
4.40560903983186));
#54801=CARTESIAN_POINT('Ctrl Pts',(-0.00669482120962326,1.77779413705707,
4.40552523237389));
#54802=CARTESIAN_POINT('Ctrl Pts',(-0.00720765327246761,1.77780520104246,
4.40549383269388));
#54803=CARTESIAN_POINT('Ctrl Pts',(-0.00811388734251212,1.77782691711509,
4.40543827416123));
#54804=CARTESIAN_POINT('Ctrl Pts',(-0.00850730129608764,1.77783706556179,
4.40541413125278));
#54805=CARTESIAN_POINT('Ctrl Pts',(-0.00932182339267204,1.77785956987869,
4.40536409609776));
#54806=CARTESIAN_POINT('Ctrl Pts',(-0.00974292766759119,1.77787203091338,
4.4053382005767));
#54807=CARTESIAN_POINT('Ctrl Pts',(-0.0108234410920633,1.77790612542731,
4.40527168380189));
#54808=CARTESIAN_POINT('Ctrl Pts',(-0.0114828080472422,1.77792895811133,
4.40523102475855));
#54809=CARTESIAN_POINT('Ctrl Pts',(-0.014193643489848,1.77803116464757,
4.40506358065614));
#54810=CARTESIAN_POINT('Ctrl Pts',(-0.0162443651213139,1.77812811439979,
4.40493624190347));
#54811=CARTESIAN_POINT('Ctrl Pts',(-0.0298764253930816,1.77890318985903,
4.40408517331389));
#54812=CARTESIAN_POINT('Ctrl Pts',(-0.0414135041611636,1.78018657168362,
4.40334237160816));
#54813=CARTESIAN_POINT('Ctrl Pts',(-0.0618461876082502,1.78358366573439,
4.40198574524155));
#54814=CARTESIAN_POINT('Ctrl Pts',(-0.0707691234933321,1.78545912929497,
4.40137909932707));
#54815=CARTESIAN_POINT('Ctrl Pts',(-0.0821953293102451,1.78837157324676,
4.40058672004942));
#54816=CARTESIAN_POINT('Ctrl Pts',(-0.0847822030411975,1.7890653986954,
4.40040629262924));
#54817=CARTESIAN_POINT('Ctrl Pts',(-0.0895568653694782,1.79041002603614,
4.40007152438889));
#54818=CARTESIAN_POINT('Ctrl Pts',(-0.0917469827105972,1.79105198630164,
4.39991727997557));
#54819=CARTESIAN_POINT('Ctrl Pts',(-0.0958291656182346,1.79229577845136,
4.39962861686701));
#54820=CARTESIAN_POINT('Ctrl Pts',(-0.0977228552277498,1.79289194006671,
4.39949423555541));
#54821=CARTESIAN_POINT('Ctrl Pts',(-0.118423162978865,1.79961955482423,
4.39802061865691));
#54822=CARTESIAN_POINT('Ctrl Pts',(-0.136634588979585,1.80745323094136,
4.39667887427147));
#54823=CARTESIAN_POINT('Ctrl Pts',(-0.155895771020906,1.81793214827442,
4.39528414492368));
#54824=CARTESIAN_POINT('Ctrl Pts',(-0.157767271604775,1.81897463992516,
4.39514892738152));
#54825=CARTESIAN_POINT('Ctrl Pts',(-0.160006977809383,1.82025166185578,
4.39498759895547));
#54826=CARTESIAN_POINT('Ctrl Pts',(-0.160385222006933,1.82046834488869,
4.39496037066216));
#54827=CARTESIAN_POINT('Ctrl Pts',(-0.161002284248947,1.82082350332021,
4.39491598016177));
#54828=CARTESIAN_POINT('Ctrl Pts',(-0.161241364498036,1.82096151841016,
4.39489878831537));
#54829=CARTESIAN_POINT('Ctrl Pts',(-0.161659881438182,1.82120383533108,
4.39486870654485));
#54830=CARTESIAN_POINT('Ctrl Pts',(-0.161839393179539,1.82130800241799,
4.39485580801692));
#54831=CARTESIAN_POINT('Ctrl Pts',(-0.162225806844437,1.821532729821,4.39482805188359));
#54832=CARTESIAN_POINT('Ctrl Pts',(-0.162432674537413,1.82165334704583,
4.39481319810085));
#54833=CARTESIAN_POINT('Ctrl Pts',(-0.162977671823719,1.82197193013445,
4.39477407960757));
#54834=CARTESIAN_POINT('Ctrl Pts',(-0.163315576474736,1.82217028303146,
4.39474984002556));
#54835=CARTESIAN_POINT('Ctrl Pts',(-0.164056412161959,1.82260697843853,
4.39469672581033));
#54836=CARTESIAN_POINT('Ctrl Pts',(-0.16445918814923,1.82284558415538,4.39466786806795));
#54837=CARTESIAN_POINT('Ctrl Pts',(-0.165647719278523,1.8235531767693,4.39458276593566));
#54838=CARTESIAN_POINT('Ctrl Pts',(-0.166432006372451,1.82402463827811,
4.39452667704528));
#54839=CARTESIAN_POINT('Ctrl Pts',(-0.169162714998928,1.82568203415616,
4.39433158888757));
#54840=CARTESIAN_POINT('Ctrl Pts',(-0.171098605387895,1.82688530172058,
4.39419364168322));
#54841=CARTESIAN_POINT('Ctrl Pts',(-0.180054863384314,1.8325847422329,4.39355632571406));
#54842=CARTESIAN_POINT('Ctrl Pts',(-0.186912378454082,1.83733203584922,
4.39307088697199));
#54843=CARTESIAN_POINT('Ctrl Pts',(-0.214988641288412,1.85842560678748,
4.39106025797942));
#54844=CARTESIAN_POINT('Ctrl Pts',(-0.2343105539658,1.87711664615387,4.38960940869498));
#54845=CARTESIAN_POINT('Ctrl Pts',(-0.252607669201272,1.89985920467212,
4.38792777434474));
#54846=CARTESIAN_POINT('Ctrl Pts',(-0.254095812546078,1.9017519478463,4.38778845887559));
#54847=CARTESIAN_POINT('Ctrl Pts',(-0.261683017159232,1.91162776060205,
4.38706430365587));
#54848=CARTESIAN_POINT('Ctrl Pts',(-0.267427041060778,1.91987546425222,
4.38646847932064));
#54849=CARTESIAN_POINT('Ctrl Pts',(-0.273336076576221,1.92926725471254,
4.38579363179422));
#54850=CARTESIAN_POINT('Ctrl Pts',(-0.27389162129599,1.9301598963303,4.38572952870617));
#54851=CARTESIAN_POINT('Ctrl Pts',(-0.274715372125618,1.93149804058435,
4.38563348280659));
#54852=CARTESIAN_POINT('Ctrl Pts',(-0.274986887969283,1.93194150587066,
4.38560166104879));
#54853=CARTESIAN_POINT('Ctrl Pts',(-0.275452373532967,1.93270592904141,
4.38554682152066));
#54854=CARTESIAN_POINT('Ctrl Pts',(-0.275646859058124,1.93302657291559,
4.3855238225981));
#54855=CARTESIAN_POINT('Ctrl Pts',(-0.276046835904073,1.93368860896503,
4.38547634440509));
#54856=CARTESIAN_POINT('Ctrl Pts',(-0.276252254557321,1.93403004413321,
4.38545186254307));
#54857=CARTESIAN_POINT('Ctrl Pts',(-0.27672848620391,1.93482494281015,4.38539487561855));
#54858=CARTESIAN_POINT('Ctrl Pts',(-0.276998818122395,1.9352786918826,4.38536235318719));
#54859=CARTESIAN_POINT('Ctrl Pts',(-0.277855087040688,1.93672399827022,
4.38525878246725));
#54860=CARTESIAN_POINT('Ctrl Pts',(-0.278436819706205,1.93771802468459,
4.38518758256341));
#54861=CARTESIAN_POINT('Ctrl Pts',(-0.290061833012129,1.95782860533378,
4.38374766923735));
#54862=CARTESIAN_POINT('Ctrl Pts',(-0.299114980480026,1.9780227663809,4.38230575172274));
#54863=CARTESIAN_POINT('Ctrl Pts',(-0.313616405766477,2.02195357590079,
4.37919979833315));
#54864=CARTESIAN_POINT('Ctrl Pts',(-0.318589153887707,2.04570886986425,
4.37753747090088));
#54865=CARTESIAN_POINT('Ctrl Pts',(-0.320986583694565,2.07117793557682,
4.3758874634548));
#54866=CARTESIAN_POINT('Ctrl Pts',(-0.321107623629924,2.07255929128988,
4.37579839930321));
#54867=CARTESIAN_POINT('Ctrl Pts',(-0.321455123307179,2.07684285985011,
4.37552361944549));
#54868=CARTESIAN_POINT('Ctrl Pts',(-0.321651187999729,2.07974749065067,
4.37533929403666));
#54869=CARTESIAN_POINT('Ctrl Pts',(-0.321834175319448,2.08314242069002,
4.37512649291554));
#54870=CARTESIAN_POINT('Ctrl Pts',(-0.321859364856429,2.08363040485127,
4.37509596868315));
#54871=CARTESIAN_POINT('Ctrl Pts',(-0.321897798115476,2.08440936083387,
4.37504734719406));
#54872=CARTESIAN_POINT('Ctrl Pts',(-0.321911757277751,2.08470029446399,
4.37502921051265));
#54873=CARTESIAN_POINT('Ctrl Pts',(-0.321935546127147,2.08521054562655,
4.37499744254248));
#54874=CARTESIAN_POINT('Ctrl Pts',(-0.321945546126175,2.08542985411713,
4.37498380173922));
#54875=CARTESIAN_POINT('Ctrl Pts',(-0.321964675993694,2.08585902540057,
4.37495713323466));
#54876=CARTESIAN_POINT('Ctrl Pts',(-0.321973824784277,2.08606888716867,
4.37494410449256));
#54877=CARTESIAN_POINT('Ctrl Pts',(-0.321993022699707,2.08651938561134,
4.37491616183459));
#54878=CARTESIAN_POINT('Ctrl Pts',(-0.322003007280448,2.0867600251201,4.37490125146639));
#54879=CARTESIAN_POINT('Ctrl Pts',(-0.322026432696717,2.08734030778371,
4.37486533335715));
#54880=CARTESIAN_POINT('Ctrl Pts',(-0.322039606005793,2.08767996231985,
4.37484434014324));
#54881=CARTESIAN_POINT('Ctrl Pts',(-0.322098762712622,2.0892701940173,4.37474619238116));
#54882=CARTESIAN_POINT('Ctrl Pts',(-0.322137999888886,2.09052103270796,
4.37466939859012));
#54883=CARTESIAN_POINT('Ctrl Pts',(-0.322238911436358,2.09447230018914,
4.37442801115635));
#54884=CARTESIAN_POINT('Ctrl Pts',(-0.322273924581758,2.09717335249639,
4.37426476447746));
#54885=CARTESIAN_POINT('Ctrl Pts',(-0.322274975605568,2.09987460689646,
4.37410298671292));
#54886=CARTESIAN_POINT('',(-0.203129159293197,2.35019936105002,4.35670055803058));
#54887=CARTESIAN_POINT('Ctrl Pts',(-0.203129159293197,2.35019936105002,
4.35670055803058));
#54888=CARTESIAN_POINT('Ctrl Pts',(-0.216614563769107,2.33925097628028,
4.35777896221699));
#54889=CARTESIAN_POINT('Ctrl Pts',(-0.229260010381491,2.32717006691284,
4.3588573664034));
#54890=CARTESIAN_POINT('Ctrl Pts',(-0.240866999069484,2.31411273755725,
4.35993577058981));
#54891=CARTESIAN_POINT('Ctrl Pts',(-0.252452758994495,2.30107928958534,
4.36101220241392));
#54892=CARTESIAN_POINT('Ctrl Pts',(-0.263003251354075,2.28707351158869,
4.36208863423803));
#54893=CARTESIAN_POINT('Ctrl Pts',(-0.272355508139451,2.27228944486271,
4.36316506606214));
#54894=CARTESIAN_POINT('Ctrl Pts',(-0.281706384805359,2.25750755983242,
4.36424133903641));
#54895=CARTESIAN_POINT('Ctrl Pts',(-0.289858909139876,2.2419482646331,4.36531761201069));
#54896=CARTESIAN_POINT('Ctrl Pts',(-0.296692758115266,2.2258355391253,4.36639388498496));
#54897=CARTESIAN_POINT('Ctrl Pts',(-0.303525842065698,2.20972461737952,
4.36747003747432));
#54898=CARTESIAN_POINT('Ctrl Pts',(-0.309040250270101,2.19306113470876,
4.36854618996367));
#54899=CARTESIAN_POINT('Ctrl Pts',(-0.313164036280824,2.17608851427977,
4.36962234245303));
#54900=CARTESIAN_POINT('Ctrl Pts',(-0.317296249751049,2.15908120823156,
4.37070069419121));
#54901=CARTESIAN_POINT('Ctrl Pts',(-0.320032030726004,2.14176429471861,
4.37177904592939));
#54902=CARTESIAN_POINT('Ctrl Pts',(-0.321350696853865,2.1243906797063,4.37285739766757));
#54903=CARTESIAN_POINT('Ctrl Pts',(-0.321970254428679,2.11622791996345,
4.37336404675303));
#54904=CARTESIAN_POINT('Ctrl Pts',(-0.322277741048769,2.10805268328092,
4.37387069583848));
#54905=CARTESIAN_POINT('Ctrl Pts',(-0.322274981579892,2.09989103817067,
4.37437734492394));
#54906=CARTESIAN_POINT('',(-0.30265674053785,1.98927478592477,4.3567));
#54907=CARTESIAN_POINT('Origin',(0.,2.1,4.3567));
#54908=CARTESIAN_POINT('',(-0.322274978099547,2.0998811894946,4.4747226550683));
#54909=CARTESIAN_POINT('Ctrl Pts',(-0.302656740537849,1.98927478592477,
4.35670000000001));
#54910=CARTESIAN_POINT('Ctrl Pts',(-0.296404879462199,1.97218592399522,
4.35782329269583));
#54911=CARTESIAN_POINT('Ctrl Pts',(-0.288694193033434,1.95560777832229,
4.35894658539165));
#54912=CARTESIAN_POINT('Ctrl Pts',(-0.279632519152931,1.9397912928172,4.36006987808747));
#54913=CARTESIAN_POINT('Ctrl Pts',(-0.270577330574803,1.92398612693056,
4.36119236685978));
#54914=CARTESIAN_POINT('Ctrl Pts',(-0.260173420581183,1.90894216953555,
4.36231485563208));
#54915=CARTESIAN_POINT('Ctrl Pts',(-0.248574373589272,1.89488550412099,
4.36343734440438));
#54916=CARTESIAN_POINT('Ctrl Pts',(-0.23696239461704,1.88081316668436,4.36456108465904));
#54917=CARTESIAN_POINT('Ctrl Pts',(-0.224153067988682,1.86773088506809,
4.3656848249137));
#54918=CARTESIAN_POINT('Ctrl Pts',(-0.21034067269066,1.85583207205482,4.36680856516836));
#54919=CARTESIAN_POINT('Ctrl Pts',(-0.196522621340862,1.84392838658454,
4.36793276558456));
#54920=CARTESIAN_POINT('Ctrl Pts',(-0.181701252710663,1.83320958091786,
4.36905696600076));
#54921=CARTESIAN_POINT('Ctrl Pts',(-0.166103519464854,1.8238283207018,4.37018116641696));
#54922=CARTESIAN_POINT('Ctrl Pts',(-0.150460516351211,1.81441983291341,
4.37130862964087));
#54923=CARTESIAN_POINT('Ctrl Pts',(-0.134037286039767,1.80635699061725,
4.37243609286478));
#54924=CARTESIAN_POINT('Ctrl Pts',(-0.117086170482513,1.79974676636755,
4.37356355608868));
#54925=CARTESIAN_POINT('Ctrl Pts',(-0.102017415490227,1.79387058380445,
4.37456581856672));
#54926=CARTESIAN_POINT('Ctrl Pts',(-0.086532162885214,1.7891417213372,4.37556808104475));
#54927=CARTESIAN_POINT('Ctrl Pts',(-0.070816614222938,1.78560187218274,
4.37657034352279));
#54928=CARTESIAN_POINT('Ctrl Pts',(-0.0537834963462461,1.78176524711737,
4.37765663425935));
#54929=CARTESIAN_POINT('Ctrl Pts',(-0.036373093928319,1.77930248748307,
4.37874292499591));
#54930=CARTESIAN_POINT('Ctrl Pts',(-0.0188326652239015,1.77827572931847,
4.37982921573246));
#54931=CARTESIAN_POINT('Ctrl Pts',(-0.00132981533986302,1.77725117089261,
4.380913179187));
#54932=CARTESIAN_POINT('Ctrl Pts',(0.0163017347981785,1.77765663538176,
4.38199714264153));
#54933=CARTESIAN_POINT('Ctrl Pts',(0.0338062062375431,1.77950301710496,
4.38308110609606));
#54934=CARTESIAN_POINT('Ctrl Pts',(0.0517843956155461,1.781399366869,4.38419440450852));
#54935=CARTESIAN_POINT('Ctrl Pts',(0.0696276570204186,1.78481592139951,
4.38530770292098));
#54936=CARTESIAN_POINT('Ctrl Pts',(0.0870607697616642,1.78970723825151,
4.38642100133344));
#54937=CARTESIAN_POINT('Ctrl Pts',(0.104020876238972,1.79446584079458,4.38750409302777));
#54938=CARTESIAN_POINT('Ctrl Pts',(0.120592055650822,1.80061981374593,4.3885871847221));
#54939=CARTESIAN_POINT('Ctrl Pts',(0.136534628114959,1.80807625833018,4.38967027641643));
#54940=CARTESIAN_POINT('Ctrl Pts',(0.153144142439005,1.81584463594973,4.39079867818795));
#54941=CARTESIAN_POINT('Ctrl Pts',(0.169070369245532,1.82502664665808,4.39192707995948));
#54942=CARTESIAN_POINT('Ctrl Pts',(0.184070819008737,1.83546435171332,4.393055481731));
#54943=CARTESIAN_POINT('Ctrl Pts',(0.199071268771941,1.84590205676856,4.39418388350253));
#54944=CARTESIAN_POINT('Ctrl Pts',(0.213145247532986,1.85759478899131,4.39531228527405));
#54945=CARTESIAN_POINT('Ctrl Pts',(0.226090844627291,1.87033915091876,4.39644068704558));
#54946=CARTESIAN_POINT('Ctrl Pts',(0.238695992515106,1.88274835581375,4.39753941359356));
#54947=CARTESIAN_POINT('Ctrl Pts',(0.250315384053979,1.89623671552766,4.39863814014154));
#54948=CARTESIAN_POINT('Ctrl Pts',(0.260762804773581,1.91062224187721,4.39973686668952));
#54949=CARTESIAN_POINT('Ctrl Pts',(0.271190233577476,1.92498024045335,4.40083349074262));
#54950=CARTESIAN_POINT('Ctrl Pts',(0.280449643884497,1.94023141810416,4.40193011479572));
#54951=CARTESIAN_POINT('Ctrl Pts',(0.288394111067946,1.95615976805383,4.40302673884883));
#54952=CARTESIAN_POINT('Ctrl Pts',(0.296413922667818,1.9722391806492,4.40413376315879));
#54953=CARTESIAN_POINT('Ctrl Pts',(0.303093248446507,1.98900802855614,4.40524078746875));
#54954=CARTESIAN_POINT('Ctrl Pts',(0.308327722020033,2.00621731791563,4.40634781177871));
#54955=CARTESIAN_POINT('Ctrl Pts',(0.313510317810215,2.02325604957294,4.40744386460004));
#54956=CARTESIAN_POINT('Ctrl Pts',(0.317276412305712,2.04072576159458,4.40853991742137));
#54957=CARTESIAN_POINT('Ctrl Pts',(0.319574828048716,2.05836942346504,4.4096359702427));
#54958=CARTESIAN_POINT('Ctrl Pts',(0.321907754503758,2.07627800491584,4.41074848029698));
#54959=CARTESIAN_POINT('Ctrl Pts',(0.322728416857932,2.09436499939892,4.41186099035126));
#54960=CARTESIAN_POINT('Ctrl Pts',(0.32203798925476,2.11235755241749,4.41297350040554));
#54961=CARTESIAN_POINT('Ctrl Pts',(0.321347561651589,2.13035010543605,4.41408601045981));
#54962=CARTESIAN_POINT('Ctrl Pts',(0.319146197115451,2.14824740746737,4.41519852051409));
#54963=CARTESIAN_POINT('Ctrl Pts',(0.315489363474537,2.16578477908629,4.41631103056837));
#54964=CARTESIAN_POINT('Ctrl Pts',(0.311876365368133,2.18311192510176,4.41741020463921));
#54965=CARTESIAN_POINT('Ctrl Pts',(0.306820812234803,2.2001926869356,4.41850937871005));
#54966=CARTESIAN_POINT('Ctrl Pts',(0.300375610800813,2.21677186331064,4.41960855278089));
#54967=CARTESIAN_POINT('Ctrl Pts',(0.29394238844351,2.23332022556338,4.42070568392248));
#54968=CARTESIAN_POINT('Ctrl Pts',(0.286124863992888,2.24936812040546,4.42180281506408));
#54969=CARTESIAN_POINT('Ctrl Pts',(0.277025776962371,2.26467511810651,4.42289994620567));
#54970=CARTESIAN_POINT('Ctrl Pts',(0.267846619944137,2.28011681405958,4.4240067318628));
#54971=CARTESIAN_POINT('Ctrl Pts',(0.257363532542741,2.29480376905319,4.42511351751992));
#54972=CARTESIAN_POINT('Ctrl Pts',(0.245729626709979,2.30851409108733,4.42622030317704));
#54973=CARTESIAN_POINT('Ctrl Pts',(0.234201794628709,2.32209940735701,4.42731699756229));
#54974=CARTESIAN_POINT('Ctrl Pts',(0.221544601532698,2.33472527546789,4.42841369194754));
#54975=CARTESIAN_POINT('Ctrl Pts',(0.207946939793699,2.34620975987039,4.42951038633278));
#54976=CARTESIAN_POINT('Ctrl Pts',(0.194161599012098,2.35785275660235,4.43062221762585));
#54977=CARTESIAN_POINT('Ctrl Pts',(0.179410229651956,2.36832207423201,4.43173404891891));
#54978=CARTESIAN_POINT('Ctrl Pts',(0.163922416644867,2.37747183090596,4.43284588021197));
#54979=CARTESIAN_POINT('Ctrl Pts',(0.148434603637777,2.38662158757992,4.43395771150504));
#54980=CARTESIAN_POINT('Ctrl Pts',(0.132211106067836,2.39445147857908,4.4350695427981));
#54981=CARTESIAN_POINT('Ctrl Pts',(0.115503787987989,2.40086550248479,4.43618137409116));
#54982=CARTESIAN_POINT('Ctrl Pts',(0.0990367795359562,2.40718727030906,
4.43727721336426));
#54983=CARTESIAN_POINT('Ctrl Pts',(0.081996347123964,2.4121733903919,4.43837305263736));
#54984=CARTESIAN_POINT('Ctrl Pts',(0.0646237538508256,2.41572922902897,
4.43946889191047));
#54985=CARTESIAN_POINT('Ctrl Pts',(0.0472848784563243,2.41927816625911,
4.44056260430619));
#54986=CARTESIAN_POINT('Ctrl Pts',(0.0296158596789326,2.42140211334889,
4.44165631670191));
#54987=CARTESIAN_POINT('Ctrl Pts',(0.011872857537185,2.42205622316437,4.44275002909764));
#54988=CARTESIAN_POINT('Ctrl Pts',(-0.00610961883994167,2.42271916138707,
4.44385850314066));
#54989=CARTESIAN_POINT('Ctrl Pts',(-0.0241672924948265,2.42187210391943,
4.44496697718369));
#54990=CARTESIAN_POINT('Ctrl Pts',(-0.042028264297906,2.41952277011992,
4.44607545122672));
#54991=CARTESIAN_POINT('Ctrl Pts',(-0.0596422300846304,2.41720592613055,
4.44716859577028));
#54992=CARTESIAN_POINT('Ctrl Pts',(-0.0770641265237543,2.41342829230801,
4.44826174031385));
#54993=CARTESIAN_POINT('Ctrl Pts',(-0.0940399066885015,2.40824936589557,
4.44935488485742));
#54994=CARTESIAN_POINT('Ctrl Pts',(-0.111372771670244,2.40296150098531,
4.45047102365017));
#54995=CARTESIAN_POINT('Ctrl Pts',(-0.128239712338758,2.39621289405118,
4.45158716244293));
#54996=CARTESIAN_POINT('Ctrl Pts',(-0.144389702293705,2.38811940145803,
4.45270330123568));
#54997=CARTESIAN_POINT('Ctrl Pts',(-0.160539692248653,2.38002590886489,
4.45381944002844));
#54998=CARTESIAN_POINT('Ctrl Pts',(-0.175972035610441,2.37058802489359,
4.4549355788212));
#54999=CARTESIAN_POINT('Ctrl Pts',(-0.190466496365977,2.3599686315444,4.45605171761395));
#55000=CARTESIAN_POINT('Ctrl Pts',(-0.204594111146087,2.34961800857428,
4.45713960761353));
#55001=CARTESIAN_POINT('Ctrl Pts',(-0.217923393648165,2.33807715066765,
4.4582274976131));
#55002=CARTESIAN_POINT('Ctrl Pts',(-0.230246003460366,2.3254949079592,4.45931538761268));
#55003=CARTESIAN_POINT('Ctrl Pts',(-0.242545064567707,2.31293671011825,
4.46040119863703));
#55004=CARTESIAN_POINT('Ctrl Pts',(-0.253840676982854,2.29934158552362,
4.46148700966138));
#55005=CARTESIAN_POINT('Ctrl Pts',(-0.263958165993931,2.28489797789625,
4.46257282068573));
#55006=CARTESIAN_POINT('Ctrl Pts',(-0.274073351784462,2.27045765831928,
4.46365838452797));
#55007=CARTESIAN_POINT('Ctrl Pts',(-0.283010453362923,2.25516985310587,
4.46474394837021));
#55008=CARTESIAN_POINT('Ctrl Pts',(-0.290635823550638,2.23925513884249,
4.46582951221245));
#55009=CARTESIAN_POINT('Ctrl Pts',(-0.298259388333677,2.22334419259285,
4.46691481903346));
#55010=CARTESIAN_POINT('Ctrl Pts',(-0.304571509155866,2.20680734850197,
4.46800012585447));
#55011=CARTESIAN_POINT('Ctrl Pts',(-0.309485782603731,2.18988729604987,
4.46908543267548));
#55012=CARTESIAN_POINT('Ctrl Pts',(-0.31441066678873,2.17293071037861,4.47017308285518));
#55013=CARTESIAN_POINT('Ctrl Pts',(-0.317931490025487,2.15559003286069,
4.47126073303488));
#55014=CARTESIAN_POINT('Ctrl Pts',(-0.32001248200996,2.13812068969503,4.47234838321458));
#55015=CARTESIAN_POINT('Ctrl Pts',(-0.321526706831123,2.12540919766228,
4.47313980716582));
#55016=CARTESIAN_POINT('Ctrl Pts',(-0.322279678047781,2.11262985771029,
4.47393123111706));
#55017=CARTESIAN_POINT('Ctrl Pts',(-0.322274978099547,2.0998811894946,4.4747226550683));
#55018=CARTESIAN_POINT('',(-0.322274995052385,2.09994352890236,4.72441933817791));
#55019=CARTESIAN_POINT('Ctrl Pts',(-0.322274984171188,2.09989899277133,
4.47499672223609));
#55020=CARTESIAN_POINT('Ctrl Pts',(-0.322273429072572,2.09493727479805,
4.4753190331803));
#55021=CARTESIAN_POINT('Ctrl Pts',(-0.322157288520209,2.08997587454079,
4.47563692052927));
#55022=CARTESIAN_POINT('Ctrl Pts',(-0.32189880254931,2.08442135331536,4.47598643353917));
#55023=CARTESIAN_POINT('Ctrl Pts',(-0.321869337429171,2.0838240007594,4.47602393855795));
#55024=CARTESIAN_POINT('Ctrl Pts',(-0.321820232419069,2.08288179528726,
4.47608296095535));
#55025=CARTESIAN_POINT('Ctrl Pts',(-0.32180170090614,2.08253688964145,4.4761045384053));
#55026=CARTESIAN_POINT('Ctrl Pts',(-0.321769318457598,2.08195175283111,
4.47614109585607));
#55027=CARTESIAN_POINT('Ctrl Pts',(-0.321755752949808,2.08171150713891,
4.47615609161978));
#55028=CARTESIAN_POINT('Ctrl Pts',(-0.321730105701105,2.08126615564203,
4.47618386351632));
#55029=CARTESIAN_POINT('Ctrl Pts',(-0.321718096881468,2.08106104600555,
4.47619664372542));
#55030=CARTESIAN_POINT('Ctrl Pts',(-0.321693417195328,2.08064631666016,
4.47622246409026));
#55031=CARTESIAN_POINT('Ctrl Pts',(-0.321680737662999,2.08043669908492,
4.47623550361519));
#55032=CARTESIAN_POINT('Ctrl Pts',(-0.321650685303944,2.07994780398357,
4.47626589056541));
#55033=CARTESIAN_POINT('Ctrl Pts',(-0.32163315366901,2.07966853709335,4.47628322893535));
#55034=CARTESIAN_POINT('Ctrl Pts',(-0.321578713976487,2.0788190448839,4.47633591222419));
#55035=CARTESIAN_POINT('Ctrl Pts',(-0.321540652791955,2.07824889068717,
4.47637119260462));
#55036=CARTESIAN_POINT('Ctrl Pts',(-0.321258436483804,2.07418401106051,
4.47662217694601));
#55037=CARTESIAN_POINT('Ctrl Pts',(-0.32095881712453,2.07069320152637,4.47683484267544));
#55038=CARTESIAN_POINT('Ctrl Pts',(-0.320499294592935,2.06620054785817,
4.47710563012839));
#55039=CARTESIAN_POINT('Ctrl Pts',(-0.320391522006456,2.06519377243649,
4.47716612289197));
#55040=CARTESIAN_POINT('Ctrl Pts',(-0.320124646487641,2.06280704580368,
4.4773091175874));
#55041=CARTESIAN_POINT('Ctrl Pts',(-0.319961361917081,2.06142757289138,
4.47739143708493));
#55042=CARTESIAN_POINT('Ctrl Pts',(-0.317109083622791,2.03859631139614,
4.47874907546743));
#55043=CARTESIAN_POINT('Ctrl Pts',(-0.31227681142198,2.01746528692992,4.47993814989359));
#55044=CARTESIAN_POINT('Ctrl Pts',(-0.297966718749578,1.97505017629298,
4.48244714670141));
#55045=CARTESIAN_POINT('Ctrl Pts',(-0.288231033890626,1.95398885226982,
4.48376561588582));
#55046=CARTESIAN_POINT('Ctrl Pts',(-0.275733533737731,1.93316619672375,
4.48524244698808));
#55047=CARTESIAN_POINT('Ctrl Pts',(-0.275136137255755,1.93218282130435,
4.48531260848586));
#55048=CARTESIAN_POINT('Ctrl Pts',(-0.274257707511894,1.93075413522918,
4.48541515868244));
#55049=CARTESIAN_POINT('Ctrl Pts',(-0.27398082402183,1.93030627314239,4.48544739485242));
#55050=CARTESIAN_POINT('Ctrl Pts',(-0.273493376315486,1.92952212412634,
4.48550399324385));
#55051=CARTESIAN_POINT('Ctrl Pts',(-0.27328328577089,1.92918554286353,4.48552833795757));
#55052=CARTESIAN_POINT('Ctrl Pts',(-0.272874444355994,1.9285332322881,4.48557561846849));
#55053=CARTESIAN_POINT('Ctrl Pts',(-0.272675765644358,1.92821745827761,
4.48559855157041));
#55054=CARTESIAN_POINT('Ctrl Pts',(-0.272200589289356,1.92746512860334,
4.48565329808707));
#55055=CARTESIAN_POINT('Ctrl Pts',(-0.271923589736859,1.92702889259477,
4.48568513008761));
#55056=CARTESIAN_POINT('Ctrl Pts',(-0.271084245857539,1.92571404109614,
4.48578133984946));
#55057=CARTESIAN_POINT('Ctrl Pts',(-0.270518687710994,1.92483749436224,
4.48584583711899));
#55058=CARTESIAN_POINT('Ctrl Pts',(-0.264558489828369,1.9156976240433,4.48652215719101));
#55059=CARTESIAN_POINT('Ctrl Pts',(-0.258791805671756,1.90768430292009,
4.48714796730868));
#55060=CARTESIAN_POINT('Ctrl Pts',(-0.234716198265635,1.87727652148885,
4.48965945756845));
#55061=CARTESIAN_POINT('Ctrl Pts',(-0.213795990968193,1.85712577176646,
4.49164875303043));
#55062=CARTESIAN_POINT('Ctrl Pts',(-0.183586135610912,1.83499029574287,
4.49415043452161));
#55063=CARTESIAN_POINT('Ctrl Pts',(-0.176487091884017,1.83020992720397,
4.49471436695229));
#55064=CARTESIAN_POINT('Ctrl Pts',(-0.16724144964405,1.82450626449113,4.49541179000964));
#55065=CARTESIAN_POINT('Ctrl Pts',(-0.165264447753006,1.82331576881747,
4.49555883752627));
#55066=CARTESIAN_POINT('Ctrl Pts',(-0.162478947992507,1.82167892802945,
4.49576294005663));
#55067=CARTESIAN_POINT('Ctrl Pts',(-0.161681113409922,1.82121469683959,
4.49582105017541));
#55068=CARTESIAN_POINT('Ctrl Pts',(-0.160473232347745,1.82051880367673,
4.49590848614731));
#55069=CARTESIAN_POINT('Ctrl Pts',(-0.160064662739322,1.82028460688197,
4.49593796883971));
#55070=CARTESIAN_POINT('Ctrl Pts',(-0.159313690036746,1.81985632490354,
4.49599198735746));
#55071=CARTESIAN_POINT('Ctrl Pts',(-0.158971442788583,1.81966197027282,
4.49601654022928));
#55072=CARTESIAN_POINT('Ctrl Pts',(-0.158420205062174,1.8193502686648,4.49605597983617));
#55073=CARTESIAN_POINT('Ctrl Pts',(-0.158211439573286,1.81923252777519,
4.49607089198801));
#55074=CARTESIAN_POINT('Ctrl Pts',(-0.157820996831486,1.81901289714336,
4.49609873538693));
#55075=CARTESIAN_POINT('Ctrl Pts',(-0.157639353556617,1.81891095143494,
4.49611167019485));
#55076=CARTESIAN_POINT('Ctrl Pts',(-0.157216061234975,1.81867392165739,
4.49614176966104));
#55077=CARTESIAN_POINT('Ctrl Pts',(-0.156974337243435,1.81853897301005,
4.49615892548677));
#55078=CARTESIAN_POINT('Ctrl Pts',(-0.156351449984595,1.8181922821646,4.49620305022385));
#55079=CARTESIAN_POINT('Ctrl Pts',(-0.155970028786825,1.81798100087157,
4.4962299895395));
#55080=CARTESIAN_POINT('Ctrl Pts',(-0.153731161948265,1.81674675285051,
4.49638765529263));
#55081=CARTESIAN_POINT('Ctrl Pts',(-0.151864029219147,1.81574133369301,
4.49651727847567));
#55082=CARTESIAN_POINT('Ctrl Pts',(-0.133210569991579,1.8059330239884,4.49779520521927));
#55083=CARTESIAN_POINT('Ctrl Pts',(-0.115685945269864,1.79860753928493,
4.49886054912733));
#55084=CARTESIAN_POINT('Ctrl Pts',(-0.0958487973092332,1.79230270555119,
4.50002506625158));
#55085=CARTESIAN_POINT('Ctrl Pts',(-0.0940760399937242,1.79175607763204,
4.50012876922808));
#55086=CARTESIAN_POINT('Ctrl Pts',(-0.0902724485436537,1.7906191133431,
4.50035065485709));
#55087=CARTESIAN_POINT('Ctrl Pts',(-0.088240325712086,1.7900334003384,4.50046882658662));
#55088=CARTESIAN_POINT('Ctrl Pts',(-0.0838379982918046,1.78881133085156,
4.50072425673073));
#55089=CARTESIAN_POINT('Ctrl Pts',(-0.0814659975071729,1.78818196181416,
4.50086152785652));
#55090=CARTESIAN_POINT('Ctrl Pts',(-0.0762568713917799,1.78686330720148,
4.50116255987996));
#55091=CARTESIAN_POINT('Ctrl Pts',(-0.0734171113129211,1.78618536310497,
4.50132639265848));
#55092=CARTESIAN_POINT('Ctrl Pts',(-0.0512738315672547,1.7812160521037,
4.50260372406697));
#55093=CARTESIAN_POINT('Ctrl Pts',(-0.031624580851592,1.77867162528165,
4.50373981570125));
#55094=CARTESIAN_POINT('Ctrl Pts',(-0.0102723125877482,1.77788479691748,
4.50503521350223));
#55095=CARTESIAN_POINT('Ctrl Pts',(-0.00867649551879349,1.77783786264474,
4.5051323690496));
#55096=CARTESIAN_POINT('Ctrl Pts',(-0.00647980535113511,1.77778958946529,
4.50526659622268));
#55097=CARTESIAN_POINT('Ctrl Pts',(-0.00587916056410101,1.77777807027193,
4.50530334853987));
#55098=CARTESIAN_POINT('Ctrl Pts',(-0.00486822641532941,1.77776151012307,
4.50536529165778));
#55099=CARTESIAN_POINT('Ctrl Pts',(-0.00445795161193327,1.77775557312569,
4.50539045431464));
#55100=CARTESIAN_POINT('Ctrl Pts',(-0.00364843140309706,1.77774540501589,
4.50544015063562));
#55101=CARTESIAN_POINT('Ctrl Pts',(-0.00324918718173291,1.77774113228578,
4.50546468294935));
#55102=CARTESIAN_POINT('Ctrl Pts',(-0.00237200160275339,1.77773337486801,
4.50551863373672));
#55103=CARTESIAN_POINT('Ctrl Pts',(-0.00189405898876175,1.77773021146533,
4.50554806223401));
#55104=CARTESIAN_POINT('Ctrl Pts',(-0.000238787662817182,1.77772293794388,
4.50565009784488));
#55105=CARTESIAN_POINT('Ctrl Pts',(0.000938544586681608,1.77772421620278,
4.5057228736675));
#55106=CARTESIAN_POINT('Ctrl Pts',(0.0126705599419939,1.77780124202494,
4.50645013273548));
#55107=CARTESIAN_POINT('Ctrl Pts',(0.0232143808413407,1.77838900303163,
4.50712063283737));
#55108=CARTESIAN_POINT('Ctrl Pts',(0.0492137169969657,1.78112349321522,
4.50881827390047));
#55109=CARTESIAN_POINT('Ctrl Pts',(0.064577608017244,1.78387683625848,4.50986148372357));
#55110=CARTESIAN_POINT('Ctrl Pts',(0.0946031864249646,1.79153833225944,
4.51195559625379));
#55111=CARTESIAN_POINT('Ctrl Pts',(0.109234244934967,1.7964110092605,4.51300343283825));
#55112=CARTESIAN_POINT('Ctrl Pts',(0.12926124482282,1.80471685903077,4.51443735080164));
#55113=CARTESIAN_POINT('Ctrl Pts',(0.134990194753682,1.8072915083247,4.51484732751742));
#55114=CARTESIAN_POINT('Ctrl Pts',(0.142387251647469,1.8108792387982,4.51537312621331));
#55115=CARTESIAN_POINT('Ctrl Pts',(0.144126236527113,1.8117421772867,4.51549647230797));
#55116=CARTESIAN_POINT('Ctrl Pts',(0.146582072772296,1.81298862033187,4.5156701764144));
#55117=CARTESIAN_POINT('Ctrl Pts',(0.147305395143184,1.81335918519505,4.51572127722593));
#55118=CARTESIAN_POINT('Ctrl Pts',(0.14840861895822,1.81392965600966,4.51579911536518));
#55119=CARTESIAN_POINT('Ctrl Pts',(0.14878952920448,1.81412758808173,4.51582597194781));
#55120=CARTESIAN_POINT('Ctrl Pts',(0.149493707965175,1.81449528861242,4.51587558494555));
#55121=CARTESIAN_POINT('Ctrl Pts',(0.14981708495877,1.81466484618385,4.51589835439699));
#55122=CARTESIAN_POINT('Ctrl Pts',(0.150346248052047,1.81494345199662,4.51593558954295));
#55123=CARTESIAN_POINT('Ctrl Pts',(0.150552204228655,1.81505217378326,4.51595007590823));
#55124=CARTESIAN_POINT('Ctrl Pts',(0.150949392889979,1.81526239573457,4.51597800122498));
#55125=CARTESIAN_POINT('Ctrl Pts',(0.151140640615144,1.81536386516929,4.51599144205147));
#55126=CARTESIAN_POINT('Ctrl Pts',(0.151586931768654,1.81560122845572,4.51602279514631));
#55127=CARTESIAN_POINT('Ctrl Pts',(0.151841895716483,1.81573727320361,4.51604069778581));
#55128=CARTESIAN_POINT('Ctrl Pts',(0.15265736176679,1.81617380322568,4.5160979283893));
#55129=CARTESIAN_POINT('Ctrl Pts',(0.153217161984782,1.81647560710487,4.51613717290932));
#55130=CARTESIAN_POINT('Ctrl Pts',(0.158258887874711,1.81921303471953,4.5164902647909));
#55131=CARTESIAN_POINT('Ctrl Pts',(0.162683595728975,1.82175325649428,4.51679760408254));
#55132=CARTESIAN_POINT('Ctrl Pts',(0.167433248370488,1.82463208689165,4.51712678488508));
#55133=CARTESIAN_POINT('Ctrl Pts',(0.167819580790366,1.82486736191966,4.51715355479696));
#55134=CARTESIAN_POINT('Ctrl Pts',(0.192055871337686,1.83969721484594,4.51883269213715));
#55135=CARTESIAN_POINT('Ctrl Pts',(0.213908211452221,1.85733426529815,4.52034026122556));
#55136=CARTESIAN_POINT('Ctrl Pts',(0.243831900989314,1.8887087619504,4.52280023365836));
#55137=CARTESIAN_POINT('Ctrl Pts',(0.253640194960309,1.90058951255121,4.52369215267718));
#55138=CARTESIAN_POINT('Ctrl Pts',(0.263980035772892,1.91511706693387,4.5247677908075));
#55139=CARTESIAN_POINT('Ctrl Pts',(0.265375582445543,1.91712584119527,4.52491617885086));
#55140=CARTESIAN_POINT('Ctrl Pts',(0.267145037090441,1.91973573532518,4.52510860594292));
#55141=CARTESIAN_POINT('Ctrl Pts',(0.267540043399601,1.92032250801508,4.52515184499288));
#55142=CARTESIAN_POINT('Ctrl Pts',(0.268174319801933,1.92127143980358,4.52522173536099));
#55143=CARTESIAN_POINT('Ctrl Pts',(0.268414797074188,1.92163279242019,4.52524834117387));
#55144=CARTESIAN_POINT('Ctrl Pts',(0.268872018326673,1.92232285342988,4.52529913377999));
#55145=CARTESIAN_POINT('Ctrl Pts',(0.269088891529336,1.9226514756033,4.52532331566262));
#55146=CARTESIAN_POINT('Ctrl Pts',(0.269582789506912,1.92340285762271,4.52537859183644));
#55147=CARTESIAN_POINT('Ctrl Pts',(0.269859422537255,1.92382587262208,4.52540970071205));
#55148=CARTESIAN_POINT('Ctrl Pts',(0.270702959103565,1.92512241996806,4.5255050185312));
#55149=CARTESIAN_POINT('Ctrl Pts',(0.271266620592019,1.92599804432972,4.52556934810237));
#55150=CARTESIAN_POINT('Ctrl Pts',(0.275411781158541,1.93250647161751,4.5260472057192));
#55151=CARTESIAN_POINT('Ctrl Pts',(0.278821521692072,1.93824623788067,4.52646703391546));
#55152=CARTESIAN_POINT('Ctrl Pts',(0.282338608137678,1.94460874914244,4.52693120093886));
#55153=CARTESIAN_POINT('Ctrl Pts',(0.282625354636898,1.94513089592826,4.52696928421607));
#55154=CARTESIAN_POINT('Ctrl Pts',(0.284963396136583,1.94941643697788,4.52728178022675));
#55155=CARTESIAN_POINT('Ctrl Pts',(0.286940797829966,1.95321947514137,4.52755863460151));
#55156=CARTESIAN_POINT('Ctrl Pts',(0.301071213224542,1.98177322304823,4.52963367474962));
#55157=CARTESIAN_POINT('Ctrl Pts',(0.310077764914263,2.00795189407541,4.53153000844516));
#55158=CARTESIAN_POINT('Ctrl Pts',(0.317760004095797,2.04522883458338,4.53407014202454));
#55159=CARTESIAN_POINT('Ctrl Pts',(0.319375124750885,2.05560541692728,4.53475915640031));
#55160=CARTESIAN_POINT('Ctrl Pts',(0.320585116538556,2.06702525761937,4.53548524260158));
#55161=CARTESIAN_POINT('Ctrl Pts',(0.320684642660192,2.0680076477637,4.53554744368912));
#55162=CARTESIAN_POINT('Ctrl Pts',(0.320827258125165,2.06948294182772,4.53564044721951));
#55163=CARTESIAN_POINT('Ctrl Pts',(0.320873728940259,2.06997550201573,4.53567143062338));
#55164=CARTESIAN_POINT('Ctrl Pts',(0.320946794833823,2.07076950086914,4.53572126378663));
#55165=CARTESIAN_POINT('Ctrl Pts',(0.320974099721045,2.07107087101923,4.53574015256685));
#55166=CARTESIAN_POINT('Ctrl Pts',(0.321025765019208,2.07165019105327,4.53577641188889));
#55167=CARTESIAN_POINT('Ctrl Pts',(0.321050189003121,2.07192813479736,4.53579378597075));
#55168=CARTESIAN_POINT('Ctrl Pts',(0.321092794384865,2.072420311015,4.5358245117469));
#55169=CARTESIAN_POINT('Ctrl Pts',(0.321111122356962,2.07263452996741,4.53583787172114));
#55170=CARTESIAN_POINT('Ctrl Pts',(0.321147282533309,2.07306221185723,4.53586451770843));
#55171=CARTESIAN_POINT('Ctrl Pts',(0.321165116224875,2.0732756734519,4.53587780377392));
#55172=CARTESIAN_POINT('Ctrl Pts',(0.321213828891136,2.0738658344423,4.53591449963487));
#55173=CARTESIAN_POINT('Ctrl Pts',(0.321244258151676,2.07424257217133,4.53593788402296));
#55174=CARTESIAN_POINT('Ctrl Pts',(0.321360996281057,2.07572027075689,4.53602944836725));
#55175=CARTESIAN_POINT('Ctrl Pts',(0.321442310019689,2.0768216351914,4.53609735070477));
#55176=CARTESIAN_POINT('Ctrl Pts',(0.322866683562374,2.09756586122998,4.53737020625869));
#55177=CARTESIAN_POINT('Ctrl Pts',(0.322412765451218,2.11729400059599,4.53847928736019));
#55178=CARTESIAN_POINT('Ctrl Pts',(0.318285467855231,2.15314316759343,4.5404992695517));
#55179=CARTESIAN_POINT('Ctrl Pts',(0.315171292177117,2.1692594025311,4.54140942897139));
#55180=CARTESIAN_POINT('Ctrl Pts',(0.309294688855034,2.19073292954909,4.54268546926145));
#55181=CARTESIAN_POINT('Ctrl Pts',(0.307589917170555,2.19635406947532,4.54302543240003));
#55182=CARTESIAN_POINT('Ctrl Pts',(0.303401872052834,2.20891642579411,4.5438019245872));
#55183=CARTESIAN_POINT('Ctrl Pts',(0.300832208524172,2.21582509775483,4.54424077320023));
#55184=CARTESIAN_POINT('Ctrl Pts',(0.297434067949031,2.22408298909304,4.54478229419096));
#55185=CARTESIAN_POINT('Ctrl Pts',(0.296829492135799,2.22552237021234,4.5448773173132));
#55186=CARTESIAN_POINT('Ctrl Pts',(0.295979786774727,2.22750488776175,4.54500909465397));
#55187=CARTESIAN_POINT('Ctrl Pts',(0.295743566719805,2.22805183840413,4.54504554525152));
#55188=CARTESIAN_POINT('Ctrl Pts',(0.295342401668063,2.22897367618259,4.54510714119497));
#55189=CARTESIAN_POINT('Ctrl Pts',(0.295178255578197,2.22934891109889,4.54513225920044));
#55190=CARTESIAN_POINT('Ctrl Pts',(0.294852143655695,2.23009054341848,4.54518199379408));
#55191=CARTESIAN_POINT('Ctrl Pts',(0.294690209042942,2.23045695380928,4.54520660927791));
#55192=CARTESIAN_POINT('Ctrl Pts',(0.294331918435954,2.23126358889178,4.54526089577067));
#55193=CARTESIAN_POINT('Ctrl Pts',(0.294135257366237,2.23170367629269,4.54529057720867));
#55194=CARTESIAN_POINT('Ctrl Pts',(0.293445449579098,2.23323807435634,4.54539428707664));
#55195=CARTESIAN_POINT('Ctrl Pts',(0.292947181853805,2.23433005962283,4.54546849143462));
#55196=CARTESIAN_POINT('Ctrl Pts',(0.287654945151131,2.24575884081851,4.54624934514555));
#55197=CARTESIAN_POINT('Ctrl Pts',(0.282322642950932,2.25583606772135,4.54697469429424));
#55198=CARTESIAN_POINT('Ctrl Pts',(0.262322469519647,2.28922447973946,4.5495104820285));
#55199=CARTESIAN_POINT('Ctrl Pts',(0.245209377628064,2.31092883693061,4.55140397180431));
#55200=CARTESIAN_POINT('Ctrl Pts',(0.218054649140363,2.33753633856572,4.55394146292063));
#55201=CARTESIAN_POINT('Ctrl Pts',(0.210202416086392,2.34451244356362,4.55463064573098));
#55202=CARTESIAN_POINT('Ctrl Pts',(0.201253644195357,2.35171237762961,4.55535686228635));
#55203=CARTESIAN_POINT('Ctrl Pts',(0.200481572377854,2.35232774233007,4.55541905704884));
#55204=CARTESIAN_POINT('Ctrl Pts',(0.199318475409572,2.35324605747116,4.55551204616128));
#55205=CARTESIAN_POINT('Ctrl Pts',(0.19892956934423,2.35355166477946,4.55554302159676));
#55206=CARTESIAN_POINT('Ctrl Pts',(0.198301694463696,2.3540427229659,4.55559283927684));
#55207=CARTESIAN_POINT('Ctrl Pts',(0.198063167304039,2.35422873338466,4.5556117205588));
#55208=CARTESIAN_POINT('Ctrl Pts',(0.197606777482922,2.35458360728011,4.55564776229534));
#55209=CARTESIAN_POINT('Ctrl Pts',(0.197388959546763,2.35475252747195,4.55566492675871));
#55210=CARTESIAN_POINT('Ctrl Pts',(0.197000773153382,2.3550527735061,4.55569545049949));
#55211=CARTESIAN_POINT('Ctrl Pts',(0.196830489941176,2.35518420822371,4.55570881755598));
#55212=CARTESIAN_POINT('Ctrl Pts',(0.196491025074465,2.35544568546526,4.55573542010897));
#55213=CARTESIAN_POINT('Ctrl Pts',(0.196321846496122,2.35557572996395,4.55574865576223));
#55214=CARTESIAN_POINT('Ctrl Pts',(0.195855732115731,2.35593328770389,4.55578506138897));
#55215=CARTESIAN_POINT('Ctrl Pts',(0.195558527953201,2.3561604530478,4.55580820661613));
#55216=CARTESIAN_POINT('Ctrl Pts',(0.194404023995219,2.35703970754884,4.55589785579956));
#55217=CARTESIAN_POINT('Ctrl Pts',(0.193543840227857,2.35768802414824,4.5559640965188));
#55218=CARTESIAN_POINT('Ctrl Pts',(0.192556592926056,2.35842437579343,4.55603951158739));
#55219=CARTESIAN_POINT('Ctrl Pts',(0.192432711236372,2.35851663607969,4.55604896387689));
#55220=CARTESIAN_POINT('Ctrl Pts',(0.176345220602216,2.37047974535436,4.55727504247922));
#55221=CARTESIAN_POINT('Ctrl Pts',(0.159314025071371,2.38084912082708,4.55839404301133));
#55222=CARTESIAN_POINT('Ctrl Pts',(0.123860509620407,2.3981646991722,4.56060192419195));
#55223=CARTESIAN_POINT('Ctrl Pts',(0.105544873422519,2.40512920851287,4.56168752404402));
#55224=CARTESIAN_POINT('Ctrl Pts',(0.0784877550954512,2.41268795239035,
4.56331861799718));
#55225=CARTESIAN_POINT('Ctrl Pts',(0.0701765878628224,2.41465745008404,
4.56382269244057));
#55226=CARTESIAN_POINT('Ctrl Pts',(0.0601589745572409,2.41661468814422,
4.56443808780219));
#55227=CARTESIAN_POINT('Ctrl Pts',(0.0585179834362899,2.41692208572791,
4.56453913935081));
#55228=CARTESIAN_POINT('Ctrl Pts',(0.0556504919857703,2.41743620655454,
4.56471617541852));
#55229=CARTESIAN_POINT('Ctrl Pts',(0.0544250360756299,2.41764860753722,
4.56479197898809));
#55230=CARTESIAN_POINT('Ctrl Pts',(0.0526624736373075,2.41794360309979,
4.56490122499572));
#55231=CARTESIAN_POINT('Ctrl Pts',(0.0521263292292006,2.41803194285645,
4.56493448492785));
#55232=CARTESIAN_POINT('Ctrl Pts',(0.0511957384668416,2.41818285857508,
4.56499226568274));
#55233=CARTESIAN_POINT('Ctrl Pts',(0.0508013932965448,2.41824605820809,
4.5650167666638));
#55234=CARTESIAN_POINT('Ctrl Pts',(0.0500430867522277,2.41836614266802,
4.56506391186514));
#55235=CARTESIAN_POINT('Ctrl Pts',(0.0496791430923102,2.41842313683033,
4.56508655257814));
#55236=CARTESIAN_POINT('Ctrl Pts',(0.0488217516405681,2.41855589999861,
4.56513992304476));
#55237=CARTESIAN_POINT('Ctrl Pts',(0.0483282249879684,2.41863114650362,
4.56517066930899));
#55238=CARTESIAN_POINT('Ctrl Pts',(0.0468705708701003,2.41884992607259,
4.56526155609528));
#55239=CARTESIAN_POINT('Ctrl Pts',(0.0459059712172327,2.41899023110956,
4.56532179868413));
#55240=CARTESIAN_POINT('Ctrl Pts',(0.0373567378187211,2.4201941720082,4.56585662154304));
#55241=CARTESIAN_POINT('Ctrl Pts',(0.0297376352563984,2.42099141814585,
4.56633957241109));
#55242=CARTESIAN_POINT('Ctrl Pts',(0.0164784128669503,2.42190272585278,
4.56719198240653));
#55243=CARTESIAN_POINT('Ctrl Pts',(0.010850083851793,2.42214154155815,4.56755750914741));
#55244=CARTESIAN_POINT('Ctrl Pts',(-0.0195724645750351,2.42263424223003,
4.56955242233473));
#55245=CARTESIAN_POINT('Ctrl Pts',(-0.044325918813064,2.42017325086526,
4.57125300857453));
#55246=CARTESIAN_POINT('Ctrl Pts',(-0.0771812358358951,2.41302123406358,
4.57350370546215));
#55247=CARTESIAN_POINT('Ctrl Pts',(-0.0857340532573378,2.41078760200592,
4.57408795793851));
#55248=CARTESIAN_POINT('Ctrl Pts',(-0.0979308668506281,2.40706035852617,
4.57490912655983));
#55249=CARTESIAN_POINT('Ctrl Pts',(-0.101655884504313,2.40584735252556,
4.57515824850686));
#55250=CARTESIAN_POINT('Ctrl Pts',(-0.105868682425279,2.40439002881244,
4.57543734981006));
#55251=CARTESIAN_POINT('Ctrl Pts',(-0.106378862062687,2.40421210573421,
4.57547110513695));
#55252=CARTESIAN_POINT('Ctrl Pts',(-0.1071463820999,2.40394226934598,4.57552181738757));
#55253=CARTESIAN_POINT('Ctrl Pts',(-0.107404053759997,2.40385131154815,
4.57553883065291));
#55254=CARTESIAN_POINT('Ctrl Pts',(-0.107865550050935,2.40368774350185,
4.57556928020374));
#55255=CARTESIAN_POINT('Ctrl Pts',(-0.108069416789901,2.40361525586942,
4.57558272374858));
#55256=CARTESIAN_POINT('Ctrl Pts',(-0.108478292294501,2.40346941054224,
4.57560967084974));
#55257=CARTESIAN_POINT('Ctrl Pts',(-0.108683298832308,2.40339605071521,
4.5756231742007));
#55258=CARTESIAN_POINT('Ctrl Pts',(-0.109260566270517,2.40318882034475,
4.57566117635787));
#55259=CARTESIAN_POINT('Ctrl Pts',(-0.109632656885098,2.4030544714603,4.57568564659828));
#55260=CARTESIAN_POINT('Ctrl Pts',(-0.111166901631901,2.4024973139853,4.57578644584669));
#55261=CARTESIAN_POINT('Ctrl Pts',(-0.112326884428536,2.40206849577114,
4.57586242131542));
#55262=CARTESIAN_POINT('Ctrl Pts',(-0.133710823667689,2.39402314489708,
4.5772591602468));
#55263=CARTESIAN_POINT('Ctrl Pts',(-0.153124142202206,2.38439673994208,
4.5784655144129));
#55264=CARTESIAN_POINT('Ctrl Pts',(-0.180830571058473,2.36699199969083,
4.58029457413922));
#55265=CARTESIAN_POINT('Ctrl Pts',(-0.189919716259851,2.3606049020487,4.58091404916114));
#55266=CARTESIAN_POINT('Ctrl Pts',(-0.208035118612865,2.34642300458966,
4.58221957665366));
#55267=CARTESIAN_POINT('Ctrl Pts',(-0.216994636469219,2.33857115186426,
4.58290627110753));
#55268=CARTESIAN_POINT('Ctrl Pts',(-0.229429862357396,2.32639211731332,
4.5839397048306));
#55269=CARTESIAN_POINT('Ctrl Pts',(-0.233261516908457,2.32244215351955,
4.58427042418844));
#55270=CARTESIAN_POINT('Ctrl Pts',(-0.237607693179668,2.31772595285347,
4.58466112546756));
#55271=CARTESIAN_POINT('Ctrl Pts',(-0.23822251863537,2.31705307644062,4.58471677159636));
#55272=CARTESIAN_POINT('Ctrl Pts',(-0.239155897709731,2.31602282610005,
4.58480182954323));
#55273=CARTESIAN_POINT('Ctrl Pts',(-0.239476526683884,2.31566733171502,
4.58483115362675));
#55274=CARTESIAN_POINT('Ctrl Pts',(-0.240032502258556,2.31504813045852,
4.58488218646046));
#55275=CARTESIAN_POINT('Ctrl Pts',(-0.240268209950572,2.31478474768886,
4.58490387997611));
#55276=CARTESIAN_POINT('Ctrl Pts',(-0.240758418379112,2.31423516584687,
4.58494911794823));
#55277=CARTESIAN_POINT('Ctrl Pts',(-0.241012843059035,2.31394889993752,
4.58497266554279));
#55278=CARTESIAN_POINT('Ctrl Pts',(-0.241633761859633,2.31324776011363,
4.58503030125001));
#55279=CARTESIAN_POINT('Ctrl Pts',(-0.241999697497565,2.31283239525246,
4.58506441260506));
#55280=CARTESIAN_POINT('Ctrl Pts',(-0.243394687857498,2.31124072570819,
4.58519500327344));
#55281=CARTESIAN_POINT('Ctrl Pts',(-0.244416237815886,2.31005789875355,
4.58529179347486));
#55282=CARTESIAN_POINT('Ctrl Pts',(-0.262445993604225,2.28887210903096,
4.58702105726295));
#55283=CARTESIAN_POINT('Ctrl Pts',(-0.276951741692165,2.26687637185957,
4.58876020289764));
#55284=CARTESIAN_POINT('Ctrl Pts',(-0.294170264108086,2.23221293817648,
4.59137692502761));
#55285=CARTESIAN_POINT('Ctrl Pts',(-0.299061372503493,2.22074235227141,
4.59222284591545));
#55286=CARTESIAN_POINT('Ctrl Pts',(-0.307044154341661,2.19853495494782,
4.59379613557797));
#55287=CARTESIAN_POINT('Ctrl Pts',(-0.310266642655159,2.18786308314059,
4.59452540731873));
#55288=CARTESIAN_POINT('Ctrl Pts',(-0.313100194145897,2.17635410698771,
4.59526905477803));
#55289=CARTESIAN_POINT('Ctrl Pts',(-0.313267899292191,2.17566309882598,
4.59531354140973));
#55290=CARTESIAN_POINT('Ctrl Pts',(-0.313504456451249,2.17467412485468,
4.59537697297875));
#55291=CARTESIAN_POINT('Ctrl Pts',(-0.313575171988812,2.17437661360702,
4.59539602424065));
#55292=CARTESIAN_POINT('Ctrl Pts',(-0.31369669186866,2.17386210667814,4.59542891724439));
#55293=CARTESIAN_POINT('Ctrl Pts',(-0.313747694693875,2.17364515848125,
4.59544277049775));
#55294=CARTESIAN_POINT('Ctrl Pts',(-0.313845525207081,2.17322707545613,
4.59546943527407));
#55295=CARTESIAN_POINT('Ctrl Pts',(-0.313892384510236,2.1730259489459,4.5954822486356));
#55296=CARTESIAN_POINT('Ctrl Pts',(-0.314003180742505,2.17254831941527,
4.59551264399341));
#55297=CARTESIAN_POINT('Ctrl Pts',(-0.314066945951606,2.17227177615401,
4.59553021603536));
#55298=CARTESIAN_POINT('Ctrl Pts',(-0.314290128697797,2.1712979817325,4.59559200017891));
#55299=CARTESIAN_POINT('Ctrl Pts',(-0.314447591796843,2.17060027784849,
4.59563610049465));
#55300=CARTESIAN_POINT('Ctrl Pts',(-0.316547933216148,2.1611474338762,4.59623140901051));
#55301=CARTESIAN_POINT('Ctrl Pts',(-0.318127068217185,2.15231448505691,
4.59676235231723));
#55302=CARTESIAN_POINT('Ctrl Pts',(-0.321279572688121,2.12913249526383,
4.59811708324573));
#55303=CARTESIAN_POINT('Ctrl Pts',(-0.322261603439283,2.11472339687742,
4.59892147974423));
#55304=CARTESIAN_POINT('Ctrl Pts',(-0.322299026505738,2.07400756785731,
4.60119725886281));
#55305=CARTESIAN_POINT('Ctrl Pts',(-0.319106828542065,2.04781913843993,
4.60267310959814));
#55306=CARTESIAN_POINT('Ctrl Pts',(-0.312368014685267,2.02068928395737,
4.60436678591414));
#55307=CARTESIAN_POINT('Ctrl Pts',(-0.311952714799364,2.01907120510316,
4.60446839672546));
#55308=CARTESIAN_POINT('Ctrl Pts',(-0.311362874120434,2.01684510702386,
4.60460903767301));
#55309=CARTESIAN_POINT('Ctrl Pts',(-0.311199090208047,2.01623424416204,
4.60464771926073));
#55310=CARTESIAN_POINT('Ctrl Pts',(-0.310935168011888,2.01526135469867,
4.60470946771727));
#55311=CARTESIAN_POINT('Ctrl Pts',(-0.310836192490293,2.0148990120487,4.60473249681103));
#55312=CARTESIAN_POINT('Ctrl Pts',(-0.310631776091599,2.01415577184085,
4.60477979934079));
#55313=CARTESIAN_POINT('Ctrl Pts',(-0.310526267584728,2.0137748936574,4.6048040749418));
#55314=CARTESIAN_POINT('Ctrl Pts',(-0.310281018652486,2.0128958509323,4.60486018306977));
#55315=CARTESIAN_POINT('Ctrl Pts',(-0.310140778941195,2.01239782791733,
4.60489203179511));
#55316=CARTESIAN_POINT('Ctrl Pts',(-0.309697752560719,2.01083893898023,
4.60499191439398));
#55317=CARTESIAN_POINT('Ctrl Pts',(-0.309390719785355,2.00977929724539,
4.60506008647354));
#55318=CARTESIAN_POINT('Ctrl Pts',(-0.304901515995812,1.99457843748915,
4.60604208251637));
#55319=CARTESIAN_POINT('Ctrl Pts',(-0.299759637922862,1.98074108866683,
4.60698767135027));
#55320=CARTESIAN_POINT('Ctrl Pts',(-0.286766629181926,1.95198390853262,
4.60906713271287));
#55321=CARTESIAN_POINT('Ctrl Pts',(-0.278655926364474,1.93722821147532,
4.61020604344051));
#55322=CARTESIAN_POINT('Ctrl Pts',(-0.259274656885136,1.90769674605257,
4.6125951384316));
#55323=CARTESIAN_POINT('Ctrl Pts',(-0.247801096856571,1.89312157228115,
4.61384048601969));
#55324=CARTESIAN_POINT('Ctrl Pts',(-0.234428109079249,1.87885363507568,
4.61507192906011));
#55325=CARTESIAN_POINT('Ctrl Pts',(-0.233714610064458,1.87809972023885,
4.61513703212251));
#55326=CARTESIAN_POINT('Ctrl Pts',(-0.232742862269487,1.87708281469978,
4.61522487493555));
#55327=CARTESIAN_POINT('Ctrl Pts',(-0.232487796699551,1.87681681105292,
4.61524785575522));
#55328=CARTESIAN_POINT('Ctrl Pts',(-0.232085083044099,1.87639826717924,
4.61528401846936));
#55329=CARTESIAN_POINT('Ctrl Pts',(-0.231937740557124,1.87624543535846,
4.6152972240691));
#55330=CARTESIAN_POINT('Ctrl Pts',(-0.231652795611825,1.87595045849294,
4.61532271309303));
#55331=CARTESIAN_POINT('Ctrl Pts',(-0.231515214329933,1.87580829565245,
4.61533499794245));
#55332=CARTESIAN_POINT('Ctrl Pts',(-0.231186110477615,1.87546885840849,
4.61536433146544));
#55333=CARTESIAN_POINT('Ctrl Pts',(-0.230994466437707,1.87527170249685,
4.61538137047583));
#55334=CARTESIAN_POINT('Ctrl Pts',(-0.230419757571968,1.87468197632246,
4.61543234139994));
#55335=CARTESIAN_POINT('Ctrl Pts',(-0.230035940138853,1.87429013595239,
4.61546621461641));
#55336=CARTESIAN_POINT('Ctrl Pts',(-0.226716140520434,1.87091820647289,
4.61575777720764));
#55337=CARTESIAN_POINT('Ctrl Pts',(-0.223723221455666,1.86799439499913,
4.6160110738012));
#55338=CARTESIAN_POINT('Ctrl Pts',(-0.214381593815384,1.85921740940135,
4.61677617419931));
#55339=CARTESIAN_POINT('Ctrl Pts',(-0.207853577369733,1.85356007302027,
4.61727608034494));
#55340=CARTESIAN_POINT('Ctrl Pts',(-0.184251942007615,1.83471223975982,
4.61899762475195));
#55341=CARTESIAN_POINT('Ctrl Pts',(-0.166089431374551,1.8229788198299,4.62017786115513));
#55342=CARTESIAN_POINT('Ctrl Pts',(-0.132535560478973,1.80579667449252,
4.62232136031678));
#55343=CARTESIAN_POINT('Ctrl Pts',(-0.11765119019602,1.7995347634027,4.62326037122781));
#55344=CARTESIAN_POINT('Ctrl Pts',(-0.101164914717352,1.794012370056,4.6243166338652));
#55345=CARTESIAN_POINT('Ctrl Pts',(-0.0999654141651552,1.79361839880892,
4.62439356419384));
#55346=CARTESIAN_POINT('Ctrl Pts',(-0.0982824005210525,1.79307655519359,
4.62450162589741));
#55347=CARTESIAN_POINT('Ctrl Pts',(-0.0978007965386315,1.79292275334075,
4.62453256220524));
#55348=CARTESIAN_POINT('Ctrl Pts',(-0.0969660799568446,1.79265834664908,
4.62458620574611));
#55349=CARTESIAN_POINT('Ctrl Pts',(-0.0966131341034557,1.79254721522886,
4.62460889564694));
#55350=CARTESIAN_POINT('Ctrl Pts',(-0.09587990092875,1.79231773068773,4.62465604933553));
#55351=CARTESIAN_POINT('Ctrl Pts',(-0.0954995841951934,1.79219947422466,
4.62468051624962));
#55352=CARTESIAN_POINT('Ctrl Pts',(-0.0946061665433012,1.79192348835285,
4.62473801411775));
#55353=CARTESIAN_POINT('Ctrl Pts',(-0.0940928899854948,1.7917663356716,
4.62477106389711));
#55354=CARTESIAN_POINT('Ctrl Pts',(-0.0924241912953026,1.7912599775936,
4.62487856689298));
#55355=CARTESIAN_POINT('Ctrl Pts',(-0.0912672098014756,1.79091598403735,
4.62495319024206));
#55356=CARTESIAN_POINT('Ctrl Pts',(-0.0760782504437914,1.78649272367566,
4.62593405077409));
#55357=CARTESIAN_POINT('Ctrl Pts',(-0.061788615253312,1.78336650396834,
4.62687142269172));
#55358=CARTESIAN_POINT('Ctrl Pts',(-0.0306958863038654,1.77874931602146,
4.62894295983905));
#55359=CARTESIAN_POINT('Ctrl Pts',(-0.013887026758127,1.77758519350702,
4.63008269858988));
#55360=CARTESIAN_POINT('Ctrl Pts',(0.0214220791628359,1.77790669745729,
4.6324708735153));
#55361=CARTESIAN_POINT('Ctrl Pts',(0.0398635927146037,1.77966568542667,
4.63371446601899));
#55362=CARTESIAN_POINT('Ctrl Pts',(0.0590672106276965,1.78318254397015,
4.63494377210031));
#55363=CARTESIAN_POINT('Ctrl Pts',(0.0600791442978562,1.78337288128574,
4.63500834915202));
#55364=CARTESIAN_POINT('Ctrl Pts',(0.0614509764940646,1.78363772641091,
4.6350956039724));
#55365=CARTESIAN_POINT('Ctrl Pts',(0.0618116711996511,1.78370800204677,
4.63511851862635));
#55366=CARTESIAN_POINT('Ctrl Pts',(0.0623803427114498,1.78381980858071,
4.63515460214095));
#55367=CARTESIAN_POINT('Ctrl Pts',(0.062588398669669,1.78386092782553,4.63516779452849));
#55368=CARTESIAN_POINT('Ctrl Pts',(0.0629905290240198,1.78394081559652,
4.63519327469142));
#55369=CARTESIAN_POINT('Ctrl Pts',(0.0631846068119249,1.78397955722021,
4.63520556386088));
#55370=CARTESIAN_POINT('Ctrl Pts',(0.0636487278928227,1.78407264927036,
4.63523493302334));
#55371=CARTESIAN_POINT('Ctrl Pts',(0.0639187370909483,1.78412716712025,
4.63525200328792));
#55372=CARTESIAN_POINT('Ctrl Pts',(0.064728604533257,1.78429176928048,4.63530315782323));
#55373=CARTESIAN_POINT('Ctrl Pts',(0.0652682542201548,1.78440289261378,
4.63533718276731));
#55374=CARTESIAN_POINT('Ctrl Pts',(0.0699864197292205,1.78538706505165,
4.63563414586314));
#55375=CARTESIAN_POINT('Ctrl Pts',(0.0741477362072086,1.78634172207099,
4.63589250816159));
#55376=CARTESIAN_POINT('Ctrl Pts',(0.0866041041611286,1.7894611455429,4.63665851176773));
#55377=CARTESIAN_POINT('Ctrl Pts',(0.0948333957680858,1.79187453699471,
4.6371546834383));
#55378=CARTESIAN_POINT('Ctrl Pts',(0.121871621331492,1.80099013403117,4.63878085445742));
#55379=CARTESIAN_POINT('Ctrl Pts',(0.140153026986773,1.8091103756087,4.63987617315425));
#55380=CARTESIAN_POINT('Ctrl Pts',(0.164519052022037,1.8227669117983,4.64145749701418));
#55381=CARTESIAN_POINT('Ctrl Pts',(0.17132462644364,1.8269202220289,4.64191331240111));
#55382=CARTESIAN_POINT('Ctrl Pts',(0.186236716628233,1.83679778107081,4.64295356414291));
#55383=CARTESIAN_POINT('Ctrl Pts',(0.19424653956578,1.84265242526862,4.64354173476242));
#55384=CARTESIAN_POINT('Ctrl Pts',(0.202786776778855,1.84952088143951,4.64420813967507));
#55385=CARTESIAN_POINT('Ctrl Pts',(0.203597164951073,1.85017914407529,4.64427178102764));
#55386=CARTESIAN_POINT('Ctrl Pts',(0.20480391789763,1.8511691378325,4.644367164899));
#55387=CARTESIAN_POINT('Ctrl Pts',(0.205202711991843,1.85149790797758,4.64439878752968));
#55388=CARTESIAN_POINT('Ctrl Pts',(0.20588793309469,1.85206558579343,4.64445329802884));
#55389=CARTESIAN_POINT('Ctrl Pts',(0.206174740260987,1.85230403471518,4.64447616720529));
#55390=CARTESIAN_POINT('Ctrl Pts',(0.206759501683683,1.85279191946094,4.64452290347942));
#55391=CARTESIAN_POINT('Ctrl Pts',(0.207057419982652,1.85304139729833,4.64454677227234));
#55392=CARTESIAN_POINT('Ctrl Pts',(0.207745912683269,1.8536200651365,4.64460206836851));
#55393=CARTESIAN_POINT('Ctrl Pts',(0.208136156306218,1.85394964545194,4.64463351164323));
#55394=CARTESIAN_POINT('Ctrl Pts',(0.20895482807744,1.85464439613383,4.6446996883537));
#55395=CARTESIAN_POINT('Ctrl Pts',(0.209383085895758,1.8550097637461,4.64473442986127));
#55396=CARTESIAN_POINT('Ctrl Pts',(0.210519143736123,1.85598414472606,4.64482692085497));
#55397=CARTESIAN_POINT('Ctrl Pts',(0.211225254064813,1.85659511196311,4.64488475112242));
#55398=CARTESIAN_POINT('Ctrl Pts',(0.226687429799513,1.87009182522492,4.64615871340064));
#55399=CARTESIAN_POINT('Ctrl Pts',(0.240237970170727,1.88429088100175,4.64743212855514));
#55400=CARTESIAN_POINT('Ctrl Pts',(0.270803958182613,1.92279597791174,4.65072014737897));
#55401=CARTESIAN_POINT('Ctrl Pts',(0.285917071594265,1.9483835019075,4.65277360865473));
#55402=CARTESIAN_POINT('Ctrl Pts',(0.297897221732843,1.97703416707449,4.65473729202593));
#55403=CARTESIAN_POINT('Ctrl Pts',(0.298456848714247,1.9783987646595,4.6548300391783));
#55404=CARTESIAN_POINT('Ctrl Pts',(0.299165215498802,1.98016040270523,4.65494872468456));
#55405=CARTESIAN_POINT('Ctrl Pts',(0.299322555661424,1.98055393300142,4.65497517072323));
#55406=CARTESIAN_POINT('Ctrl Pts',(0.299570806395052,1.98117841449606,4.65501702970987));
#55407=CARTESIAN_POINT('Ctrl Pts',(0.29966222656197,1.98140916056131,4.65503247339567));
#55408=CARTESIAN_POINT('Ctrl Pts',(0.299825665835762,1.98182307979224,4.65506013482778));
#55409=CARTESIAN_POINT('Ctrl Pts',(0.299897783174249,1.98200621198075,4.65507235848008));
#55410=CARTESIAN_POINT('Ctrl Pts',(0.300067076222544,1.98243726653436,4.65510109585825));
#55411=CARTESIAN_POINT('Ctrl Pts',(0.300164112315517,1.98268524299252,4.65511760104362));
#55412=CARTESIAN_POINT('Ctrl Pts',(0.300444940144499,1.9834055300544,4.65516546595973));
#55413=CARTESIAN_POINT('Ctrl Pts',(0.300627926301566,1.9838781570236,4.65519677718011));
#55414=CARTESIAN_POINT('Ctrl Pts',(0.301895846891044,1.98717609867468,4.65541460765242));
#55415=CARTESIAN_POINT('Ctrl Pts',(0.302942096851317,1.99001626194707,4.6555988496368));
#55416=CARTESIAN_POINT('Ctrl Pts',(0.306066871507953,1.99888191474616,4.65616484819768));
#55417=CARTESIAN_POINT('Ctrl Pts',(0.308006882444144,2.00495491315872,4.6565396150681));
#55418=CARTESIAN_POINT('Ctrl Pts',(0.314128170108212,2.02627974410496,4.65782373099043));
#55419=CARTESIAN_POINT('Ctrl Pts',(0.317366622463534,2.04177907990649,4.6587020689851));
#55420=CARTESIAN_POINT('Ctrl Pts',(0.322762261479198,2.08229228629075,4.66098751549565));
#55421=CARTESIAN_POINT('Ctrl Pts',(0.323161917841359,2.10742696744241,4.66240212454196));
#55422=CARTESIAN_POINT('Ctrl Pts',(0.320497480109653,2.13383428389503,4.66401208311936));
#55423=CARTESIAN_POINT('Ctrl Pts',(0.320337709099968,2.135314947768,4.66410273651061));
#55424=CARTESIAN_POINT('Ctrl Pts',(0.320105751795304,2.13733333013961,4.66422685081282));
#55425=CARTESIAN_POINT('Ctrl Pts',(0.320042460144643,2.13787206847587,4.66426003135707));
#55426=CARTESIAN_POINT('Ctrl Pts',(0.319932530391134,2.1387878324401,4.66431652282108));
#55427=CARTESIAN_POINT('Ctrl Pts',(0.319886585078825,2.13916494136957,4.66433981185553));
#55428=CARTESIAN_POINT('Ctrl Pts',(0.319792647454913,2.1399247671823,4.66438678905129));
#55429=CARTESIAN_POINT('Ctrl Pts',(0.319744634643312,2.14030748088862,4.66441047782506));
#55430=CARTESIAN_POINT('Ctrl Pts',(0.31963403662193,2.14117643261107,4.66446432497043));
#55431=CARTESIAN_POINT('Ctrl Pts',(0.31957102884465,2.14166261500123,4.66449449664035));
#55432=CARTESIAN_POINT('Ctrl Pts',(0.319436910891427,2.14267929319894,4.66455768269616));
#55433=CARTESIAN_POINT('Ctrl Pts',(0.31936558804735,2.14320975900721,4.66459070372861));
#55434=CARTESIAN_POINT('Ctrl Pts',(0.319175221626972,2.14459939312543,4.66467734689045));
#55435=CARTESIAN_POINT('Ctrl Pts',(0.319054030966084,2.14545825852875,4.66473103683525));
#55436=CARTESIAN_POINT('Ctrl Pts',(0.318683923880575,2.14800676115965,4.6648907714494));
#55437=CARTESIAN_POINT('Ctrl Pts',(0.318425044839465,2.14969490009154,4.66499713056754));
#55438=CARTESIAN_POINT('Ctrl Pts',(0.315434455823464,2.1682127658467,4.66616999668355));
#55439=CARTESIAN_POINT('Ctrl Pts',(0.31138518744132,2.18479962864227,4.66727885149815));
#55440=CARTESIAN_POINT('Ctrl Pts',(0.297230501974381,2.22769610971411,4.67029278758103));
#55441=CARTESIAN_POINT('Ctrl Pts',(0.284958865483838,2.25313622796883,4.672241951265));
#55442=CARTESIAN_POINT('Ctrl Pts',(0.267546094463786,2.27970394409235,4.67428443061787));
#55443=CARTESIAN_POINT('Ctrl Pts',(0.265499628615286,2.28271390248755,4.6745157356746));
#55444=CARTESIAN_POINT('Ctrl Pts',(0.263069784324188,2.28616067701977,4.67477990000651));
#55445=CARTESIAN_POINT('Ctrl Pts',(0.262735787982972,2.2866317626185,4.67481598887121));
#55446=CARTESIAN_POINT('Ctrl Pts',(0.262237506826088,2.28733057540571,4.6748694970489));
#55447=CARTESIAN_POINT('Ctrl Pts',(0.262074190014144,2.28755898644978,4.67488698230461));
#55448=CARTESIAN_POINT('Ctrl Pts',(0.261782900219347,2.28796525420165,4.6749180748701));
#55449=CARTESIAN_POINT('Ctrl Pts',(0.261655044443343,2.28814319374556,4.67493169024392));
#55450=CARTESIAN_POINT('Ctrl Pts',(0.261383359098157,2.28852049130286,4.67496055395379));
#55451=CARTESIAN_POINT('Ctrl Pts',(0.261239483285007,2.28871981461537,4.6749757989636));
#55452=CARTESIAN_POINT('Ctrl Pts',(0.260853150421691,2.28925374576728,4.67501662735212));
#55453=CARTESIAN_POINT('Ctrl Pts',(0.260610276632537,2.28958805365819,4.67504218185907));
#55454=CARTESIAN_POINT('Ctrl Pts',(0.259448110138156,2.29118128503546,4.67516392946409));
#55455=CARTESIAN_POINT('Ctrl Pts',(0.258520314224159,2.29243402237016,4.67525954140931));
#55456=CARTESIAN_POINT('Ctrl Pts',(0.250781443599317,2.30272628208356,4.67604455355918));
#55457=CARTESIAN_POINT('Ctrl Pts',(0.243506784677752,2.31140904268779,4.67670357887331));
#55458=CARTESIAN_POINT('Ctrl Pts',(0.233014739499046,2.32266987799107,4.67758142280991));
#55459=CARTESIAN_POINT('Ctrl Pts',(0.23018379125078,2.3255951395105,4.67781175694168));
#55460=CARTESIAN_POINT('Ctrl Pts',(0.214761491605272,2.34093860104124,4.67903711657215));
#55461=CARTESIAN_POINT('Ctrl Pts',(0.201219721161123,2.35235794525604,4.68001284188649));
#55462=CARTESIAN_POINT('Ctrl Pts',(0.173682591858064,2.37194677357373,4.68193448394837));
#55463=CARTESIAN_POINT('Ctrl Pts',(0.159875810243121,2.38028611346861,4.68287249711085));
#55464=CARTESIAN_POINT('Ctrl Pts',(0.14437829177132,2.38812788553139,4.68392766341475));
#55465=CARTESIAN_POINT('Ctrl Pts',(0.143248459144363,2.3886912683776,4.68400459154756));
#55466=CARTESIAN_POINT('Ctrl Pts',(0.141661602715333,2.38947093383952,4.68411265091945));
#55467=CARTESIAN_POINT('Ctrl Pts',(0.141207325774261,2.38969280689186,4.68414358710722));
#55468=CARTESIAN_POINT('Ctrl Pts',(0.140419655457845,2.39007521939989,4.68419723071261));
#55469=CARTESIAN_POINT('Ctrl Pts',(0.140086503264321,2.39023625574714,4.68421992079886));
#55470=CARTESIAN_POINT('Ctrl Pts',(0.139401403631416,2.39056595913233,4.68426658354593));
#55471=CARTESIAN_POINT('Ctrl Pts',(0.139049425773298,2.3907345612942,4.68429055841434));
#55472=CARTESIAN_POINT('Ctrl Pts',(0.138226718983486,2.39112681324392,4.68434660041197));
#55473=CARTESIAN_POINT('Ctrl Pts',(0.137755753100695,2.39134996089424,4.68437868487787));
#55474=CARTESIAN_POINT('Ctrl Pts',(0.136761938317653,2.39181789037348,4.68444639494943));
#55475=CARTESIAN_POINT('Ctrl Pts',(0.136238969293794,2.39206241140081,4.68448202945224));
#55476=CARTESIAN_POINT('Ctrl Pts',(0.134836996976981,2.3927133370451,4.68457756995864));
#55477=CARTESIAN_POINT('Ctrl Pts',(0.133956819288346,2.39311718470795,4.68463756395158));
#55478=CARTESIAN_POINT('Ctrl Pts',(0.131267936224006,2.39433627124205,4.68482088614121));
#55479=CARTESIAN_POINT('Ctrl Pts',(0.12945353735844,2.39513876910877,4.68494464951488));
#55480=CARTESIAN_POINT('Ctrl Pts',(0.0999151119131207,2.40787865824408,
4.68696077727994));
#55481=CARTESIAN_POINT('Ctrl Pts',(0.0706616876727685,2.4158771888731,4.68899680475839));
#55482=CARTESIAN_POINT('Ctrl Pts',(0.0260240969215149,2.42156456831388,
4.69203793276011));
#55483=CARTESIAN_POINT('Ctrl Pts',(0.0112023207511253,2.4224214970483,4.69303316923491));
#55484=CARTESIAN_POINT('Ctrl Pts',(-0.00695842717649646,2.4222170935713,
4.69419847524837));
#55485=CARTESIAN_POINT('Ctrl Pts',(-0.0102891855150253,2.42212794027649,
4.69440992858046));
#55486=CARTESIAN_POINT('Ctrl Pts',(-0.0141728397428451,2.42196368507066,
4.69465337243868));
#55487=CARTESIAN_POINT('Ctrl Pts',(-0.0147275039674132,2.42193879003388,
4.69468806703854));
#55488=CARTESIAN_POINT('Ctrl Pts',(-0.0155619406349865,2.42189917693679,
4.6947401472688));
#55489=CARTESIAN_POINT('Ctrl Pts',(-0.0158417591231338,2.42188552744451,
4.69475759241391));
#55490=CARTESIAN_POINT('Ctrl Pts',(-0.0163403256655439,2.42186055576958,
4.69478864039519));
#55491=CARTESIAN_POINT('Ctrl Pts',(-0.0165590798269971,2.42184937545304,
4.69480225120741));
#55492=CARTESIAN_POINT('Ctrl Pts',(-0.0170236935492711,2.42182515454647,
4.69483113373689));
#55493=CARTESIAN_POINT('Ctrl Pts',(-0.017269548905499,2.42181205527838,
4.69484640206994));
#55494=CARTESIAN_POINT('Ctrl Pts',(-0.0179296832100263,2.42177612439762,
4.69488735817403));
#55495=CARTESIAN_POINT('Ctrl Pts',(-0.0183439352442097,2.42175277437296,
4.69491301675766));
#55496=CARTESIAN_POINT('Ctrl Pts',(-0.0203327488817649,2.42163681810002,
4.69503600394895));
#55497=CARTESIAN_POINT('Ctrl Pts',(-0.0219066964851299,2.42153345132637,
4.69513273696171));
#55498=CARTESIAN_POINT('Ctrl Pts',(-0.0350170550928157,2.42057573002211,
4.69593396012065));
#55499=CARTESIAN_POINT('Ctrl Pts',(-0.0465019223588754,2.4191122484282,
4.69660673674212));
#55500=CARTESIAN_POINT('Ctrl Pts',(-0.0657090124969458,2.41560539687204,
4.69771919109732));
#55501=CARTESIAN_POINT('Ctrl Pts',(-0.0734782777856998,2.41388754536831,
4.69816558584579));
#55502=CARTESIAN_POINT('Ctrl Pts',(-0.0908731623428266,2.40936005653806,
4.69917135699064));
#55503=CARTESIAN_POINT('Ctrl Pts',(-0.100447052820797,2.40638531697912,
4.69972949918874));
#55504=CARTESIAN_POINT('Ctrl Pts',(-0.128265513933019,2.39629742999938,
4.70139718930113));
#55505=CARTESIAN_POINT('Ctrl Pts',(-0.146015461841703,2.38796444472437,
4.70252435249028));
#55506=CARTESIAN_POINT('Ctrl Pts',(-0.164015571338357,2.37741979672301,
4.70379142741676));
#55507=CARTESIAN_POINT('Ctrl Pts',(-0.165128528534599,2.37675877627077,
4.70387029084024));
#55508=CARTESIAN_POINT('Ctrl Pts',(-0.166675245351863,2.37582748113571,
4.7039806283394));
#55509=CARTESIAN_POINT('Ctrl Pts',(-0.167112400493743,2.37556284647834,
4.70401189626538));
#55510=CARTESIAN_POINT('Ctrl Pts',(-0.16786622551124,2.37510406018809,4.70406595821423));
#55511=CARTESIAN_POINT('Ctrl Pts',(-0.168183193461786,2.37491039819273,
4.70408873425139));
#55512=CARTESIAN_POINT('Ctrl Pts',(-0.168831757256897,2.37451259533248,
4.70413542818665));
#55513=CARTESIAN_POINT('Ctrl Pts',(-0.169163319262705,2.37430840065258,
4.70415934803914));
#55514=CARTESIAN_POINT('Ctrl Pts',(-0.169933336135604,2.37383225357167,
4.70421501319779));
#55515=CARTESIAN_POINT('Ctrl Pts',(-0.17037150870673,2.37355984873948,4.70424677515324));
#55516=CARTESIAN_POINT('Ctrl Pts',(-0.171292476621976,2.37298422685196,
4.7043137160109));
#55517=CARTESIAN_POINT('Ctrl Pts',(-0.171775124849703,2.37268077881185,
4.70434890339712));
#55518=CARTESIAN_POINT('Ctrl Pts',(-0.173060744986607,2.37186772268018,
4.70444291582998));
#55519=CARTESIAN_POINT('Ctrl Pts',(-0.173862266021968,2.37135584112599,
4.70450182521601));
#55520=CARTESIAN_POINT('Ctrl Pts',(-0.176288355197909,2.36979128744708,
4.70468104698536));
#55521=CARTESIAN_POINT('Ctrl Pts',(-0.177905692503867,2.3687275335206,4.70480177206373));
#55522=CARTESIAN_POINT('Ctrl Pts',(-0.204629980063425,2.35080345996794,
4.70681770899292));
#55523=CARTESIAN_POINT('Ctrl Pts',(-0.227245378051158,2.33050924126038,
4.70885731178849));
#55524=CARTESIAN_POINT('Ctrl Pts',(-0.256249319694636,2.29600477968466,
4.71190371340892));
#55525=CARTESIAN_POINT('Ctrl Pts',(-0.265006514246938,2.28399245517173,
4.71290030552239));
#55526=CARTESIAN_POINT('Ctrl Pts',(-0.274681802839067,2.26858897876081,
4.71406749375441));
#55527=CARTESIAN_POINT('Ctrl Pts',(-0.276414764126198,2.26573236529977,
4.71427954070437));
#55528=CARTESIAN_POINT('Ctrl Pts',(-0.278383866661579,2.26236966217774,
4.71452359260699));
#55529=CARTESIAN_POINT('Ctrl Pts',(-0.278663423404615,2.2618894094144,4.71455831674827));
#55530=CARTESIAN_POINT('Ctrl Pts',(-0.279082100035496,2.26116586364756,
4.71461043272201));
#55531=CARTESIAN_POINT('Ctrl Pts',(-0.279222145190115,2.26092311146118,
4.71462788418872));
#55532=CARTESIAN_POINT('Ctrl Pts',(-0.279471088676323,2.26049029317157,
4.71465893921821));
#55533=CARTESIAN_POINT('Ctrl Pts',(-0.279580109807511,2.26030029884351,
4.71467255077093));
#55534=CARTESIAN_POINT('Ctrl Pts',(-0.279811225277397,2.25989657413593,
4.71470143037109));
#55535=CARTESIAN_POINT('Ctrl Pts',(-0.27993326814201,2.25968281560628,4.71471669504349));
#55536=CARTESIAN_POINT('Ctrl Pts',(-0.280260240178963,2.25910859601858,
4.71475763110251));
#55537=CARTESIAN_POINT('Ctrl Pts',(-0.280464719663853,2.25874787740508,
4.71478327335133));
#55538=CARTESIAN_POINT('Ctrl Pts',(-0.281442251445843,2.25701564689641,
4.7149060651389));
#55539=CARTESIAN_POINT('Ctrl Pts',(-0.282205960011085,2.25563884682263,
4.71500262137186));
#55540=CARTESIAN_POINT('Ctrl Pts',(-0.288477484608659,2.24413470796355,
4.71580126160416));
#55541=CARTESIAN_POINT('Ctrl Pts',(-0.293449001894129,2.23372291856966,
4.71647184744707));
#55542=CARTESIAN_POINT('Ctrl Pts',(-0.311817612255427,2.18926600017448,
4.71921301145395));
#55543=CARTESIAN_POINT('Ctrl Pts',(-0.319927756985202,2.15333862351635,
4.72117565196667));
#55544=CARTESIAN_POINT('Ctrl Pts',(-0.321945817749436,2.11471374155642,
4.72351278071896));
#55545=CARTESIAN_POINT('Ctrl Pts',(-0.322035026497539,2.11261131002231,
4.72364056323453));
#55546=CARTESIAN_POINT('Ctrl Pts',(-0.322126306221127,2.10981334754542,
4.72381142215885));
#55547=CARTESIAN_POINT('Ctrl Pts',(-0.322146726029427,2.10911843442186,
4.72385392318663));
#55548=CARTESIAN_POINT('Ctrl Pts',(-0.322175041291975,2.10803548533588,
4.72392026093351));
#55549=CARTESIAN_POINT('Ctrl Pts',(-0.322184484673896,2.10764748908873,
4.72394404912277));
#55550=CARTESIAN_POINT('Ctrl Pts',(-0.32220194332813,2.10687263171224,4.72399159796329));
#55551=CARTESIAN_POINT('Ctrl Pts',(-0.322209962787825,2.10648577129614,
4.72401535844456));
#55552=CARTESIAN_POINT('Ctrl Pts',(-0.322224409897198,2.10572250097408,
4.72406227920662));
#55553=CARTESIAN_POINT('Ctrl Pts',(-0.322230874755522,2.10534609234585,
4.72408543828096));
#55554=CARTESIAN_POINT('Ctrl Pts',(-0.322243969803928,2.10449700154428,
4.7241377252403));
#55555=CARTESIAN_POINT('Ctrl Pts',(-0.322250219521799,2.10402431512527,
4.72416686500768));
#55556=CARTESIAN_POINT('Ctrl Pts',(-0.3222686839118,2.10234895229109,4.72427026000821));
#55557=CARTESIAN_POINT('Ctrl Pts',(-0.322275205798636,2.10114623701008,
4.72434469321685));
#55558=CARTESIAN_POINT('Ctrl Pts',(-0.322274995052385,2.09994352890236,
4.72441933817791));
#55559=CARTESIAN_POINT('',(-0.322274937371842,2.10020091534284,4.97494943677011));
#55560=CARTESIAN_POINT('Ctrl Pts',(-0.322274995069378,2.0999436259616,4.72441933215401));
#55561=CARTESIAN_POINT('Ctrl Pts',(-0.322274547943088,2.09738752696416,
4.7245779740387));
#55562=CARTESIAN_POINT('Ctrl Pts',(-0.322243690626771,2.09483157014679,
4.72473756644637));
#55563=CARTESIAN_POINT('Ctrl Pts',(-0.321335065755551,2.05692969309682,
4.72711886872579));
#55564=CARTESIAN_POINT('Ctrl Pts',(-0.314676157708159,2.02196848964178,
4.72954509116856));
#55565=CARTESIAN_POINT('Ctrl Pts',(-0.298601357054798,1.97824230550722,
4.73266195050605));
#55566=CARTESIAN_POINT('Ctrl Pts',(-0.294169496817719,1.96789371210595,
4.73340268415641));
#55567=CARTESIAN_POINT('Ctrl Pts',(-0.288752555336678,1.9568770158005,4.73417929989949));
#55568=CARTESIAN_POINT('Ctrl Pts',(-0.288295759312503,1.9559590959222,4.73424391317211));
#55569=CARTESIAN_POINT('Ctrl Pts',(-0.28750009264393,1.95437917257349,4.73435494116238));
#55570=CARTESIAN_POINT('Ctrl Pts',(-0.2871632999874,1.95371613958796,4.73440147898744));
#55571=CARTESIAN_POINT('Ctrl Pts',(-0.28668221313438,1.95277710340268,4.73446730283752));
#55572=CARTESIAN_POINT('Ctrl Pts',(-0.286539812508352,1.95250014081441,
4.73448670644769));
#55573=CARTESIAN_POINT('Ctrl Pts',(-0.28629435605936,1.95202443637072,4.73452001465143));
#55574=CARTESIAN_POINT('Ctrl Pts',(-0.286191494392835,1.95182559505374,
4.73453393154702));
#55575=CARTESIAN_POINT('Ctrl Pts',(-0.285993950484522,1.95144469709913,
4.73456057940287));
#55576=CARTESIAN_POINT('Ctrl Pts',(-0.285899301700763,1.95126262399343,
4.73457331246777));
#55577=CARTESIAN_POINT('Ctrl Pts',(-0.28567567681513,1.95083344544871,4.73460331533039));
#55578=CARTESIAN_POINT('Ctrl Pts',(-0.285546553653665,1.95058641621874,
4.73462057577588));
#55579=CARTESIAN_POINT('Ctrl Pts',(-0.285163434367359,1.9498557702661,4.734671602424));
#55580=CARTESIAN_POINT('Ctrl Pts',(-0.284908527335595,1.94937262836942,
4.73470531135803));
#55581=CARTESIAN_POINT('Ctrl Pts',(-0.282632449248504,1.94508507864646,
4.73500418561647));
#55582=CARTESIAN_POINT('Ctrl Pts',(-0.280536294570565,1.94132068168172,
4.73526470628351));
#55583=CARTESIAN_POINT('Ctrl Pts',(-0.278246628046583,1.93739604882048,
4.73553551695539));
#55584=CARTESIAN_POINT('Ctrl Pts',(-0.278127867869703,1.93719299746828,
4.73554952578012));
#55585=CARTESIAN_POINT('Ctrl Pts',(-0.277944061789395,1.93687952131825,
4.73557114973181));
#55586=CARTESIAN_POINT('Ctrl Pts',(-0.277879172390624,1.93676900539128,
4.73557877262503));
#55587=CARTESIAN_POINT('Ctrl Pts',(-0.265493573508929,1.91570334818976,
4.7370316737817));
#55588=CARTESIAN_POINT('Ctrl Pts',(-0.250840055453509,1.89620681532173,
4.73835956307186));
#55589=CARTESIAN_POINT('Ctrl Pts',(-0.219493124091191,1.86306596888579,
4.74092149802996));
#55590=CARTESIAN_POINT('Ctrl Pts',(-0.203358906735829,1.84908184896662,
4.74214082725452));
#55591=CARTESIAN_POINT('Ctrl Pts',(-0.185189197729576,1.83624435840432,
4.74349138570597));
#55592=CARTESIAN_POINT('Ctrl Pts',(-0.184411203423234,1.83569981942645,
4.74354916423492));
#55593=CARTESIAN_POINT('Ctrl Pts',(-0.183162783934418,1.83483421303547,
4.74364180484366));
#55594=CARTESIAN_POINT('Ctrl Pts',(-0.182693890665827,1.83451093750973,
4.74367658297569));
#55595=CARTESIAN_POINT('Ctrl Pts',(-0.18179888319161,1.83389737405409,4.74374293574978));
#55596=CARTESIAN_POINT('Ctrl Pts',(-0.181372924060936,1.83360686217973,
4.74377450178129));
#55597=CARTESIAN_POINT('Ctrl Pts',(-0.180624074078974,1.83309876154052,
4.74382997371869));
#55598=CARTESIAN_POINT('Ctrl Pts',(-0.180301481812524,1.83288073285114,
4.74385386292528));
#55599=CARTESIAN_POINT('Ctrl Pts',(-0.179670254216398,1.83245577290588,
4.74390059410385));
#55600=CARTESIAN_POINT('Ctrl Pts',(-0.179361654428296,1.83224878969363,
4.74392343406777));
#55601=CARTESIAN_POINT('Ctrl Pts',(-0.178627371745863,1.83175813271335,
4.74397776477584));
#55602=CARTESIAN_POINT('Ctrl Pts',(-0.178201371029061,1.83147493848653,
4.74400927349607));
#55603=CARTESIAN_POINT('Ctrl Pts',(-0.176692369059128,1.83047696546601,
4.74412084530581));
#55604=CARTESIAN_POINT('Ctrl Pts',(-0.175605737973411,1.82976772187624,
4.74420111543285));
#55605=CARTESIAN_POINT('Ctrl Pts',(-0.157489377820834,1.81809859475036,
4.74553827735376));
#55606=CARTESIAN_POINT('Ctrl Pts',(-0.139471499948845,1.80876344994324,
4.74685647753258));
#55607=CARTESIAN_POINT('Ctrl Pts',(-0.100979544123374,1.79321560880284,
4.74963667777787));
#55608=CARTESIAN_POINT('Ctrl Pts',(-0.0805193728849704,1.78722188406425,
4.7510956986516));
#55609=CARTESIAN_POINT('Ctrl Pts',(-0.0517850699502814,1.78181292845422,
4.75302784297435));
#55610=CARTESIAN_POINT('Ctrl Pts',(-0.04389927028912,1.78062939387546,4.75354584820889));
#55611=CARTESIAN_POINT('Ctrl Pts',(-0.0347137491669791,1.77959752312098,
4.75412910121221));
#55612=CARTESIAN_POINT('Ctrl Pts',(-0.0334496425227513,1.77946308619111,
4.75420892755528));
#55613=CARTESIAN_POINT('Ctrl Pts',(-0.0318026092067258,1.77929777491508,
4.75431233263403));
#55614=CARTESIAN_POINT('Ctrl Pts',(-0.0314203989883882,1.77926010279693,
4.75433628658921));
#55615=CARTESIAN_POINT('Ctrl Pts',(-0.0307999376527302,1.77920006744461,
4.75437510276674));
#55616=CARTESIAN_POINT('Ctrl Pts',(-0.0305617287982219,1.77917728630798,
4.75438998853751));
#55617=CARTESIAN_POINT('Ctrl Pts',(-0.0301036265495518,1.77913399047732,
4.75441858329381));
#55618=CARTESIAN_POINT('Ctrl Pts',(-0.0298837380949415,1.7791134365603,
4.75443229442039));
#55619=CARTESIAN_POINT('Ctrl Pts',(-0.0293763572658202,1.77906653554926,
4.75446389936115));
#55620=CARTESIAN_POINT('Ctrl Pts',(-0.0290888495932546,1.77904034863949,
4.75448178408523));
#55621=CARTESIAN_POINT('Ctrl Pts',(-0.0281693468069803,1.77895784371366,
4.75453890635953));
#55622=CARTESIAN_POINT('Ctrl Pts',(-0.0275372154203691,1.77890300531529,
4.75457806089332));
#55623=CARTESIAN_POINT('Ctrl Pts',(-0.0218635453144588,1.77842768333002,
4.75492848888543));
#55624=CARTESIAN_POINT('Ctrl Pts',(-0.0168125786775542,1.77812407106975,
4.75523336089768));
#55625=CARTESIAN_POINT('Ctrl Pts',(-0.0105768964562659,1.77789644902548,
4.7556032965631));
#55626=CARTESIAN_POINT('Ctrl Pts',(-0.00939732711859988,1.77785987737585,
4.75567299116233));
#55627=CARTESIAN_POINT('Ctrl Pts',(0.0236689207366504,1.77701645939498,
4.75761939655843));
#55628=CARTESIAN_POINT('Ctrl Pts',(0.0555020713937053,1.7809410735263,4.75931959009532));
#55629=CARTESIAN_POINT('Ctrl Pts',(0.0977623471692265,1.79267829686755,
4.76184549427587));
#55630=CARTESIAN_POINT('Ctrl Pts',(0.109093487027939,1.79651578830825,4.76254896510335));
#55631=CARTESIAN_POINT('Ctrl Pts',(0.121135349328311,1.80135564116716,4.76333620574593));
#55632=CARTESIAN_POINT('Ctrl Pts',(0.122084420615296,1.80174235948617,4.76339852203811));
#55633=CARTESIAN_POINT('Ctrl Pts',(0.123586707155374,1.80236286837052,4.76349759883531));
#55634=CARTESIAN_POINT('Ctrl Pts',(0.124141146611156,1.80259369202969,4.76353425912491));
#55635=CARTESIAN_POINT('Ctrl Pts',(0.125190972817312,1.80303420175775,4.76360385612501));
#55636=CARTESIAN_POINT('Ctrl Pts',(0.125686486637661,1.80324358124593,4.76363678235485));
#55637=CARTESIAN_POINT('Ctrl Pts',(0.126543417496122,1.80360820889033,4.76369385812731));
#55638=CARTESIAN_POINT('Ctrl Pts',(0.126905079899416,1.80376288037739,4.76371798799422));
#55639=CARTESIAN_POINT('Ctrl Pts',(0.127602783897303,1.80406277831003,4.76376461867095));
#55640=CARTESIAN_POINT('Ctrl Pts',(0.127938863182336,1.80420791605282,4.76378711642586));
#55641=CARTESIAN_POINT('Ctrl Pts',(0.128724131392164,1.80454862727937,4.76383976846701));
#55642=CARTESIAN_POINT('Ctrl Pts',(0.129173122177034,1.8047446526344,4.7638699381659));
#55643=CARTESIAN_POINT('Ctrl Pts',(0.130695925320206,1.80541363322174,4.76397248411289));
#55644=CARTESIAN_POINT('Ctrl Pts',(0.131767591425263,1.80589142450702,4.76404502586968));
#55645=CARTESIAN_POINT('Ctrl Pts',(0.143118691695756,1.8110266888249,4.76481743173806));
#55646=CARTESIAN_POINT('Ctrl Pts',(0.153148163358532,1.81621465226782,4.76553564155586));
#55647=CARTESIAN_POINT('Ctrl Pts',(0.18124070703955,1.83266956877606,4.7676559135239));
#55648=CARTESIAN_POINT('Ctrl Pts',(0.198485828572135,1.84521199137991,4.76909893007554));
#55649=CARTESIAN_POINT('Ctrl Pts',(0.218240208679316,1.86280959470392,4.77088674085388));
#55650=CARTESIAN_POINT('Ctrl Pts',(0.222029278360146,1.86635266157439,4.77123637371201));
#55651=CARTESIAN_POINT('Ctrl Pts',(0.231768501317145,1.87591053250826,4.77215013439335));
#55652=CARTESIAN_POINT('Ctrl Pts',(0.237570621916372,1.88207122988262,4.77271015816524));
#55653=CARTESIAN_POINT('Ctrl Pts',(0.246029783771259,1.89179308984146,4.77354261721365));
#55654=CARTESIAN_POINT('Ctrl Pts',(0.248866656728988,1.89519237319296,4.77382477416132));
#55655=CARTESIAN_POINT('Ctrl Pts',(0.251979726887251,1.89908284973005,4.77413680249407));
#55656=CARTESIAN_POINT('Ctrl Pts',(0.252325577625095,1.89951736503658,4.77417150206428));
#55657=CARTESIAN_POINT('Ctrl Pts',(0.252841844430484,1.90016943752902,4.77422334848586));
#55658=CARTESIAN_POINT('Ctrl Pts',(0.253013104371194,1.90038632058323,4.77424055547313));
#55659=CARTESIAN_POINT('Ctrl Pts',(0.253306610247418,1.90075900008808,4.77427005839593));
#55660=CARTESIAN_POINT('Ctrl Pts',(0.253428991500558,1.90091468886734,4.77428236408162));
#55661=CARTESIAN_POINT('Ctrl Pts',(0.253681914753753,1.90123705935169,4.77430780431052));
#55662=CARTESIAN_POINT('Ctrl Pts',(0.253812435649459,1.90140375643383,4.77432093733637));
#55663=CARTESIAN_POINT('Ctrl Pts',(0.254167918921418,1.90185869106997,4.77435671906143));
#55664=CARTESIAN_POINT('Ctrl Pts',(0.25439255606977,1.90214718416767,4.77437934445946));
#55665=CARTESIAN_POINT('Ctrl Pts',(0.255240196448918,1.90323960720513,4.77446477504665));
#55666=CARTESIAN_POINT('Ctrl Pts',(0.255859892270745,1.90404611346424,4.77452734770043));
#55667=CARTESIAN_POINT('Ctrl Pts',(0.267643829345911,1.9195335862945,4.77571972799984));
#55668=CARTESIAN_POINT('Ctrl Pts',(0.27753313523343,1.93514575471937,4.77676487777652));
#55669=CARTESIAN_POINT('Ctrl Pts',(0.29379133191771,1.96646582358621,4.77874347161244));
#55670=CARTESIAN_POINT('Ctrl Pts',(0.300365881084286,1.98199558572142,4.77967607794931));
#55671=CARTESIAN_POINT('Ctrl Pts',(0.310244164514636,2.01159171432753,4.78145894755035));
#55672=CARTESIAN_POINT('Ctrl Pts',(0.313875044148507,2.02550274275552,4.78229889245078));
#55673=CARTESIAN_POINT('Ctrl Pts',(0.316745730245191,2.04055054206694,4.78322877664618));
#55674=CARTESIAN_POINT('Ctrl Pts',(0.316921266267282,2.04149353340299,4.78328713222741));
#55675=CARTESIAN_POINT('Ctrl Pts',(0.317195022981206,2.04300156211961,4.7833805922474));
#55676=CARTESIAN_POINT('Ctrl Pts',(0.317295950610439,2.04356610730783,4.78341561074861));
#55677=CARTESIAN_POINT('Ctrl Pts',(0.317485243078731,2.044641488338,4.78348237612829));
#55678=CARTESIAN_POINT('Ctrl Pts',(0.317573883333443,2.04515227437982,4.78351411416085));
#55679=CARTESIAN_POINT('Ctrl Pts',(0.317722575851088,2.04602155482355,4.78356817200388));
#55680=CARTESIAN_POINT('Ctrl Pts',(0.317783254983974,2.04637994219333,4.78359047185833));
#55681=CARTESIAN_POINT('Ctrl Pts',(0.317903871892142,2.04709973471263,4.78363528546525));
#55682=CARTESIAN_POINT('Ctrl Pts',(0.317963800007859,2.0474611409114,4.7836577994882));
#55683=CARTESIAN_POINT('Ctrl Pts',(0.318102602501957,2.0483071478249,4.78371053327904));
#55684=CARTESIAN_POINT('Ctrl Pts',(0.318180985784851,2.04879182716364,4.78374076858309));
#55685=CARTESIAN_POINT('Ctrl Pts',(0.318443867997036,2.05044125465171,4.78384374607425));
#55686=CARTESIAN_POINT('Ctrl Pts',(0.318623079619836,2.05160682507111,4.78391665564451));
#55687=CARTESIAN_POINT('Ctrl Pts',(0.3204852304953,2.06417697187075,4.78470451103431));
#55688=CARTESIAN_POINT('Ctrl Pts',(0.321561292627095,2.07566169388501,4.78543861549542));
#55689=CARTESIAN_POINT('Ctrl Pts',(0.323072952801183,2.11362736853598,4.78791544009857));
#55690=CARTESIAN_POINT('Ctrl Pts',(0.320863191711508,2.14010385172059,4.78973224530757));
#55691=CARTESIAN_POINT('Ctrl Pts',(0.313122989998399,2.1770939750261,4.79226121142413));
#55692=CARTESIAN_POINT('Ctrl Pts',(0.310219724754215,2.18805264762559,4.79300736399185));
#55693=CARTESIAN_POINT('Ctrl Pts',(0.306429352962278,2.19981626285489,4.79378925525127));
#55694=CARTESIAN_POINT('Ctrl Pts',(0.306109046731703,2.20079427693285,4.79385411240761));
#55695=CARTESIAN_POINT('Ctrl Pts',(0.305548521924831,2.20247844984597,4.793965521861));
#55696=CARTESIAN_POINT('Ctrl Pts',(0.305310528760909,2.20318533319857,4.79401219837646));
#55697=CARTESIAN_POINT('Ctrl Pts',(0.304969566324361,2.20418654644486,4.79407818365519));
#55698=CARTESIAN_POINT('Ctrl Pts',(0.304868622981311,2.20448155611217,4.79409761078358));
#55699=CARTESIAN_POINT('Ctrl Pts',(0.30469444485817,2.20498819479714,4.7941309468645));
#55700=CARTESIAN_POINT('Ctrl Pts',(0.304621417477834,2.20519989443491,4.79414486817189));
#55701=CARTESIAN_POINT('Ctrl Pts',(0.304481076289535,2.20560535915375,4.79417151544452));
#55702=CARTESIAN_POINT('Ctrl Pts',(0.304413798251961,2.20579913579435,4.79418424353182));
#55703=CARTESIAN_POINT('Ctrl Pts',(0.304254765406981,2.20625578040847,4.7942142217656));
#55704=CARTESIAN_POINT('Ctrl Pts',(0.304162854693844,2.20651859447494,4.79423146259749));
#55705=CARTESIAN_POINT('Ctrl Pts',(0.303890019737201,2.20729551981103,4.79428239311764));
#55706=CARTESIAN_POINT('Ctrl Pts',(0.303708130637591,2.20780929487872,4.79431602584079));
#55707=CARTESIAN_POINT('Ctrl Pts',(0.302088659480754,2.21234712755753,4.79461268370196));
#55708=CARTESIAN_POINT('Ctrl Pts',(0.300572395077036,2.21634291934177,4.79487113964616));
#55709=CARTESIAN_POINT('Ctrl Pts',(0.298879635831992,2.22054960372375,4.79514146905773));
#55710=CARTESIAN_POINT('Ctrl Pts',(0.298781960745809,2.22079148813868,4.79515700674482));
#55711=CARTESIAN_POINT('Ctrl Pts',(0.298608901267073,2.22121856164141,4.79518442962557));
#55712=CARTESIAN_POINT('Ctrl Pts',(0.298533638147916,2.22140379935112,4.79519632042079));
#55713=CARTESIAN_POINT('Ctrl Pts',(0.288243589254833,2.24666225465086,4.79681724708452));
#55714=CARTESIAN_POINT('Ctrl Pts',(0.274908960551781,2.27035150890766,4.7982823088134));
#55715=CARTESIAN_POINT('Ctrl Pts',(0.248655272503861,2.30571704761376,4.80077010726724));
#55716=CARTESIAN_POINT('Ctrl Pts',(0.237485478497587,2.31851654493557,4.80174798534859));
#55717=CARTESIAN_POINT('Ctrl Pts',(0.224143846496643,2.33156772791971,4.80287291557645));
#55718=CARTESIAN_POINT('Ctrl Pts',(0.222916913683114,2.33274906220982,4.80297598299758));
#55719=CARTESIAN_POINT('Ctrl Pts',(0.221052375225113,2.33451603860636,4.80313206757275));
#55720=CARTESIAN_POINT('Ctrl Pts',(0.220421666608549,2.33510894032972,4.80318477299008));
#55721=CARTESIAN_POINT('Ctrl Pts',(0.21939765974554,2.33606382236053,4.80327019926381));
#55722=CARTESIAN_POINT('Ctrl Pts',(0.219005833382308,2.33642738053874,4.80330285268552));
#55723=CARTESIAN_POINT('Ctrl Pts',(0.218252907105572,2.33712250946958,4.80336553465834));
#55724=CARTESIAN_POINT('Ctrl Pts',(0.217891951249932,2.33745423460845,4.80339555652448));
#55725=CARTESIAN_POINT('Ctrl Pts',(0.217245818113449,2.33804532916167,4.80344924808123));
#55726=CARTESIAN_POINT('Ctrl Pts',(0.216960929132252,2.33830501348366,4.80347290435363));
#55727=CARTESIAN_POINT('Ctrl Pts',(0.216394139896661,2.33881979898669,4.80351993523174));
#55728=CARTESIAN_POINT('Ctrl Pts',(0.216112252737284,2.33907491374995,4.80354330920985));
#55729=CARTESIAN_POINT('Ctrl Pts',(0.215426295066431,2.33969351767809,4.8036001492532));
#55730=CARTESIAN_POINT('Ctrl Pts',(0.215021756246044,2.34005648368256,4.80363363726486));
#55731=CARTESIAN_POINT('Ctrl Pts',(0.213500134666006,2.34141480221091,4.80375947633488));
#55732=CARTESIAN_POINT('Ctrl Pts',(0.212377056454096,2.34240338281396,4.80385211023167));
#55733=CARTESIAN_POINT('Ctrl Pts',(0.192193098774542,2.35992220858378,4.80551272578128));
#55734=CARTESIAN_POINT('Ctrl Pts',(0.171267145774927,2.37416196981549,4.80717858195709));
#55735=CARTESIAN_POINT('Ctrl Pts',(0.134973045136161,2.39307008041397,4.80994275748884));
#55736=CARTESIAN_POINT('Ctrl Pts',(0.120533535663463,2.3992983334101,4.81101174144656));
#55737=CARTESIAN_POINT('Ctrl Pts',(0.0996979530953711,2.40653192623375,
4.81247102143551));
#55738=CARTESIAN_POINT('Ctrl Pts',(0.0936380881739768,2.4084370655673,4.81288583197488));
#55739=CARTESIAN_POINT('Ctrl Pts',(0.0846564720144243,2.41097161295694,
4.81348286928738));
#55740=CARTESIAN_POINT('Ctrl Pts',(0.0817762387361333,2.41174141633265,
4.8136716819946));
#55741=CARTESIAN_POINT('Ctrl Pts',(0.0783961997869921,2.41259473168522,
4.81388984402913));
#55742=CARTESIAN_POINT('Ctrl Pts',(0.0779064910381102,2.41271713909021,
4.81392136845973));
#55743=CARTESIAN_POINT('Ctrl Pts',(0.0771584243834943,2.41290225925904,
4.81396939490895));
#55744=CARTESIAN_POINT('Ctrl Pts',(0.0769002759501127,2.41296580302451,
4.81398594472511));
#55745=CARTESIAN_POINT('Ctrl Pts',(0.076432352612189,2.4130803694059,4.81401590018309));
#55746=CARTESIAN_POINT('Ctrl Pts',(0.0762226058937506,2.41313150046699,
4.81402931206462));
#55747=CARTESIAN_POINT('Ctrl Pts',(0.0757970786081907,2.41323478060272,
4.81405648989239));
#55748=CARTESIAN_POINT('Ctrl Pts',(0.0755812964742037,2.41328691726399,
4.81407025507855));
#55749=CARTESIAN_POINT('Ctrl Pts',(0.0749603002214063,2.41343628166926,
4.81410982265611));
#55750=CARTESIAN_POINT('Ctrl Pts',(0.0745549492616168,2.41353294694683,
4.81413559250593));
#55751=CARTESIAN_POINT('Ctrl Pts',(0.0727755942865998,2.41395362932403,
4.8142484654288));
#55752=CARTESIAN_POINT('Ctrl Pts',(0.0713996304504149,2.41426940899893,
4.81433510075792));
#55753=CARTESIAN_POINT('Ctrl Pts',(0.0458100076429556,2.41996541149745,
4.81593503546628));
#55754=CARTESIAN_POINT('Ctrl Pts',(0.0210527262711037,2.42254245797922,
4.81729979469515));
#55755=CARTESIAN_POINT('Ctrl Pts',(-0.0181377052763326,2.42208537688345,
4.81949260754807));
#55756=CARTESIAN_POINT('Ctrl Pts',(-0.0324888165575953,2.4209554488909,
4.82030169016366));
#55757=CARTESIAN_POINT('Ctrl Pts',(-0.0551670736788468,2.41763300957231,
4.82163243785005));
#55758=CARTESIAN_POINT('Ctrl Pts',(-0.0635652816464482,2.41605944195539,
4.82213668544881));
#55759=CARTESIAN_POINT('Ctrl Pts',(-0.0735190890367058,2.41378162801453,
4.82275232407146));
#55760=CARTESIAN_POINT('Ctrl Pts',(-0.075144647552223,2.41339631190449,
4.82285343992258));
#55761=CARTESIAN_POINT('Ctrl Pts',(-0.0779756927401721,2.41270195953203,
4.82303058133914));
#55762=CARTESIAN_POINT('Ctrl Pts',(-0.0791825313281298,2.41239854483979,
4.82310642569914));
#55763=CARTESIAN_POINT('Ctrl Pts',(-0.0809139239891755,2.41195257325496,
4.82321572256215));
#55764=CARTESIAN_POINT('Ctrl Pts',(-0.0814399322665852,2.41181566426723,
4.82324899236324));
#55765=CARTESIAN_POINT('Ctrl Pts',(-0.0823518991976577,2.41157583327347,
4.8233067871556));
#55766=CARTESIAN_POINT('Ctrl Pts',(-0.0827380186489511,2.41147352287031,
4.82333129228985));
#55767=CARTESIAN_POINT('Ctrl Pts',(-0.0834798861566364,2.41127547278139,
4.82337844328639));
#55768=CARTESIAN_POINT('Ctrl Pts',(-0.0838356624413832,2.41117984036449,
4.8234010856368));
#55769=CARTESIAN_POINT('Ctrl Pts',(-0.0846731491461758,2.41095318401872,
4.82345445661156));
#55770=CARTESIAN_POINT('Ctrl Pts',(-0.0851547196179992,2.41082165072596,
4.82348520173893));
#55771=CARTESIAN_POINT('Ctrl Pts',(-0.0865755000462562,2.41043003748887,
4.82357607526605));
#55772=CARTESIAN_POINT('Ctrl Pts',(-0.0875138318464044,2.41016681735112,
4.82363630566708));
#55773=CARTESIAN_POINT('Ctrl Pts',(-0.0958083217458707,2.40779941808609,
4.82417064160083));
#55774=CARTESIAN_POINT('Ctrl Pts',(-0.103088020073232,2.40543830847302,
4.82465309972509));
#55775=CARTESIAN_POINT('Ctrl Pts',(-0.131813020240103,2.3949776981861,4.82661371616162));
#55776=CARTESIAN_POINT('Ctrl Pts',(-0.152448508420773,2.38486076554084,
4.82815789406693));
#55777=CARTESIAN_POINT('Ctrl Pts',(-0.181669467611517,2.36644429523975,
4.83049503711453));
#55778=CARTESIAN_POINT('Ctrl Pts',(-0.191163510464489,2.35971695566081,
4.83128033285603));
#55779=CARTESIAN_POINT('Ctrl Pts',(-0.204205464423418,2.34937219174579,
4.8323788449472));
#55780=CARTESIAN_POINT('Ctrl Pts',(-0.208064178027766,2.34616186775728,
4.83270648303304));
#55781=CARTESIAN_POINT('Ctrl Pts',(-0.214583399585041,2.34047521713428,
4.83326243420519));
#55782=CARTESIAN_POINT('Ctrl Pts',(-0.217279858907874,2.33804165835473,
4.83349312998607));
#55783=CARTESIAN_POINT('Ctrl Pts',(-0.220322711220529,2.33520068086404,
4.83375374112989));
#55784=CARTESIAN_POINT('Ctrl Pts',(-0.220709790269944,2.3348374881637,4.83378689854286));
#55785=CARTESIAN_POINT('Ctrl Pts',(-0.221293365339988,2.33428720769479,
4.83383689341249));
#55786=CARTESIAN_POINT('Ctrl Pts',(-0.22149052290109,2.33410082763464,4.83385378485063));
#55787=CARTESIAN_POINT('Ctrl Pts',(-0.221845843194195,2.33376408002005,
4.83388422817723));
#55788=CARTESIAN_POINT('Ctrl Pts',(-0.222004088137277,2.33361380117925,
4.83389778682475));
#55789=CARTESIAN_POINT('Ctrl Pts',(-0.222321074933184,2.33331215865124,
4.83392494755549));
#55790=CARTESIAN_POINT('Ctrl Pts',(-0.222479814201102,2.33316079431946,
4.83393854946002));
#55791=CARTESIAN_POINT('Ctrl Pts',(-0.222930173794775,2.3327304795077,4.83397714123216));
#55792=CARTESIAN_POINT('Ctrl Pts',(-0.223221426184596,2.33245114191241,
4.83400210106155));
#55793=CARTESIAN_POINT('Ctrl Pts',(-0.224449032432517,2.33126932068924,
4.83410731775268));
#55794=CARTESIAN_POINT('Ctrl Pts',(-0.225380460588576,2.33036170465509,
4.83418718125985));
#55795=CARTESIAN_POINT('Ctrl Pts',(-0.250771147196566,2.30531871838263,
4.83636600503686));
#55796=CARTESIAN_POINT('Ctrl Pts',(-0.271224248489784,2.2774270288178,4.83818434348403));
#55797=CARTESIAN_POINT('Ctrl Pts',(-0.293188683860187,2.23451005768142,
4.84093381071334));
#55798=CARTESIAN_POINT('Ctrl Pts',(-0.298691174732031,2.22180341126569,
4.84173989535427));
#55799=CARTESIAN_POINT('Ctrl Pts',(-0.304134261484152,2.20662451764932,
4.842713452436));
#55800=CARTESIAN_POINT('Ctrl Pts',(-0.304885415788433,2.20445726203305,
4.84285267810548));
#55801=CARTESIAN_POINT('Ctrl Pts',(-0.305832599472033,2.20162713184336,
4.84303483420693));
#55802=CARTESIAN_POINT('Ctrl Pts',(-0.306049733622719,2.20097134922485,
4.84307706648878));
#55803=CARTESIAN_POINT('Ctrl Pts',(-0.306398679645331,2.19990600506856,
4.84314571527919));
#55804=CARTESIAN_POINT('Ctrl Pts',(-0.306531783527915,2.19949686639042,
4.84317208915837));
#55805=CARTESIAN_POINT('Ctrl Pts',(-0.306785370610973,2.19871204414177,
4.84322269950382));
#55806=CARTESIAN_POINT('Ctrl Pts',(-0.306905984103844,2.19833640322185,
4.8432469316295));
#55807=CARTESIAN_POINT('Ctrl Pts',(-0.307179105977551,2.19748039029691,
4.84330217151592));
#55808=CARTESIAN_POINT('Ctrl Pts',(-0.307331177604268,2.19699988097611,
4.84333319356386));
#55809=CARTESIAN_POINT('Ctrl Pts',(-0.307800303592523,2.19550537911362,
4.84342972444637));
#55810=CARTESIAN_POINT('Ctrl Pts',(-0.308113469068286,2.19449018185342,
4.84349536061404));
#55811=CARTESIAN_POINT('Ctrl Pts',(-0.310498057020221,2.18662208312165,
4.84400458072169));
#55812=CARTESIAN_POINT('Ctrl Pts',(-0.312345487444632,2.17970390166747,
4.84445543271626));
#55813=CARTESIAN_POINT('Ctrl Pts',(-0.31950725476006,2.14878813394352,4.84648616264434));
#55814=CARTESIAN_POINT('Ctrl Pts',(-0.322295837656254,2.12429352717107,
4.84814582981022));
#55815=CARTESIAN_POINT('Ctrl Pts',(-0.322265261789212,2.08844506048664,
4.85057028780775));
#55816=CARTESIAN_POINT('Ctrl Pts',(-0.321663418753319,2.0771726175823,4.85133039379503));
#55817=CARTESIAN_POINT('Ctrl Pts',(-0.31966821847208,2.05839177309774,4.85257245571714));
#55818=CARTESIAN_POINT('Ctrl Pts',(-0.318597266857262,2.05085920061318,
4.85306388510344));
#55819=CARTESIAN_POINT('Ctrl Pts',(-0.317139531205371,2.0426923346232,4.85358433770952));
#55820=CARTESIAN_POINT('Ctrl Pts',(-0.317016231029612,2.04201413923544,
4.85362746337546));
#55821=CARTESIAN_POINT('Ctrl Pts',(-0.316839910972375,2.04106168939858,
4.85368789149017));
#55822=CARTESIAN_POINT('Ctrl Pts',(-0.316788710151355,2.04078710644104,
4.85370529636091));
#55823=CARTESIAN_POINT('Ctrl Pts',(-0.316699247274855,2.0403107667193,4.85373546167032));
#55824=CARTESIAN_POINT('Ctrl Pts',(-0.316661149349566,2.04010897991143,
4.85374823148886));
#55825=CARTESIAN_POINT('Ctrl Pts',(-0.316581137717659,2.03968740654789,
4.85377489163569));
#55826=CARTESIAN_POINT('Ctrl Pts',(-0.316539188019205,2.03946762737182,
4.85378877980809));
#55827=CARTESIAN_POINT('Ctrl Pts',(-0.31643842938532,2.0389427105068,4.85382192516007));
#55828=CARTESIAN_POINT('Ctrl Pts',(-0.316379407720406,2.03863761278658,
4.85384117012793));
#55829=CARTESIAN_POINT('Ctrl Pts',(-0.316178398267344,2.03760654453316,
4.85390614131245));
#55830=CARTESIAN_POINT('Ctrl Pts',(-0.316034350960006,2.03688097074001,
4.85395175058863));
#55831=CARTESIAN_POINT('Ctrl Pts',(-0.315686045254178,2.03515762419322,
4.85405982776758));
#55832=CARTESIAN_POINT('Ctrl Pts',(-0.31547955146576,2.03416030423277,4.8541221723812));
#55833=CARTESIAN_POINT('Ctrl Pts',(-0.312964366910576,2.02229607512246,
4.85486161767935));
#55834=CARTESIAN_POINT('Ctrl Pts',(-0.310099710828364,2.01155328689114,
4.85550912136439));
#55835=CARTESIAN_POINT('Ctrl Pts',(-0.297780652426222,1.97339905809882,
4.85779789265055));
#55836=CARTESIAN_POINT('Ctrl Pts',(-0.285196755739902,1.94714701531693,
4.85936438115177));
#55837=CARTESIAN_POINT('Ctrl Pts',(-0.264134978644012,1.91511812636728,
4.86159914486023));
#55838=CARTESIAN_POINT('Ctrl Pts',(-0.258660770473499,1.90753396594059,
4.86215458182131));
#55839=CARTESIAN_POINT('Ctrl Pts',(-0.252156573781885,1.89930235740854,
4.86279258404127));
#55840=CARTESIAN_POINT('Ctrl Pts',(-0.251443361930493,1.89840953114887,
4.86286226477275));
#55841=CARTESIAN_POINT('Ctrl Pts',(-0.250399203620586,1.89711657522875,
4.86296388398589));
#55842=CARTESIAN_POINT('Ctrl Pts',(-0.250072009158192,1.8967134154664,4.86299567138536));
#55843=CARTESIAN_POINT('Ctrl Pts',(-0.249492997884153,1.89600348740729,
4.86305182597509));
#55844=CARTESIAN_POINT('Ctrl Pts',(-0.249241585388863,1.89569638952329,
4.86307617677848));
#55845=CARTESIAN_POINT('Ctrl Pts',(-0.248720769463517,1.89506261014191,
4.86312655516956));
#55846=CARTESIAN_POINT('Ctrl Pts',(-0.248451288315194,1.89473599376372,
4.86315258588599));
#55847=CARTESIAN_POINT('Ctrl Pts',(-0.247760010890798,1.89390150783462,
4.86321926867271));
#55848=CARTESIAN_POINT('Ctrl Pts',(-0.247337297829863,1.89339440336402,
4.86325995807122));
#55849=CARTESIAN_POINT('Ctrl Pts',(-0.245607411054075,1.89133207556412,
4.86342612373572));
#55850=CARTESIAN_POINT('Ctrl Pts',(-0.244287125542864,1.88978795694985,
4.86355213689264));
#55851=CARTESIAN_POINT('Ctrl Pts',(-0.235490870777365,1.87969522536101,
4.86438655768729));
#55852=CARTESIAN_POINT('Ctrl Pts',(-0.227582937952363,1.87153534418111,
4.86511309085673));
#55853=CARTESIAN_POINT('Ctrl Pts',(-0.195678319830756,1.84191734953361,
4.86796076437346));
#55854=CARTESIAN_POINT('Ctrl Pts',(-0.168953727629281,1.82368343088164,
4.8702016052494));
#55855=CARTESIAN_POINT('Ctrl Pts',(-0.134698442587637,1.80716588646477,
4.87268038720507));
#55856=CARTESIAN_POINT('Ctrl Pts',(-0.129353278372291,1.80476580715939,
4.87305623874594));
#55857=CARTESIAN_POINT('Ctrl Pts',(-0.123336330879813,1.80225890397114,
4.87346495857367));
#55858=CARTESIAN_POINT('Ctrl Pts',(-0.122726622223432,1.80200706888379,
4.87350621293542));
#55859=CARTESIAN_POINT('Ctrl Pts',(-0.121869100873056,1.80165595508512,
4.87356400324145));
#55860=CARTESIAN_POINT('Ctrl Pts',(-0.121621936810504,1.80155511166799,
4.87358063321549));
#55861=CARTESIAN_POINT('Ctrl Pts',(-0.121168517609294,1.80137077256667,
4.87361109087047));
#55862=CARTESIAN_POINT('Ctrl Pts',(-0.120962300846453,1.80128718321444,
4.87362492425928));
#55863=CARTESIAN_POINT('Ctrl Pts',(-0.12054181084276,1.80111724567625,4.87365309280054));
#55864=CARTESIAN_POINT('Ctrl Pts',(-0.120327531281979,1.8010309142908,4.87366742691741));
#55865=CARTESIAN_POINT('Ctrl Pts',(-0.119791611534497,1.80081566634908,
4.87370322637883));
#55866=CARTESIAN_POINT('Ctrl Pts',(-0.119469854925936,1.80068703759638,
4.87372467421235));
#55867=CARTESIAN_POINT('Ctrl Pts',(-0.118245975170635,1.80020005466924,
4.87380608562438));
#55868=CARTESIAN_POINT('Ctrl Pts',(-0.117342430262574,1.79984525327537,
4.87386583657852));
#55869=CARTESIAN_POINT('Ctrl Pts',(-0.096995564250157,1.79196142400602,
4.87520375984501));
#55870=CARTESIAN_POINT('Ctrl Pts',(-0.0768651435166155,1.7863314655387,
4.87637331379111));
#55871=CARTESIAN_POINT('Ctrl Pts',(-0.0332567888343984,1.77859019553519,
4.87885051167343));
#55872=CARTESIAN_POINT('Ctrl Pts',(-0.00980932474648738,1.77702333968839,
4.8801534401622));
#55873=CARTESIAN_POINT('Ctrl Pts',(0.0139488372131563,1.77802682172866,
4.88156073206936));
#55874=CARTESIAN_POINT('Ctrl Pts',(0.0142977297635525,1.77804212619036,
4.88158141594368));
#55875=CARTESIAN_POINT('Ctrl Pts',(0.0203749903211787,1.77831860822223,
4.8819420125137));
#55876=CARTESIAN_POINT('Ctrl Pts',(0.0260951100757931,1.77873204799749,
4.88228624451177));
#55877=CARTESIAN_POINT('Ctrl Pts',(0.032778429286154,1.77939476741297,4.88269511973009));
#55878=CARTESIAN_POINT('Ctrl Pts',(0.0337555038563629,1.77949616770693,
4.88275506263294));
#55879=CARTESIAN_POINT('Ctrl Pts',(0.0352293743224789,1.77965593964246,
4.88284574085923));
#55880=CARTESIAN_POINT('Ctrl Pts',(0.0357265290834473,1.77971100403432,
4.88287637195565));
#55881=CARTESIAN_POINT('Ctrl Pts',(0.0366140320804729,1.77981139510296,
4.88293113320139));
#55882=CARTESIAN_POINT('Ctrl Pts',(0.0370044302345017,1.77985627884971,
4.88295524934095));
#55883=CARTESIAN_POINT('Ctrl Pts',(0.037828421228792,1.77995253974591,4.88300620848894));
#55884=CARTESIAN_POINT('Ctrl Pts',(0.0382619933879894,1.78000408420302,
4.88303305672985));
#55885=CARTESIAN_POINT('Ctrl Pts',(0.0394095694647336,1.78014287740532,
4.88310420991677));
#55886=CARTESIAN_POINT('Ctrl Pts',(0.0401233853250986,1.78023163543497,
4.88314856241899));
#55887=CARTESIAN_POINT('Ctrl Pts',(0.0433811805793674,1.78064779971001,
4.883351416637));
#55888=CARTESIAN_POINT('Ctrl Pts',(0.0459214354545084,1.78100317272342,
4.88351079937893));
#55889=CARTESIAN_POINT('Ctrl Pts',(0.0569570318977422,1.78268156086102,
4.88420864086914));
#55890=CARTESIAN_POINT('Ctrl Pts',(0.065401087692953,1.78431380999952,4.88475680122686));
#55891=CARTESIAN_POINT('Ctrl Pts',(0.0878737946854206,1.78959814530528,
4.88625498031525));
#55892=CARTESIAN_POINT('Ctrl Pts',(0.101737249171859,1.793861846152,4.88722192190025));
#55893=CARTESIAN_POINT('Ctrl Pts',(0.135926778861214,1.80695633384551,4.88969259580636));
#55894=CARTESIAN_POINT('Ctrl Pts',(0.155719355249845,1.81697652314565,4.89120658296429));
#55895=CARTESIAN_POINT('Ctrl Pts',(0.177370872869418,1.83090183886975,4.89286155542775));
#55896=CARTESIAN_POINT('Ctrl Pts',(0.18037870556673,1.83290868197584,4.89309131771158));
#55897=CARTESIAN_POINT('Ctrl Pts',(0.183826325482239,1.83529376669032,4.89335391664071));
#55898=CARTESIAN_POINT('Ctrl Pts',(0.184299494311144,1.83562298832504,4.89338994020404));
#55899=CARTESIAN_POINT('Ctrl Pts',(0.185001669839254,1.83611434955825,4.89344337043796));
#55900=CARTESIAN_POINT('Ctrl Pts',(0.185231348924223,1.83627551928286,4.8934608427724));
#55901=CARTESIAN_POINT('Ctrl Pts',(0.185639992611315,1.83656306870964,4.89349192099115));
#55902=CARTESIAN_POINT('Ctrl Pts',(0.18581903871964,1.83668933087549,4.89350553491112));
#55903=CARTESIAN_POINT('Ctrl Pts',(0.186194756266568,1.83695485855592,4.89353409666998));
#55904=CARTESIAN_POINT('Ctrl Pts',(0.186391399687352,1.8370941616814,4.89354904180288));
#55905=CARTESIAN_POINT('Ctrl Pts',(0.186913734512173,1.83746506672604,4.89358873096248));
#55906=CARTESIAN_POINT('Ctrl Pts',(0.187239152993307,1.83769705505105,4.89361344838351));
#55907=CARTESIAN_POINT('Ctrl Pts',(0.187954110498187,1.83820875120506,4.89366773526208));
#55908=CARTESIAN_POINT('Ctrl Pts',(0.188343459285105,1.83848872500367,4.89369728661286));
#55909=CARTESIAN_POINT('Ctrl Pts',(0.189499239362217,1.83932374601552,4.89378497868441));
#55910=CARTESIAN_POINT('Ctrl Pts',(0.190263860468096,1.83988130678276,4.89384295186516));
#55911=CARTESIAN_POINT('Ctrl Pts',(0.198864769113692,1.84621129423566,4.89449474605051));
#55912=CARTESIAN_POINT('Ctrl Pts',(0.206439006730695,1.85233312630594,4.89506575189868));
#55913=CARTESIAN_POINT('Ctrl Pts',(0.235457423415743,1.87804492827192,4.89729303033909));
#55914=CARTESIAN_POINT('Ctrl Pts',(0.254487949032189,1.90014927149583,4.89885814034142));
#55915=CARTESIAN_POINT('Ctrl Pts',(0.271396762730176,1.92619257382369,4.90065781662078));
#55916=CARTESIAN_POINT('Ctrl Pts',(0.272476614457511,1.92789038793251,4.90077489168021));
#55917=CARTESIAN_POINT('Ctrl Pts',(0.274882271260998,1.93175211030656,4.90104074660629));
#55918=CARTESIAN_POINT('Ctrl Pts',(0.276198546578949,1.93392177197681,4.90118980989194));
#55919=CARTESIAN_POINT('Ctrl Pts',(0.280757448272113,1.94164048492708,4.90171939884683));
#55920=CARTESIAN_POINT('Ctrl Pts',(0.283859403515536,1.94727046441732,4.90210442863076));
#55921=CARTESIAN_POINT('Ctrl Pts',(0.287260497011978,1.95390536437986,4.90255821890697));
#55922=CARTESIAN_POINT('Ctrl Pts',(0.287725767507003,1.9548238367552,4.90262103696446));
#55923=CARTESIAN_POINT('Ctrl Pts',(0.288411766273436,1.95619429187825,4.90271477325147));
#55924=CARTESIAN_POINT('Ctrl Pts',(0.288635853713503,1.9566445935449,4.90274557379243));
#55925=CARTESIAN_POINT('Ctrl Pts',(0.289033283495843,1.95744793463144,4.90280052440996));
#55926=CARTESIAN_POINT('Ctrl Pts',(0.289207035847639,1.95780077101729,4.90282466010733));
#55927=CARTESIAN_POINT('Ctrl Pts',(0.289571640620388,1.9585446011121,4.90287554367883));
#55928=CARTESIAN_POINT('Ctrl Pts',(0.289762347868402,1.95893566474493,4.9029022965523));
#55929=CARTESIAN_POINT('Ctrl Pts',(0.29026324199799,1.95996809812808,4.90297292965072));
#55930=CARTESIAN_POINT('Ctrl Pts',(0.290572093748385,1.96061010969693,4.90301685619378));
#55931=CARTESIAN_POINT('Ctrl Pts',(0.291953819240987,1.9635068574753,4.90321507413395));
#55932=CARTESIAN_POINT('Ctrl Pts',(0.293002572165233,1.96577294361475,4.90337019803546));
#55933=CARTESIAN_POINT('Ctrl Pts',(0.300553045159915,1.98259782097038,4.90452265563934));
#55934=CARTESIAN_POINT('Ctrl Pts',(0.305991679295684,1.99760683553069,4.90555635586953));
#55935=CARTESIAN_POINT('Ctrl Pts',(0.318073317936753,2.04067516462421,4.90853125377937));
#55936=CARTESIAN_POINT('Ctrl Pts',(0.322099627098489,2.06931079529919,4.91052896425579));
#55937=CARTESIAN_POINT('Ctrl Pts',(0.322293940540496,2.10226162305399,4.91265505538569));
#55938=CARTESIAN_POINT('Ctrl Pts',(0.322237854692327,2.10642402756504,4.91292020236123));
#55939=CARTESIAN_POINT('Ctrl Pts',(0.322083375255219,2.1111250913408,4.9132149238937));
#55940=CARTESIAN_POINT('Ctrl Pts',(0.322064246802898,2.11166572820254,4.91324874687412));
#55941=CARTESIAN_POINT('Ctrl Pts',(0.32203325103478,2.11248350083632,4.9132997979569));
#55942=CARTESIAN_POINT('Ctrl Pts',(0.322022387203129,2.11276067030295,4.91331708171227));
#55943=CARTESIAN_POINT('Ctrl Pts',(0.322002877802161,2.11324251786208,4.91334709518598));
#55944=CARTESIAN_POINT('Ctrl Pts',(0.321994394914889,2.11344720179584,4.91335983405732));
#55945=CARTESIAN_POINT('Ctrl Pts',(0.321976417707225,2.11387120236315,4.91338620044791));
#55946=CARTESIAN_POINT('Ctrl Pts',(0.321966894474799,2.11409051727788,4.91339982626128));
#55947=CARTESIAN_POINT('Ctrl Pts',(0.321943664635465,2.11461316615525,4.91343226907822));
#55948=CARTESIAN_POINT('Ctrl Pts',(0.321929753358055,2.11491649183373,4.91345107452457));
#55949=CARTESIAN_POINT('Ctrl Pts',(0.321899290027875,2.11556082462684,4.9134909732681));
#55950=CARTESIAN_POINT('Ctrl Pts',(0.321882624731105,2.1159018263813,4.91351206022582));
#55951=CARTESIAN_POINT('Ctrl Pts',(0.321835717218445,2.11683133998055,4.91356946292282));
#55952=CARTESIAN_POINT('Ctrl Pts',(0.321804402497657,2.11741979990875,4.91360571968249));
#55953=CARTESIAN_POINT('Ctrl Pts',(0.321701412792414,2.11926002788214,4.91371884817332));
#55954=CARTESIAN_POINT('Ctrl Pts',(0.321624045793445,2.12051148337365,4.91379541489961));
#55955=CARTESIAN_POINT('Ctrl Pts',(0.320123871491914,2.14267647295589,4.9151455171179));
#55956=CARTESIAN_POINT('Ctrl Pts',(0.316671021991063,2.1634059458373,4.91631539996858));
#55957=CARTESIAN_POINT('Ctrl Pts',(0.30416033530231,2.20995006885759,4.9190095336928));
#55958=CARTESIAN_POINT('Ctrl Pts',(0.293790381414986,2.23523860195805,4.92053236685435));
#55959=CARTESIAN_POINT('Ctrl Pts',(0.279521873082247,2.26041081259793,4.92228499936186));
#55960=CARTESIAN_POINT('Ctrl Pts',(0.278665838976018,2.26189334866414,4.92238911129845));
#55961=CARTESIAN_POINT('Ctrl Pts',(0.277474157852359,2.2639197229722,4.92253266741629));
#55962=CARTESIAN_POINT('Ctrl Pts',(0.277148634100527,2.26446950617699,4.92257174382178));
#55963=CARTESIAN_POINT('Ctrl Pts',(0.276628496067899,2.26534204799168,4.92263396535432));
#55964=CARTESIAN_POINT('Ctrl Pts',(0.276434945627879,2.26566544149166,4.92265707164365));
#55965=CARTESIAN_POINT('Ctrl Pts',(0.276057875014385,2.26629296871717,4.92270199574014));
#55966=CARTESIAN_POINT('Ctrl Pts',(0.275874418336761,2.2665971401556,4.92272381120328));
#55967=CARTESIAN_POINT('Ctrl Pts',(0.275435318834114,2.26732245359808,4.92277592753903));
#55968=CARTESIAN_POINT('Ctrl Pts',(0.275179213030766,2.26774331298386,4.92280624535523));
#55969=CARTESIAN_POINT('Ctrl Pts',(0.274411543463086,2.26899833717915,4.92289688769907));
#55970=CARTESIAN_POINT('Ctrl Pts',(0.273897147919139,2.26983075540977,4.92295731628401));
#55971=CARTESIAN_POINT('Ctrl Pts',(0.269465085201235,2.2769304097023,4.92347537566626));
#55972=CARTESIAN_POINT('Ctrl Pts',(0.265336967146784,2.28306305288221,4.92394079015998));
#55973=CARTESIAN_POINT('Ctrl Pts',(0.25733055427579,2.29411680371633,4.92481456216514));
#55974=CARTESIAN_POINT('Ctrl Pts',(0.253512465989989,2.29907729438206,4.92522054433851));
#55975=CARTESIAN_POINT('Ctrl Pts',(0.229418085230222,2.32856297125221,4.92771881997399));
#55976=CARTESIAN_POINT('Ctrl Pts',(0.205749159318426,2.35008116908336,4.92993498557596));
#55977=CARTESIAN_POINT('Ctrl Pts',(0.178597806776332,2.36826245160499,4.93205933604973));
#55978=CARTESIAN_POINT('Ctrl Pts',(0.177879215421006,2.36873947286963,4.93211527549247));
#55979=CARTESIAN_POINT('Ctrl Pts',(0.177031379824794,2.36929739957222,4.93218093515087));
#55980=CARTESIAN_POINT('Ctrl Pts',(0.176903989608042,2.36938110052481,4.93219079171582));
#55981=CARTESIAN_POINT('Ctrl Pts',(0.176281323502011,2.36978958725832,4.93223892501936));
#55982=CARTESIAN_POINT('Ctrl Pts',(0.175785208840704,2.37011309996359,4.93227713897255));
#55983=CARTESIAN_POINT('Ctrl Pts',(0.172033118376223,2.37254509505325,4.93256510292587));
#55984=CARTESIAN_POINT('Ctrl Pts',(0.1687400240406,2.37459612210321,4.93281190831192));
#55985=CARTESIAN_POINT('Ctrl Pts',(0.164905471058264,2.37688934170053,4.9330918218446));
#55986=CARTESIAN_POINT('Ctrl Pts',(0.164399587554018,2.37719000262882,4.93312860246759));
#55987=CARTESIAN_POINT('Ctrl Pts',(0.163649232140557,2.37763318338571,4.93318293591792));
#55988=CARTESIAN_POINT('Ctrl Pts',(0.163405395117226,2.37777676746829,4.93320055767154));
#55989=CARTESIAN_POINT('Ctrl Pts',(0.162972193694406,2.37803109147877,4.93323180278278));
#55990=CARTESIAN_POINT('Ctrl Pts',(0.16278290536923,2.37814195919908,4.93324543450341));
#55991=CARTESIAN_POINT('Ctrl Pts',(0.16238659063629,2.3783735408355,4.93327393153319));
#55992=CARTESIAN_POINT('Ctrl Pts',(0.16217954336044,2.37849421676593,4.93328879434037));
#55993=CARTESIAN_POINT('Ctrl Pts',(0.161632407778791,2.3788122935003,4.93332800496262));
#55994=CARTESIAN_POINT('Ctrl Pts',(0.161292091125194,2.37900930377969,4.9333523273292));
#55995=CARTESIAN_POINT('Ctrl Pts',(0.160543749364406,2.3794406942097,4.93340566712659));
#55996=CARTESIAN_POINT('Ctrl Pts',(0.160135568931605,2.37967480510382,4.93343466733614));
#55997=CARTESIAN_POINT('Ctrl Pts',(0.158926096305574,2.38036497925462,4.93352032456823));
#55998=CARTESIAN_POINT('Ctrl Pts',(0.158123350016578,2.3808185034968,4.93357682318576));
#55999=CARTESIAN_POINT('Ctrl Pts',(0.155307865814115,2.38239325525237,4.93377378738386));
#56000=CARTESIAN_POINT('Ctrl Pts',(0.153285007730874,2.38349636836024,4.9339131753335));
#56001=CARTESIAN_POINT('Ctrl Pts',(0.143727730534213,2.38857597279667,4.93456262951908));
#56002=CARTESIAN_POINT('Ctrl Pts',(0.136048807342316,2.39227469719597,4.93505813523177));
#56003=CARTESIAN_POINT('Ctrl Pts',(0.101801745661704,2.40712785768207,4.93719304753925));
#56004=CARTESIAN_POINT('Ctrl Pts',(0.0739545566416514,2.41499518762634,
4.93874921222989));
#56005=CARTESIAN_POINT('Ctrl Pts',(0.0355731158524276,2.42046042553011,
4.9410035141464));
#56006=CARTESIAN_POINT('Ctrl Pts',(0.0256560087534891,2.4214063929849,4.94159402708941));
#56007=CARTESIAN_POINT('Ctrl Pts',(0.0146678372804947,2.42194273162756,
4.94226296312359));
#56008=CARTESIAN_POINT('Ctrl Pts',(0.0136237293338335,2.42198860516654,
4.94232666906711));
#56009=CARTESIAN_POINT('Ctrl Pts',(0.0120627116730934,2.42204958315988,
4.94242213388536));
#56010=CARTESIAN_POINT('Ctrl Pts',(0.0115459516608255,2.42206852379841,
4.94245377258649));
#56011=CARTESIAN_POINT('Ctrl Pts',(0.0106563176493978,2.42209898740388,
4.94250830329072));
#56012=CARTESIAN_POINT('Ctrl Pts',(0.0102834639957898,2.42211110685414,
4.94253117656916));
#56013=CARTESIAN_POINT('Ctrl Pts',(0.00951430126319144,2.42213477131627,
4.94257840150632));
#56014=CARTESIAN_POINT('Ctrl Pts',(0.00911799037340792,2.42214623243005,
4.94260275575507));
#56015=CARTESIAN_POINT('Ctrl Pts',(0.00819614545506967,2.42217118926649,
4.94265945604237));
#56016=CARTESIAN_POINT('Ctrl Pts',(0.0076705986699563,2.42218413043557,
4.94269181939801));
#56017=CARTESIAN_POINT('Ctrl Pts',(0.00599829233637522,2.42222121555949,
4.94279492396209));
#56018=CARTESIAN_POINT('Ctrl Pts',(0.00485144411905283,2.42224052306163,
4.94286581645272));
#56019=CARTESIAN_POINT('Ctrl Pts',(-0.0183774249295346,2.42250755496071,
4.9443055311557));
#56020=CARTESIAN_POINT('Ctrl Pts',(-0.0404223272764245,2.42049107446837,
4.94574808159247));
#56021=CARTESIAN_POINT('Ctrl Pts',(-0.0643358711676005,2.41579635396005,
4.94738540654633));
#56022=CARTESIAN_POINT('Ctrl Pts',(-0.0665828307877071,2.41533025221395,
4.94753990778047));
#56023=CARTESIAN_POINT('Ctrl Pts',(-0.0707411789875144,2.41442123023292,
4.94782694680699));
#56024=CARTESIAN_POINT('Ctrl Pts',(-0.0726538807611539,2.41398477345302,
4.94795941364434));
#56025=CARTESIAN_POINT('Ctrl Pts',(-0.0906458012331739,2.40970601789076,
4.94920922434033));
#56026=CARTESIAN_POINT('Ctrl Pts',(-0.106411610203028,2.40464913410129,
4.95033431165134));
#56027=CARTESIAN_POINT('Ctrl Pts',(-0.128772903870237,2.39552788300091,
4.95192261183336));
#56028=CARTESIAN_POINT('Ctrl Pts',(-0.135721989468169,2.39240170012366,
4.95241481061547));
#56029=CARTESIAN_POINT('Ctrl Pts',(-0.143172776405399,2.38872687298559,
4.95293600480697));
#56030=CARTESIAN_POINT('Ctrl Pts',(-0.143790213867807,2.38841987709633,
4.95297914523595));
#56031=CARTESIAN_POINT('Ctrl Pts',(-0.144656409135474,2.38798572353584,
4.95303959060412));
#56032=CARTESIAN_POINT('Ctrl Pts',(-0.144905988589138,2.38786022326276,
4.95305699804221));
#56033=CARTESIAN_POINT('Ctrl Pts',(-0.145338757143185,2.38764190145123,
4.95308716657351));
#56034=CARTESIAN_POINT('Ctrl Pts',(-0.145522020748349,2.38754922930911,
4.95309993705138));
#56035=CARTESIAN_POINT('Ctrl Pts',(-0.14589015847889,2.3873626285457,4.95312558013461));
#56036=CARTESIAN_POINT('Ctrl Pts',(-0.146075030331999,2.38726869676218,
4.95313845246242));
#56037=CARTESIAN_POINT('Ctrl Pts',(-0.146521737729971,2.38704118589238,
4.95316954381583));
#56038=CARTESIAN_POINT('Ctrl Pts',(-0.146783482308285,2.3869074264445,4.95318775143665));
#56039=CARTESIAN_POINT('Ctrl Pts',(-0.147622961103616,2.38647697774722,
4.95324611644008));
#56040=CARTESIAN_POINT('Ctrl Pts',(-0.1481999862815,2.38617889773293,4.95328618666301));
#56041=CARTESIAN_POINT('Ctrl Pts',(-0.149551259978411,2.38547567295452,
4.95337992023138));
#56042=CARTESIAN_POINT('Ctrl Pts',(-0.150324773973997,2.38506911719797,
4.95343349712333));
#56043=CARTESIAN_POINT('Ctrl Pts',(-0.152988342000505,2.38365530073962,
4.95361774609478));
#56044=CARTESIAN_POINT('Ctrl Pts',(-0.15487004916085,2.38263232448624,4.9537474901944));
#56045=CARTESIAN_POINT('Ctrl Pts',(-0.162762212164817,2.37823931880452,
4.95429046856925));
#56046=CARTESIAN_POINT('Ctrl Pts',(-0.168674362870796,2.37469552090784,
4.95469430417393));
#56047=CARTESIAN_POINT('Ctrl Pts',(-0.179591400865977,2.36766625739586,
4.95544310770418));
#56048=CARTESIAN_POINT('Ctrl Pts',(-0.18461969152328,2.36422314723462,4.95578931756166));
#56049=CARTESIAN_POINT('Ctrl Pts',(-0.208382651068145,2.34694176439733,
4.95744652111076));
#56050=CARTESIAN_POINT('Ctrl Pts',(-0.225676777211939,2.33124347392579,
4.95872327563729));
#56051=CARTESIAN_POINT('Ctrl Pts',(-0.243510518413488,2.31113193993891,
4.96027835107427));
#56052=CARTESIAN_POINT('Ctrl Pts',(-0.245847687628171,2.3084058105027,4.96048750253086));
#56053=CARTESIAN_POINT('Ctrl Pts',(-0.249426807870841,2.30408703493889,
4.96081680344968));
#56054=CARTESIAN_POINT('Ctrl Pts',(-0.250700201293458,2.3025207622361,4.96093582178142));
#56055=CARTESIAN_POINT('Ctrl Pts',(-0.255625107782704,2.29634550081298,
4.9614036739144));
#56056=CARTESIAN_POINT('Ctrl Pts',(-0.259164738971889,2.29164911354047,
4.96175650744875));
#56057=CARTESIAN_POINT('Ctrl Pts',(-0.263147745531854,2.2860521959901,4.96217469634275));
#56058=CARTESIAN_POINT('Ctrl Pts',(-0.26371800117585,2.28524300643413,4.96223510156464));
#56059=CARTESIAN_POINT('Ctrl Pts',(-0.26457170138322,2.28401967907161,4.96232634352333));
#56060=CARTESIAN_POINT('Ctrl Pts',(-0.26485792528649,2.28360748042186,4.96235707408239));
#56061=CARTESIAN_POINT('Ctrl Pts',(-0.265366673574097,2.28287115343142,
4.9624119463717));
#56062=CARTESIAN_POINT('Ctrl Pts',(-0.265589570266834,2.28254728254462,
4.96243607387539));
#56063=CARTESIAN_POINT('Ctrl Pts',(-0.266058238527429,2.28186362798819,
4.96248698809765));
#56064=CARTESIAN_POINT('Ctrl Pts',(-0.266303874046762,2.28150375240767,
4.96251377991105));
#56065=CARTESIAN_POINT('Ctrl Pts',(-0.266950802510136,2.28055181041424,
4.96258462536978));
#56066=CARTESIAN_POINT('Ctrl Pts',(-0.267350853876713,2.27995890676172,
4.9626287258372));
#56067=CARTESIAN_POINT('Ctrl Pts',(-0.269153972644418,2.27726727810525,
4.96282882397911));
#56068=CARTESIAN_POINT('Ctrl Pts',(-0.270534292955428,2.27515348877182,
4.96298567365845));
#56069=CARTESIAN_POINT('Ctrl Pts',(-0.27646299142556,2.26583712897176,4.96367587801448));
#56070=CARTESIAN_POINT('Ctrl Pts',(-0.280749260932982,2.25847261461545,
4.96421877064474));
#56071=CARTESIAN_POINT('Ctrl Pts',(-0.298757239437896,2.22450342002641,
4.96671262057183));
#56072=CARTESIAN_POINT('Ctrl Pts',(-0.309022719174845,2.19623639185006,
4.96877833908566));
#56073=CARTESIAN_POINT('Ctrl Pts',(-0.315558407868929,2.16547067616215,
4.97086902698191));
#56074=CARTESIAN_POINT('Ctrl Pts',(-0.315865786832819,2.16397126731309,
4.97097049201869));
#56075=CARTESIAN_POINT('Ctrl Pts',(-0.31784894469439,2.15393440094963,4.97164660841912));
#56076=CARTESIAN_POINT('Ctrl Pts',(-0.31918926896389,2.14533336180689,4.97221121623603));
#56077=CARTESIAN_POINT('Ctrl Pts',(-0.320260804481919,2.13598190569201,
4.97280187248485));
#56078=CARTESIAN_POINT('Ctrl Pts',(-0.320339353353755,2.13527575853472,
4.97284633134776));
#56079=CARTESIAN_POINT('Ctrl Pts',(-0.320445921569804,2.1342880015794,4.97290831526014));
#56080=CARTESIAN_POINT('Ctrl Pts',(-0.320475905508153,2.13400661249329,
4.97292594978955));
#56081=CARTESIAN_POINT('Ctrl Pts',(-0.320527107307109,2.13352001886538,
4.97295640376962));
#56082=CARTESIAN_POINT('Ctrl Pts',(-0.32054849876368,2.13331483339738,4.97296923303459));
#56083=CARTESIAN_POINT('Ctrl Pts',(-0.320591059542951,2.13290275699368,
4.9729949729349));
#56084=CARTESIAN_POINT('Ctrl Pts',(-0.320612225587194,2.1326958664191,4.973007883319));
#56085=CARTESIAN_POINT('Ctrl Pts',(-0.320655156004477,2.13227218653559,
4.97303429580221));
#56086=CARTESIAN_POINT('Ctrl Pts',(-0.320676900863282,2.13205539501295,
4.97304779680586));
#56087=CARTESIAN_POINT('Ctrl Pts',(-0.320726893598553,2.13155183640301,
4.97307912465446));
#56088=CARTESIAN_POINT('Ctrl Pts',(-0.320754976805667,2.13126505259401,
4.97309694222366));
#56089=CARTESIAN_POINT('Ctrl Pts',(-0.320826916153189,2.13052011344701,
4.9731431628323));
#56090=CARTESIAN_POINT('Ctrl Pts',(-0.320870175738407,2.13006189915664,
4.97317153271127));
#56091=CARTESIAN_POINT('Ctrl Pts',(-0.32181409468499,2.1198295138048,4.97380374020075));
#56092=CARTESIAN_POINT('Ctrl Pts',(-0.322268816889106,2.11001837458985,
4.9743830666047));
#56093=CARTESIAN_POINT('Ctrl Pts',(-0.322274937371842,2.10020091534284,
4.97494943677011));
#56094=CARTESIAN_POINT('',(-0.322021731191934,2.09973199008727,5.22472278440197));
#56095=CARTESIAN_POINT('Ctrl Pts',(-0.322274937078364,2.10020138554251,
4.97494940964423));
#56096=CARTESIAN_POINT('Ctrl Pts',(-0.322285045080913,2.08402566684362,
4.97588258911077));
#56097=CARTESIAN_POINT('Ctrl Pts',(-0.321077299150837,2.06787059725422,
4.97677927466193));
#56098=CARTESIAN_POINT('Ctrl Pts',(-0.314995452800083,2.02760098425642,
4.97905824022963));
#56099=CARTESIAN_POINT('Ctrl Pts',(-0.308569406782582,2.00383133143984,
4.98044985199316));
#56100=CARTESIAN_POINT('Ctrl Pts',(-0.299083168913247,1.97995099337579,
4.98201236551914));
#56101=CARTESIAN_POINT('Ctrl Pts',(-0.298651617283599,1.97888139136204,
4.98208269263931));
#56102=CARTESIAN_POINT('Ctrl Pts',(-0.298014570617035,1.97732657602321,
4.98218543030167));
#56103=CARTESIAN_POINT('Ctrl Pts',(-0.297813609123736,1.97683950525542,
4.98221768735976));
#56104=CARTESIAN_POINT('Ctrl Pts',(-0.297459266665263,1.97598662312765,
4.98227429953891));
#56105=CARTESIAN_POINT('Ctrl Pts',(-0.297306402710333,1.97562059706895,
4.98229863707631));
#56106=CARTESIAN_POINT('Ctrl Pts',(-0.297008598236242,1.97491120310649,
4.98234588680405));
#56107=CARTESIAN_POINT('Ctrl Pts',(-0.296863736989732,1.97456780240623,
4.98236879626946));
#56108=CARTESIAN_POINT('Ctrl Pts',(-0.296516977586349,1.9737497577096,4.98242345954799));
#56109=CARTESIAN_POINT('Ctrl Pts',(-0.29631453545269,1.9732753467164,4.98245523185294));
#56110=CARTESIAN_POINT('Ctrl Pts',(-0.295700521480166,1.97184595754359,
4.98255117746212));
#56111=CARTESIAN_POINT('Ctrl Pts',(-0.295285468521383,1.97089249037709,
4.98261546947633));
#56112=CARTESIAN_POINT('Ctrl Pts',(-0.290926355204326,1.96100963677147,
4.98328493776214));
#56113=CARTESIAN_POINT('Ctrl Pts',(-0.2865835314591,1.95226269427122,4.98390380151509));
#56114=CARTESIAN_POINT('Ctrl Pts',(-0.269002211865862,1.92055337908637,
4.98625051312027));
#56115=CARTESIAN_POINT('Ctrl Pts',(-0.253345668210878,1.89905508372831,
4.98806199798688));
#56116=CARTESIAN_POINT('Ctrl Pts',(-0.231727110796095,1.87596847033774,
4.99018778715869));
#56117=CARTESIAN_POINT('Ctrl Pts',(-0.228125502853717,1.8723020890074,4.99053127295136));
#56118=CARTESIAN_POINT('Ctrl Pts',(-0.219891384771832,1.8643114613683,4.99129062357023));
#56119=CARTESIAN_POINT('Ctrl Pts',(-0.215215694283978,1.8600343265057,4.99170457842632));
#56120=CARTESIAN_POINT('Ctrl Pts',(-0.208106270461783,1.8539059937815,4.9923053726836));
#56121=CARTESIAN_POINT('Ctrl Pts',(-0.205767634006069,1.8519472593076,4.99249863541314));
#56122=CARTESIAN_POINT('Ctrl Pts',(-0.203008678567032,1.84970236029569,
4.99272124499645));
#56123=CARTESIAN_POINT('Ctrl Pts',(-0.202615163983639,1.84938370494463,
4.99275287033279));
#56124=CARTESIAN_POINT('Ctrl Pts',(-0.202051548841236,1.84892950284937,
4.99279798443158));
#56125=CARTESIAN_POINT('Ctrl Pts',(-0.201882062134013,1.84879320089258,
4.99281152745962));
#56126=CARTESIAN_POINT('Ctrl Pts',(-0.201550025902481,1.84852672895536,
4.99283801321791));
#56127=CARTESIAN_POINT('Ctrl Pts',(-0.201387487766252,1.84839654461164,
4.99285095698887));
#56128=CARTESIAN_POINT('Ctrl Pts',(-0.201063352672803,1.84813744508352,
4.9928767265649));
#56129=CARTESIAN_POINT('Ctrl Pts',(-0.20090175815639,1.8480085280662,4.99288955251658));
#56130=CARTESIAN_POINT('Ctrl Pts',(-0.200517398105693,1.84770249768361,
4.99292000952176));
#56131=CARTESIAN_POINT('Ctrl Pts',(-0.200294521334867,1.84752552338336,
4.99293763052492));
#56132=CARTESIAN_POINT('Ctrl Pts',(-0.199625109026554,1.84699542383421,
4.99299043666155));
#56133=CARTESIAN_POINT('Ctrl Pts',(-0.199177868935805,1.84664318392328,
4.9930255587589));
#56134=CARTESIAN_POINT('Ctrl Pts',(-0.194800624192822,1.84321448263786,
4.99336779169078));
#56135=CARTESIAN_POINT('Ctrl Pts',(-0.190800324775829,1.84022831586212,
4.99366865473377));
#56136=CARTESIAN_POINT('Ctrl Pts',(-0.186472322953587,1.83715146963094,
4.99398362557414));
#56137=CARTESIAN_POINT('Ctrl Pts',(-0.186212361882987,1.83696723886878,
4.99400250457603));
#56138=CARTESIAN_POINT('Ctrl Pts',(-0.184431822847895,1.83570935842939,
4.99413154346191));
#56139=CARTESIAN_POINT('Ctrl Pts',(-0.182902211796027,1.83464849408067,
4.9942410609518));
#56140=CARTESIAN_POINT('Ctrl Pts',(-0.170434786230683,1.82616071882682,
4.99512368523359));
#56141=CARTESIAN_POINT('Ctrl Pts',(-0.159057739484304,1.81939946929525,
4.99586745403962));
#56142=CARTESIAN_POINT('Ctrl Pts',(-0.13746713155384,1.80830478646286,4.99722617819139));
#56143=CARTESIAN_POINT('Ctrl Pts',(-0.127384300725526,1.80376268755188,
4.99784129090588));
#56144=CARTESIAN_POINT('Ctrl Pts',(-0.101031843765891,1.79348612395394,
4.99943781658683));
#56145=CARTESIAN_POINT('Ctrl Pts',(-0.0845012519627029,1.78852350216596,
5.00043034144248));
#56146=CARTESIAN_POINT('Ctrl Pts',(-0.0651026808327272,1.7843583852689,
5.00162606144927));
#56147=CARTESIAN_POINT('Ctrl Pts',(-0.0625442860651763,1.78384149597908,
5.00178431716365));
#56148=CARTESIAN_POINT('Ctrl Pts',(-0.0592688166274296,1.78322104416558,
5.0019877296404));
#56149=CARTESIAN_POINT('Ctrl Pts',(-0.0585572342652978,1.78308873515493,
5.00203196816155));
#56150=CARTESIAN_POINT('Ctrl Pts',(-0.0574146976721475,1.7828802755536,
5.00210307783264));
#56151=CARTESIAN_POINT('Ctrl Pts',(-0.056984020711297,1.78280260322265,
5.00212990048609));
#56152=CARTESIAN_POINT('Ctrl Pts',(-0.0561665108796347,1.78265688450705,
5.00218084983699));
#56153=CARTESIAN_POINT('Ctrl Pts',(-0.0557797088943821,1.78258866754848,
5.00220497105818));
#56154=CARTESIAN_POINT('Ctrl Pts',(-0.05490175715466,1.78243548508362,5.00225975449271));
#56155=CARTESIAN_POINT('Ctrl Pts',(-0.0544105339023778,1.78235095172698,
5.00229043038341));
#56156=CARTESIAN_POINT('Ctrl Pts',(-0.0529586595425619,1.78210456899808,
5.00238116889875));
#56157=CARTESIAN_POINT('Ctrl Pts',(-0.0519974748410022,1.78194593659375,
5.00244133350966));
#56158=CARTESIAN_POINT('Ctrl Pts',(-0.0455260274660343,1.78090801858261,
5.00284705095586));
#56159=CARTESIAN_POINT('Ctrl Pts',(-0.0399947413692446,1.78016765930278,
5.00319698100972));
#56160=CARTESIAN_POINT('Ctrl Pts',(-0.0325023336891928,1.7793621973218,
5.003675625501));
#56161=CARTESIAN_POINT('Ctrl Pts',(-0.0305555478140931,1.77917082359186,
5.00380041271909));
#56162=CARTESIAN_POINT('Ctrl Pts',(-0.0048009350987952,1.7768756204169,
5.00545684222292));
#56163=CARTESIAN_POINT('Ctrl Pts',(0.0191640134420057,1.77740923559079,
5.00706951958968));
#56164=CARTESIAN_POINT('Ctrl Pts',(0.0535259227642527,1.78201842300329,
5.00941478483482));
#56165=CARTESIAN_POINT('Ctrl Pts',(0.0641286817172353,1.78398600873702,
5.01014172067818));
#56166=CARTESIAN_POINT('Ctrl Pts',(0.0795297220992006,1.78765125519509,
5.01118703679555));
#56167=CARTESIAN_POINT('Ctrl Pts',(0.0844181516588503,1.78893682889579,
5.0115171786066));
#56168=CARTESIAN_POINT('Ctrl Pts',(0.0916596000014079,1.79102450830991,
5.01200182180603));
#56169=CARTESIAN_POINT('Ctrl Pts',(0.0940366823353032,1.7917396555413,5.0121601912217));
#56170=CARTESIAN_POINT('Ctrl Pts',(0.0973345286285136,1.79277351449441,
5.01237867326754));
#56171=CARTESIAN_POINT('Ctrl Pts',(0.0982624009441628,1.79306902327,5.01244000804325));
#56172=CARTESIAN_POINT('Ctrl Pts',(0.0996548334102818,1.79351944665416,
5.01253183071055));
#56173=CARTESIAN_POINT('Ctrl Pts',(0.100120393080221,1.79367121862601,5.01256249441605));
#56174=CARTESIAN_POINT('Ctrl Pts',(0.100971991974085,1.79395098780339,5.01261851379667));
#56175=CARTESIAN_POINT('Ctrl Pts',(0.101358137245699,1.79407865545512,5.01264388839978));
#56176=CARTESIAN_POINT('Ctrl Pts',(0.101974146494986,1.79428361528847,5.01268432432849));
#56177=CARTESIAN_POINT('Ctrl Pts',(0.102204165083954,1.7943604360118,5.01269941342867));
#56178=CARTESIAN_POINT('Ctrl Pts',(0.102641565350218,1.7945070662561,5.01272808785687));
#56179=CARTESIAN_POINT('Ctrl Pts',(0.102848960970675,1.79457682679176,5.01274167589739));
#56180=CARTESIAN_POINT('Ctrl Pts',(0.103319718082555,1.79473570667262,5.01277250052962));
#56181=CARTESIAN_POINT('Ctrl Pts',(0.103583034892043,1.79482495546117,5.01278972930331));
#56182=CARTESIAN_POINT('Ctrl Pts',(0.104379841921049,1.79509617590237,5.01284182609504));
#56183=CARTESIAN_POINT('Ctrl Pts',(0.104912974113302,1.7952792077608,5.01287663148807));
#56184=CARTESIAN_POINT('Ctrl Pts',(0.108620466812036,1.79656292605023,5.0131183310444));
#56185=CARTESIAN_POINT('Ctrl Pts',(0.111778073282456,1.79771184583542,5.01332242958655));
#56186=CARTESIAN_POINT('Ctrl Pts',(0.137235139330595,1.80742806616125,5.01495803001313));
#56187=CARTESIAN_POINT('Ctrl Pts',(0.158539998096427,1.81840238153108,5.01626889402307));
#56188=CARTESIAN_POINT('Ctrl Pts',(0.197976332303377,1.84462369416768,5.01892183769232));
#56189=CARTESIAN_POINT('Ctrl Pts',(0.216034177682866,1.85970710688899,5.02025711030116));
#56190=CARTESIAN_POINT('Ctrl Pts',(0.233091693737246,1.87744492204922,5.02175356272773));
#56191=CARTESIAN_POINT('Ctrl Pts',(0.233885045666559,1.87827881073132,5.02182374491815));
#56192=CARTESIAN_POINT('Ctrl Pts',(0.235034730272235,1.87950027586249,5.02192630967003));
#56193=CARTESIAN_POINT('Ctrl Pts',(0.235394613413208,1.87988451042756,5.02195853948149));
#56194=CARTESIAN_POINT('Ctrl Pts',(0.236023954099939,1.88055974388594,5.02201512010935));
#56195=CARTESIAN_POINT('Ctrl Pts',(0.236293819689449,1.88085036233963,5.02203945340265));
#56196=CARTESIAN_POINT('Ctrl Pts',(0.236816341037455,1.88141515320515,5.02208670687443));
#56197=CARTESIAN_POINT('Ctrl Pts',(0.23706905894509,1.88168926751126,5.02210962435014));
#56198=CARTESIAN_POINT('Ctrl Pts',(0.237739473036178,1.88241897917038,5.02217058915443));
#56199=CARTESIAN_POINT('Ctrl Pts',(0.23815633363553,1.88287533902027,5.02220867185819));
#56200=CARTESIAN_POINT('Ctrl Pts',(0.239635076218769,1.88450358059975,5.02234439114973));
#56201=CARTESIAN_POINT('Ctrl Pts',(0.240689629006266,1.88568206123985,5.02244233604848));
#56202=CARTESIAN_POINT('Ctrl Pts',(0.259141142097004,1.90660988922329,5.02417685142317));
#56203=CARTESIAN_POINT('Ctrl Pts',(0.274059139456869,1.9284049288921,5.02592064059716));
#56204=CARTESIAN_POINT('Ctrl Pts',(0.293787468080232,1.96648934222579,5.02882061511528));
#56205=CARTESIAN_POINT('Ctrl Pts',(0.300267564250743,1.98178148318281,5.0299482434542));
#56206=CARTESIAN_POINT('Ctrl Pts',(0.307094746972246,2.00213363090361,5.03135562599535));
#56207=CARTESIAN_POINT('Ctrl Pts',(0.30854212526078,2.00679714375217,5.03167191579786));
#56208=CARTESIAN_POINT('Ctrl Pts',(0.310320612606232,2.01302396104813,5.03208448085106));
#56209=CARTESIAN_POINT('Ctrl Pts',(0.310746809413888,2.01455917464978,5.0321854199144));
#56210=CARTESIAN_POINT('Ctrl Pts',(0.311344605301387,2.01677616675163,5.03233000337358));
#56211=CARTESIAN_POINT('Ctrl Pts',(0.311525378488111,2.01745541659061,5.03237414205912));
#56212=CARTESIAN_POINT('Ctrl Pts',(0.311842432005389,2.01866261308421,5.03245229818241));
#56213=CARTESIAN_POINT('Ctrl Pts',(0.311979596768773,2.01919032162126,5.03248636504559));
#56214=CARTESIAN_POINT('Ctrl Pts',(0.312180118579282,2.01996990167836,5.03253654463823));
#56215=CARTESIAN_POINT('Ctrl Pts',(0.312244510550553,2.02022150223443,5.03255271693116));
#56216=CARTESIAN_POINT('Ctrl Pts',(0.312361825730554,2.02068220895086,5.0325822883727));
#56217=CARTESIAN_POINT('Ctrl Pts',(0.312414843192067,2.02089129058684,5.03259569299979));
#56218=CARTESIAN_POINT('Ctrl Pts',(0.312519471399414,2.02130565189407,5.03262222722457));
#56219=CARTESIAN_POINT('Ctrl Pts',(0.312571089637877,2.02151092846271,5.03263535724331));
#56220=CARTESIAN_POINT('Ctrl Pts',(0.312711262192331,2.02207070106962,5.03267112078711));
#56221=CARTESIAN_POINT('Ctrl Pts',(0.312799416272429,2.02242529847646,5.03269373105243));
#56222=CARTESIAN_POINT('Ctrl Pts',(0.313130266685761,2.02376586886925,5.03277904370457));
#56223=CARTESIAN_POINT('Ctrl Pts',(0.313368909141737,2.0247528504716,5.03284151438046));
#56224=CARTESIAN_POINT('Ctrl Pts',(0.31775834800345,2.04328986196905,5.03400872135404));
#56225=CARTESIAN_POINT('Ctrl Pts',(0.32043413285657,2.06115956095556,5.03503251121383));
#56226=CARTESIAN_POINT('Ctrl Pts',(0.321702277965392,2.08073103206813,5.03613286385662));
#56227=CARTESIAN_POINT('Ctrl Pts',(0.321792475893252,2.08230109426493,5.03622098277257));
#56228=CARTESIAN_POINT('Ctrl Pts',(0.322671373706601,2.09984125062288,5.03720423402327));
#56229=CARTESIAN_POINT('Ctrl Pts',(0.322281959900942,2.1158479015747,5.03809191552928));
#56230=CARTESIAN_POINT('Ctrl Pts',(0.319277074930664,2.14619171240716,5.03983607345623));
#56231=CARTESIAN_POINT('Ctrl Pts',(0.316875384936777,2.16050975003607,5.04068567357673));
#56232=CARTESIAN_POINT('Ctrl Pts',(0.313263205060972,2.1756871980551,5.04163473331104));
#56233=CARTESIAN_POINT('Ctrl Pts',(0.313002831729384,2.17675685556859,5.04170187709708));
#56234=CARTESIAN_POINT('Ctrl Pts',(0.312612150057299,2.17832679294692,5.04180080945977));
#56235=CARTESIAN_POINT('Ctrl Pts',(0.312486108524085,2.17882813477021,5.04183246028464));
#56236=CARTESIAN_POINT('Ctrl Pts',(0.312261592242,2.17971216836523,5.04188837430691));
#56237=CARTESIAN_POINT('Ctrl Pts',(0.312163618613665,2.18009498727615,5.04191262126205));
#56238=CARTESIAN_POINT('Ctrl Pts',(0.311971106357432,2.18084148454154,5.04195996986228));
#56239=CARTESIAN_POINT('Ctrl Pts',(0.311876635219036,2.18120517980618,5.04198306929006));
#56240=CARTESIAN_POINT('Ctrl Pts',(0.31164807551653,2.18207880763858,5.0420386312419));
#56241=CARTESIAN_POINT('Ctrl Pts',(0.311513371500428,2.18258857673849,5.04207111366669));
#56242=CARTESIAN_POINT('Ctrl Pts',(0.311097370856156,2.18414737706962,5.04217063004478));
#56243=CARTESIAN_POINT('Ctrl Pts',(0.310812023904342,2.18519531073634,5.04223779526339));
#56244=CARTESIAN_POINT('Ctrl Pts',(0.307401108742523,2.19747662277672,5.04302807715991));
#56245=CARTESIAN_POINT('Ctrl Pts',(0.303673786495036,2.20853252481737,5.0437708343792));
#56246=CARTESIAN_POINT('Ctrl Pts',(0.289255985146281,2.24469216422925,5.04630973299465));
#56247=CARTESIAN_POINT('Ctrl Pts',(0.275981755803391,2.26863738590936,5.0481853382273));
#56248=CARTESIAN_POINT('Ctrl Pts',(0.253661686238835,2.29906426559523,5.05070377191487));
#56249=CARTESIAN_POINT('Ctrl Pts',(0.247059235152875,2.30720187155542,5.05139128886121));
#56250=CARTESIAN_POINT('Ctrl Pts',(0.239413697998304,2.31573879830375,5.05211587425953));
#56251=CARTESIAN_POINT('Ctrl Pts',(0.238752494286659,2.31647030838679,5.05217798906159));
#56252=CARTESIAN_POINT('Ctrl Pts',(0.237754891682736,2.3175638556859,5.05227087026417));
#56253=CARTESIAN_POINT('Ctrl Pts',(0.237421007742963,2.31792816456326,5.05230181723936));
#56254=CARTESIAN_POINT('Ctrl Pts',(0.23688152300107,2.31851409810551,5.05235159516165));
#56255=CARTESIAN_POINT('Ctrl Pts',(0.23667644760993,2.31873620221328,5.05237046505801));
#56256=CARTESIAN_POINT('Ctrl Pts',(0.236283789201891,2.31916026683631,5.05240649491942));
#56257=CARTESIAN_POINT('Ctrl Pts',(0.236096259156231,2.31936227572936,5.05242365886563));
#56258=CARTESIAN_POINT('Ctrl Pts',(0.235761926266498,2.3197214964769,5.05245418124618));
#56259=CARTESIAN_POINT('Ctrl Pts',(0.235615225219009,2.31987880192731,5.05246754745773));
#56260=CARTESIAN_POINT('Ctrl Pts',(0.235322598288376,2.32019195248919,5.05249415615056));
#56261=CARTESIAN_POINT('Ctrl Pts',(0.235176675583811,2.32034779887298,5.05250739877382));
#56262=CARTESIAN_POINT('Ctrl Pts',(0.234774322725495,2.32077665933305,5.05254384099689));
#56263=CARTESIAN_POINT('Ctrl Pts',(0.234517570276904,2.32104937265749,5.05256701577288));
#56264=CARTESIAN_POINT('Ctrl Pts',(0.233444142118669,2.32218555458504,5.05266357452925));
#56265=CARTESIAN_POINT('Ctrl Pts',(0.232623155139511,2.3230449639695,5.05273663027835));
#56266=CARTESIAN_POINT('Ctrl Pts',(0.218533372782861,2.33763173342188,5.05397733815393));
#56267=CARTESIAN_POINT('Ctrl Pts',(0.204073050422405,2.3501601476604,5.05505520457786));
#56268=CARTESIAN_POINT('Ctrl Pts',(0.175155981008347,2.37102741479991,5.0570524258703));
#56269=CARTESIAN_POINT('Ctrl Pts',(0.160998725708501,2.37966920374122,5.05797113804771));
#56270=CARTESIAN_POINT('Ctrl Pts',(0.140343932853513,2.39018708462406,5.05929804833022));
#56271=CARTESIAN_POINT('Ctrl Pts',(0.13435639512478,2.39300736378414,5.05968102060005));
#56272=CARTESIAN_POINT('Ctrl Pts',(0.121124344038216,2.39874909985578,5.06052824351389));
#56273=CARTESIAN_POINT('Ctrl Pts',(0.113852095929765,2.40159545122321,5.0609944560831));
#56274=CARTESIAN_POINT('Ctrl Pts',(0.10554948159414,2.40450199200812,5.0615300147376));
#56275=CARTESIAN_POINT('Ctrl Pts',(0.104613361828836,2.40482486889071,5.06159044383869));
#56276=CARTESIAN_POINT('Ctrl Pts',(0.103207043588835,2.40530268071623,5.06168129791067));
#56277=CARTESIAN_POINT('Ctrl Pts',(0.102737945945071,2.40546085699733,5.06171161562632));
#56278=CARTESIAN_POINT('Ctrl Pts',(0.101931307225233,2.40573078133177,5.06176376993145));
#56279=CARTESIAN_POINT('Ctrl Pts',(0.101593941276093,2.40584305311827,5.06178558918454));
#56280=CARTESIAN_POINT('Ctrl Pts',(0.100899451990349,2.40607289584898,5.06183051897494));
#56281=CARTESIAN_POINT('Ctrl Pts',(0.100542307411169,2.40619040057439,5.06185363165984));
#56282=CARTESIAN_POINT('Ctrl Pts',(0.0996830626629651,2.40647143666381,
5.06190925583489));
#56283=CARTESIAN_POINT('Ctrl Pts',(0.0991807658248759,2.40663435906262,
5.06194178732419));
#56284=CARTESIAN_POINT('Ctrl Pts',(0.0976410772466343,2.40712958546628,
5.06204155240271));
#56285=CARTESIAN_POINT('Ctrl Pts',(0.0966024072354025,2.40745786232287,
5.06210891815628));
#56286=CARTESIAN_POINT('Ctrl Pts',(0.084285899739606,2.41128198362624,5.06290854171715));
#56287=CARTESIAN_POINT('Ctrl Pts',(0.0728271702375305,2.41416035920824,
5.06366094794572));
#56288=CARTESIAN_POINT('Ctrl Pts',(0.0346019510344244,2.42155855938874,
5.0662017146396));
#56289=CARTESIAN_POINT('Ctrl Pts',(0.00742329798941937,2.42332917726726,
5.06806759087787));
#56290=CARTESIAN_POINT('Ctrl Pts',(-0.0300907877523687,2.42103760141242,
5.07057580847388));
#56291=CARTESIAN_POINT('Ctrl Pts',(-0.0404957642956893,2.41989176032202,
5.0712625553953));
#56292=CARTESIAN_POINT('Ctrl Pts',(-0.0523008765267065,2.41800632049263,
5.07201841007402));
#56293=CARTESIAN_POINT('Ctrl Pts',(-0.0537725429164855,2.41776078328165,
5.07211221664668));
#56294=CARTESIAN_POINT('Ctrl Pts',(-0.0556433804115265,2.41743527753573,
5.07223088488691));
#56295=CARTESIAN_POINT('Ctrl Pts',(-0.0560441464761551,2.41736476625156,
5.07225627162892));
#56296=CARTESIAN_POINT('Ctrl Pts',(-0.0566854172699531,2.41725068767852,
5.07229683754336));
#56297=CARTESIAN_POINT('Ctrl Pts',(-0.0569260061898422,2.41720760581012,
5.07231204430483));
#56298=CARTESIAN_POINT('Ctrl Pts',(-0.0573824715228527,2.41712533125735,
5.0723408716858));
#56299=CARTESIAN_POINT('Ctrl Pts',(-0.0575983551238477,2.41708619214727,
5.07235449519227));
#56300=CARTESIAN_POINT('Ctrl Pts',(-0.0580928781320035,2.41699601476829,
5.07238567908276));
#56301=CARTESIAN_POINT('Ctrl Pts',(-0.058371489918554,2.41694482963885,
5.07240323094593));
#56302=CARTESIAN_POINT('Ctrl Pts',(-0.0592302010320829,2.4167859009375,
5.07245727628635));
#56303=CARTESIAN_POINT('Ctrl Pts',(-0.0598100763818755,2.41667693083535,
5.07249370003249));
#56304=CARTESIAN_POINT('Ctrl Pts',(-0.0642341636128275,2.41583297163124,
5.07277106087828));
#56305=CARTESIAN_POINT('Ctrl Pts',(-0.0680652047929457,2.41502956208742,
5.0730081875616));
#56306=CARTESIAN_POINT('Ctrl Pts',(-0.0991596439612118,2.4079149709497,
5.07491485403923));
#56307=CARTESIAN_POINT('Ctrl Pts',(-0.125513030189108,2.39814627749829,
5.07642607198489));
#56308=CARTESIAN_POINT('Ctrl Pts',(-0.165231814284946,2.37721014769211,
5.07896246564542));
#56309=CARTESIAN_POINT('Ctrl Pts',(-0.179542591847503,2.36816293869034,
5.07993725185203));
#56310=CARTESIAN_POINT('Ctrl Pts',(-0.195144269511299,2.3564889039339,5.08111176575143));
#56311=CARTESIAN_POINT('Ctrl Pts',(-0.197193102325694,2.35491709154408,
5.08126835171411));
#56312=CARTESIAN_POINT('Ctrl Pts',(-0.199789545535448,2.35287513325113,
5.08146990713136));
#56313=CARTESIAN_POINT('Ctrl Pts',(-0.200354809388862,2.35242750615471,
5.0815139788756));
#56314=CARTESIAN_POINT('Ctrl Pts',(-0.201260250690224,2.35170553847089,
5.08158488393191));
#56315=CARTESIAN_POINT('Ctrl Pts',(-0.201601382816849,2.35143239458783,
5.0816116692467));
#56316=CARTESIAN_POINT('Ctrl Pts',(-0.202248150215842,2.35091236662254,
5.08166258879869));
#56317=CARTESIAN_POINT('Ctrl Pts',(-0.202553891895389,2.35066561564306,
5.08168671765172));
#56318=CARTESIAN_POINT('Ctrl Pts',(-0.203247320558231,2.35010388207035,
5.08174157481916));
#56319=CARTESIAN_POINT('Ctrl Pts',(-0.203634727298463,2.34978855653204,
5.08177231695273));
#56320=CARTESIAN_POINT('Ctrl Pts',(-0.204779362116287,2.34885246076335,
5.08186342887907));
#56321=CARTESIAN_POINT('Ctrl Pts',(-0.205534490851644,2.34822914295706,
5.08192390191535));
#56322=CARTESIAN_POINT('Ctrl Pts',(-0.210646742006857,2.34396993652484,
5.08233581711139));
#56323=CARTESIAN_POINT('Ctrl Pts',(-0.214909776044909,2.34022314916051,
5.08269178983913));
#56324=CARTESIAN_POINT('Ctrl Pts',(-0.219976533234906,2.33552711785698,
5.08313079215456));
#56325=CARTESIAN_POINT('Ctrl Pts',(-0.220876761198919,2.33468309422648,
5.08320942332677));
#56326=CARTESIAN_POINT('Ctrl Pts',(-0.226198130864565,2.32963621597357,
5.08367800649076));
#56327=CARTESIAN_POINT('Ctrl Pts',(-0.230503834916903,2.32531391566893,
5.08407283026291));
#56328=CARTESIAN_POINT('Ctrl Pts',(-0.251979375367832,2.30249544232156,
5.08612418117315));
#56329=CARTESIAN_POINT('Ctrl Pts',(-0.267055321515111,2.28215159696037,
5.08785533599168));
#56330=CARTESIAN_POINT('Ctrl Pts',(-0.284020248806697,2.25255364193745,
5.09013874298989));
#56331=CARTESIAN_POINT('Ctrl Pts',(-0.288118235529243,2.24466521202856,
5.09072619161299));
#56332=CARTESIAN_POINT('Ctrl Pts',(-0.293519304037409,2.23312570164678,
5.09154620641875));
#56333=CARTESIAN_POINT('Ctrl Pts',(-0.295090686226717,2.22960526404774,
5.09179129964355));
#56334=CARTESIAN_POINT('Ctrl Pts',(-0.296809184386449,2.22556183142715,
5.09206636977017));
#56335=CARTESIAN_POINT('Ctrl Pts',(-0.297018519677702,2.22506584036391,
5.09210000219524));
#56336=CARTESIAN_POINT('Ctrl Pts',(-0.297332086313077,2.22431765977784,
5.09215056814716));
#56337=CARTESIAN_POINT('Ctrl Pts',(-0.297437240494103,2.22406586175295,
5.09216755751857));
#56338=CARTESIAN_POINT('Ctrl Pts',(-0.297625961574288,2.22361233877598,
5.09219810612257));
#56339=CARTESIAN_POINT('Ctrl Pts',(-0.297709643081217,2.22341066290273,
5.09221167233033));
#56340=CARTESIAN_POINT('Ctrl Pts',(-0.297889059914329,2.22297701648203,
5.09224080307109));
#56341=CARTESIAN_POINT('Ctrl Pts',(-0.297984728986997,2.22274501982174,
5.09225636351185));
#56342=CARTESIAN_POINT('Ctrl Pts',(-0.298241726796195,2.22211973111332,
5.09229823815228));
#56343=CARTESIAN_POINT('Ctrl Pts',(-0.298402549229552,2.22172622949794,
5.09232452156681));
#56344=CARTESIAN_POINT('Ctrl Pts',(-0.299139804960049,2.21991206470504,
5.09244538471539));
#56345=CARTESIAN_POINT('Ctrl Pts',(-0.299706886859887,2.21848758737001,
5.09253940710168));
#56346=CARTESIAN_POINT('Ctrl Pts',(-0.311864296941188,2.18730307825963,
5.09457973190748));
#56347=CARTESIAN_POINT('Ctrl Pts',(-0.318979528599732,2.15598244022577,
5.09628545726322));
#56348=CARTESIAN_POINT('Ctrl Pts',(-0.321969437543412,2.11614891405994,
5.09854943707508));
#56349=CARTESIAN_POINT('Ctrl Pts',(-0.322270950202066,2.10815656070147,
5.09900739530887));
#56350=CARTESIAN_POINT('Ctrl Pts',(-0.322279716646284,2.09067528164424,
5.10002592410256));
#56351=CARTESIAN_POINT('Ctrl Pts',(-0.321865625026729,2.08119418185082,
5.10058925107366));
#56352=CARTESIAN_POINT('Ctrl Pts',(-0.320933513765265,2.07060321553701,
5.10123579416297));
#56353=CARTESIAN_POINT('Ctrl Pts',(-0.320826858603185,2.06946120598247,
5.10130573314836));
#56354=CARTESIAN_POINT('Ctrl Pts',(-0.320662991998946,2.06780230437277,
5.10140765999625));
#56355=CARTESIAN_POINT('Ctrl Pts',(-0.320610621314186,2.06728493409842,
5.1014394954748));
#56356=CARTESIAN_POINT('Ctrl Pts',(-0.320516059384775,2.066372794886,5.10149570614405));
#56357=CARTESIAN_POINT('Ctrl Pts',(-0.320474390321553,2.06597797194295,
5.10152006484342));
#56358=CARTESIAN_POINT('Ctrl Pts',(-0.320386805594868,2.06516252798548,
5.10157043149906));
#56359=CARTESIAN_POINT('Ctrl Pts',(-0.320340790950744,2.06474191857204,
5.10159644252975));
#56360=CARTESIAN_POINT('Ctrl Pts',(-0.320221019099625,2.06366670256384,
5.10166301694102));
#56361=CARTESIAN_POINT('Ctrl Pts',(-0.320146083147756,2.06301223160768,
5.10170361741313));
#56362=CARTESIAN_POINT('Ctrl Pts',(-0.319833205707336,2.06035184133243,
5.10186897457095));
#56363=CARTESIAN_POINT('Ctrl Pts',(-0.319578417977619,2.05834798416497,
5.10199426158106));
#56364=CARTESIAN_POINT('Ctrl Pts',(-0.315110225282228,2.02566511415882,
5.1040500691332));
#56365=CARTESIAN_POINT('Ctrl Pts',(-0.306516127007977,1.99575475164704,
5.10613370126422));
#56366=CARTESIAN_POINT('Ctrl Pts',(-0.287853086921499,1.95436104566144,
5.10920349140419));
#56367=CARTESIAN_POINT('Ctrl Pts',(-0.281031677762897,1.9415974197239,5.11017512544206));
#56368=CARTESIAN_POINT('Ctrl Pts',(-0.271216533664863,1.92587535603576,
5.11137033799005));
#56369=CARTESIAN_POINT('Ctrl Pts',(-0.268991779029281,1.92245781789046,
5.11162998218112));
#56370=CARTESIAN_POINT('Ctrl Pts',(-0.26640072138197,1.91863815030557,5.11191917492675));
#56371=CARTESIAN_POINT('Ctrl Pts',(-0.266097685937063,1.91819382181492,
5.11195280004526));
#56372=CARTESIAN_POINT('Ctrl Pts',(-0.265637133960592,1.91752215154401,
5.11200360322074));
#56373=CARTESIAN_POINT('Ctrl Pts',(-0.265480436609093,1.91729425325081,
5.11202083617721));
#56374=CARTESIAN_POINT('Ctrl Pts',(-0.2652072772758,1.91689806776479,5.11205078606386));
#56375=CARTESIAN_POINT('Ctrl Pts',(-0.265090948321882,1.91672968972943,
5.11206351205307));
#56376=CARTESIAN_POINT('Ctrl Pts',(-0.264846753241866,1.91637695335379,
5.11209016605967));
#56377=CARTESIAN_POINT('Ctrl Pts',(-0.264718855019159,1.91619261777585,
5.11210409178066));
#56378=CARTESIAN_POINT('Ctrl Pts',(-0.264411480430327,1.91575059496508,
5.11213747699517));
#56379=CARTESIAN_POINT('Ctrl Pts',(-0.264231819082923,1.91549303529349,
5.11215692381319));
#56380=CARTESIAN_POINT('Ctrl Pts',(-0.263616616120723,1.9146138315163,5.11222328758627));
#56381=CARTESIAN_POINT('Ctrl Pts',(-0.263179250656773,1.91399345761182,
5.11227008066282));
#56382=CARTESIAN_POINT('Ctrl Pts',(-0.262130447270882,1.91251690447786,
5.11238138716638));
#56383=CARTESIAN_POINT('Ctrl Pts',(-0.261516996229678,1.91166215662917,
5.11244576723247));
#56384=CARTESIAN_POINT('Ctrl Pts',(-0.25396362616563,1.90124578291539,5.11322988744973));
#56385=CARTESIAN_POINT('Ctrl Pts',(-0.246506309745506,1.89206859775676,
5.11391622223745));
#56386=CARTESIAN_POINT('Ctrl Pts',(-0.217350367933014,1.85996829302401,
5.11638458808503));
#56387=CARTESIAN_POINT('Ctrl Pts',(-0.192827395105979,1.83985757320203,
5.11808734392856));
#56388=CARTESIAN_POINT('Ctrl Pts',(-0.165100649834053,1.82322650957429,
5.11999929621495));
#56389=CARTESIAN_POINT('Ctrl Pts',(-0.164427243152219,1.8228259188302,5.12004571186467));
#56390=CARTESIAN_POINT('Ctrl Pts',(-0.159018062486628,1.81963479878462,
5.12041840638111));
#56391=CARTESIAN_POINT('Ctrl Pts',(-0.154213293777334,1.81696352759643,
5.12074860954042));
#56392=CARTESIAN_POINT('Ctrl Pts',(-0.148559776674896,1.81400708203306,
5.12113705437957));
#56393=CARTESIAN_POINT('Ctrl Pts',(-0.147775102054241,1.81360084573901,
5.12119096569368));
#56394=CARTESIAN_POINT('Ctrl Pts',(-0.14652381581915,1.81295954990248,5.12127693562017));
#56395=CARTESIAN_POINT('Ctrl Pts',(-0.146058282230693,1.8127223872608,5.12130892019706));
#56396=CARTESIAN_POINT('Ctrl Pts',(-0.145237615255287,1.81230681501058,
5.12136530508642));
#56397=CARTESIAN_POINT('Ctrl Pts',(-0.144882723817743,1.81212792787193,
5.12138968858301));
#56398=CARTESIAN_POINT('Ctrl Pts',(-0.144150179515521,1.8117603781812,5.12144002040104));
#56399=CARTESIAN_POINT('Ctrl Pts',(-0.143772485195432,1.8115718003755,5.12146597163043));
#56400=CARTESIAN_POINT('Ctrl Pts',(-0.142808385927782,1.81109280253147,
5.1215322164389));
#56401=CARTESIAN_POINT('Ctrl Pts',(-0.142221467024086,1.81080342645902,
5.12157254639289));
#56402=CARTESIAN_POINT('Ctrl Pts',(-0.139850669662212,1.80964348477773,
5.12173546560285));
#56403=CARTESIAN_POINT('Ctrl Pts',(-0.138059676498706,1.80878763560113,
5.12185856564488));
#56404=CARTESIAN_POINT('Ctrl Pts',(-0.126350141681476,1.80332438175122,
5.12266368052197));
#56405=CARTESIAN_POINT('Ctrl Pts',(-0.116211501170433,1.79920834159235,
5.1233624795124));
#56406=CARTESIAN_POINT('Ctrl Pts',(-0.0770503066071499,1.7855855831329,
5.12606999354659));
#56407=CARTESIAN_POINT('Ctrl Pts',(-0.046943100351864,1.77970468702387,
5.12818630696107));
#56408=CARTESIAN_POINT('Ctrl Pts',(-0.0153677196784037,1.77808975162365,
5.13026843510386));
#56409=CARTESIAN_POINT('Ctrl Pts',(-0.0142737823858288,1.77803939059718,
5.13034037735279));
#56410=CARTESIAN_POINT('Ctrl Pts',(-0.0116690858419834,1.77793278103843,
5.13051118243553));
#56411=CARTESIAN_POINT('Ctrl Pts',(-0.010158132163823,1.77788158451176,
5.13060987108058));
#56412=CARTESIAN_POINT('Ctrl Pts',(-0.00849108474651263,1.7778368404287,
5.13071828295553));
#56413=CARTESIAN_POINT('Ctrl Pts',(-0.00833531671228995,1.7778327726155,
5.13072840835777));
#56414=CARTESIAN_POINT('Ctrl Pts',(-0.00805012154474173,1.7778255318473,
5.13074693852835));
#56415=CARTESIAN_POINT('Ctrl Pts',(-0.00792069541683257,1.77782232391028,
5.13075534465113));
#56416=CARTESIAN_POINT('Ctrl Pts',(-0.00680945594168689,1.77779545091379,
5.1308274913965));
#56417=CARTESIAN_POINT('Ctrl Pts',(-0.00582752944657534,1.77777619565147,
5.13089105916989));
#56418=CARTESIAN_POINT('Ctrl Pts',(-0.000655327699106262,1.77769842097698,
5.1312248790249));
#56419=CARTESIAN_POINT('Ctrl Pts',(0.00353594717595642,1.77771714514683,
5.1314918759806));
#56420=CARTESIAN_POINT('Ctrl Pts',(0.0082676932618976,1.77783061197874,
5.13178845024824));
#56421=CARTESIAN_POINT('Ctrl Pts',(0.00880945400669028,1.77784497076702,
5.13182233456962));
#56422=CARTESIAN_POINT('Ctrl Pts',(0.00962869562767096,1.77786875202025,
5.13187346248299));
#56423=CARTESIAN_POINT('Ctrl Pts',(0.00990620140697552,1.7778771664728,
5.13189076196259));
#56424=CARTESIAN_POINT('Ctrl Pts',(0.0103885174154802,1.77789241498503,
5.13192079513109));
#56425=CARTESIAN_POINT('Ctrl Pts',(0.0105933320553065,1.77789908579023,
5.13193353800224));
#56426=CARTESIAN_POINT('Ctrl Pts',(0.0110221318756865,1.77791346122156,
5.13196019395179));
#56427=CARTESIAN_POINT('Ctrl Pts',(0.0112461152896326,1.77792120413692,
5.1319741047886));
#56428=CARTESIAN_POINT('Ctrl Pts',(0.0117826324977038,1.77794031142885,
5.13200739551768));
#56429=CARTESIAN_POINT('Ctrl Pts',(0.0120951592698433,1.77795189714061,
5.13202676291682));
#56430=CARTESIAN_POINT('Ctrl Pts',(0.0131585098058498,1.7779928667846,5.13209257627652));
#56431=CARTESIAN_POINT('Ctrl Pts',(0.0139092547403826,1.77802442191818,
5.13213890112612));
#56432=CARTESIAN_POINT('Ctrl Pts',(0.0156975597044053,1.77810585399429,
5.13224892836011));
#56433=CARTESIAN_POINT('Ctrl Pts',(0.0167350097324752,1.77815812247363,
5.13231250142758));
#56434=CARTESIAN_POINT('Ctrl Pts',(0.0292834884766979,1.77885117658798,
5.13307853371981));
#56435=CARTESIAN_POINT('Ctrl Pts',(0.0407537751593051,1.78010426418285,
5.13374915848192));
#56436=CARTESIAN_POINT('Ctrl Pts',(0.0726210816245385,1.78532814360564,
5.13558938850359));
#56437=CARTESIAN_POINT('Ctrl Pts',(0.092736571261693,1.79065846965798,5.13672705814357));
#56438=CARTESIAN_POINT('Ctrl Pts',(0.119255394257325,1.80050714583129,5.13833211620569));
#56439=CARTESIAN_POINT('Ctrl Pts',(0.126216437450541,1.80337360179638,5.13876353147201));
#56440=CARTESIAN_POINT('Ctrl Pts',(0.141770288126491,1.8104251319774,5.13975826371954));
#56441=CARTESIAN_POINT('Ctrl Pts',(0.150289691357093,1.81475379026526,5.14032539026622));
#56442=CARTESIAN_POINT('Ctrl Pts',(0.159603974827992,1.82001952376744,5.14097604735303));
#56443=CARTESIAN_POINT('Ctrl Pts',(0.160601167524356,1.82059033519116,5.141046109356));
#56444=CARTESIAN_POINT('Ctrl Pts',(0.162045520927383,1.82142739621505,5.14114818270856));
#56445=CARTESIAN_POINT('Ctrl Pts',(0.162495130696303,1.82168942002301,5.14118004105223));
#56446=CARTESIAN_POINT('Ctrl Pts',(0.163286687866008,1.82215329610949,5.14123627840878));
#56447=CARTESIAN_POINT('Ctrl Pts',(0.163628901384876,1.82235469403137,5.14126064088062));
#56448=CARTESIAN_POINT('Ctrl Pts',(0.164327457883124,1.82276754536333,5.14131047318749));
#56449=CARTESIAN_POINT('Ctrl Pts',(0.164683766902341,1.82297905452023,5.14133594502139));
#56450=CARTESIAN_POINT('Ctrl Pts',(0.165585756467785,1.82351684119085,5.14140056439152));
#56451=CARTESIAN_POINT('Ctrl Pts',(0.166130879387406,1.82384404631657,5.1414397457614));
#56452=CARTESIAN_POINT('Ctrl Pts',(0.167307801958041,1.82455522942232,5.14152461800237));
#56453=CARTESIAN_POINT('Ctrl Pts',(0.16793925458826,1.824939772071,5.14157032945591));
#56454=CARTESIAN_POINT('Ctrl Pts',(0.169738432072969,1.82604394193958,5.14170107762166));
#56455=CARTESIAN_POINT('Ctrl Pts',(0.170902882731435,1.82676884941304,5.14178630844597));
#56456=CARTESIAN_POINT('Ctrl Pts',(0.181936421360456,1.83373570460249,5.14259977101199));
#56457=CARTESIAN_POINT('Ctrl Pts',(0.191462885565185,1.84050155263272,5.14334754010476));
#56458=CARTESIAN_POINT('Ctrl Pts',(0.218837672325478,1.86227280956496,5.14563850887266));
#56459=CARTESIAN_POINT('Ctrl Pts',(0.235446867315453,1.87871126883502,5.14723100970842));
#56460=CARTESIAN_POINT('Ctrl Pts',(0.258964221731378,1.90765990091767,5.14973802926356));
#56461=CARTESIAN_POINT('Ctrl Pts',(0.267075657761865,1.91909151874405,5.15066512796842));
#56462=CARTESIAN_POINT('Ctrl Pts',(0.274880006191671,1.93176524669219,5.15160086912769));
#56463=CARTESIAN_POINT('Ctrl Pts',(0.275338367135858,1.93251646752497,5.15165600397935));
#56464=CARTESIAN_POINT('Ctrl Pts',(0.275953856730147,1.93353456673698,5.1517302707603));
#56465=CARTESIAN_POINT('Ctrl Pts',(0.276113680676089,1.93379979885345,5.15174957692328));
#56466=CARTESIAN_POINT('Ctrl Pts',(0.276383062739164,1.93424830665128,5.15178215290319));
#56467=CARTESIAN_POINT('Ctrl Pts',(0.276492821015366,1.93443146088517,5.15179543584986));
#56468=CARTESIAN_POINT('Ctrl Pts',(0.27670373915598,1.93478421576785,5.15182098031268));
#56469=CARTESIAN_POINT('Ctrl Pts',(0.276804924396527,1.93495379903676,5.15183324343165));
#56470=CARTESIAN_POINT('Ctrl Pts',(0.277045192114745,1.93535732259782,5.15186238299627));
#56471=CARTESIAN_POINT('Ctrl Pts',(0.277184134030369,1.93559134591149,5.15187925014069));
#56472=CARTESIAN_POINT('Ctrl Pts',(0.277595271819646,1.93628583809265,5.15192921045948));
#56473=CARTESIAN_POINT('Ctrl Pts',(0.277866619623585,1.93674681180957,5.1519622483578));
#56474=CARTESIAN_POINT('Ctrl Pts',(0.280031522978218,1.94044564865951,5.15222637213945));
#56475=CARTESIAN_POINT('Ctrl Pts',(0.281869665871285,1.94371583787578,5.15245393640567));
#56476=CARTESIAN_POINT('Ctrl Pts',(0.288300240432539,1.95563900236441,5.15326510037742));
#56477=CARTESIAN_POINT('Ctrl Pts',(0.292555032621645,1.9644687736137,5.15383121011053));
#56478=CARTESIAN_POINT('Ctrl Pts',(0.308502694031347,2.00182954216195,5.15614063547757));
#56479=CARTESIAN_POINT('Ctrl Pts',(0.316473918900532,2.03176751124718,5.15780730371048));
#56480=CARTESIAN_POINT('Ctrl Pts',(0.32083882184001,2.06890692824254,5.16001497058225));
#56481=CARTESIAN_POINT('Ctrl Pts',(0.321405891622924,2.07545265401265,5.1604083568191));
#56482=CARTESIAN_POINT('Ctrl Pts',(0.321830377040606,2.08304541903164,5.1608711804083));
#56483=CARTESIAN_POINT('Ctrl Pts',(0.321883228015103,2.08408029883549,5.16093440096425));
#56484=CARTESIAN_POINT('Ctrl Pts',(0.321954378170445,2.08561916828983,5.16102862197144));
#56485=CARTESIAN_POINT('Ctrl Pts',(0.321976487207062,2.08612298212779,5.16105950293105));
#56486=CARTESIAN_POINT('Ctrl Pts',(0.322013740584781,2.08701996492306,5.1611145437547));
#56487=CARTESIAN_POINT('Ctrl Pts',(0.322029347648736,2.08741311449356,5.16113868906402));
#56488=CARTESIAN_POINT('Ctrl Pts',(0.322058106416754,2.08817265327619,5.16118537673314));
#56489=CARTESIAN_POINT('Ctrl Pts',(0.322071352961083,2.08853903846443,5.16120791608106));
#56490=CARTESIAN_POINT('Ctrl Pts',(0.322105694241859,2.08953599376847,5.16126929693301));
#56491=CARTESIAN_POINT('Ctrl Pts',(0.322125562422325,2.09016660208763,5.16130817682191));
#56492=CARTESIAN_POINT('Ctrl Pts',(0.322195463509988,2.09261350260604,5.16145925332203));
#56493=CARTESIAN_POINT('Ctrl Pts',(0.322231986721765,2.09443011972202,5.1615718723004));
#56494=CARTESIAN_POINT('Ctrl Pts',(0.322418580025097,2.11045169821216,5.16256927685574));
#56495=CARTESIAN_POINT('Ctrl Pts',(0.321644624980028,2.12464984545561,5.16348311104624));
#56496=CARTESIAN_POINT('Ctrl Pts',(0.317895137290635,2.15560800605637,5.16554116404712));
#56497=CARTESIAN_POINT('Ctrl Pts',(0.314524023080926,2.1722781253663,5.16669284883827));
#56498=CARTESIAN_POINT('Ctrl Pts',(0.305867290901938,2.20255160394687,5.16882154949197));
#56499=CARTESIAN_POINT('Ctrl Pts',(0.300941197331393,2.21621576799354,5.16979665749187));
#56500=CARTESIAN_POINT('Ctrl Pts',(0.293498400759003,2.23317642903458,5.17099055628135));
#56501=CARTESIAN_POINT('Ctrl Pts',(0.291817628276304,2.23682013008512,5.17124597609863));
#56502=CARTESIAN_POINT('Ctrl Pts',(0.289810189033462,2.24096660295828,5.17153461194444));
#56503=CARTESIAN_POINT('Ctrl Pts',(0.289549740657808,2.24150080040618,5.17157175826703));
#56504=CARTESIAN_POINT('Ctrl Pts',(0.289163938571284,2.24228658143442,5.17162633776634));
#56505=CARTESIAN_POINT('Ctrl Pts',(0.289039732947551,2.2425387224771,5.1716438419173));
#56506=CARTESIAN_POINT('Ctrl Pts',(0.288817844182879,2.24298768053485,5.17167499250948));
#56507=CARTESIAN_POINT('Ctrl Pts',(0.288720289587857,2.24318456021731,5.17168864699748));
#56508=CARTESIAN_POINT('Ctrl Pts',(0.288514395659611,2.24359901879592,5.17171737908938));
#56509=CARTESIAN_POINT('Ctrl Pts',(0.28840601179599,2.24381657436767,5.17173245379939));
#56510=CARTESIAN_POINT('Ctrl Pts',(0.288118224759445,2.24439260672437,5.17177234929841));
#56511=CARTESIAN_POINT('Ctrl Pts',(0.287938397974384,2.24475087319692,5.17179714348035));
#56512=CARTESIAN_POINT('Ctrl Pts',(0.287113923596844,2.24638584645943,5.17191021057851));
#56513=CARTESIAN_POINT('Ctrl Pts',(0.286461437160134,2.24765861426111,5.17199799820846));
#56514=CARTESIAN_POINT('Ctrl Pts',(0.281308353988924,2.25754771049502,5.17267860771744));
#56515=CARTESIAN_POINT('Ctrl Pts',(0.276427986163082,2.26596168141894,5.17324894535946));
#56516=CARTESIAN_POINT('Ctrl Pts',(0.256734256922605,2.29662861870966,5.17534279486634));
#56517=CARTESIAN_POINT('Ctrl Pts',(0.239553610959685,2.31723146585915,5.17678939251239));
#56518=CARTESIAN_POINT('Ctrl Pts',(0.219924291886246,2.33557270801519,5.17833301241377));
#56519=CARTESIAN_POINT('Ctrl Pts',(0.219822727252329,2.33566748504275,5.17834099644943));
#56520=CARTESIAN_POINT('Ctrl Pts',(0.218761212821919,2.33665677477419,5.17842441294535));
#56521=CARTESIAN_POINT('Ctrl Pts',(0.21779587763854,2.33754547545778,5.17850001910827));
#56522=CARTESIAN_POINT('Ctrl Pts',(0.20825912408366,2.34621813914642,5.17924465101702));
#56523=CARTESIAN_POINT('Ctrl Pts',(0.199280421179306,2.35353994164118,5.17992804960406));
#56524=CARTESIAN_POINT('Ctrl Pts',(0.188967432666075,2.36106301668377,5.18070401411057));
#56525=CARTESIAN_POINT('Ctrl Pts',(0.188003012540059,2.36175839338033,5.18077649114619));
#56526=CARTESIAN_POINT('Ctrl Pts',(0.18663717401669,2.36273176297626,5.18087902101642));
#56527=CARTESIAN_POINT('Ctrl Pts',(0.186238929871124,2.36301421063864,5.18090890255137));
#56528=CARTESIAN_POINT('Ctrl Pts',(0.185541300035437,2.36350661342546,5.18096122490166));
#56529=CARTESIAN_POINT('Ctrl Pts',(0.185242195240774,2.36371696653493,5.18098365042736));
#56530=CARTESIAN_POINT('Ctrl Pts',(0.184613714848363,2.36415736469812,5.18103075590447));
#56531=CARTESIAN_POINT('Ctrl Pts',(0.184284265967452,2.36438730368329,5.18105543985585));
#56532=CARTESIAN_POINT('Ctrl Pts',(0.183506759316075,2.36492780547902,5.18111367452699));
#56533=CARTESIAN_POINT('Ctrl Pts',(0.183058342826739,2.3652378478768,5.18114724498544));
#56534=CARTESIAN_POINT('Ctrl Pts',(0.181568867564697,2.36626211875618,5.18125870369161));
#56535=CARTESIAN_POINT('Ctrl Pts',(0.180524408533545,2.36697136064405,5.18133678068782));
#56536=CARTESIAN_POINT('Ctrl Pts',(0.178050651552201,2.36863001571106,5.18152152569188));
#56537=CARTESIAN_POINT('Ctrl Pts',(0.176617896146414,2.36957417984018,5.18162838867972));
#56538=CARTESIAN_POINT('Ctrl Pts',(0.171574758600473,2.37284006835595,5.18200409272662));
#56539=CARTESIAN_POINT('Ctrl Pts',(0.167925718551589,2.37510098307525,5.18227516160093));
#56540=CARTESIAN_POINT('Ctrl Pts',(0.158555985024941,2.38065050428849,5.18296949346351));
#56541=CARTESIAN_POINT('Ctrl Pts',(0.152777652720028,2.38383742727995,5.1833961552431));
#56542=CARTESIAN_POINT('Ctrl Pts',(0.135213363206224,2.39283288197974,5.184688131128));
#56543=CARTESIAN_POINT('Ctrl Pts',(0.123166561089593,2.39810014522031,5.18556838158964));
#56544=CARTESIAN_POINT('Ctrl Pts',(0.100782104942607,2.40629840500096,5.18717882015782));
#56545=CARTESIAN_POINT('Ctrl Pts',(0.0905540495958589,2.40947651557396,
5.18790546814082));
#56546=CARTESIAN_POINT('Ctrl Pts',(0.0668971765186751,2.41555381744271,
5.18954572938213));
#56547=CARTESIAN_POINT('Ctrl Pts',(0.0534012488364664,2.41811609645066,
5.19045283985469));
#56548=CARTESIAN_POINT('Ctrl Pts',(0.0390165034065126,2.41990542714555,
5.19136308624037));
#56549=CARTESIAN_POINT('Ctrl Pts',(0.0382511872849979,2.41999783836065,
5.19141134528465));
#56550=CARTESIAN_POINT('Ctrl Pts',(0.0371944704604102,2.42012159076548,
5.19147773921923));
#56551=CARTESIAN_POINT('Ctrl Pts',(0.0369033554559773,2.42015528086354,
5.19149600495293));
#56552=CARTESIAN_POINT('Ctrl Pts',(0.0364045807530623,2.42021231361684,
5.1915272565701));
#56553=CARTESIAN_POINT('Ctrl Pts',(0.0361969442689838,2.42023585139364,
5.19154025348698));
#56554=CARTESIAN_POINT('Ctrl Pts',(0.0357693584790864,2.42028390155794,
5.19156699123645));
#56555=CARTESIAN_POINT('Ctrl Pts',(0.03554940732181,2.42030838927893,5.19158073056709));
#56556=CARTESIAN_POINT('Ctrl Pts',(0.0350345376077072,2.42036517416729,
5.19161285815161));
#56557=CARTESIAN_POINT('Ctrl Pts',(0.0347395985056996,2.42039729078439,
5.19163123614439));
#56558=CARTESIAN_POINT('Ctrl Pts',(0.0337879300774918,2.42049959067515,
5.1916904528953));
#56559=CARTESIAN_POINT('Ctrl Pts',(0.0331310238048297,2.42056816298829,
5.19173120115618));
#56560=CARTESIAN_POINT('Ctrl Pts',(0.0168108740217263,2.4222210688014,5.1927404946942));
#56561=CARTESIAN_POINT('Ctrl Pts',(0.00105012008026275,2.42265782422649,
5.19364574104255));
#56562=CARTESIAN_POINT('Ctrl Pts',(-0.0334936255536876,2.42108251990121,
5.19559734031623));
#56563=CARTESIAN_POINT('Ctrl Pts',(-0.0521941154928808,2.41857744682543,
5.19663424528499));
#56564=CARTESIAN_POINT('Ctrl Pts',(-0.0765884891096376,2.41310291992299,
5.19805736687232));
#56565=CARTESIAN_POINT('Ctrl Pts',(-0.0825677460721462,2.41157951951921,
5.19841174866557));
#56566=CARTESIAN_POINT('Ctrl Pts',(-0.0979066214174795,2.40719893041556,
5.19934000960093));
#56567=CARTESIAN_POINT('Ctrl Pts',(-0.107185806087738,2.40408561813031,
5.19992047626176));
#56568=CARTESIAN_POINT('Ctrl Pts',(-0.117278766227451,2.40017986144128,
5.20057855681905));
#56569=CARTESIAN_POINT('Ctrl Pts',(-0.118247289734139,2.39979966086297,
5.20064198161484));
#56570=CARTESIAN_POINT('Ctrl Pts',(-0.119693295871762,2.39922392409437,
5.20073709339893));
#56571=CARTESIAN_POINT('Ctrl Pts',(-0.120172184200983,2.39903191797291,
5.20076866144768));
#56572=CARTESIAN_POINT('Ctrl Pts',(-0.120996245324255,2.39869921858108,
5.20082310272895));
#56573=CARTESIAN_POINT('Ctrl Pts',(-0.121341639935803,2.3985590745218,5.20084595737828));
#56574=CARTESIAN_POINT('Ctrl Pts',(-0.122054071500556,2.39826856452117,
5.2008931740433));
#56575=CARTESIAN_POINT('Ctrl Pts',(-0.122421075419096,2.39811811961439,
5.20091753870167));
#56576=CARTESIAN_POINT('Ctrl Pts',(-0.123147036590687,2.39781896173692,
5.2009658160954));
#56577=CARTESIAN_POINT('Ctrl Pts',(-0.123506004520981,2.39767027637351,
5.20098972785973));
#56578=CARTESIAN_POINT('Ctrl Pts',(-0.124690891944273,2.39717698092486,
5.20106878874426));
#56579=CARTESIAN_POINT('Ctrl Pts',(-0.125515639377708,2.39682958203525,
5.20112403252878));
#56580=CARTESIAN_POINT('Ctrl Pts',(-0.13112391867334,2.39443971783413,5.20150115728883));
#56581=CARTESIAN_POINT('Ctrl Pts',(-0.135858607999843,2.39228524256525,
5.20182684583936));
#56582=CARTESIAN_POINT('Ctrl Pts',(-0.1439124217978,2.38838246093822,5.2023939968143));
#56583=CARTESIAN_POINT('Ctrl Pts',(-0.147257067590164,2.38668900068895,
5.2026335381937));
#56584=CARTESIAN_POINT('Ctrl Pts',(-0.161135482297279,2.3793551467279,5.20364452524249));
#56585=CARTESIAN_POINT('Ctrl Pts',(-0.171380001700075,2.37319001940358,
5.20443296575815));
#56586=CARTESIAN_POINT('Ctrl Pts',(-0.205159586133253,2.35021261077742,
5.20716906570496));
#56587=CARTESIAN_POINT('Ctrl Pts',(-0.22676542242463,2.33081238797812,5.20917293808333));
#56588=CARTESIAN_POINT('Ctrl Pts',(-0.246483878120763,2.30762756286976,
5.21109840967081));
#56589=CARTESIAN_POINT('Ctrl Pts',(-0.24746484543768,2.30645739882126,5.21119445853409));
#56590=CARTESIAN_POINT('Ctrl Pts',(-0.248707834553097,2.30495308926973,
5.2113164473278));
#56591=CARTESIAN_POINT('Ctrl Pts',(-0.248977542574868,2.30462536271829,
5.21134293423166));
#56592=CARTESIAN_POINT('Ctrl Pts',(-0.249405587347312,2.30410313942243,
5.211384997083));
#56593=CARTESIAN_POINT('Ctrl Pts',(-0.249564344672945,2.30390899046178,
5.21140060355169));
#56594=CARTESIAN_POINT('Ctrl Pts',(-0.249860907797609,2.30354544962497,
5.21142976740907));
#56595=CARTESIAN_POINT('Ctrl Pts',(-0.249998767015926,2.30337610429794,
5.21144332864786));
#56596=CARTESIAN_POINT('Ctrl Pts',(-0.25030864763161,2.30299465786778,5.21147382135945));
#56597=CARTESIAN_POINT('Ctrl Pts',(-0.250480571219786,2.30278247864338,
5.21149074567707));
#56598=CARTESIAN_POINT('Ctrl Pts',(-0.250991273783402,2.30215055543887,
5.21154104079314));
#56599=CARTESIAN_POINT('Ctrl Pts',(-0.251329271014511,2.30173017652534,
5.2115743551942));
#56600=CARTESIAN_POINT('Ctrl Pts',(-0.254094267568999,2.29827351836931,
5.21184713112828));
#56601=CARTESIAN_POINT('Ctrl Pts',(-0.256467338468236,2.29519424298539,
5.21208280714787));
#56602=CARTESIAN_POINT('Ctrl Pts',(-0.264064411276896,2.28495851690477,
5.21284531377718));
#56603=CARTESIAN_POINT('Ctrl Pts',(-0.269049428639147,2.27762909967955,
5.21335870854257));
#56604=CARTESIAN_POINT('Ctrl Pts',(-0.284019051411226,2.25354027504166,
5.21497575069274));
#56605=CARTESIAN_POINT('Ctrl Pts',(-0.29278742907882,2.23607722545153,5.21604669004016));
#56606=CARTESIAN_POINT('Ctrl Pts',(-0.300792637237424,2.2157177855621,5.2172834079808));
#56607=CARTESIAN_POINT('Ctrl Pts',(-0.301637256681434,2.21349793680584,
5.21741806057806));
#56608=CARTESIAN_POINT('Ctrl Pts',(-0.304631272000374,2.20535944513291,
5.2179114739331));
#56609=CARTESIAN_POINT('Ctrl Pts',(-0.30663154489143,2.19938769776535,5.21827306740836));
#56610=CARTESIAN_POINT('Ctrl Pts',(-0.31129230346613,2.18398907768822,5.21920922880558));
#56611=CARTESIAN_POINT('Ctrl Pts',(-0.313700180163125,2.17449316125589,
5.21979020794796));
#56612=CARTESIAN_POINT('Ctrl Pts',(-0.315881528741162,2.16388363264929,
5.22044884215179));
#56613=CARTESIAN_POINT('Ctrl Pts',(-0.316086178221075,2.16286323741401,
5.22051228143699));
#56614=CARTESIAN_POINT('Ctrl Pts',(-0.316384897315462,2.16133545988705,
5.22060741141829));
#56615=CARTESIAN_POINT('Ctrl Pts',(-0.316482697994233,2.16082880694437,
5.22063898311141));
#56616=CARTESIAN_POINT('Ctrl Pts',(-0.316649052538471,2.15995575119867,
5.22069342900424));
#56617=CARTESIAN_POINT('Ctrl Pts',(-0.316718188492703,2.15958945922992,
5.22071628461343));
#56618=CARTESIAN_POINT('Ctrl Pts',(-0.316859576463072,2.1588331687754,5.22076350169901));
#56619=CARTESIAN_POINT('Ctrl Pts',(-0.316931744286872,2.15844315533578,
5.22078786581536));
#56620=CARTESIAN_POINT('Ctrl Pts',(-0.317073178982807,2.15767083966702,
5.2208361416299));
#56621=CARTESIAN_POINT('Ctrl Pts',(-0.317142474875327,2.15728854340972,
5.22086005235616));
#56622=CARTESIAN_POINT('Ctrl Pts',(-0.317301096401533,2.15640434146702,
5.22091538800589));
#56623=CARTESIAN_POINT('Ctrl Pts',(-0.31738992259949,2.15590234826415,5.22094682877375));
#56624=CARTESIAN_POINT('Ctrl Pts',(-0.317616246264796,2.15460537188408,
5.22102812563903));
#56625=CARTESIAN_POINT('Ctrl Pts',(-0.31775194961828,2.15381008292821,5.22107803865954));
#56626=CARTESIAN_POINT('Ctrl Pts',(-0.320822267103388,2.13539982626745,
5.22223496737217));
#56627=CARTESIAN_POINT('Ctrl Pts',(-0.322290159470362,2.11757536368981,
5.22338921839787));
#56628=CARTESIAN_POINT('Ctrl Pts',(-0.322274881976907,2.09972418888649,
5.22457701413596));
#56629=CARTESIAN_POINT('',(-0.322324149694691,2.09995053291872,5.34972264852953));
#56630=CARTESIAN_POINT('Ctrl Pts',(-0.322021731191934,2.09973199008727,
5.22472278440197));
#56631=CARTESIAN_POINT('Ctrl Pts',(-0.322284766309565,2.06580495458856,
5.22681356126889));
#56632=CARTESIAN_POINT('Ctrl Pts',(-0.301715959323295,1.92471043066922,
5.23552778597674));
#56633=CARTESIAN_POINT('Ctrl Pts',(-0.0967559193787474,1.73141707993042,
5.25086545852553));
#56634=CARTESIAN_POINT('Ctrl Pts',(0.257535391016418,1.81912529612678,5.27073580204831));
#56635=CARTESIAN_POINT('Ctrl Pts',(0.375573040431588,2.16449781548873,5.29060614557111));
#56636=CARTESIAN_POINT('Ctrl Pts',(0.149073554903257,2.45070236972446,5.31047648909389));
#56637=CARTESIAN_POINT('Ctrl Pts',(-0.211166715081224,2.41547992794995,
5.33018196904799));
#56638=CARTESIAN_POINT('Ctrl Pts',(-0.322574663534915,2.20410493244714,
5.34326400116115));
#56639=CARTESIAN_POINT('Ctrl Pts',(-0.322798140628015,2.09995147753102,
5.34972258543339));
#56640=CARTESIAN_POINT('',(-0.322274866580731,2.10029324967485,5.47472265506957));
#56641=CARTESIAN_POINT('Ctrl Pts',(-0.322274996188514,2.09995043496114,
5.34972265507269));
#56642=CARTESIAN_POINT('Ctrl Pts',(-0.322274588015624,2.0972964691886,5.34988749542828));
#56643=CARTESIAN_POINT('Ctrl Pts',(-0.322241396999529,2.09464278843267,
5.35005233578388));
#56644=CARTESIAN_POINT('Ctrl Pts',(-0.32217544030333,2.091989925696,5.35021717613947));
#56645=CARTESIAN_POINT('Ctrl Pts',(-0.321736399743732,2.07433115247729,
5.351314435495));
#56646=CARTESIAN_POINT('Ctrl Pts',(-0.319839819770441,2.0566532640631,5.35241169485053));
#56647=CARTESIAN_POINT('Ctrl Pts',(-0.316490882531739,2.03921598154711,
5.35350895420606));
#56648=CARTESIAN_POINT('Ctrl Pts',(-0.313148351723602,2.02181205610285,
5.35460411453274));
#56649=CARTESIAN_POINT('Ctrl Pts',(-0.308359059551374,2.00464858611462,
5.35569927485942));
#56650=CARTESIAN_POINT('Ctrl Pts',(-0.302179881901054,1.98797993662176,
5.3567944351861));
#56651=CARTESIAN_POINT('Ctrl Pts',(-0.295929630339874,1.97111956159919,
5.35790219222578));
#56652=CARTESIAN_POINT('Ctrl Pts',(-0.288257459219722,1.95476626028155,
5.35900994926546));
#56653=CARTESIAN_POINT('Ctrl Pts',(-0.27927412115275,1.93916735132642,5.36011770630514));
#56654=CARTESIAN_POINT('Ctrl Pts',(-0.270397237075894,1.92375329193248,
5.36121233624707));
#56655=CARTESIAN_POINT('Ctrl Pts',(-0.260240559951294,1.90907648271744,
5.362306966189));
#56656=CARTESIAN_POINT('Ctrl Pts',(-0.248956461332729,1.89534942954957,
5.36340159613092));
#56657=CARTESIAN_POINT('Ctrl Pts',(-0.237469379779092,1.88137544859101,
5.36451591671948));
#56658=CARTESIAN_POINT('Ctrl Pts',(-0.224814399824077,1.8683864042059,5.36563023730803));
#56659=CARTESIAN_POINT('Ctrl Pts',(-0.211192980042452,1.85656889926349,
5.36674455789659));
#56660=CARTESIAN_POINT('Ctrl Pts',(-0.197571560260828,1.84475139432108,
5.36785887848515));
#56661=CARTESIAN_POINT('Ctrl Pts',(-0.182984409865951,1.83410587602989,
5.3689731990737));
#56662=CARTESIAN_POINT('Ctrl Pts',(-0.167664373286722,1.82477312348651,
5.37008751966226));
#56663=CARTESIAN_POINT('Ctrl Pts',(-0.152578900007102,1.8155832636327,5.37118477901779));
#56664=CARTESIAN_POINT('Ctrl Pts',(-0.136688361908179,1.80760858161357,
5.37228203837332));
#56665=CARTESIAN_POINT('Ctrl Pts',(-0.120213942326157,1.80098531190692,
5.37337929772885));
#56666=CARTESIAN_POINT('Ctrl Pts',(-0.103771037883913,1.7943747123444,5.37447445805553));
#56667=CARTESIAN_POINT('Ctrl Pts',(-0.0867471546266051,1.78911073852328,
5.37556961838221));
#56668=CARTESIAN_POINT('Ctrl Pts',(-0.0693869551783361,1.78528326057218,
5.37666477870889));
#56669=CARTESIAN_POINT('Ctrl Pts',(-0.0518270758797871,1.78141175834436,
5.37777253574857));
#56670=CARTESIAN_POINT('Ctrl Pts',(-0.0339238424814607,1.77901031969905,
5.37888029278825));
#56671=CARTESIAN_POINT('Ctrl Pts',(-0.0159451573288649,1.77811969991508,
5.37998804982793));
#56672=CARTESIAN_POINT('Ctrl Pts',(0.0018204775347214,1.77723963411773,
5.38108267976986));
#56673=CARTESIAN_POINT('Ctrl Pts',(0.0196589943490197,1.77783472807192,
5.38217730971178));
#56674=CARTESIAN_POINT('Ctrl Pts',(0.0373092328999541,1.77989189831337,
5.38327193965371));
#56675=CARTESIAN_POINT('Ctrl Pts',(0.0552769710888044,1.7819860737661,5.38438626024227));
#56676=CARTESIAN_POINT('Ctrl Pts',(0.0730487614792567,1.78559540306911,
5.38550058083083));
#56677=CARTESIAN_POINT('Ctrl Pts',(0.0903586518712053,1.79065150775053,
5.38661490141938));
#56678=CARTESIAN_POINT('Ctrl Pts',(0.107668542263155,1.79570761243196,5.38772922200794));
#56679=CARTESIAN_POINT('Ctrl Pts',(0.12451577272566,1.80221013825458,5.38884354259649));
#56680=CARTESIAN_POINT('Ctrl Pts',(0.140655930777141,1.81003951172234,5.38995786318505));
#56681=CARTESIAN_POINT('Ctrl Pts',(0.15654896874447,1.81774901056286,5.39105512254058));
#56682=CARTESIAN_POINT('Ctrl Pts',(0.171856059564678,1.82679322003641,5.39215238189611));
#56683=CARTESIAN_POINT('Ctrl Pts',(0.186342924313215,1.83705991141821,5.39324964125164));
#56684=CARTESIAN_POINT('Ctrl Pts',(0.200802076063112,1.84730696288418,5.39434480157832));
#56685=CARTESIAN_POINT('Ctrl Pts',(0.214443455109349,1.85877146458573,5.395439961905));
#56686=CARTESIAN_POINT('Ctrl Pts',(0.227059056739523,1.87129634813244,5.39653512223168));
#56687=CARTESIAN_POINT('Ctrl Pts',(0.239819765080723,1.88396529493596,5.39764287927136));
#56688=CARTESIAN_POINT('Ctrl Pts',(0.2515302814194,1.89771871199369,5.39875063631104));
#56689=CARTESIAN_POINT('Ctrl Pts',(0.262011317607084,1.91235340378573,5.39985839335072));
#56690=CARTESIAN_POINT('Ctrl Pts',(0.272368151842847,1.9268146721439,5.40095302329265));
#56691=CARTESIAN_POINT('Ctrl Pts',(0.281524097664492,1.94213575157908,5.40204765323458));
#56692=CARTESIAN_POINT('Ctrl Pts',(0.289348785140309,1.95808997159176,5.4031422831765));
#56693=CARTESIAN_POINT('Ctrl Pts',(0.297314226262783,1.97433118257415,5.40425660376506));
#56694=CARTESIAN_POINT('Ctrl Pts',(0.30389962881623,1.99122781729556,5.40537092435362));
#56695=CARTESIAN_POINT('Ctrl Pts',(0.309018521912682,2.00851924388211,5.40648524494217));
#56696=CARTESIAN_POINT('Ctrl Pts',(0.314137415009134,2.02581067046866,5.40759956553073));
#56697=CARTESIAN_POINT('Ctrl Pts',(0.317789685133248,2.04349605820179,5.40871388611929));
#56698=CARTESIAN_POINT('Ctrl Pts',(0.319943566928859,2.06130517339696,5.40982820670784));
#56699=CARTESIAN_POINT('Ctrl Pts',(0.322064470890616,2.07884161529912,5.41092546606337));
#56700=CARTESIAN_POINT('Ctrl Pts',(0.322745942476812,2.09660788533131,5.4120227254189));
#56701=CARTESIAN_POINT('Ctrl Pts',(0.321955526193629,2.11434624614258,5.41311998477443));
#56702=CARTESIAN_POINT('Ctrl Pts',(0.32116662195641,2.1320506739271,5.41421514510111));
#56703=CARTESIAN_POINT('Ctrl Pts',(0.318911388622714,2.14972653159111,5.41531030542779));
#56704=CARTESIAN_POINT('Ctrl Pts',(0.315209295398185,2.16711390109046,5.41640546575447));
#56705=CARTESIAN_POINT('Ctrl Pts',(0.311464620092556,2.18470126295445,5.41751322279415));
#56706=CARTESIAN_POINT('Ctrl Pts',(0.306239614873689,2.20199264792342,5.41862097983383));
#56707=CARTESIAN_POINT('Ctrl Pts',(0.299608078258493,2.21872731390566,5.41972873687351));
#56708=CARTESIAN_POINT('Ctrl Pts',(0.293055126410787,2.23526367142464,5.42082336681544));
#56709=CARTESIAN_POINT('Ctrl Pts',(0.285129167417892,2.25125573173565,5.42191799675736));
#56710=CARTESIAN_POINT('Ctrl Pts',(0.275950218294543,2.26647117662885,5.42301262669929));
#56711=CARTESIAN_POINT('Ctrl Pts',(0.266606154517656,2.28196032310577,5.42412694728785));
#56712=CARTESIAN_POINT('Ctrl Pts',(0.255963958912909,2.29664390115781,5.4252412678764));
#56713=CARTESIAN_POINT('Ctrl Pts',(0.244195967172233,2.31030811977149,5.42635558846496));
#56714=CARTESIAN_POINT('Ctrl Pts',(0.232427975431557,2.32397233838516,5.42746990905352));
#56715=CARTESIAN_POINT('Ctrl Pts',(0.219534824590082,2.33661665243179,5.42858422964207));
#56716=CARTESIAN_POINT('Ctrl Pts',(0.205726536806876,2.34806807065491,5.42969855023063));
#56717=CARTESIAN_POINT('Ctrl Pts',(0.192129666113152,2.35934415754447,5.43079580958616));
#56718=CARTESIAN_POINT('Ctrl Pts',(0.177560361058981,2.36953435404003,5.43189306894169));
#56719=CARTESIAN_POINT('Ctrl Pts',(0.162217763078438,2.37847185309619,5.43299032829722));
#56720=CARTESIAN_POINT('Ctrl Pts',(0.14690451509214,2.38739225494716,5.4340854886239));
#56721=CARTESIAN_POINT('Ctrl Pts',(0.130821538939885,2.39506427551764,5.43518064895058));
#56722=CARTESIAN_POINT('Ctrl Pts',(0.114197917399677,2.40136358653058,5.43627580927726));
#56723=CARTESIAN_POINT('Ctrl Pts',(0.0973830882486234,2.40773535324795,
5.43738356631694));
#56724=CARTESIAN_POINT('Ctrl Pts',(0.0800157924402915,2.41270221442863,
5.43849132335662));
#56725=CARTESIAN_POINT('Ctrl Pts',(0.0623552150644683,2.41618507678141,
5.4395990803963));
#56726=CARTESIAN_POINT('Ctrl Pts',(0.0449039183497231,2.41962666665933,
5.44069371033823));
#56727=CARTESIAN_POINT('Ctrl Pts',(0.027167042896384,2.42161916963324,5.44178834028015));
#56728=CARTESIAN_POINT('Ctrl Pts',(0.00940489339345394,2.42213774011323,
5.44288297022208));
#56729=CARTESIAN_POINT('Ctrl Pts',(-0.00867676884691561,2.42266563884899,
5.44399729081064));
#56730=CARTESIAN_POINT('Ctrl Pts',(-0.026783796946607,2.42166597635755,
5.4451116113992));
#56731=CARTESIAN_POINT('Ctrl Pts',(-0.0446431431697494,2.41916792663569,
5.44622593198775));
#56732=CARTESIAN_POINT('Ctrl Pts',(-0.0625024893928918,2.41666987691383,
5.44734025257631));
#56733=CARTESIAN_POINT('Ctrl Pts',(-0.0801133505468911,2.41267368050409,
5.44845457316486));
#56734=CARTESIAN_POINT('Ctrl Pts',(-0.0972165836964554,2.40726228450526,
5.44956889375342));
#56735=CARTESIAN_POINT('Ctrl Pts',(-0.114057951230964,2.40193374176166,
5.45066615310895));
#56736=CARTESIAN_POINT('Ctrl Pts',(-0.13051267897008,2.39519974670589,5.45176341246448));
#56737=CARTESIAN_POINT('Ctrl Pts',(-0.146332713706938,2.38713744535355,
5.45286067182001));
#56738=CARTESIAN_POINT('Ctrl Pts',(-0.162122485125355,2.37909056697576,
5.45395583214669));
#56739=CARTESIAN_POINT('Ctrl Pts',(-0.177279262975971,2.36972071603058,
5.45505099247337));
#56740=CARTESIAN_POINT('Ctrl Pts',(-0.191574503170435,2.3591532082765,5.45614615280005));
#56741=CARTESIAN_POINT('Ctrl Pts',(-0.206034169553102,2.34846415132176,
5.45725390983973));
#56742=CARTESIAN_POINT('Ctrl Pts',(-0.219611626390578,2.33655006975797,
5.45836166687941));
#56743=CARTESIAN_POINT('Ctrl Pts',(-0.232100069055215,2.32358607642151,
5.45946942391909));
#56744=CARTESIAN_POINT('Ctrl Pts',(-0.244440521680733,2.31077570847554,
5.46056405386101));
#56745=CARTESIAN_POINT('Ctrl Pts',(-0.255717145023625,2.29694080388856,
5.46165868380294));
#56746=CARTESIAN_POINT('Ctrl Pts',(-0.265768140835497,2.28228678213695,
5.46275331374487));
#56747=CARTESIAN_POINT('Ctrl Pts',(-0.275999938029845,2.26736915790842,
5.46386763433343));
#56748=CARTESIAN_POINT('Ctrl Pts',(-0.284961065392298,2.25160330911764,
5.46498195492198));
#56749=CARTESIAN_POINT('Ctrl Pts',(-0.292528247268615,2.23523461160129,
5.46609627551054));
#56750=CARTESIAN_POINT('Ctrl Pts',(-0.300095429144934,2.21886591408494,
5.46721059609909));
#56751=CARTESIAN_POINT('Ctrl Pts',(-0.306268433004919,2.20189517339176,
5.46832491668765));
#56752=CARTESIAN_POINT('Ctrl Pts',(-0.310976723501059,2.18458518230486,
5.46943923727621));
#56753=CARTESIAN_POINT('Ctrl Pts',(-0.316842100935001,2.16302117065645,
5.47082740795931));
#56754=CARTESIAN_POINT('Ctrl Pts',(-0.320466759043346,2.14082296958456,
5.47221557864242));
#56755=CARTESIAN_POINT('Ctrl Pts',(-0.321749112810183,2.11840337009517,
5.47360374932553));
#56756=CARTESIAN_POINT('Ctrl Pts',(-0.32209365089258,2.11237975475911,5.47397671790688));
#56757=CARTESIAN_POINT('Ctrl Pts',(-0.322269364165322,2.10634028175669,
5.47434968648822));
#56758=CARTESIAN_POINT('Ctrl Pts',(-0.322274866580731,2.10029324967485,
5.47472265506957));
#56759=CARTESIAN_POINT('',(-0.322274952656718,2.09975862400584,5.72487098172704));
#56760=CARTESIAN_POINT('Ctrl Pts',(-0.322274869645138,2.1002898623972,5.47466220412381));
#56761=CARTESIAN_POINT('Ctrl Pts',(-0.322295039416003,2.07786470363518,
5.47591876512393));
#56762=CARTESIAN_POINT('Ctrl Pts',(-0.319974701019861,2.05550143112443,
5.47719494582332));
#56763=CARTESIAN_POINT('Ctrl Pts',(-0.31511241078133,2.0324226576908,5.47862363347245));
#56764=CARTESIAN_POINT('Ctrl Pts',(-0.314866454738616,2.03128577841999,
5.47869428649189));
#56765=CARTESIAN_POINT('Ctrl Pts',(-0.314472000395494,2.02950909306706,
5.47880514099861));
#56766=CARTESIAN_POINT('Ctrl Pts',(-0.314327690013433,2.0288683595453,5.47884520864498));
#56767=CARTESIAN_POINT('Ctrl Pts',(-0.314081940527683,2.02779259177882,
5.47891263327804));
#56768=CARTESIAN_POINT('Ctrl Pts',(-0.3139815532966,2.02735731727185,5.47893995649529));
#56769=CARTESIAN_POINT('Ctrl Pts',(-0.313781840838838,2.02649952126034,
5.47899388589563));
#56770=CARTESIAN_POINT('Ctrl Pts',(-0.313682566348333,2.02607698882368,
5.47902049039843));
#56771=CARTESIAN_POINT('Ctrl Pts',(-0.313491653720592,2.02527173529575,
5.47907126952667));
#56772=CARTESIAN_POINT('Ctrl Pts',(-0.313400167479033,2.02488897870412,
5.47909543921964));
#56773=CARTESIAN_POINT('Ctrl Pts',(-0.313189697854583,2.02401550325668,
5.47915067215672));
#56774=CARTESIAN_POINT('Ctrl Pts',(-0.313070262025087,2.02352489543324,
5.47918174993945));
#56775=CARTESIAN_POINT('Ctrl Pts',(-0.312701435295801,2.02202520643533,
5.47927691768361));
#56776=CARTESIAN_POINT('Ctrl Pts',(-0.312448316870483,2.02101705683022,
5.47934112781115));
#56777=CARTESIAN_POINT('Ctrl Pts',(-0.310542503289915,2.01357890521393,
5.47981662985734));
#56778=CARTESIAN_POINT('Ctrl Pts',(-0.308696451843209,2.00720052787361,
5.48023415560076));
#56779=CARTESIAN_POINT('Ctrl Pts',(-0.306086022594601,1.99912411889603,
5.48077599848467));
#56780=CARTESIAN_POINT('Ctrl Pts',(-0.305502048030464,1.99736913210421,
5.48089454325521));
#56781=CARTESIAN_POINT('Ctrl Pts',(-0.300225244363447,1.98195523596384,
5.48194281753255));
#56782=CARTESIAN_POINT('Ctrl Pts',(-0.294634795383065,1.96862262230926,
5.48290000506907));
#56783=CARTESIAN_POINT('Ctrl Pts',(-0.285867025182904,1.95111186864262,
5.4842173697174));
#56784=CARTESIAN_POINT('Ctrl Pts',(-0.283454410104206,1.94656849169576,
5.48456486695539));
#56785=CARTESIAN_POINT('Ctrl Pts',(-0.278571130692444,1.93788104162778,
5.48523905315639));
#56786=CARTESIAN_POINT('Ctrl Pts',(-0.276114066707337,1.93373077887201,
5.48556560446138));
#56787=CARTESIAN_POINT('Ctrl Pts',(-0.267446515115443,1.9198126166023,5.48667350921797));
#56788=CARTESIAN_POINT('Ctrl Pts',(-0.260802985595397,1.9103240359307,5.48745106172768));
#56789=CARTESIAN_POINT('Ctrl Pts',(-0.251070460141749,1.89790481434811,
5.48848148880088));
#56790=CARTESIAN_POINT('Ctrl Pts',(-0.248413401897396,1.89464755786082,
5.48875298747842));
#56791=CARTESIAN_POINT('Ctrl Pts',(-0.244191156615343,1.88967348648262,
5.48916835237233));
#56792=CARTESIAN_POINT('Ctrl Pts',(-0.242669936333266,1.887920142379,5.48931491930548));
#56793=CARTESIAN_POINT('Ctrl Pts',(-0.240904976852216,1.88592972500554,
5.48948132529066));
#56794=CARTESIAN_POINT('Ctrl Pts',(-0.240679699471364,1.88567647638853,
5.48950249817451));
#56795=CARTESIAN_POINT('Ctrl Pts',(-0.240250549294356,1.88519557132406,
5.48954270425292));
#56796=CARTESIAN_POINT('Ctrl Pts',(-0.240046751602167,1.88496784877108,
5.48956174297938));
#56797=CARTESIAN_POINT('Ctrl Pts',(-0.239693804421044,1.88457459436594,
5.48959462040412));
#56798=CARTESIAN_POINT('Ctrl Pts',(-0.239544806859487,1.88440892695135,
5.48960847058834));
#56799=CARTESIAN_POINT('Ctrl Pts',(-0.239257355483712,1.88408998139295,
5.48963513462629));
#56800=CARTESIAN_POINT('Ctrl Pts',(-0.239118926426719,1.88393668216679,
5.4896479503082));
#56801=CARTESIAN_POINT('Ctrl Pts',(-0.238789843609458,1.88357295260691,
5.48967835755085));
#56802=CARTESIAN_POINT('Ctrl Pts',(-0.23859905854623,1.88336264053352,5.48969593913818));
#56803=CARTESIAN_POINT('Ctrl Pts',(-0.2380266477082,1.88273331637492,5.48974854956863));
#56804=CARTESIAN_POINT('Ctrl Pts',(-0.23764419177435,1.88231505573409,5.489783516024));
#56805=CARTESIAN_POINT('Ctrl Pts',(-0.233936589356397,1.87828177180005,
5.49012072819342));
#56806=CARTESIAN_POINT('Ctrl Pts',(-0.230530093007673,1.87474196312295,
5.49041692418063));
#56807=CARTESIAN_POINT('Ctrl Pts',(-0.213017856733913,1.85735797837242,
5.49188133070462));
#56808=CARTESIAN_POINT('Ctrl Pts',(-0.197739266187922,1.84475282556504,
5.49297726249604));
#56809=CARTESIAN_POINT('Ctrl Pts',(-0.174691618674529,1.82905739518009,
5.49453626283725));
#56810=CARTESIAN_POINT('Ctrl Pts',(-0.167812732251578,1.82474386706052,
5.49499075892837));
#56811=CARTESIAN_POINT('Ctrl Pts',(-0.152286048325084,1.81580613145408,
5.49600530570774));
#56812=CARTESIAN_POINT('Ctrl Pts',(-0.143575614649371,1.81130774670117,
5.49656723894533));
#56813=CARTESIAN_POINT('Ctrl Pts',(-0.129697927002537,1.80492437166496,
5.49746281379729));
#56814=CARTESIAN_POINT('Ctrl Pts',(-0.124664300869996,1.80276274522428,
5.49778766088663));
#56815=CARTESIAN_POINT('Ctrl Pts',(-0.11767006635181,1.79996807908464,5.49824027529802));
#56816=CARTESIAN_POINT('Ctrl Pts',(-0.115754676201834,1.79922391597172,
5.49836434768622));
#56817=CARTESIAN_POINT('Ctrl Pts',(-0.112467638040274,1.79798289139977,
5.49857754291374));
#56818=CARTESIAN_POINT('Ctrl Pts',(-0.111099477821311,1.79747692747115,
5.49866636074617));
#56819=CARTESIAN_POINT('Ctrl Pts',(-0.109307685550258,1.79682809285152,
5.49878279885299));
#56820=CARTESIAN_POINT('Ctrl Pts',(-0.108887109562394,1.7966767849762,5.49881013815319));
#56821=CARTESIAN_POINT('Ctrl Pts',(-0.108057329994095,1.79638020879685,
5.49886409489106));
#56822=CARTESIAN_POINT('Ctrl Pts',(-0.107648144806369,1.79623489158147,
5.49889071063728));
#56823=CARTESIAN_POINT('Ctrl Pts',(-0.106867596877025,1.79595946454169,
5.49894149830139));
#56824=CARTESIAN_POINT('Ctrl Pts',(-0.106496286811176,1.79582920692924,
5.49896566525841));
#56825=CARTESIAN_POINT('Ctrl Pts',(-0.105648294629428,1.79553346969367,
5.49902087388109));
#56826=CARTESIAN_POINT('Ctrl Pts',(-0.105171461435552,1.79536842919721,
5.49905193003896));
#56827=CARTESIAN_POINT('Ctrl Pts',(-0.103712842552697,1.79486740799666,
5.49914696738483));
#56828=CARTESIAN_POINT('Ctrl Pts',(-0.102729827265973,1.79453505117183,
5.49921106825836));
#56829=CARTESIAN_POINT('Ctrl Pts',(-0.0954821775133347,1.79212356725776,
5.49968407946031));
#56830=CARTESIAN_POINT('Ctrl Pts',(-0.0891569879735945,1.79023272417629,
5.50009915048292));
#56831=CARTESIAN_POINT('Ctrl Pts',(-0.0810052264134533,1.78806619968929,
5.50063751076568));
#56832=CARTESIAN_POINT('Ctrl Pts',(-0.0792279247514117,1.78761005424845,
5.50075508955459));
#56833=CARTESIAN_POINT('Ctrl Pts',(-0.0752122807052728,1.7866159100921,
5.50102120425307));
#56834=CARTESIAN_POINT('Ctrl Pts',(-0.0729718900094262,1.78608667146019,
5.50116999219249));
#56835=CARTESIAN_POINT('Ctrl Pts',(-0.0664200754710443,1.78461289036432,
5.50160601784391));
#56836=CARTESIAN_POINT('Ctrl Pts',(-0.0620947977488439,1.78373288378242,
5.50189501680985));
#56837=CARTESIAN_POINT('Ctrl Pts',(-0.0491804405426671,1.78138049933143,
5.50276091374107));
#56838=CARTESIAN_POINT('Ctrl Pts',(-0.0405485689226521,1.78016738635559,
5.50334370992194));
#56839=CARTESIAN_POINT('Ctrl Pts',(-0.00797611926683815,1.77692952782993,
5.50554898081245));
#56840=CARTESIAN_POINT('Ctrl Pts',(0.0161181246918636,1.77723307199857,
5.50719833123795));
#56841=CARTESIAN_POINT('Ctrl Pts',(0.042996590793723,1.78059139142204,5.50893232954168));
#56842=CARTESIAN_POINT('Ctrl Pts',(0.0460318940539969,1.78101468298175,
5.50912649934827));
#56843=CARTESIAN_POINT('Ctrl Pts',(0.0495659346278239,1.78155902441389,
5.50935028950308));
#56844=CARTESIAN_POINT('Ctrl Pts',(0.0500708568414377,1.78163802659319,
5.5093822087016));
#56845=CARTESIAN_POINT('Ctrl Pts',(0.0508394651533864,1.78176015995089,
5.5094307117353));
#56846=CARTESIAN_POINT('Ctrl Pts',(0.0511032861045851,1.78180241804483,
5.50944734483163));
#56847=CARTESIAN_POINT('Ctrl Pts',(0.0515614476923745,1.7818763895743,5.50947620351358));
#56848=CARTESIAN_POINT('Ctrl Pts',(0.0517558113507193,1.78190795295927,
5.50948843763293));
#56849=CARTESIAN_POINT('Ctrl Pts',(0.0521632878405286,1.78197450783408,
5.50951406824309));
#56850=CARTESIAN_POINT('Ctrl Pts',(0.0523763937597191,1.78200953529534,
5.50952746261199));
#56851=CARTESIAN_POINT('Ctrl Pts',(0.0529711104062391,1.78210790081363,
5.50956481441183));
#56852=CARTESIAN_POINT('Ctrl Pts',(0.0533526441683417,1.78217171204132,
5.5095887448618));
#56853=CARTESIAN_POINT('Ctrl Pts',(0.0548871891364662,1.7824312045983,5.50968486800382));
#56854=CARTESIAN_POINT('Ctrl Pts',(0.0560392645927981,1.78263247761223,
5.50975674678841));
#56855=CARTESIAN_POINT('Ctrl Pts',(0.0765077279115629,1.78632334783021,
5.51102909510853));
#56856=CARTESIAN_POINT('Ctrl Pts',(0.0954699152458125,1.7915648854506,5.51213467515926));
#56857=CARTESIAN_POINT('Ctrl Pts',(0.125460328708668,1.80288861042201,5.51392904866884));
#56858=CARTESIAN_POINT('Ctrl Pts',(0.136817650594346,1.80794453532368,5.51461996365921));
#56859=CARTESIAN_POINT('Ctrl Pts',(0.157552125344653,1.81865036391846,5.51594149064312));
#56860=CARTESIAN_POINT('Ctrl Pts',(0.16698835011805,1.82414650456605,5.5165683155795));
#56861=CARTESIAN_POINT('Ctrl Pts',(0.181939144824755,1.83390323392207,5.51762012449362));
#56862=CARTESIAN_POINT('Ctrl Pts',(0.18762678391317,1.83788262103993,5.51803515410984));
#56863=CARTESIAN_POINT('Ctrl Pts',(0.194048595074708,1.84269183340754,5.51852322293015));
#56864=CARTESIAN_POINT('Ctrl Pts',(0.194912659816613,1.8433457484398,5.5185893123363));
#56865=CARTESIAN_POINT('Ctrl Pts',(0.19609925589007,1.84425319993321,5.51868065715743));
#56866=CARTESIAN_POINT('Ctrl Pts',(0.196424632452732,1.84450301827929,5.51870576598485));
#56867=CARTESIAN_POINT('Ctrl Pts',(0.19707381415707,1.84500342151033,5.51875598522046));
#56868=CARTESIAN_POINT('Ctrl Pts',(0.197397620497288,1.84525400358905,5.51878109548911));
#56869=CARTESIAN_POINT('Ctrl Pts',(0.198037357830995,1.84575102542282,5.518830827297));
#56870=CARTESIAN_POINT('Ctrl Pts',(0.19835330854856,1.84599743868267,5.51885544775638));
#56871=CARTESIAN_POINT('Ctrl Pts',(0.199048614515774,1.84654180350524,5.51890976041343));
#56872=CARTESIAN_POINT('Ctrl Pts',(0.199427761483535,1.84684001845344,5.51893946307942));
#56873=CARTESIAN_POINT('Ctrl Pts',(0.200749692709195,1.84788458518436,5.51904332708928));
#56874=CARTESIAN_POINT('Ctrl Pts',(0.201688959393291,1.84863535430274,5.51911766507012));
#56875=CARTESIAN_POINT('Ctrl Pts',(0.211554417011902,1.85661184850422,5.51990423461445));
#56876=CARTESIAN_POINT('Ctrl Pts',(0.22009146974321,1.86430368066689,5.52063546820119));
#56877=CARTESIAN_POINT('Ctrl Pts',(0.232070027442631,1.87631555881756,5.52174109823591));
#56878=CARTESIAN_POINT('Ctrl Pts',(0.235841094106152,1.88029519713349,5.52210202317852));
#56879=CARTESIAN_POINT('Ctrl Pts',(0.252357779804051,1.89864083490154,5.52374070465222));
#56880=CARTESIAN_POINT('Ctrl Pts',(0.263905081720795,1.91403228004728,5.52505158731254));
#56881=CARTESIAN_POINT('Ctrl Pts',(0.277753991620937,1.93640167190296,5.52681986889858));
#56882=CARTESIAN_POINT('Ctrl Pts',(0.281294573733258,1.94256726513338,5.52729395957921));
#56883=CARTESIAN_POINT('Ctrl Pts',(0.287948678308964,1.95509712106857,5.52822484751959));
#56884=CARTESIAN_POINT('Ctrl Pts',(0.291062250707027,1.96145733498274,5.5286814642977));
#56885=CARTESIAN_POINT('Ctrl Pts',(0.294260508014744,1.96857529804747,5.52917116638926));
#56886=CARTESIAN_POINT('Ctrl Pts',(0.294554754441885,1.96923610773584,5.52921642971607));
#56887=CARTESIAN_POINT('Ctrl Pts',(0.294972547887366,1.97018294149415,5.52928099442377));
#56888=CARTESIAN_POINT('Ctrl Pts',(0.29509790618423,1.97046815660263,5.52930040568847));
#56889=CARTESIAN_POINT('Ctrl Pts',(0.295312642258065,1.97095865361975,5.52933372296816));
#56890=CARTESIAN_POINT('Ctrl Pts',(0.295402219895857,1.97116384733002,5.52934764130235));
#56891=CARTESIAN_POINT('Ctrl Pts',(0.2955734775248,1.97155726136999,5.52937428897157));
#56892=CARTESIAN_POINT('Ctrl Pts',(0.295655191478141,1.97174546606261,5.52938702041693));
#56893=CARTESIAN_POINT('Ctrl Pts',(0.295847450587662,1.97218944001578,5.52941701526175));
#56894=CARTESIAN_POINT('Ctrl Pts',(0.295957844097497,1.97244527534732,5.52943426932124));
#56895=CARTESIAN_POINT('Ctrl Pts',(0.296283518378198,1.97320271959478,5.52948526465528));
#56896=CARTESIAN_POINT('Ctrl Pts',(0.296497858076163,1.97370473584789,5.52951894876024));
#56897=CARTESIAN_POINT('Ctrl Pts',(0.298387981115609,1.97816302432943,5.52981709633304));
#56898=CARTESIAN_POINT('Ctrl Pts',(0.299985865234027,1.9821521279428,5.53007693996119));
#56899=CARTESIAN_POINT('Ctrl Pts',(0.301532487609039,1.98624877479189,5.53033794780547));
#56900=CARTESIAN_POINT('Ctrl Pts',(0.301561358511304,1.98632533539577,5.53034282361473));
#56901=CARTESIAN_POINT('Ctrl Pts',(0.301945366214564,1.98734483279348,5.53040772358156));
#56902=CARTESIAN_POINT('Ctrl Pts',(0.302296112262658,1.98828943006488,5.5304675440082));
#56903=CARTESIAN_POINT('Ctrl Pts',(0.302743891859443,1.98951290246778,5.53054464211683));
#56904=CARTESIAN_POINT('Ctrl Pts',(0.302844976545546,1.98979027737278,5.53056209572466));
#56905=CARTESIAN_POINT('Ctrl Pts',(0.303592262984062,1.99184961195699,5.53069149214904));
#56906=CARTESIAN_POINT('Ctrl Pts',(0.304223125769417,1.99363713709346,5.53080277885917));
#56907=CARTESIAN_POINT('Ctrl Pts',(0.30637900156563,1.99992186768926,5.53119078535168));
#56908=CARTESIAN_POINT('Ctrl Pts',(0.307820405502191,2.00444725779309,5.53146435081629));
#56909=CARTESIAN_POINT('Ctrl Pts',(0.313773653113842,2.02467335495098,5.53266793579159));
#56910=CARTESIAN_POINT('Ctrl Pts',(0.317188058125169,2.04067221641019,5.53357049460153));
#56911=CARTESIAN_POINT('Ctrl Pts',(0.321054278317949,2.06929567536191,5.53519182435985));
#56912=CARTESIAN_POINT('Ctrl Pts',(0.322006106270631,2.08181656449784,5.53590303811867));
#56913=CARTESIAN_POINT('Ctrl Pts',(0.322338286338671,2.10079584545927,5.53700936454063));
#56914=CARTESIAN_POINT('Ctrl Pts',(0.322258096219163,2.10723294464565,5.53738938925162));
#56915=CARTESIAN_POINT('Ctrl Pts',(0.321835752299973,2.11718597211689,5.5379867600805));
#56916=CARTESIAN_POINT('Ctrl Pts',(0.321628457296497,2.12070611132324,5.53819992446199));
#56917=CARTESIAN_POINT('Ctrl Pts',(0.321303752563177,2.12501409880645,5.53846333773981));
#56918=CARTESIAN_POINT('Ctrl Pts',(0.321241125094297,2.12580593111411,5.53851185972658));
#56919=CARTESIAN_POINT('Ctrl Pts',(0.321144266226192,2.12697554032314,5.53858368915228));
#56920=CARTESIAN_POINT('Ctrl Pts',(0.321112293814993,2.12735350552724,5.53860692558892));
#56921=CARTESIAN_POINT('Ctrl Pts',(0.321049057875516,2.12808566346722,5.53865198459456));
#56922=CARTESIAN_POINT('Ctrl Pts',(0.321017875294259,2.12843986278171,5.53867380458778));
#56923=CARTESIAN_POINT('Ctrl Pts',(0.32095251725464,2.12916845264115,5.53871873316167));
#56924=CARTESIAN_POINT('Ctrl Pts',(0.320918272742553,2.12954283635068,5.53874184388517));
#56925=CARTESIAN_POINT('Ctrl Pts',(0.320834363764139,2.13044282143607,5.53879745885791));
#56926=CARTESIAN_POINT('Ctrl Pts',(0.320784062814432,2.13096836107868,5.53882998309175));
#56927=CARTESIAN_POINT('Ctrl Pts',(0.320626066032162,2.13257739977866,5.53892971137704));
#56928=CARTESIAN_POINT('Ctrl Pts',(0.320514171124259,2.13366047024979,5.53899704745965));
#56929=CARTESIAN_POINT('Ctrl Pts',(0.319126221929996,2.14646003292185,5.53979530860743));
#56930=CARTESIAN_POINT('Ctrl Pts',(0.317214025059591,2.15809719954957,5.54054630763282));
#56931=CARTESIAN_POINT('Ctrl Pts',(0.314392653969702,2.17085247937803,5.54139873219072));
#56932=CARTESIAN_POINT('Ctrl Pts',(0.314108708655933,2.17210085842848,5.54148246953287));
#56933=CARTESIAN_POINT('Ctrl Pts',(0.307715381607373,2.19945471301917,5.54332400606755));
#56934=CARTESIAN_POINT('Ctrl Pts',(0.298379292015336,2.22469767921069,5.54517058108146));
#56935=CARTESIAN_POINT('Ctrl Pts',(0.281603260167049,2.25701283143421,5.54759307076845));
#56936=CARTESIAN_POINT('Ctrl Pts',(0.276798542339603,2.2653361160755,5.54822150001533));
#56937=CARTESIAN_POINT('Ctrl Pts',(0.270875548856404,2.27461263169682,5.54891693542782));
#56938=CARTESIAN_POINT('Ctrl Pts',(0.270114733885519,2.27578727150623,5.54900489812689));
#56939=CARTESIAN_POINT('Ctrl Pts',(0.269120787197656,2.27730015838857,5.54911802608913));
#56940=CARTESIAN_POINT('Ctrl Pts',(0.268894642009926,2.27764294460887,5.54914364736011));
#56941=CARTESIAN_POINT('Ctrl Pts',(0.268532393220227,2.27818975718383,5.5491844996308));
#56942=CARTESIAN_POINT('Ctrl Pts',(0.268396711813417,2.27839406061448,5.54919975890493));
#56943=CARTESIAN_POINT('Ctrl Pts',(0.268139306283006,2.27878069278044,5.5492286279143));
#56944=CARTESIAN_POINT('Ctrl Pts',(0.268017630345328,2.27896305068184,5.54924224066575));
#56945=CARTESIAN_POINT('Ctrl Pts',(0.267739131897342,2.27937952022521,5.54927332164872));
#56946=CARTESIAN_POINT('Ctrl Pts',(0.267582188607598,2.27961355006454,5.54929078155951));
#56947=CARTESIAN_POINT('Ctrl Pts',(0.267099895655398,2.28033069794003,5.54934426834693));
#56948=CARTESIAN_POINT('Ctrl Pts',(0.266773540765566,2.28081314343429,5.54938022756913));
#56949=CARTESIAN_POINT('Ctrl Pts',(0.264338631138373,2.28439169045772,5.54964680676294));
#56950=CARTESIAN_POINT('Ctrl Pts',(0.2621774385234,2.28745186342891,5.54987394035509));
#56951=CARTESIAN_POINT('Ctrl Pts',(0.259261333730675,2.29143183373422,5.55016923247058));
#56952=CARTESIAN_POINT('Ctrl Pts',(0.258554098592807,2.29238597744342,5.55024001611934));
#56953=CARTESIAN_POINT('Ctrl Pts',(0.257006213827043,2.29445030409225,5.55039319247933));
#56954=CARTESIAN_POINT('Ctrl Pts',(0.256163607684727,2.29555899602032,5.5504754803148));
#56955=CARTESIAN_POINT('Ctrl Pts',(0.254379999302698,2.29787453945384,5.55064746651978));
#56956=CARTESIAN_POINT('Ctrl Pts',(0.253437532002508,2.2990802223354,5.55073709053411));
#56957=CARTESIAN_POINT('Ctrl Pts',(0.250009880001951,2.30340137003331,5.55105874574034));
#56958=CARTESIAN_POINT('Ctrl Pts',(0.247475480406074,2.30647747109506,5.5512885654422));
#56959=CARTESIAN_POINT('Ctrl Pts',(0.228932302030499,2.32815198966563,5.55292027719812));
#56960=CARTESIAN_POINT('Ctrl Pts',(0.210902487277469,2.34491542995423,5.55425524586823));
#56961=CARTESIAN_POINT('Ctrl Pts',(0.180767606197172,2.36711486715365,5.55639719107328));
#56962=CARTESIAN_POINT('Ctrl Pts',(0.169943035446717,2.37412877452456,5.55715056787063));
#56963=CARTESIAN_POINT('Ctrl Pts',(0.157463177791235,2.38119145992263,5.55801681056844));
#56964=CARTESIAN_POINT('Ctrl Pts',(0.156193023137833,2.381898969331,5.5581049390324));
#56965=CARTESIAN_POINT('Ctrl Pts',(0.153949719159728,2.38312873268272,5.55826054958932));
#56966=CARTESIAN_POINT('Ctrl Pts',(0.152978585097126,2.38365462759139,5.55832790118789));
#56967=CARTESIAN_POINT('Ctrl Pts',(0.151550044107019,2.38441875061441,5.55842696405328));
#56968=CARTESIAN_POINT('Ctrl Pts',(0.151094730660062,2.38466089287393,5.55845853626862));
#56969=CARTESIAN_POINT('Ctrl Pts',(0.150288265126148,2.38508730286089,5.55851445575335));
#56970=CARTESIAN_POINT('Ctrl Pts',(0.149937349604948,2.3852720176924,5.55853878713094));
#56971=CARTESIAN_POINT('Ctrl Pts',(0.149255803872446,2.38562916462576,5.55858604231771));
#56972=CARTESIAN_POINT('Ctrl Pts',(0.148925213398252,2.38580167159569,5.55860896343416));
#56973=CARTESIAN_POINT('Ctrl Pts',(0.14813599489041,2.38621175626834,5.55866368224964));
#56974=CARTESIAN_POINT('Ctrl Pts',(0.147677094712553,2.38644880537485,5.5586954985269));
#56975=CARTESIAN_POINT('Ctrl Pts',(0.146037041604601,2.38729100130721,5.55880920529237));
#56976=CARTESIAN_POINT('Ctrl Pts',(0.144852735260972,2.387889947646,5.55889131335468));
#56977=CARTESIAN_POINT('Ctrl Pts',(0.123358872762979,2.39859396291889,5.56038157408449));
#56978=CARTESIAN_POINT('Ctrl Pts',(0.102046377603564,2.40653208142139,5.56186769253266));
#56979=CARTESIAN_POINT('Ctrl Pts',(0.0658924549141328,2.41580680735454,
5.56437939030894));
#56980=CARTESIAN_POINT('Ctrl Pts',(0.051471858556127,2.41847511877644,5.56537709262186));
#56981=CARTESIAN_POINT('Ctrl Pts',(0.0252655019948851,2.42149721532713,
5.5671444763503));
#56982=CARTESIAN_POINT('Ctrl Pts',(0.0135450624519604,2.42220397259656,
5.56791842020518));
#56983=CARTESIAN_POINT('Ctrl Pts',(0.000221912068356351,2.42227884137083,
5.56876152563732));
#56984=CARTESIAN_POINT('Ctrl Pts',(-0.00136723884647932,2.42227601794867,
5.56886149261588));
#56985=CARTESIAN_POINT('Ctrl Pts',(-0.00337230365008466,2.42225762400849,
5.56898681551018));
#56986=CARTESIAN_POINT('Ctrl Pts',(-0.00378826013363588,2.42225300270642,
5.56901277025045));
#56987=CARTESIAN_POINT('Ctrl Pts',(-0.00445063106545653,2.42224436107115,
5.56905402959807));
#56988=CARTESIAN_POINT('Ctrl Pts',(-0.00469705007615137,2.42224086345557,
5.56906936346601));
#56989=CARTESIAN_POINT('Ctrl Pts',(-0.00516243649555589,2.42223372392391,
5.56909829307104));
#56990=CARTESIAN_POINT('Ctrl Pts',(-0.00538140240343053,2.42223014150282,
5.5691118920063));
#56991=CARTESIAN_POINT('Ctrl Pts',(-0.00588007284775842,2.42222147449788,
5.56914283369319));
#56992=CARTESIAN_POINT('Ctrl Pts',(-0.00615977402736211,2.42221624892242,
5.5691601683964));
#56993=CARTESIAN_POINT('Ctrl Pts',(-0.00701159420103367,2.42219922506018,
5.56921289976747));
#56994=CARTESIAN_POINT('Ctrl Pts',(-0.00758369280629195,2.42218626708462,
5.56924823153866));
#56995=CARTESIAN_POINT('Ctrl Pts',(-0.0116853252403361,2.42208243451034,
5.56950096066145));
#56996=CARTESIAN_POINT('Ctrl Pts',(-0.0152133617157631,2.42193508283617,
5.56971526595571));
#56997=CARTESIAN_POINT('Ctrl Pts',(-0.0510842193015345,2.41984586426108,
5.57186925757705));
#56998=CARTESIAN_POINT('Ctrl Pts',(-0.0829654846381817,2.41309486697978,
5.57359321169757));
#56999=CARTESIAN_POINT('Ctrl Pts',(-0.127066442583779,2.39653213187297,
5.57628469362726));
#57000=CARTESIAN_POINT('Ctrl Pts',(-0.140454032552032,2.39043030645595,
5.57714452415153));
#57001=CARTESIAN_POINT('Ctrl Pts',(-0.15443994632272,2.38286204756227,5.57811115292283));
#57002=CARTESIAN_POINT('Ctrl Pts',(-0.155499145147346,2.38228115553036,
5.57818479329279));
#57003=CARTESIAN_POINT('Ctrl Pts',(-0.15702440872034,2.38143347178752,5.57829147529698));
#57004=CARTESIAN_POINT('Ctrl Pts',(-0.157493120678105,2.3811714439802,5.57832434619832));
#57005=CARTESIAN_POINT('Ctrl Pts',(-0.158308361753162,2.3807130151585,5.57838167302838));
#57006=CARTESIAN_POINT('Ctrl Pts',(-0.158655186683821,2.38051714032545,
5.57840611000084));
#57007=CARTESIAN_POINT('Ctrl Pts',(-0.15932347086983,2.38013808050322,5.57845329100383));
#57008=CARTESIAN_POINT('Ctrl Pts',(-0.159644979734389,2.37995498381324,
5.57847603182433));
#57009=CARTESIAN_POINT('Ctrl Pts',(-0.160404918846401,2.37952046985351,
5.57852988387269));
#57010=CARTESIAN_POINT('Ctrl Pts',(-0.160843073409277,2.37926857465325,
5.57856101233922));
#57011=CARTESIAN_POINT('Ctrl Pts',(-0.162372849968561,2.37838431124759,
5.57866997327037));
#57012=CARTESIAN_POINT('Ctrl Pts',(-0.163461339086637,2.37774657100877,
5.57874800025504));
#57013=CARTESIAN_POINT('Ctrl Pts',(-0.178340752657707,2.36891103558384,
5.5798215333238));
#57014=CARTESIAN_POINT('Ctrl Pts',(-0.191502307695084,2.35970231571622,
5.58085476216332));
#57015=CARTESIAN_POINT('Ctrl Pts',(-0.2103070685247,2.34433604229763,5.58246300907199));
#57016=CARTESIAN_POINT('Ctrl Pts',(-0.21648912836491,2.3388757217534,5.58301579169205));
#57017=CARTESIAN_POINT('Ctrl Pts',(-0.233515297686581,2.3226330013751,5.58460288321765));
#57018=CARTESIAN_POINT('Ctrl Pts',(-0.243811198661628,2.31130774121618,
5.58564413352071));
#57019=CARTESIAN_POINT('Ctrl Pts',(-0.259296612193892,2.29162878138581,
5.58731113280887));
#57020=CARTESIAN_POINT('Ctrl Pts',(-0.264978226450914,2.28369241399321,
5.58794973818881));
#57021=CARTESIAN_POINT('Ctrl Pts',(-0.271071994922174,2.27430778224615,
5.58865684087102));
#57022=CARTESIAN_POINT('Ctrl Pts',(-0.271844443778486,2.27310062955182,
5.58874691699477));
#57023=CARTESIAN_POINT('Ctrl Pts',(-0.272822787754532,2.27154901056902,
5.58886153546993));
#57024=CARTESIAN_POINT('Ctrl Pts',(-0.273036111798481,2.27120928188474,
5.58888656052523));
#57025=CARTESIAN_POINT('Ctrl Pts',(-0.273377704766443,2.27066301670217,
5.5889266847581));
#57026=CARTESIAN_POINT('Ctrl Pts',(-0.273506374407568,2.27045673319825,
5.58894181048111));
#57027=CARTESIAN_POINT('Ctrl Pts',(-0.273750877682042,2.27006375529491,
5.58897057541734));
#57028=CARTESIAN_POINT('Ctrl Pts',(-0.273866752865476,2.26987708960266,
5.58898421731618));
#57029=CARTESIAN_POINT('Ctrl Pts',(-0.274130370536744,2.2694514517753,5.58901527496823));
#57030=CARTESIAN_POINT('Ctrl Pts',(-0.274277991268687,2.26921240517888,
5.58903268258323));
#57031=CARTESIAN_POINT('Ctrl Pts',(-0.274736576057089,2.26846762852597,
5.58908681017239));
#57032=CARTESIAN_POINT('Ctrl Pts',(-0.275046457640657,2.26796122837524,
5.58912345895247));
#57033=CARTESIAN_POINT('Ctrl Pts',(-0.277432197536317,2.26403820840733,
5.58940620301845));
#57034=CARTESIAN_POINT('Ctrl Pts',(-0.279445831974639,2.26058389893638,
5.58964832050689));
#57035=CARTESIAN_POINT('Ctrl Pts',(-0.281631774391969,2.25666829822584,
5.58991620644255));
#57036=CARTESIAN_POINT('Ctrl Pts',(-0.281867813153797,2.25624323322828,
5.58994520163774));
#57037=CARTESIAN_POINT('Ctrl Pts',(-0.282171692339081,2.25569306958657,
5.58998262181291));
#57038=CARTESIAN_POINT('Ctrl Pts',(-0.282240411817415,2.25556846020985,
5.58999109012269));
#57039=CARTESIAN_POINT('Ctrl Pts',(-0.288542184469433,2.24412350464023,
5.59076822119098));
#57040=CARTESIAN_POINT('Ctrl Pts',(-0.294089414241081,2.23243737516183,
5.59150318956021));
#57041=CARTESIAN_POINT('Ctrl Pts',(-0.310538650271962,2.19161492203197,
5.59397735034514));
#57042=CARTESIAN_POINT('Ctrl Pts',(-0.317923142611618,2.16125577184274,
5.59568122426102));
#57043=CARTESIAN_POINT('Ctrl Pts',(-0.321103356018776,2.12759105351112,
5.59771772940258));
#57044=CARTESIAN_POINT('Ctrl Pts',(-0.321325593972288,2.1248695281943,5.59788322444787));
#57045=CARTESIAN_POINT('Ctrl Pts',(-0.321563749271872,2.12141194838804,
5.59809467219416));
#57046=CARTESIAN_POINT('Ctrl Pts',(-0.321611769132162,2.12067816048703,
5.59813961491862));
#57047=CARTESIAN_POINT('Ctrl Pts',(-0.321684520013776,2.11950484555407,
5.59821158855182));
#57048=CARTESIAN_POINT('Ctrl Pts',(-0.321710862805945,2.11906541807021,
5.59823856883306));
#57049=CARTESIAN_POINT('Ctrl Pts',(-0.321758978611058,2.11823428677734,
5.59828964676918));
#57050=CARTESIAN_POINT('Ctrl Pts',(-0.321780936916443,2.11784259415342,
5.59831373856303));
#57051=CARTESIAN_POINT('Ctrl Pts',(-0.321828934879923,2.11695748901073,
5.59836822415722));
#57052=CARTESIAN_POINT('Ctrl Pts',(-0.3218545550857,2.116464055568,5.59839863105959));
#57053=CARTESIAN_POINT('Ctrl Pts',(-0.321917255910508,2.11520035084856,
5.5984765872401));
#57054=CARTESIAN_POINT('Ctrl Pts',(-0.321952706550846,2.1144300050905,5.59852418752623));
#57055=CARTESIAN_POINT('Ctrl Pts',(-0.32214014786984,2.11001160262876,5.59879766296652));
#57056=CARTESIAN_POINT('Ctrl Pts',(-0.322232893435412,2.10636142117186,
5.59902538734719));
#57057=CARTESIAN_POINT('Ctrl Pts',(-0.322268819383934,2.1020901311049,5.59929408196456));
#57058=CARTESIAN_POINT('Ctrl Pts',(-0.322272246117975,2.10146968315857,
5.59933316725188));
#57059=CARTESIAN_POINT('Ctrl Pts',(-0.322274729611917,2.10052722618315,
5.5993926211616));
#57060=CARTESIAN_POINT('Ctrl Pts',(-0.322275095528039,2.10020521956859,
5.59941294943006));
#57061=CARTESIAN_POINT('Ctrl Pts',(-0.322271684120159,2.09079133210786,
5.6000076823408));
#57062=CARTESIAN_POINT('Ctrl Pts',(-0.321883651494965,2.08170444921664,
5.60059378601718));
#57063=CARTESIAN_POINT('Ctrl Pts',(-0.318099653150887,2.03728234170793,
5.60351711798254));
#57064=CARTESIAN_POINT('Ctrl Pts',(-0.309267229173563,2.00266449487461,
5.60600990815023));
#57065=CARTESIAN_POINT('Ctrl Pts',(-0.294100133651789,1.96820096658294,
5.60840486522824));
#57066=CARTESIAN_POINT('Ctrl Pts',(-0.293207011460761,1.9662258512745,5.60854167595591));
#57067=CARTESIAN_POINT('Ctrl Pts',(-0.292108909905293,1.96386127116063,
5.60870479395439));
#57068=CARTESIAN_POINT('Ctrl Pts',(-0.291923002579937,1.96346308445623,
5.60873223942929));
#57069=CARTESIAN_POINT('Ctrl Pts',(-0.291618151489236,1.96281360621666,
5.60877696635384));
#57070=CARTESIAN_POINT('Ctrl Pts',(-0.291499696754035,1.96256208779605,
5.60879427780816));
#57071=CARTESIAN_POINT('Ctrl Pts',(-0.29128743039153,1.96211288530184,5.60882517783779));
#57072=CARTESIAN_POINT('Ctrl Pts',(-0.291193743007796,1.96191514370491,
5.60883877409607));
#57073=CARTESIAN_POINT('Ctrl Pts',(-0.290993653015017,1.96149393230199,
5.60886772248641));
#57074=CARTESIAN_POINT('Ctrl Pts',(-0.290887194655796,1.96127049026808,
5.60888307103652));
#57075=CARTESIAN_POINT('Ctrl Pts',(-0.290599072890201,1.96066755051505,
5.60892446722927));
#57076=CARTESIAN_POINT('Ctrl Pts',(-0.290416922765928,1.96028828388406,
5.60895048458479));
#57077=CARTESIAN_POINT('Ctrl Pts',(-0.289520027814286,1.95843013362637,
5.60907784905689));
#57078=CARTESIAN_POINT('Ctrl Pts',(-0.288794710214921,1.95695633816627,
5.60917854804987));
#57079=CARTESIAN_POINT('Ctrl Pts',(-0.284575686806505,1.9485464828899,5.60975168573835));
#57080=CARTESIAN_POINT('Ctrl Pts',(-0.280843136534661,1.94173236770354,
5.61021030464034));
#57081=CARTESIAN_POINT('Ctrl Pts',(-0.268909142489587,1.92170010365539,
5.61156089960037));
#57082=CARTESIAN_POINT('Ctrl Pts',(-0.259993622897372,1.90893362416738,
5.61242554942837));
#57083=CARTESIAN_POINT('Ctrl Pts',(-0.240018087235018,1.88433140560677,
5.61419730733332));
#57084=CARTESIAN_POINT('Ctrl Pts',(-0.228919360810158,1.87258519057617,
5.61510269000134));
#57085=CARTESIAN_POINT('Ctrl Pts',(-0.209729049058428,1.85510961442861,
5.61661280011476));
#57086=CARTESIAN_POINT('Ctrl Pts',(-0.202172048187132,1.8488346990185,5.61719528319366));
#57087=CARTESIAN_POINT('Ctrl Pts',(-0.193510220840325,1.8422868753659,5.61785554221577));
#57088=CARTESIAN_POINT('Ctrl Pts',(-0.192676429016835,1.84166290657392,
5.61791902393836));
#57089=CARTESIAN_POINT('Ctrl Pts',(-0.191424867564646,1.84073572913391,
5.61801420721487));
#57090=CARTESIAN_POINT('Ctrl Pts',(-0.191009364358687,1.84042946085453,
5.61804578957989));
#57091=CARTESIAN_POINT('Ctrl Pts',(-0.190292505518085,1.83990371599445,
5.61810024897742));
#57092=CARTESIAN_POINT('Ctrl Pts',(-0.189991500655529,1.83968376100095,
5.61812310739805));
#57093=CARTESIAN_POINT('Ctrl Pts',(-0.189369485804514,1.83923088608776,
5.61817032571903));
#57094=CARTESIAN_POINT('Ctrl Pts',(-0.189048426260731,1.83899803554266,
5.61819468825139));
#57095=CARTESIAN_POINT('Ctrl Pts',(-0.188300119670472,1.83845742638522,
5.6182514488994));
#57096=CARTESIAN_POINT('Ctrl Pts',(-0.187872547495064,1.8381501216853,5.61828386444611));
#57097=CARTESIAN_POINT('Ctrl Pts',(-0.186507523867209,1.83717411629757,
5.61838729925704));
#57098=CARTESIAN_POINT('Ctrl Pts',(-0.185567248635086,1.83650939716588,
5.61845847117841));
#57099=CARTESIAN_POINT('Ctrl Pts',(-0.165216861119755,1.8222858316003,5.61999726991051));
#57100=CARTESIAN_POINT('Ctrl Pts',(-0.14437894263507,1.81090476902241,5.62155045089508));
#57101=CARTESIAN_POINT('Ctrl Pts',(-0.100697226864652,1.79295566204286,
5.62473192888082));
#57102=CARTESIAN_POINT('Ctrl Pts',(-0.0779901020985928,1.78641775892956,
5.62634890546494));
#57103=CARTESIAN_POINT('Ctrl Pts',(-0.0513527190731283,1.78182376753071,
5.62808492019714));
#57104=CARTESIAN_POINT('Ctrl Pts',(-0.0479237049567799,1.78128925718876,
5.6283052979047));
#57105=CARTESIAN_POINT('Ctrl Pts',(-0.0439228096747885,1.78073163889518,
5.62855831144904));
#57106=CARTESIAN_POINT('Ctrl Pts',(-0.0433588476256891,1.78065456014429,
5.62859388099007));
#57107=CARTESIAN_POINT('Ctrl Pts',(-0.0425180110532875,1.78054190841317,
5.62864676870856));
#57108=CARTESIAN_POINT('Ctrl Pts',(-0.0422412935829531,1.78050520088414,
5.62866415062883));
#57109=CARTESIAN_POINT('Ctrl Pts',(-0.0417474617536401,1.78044034517424,
5.62869512850483));
#57110=CARTESIAN_POINT('Ctrl Pts',(-0.0415303665944644,1.78041205872747,
5.62870873229801));
#57111=CARTESIAN_POINT('Ctrl Pts',(-0.0410684664279713,1.78035235398053,
5.62873764531517));
#57112=CARTESIAN_POINT('Ctrl Pts',(-0.04082365481761,1.78032099576474,5.62875295106238));
#57113=CARTESIAN_POINT('Ctrl Pts',(-0.0401645054337035,1.78023733404486,
5.62879411238003));
#57114=CARTESIAN_POINT('Ctrl Pts',(-0.0397500998336552,1.78018555441733,
5.62881993825236));
#57115=CARTESIAN_POINT('Ctrl Pts',(-0.0377402231692326,1.77993838894242,
5.62894494661227));
#57116=CARTESIAN_POINT('Ctrl Pts',(-0.036143370007888,1.77975413137111,
5.62904350954445));
#57117=CARTESIAN_POINT('Ctrl Pts',(-0.0226233437624814,1.77829650008731,
5.62987211979563));
#57118=CARTESIAN_POINT('Ctrl Pts',(-0.0106375794744982,1.77767738433408,
5.63056812075044));
#57119=CARTESIAN_POINT('Ctrl Pts',(0.0292505477647775,1.77784523171065,
5.63283706223557));
#57120=CARTESIAN_POINT('Ctrl Pts',(0.0570108113776403,1.78158341673356,
5.63434997488827));
#57121=CARTESIAN_POINT('Ctrl Pts',(0.0930871735592631,1.79131627596256,
5.63652722643062));
#57122=CARTESIAN_POINT('Ctrl Pts',(0.102116670787986,1.79418465984062,5.63708963085385));
#57123=CARTESIAN_POINT('Ctrl Pts',(0.112082515384229,1.79784110172805,5.63773517514946));
#57124=CARTESIAN_POINT('Ctrl Pts',(0.113156719533934,1.79824174107257,5.63780508413283));
#57125=CARTESIAN_POINT('Ctrl Pts',(0.114714921317338,1.79883238425544,5.63790697524715));
#57126=CARTESIAN_POINT('Ctrl Pts',(0.115200641417765,1.79901784412022,5.63793880514564));
#57127=CARTESIAN_POINT('Ctrl Pts',(0.116056449915167,1.79934698792746,5.63799500930376));
#57128=CARTESIAN_POINT('Ctrl Pts',(0.116426726497803,1.79949018220701,5.63801936708417));
#57129=CARTESIAN_POINT('Ctrl Pts',(0.117191125786115,1.79978741744612,5.63806973508912));
#57130=CARTESIAN_POINT('Ctrl Pts',(0.117585211404007,1.79994155112205,5.63809574839436));
#57131=CARTESIAN_POINT('Ctrl Pts',(0.118592166048454,1.80033767679874,5.63816233533064));
#57132=CARTESIAN_POINT('Ctrl Pts',(0.119204596382314,1.80058077218477,5.63820294608055));
#57133=CARTESIAN_POINT('Ctrl Pts',(0.121692708438512,1.80157723597374,5.6383683965021));
#57134=CARTESIAN_POINT('Ctrl Pts',(0.123561996595663,1.80234635215689,5.6384937672534));
#57135=CARTESIAN_POINT('Ctrl Pts',(0.153976087073731,1.81519605743917,5.64055147676102));
#57136=CARTESIAN_POINT('Ctrl Pts',(0.180632608726762,1.83131271353187,5.64263724661702));
#57137=CARTESIAN_POINT('Ctrl Pts',(0.218323451649387,1.86227581723676,5.64593491201262));
#57138=CARTESIAN_POINT('Ctrl Pts',(0.231117783291788,1.87469431377972,5.64712971177108));
#57139=CARTESIAN_POINT('Ctrl Pts',(0.243540059172243,1.88892985330789,5.64832011129109));
#57140=CARTESIAN_POINT('Ctrl Pts',(0.244253613387702,1.88975599967063,5.64838860131622));
#57141=CARTESIAN_POINT('Ctrl Pts',(0.245207392567154,1.89087168592748,5.64848028122478));
#57142=CARTESIAN_POINT('Ctrl Pts',(0.245451317709631,1.89115803162573,5.64850373971649));
#57143=CARTESIAN_POINT('Ctrl Pts',(0.245833111200154,1.89160781497218,5.6485404746464));
#57144=CARTESIAN_POINT('Ctrl Pts',(0.245971318198467,1.89177096271804,5.64855377609165));
#57145=CARTESIAN_POINT('Ctrl Pts',(0.246236806859725,1.89208499443579,5.64857933425364));
#57146=CARTESIAN_POINT('Ctrl Pts',(0.246364111307641,1.89223585667622,5.64859159261534));
#57147=CARTESIAN_POINT('Ctrl Pts',(0.246662670320094,1.89259032453136,5.64862034849148));
#57148=CARTESIAN_POINT('Ctrl Pts',(0.246833811213905,1.89279402506132,5.64863683756304));
#57149=CARTESIAN_POINT('Ctrl Pts',(0.247334050469771,1.89339093432121,5.64868505162227));
#57150=CARTESIAN_POINT('Ctrl Pts',(0.247662464839708,1.89378471913909,5.6487167265097));
#57151=CARTESIAN_POINT('Ctrl Pts',(0.2484057286578,1.89468026531379,5.64878846646553));
#57152=CARTESIAN_POINT('Ctrl Pts',(0.248820001803071,1.89518250513845,5.64882849043117));
#57153=CARTESIAN_POINT('Ctrl Pts',(0.263077815607167,1.9125749219,5.65020743692388));
#57154=CARTESIAN_POINT('Ctrl Pts',(0.275172887664815,1.93083052747052,5.65142712721316));
#57155=CARTESIAN_POINT('Ctrl Pts',(0.295568074914054,1.96967074543919,5.65387957986407));
#57156=CARTESIAN_POINT('Ctrl Pts',(0.303780200765764,1.99016526284765,5.65510798192187));
#57157=CARTESIAN_POINT('Ctrl Pts',(0.311612463255215,2.01753530250231,5.65678963381482));
#57158=CARTESIAN_POINT('Ctrl Pts',(0.313199901941567,2.02378605010888,5.65717590930341));
#57159=CARTESIAN_POINT('Ctrl Pts',(0.314822314881139,2.03108593897024,5.65763104627727));
#57160=CARTESIAN_POINT('Ctrl Pts',(0.315041081815506,2.03209304538884,5.65769392484574));
#57161=CARTESIAN_POINT('Ctrl Pts',(0.315359463626633,2.03359339253839,5.65778773402111));
#57162=CARTESIAN_POINT('Ctrl Pts',(0.315462761528865,2.03408585206891,5.65781854666922));
#57163=CARTESIAN_POINT('Ctrl Pts',(0.315644749385013,2.03496368311615,5.65787351085414));
#57164=CARTESIAN_POINT('Ctrl Pts',(0.315723888129888,2.03534896141504,5.65789764798533));
#57165=CARTESIAN_POINT('Ctrl Pts',(0.315889061429835,2.03616062577541,5.65794852633307));
#57166=CARTESIAN_POINT('Ctrl Pts',(0.315974938382422,2.03658704277768,5.65797527253255));
#57167=CARTESIAN_POINT('Ctrl Pts',(0.316199098944816,2.03771186037276,5.6580458692332));
#57168=CARTESIAN_POINT('Ctrl Pts',(0.316335931405178,2.03841054472757,5.65808976596633));
#57169=CARTESIAN_POINT('Ctrl Pts',(0.316941336482345,2.04155706770522,5.65828766340539));
#57170=CARTESIAN_POINT('Ctrl Pts',(0.317383809385245,2.04400978580732,5.65844249331573));
#57171=CARTESIAN_POINT('Ctrl Pts',(0.32043777427336,2.06213971196706,5.65959141615244));
#57172=CARTESIAN_POINT('Ctrl Pts',(0.32191443786841,2.07798346376891,5.66062163362133));
#57173=CARTESIAN_POINT('Ctrl Pts',(0.32272480736288,2.12057617880755,5.66345439825226));
#57174=CARTESIAN_POINT('Ctrl Pts',(0.319910808831705,2.14724052951334,5.66530113995622));
#57175=CARTESIAN_POINT('Ctrl Pts',(0.313577984584291,2.17437304659382,5.66712043648747));
#57176=CARTESIAN_POINT('Ctrl Pts',(0.313310150769913,2.17549339023988,5.6671954287632));
#57177=CARTESIAN_POINT('Ctrl Pts',(0.311827501636082,2.18155146561861,5.66760015246425));
#57178=CARTESIAN_POINT('Ctrl Pts',(0.310501875523857,2.18646169578967,5.66792537074629));
#57179=CARTESIAN_POINT('Ctrl Pts',(0.308880426357622,2.19194814593583,5.66828399507165));
#57180=CARTESIAN_POINT('Ctrl Pts',(0.308698545359132,2.1925569415948,5.66832372269519));
#57181=CARTESIAN_POINT('Ctrl Pts',(0.308431357950041,2.19344172782026,5.6683813593692));
#57182=CARTESIAN_POINT('Ctrl Pts',(0.308347480500788,2.19371814304244,5.66839935122224));
#57183=CARTESIAN_POINT('Ctrl Pts',(0.308198811824424,2.19420571532244,5.66843106145133));
#57184=CARTESIAN_POINT('Ctrl Pts',(0.308134175070046,2.19441691884663,5.66844478892069));
#57185=CARTESIAN_POINT('Ctrl Pts',(0.30800935594309,2.19482327764441,5.66847118411638));
#57186=CARTESIAN_POINT('Ctrl Pts',(0.307949205411923,2.19501844146495,5.66848385368565));
#57187=CARTESIAN_POINT('Ctrl Pts',(0.307787191206201,2.19554234138585,5.66851784454146));
#57188=CARTESIAN_POINT('Ctrl Pts',(0.307684986031808,2.19587097288192,5.66853914569239));
#57189=CARTESIAN_POINT('Ctrl Pts',(0.307296060059555,2.19711450116972,5.668619672563));
#57190=CARTESIAN_POINT('Ctrl Pts',(0.307005779755647,2.19802829243136,5.66867869121788));
#57191=CARTESIAN_POINT('Ctrl Pts',(0.306273711829903,2.20029766584284,5.66882490653003));
#57192=CARTESIAN_POINT('Ctrl Pts',(0.305826993786587,2.20165165208551,5.66891182686689));
#57193=CARTESIAN_POINT('Ctrl Pts',(0.302633307000184,2.21111995416262,5.66951772033062));
#57194=CARTESIAN_POINT('Ctrl Pts',(0.299572489523979,2.21912561921818,5.67002006997595));
#57195=CARTESIAN_POINT('Ctrl Pts',(0.290050709682761,2.24133272623132,5.67141015765725));
#57196=CARTESIAN_POINT('Ctrl Pts',(0.282872964539985,2.25520081274931,5.67227496391193));
#57197=CARTESIAN_POINT('Ctrl Pts',(0.266578006325859,2.28176852374226,5.67401900742099));
#57198=CARTESIAN_POINT('Ctrl Pts',(0.257486302370868,2.29443347500778,5.67489617462869));
#57199=CARTESIAN_POINT('Ctrl Pts',(0.241762138362382,2.31329077274653,5.67632983483744));
#57200=CARTESIAN_POINT('Ctrl Pts',(0.235723185319355,2.31994645311042,5.67686409547644));
#57201=CARTESIAN_POINT('Ctrl Pts',(0.228699589142733,2.32706543064022,5.67747231382474));
#57202=CARTESIAN_POINT('Ctrl Pts',(0.227981231297449,2.32778667653042,5.67753437368575));
#57203=CARTESIAN_POINT('Ctrl Pts',(0.226897667255206,2.32886433668427,5.67762776975596));
#57204=CARTESIAN_POINT('Ctrl Pts',(0.226535007248728,2.32922331141897,5.67765899292806));
#57205=CARTESIAN_POINT('Ctrl Pts',(0.225907023032041,2.32984196832012,5.67771299836074));
#57206=CARTESIAN_POINT('Ctrl Pts',(0.225642099081592,2.33010205687184,5.67773576272422));
#57207=CARTESIAN_POINT('Ctrl Pts',(0.225092591286237,2.33063967348047,5.67778294270911));
#57208=CARTESIAN_POINT('Ctrl Pts',(0.224807942317624,2.33091713384641,5.6778073612343));
#57209=CARTESIAN_POINT('Ctrl Pts',(0.22414105027979,2.331564782197,5.67786452169802));
#57210=CARTESIAN_POINT('Ctrl Pts',(0.223758403101919,2.33193455070415,5.67789728182263));
#57211=CARTESIAN_POINT('Ctrl Pts',(0.222523215724299,2.3331222639505,5.67800291356466));
#57212=CARTESIAN_POINT('Ctrl Pts',(0.221667100290692,2.33393646161901,5.67807594715105));
#57213=CARTESIAN_POINT('Ctrl Pts',(0.208875399421384,2.34596858172557,5.67916458227217));
#57214=CARTESIAN_POINT('Ctrl Pts',(0.196108035538481,2.35626346296337,5.68021959986638));
#57215=CARTESIAN_POINT('Ctrl Pts',(0.163663320877388,2.37857593095105,5.68282873056233));
#57216=CARTESIAN_POINT('Ctrl Pts',(0.143372160346033,2.38954194220059,5.68440759184431));
#57217=CARTESIAN_POINT('Ctrl Pts',(0.118369341016072,2.39977661305382,5.68620824855694));
#57218=CARTESIAN_POINT('Ctrl Pts',(0.114622699869233,2.40122907817368,5.6864742988123));
#57219=CARTESIAN_POINT('Ctrl Pts',(0.108358362013218,2.40352377324617,5.68691188641338));
#57220=CARTESIAN_POINT('Ctrl Pts',(0.105855718431158,2.40440562291175,5.68708481488433));
#57221=CARTESIAN_POINT('Ctrl Pts',(0.10309639820632,2.40533977099777,5.68727320542469));
#57222=CARTESIAN_POINT('Ctrl Pts',(0.102850298155727,2.40542275495817,5.68728998795915));
#57223=CARTESIAN_POINT('Ctrl Pts',(0.0985518700657273,2.40686638336472,
5.68758276666533));
#57224=CARTESIAN_POINT('Ctrl Pts',(0.0944727170032536,2.40814665092759,
5.68785521477102));
#57225=CARTESIAN_POINT('Ctrl Pts',(0.0898458584428837,2.40949829474201,
5.68815726206931));
#57226=CARTESIAN_POINT('Ctrl Pts',(0.0893222638756283,2.40964981174545,
5.68819134288011));
#57227=CARTESIAN_POINT('Ctrl Pts',(0.0885306261060259,2.409876719668,5.68824271681912));
#57228=CARTESIAN_POINT('Ctrl Pts',(0.0882628687613149,2.40995309185485,
5.68826006658954));
#57229=CARTESIAN_POINT('Ctrl Pts',(0.0877976794361183,2.41008512571158,
5.6882901627852));
#57230=CARTESIAN_POINT('Ctrl Pts',(0.0876002932395677,2.41014094590495,
5.68830291848679));
#57231=CARTESIAN_POINT('Ctrl Pts',(0.0871873081877042,2.41025731105677,
5.68832957627332));
#57232=CARTESIAN_POINT('Ctrl Pts',(0.0869716996354782,2.41031781972045,
5.68834347615774));
#57233=CARTESIAN_POINT('Ctrl Pts',(0.0864617969686547,2.4104603463013,5.68837630778164));
#57234=CARTESIAN_POINT('Ctrl Pts',(0.0861674479696204,2.41054217084451,
5.688395228182));
#57235=CARTESIAN_POINT('Ctrl Pts',(0.0852298445650234,2.41080137460705,
5.68845539518268));
#57236=CARTESIAN_POINT('Ctrl Pts',(0.0845861501278494,2.41097717615213,
5.68849655045149));
#57237=CARTESIAN_POINT('Ctrl Pts',(0.0770385627496673,2.41301335448509,
5.68897739244752));
#57238=CARTESIAN_POINT('Ctrl Pts',(0.0700745191519581,2.41464564256456,
5.68940421491959));
#57239=CARTESIAN_POINT('Ctrl Pts',(0.0504960057673272,2.41855219743501,
5.69057213112692));
#57240=CARTESIAN_POINT('Ctrl Pts',(0.0377913431119163,2.42030799737302,
5.69129370016153));
#57241=CARTESIAN_POINT('Ctrl Pts',(0.00197268669316696,2.42309666171127,
5.69330539212059));
#57242=CARTESIAN_POINT('Ctrl Pts',(-0.0211936361763739,2.42240669334756,
5.69458529650879));
#57243=CARTESIAN_POINT('Ctrl Pts',(-0.0515550368994546,2.41821392003696,
5.6963865526067));
#57244=CARTESIAN_POINT('Ctrl Pts',(-0.0589847213401951,2.41692082523618,
5.69683679066854));
#57245=CARTESIAN_POINT('Ctrl Pts',(-0.0673114676605211,2.41516865917588,
5.69735450050088));
#57246=CARTESIAN_POINT('Ctrl Pts',(-0.0682602083284834,2.41496453980095,
5.69741368029993));
#57247=CARTESIAN_POINT('Ctrl Pts',(-0.0696945380990065,2.4146491619938,
5.69750344635019));
#57248=CARTESIAN_POINT('Ctrl Pts',(-0.0701808208012834,2.41454105641631,
5.69753393153673));
#57249=CARTESIAN_POINT('Ctrl Pts',(-0.0710260278052374,2.41435110072193,
5.69758700842962));
#57250=CARTESIAN_POINT('Ctrl Pts',(-0.0713850670894342,2.41426976206071,
5.69760958368488));
#57251=CARTESIAN_POINT('Ctrl Pts',(-0.0721335860859953,2.41409883970402,
5.69765670795708));
#57252=CARTESIAN_POINT('Ctrl Pts',(-0.0725230399259975,2.41400914639972,
5.69768126046333));
#57253=CARTESIAN_POINT('Ctrl Pts',(-0.0734428991119554,2.41379549533252,
5.69773933187717));
#57254=CARTESIAN_POINT('Ctrl Pts',(-0.073973157767019,2.41367091711715,
5.69777287069511));
#57255=CARTESIAN_POINT('Ctrl Pts',(-0.0757201339037588,2.4132558088181,
5.69788357678611));
#57256=CARTESIAN_POINT('Ctrl Pts',(-0.0769354642836219,2.41295954163662,
5.69796092864064));
#57257=CARTESIAN_POINT('Ctrl Pts',(-0.0908184268523851,2.40948946824201,
5.69884844593346));
#57258=CARTESIAN_POINT('Ctrl Pts',(-0.103281950967356,2.40555601452187,
5.69968330975698));
#57259=CARTESIAN_POINT('Ctrl Pts',(-0.127037177113129,2.3964392077659,5.70135166033467));
#57260=CARTESIAN_POINT('Ctrl Pts',(-0.138336641184565,2.39133756838317,
5.70218156951798));
#57261=CARTESIAN_POINT('Ctrl Pts',(-0.159755809498103,2.38013942817263,
5.70381385362561));
#57262=CARTESIAN_POINT('Ctrl Pts',(-0.16989078355478,2.37411155634012,5.70461431947547));
#57263=CARTESIAN_POINT('Ctrl Pts',(-0.187894537828682,2.36202079688238,
5.70606813003992));
#57264=CARTESIAN_POINT('Ctrl Pts',(-0.195858016562943,2.35612287662011,
5.7067237176934));
#57265=CARTESIAN_POINT('Ctrl Pts',(-0.20616813639496,2.3477244125013,5.70757729963383));
#57266=CARTESIAN_POINT('Ctrl Pts',(-0.208764590572189,2.34554028793596,
5.70779268181104));
#57267=CARTESIAN_POINT('Ctrl Pts',(-0.211753026051544,2.34294474927109,
5.70804058857714));
#57268=CARTESIAN_POINT('Ctrl Pts',(-0.212178885652864,2.34257290808132,
5.70807591609431));
#57269=CARTESIAN_POINT('Ctrl Pts',(-0.212812969749657,2.34201630734162,
5.70812851435845));
#57270=CARTESIAN_POINT('Ctrl Pts',(-0.213021934032479,2.34183239802683,
5.70814584783501));
#57271=CARTESIAN_POINT('Ctrl Pts',(-0.213394757707541,2.34150341799366,
5.70817677215883));
#57272=CARTESIAN_POINT('Ctrl Pts',(-0.213558707444492,2.34135845126153,
5.7081903707374));
#57273=CARTESIAN_POINT('Ctrl Pts',(-0.213876001819698,2.34107731856288,
5.70821668733534));
#57274=CARTESIAN_POINT('Ctrl Pts',(-0.214029363411063,2.34094117389576,
5.70822940685426));
#57275=CARTESIAN_POINT('Ctrl Pts',(-0.214364328487292,2.34064324102714,
5.70825718764066));
#57276=CARTESIAN_POINT('Ctrl Pts',(-0.214545879185266,2.34048139326237,
5.70827224442213));
#57277=CARTESIAN_POINT('Ctrl Pts',(-0.215281099969483,2.33982446762575,
5.70833321877181));
#57278=CARTESIAN_POINT('Ctrl Pts',(-0.215833246773317,2.33932767681374,
5.70837900861677));
#57279=CARTESIAN_POINT('Ctrl Pts',(-0.223635443495532,2.33225873547486,
5.70902611064433));
#57280=CARTESIAN_POINT('Ctrl Pts',(-0.230585042190231,2.32536085141049,
5.70960329324905));
#57281=CARTESIAN_POINT('Ctrl Pts',(-0.24165130376895,2.31332805169386,5.71054599300962));
#57282=CARTESIAN_POINT('Ctrl Pts',(-0.24594370640364,2.30836484860853,5.71091830974663));
#57283=CARTESIAN_POINT('Ctrl Pts',(-0.265923845083845,2.28378388563311,
5.71270282061998));
#57284=CARTESIAN_POINT('Ctrl Pts',(-0.279432359874984,2.26251008316921,
5.71407907431262));
#57285=CARTESIAN_POINT('Ctrl Pts',(-0.29423414796575,2.23178842069122,5.7160702635909));
#57286=CARTESIAN_POINT('Ctrl Pts',(-0.297793879060483,2.22353422313462,
5.71660464149274));
#57287=CARTESIAN_POINT('Ctrl Pts',(-0.301367622035029,2.21419180520443,
5.71721298623936));
#57288=CARTESIAN_POINT('Ctrl Pts',(-0.30172682978468,2.21323926941554,5.71727504970301));
#57289=CARTESIAN_POINT('Ctrl Pts',(-0.302259309349847,2.21180673476348,
5.71736845030554));
#57290=CARTESIAN_POINT('Ctrl Pts',(-0.302435966416557,2.21132799396412,
5.71739967439195));
#57291=CARTESIAN_POINT('Ctrl Pts',(-0.302739182661009,2.2105002295976,5.71745368097865));
#57292=CARTESIAN_POINT('Ctrl Pts',(-0.302866277512642,2.21015140218419,
5.71747644558001));
#57293=CARTESIAN_POINT('Ctrl Pts',(-0.30312820201904,2.20942863781447,5.71752362565372));
#57294=CARTESIAN_POINT('Ctrl Pts',(-0.303262943118027,2.20905466960388,
5.71754804402917));
#57295=CARTESIAN_POINT('Ctrl Pts',(-0.303576432152048,2.20817952024651,
5.7176052034412));
#57296=CARTESIAN_POINT('Ctrl Pts',(-0.303754631016065,2.20767814490327,
5.71763796266186));
#57297=CARTESIAN_POINT('Ctrl Pts',(-0.304324470392052,2.2060621893944,5.71774358860175));
#57298=CARTESIAN_POINT('Ctrl Pts',(-0.304711220734981,2.20494590605264,
5.71781661726496));
#57299=CARTESIAN_POINT('Ctrl Pts',(-0.310290095914531,2.18855267073059,
5.71889007753343));
#57300=CARTESIAN_POINT('Ctrl Pts',(-0.3143330827811,2.1729115014575,5.71992871658828));
#57301=CARTESIAN_POINT('Ctrl Pts',(-0.320587101506358,2.13813140654909,
5.72226851870401));
#57302=CARTESIAN_POINT('Ctrl Pts',(-0.322289269816695,2.1189626625909,5.72357815247994));
#57303=CARTESIAN_POINT('Ctrl Pts',(-0.322274909898337,2.09975901240904,
5.72487103019784));
#57304=CARTESIAN_POINT('',(-0.322274982545603,2.10010606710754,5.97444230798123));
#57305=CARTESIAN_POINT('Ctrl Pts',(-0.322274909611437,2.09975862903993,
5.724871056008));
#57306=CARTESIAN_POINT('Ctrl Pts',(-0.322264020214785,2.085219268876,5.7258499121261));
#57307=CARTESIAN_POINT('Ctrl Pts',(-0.321269222642355,2.07069492405067,
5.7268157023856));
#57308=CARTESIAN_POINT('Ctrl Pts',(-0.319195443610201,2.05554779287244,
5.72777898760693));
#57309=CARTESIAN_POINT('Ctrl Pts',(-0.319091896698514,2.0548104942833,5.7278257642248));
#57310=CARTESIAN_POINT('Ctrl Pts',(-0.318928349001282,2.05367456073724,
5.7278976518244));
#57311=CARTESIAN_POINT('Ctrl Pts',(-0.318870154632419,2.05327567433946,
5.72792286117238));
#57312=CARTESIAN_POINT('Ctrl Pts',(-0.318772580783095,2.05261553877446,
5.72796452348555));
#57313=CARTESIAN_POINT('Ctrl Pts',(-0.31873362840297,2.05235422840359,5.72798100023831));
#57314=CARTESIAN_POINT('Ctrl Pts',(-0.318663139620769,2.05188531236647,
5.72801054013422));
#57315=CARTESIAN_POINT('Ctrl Pts',(-0.318631721622433,2.05167768946372,
5.72802360996504));
#57316=CARTESIAN_POINT('Ctrl Pts',(-0.318570404651505,2.05127514192537,
5.72804893144045));
#57317=CARTESIAN_POINT('Ctrl Pts',(-0.318540529715395,2.05108021419087,
5.72806118441127));
#57318=CARTESIAN_POINT('Ctrl Pts',(-0.318477770839417,2.05067322067429,
5.72808674964826));
#57319=CARTESIAN_POINT('Ctrl Pts',(-0.318444854103606,2.05046116096334,
5.72810005998056));
#57320=CARTESIAN_POINT('Ctrl Pts',(-0.318363327599387,2.0499393812093,5.72813278580853));
#57321=CARTESIAN_POINT('Ctrl Pts',(-0.318314477530252,2.04962969813026,
5.7281521876118));
#57322=CARTESIAN_POINT('Ctrl Pts',(-0.318122668337188,2.04842515414412,
5.72822757134989));
#57323=CARTESIAN_POINT('Ctrl Pts',(-0.317976385209643,2.047530815421,5.72828336638451));
#57324=CARTESIAN_POINT('Ctrl Pts',(-0.315432598807844,2.03238017349651,
5.72922577782891));
#57325=CARTESIAN_POINT('Ctrl Pts',(-0.312081916676324,2.01829833798893,
5.73006006792826));
#57326=CARTESIAN_POINT('Ctrl Pts',(-0.306976563440437,2.00184596680618,
5.73103477195394));
#57327=CARTESIAN_POINT('Ctrl Pts',(-0.306122915064667,1.99921515026202,
5.73119061816042));
#57328=CARTESIAN_POINT('Ctrl Pts',(-0.304541249977357,1.99454629253937,
5.7314676554991));
#57329=CARTESIAN_POINT('Ctrl Pts',(-0.303826375874321,1.99250399645486,
5.7315889983304));
#57330=CARTESIAN_POINT('Ctrl Pts',(-0.301630030894537,1.98642633230106,
5.73195095261844));
#57331=CARTESIAN_POINT('Ctrl Pts',(-0.300088333785187,1.98241324180227,
5.73219108413579));
#57332=CARTESIAN_POINT('Ctrl Pts',(-0.295022319998671,1.96997543517858,
5.73294180271045));
#57333=CARTESIAN_POINT('Ctrl Pts',(-0.291220029513777,1.96166907638582,
5.73345270318302));
#57334=CARTESIAN_POINT('Ctrl Pts',(-0.27997183669563,1.93962261910464,5.73485597204474));
#57335=CARTESIAN_POINT('Ctrl Pts',(-0.271872288473323,1.92624587230503,
5.73576052391397));
#57336=CARTESIAN_POINT('Ctrl Pts',(-0.261408150838758,1.911497902633,5.73685120325654));
#57337=CARTESIAN_POINT('Ctrl Pts',(-0.259957515463289,1.9095023578399,5.73700086137625));
#57338=CARTESIAN_POINT('Ctrl Pts',(-0.258060482504202,1.90695475611422,
5.73719469596328));
#57339=CARTESIAN_POINT('Ctrl Pts',(-0.257634947752474,1.90638720987205,
5.73723805739455));
#57340=CARTESIAN_POINT('Ctrl Pts',(-0.256945809489131,1.90547438391682,
5.73730809102925));
#57341=CARTESIAN_POINT('Ctrl Pts',(-0.256683373954672,1.90512822200512,
5.73733471733814));
#57342=CARTESIAN_POINT('Ctrl Pts',(-0.256181905454801,1.90446953753993,
5.73738551304584));
#57343=CARTESIAN_POINT('Ctrl Pts',(-0.25594299829978,1.90415691982754,5.73740967745715));
#57344=CARTESIAN_POINT('Ctrl Pts',(-0.255396596907795,1.90344464343799,
5.73746486335632));
#57345=CARTESIAN_POINT('Ctrl Pts',(-0.255088736498328,1.90304526811376,
5.737495899293));
#57346=CARTESIAN_POINT('Ctrl Pts',(-0.254145495548868,1.90182755969468,
5.73759081479355));
#57347=CARTESIAN_POINT('Ctrl Pts',(-0.253507109766786,1.90101157254281,
5.73765481359475));
#57348=CARTESIAN_POINT('Ctrl Pts',(-0.248794707925047,1.89504764492045,
5.73812550881994));
#57349=CARTESIAN_POINT('Ctrl Pts',(-0.244568429261714,1.89002250660112,
5.73853829834352));
#57350=CARTESIAN_POINT('Ctrl Pts',(-0.239852900918646,1.88475126002786,
5.73898964479482));
#57351=CARTESIAN_POINT('Ctrl Pts',(-0.239513013314509,1.88437312183531,
5.73902212719018));
#57352=CARTESIAN_POINT('Ctrl Pts',(-0.222452284321282,1.8654825053648,5.7406500978203));
#57353=CARTESIAN_POINT('Ctrl Pts',(-0.203641755261037,1.84897588595725,
5.74233559596896));
#57354=CARTESIAN_POINT('Ctrl Pts',(-0.177549458293191,1.83095872620241,
5.74447972759449));
#57355=CARTESIAN_POINT('Ctrl Pts',(-0.171858026096936,1.82728798940623,
5.74493644773138));
#57356=CARTESIAN_POINT('Ctrl Pts',(-0.15969252041563,1.81997394975125,5.74588490190476));
#57357=CARTESIAN_POINT('Ctrl Pts',(-0.153199251541654,1.81636944053919,
5.74637550297007));
#57358=CARTESIAN_POINT('Ctrl Pts',(-0.142437215140867,1.81087281898544,
5.7471572673649));
#57359=CARTESIAN_POINT('Ctrl Pts',(-0.138241813160883,1.80884352349147,
5.7474545593267));
#57360=CARTESIAN_POINT('Ctrl Pts',(-0.133494983877891,1.80667325780593,
5.74778144830025));
#57361=CARTESIAN_POINT('Ctrl Pts',(-0.132985745640435,1.80644203319553,
5.74781639612182));
#57362=CARTESIAN_POINT('Ctrl Pts',(-0.132272460729269,1.80612039614442,
5.74786517582073));
#57363=CARTESIAN_POINT('Ctrl Pts',(-0.132068921944593,1.80602886997733,
5.74787907582819));
#57364=CARTESIAN_POINT('Ctrl Pts',(-0.131660609538261,1.80584577202053,
5.74790692088508));
#57365=CARTESIAN_POINT('Ctrl Pts',(-0.131455834728225,1.80575420230832,
5.74792086581216));
#57366=CARTESIAN_POINT('Ctrl Pts',(-0.131064006674325,1.80557947815676,
5.74794751079608));
#57367=CARTESIAN_POINT('Ctrl Pts',(-0.130876970049189,1.80549628824191,
5.74796021306663));
#57368=CARTESIAN_POINT('Ctrl Pts',(-0.130436870970177,1.80530104358354,
5.74799006303583));
#57369=CARTESIAN_POINT('Ctrl Pts',(-0.130183742689964,1.80518913628904,
5.74800720161665));
#57370=CARTESIAN_POINT('Ctrl Pts',(-0.129437617781264,1.80486042492366,
5.74805763217225));
#57371=CARTESIAN_POINT('Ctrl Pts',(-0.128944218399221,1.80464452904267,
5.74809086874667));
#57372=CARTESIAN_POINT('Ctrl Pts',(-0.124692690825109,1.8027968799296,5.74837631593897));
#57373=CARTESIAN_POINT('Ctrl Pts',(-0.120904092192029,1.80123560112782,
5.74862432923978));
#57374=CARTESIAN_POINT('Ctrl Pts',(-0.116712896374063,1.79960120459046,
5.74889286326565));
#57375=CARTESIAN_POINT('Ctrl Pts',(-0.116338980714718,1.79945619614954,
5.74891676987989));
#57376=CARTESIAN_POINT('Ctrl Pts',(-0.107420720490024,1.79601673793573,
5.74948578492848));
#57377=CARTESIAN_POINT('Ctrl Pts',(-0.0987393731918041,1.79308698671092,
5.75001391482371));
#57378=CARTESIAN_POINT('Ctrl Pts',(-0.0731892849765471,1.78566108793362,
5.75152548454611));
#57379=CARTESIAN_POINT('Ctrl Pts',(-0.0560661024676764,1.78216002814846,
5.75248713534905));
#57380=CARTESIAN_POINT('Ctrl Pts',(-0.0361929644712237,1.77975346287182,
5.75361603242056));
#57381=CARTESIAN_POINT('Ctrl Pts',(-0.0336390536165905,1.7794751350974,
5.7537613102101));
#57382=CARTESIAN_POINT('Ctrl Pts',(-0.0278258770146788,1.7789118519331,
5.75409280333765));
#57383=CARTESIAN_POINT('Ctrl Pts',(-0.0245650802082596,1.77864593609912,
5.75427932937292));
#57384=CARTESIAN_POINT('Ctrl Pts',(-0.0089746082849849,1.77761322139547,
5.75517531778487));
#57385=CARTESIAN_POINT('Ctrl Pts',(0.00338707621833142,1.77750619676307,
5.75589873554261));
#57386=CARTESIAN_POINT('Ctrl Pts',(0.0178607208586101,1.77821319323672,
5.75677439859087));
#57387=CARTESIAN_POINT('Ctrl Pts',(0.0199968357020707,1.77833887307228,
5.75690435203885));
#57388=CARTESIAN_POINT('Ctrl Pts',(0.0228031314669913,1.77853204507372,
5.75707607027264));
#57389=CARTESIAN_POINT('Ctrl Pts',(0.0234746108622119,1.77858038099205,
5.75711723314175));
#57390=CARTESIAN_POINT('Ctrl Pts',(0.0245710600039138,1.77866276220894,
5.75718457131871));
#57391=CARTESIAN_POINT('Ctrl Pts',(0.0249961246925882,1.77869554760556,
5.75721070700293));
#57392=CARTESIAN_POINT('Ctrl Pts',(0.0258156727782518,1.77876039579559,
5.75726115721789));
#57393=CARTESIAN_POINT('Ctrl Pts',(0.026210164840199,1.77879234204766,5.75728546804184));
#57394=CARTESIAN_POINT('Ctrl Pts',(0.0271152304769176,1.77886731334499,
5.75734130444039));
#57395=CARTESIAN_POINT('Ctrl Pts',(0.0276257613239366,1.77891082941257,
5.75737284539908));
#57396=CARTESIAN_POINT('Ctrl Pts',(0.0289823249762215,1.77902971801466,
5.75745677468915));
#57397=CARTESIAN_POINT('Ctrl Pts',(0.0298281630306431,1.77910721767719,
5.75750922980785));
#57398=CARTESIAN_POINT('Ctrl Pts',(0.0355108900033,1.77965055823793,5.75786249190126));
#57399=CARTESIAN_POINT('Ctrl Pts',(0.0403367945243799,1.78022237883874,
5.75816661937243));
#57400=CARTESIAN_POINT('Ctrl Pts',(0.0467085879788301,1.78112389788232,
5.75857393098527));
#57401=CARTESIAN_POINT('Ctrl Pts',(0.0482677884194959,1.78135618450388,
5.75867405959665));
#57402=CARTESIAN_POINT('Ctrl Pts',(0.0719039902823701,1.78505492229719,
5.76019893461121));
#57403=CARTESIAN_POINT('Ctrl Pts',(0.0935600316628738,1.79079651517814,
5.76169542593593));
#57404=CARTESIAN_POINT('Ctrl Pts',(0.127061324020658,1.80352276349304,5.76412026410933));
#57405=CARTESIAN_POINT('Ctrl Pts',(0.13936521000401,1.80910362186993,5.76503510033277));
#57406=CARTESIAN_POINT('Ctrl Pts',(0.155727752179207,1.81780258964203,5.76625869693939));
#57407=CARTESIAN_POINT('Ctrl Pts',(0.160116439268343,1.82026933903393,5.76658753318001));
#57408=CARTESIAN_POINT('Ctrl Pts',(0.166592007020732,1.82411142333808,5.76707180206359));
#57409=CARTESIAN_POINT('Ctrl Pts',(0.168723458823988,1.8254097619282,5.76723104332797));
#57410=CARTESIAN_POINT('Ctrl Pts',(0.171668649034083,1.8272510195755,5.76745062920414));
#57411=CARTESIAN_POINT('Ctrl Pts',(0.172495261860654,1.82777304307551,5.76751220932676));
#57412=CARTESIAN_POINT('Ctrl Pts',(0.173918737159818,1.82868108488885,5.76761814977272));
#57413=CARTESIAN_POINT('Ctrl Pts',(0.174516716215791,1.82906532776999,5.76766262169365));
#57414=CARTESIAN_POINT('Ctrl Pts',(0.175369504301298,1.82961729782662,5.76772599249199));
#57415=CARTESIAN_POINT('Ctrl Pts',(0.175625348563394,1.82978340980375,5.7677449976804));
#57416=CARTESIAN_POINT('Ctrl Pts',(0.176068531828038,1.83007205066311,5.76777790714728));
#57417=CARTESIAN_POINT('Ctrl Pts',(0.176255979434251,1.83019441175523,5.76779182269803));
#57418=CARTESIAN_POINT('Ctrl Pts',(0.176615038472122,1.83042933036116,5.76781847075867));
#57419=CARTESIAN_POINT('Ctrl Pts',(0.176786669606336,1.83054185632248,5.76783120536785));
#57420=CARTESIAN_POINT('Ctrl Pts',(0.177191235769833,1.83080765363453,5.76786121585116));
#57421=CARTESIAN_POINT('Ctrl Pts',(0.177424080046902,1.83096106379139,5.76787848236141));
#57422=CARTESIAN_POINT('Ctrl Pts',(0.178112808169605,1.8314161173708,5.76792953873331));
#57423=CARTESIAN_POINT('Ctrl Pts',(0.178568126892339,1.83171862064108,5.76796327123243));
#57424=CARTESIAN_POINT('Ctrl Pts',(0.182613911540048,1.83442140955377,5.76826283957173));
#57425=CARTESIAN_POINT('Ctrl Pts',(0.186156770692396,1.83689262732509,5.76852400698594));
#57426=CARTESIAN_POINT('Ctrl Pts',(0.189832962423795,1.8395682935528,5.76879498156927));
#57427=CARTESIAN_POINT('Ctrl Pts',(0.19001669596465,1.83970231925575,5.76880852463292));
#57428=CARTESIAN_POINT('Ctrl Pts',(0.190331989504498,1.8399328240392,5.76883176521534));
#57429=CARTESIAN_POINT('Ctrl Pts',(0.190463618150189,1.84002920855929,5.76884146774175));
#57430=CARTESIAN_POINT('Ctrl Pts',(0.192557291080573,1.84156473533348,5.76899579708992));
#57431=CARTESIAN_POINT('Ctrl Pts',(0.194503099910967,1.84302599135101,5.76913925340138));
#57432=CARTESIAN_POINT('Ctrl Pts',(0.199620658817928,1.84696058861459,5.76951716220704));
#57433=CARTESIAN_POINT('Ctrl Pts',(0.202763038178625,1.84947155110292,5.76974985090437));
#57434=CARTESIAN_POINT('Ctrl Pts',(0.225789296172022,1.86858813005397,5.77146645239087));
#57435=CARTESIAN_POINT('Ctrl Pts',(0.243653415116403,1.88747846755907,5.77287144592799));
#57436=CARTESIAN_POINT('Ctrl Pts',(0.262432066876406,1.91285660377111,5.77468258066731));
#57437=CARTESIAN_POINT('Ctrl Pts',(0.265679589454469,1.9174963246509,5.77501058313047));
#57438=CARTESIAN_POINT('Ctrl Pts',(0.272842445818083,1.92832649312977,5.77577214957779));
#57439=CARTESIAN_POINT('Ctrl Pts',(0.276672215041648,1.93456945252373,5.77620826617175));
#57440=CARTESIAN_POINT('Ctrl Pts',(0.281053451903209,1.94228965952567,5.77674659322142));
#57441=CARTESIAN_POINT('Ctrl Pts',(0.281811236515871,1.94364776573232,5.77684125427333));
#57442=CARTESIAN_POINT('Ctrl Pts',(0.282845231187349,1.94553283625092,5.77697261062435));
#57443=CARTESIAN_POINT('Ctrl Pts',(0.283129865036585,1.9460551754719,5.77700900484827));
#57444=CARTESIAN_POINT('Ctrl Pts',(0.283607932464402,1.94693830051208,5.77707053202901));
#57445=CARTESIAN_POINT('Ctrl Pts',(0.283802128513008,1.94729867369306,5.77709563778086));
#57446=CARTESIAN_POINT('Ctrl Pts',(0.284185069719855,1.9480125585161,5.77714536895957));
#57447=CARTESIAN_POINT('Ctrl Pts',(0.284373843201527,1.94836605419304,5.77716999332281));
#57448=CARTESIAN_POINT('Ctrl Pts',(0.284788501857637,1.94914603832949,5.77722432467714));
#57449=CARTESIAN_POINT('Ctrl Pts',(0.285014089031827,1.94957268336064,5.77725404216285));
#57450=CARTESIAN_POINT('Ctrl Pts',(0.28579906497395,1.95106538521777,5.77735801118651));
#57451=CARTESIAN_POINT('Ctrl Pts',(0.286353432503831,1.95213405851747,5.77743243983861));
#57452=CARTESIAN_POINT('Ctrl Pts',(0.29216026547678,1.96348321814778,5.77822284688498));
#57453=CARTESIAN_POINT('Ctrl Pts',(0.296862095679574,1.97403455187322,5.77895803127679));
#57454=CARTESIAN_POINT('Ctrl Pts',(0.301797820013975,1.98693191307256,5.77985828991696));
#57455=CARTESIAN_POINT('Ctrl Pts',(0.30258581472433,1.989057939372,5.78000672355907));
#57456=CARTESIAN_POINT('Ctrl Pts',(0.306168918568508,1.99904746098387,5.78070423647146));
#57457=CARTESIAN_POINT('Ctrl Pts',(0.308680197622661,2.00700890725271,5.78126045979066));
#57458=CARTESIAN_POINT('Ctrl Pts',(0.315345814615061,2.03140455036122,5.78296014253687));
#57459=CARTESIAN_POINT('Ctrl Pts',(0.318515844734172,2.0480772342913,5.78411679298052));
#57460=CARTESIAN_POINT('Ctrl Pts',(0.321480516982876,2.0751528316532,5.78593347850045));
#57461=CARTESIAN_POINT('Ctrl Pts',(0.322110149726099,2.08543283351798,5.7866087320004));
#57462=CARTESIAN_POINT('Ctrl Pts',(0.322259612980905,2.0967028530805,5.78732127092103));
#57463=CARTESIAN_POINT('Ctrl Pts',(0.322268124840648,2.09767941712541,5.78738278437888));
#57464=CARTESIAN_POINT('Ctrl Pts',(0.322275158787201,2.09936608214417,5.78748861377938));
#57465=CARTESIAN_POINT('Ctrl Pts',(0.322275773283339,2.1000761609614,5.78753304106816));
#57466=CARTESIAN_POINT('Ctrl Pts',(0.32227329686296,2.10109122249819,5.78759636378561));
#57467=CARTESIAN_POINT('Ctrl Pts',(0.322272119894244,2.1013962013366,5.78761536527523));
#57468=CARTESIAN_POINT('Ctrl Pts',(0.322269328447923,2.10192501137883,5.78764827017607));
#57469=CARTESIAN_POINT('Ctrl Pts',(0.322267913701746,2.10214884307118,5.78766218485182));
#57470=CARTESIAN_POINT('Ctrl Pts',(0.32226475467842,2.10257791442516,5.78768883303995));
#57471=CARTESIAN_POINT('Ctrl Pts',(0.322263047536509,2.102783153571,5.78770156864816));
#57472=CARTESIAN_POINT('Ctrl Pts',(0.32225855812668,2.10326728099141,5.78773158406687));
#57473=CARTESIAN_POINT('Ctrl Pts',(0.322255609887789,2.10354616809737,5.78774885450597));
#57474=CARTESIAN_POINT('Ctrl Pts',(0.322245808608929,2.1043719044401,5.78779993014431));
#57475=CARTESIAN_POINT('Ctrl Pts',(0.322237925581,2.10491874395003,5.78783367792004));
#57476=CARTESIAN_POINT('Ctrl Pts',(0.322155284597172,2.10979093748329,5.78813369825474));
#57477=CARTESIAN_POINT('Ctrl Pts',(0.321994830511464,2.11411465318918,5.78839528687277));
#57478=CARTESIAN_POINT('Ctrl Pts',(0.321744450091459,2.11848477858142,5.78865614477654));
#57479=CARTESIAN_POINT('Ctrl Pts',(0.321741533357088,2.11853547725027,5.78865917055703));
#57480=CARTESIAN_POINT('Ctrl Pts',(0.321675956172566,2.11967066033943,5.7887269094025));
#57481=CARTESIAN_POINT('Ctrl Pts',(0.321607824100771,2.12075483544003,5.78879138459255));
#57482=CARTESIAN_POINT('Ctrl Pts',(0.319592037439303,2.15043359813829,5.79055083800215));
#57483=CARTESIAN_POINT('Ctrl Pts',(0.313843979427069,2.17864470165379,5.79209291094241));
#57484=CARTESIAN_POINT('Ctrl Pts',(0.299036769110684,2.22128215275347,5.79465792259777));
#57485=CARTESIAN_POINT('Ctrl Pts',(0.292450916738611,2.23639902505667,5.79561639975298));
#57486=CARTESIAN_POINT('Ctrl Pts',(0.28418397398593,2.25199359293855,5.79668944121871));
#57487=CARTESIAN_POINT('Ctrl Pts',(0.283622477448984,2.25303879766774,5.79676177512135));
#57488=CARTESIAN_POINT('Ctrl Pts',(0.282800378582326,2.25454903957084,5.79686690375821));
#57489=CARTESIAN_POINT('Ctrl Pts',(0.282544369400296,2.25501657676963,5.79689953466767));
#57490=CARTESIAN_POINT('Ctrl Pts',(0.282095350755949,2.25583179020305,5.79695658125485));
#57491=CARTESIAN_POINT('Ctrl Pts',(0.281902855005901,2.25617974930586,5.79698097851482));
#57492=CARTESIAN_POINT('Ctrl Pts',(0.281529518718597,2.25685166037853,5.79702818294984));
#57493=CARTESIAN_POINT('Ctrl Pts',(0.281348761713098,2.25717565827489,5.79705098710138));
#57494=CARTESIAN_POINT('Ctrl Pts',(0.280918528383279,2.25794370977834,5.79710514550435));
#57495=CARTESIAN_POINT('Ctrl Pts',(0.28066855860949,2.25838748451468,5.79713651746574));
#57496=CARTESIAN_POINT('Ctrl Pts',(0.279784449916111,2.25994838956708,5.79724714536905));
#57497=CARTESIAN_POINT('Ctrl Pts',(0.279144691188368,2.26106230795778,5.79732660377483));
#57498=CARTESIAN_POINT('Ctrl Pts',(0.269354828356038,2.27787442160478,5.79853369159408));
#57499=CARTESIAN_POINT('Ctrl Pts',(0.258901495141235,2.29277226205717,5.7997101645988));
#57500=CARTESIAN_POINT('Ctrl Pts',(0.232144611744198,2.32477706708822,5.80248977170565));
#57501=CARTESIAN_POINT('Ctrl Pts',(0.215104426518439,2.34113455490837,5.80411004221691));
#57502=CARTESIAN_POINT('Ctrl Pts',(0.190243796952678,2.36024883379797,5.80618075224492));
#57503=CARTESIAN_POINT('Ctrl Pts',(0.183881431769681,2.36478255149144,5.80668791401487));
#57504=CARTESIAN_POINT('Ctrl Pts',(0.176664087766309,2.36953973833608,5.80723328033171));
#57505=CARTESIAN_POINT('Ctrl Pts',(0.175966326557108,2.36999578219339,5.80728570426058));
#57506=CARTESIAN_POINT('Ctrl Pts',(0.174899792244733,2.37068695860006,5.80736536704225));
#57507=CARTESIAN_POINT('Ctrl Pts',(0.17453230328793,2.37092405208418,5.80739273172469));
#57508=CARTESIAN_POINT('Ctrl Pts',(0.173852631104433,2.37136060053063,5.80744318576719));
#57509=CARTESIAN_POINT('Ctrl Pts',(0.173540585064222,2.37156026624145,5.80746628892765));
#57510=CARTESIAN_POINT('Ctrl Pts',(0.17303052537325,2.37188539472137,5.80750395228057));
#57511=CARTESIAN_POINT('Ctrl Pts',(0.172832718999569,2.37201117958238,5.8075185339523));
#57512=CARTESIAN_POINT('Ctrl Pts',(0.172448269763176,2.37225506177614,5.80754682640895));
#57513=CARTESIAN_POINT('Ctrl Pts',(0.17226164327628,2.37237318271634,5.80756053872138));
#57514=CARTESIAN_POINT('Ctrl Pts',(0.171830691427337,2.37264532368112,5.80759215244075));
#57515=CARTESIAN_POINT('Ctrl Pts',(0.171586279576572,2.37279920766786,5.80761004474133));
#57516=CARTESIAN_POINT('Ctrl Pts',(0.170803708464042,2.37329045396174,5.80766721535858));
#57517=CARTESIAN_POINT('Ctrl Pts',(0.17026475434948,2.37362655663183,5.80770641046022));
#57518=CARTESIAN_POINT('Ctrl Pts',(0.165407627397522,2.37663565180014,5.80805807585713));
#57519=CARTESIAN_POINT('Ctrl Pts',(0.161027535321424,2.37920799945013,5.80836409484753));
#57520=CARTESIAN_POINT('Ctrl Pts',(0.156401960934109,2.38177943082283,5.80867781143872));
#57521=CARTESIAN_POINT('Ctrl Pts',(0.156215639853434,2.38188276798077,5.80869043238856));
#57522=CARTESIAN_POINT('Ctrl Pts',(0.155336867165052,2.38236901287315,5.80874988480085));
#57523=CARTESIAN_POINT('Ctrl Pts',(0.154643103782922,2.38274955739266,5.80879660545504));
#57524=CARTESIAN_POINT('Ctrl Pts',(0.151923850567915,2.38422812574864,5.80897891784714));
#57525=CARTESIAN_POINT('Ctrl Pts',(0.14988797096674,2.38530699339266,5.80911365639485));
#57526=CARTESIAN_POINT('Ctrl Pts',(0.12098121698274,2.40023063584287,5.8110045253961));
#57527=CARTESIAN_POINT('Ctrl Pts',(0.0923034097621147,2.41025036243928,
5.81262513990115));
#57528=CARTESIAN_POINT('Ctrl Pts',(0.0519879773275619,2.41823969953699,
5.81499633121213));
#57529=CARTESIAN_POINT('Ctrl Pts',(0.0412297780674123,2.41981138772159,
5.81563587608256));
#57530=CARTESIAN_POINT('Ctrl Pts',(0.0284451823997788,2.4210232957224,5.81641264057607));
#57531=CARTESIAN_POINT('Ctrl Pts',(0.0264752030585762,2.42119176227135,
5.81653278789971));
#57532=CARTESIAN_POINT('Ctrl Pts',(0.0238523243728455,2.42139176899382,
5.81669340008371));
#57533=CARTESIAN_POINT('Ctrl Pts',(0.0232006712699923,2.42143946770376,
5.81673335699306));
#57534=CARTESIAN_POINT('Ctrl Pts',(0.0221279762260744,2.42151470623572,
5.81679921918326));
#57535=CARTESIAN_POINT('Ctrl Pts',(0.0217070150997383,2.42154340165906,
5.81682508813054));
#57536=CARTESIAN_POINT('Ctrl Pts',(0.0208893446200458,2.42159752631441,
5.81687537974956));
#57537=CARTESIAN_POINT('Ctrl Pts',(0.0204926420069347,2.42162304841464,
5.81689979945853));
#57538=CARTESIAN_POINT('Ctrl Pts',(0.0195738867001377,2.42168045035464,
5.81695640207538));
#57539=CARTESIAN_POINT('Ctrl Pts',(0.0190518026564808,2.42171179336684,
5.81698860177151));
#57540=CARTESIAN_POINT('Ctrl Pts',(0.0176455946837466,2.42179277921376,
5.81707542595115));
#57541=CARTESIAN_POINT('Ctrl Pts',(0.0167613433665243,2.42184004895187,
5.8171301247436));
#57542=CARTESIAN_POINT('Ctrl Pts',(0.0103496192081794,2.42215630731137,
5.81752750017183));
#57543=CARTESIAN_POINT('Ctrl Pts',(0.00481651662403091,2.42228651226943,
5.81787450419063));
#57544=CARTESIAN_POINT('Ctrl Pts',(-0.0324581831251064,2.42220359095218,
5.82024159450783));
#57545=CARTESIAN_POINT('Ctrl Pts',(-0.0640106748623482,2.41744366170526,
5.82241406808191));
#57546=CARTESIAN_POINT('Ctrl Pts',(-0.107201007305519,2.40421996711594,
5.82544508123735));
#57547=CARTESIAN_POINT('Ctrl Pts',(-0.119796447190444,2.39948414250967,
5.82633258724156));
#57548=CARTESIAN_POINT('Ctrl Pts',(-0.132741382378724,2.39366895970823,
5.82722330863282));
#57549=CARTESIAN_POINT('Ctrl Pts',(-0.133421031590975,2.39336080318858,
5.82727000871046));
#57550=CARTESIAN_POINT('Ctrl Pts',(-0.134383195337325,2.3929205177089,5.82733602140956));
#57551=CARTESIAN_POINT('Ctrl Pts',(-0.134666591300461,2.39279033808068,
5.82735545252891));
#57552=CARTESIAN_POINT('Ctrl Pts',(-0.135153171401869,2.39256596869687,
5.82738879334182));
#57553=CARTESIAN_POINT('Ctrl Pts',(-0.135356446763625,2.39247197831617,
5.8274027153992));
#57554=CARTESIAN_POINT('Ctrl Pts',(-0.135745706610365,2.3922914997595,5.82742936257808));
#57555=CARTESIAN_POINT('Ctrl Pts',(-0.135931706222862,2.39220504605283,
5.8274420898246));
#57556=CARTESIAN_POINT('Ctrl Pts',(-0.136369942710466,2.39200084218755,
5.82747206389522));
#57557=CARTESIAN_POINT('Ctrl Pts',(-0.136622110292285,2.39188294245079,
5.8274893014111));
#57558=CARTESIAN_POINT('Ctrl Pts',(-0.137367354364829,2.39153332981585,
5.82754021568627));
#57559=CARTESIAN_POINT('Ctrl Pts',(-0.137859999542672,2.39130069168305,
5.82757383553164));
#57560=CARTESIAN_POINT('Ctrl Pts',(-0.14220612006825,2.38923486106908,5.82787012221538));
#57561=CARTESIAN_POINT('Ctrl Pts',(-0.14602364610149,2.38732644241518,5.82812823243293));
#57562=CARTESIAN_POINT('Ctrl Pts',(-0.150605634383394,2.38492093922282,
5.82843676202643));
#57563=CARTESIAN_POINT('Ctrl Pts',(-0.151407132993402,2.38449583271017,
5.82849068343335));
#57564=CARTESIAN_POINT('Ctrl Pts',(-0.152306920463536,2.38401371533267,
5.82855117543504));
#57565=CARTESIAN_POINT('Ctrl Pts',(-0.152406978451895,2.38396003492989,
5.82855790167054));
#57566=CARTESIAN_POINT('Ctrl Pts',(-0.152746443308193,2.38377768332541,
5.82858071973117));
#57567=CARTESIAN_POINT('Ctrl Pts',(-0.152985716365899,2.38364876182674,
5.8285967998963));
#57568=CARTESIAN_POINT('Ctrl Pts',(-0.154159151280926,2.38301459261448,
5.8286756452471));
#57569=CARTESIAN_POINT('Ctrl Pts',(-0.155090984649795,2.38250502665968,
5.82873821192304));
#57570=CARTESIAN_POINT('Ctrl Pts',(-0.16133909018262,2.37904806617456,5.82915754318643));
#57571=CARTESIAN_POINT('Ctrl Pts',(-0.166573837786884,2.37595523042498,
5.82950795214966));
#57572=CARTESIAN_POINT('Ctrl Pts',(-0.182698062355121,2.36580246082704,
5.8305941161091));
#57573=CARTESIAN_POINT('Ctrl Pts',(-0.193250753000684,2.35823187385438,
5.83131544589907));
#57574=CARTESIAN_POINT('Ctrl Pts',(-0.214556289678984,2.34090777790732,
5.83285156777277));
#57575=CARTESIAN_POINT('Ctrl Pts',(-0.225164608822422,2.33102340738084,
5.83366603698555));
#57576=CARTESIAN_POINT('Ctrl Pts',(-0.240957268727839,2.3141840227594,5.83500588071417));
#57577=CARTESIAN_POINT('Ctrl Pts',(-0.246588786853342,2.30767559288076,
5.83551362870343));
#57578=CARTESIAN_POINT('Ctrl Pts',(-0.253554251096458,2.29894223581908,
5.83618701341247));
#57579=CARTESIAN_POINT('Ctrl Pts',(-0.255131541249635,2.29691538160539,
5.83634275524099));
#57580=CARTESIAN_POINT('Ctrl Pts',(-0.257119550015415,2.29429675887561,
5.83654337128035));
#57581=CARTESIAN_POINT('Ctrl Pts',(-0.257552771892464,2.29372212880045,
5.83658735807068));
#57582=CARTESIAN_POINT('Ctrl Pts',(-0.258245785832869,2.29279647411495,
5.83665815889976));
#57583=CARTESIAN_POINT('Ctrl Pts',(-0.258506797096817,2.29244636183457,
5.83668492519471));
#57584=CARTESIAN_POINT('Ctrl Pts',(-0.259001320849695,2.2917802018914,5.83673582966921));
#57585=CARTESIAN_POINT('Ctrl Pts',(-0.259234968672806,2.29146425529176,
5.83675996251163));
#57586=CARTESIAN_POINT('Ctrl Pts',(-0.25976463716848,2.29074527246748,5.83681485772809));
#57587=CARTESIAN_POINT('Ctrl Pts',(-0.260060298267402,2.29034197370139,
5.83684563399438));
#57588=CARTESIAN_POINT('Ctrl Pts',(-0.260933612543216,2.28914488956945,
5.83693693860547));
#57589=CARTESIAN_POINT('Ctrl Pts',(-0.261508574736918,2.28834915638252,
5.83699757084551));
#57590=CARTESIAN_POINT('Ctrl Pts',(-0.265410423022274,2.28289678895216,
5.83741263047262));
#57591=CARTESIAN_POINT('Ctrl Pts',(-0.26861621239145,2.27815513384584,5.83777166713408));
#57592=CARTESIAN_POINT('Ctrl Pts',(-0.272655307532565,2.27182390450379,
5.83824900997595));
#57593=CARTESIAN_POINT('Ctrl Pts',(-0.273604133659034,2.27030898017297,
5.83836307488627));
#57594=CARTESIAN_POINT('Ctrl Pts',(-0.287692186786489,2.2473939743284,5.84008619600989));
#57595=CARTESIAN_POINT('Ctrl Pts',(-0.298296778850963,2.22454078346523,
5.84178554796992));
#57596=CARTESIAN_POINT('Ctrl Pts',(-0.311798248017079,2.18349214116606,
5.84470636232775));
#57597=CARTESIAN_POINT('Ctrl Pts',(-0.315997054805826,2.16584168270886,
5.84592088773631));
#57598=CARTESIAN_POINT('Ctrl Pts',(-0.3187961248048,2.14723035896621,5.84710166407308));
#57599=CARTESIAN_POINT('Ctrl Pts',(-0.318899025334597,2.14653050248745,
5.84714591882361));
#57600=CARTESIAN_POINT('Ctrl Pts',(-0.319043014388169,2.14552827364399,
5.84720907806441));
#57601=CARTESIAN_POINT('Ctrl Pts',(-0.319085978136598,2.1452261792477,5.84722808765476));
#57602=CARTESIAN_POINT('Ctrl Pts',(-0.319159560840155,2.14470346695913,
5.8472609308248));
#57603=CARTESIAN_POINT('Ctrl Pts',(-0.319190380198436,2.1444828778724,5.84727477582552));
#57604=CARTESIAN_POINT('Ctrl Pts',(-0.319249355064044,2.14405754903072,
5.84730144175229));
#57605=CARTESIAN_POINT('Ctrl Pts',(-0.319277542253672,2.14385281460139,
5.84731426448387));
#57606=CARTESIAN_POINT('Ctrl Pts',(-0.319344049930595,2.14336628042638,
5.84734470589697));
#57607=CARTESIAN_POINT('Ctrl Pts',(-0.319382194458872,2.14308445622464,
5.84736231455225));
#57608=CARTESIAN_POINT('Ctrl Pts',(-0.319495469860674,2.14223912343266,
5.84741505934774));
#57609=CARTESIAN_POINT('Ctrl Pts',(-0.319569483301295,2.14167546237286,
5.84745013265542));
#57610=CARTESIAN_POINT('Ctrl Pts',(-0.320275505848948,2.13618614926962,
5.84779078692209));
#57611=CARTESIAN_POINT('Ctrl Pts',(-0.320795117685735,2.13124637773909,
5.84809018271486));
#57612=CARTESIAN_POINT('Ctrl Pts',(-0.321909745541444,2.1176315495383,5.84890057323159));
#57613=CARTESIAN_POINT('Ctrl Pts',(-0.322268267235593,2.10894103123165,
5.84940145333319));
#57614=CARTESIAN_POINT('Ctrl Pts',(-0.322299152829136,2.06848972625361,
5.85169907108656));
#57615=CARTESIAN_POINT('Ctrl Pts',(-0.317630088314807,2.03690627870991,
5.85341581292444));
#57616=CARTESIAN_POINT('Ctrl Pts',(-0.306832050915311,2.00128242650799,
5.85562514977907));
#57617=CARTESIAN_POINT('Ctrl Pts',(-0.305113297466253,1.99609168936067,
5.8559536093269));
#57618=CARTESIAN_POINT('Ctrl Pts',(-0.302964947794916,1.99011736218584,
5.85634017055159));
#57619=CARTESIAN_POINT('Ctrl Pts',(-0.302663063079958,1.98928855565854,
5.85639398950238));
#57620=CARTESIAN_POINT('Ctrl Pts',(-0.302177111718614,1.98797124796551,
5.85647983961475));
#57621=CARTESIAN_POINT('Ctrl Pts',(-0.301995252659374,1.9874819325835,5.85651179706453));
#57622=CARTESIAN_POINT('Ctrl Pts',(-0.301672873057565,1.98662094031251,
5.85656815022161));
#57623=CARTESIAN_POINT('Ctrl Pts',(-0.301532852127135,1.98624907648614,
5.85659252917215));
#57624=CARTESIAN_POINT('Ctrl Pts',(-0.301242591101558,1.98548251097197,
5.8566428671562));
#57625=CARTESIAN_POINT('Ctrl Pts',(-0.301092262221968,1.98508784392319,
5.85666882912773));
#57626=CARTESIAN_POINT('Ctrl Pts',(-0.300706746866104,1.98408167850595,
5.85673513318695));
#57627=CARTESIAN_POINT('Ctrl Pts',(-0.3004704714884,1.98347060189718,5.85677551177803));
#57628=CARTESIAN_POINT('Ctrl Pts',(-0.299508568914852,1.98100521960543,
5.85693886693759));
#57629=CARTESIAN_POINT('Ctrl Pts',(-0.298767638616338,1.97915696774651,
5.85706235775706));
#57630=CARTESIAN_POINT('Ctrl Pts',(-0.293825020448678,1.96715096315554,
5.85787138303386));
#57631=CARTESIAN_POINT('Ctrl Pts',(-0.289123547575297,1.95720806471087,
5.85857387747085));
#57632=CARTESIAN_POINT('Ctrl Pts',(-0.269376055747928,1.92043609502304,
5.86130005562987));
#57633=CARTESIAN_POINT('Ctrl Pts',(-0.251029430650001,1.89557288765733,
5.86343291900502));
#57634=CARTESIAN_POINT('Ctrl Pts',(-0.228344419024603,1.87257431339062,
5.86555761256718));
#57635=CARTESIAN_POINT('Ctrl Pts',(-0.227239172108488,1.871469968172,5.86566000864408));
#57636=CARTESIAN_POINT('Ctrl Pts',(-0.225557483889891,1.86981391538576,
5.86581406949147));
#57637=CARTESIAN_POINT('Ctrl Pts',(-0.224986965718934,1.86925625172414,
5.86586603698184));
#57638=CARTESIAN_POINT('Ctrl Pts',(-0.223645323170776,1.86795454485823,
5.86598753670674));
#57639=CARTESIAN_POINT('Ctrl Pts',(-0.222872542196176,1.86721221290131,
5.86605697687923));
#57640=CARTESIAN_POINT('Ctrl Pts',(-0.218950415745593,1.8634820592006,5.86640661482323));
#57641=CARTESIAN_POINT('Ctrl Pts',(-0.215744444940642,1.86055405630005,
5.86668337796792));
#57642=CARTESIAN_POINT('Ctrl Pts',(-0.212028799627972,1.85729580959307,
5.86699305726811));
#57643=CARTESIAN_POINT('Ctrl Pts',(-0.211576389154281,1.85690132151947,
5.8670305804367));
#57644=CARTESIAN_POINT('Ctrl Pts',(-0.210906440268504,1.85632043347992,
5.86708587341841));
#57645=CARTESIAN_POINT('Ctrl Pts',(-0.210689754539812,1.85613305878076,
5.86710371519191));
#57646=CARTESIAN_POINT('Ctrl Pts',(-0.210305837499724,1.85580196774247,
5.86713525202897));
#57647=CARTESIAN_POINT('Ctrl Pts',(-0.210138708336134,1.85565813394977,
5.86714895586355));
#57648=CARTESIAN_POINT('Ctrl Pts',(-0.209789110889789,1.85535788928486,
5.86717756894567));
#57649=CARTESIAN_POINT('Ctrl Pts',(-0.209606615653896,1.85520151132388,
5.86719247574261));
#57650=CARTESIAN_POINT('Ctrl Pts',(-0.209128514739989,1.85479275903371,
5.86723145149828));
#57651=CARTESIAN_POINT('Ctrl Pts',(-0.208832625994621,1.85454071412225,
5.86725549600962));
#57652=CARTESIAN_POINT('Ctrl Pts',(-0.207535015911361,1.85343942437933,
5.86736060971929));
#57653=CARTESIAN_POINT('Ctrl Pts',(-0.206528546636458,1.85259575621504,
5.86744127339747));
#57654=CARTESIAN_POINT('Ctrl Pts',(-0.199034289112397,1.84639133344262,
5.86803576079662));
#57655=CARTESIAN_POINT('Ctrl Pts',(-0.192343265210407,1.84127988152837,
5.86853268383402));
#57656=CARTESIAN_POINT('Ctrl Pts',(-0.172410707253764,1.82725416838901,
5.86994254398031));
#57657=CARTESIAN_POINT('Ctrl Pts',(-0.158697585376564,1.81905359487004,
5.87082832345679));
#57658=CARTESIAN_POINT('Ctrl Pts',(-0.122365344702224,1.80083907820688,
5.87310132157554));
#57659=CARTESIAN_POINT('Ctrl Pts',(-0.0991038509970655,1.79234969146709,
5.87449610614019));
#57660=CARTESIAN_POINT('Ctrl Pts',(-0.0735756788442157,1.78623215193834,
5.87608759994219));
#57661=CARTESIAN_POINT('Ctrl Pts',(-0.0720455067440576,1.78587727268379,
5.87618318314318));
#57662=CARTESIAN_POINT('Ctrl Pts',(-0.0699715425688329,1.78541222755775,
5.87631300857094));
#57663=CARTESIAN_POINT('Ctrl Pts',(-0.0694299531255458,1.7852922547147,
5.87634693602148));
#57664=CARTESIAN_POINT('Ctrl Pts',(-0.0685136230434926,1.78509174987352,
5.87640438235838));
#57665=CARTESIAN_POINT('Ctrl Pts',(-0.0681390422193349,1.7850104867402,
5.87642787777476));
#57666=CARTESIAN_POINT('Ctrl Pts',(-0.0674188622620702,1.78485559262965,
5.87647307470548));
#57667=CARTESIAN_POINT('Ctrl Pts',(-0.0670732850402093,1.78478186137555,
5.87649477297386));
#57668=CARTESIAN_POINT('Ctrl Pts',(-0.0662599227253543,1.78460972308465,
5.87654586799627));
#57669=CARTESIAN_POINT('Ctrl Pts',(-0.0657920394986536,1.78451178838659,
5.87657527981746));
#57670=CARTESIAN_POINT('Ctrl Pts',(-0.0644345674962926,1.7842308010358,
5.87666067032801));
#57671=CARTESIAN_POINT('Ctrl Pts',(-0.0635444260407747,1.78405046859499,
5.87671673582982));
#57672=CARTESIAN_POINT('Ctrl Pts',(-0.0573281479795498,1.78281845441331,
5.8771087841462));
#57673=CARTESIAN_POINT('Ctrl Pts',(-0.0519772175502979,1.78189779555488,
5.87744892169057));
#57674=CARTESIAN_POINT('Ctrl Pts',(-0.0353289799955228,1.7794646311759,
5.87851628863267));
#57675=CARTESIAN_POINT('Ctrl Pts',(-0.0239738266270041,1.77841600389988,
5.87925754506346));
#57676=CARTESIAN_POINT('Ctrl Pts',(0.018012418676957,1.77677477758248,5.88204191822955));
#57677=CARTESIAN_POINT('Ctrl Pts',(0.0486242682877354,1.77994606354785,
5.88417367464612));
#57678=CARTESIAN_POINT('Ctrl Pts',(0.0818523072166536,1.78827162418953,
5.88637615380775));
#57679=CARTESIAN_POINT('Ctrl Pts',(0.0853621925889448,1.78921441584519,
5.8866071062415));
#57680=CARTESIAN_POINT('Ctrl Pts',(0.0894103936000768,1.79037556570785,
5.88687091148799));
#57681=CARTESIAN_POINT('Ctrl Pts',(0.089964805825962,1.79053620160119,5.88690698411782));
#57682=CARTESIAN_POINT('Ctrl Pts',(0.0907882267240392,1.79077718013067,
5.88696047294389));
#57683=CARTESIAN_POINT('Ctrl Pts',(0.0910575629599759,1.7908563850427,5.88697795501326));
#57684=CARTESIAN_POINT('Ctrl Pts',(0.0915369200238509,1.79099803252306,
5.88700904406568));
#57685=CARTESIAN_POINT('Ctrl Pts',(0.0917469805518384,1.7910603372942,5.88702265910571));
#57686=CARTESIAN_POINT('Ctrl Pts',(0.0921926135113602,1.79119300836335,
5.88705152439189));
#57687=CARTESIAN_POINT('Ctrl Pts',(0.0924281683354561,1.7912634298162,5.88706677130715));
#57688=CARTESIAN_POINT('Ctrl Pts',(0.0930595400778105,1.79145297200373,
5.88710761003534));
#57689=CARTESIAN_POINT('Ctrl Pts',(0.0934552104642061,1.7915725853196,5.88713317295116));
#57690=CARTESIAN_POINT('Ctrl Pts',(0.0953433396208922,1.79214734401817,
5.88725501983132));
#57691=CARTESIAN_POINT('Ctrl Pts',(0.0968327427997494,1.79261257286985,
5.88735072149524));
#57692=CARTESIAN_POINT('Ctrl Pts',(0.109116192116552,1.79654756305845,5.88813701557171));
#57693=CARTESIAN_POINT('Ctrl Pts',(0.119724892893234,1.80057432513179,5.88879712845626));
#57694=CARTESIAN_POINT('Ctrl Pts',(0.154338764754285,1.81584756205429,5.89095481441185));
#57695=CARTESIAN_POINT('Ctrl Pts',(0.177165699417369,1.82949036538013,5.89239272813096));
#57696=CARTESIAN_POINT('Ctrl Pts',(0.207131200685941,1.85283629229838,5.89458779526385));
#57697=CARTESIAN_POINT('Ctrl Pts',(0.215811174433609,1.8603779557243,5.89526624350565));
#57698=CARTESIAN_POINT('Ctrl Pts',(0.224933673498165,1.86920254664458,5.89603777573693));
#57699=CARTESIAN_POINT('Ctrl Pts',(0.225793362954381,1.87004352774241,5.89611108865486));
#57700=CARTESIAN_POINT('Ctrl Pts',(0.226991266162491,1.8712285563584,5.89621410497054));
#57701=CARTESIAN_POINT('Ctrl Pts',(0.227333452548888,1.87156858865708,5.89624363146771));
#57702=CARTESIAN_POINT('Ctrl Pts',(0.227958460820005,1.87219245772562,5.89629774513913));
#57703=CARTESIAN_POINT('Ctrl Pts',(0.228241519733373,1.87247605654785,5.89632232174967));
#57704=CARTESIAN_POINT('Ctrl Pts',(0.228806972048985,1.87304470447661,5.89637155628299));
#57705=CARTESIAN_POINT('Ctrl Pts',(0.229089363454994,1.87332975454683,5.89639621422717));
#57706=CARTESIAN_POINT('Ctrl Pts',(0.229776626207071,1.87402608392546,5.89645639592029));
#57707=CARTESIAN_POINT('Ctrl Pts',(0.230180925434693,1.87443792371881,5.89649194469645));
#57708=CARTESIAN_POINT('Ctrl Pts',(0.231041927645179,1.87531970998233,5.89656796252592));
#57709=CARTESIAN_POINT('Ctrl Pts',(0.231498307273205,1.87578996728089,5.8966084454966));
#57710=CARTESIAN_POINT('Ctrl Pts',(0.232758231222888,1.87709615104065,5.89672073440696));
#57711=CARTESIAN_POINT('Ctrl Pts',(0.233558697347007,1.87793502095114,5.89679267348119));
#57712=CARTESIAN_POINT('Ctrl Pts',(0.240359800043001,1.88513986991649,5.89740907570609));
#57713=CARTESIAN_POINT('Ctrl Pts',(0.246102940801926,1.89174288096354,5.89796443249822));
#57714=CARTESIAN_POINT('Ctrl Pts',(0.256582180659106,1.90483066873755,5.89904868377395));
#57715=CARTESIAN_POINT('Ctrl Pts',(0.26135864552966,1.91127499845539,5.8995755344524));
#57716=CARTESIAN_POINT('Ctrl Pts',(0.283874691551311,1.94414959819888,5.90222464073648));
#57717=CARTESIAN_POINT('Ctrl Pts',(0.297869860329996,1.9729264630263,5.90444531093781));
#57718=CARTESIAN_POINT('Ctrl Pts',(0.307885441082755,2.00476279266951,5.90655707004294));
#57719=CARTESIAN_POINT('Ctrl Pts',(0.308339222323259,2.00624236193462,5.90665442845457));
#57720=CARTESIAN_POINT('Ctrl Pts',(0.308904484862313,2.00813391895601,5.90677784722743));
#57721=CARTESIAN_POINT('Ctrl Pts',(0.309025820114343,2.00854290556724,5.9068044700906));
#57722=CARTESIAN_POINT('Ctrl Pts',(0.309217339881436,2.00919319687889,5.90684670022106));
#57723=CARTESIAN_POINT('Ctrl Pts',(0.309288054330192,2.00943434300957,5.90686233842063));
#57724=CARTESIAN_POINT('Ctrl Pts',(0.309419673174766,2.00988513365147,5.90689153070262));
#57725=CARTESIAN_POINT('Ctrl Pts',(0.30948064615236,2.01009475575843,5.90690508870986));
#57726=CARTESIAN_POINT('Ctrl Pts',(0.30961721589297,2.01056606103152,5.90693553457582));
#57727=CARTESIAN_POINT('Ctrl Pts',(0.309692693751389,2.01082777755908,5.90695241537429));
#57728=CARTESIAN_POINT('Ctrl Pts',(0.309915706927583,2.0116047654323,5.90700245555047));
#57729=CARTESIAN_POINT('Ctrl Pts',(0.310062289654226,2.01212031270614,5.90703555938568));
#57730=CARTESIAN_POINT('Ctrl Pts',(0.311233043082511,2.01627737444864,5.90730171069016));
#57731=CARTESIAN_POINT('Ctrl Pts',(0.312194366312396,2.01993648878598,5.90753117559));
#57732=CARTESIAN_POINT('Ctrl Pts',(0.315448704243452,2.03327500415194,5.90835310477475));
#57733=CARTESIAN_POINT('Ctrl Pts',(0.317357915125968,2.04304300496929,5.908927525144));
#57734=CARTESIAN_POINT('Ctrl Pts',(0.323474489300776,2.08443147440125,5.91130455419184));
#57735=CARTESIAN_POINT('Ctrl Pts',(0.323428723733039,2.11649360942277,5.91302786343218));
#57736=CARTESIAN_POINT('Ctrl Pts',(0.317868565371912,2.15338648361829,5.91524277950933));
#57737=CARTESIAN_POINT('Ctrl Pts',(0.316925993521362,2.15872351131321,5.91556838657768));
#57738=CARTESIAN_POINT('Ctrl Pts',(0.315674596854227,2.16489605684914,5.91595186670328));
#57739=CARTESIAN_POINT('Ctrl Pts',(0.315496301924824,2.1657573778473,5.9160055343774));
#57740=CARTESIAN_POINT('Ctrl Pts',(0.315206728141049,2.16712798151037,5.91609118821949));
#57741=CARTESIAN_POINT('Ctrl Pts',(0.315097734921821,2.16763774692533,5.91612310120431));
#57742=CARTESIAN_POINT('Ctrl Pts',(0.314905188607795,2.16852772691989,5.91617891548017));
#57743=CARTESIAN_POINT('Ctrl Pts',(0.314822182301013,2.16890805974657,5.91620279920292));
#57744=CARTESIAN_POINT('Ctrl Pts',(0.314656638070723,2.16966003642676,5.9162500837104));
#57745=CARTESIAN_POINT('Ctrl Pts',(0.314574130317158,2.17003168632963,5.91627348349224));
#57746=CARTESIAN_POINT('Ctrl Pts',(0.314359788162189,2.17098915250499,5.91633384601408));
#57747=CARTESIAN_POINT('Ctrl Pts',(0.314226975117556,2.17157474615695,5.91637084013599));
#57748=CARTESIAN_POINT('Ctrl Pts',(0.313938373811275,2.1728309485022,5.91645036356686));
#57749=CARTESIAN_POINT('Ctrl Pts',(0.313782071901832,2.173501435035,5.91649290926483));
#57750=CARTESIAN_POINT('Ctrl Pts',(0.313337678769559,2.17538049034476,5.91661243003385));
#57751=CARTESIAN_POINT('Ctrl Pts',(0.31304474765444,2.17658789171759,5.91668956070578));
#57752=CARTESIAN_POINT('Ctrl Pts',(0.312074267648776,2.18048940537081,5.91693988521061));
#57753=CARTESIAN_POINT('Ctrl Pts',(0.31136887834961,2.18317640123909,5.9171139725925));
#57754=CARTESIAN_POINT('Ctrl Pts',(0.308434964303101,2.19379162805344,5.91780858288632));
#57755=CARTESIAN_POINT('Ctrl Pts',(0.305937793093243,2.20164174404664,5.91833763227893));
#57756=CARTESIAN_POINT('Ctrl Pts',(0.292873761551843,2.23784591173306,5.92085023836029));
#57757=CARTESIAN_POINT('Ctrl Pts',(0.278650657881394,2.26471161897201,5.92294598742858));
#57758=CARTESIAN_POINT('Ctrl Pts',(0.259556998880454,2.29104062154919,5.92509110524389));
#57759=CARTESIAN_POINT('Ctrl Pts',(0.258201452457649,2.29286877709352,5.92524047255357));
#57760=CARTESIAN_POINT('Ctrl Pts',(0.256403751806235,2.29524031783795,5.92543463936345));
#57761=CARTESIAN_POINT('Ctrl Pts',(0.255979059670027,2.29579679945235,5.92548022991581));
#57762=CARTESIAN_POINT('Ctrl Pts',(0.255339445515972,2.29662925909837,5.92554846927776));
#57763=CARTESIAN_POINT('Ctrl Pts',(0.255125884345274,2.29690627493564,5.92557118364002));
#57764=CARTESIAN_POINT('Ctrl Pts',(0.251828345878157,2.30116922834889,5.92592082487133));
#57765=CARTESIAN_POINT('Ctrl Pts',(0.248651518977412,2.30508291828741,5.92624308811138));
#57766=CARTESIAN_POINT('Ctrl Pts',(0.244973027077439,2.30940342284844,5.92659877879941));
#57767=CARTESIAN_POINT('Ctrl Pts',(0.244560640765067,2.30988489822024,5.92663841571429));
#57768=CARTESIAN_POINT('Ctrl Pts',(0.243958454311387,2.3105837873148,5.92669594528991));
#57769=CARTESIAN_POINT('Ctrl Pts',(0.243769781844406,2.31080216405658,5.92671392032301));
#57770=CARTESIAN_POINT('Ctrl Pts',(0.243436220036271,2.31118719460483,5.92674561107171));
#57771=CARTESIAN_POINT('Ctrl Pts',(0.243291452535744,2.31135395315641,5.92675933584449));
#57772=CARTESIAN_POINT('Ctrl Pts',(0.242989423724844,2.31170114044945,5.92678790897882));
#57773=CARTESIAN_POINT('Ctrl Pts',(0.242832133132022,2.31188154244571,5.92680275505514));
#57774=CARTESIAN_POINT('Ctrl Pts',(0.24242178418731,2.31235112865637,5.92684139777665));
#57775=CARTESIAN_POINT('Ctrl Pts',(0.242168408380421,2.31264003686119,5.92686517073903));
#57776=CARTESIAN_POINT('Ctrl Pts',(0.241073367799878,2.31388414565622,5.92696753955987));
#57777=CARTESIAN_POINT('Ctrl Pts',(0.240226548890328,2.31483482436609,5.9270457556523));
#57778=CARTESIAN_POINT('Ctrl Pts',(0.234023987108327,2.32171557960394,5.92761201688977));
#57779=CARTESIAN_POINT('Ctrl Pts',(0.228454476739092,2.3274502157832,5.92808481359217));
#57780=CARTESIAN_POINT('Ctrl Pts',(0.210101142790094,2.34499249367169,5.9295569879299));
#57781=CARTESIAN_POINT('Ctrl Pts',(0.196571768656621,2.35597546165371,5.93051999921938));
#57782=CARTESIAN_POINT('Ctrl Pts',(0.173825972315789,2.371568235032,5.93206343206742));
#57783=CARTESIAN_POINT('Ctrl Pts',(0.165163190686127,2.37692215798706,5.93263559221807));
#57784=CARTESIAN_POINT('Ctrl Pts',(0.144015181940963,2.38864664301284,5.93401997305151));
#57785=CARTESIAN_POINT('Ctrl Pts',(0.131340469967132,2.39463004051628,5.93484056814862));
#57786=CARTESIAN_POINT('Ctrl Pts',(0.117173716331366,2.40022160003568,5.93576604321558));
#57787=CARTESIAN_POINT('Ctrl Pts',(0.116026893538369,2.4006666739717,5.93584101174342));
#57788=CARTESIAN_POINT('Ctrl Pts',(0.114410437430141,2.40128338387601,5.93594675986202));
#57789=CARTESIAN_POINT('Ctrl Pts',(0.113942899939969,2.4014605134036,5.9359773553303));
#57790=CARTESIAN_POINT('Ctrl Pts',(0.113129961134235,2.40176633904944,5.93603057058695));
#57791=CARTESIAN_POINT('Ctrl Pts',(0.112784746772811,2.4018955322344,5.93605317370996));
#57792=CARTESIAN_POINT('Ctrl Pts',(0.112072584229157,2.40216066027659,5.93609981418559));
#57793=CARTESIAN_POINT('Ctrl Pts',(0.111705608700279,2.40229651955883,5.93612385401888));
#57794=CARTESIAN_POINT('Ctrl Pts',(0.110873656708889,2.4026027976063,5.93617836780097));
#57795=CARTESIAN_POINT('Ctrl Pts',(0.11040853387257,2.40277281336821,5.93620885512825));
#57796=CARTESIAN_POINT('Ctrl Pts',(0.109408374517544,2.40313578922414,5.93627443482322));
#57797=CARTESIAN_POINT('Ctrl Pts',(0.108873216004177,2.40332840611025,5.93630953851775));
#57798=CARTESIAN_POINT('Ctrl Pts',(0.107444924188173,2.40383821713495,5.93640326526189));
#57799=CARTESIAN_POINT('Ctrl Pts',(0.106550901832313,2.40415288789266,5.93646197197736));
#57800=CARTESIAN_POINT('Ctrl Pts',(0.103835164873879,2.4050953078456,5.93664042954428));
#57801=CARTESIAN_POINT('Ctrl Pts',(0.102009221814378,2.40571065853003,5.93676058897178));
#57802=CARTESIAN_POINT('Ctrl Pts',(0.0954059974970812,2.40787022905597,
5.93719579981648));
#57803=CARTESIAN_POINT('Ctrl Pts',(0.0905985056734264,2.4093190723698,5.93751393583382));
#57804=CARTESIAN_POINT('Ctrl Pts',(0.0739521978342939,2.41391444836124,
5.93862030998128));
#57805=CARTESIAN_POINT('Ctrl Pts',(0.0619700678904657,2.41649780896726,
5.93942544001448));
#57806=CARTESIAN_POINT('Ctrl Pts',(0.0248501533739732,2.42231204160706,
5.94193624169357));
#57807=CARTESIAN_POINT('Ctrl Pts',(-0.000544646142155328,2.42326811623638,
5.94368350304947));
#57808=CARTESIAN_POINT('Ctrl Pts',(-0.0271344272948742,2.42113349204407,
5.94542052101855));
#57809=CARTESIAN_POINT('Ctrl Pts',(-0.0284789599432046,2.42101704910268,
5.94550808000024));
#57810=CARTESIAN_POINT('Ctrl Pts',(-0.0342047096750918,2.42048491531657,
5.94587967553323));
#57811=CARTESIAN_POINT('Ctrl Pts',(-0.0385781520544983,2.41998792802032,
5.94616031979644));
#57812=CARTESIAN_POINT('Ctrl Pts',(-0.0435451644099679,2.41932016339867,
5.94647438325466));
#57813=CARTESIAN_POINT('Ctrl Pts',(-0.0441498007895482,2.41923712691536,
5.94651253518693));
#57814=CARTESIAN_POINT('Ctrl Pts',(-0.0450355919893432,2.4191129138967,
5.94656830803236));
#57815=CARTESIAN_POINT('Ctrl Pts',(-0.0453169294817579,2.41907308295328,
5.94658600442564));
#57816=CARTESIAN_POINT('Ctrl Pts',(-0.0458161543058124,2.41900173055541,
5.9466173742618));
#57817=CARTESIAN_POINT('Ctrl Pts',(-0.0460340621991443,2.4189703578882,
5.94663105616374));
#57818=CARTESIAN_POINT('Ctrl Pts',(-0.0464909019615065,2.41890410778745,
5.94665971721381));
#57819=CARTESIAN_POINT('Ctrl Pts',(-0.0467298262391742,2.418869185199,5.94667469372496));
#57820=CARTESIAN_POINT('Ctrl Pts',(-0.0473582496228737,2.4187766096347,
5.94671405147865));
#57821=CARTESIAN_POINT('Ctrl Pts',(-0.0477476842309654,2.41871851109095,
5.94673840738548));
#57822=CARTESIAN_POINT('Ctrl Pts',(-0.0494824750020427,2.418456452074,5.94684675594786));
#57823=CARTESIAN_POINT('Ctrl Pts',(-0.050826663443067,2.41824468202518,
5.94693031156555));
#57824=CARTESIAN_POINT('Ctrl Pts',(-0.0609843379672103,2.41657839232637,
5.94755898448899));
#57825=CARTESIAN_POINT('Ctrl Pts',(-0.0697361589562724,2.41476637080739,
5.9480850830531));
#57826=CARTESIAN_POINT('Ctrl Pts',(-0.0938645701930585,2.40871466333967,
5.9495200011912));
#57827=CARTESIAN_POINT('Ctrl Pts',(-0.10901879296144,2.40369435939589,5.95040413247739));
#57828=CARTESIAN_POINT('Ctrl Pts',(-0.131595136689005,2.39430642033264,
5.95177210032367));
#57829=CARTESIAN_POINT('Ctrl Pts',(-0.139317700866998,2.39073032217292,
5.95224955800796));
#57830=CARTESIAN_POINT('Ctrl Pts',(-0.161162083675026,2.3795444138845,5.95364541554557));
#57831=CARTESIAN_POINT('Ctrl Pts',(-0.174867317973763,2.37118187371701,
5.95457930833665));
#57832=CARTESIAN_POINT('Ctrl Pts',(-0.188917100596259,2.36109978106376,
5.95562988868433));
#57833=CARTESIAN_POINT('Ctrl Pts',(-0.189937538679195,2.36035840278169,
5.95570674514527));
#57834=CARTESIAN_POINT('Ctrl Pts',(-0.191360686204609,2.35931162486902,
5.95581472010645));
#57835=CARTESIAN_POINT('Ctrl Pts',(-0.19176707857674,2.35901123254883,5.95584564396108));
#57836=CARTESIAN_POINT('Ctrl Pts',(-0.19246976678205,2.35848926744706,5.95589927206847));
#57837=CARTESIAN_POINT('Ctrl Pts',(-0.192766391550058,2.35826813740253,
5.95592195901416));
#57838=CARTESIAN_POINT('Ctrl Pts',(-0.193375195427103,2.35781264863979,
5.95596862370062));
#57839=CARTESIAN_POINT('Ctrl Pts',(-0.193687330747948,2.3575782326028,5.95599260366396));
#57840=CARTESIAN_POINT('Ctrl Pts',(-0.194413626711849,2.35703071205162,
5.95604853016788));
#57841=CARTESIAN_POINT('Ctrl Pts',(-0.194827457271954,2.35671717331907,
5.95608049373833));
#57842=CARTESIAN_POINT('Ctrl Pts',(-0.195699183691634,2.35605338792739,
5.95614803171647));
#57843=CARTESIAN_POINT('Ctrl Pts',(-0.196156900599818,2.35570291024317,
5.95618361518185));
#57844=CARTESIAN_POINT('Ctrl Pts',(-0.197379406211927,2.35476161327594,
5.95627898108646));
#57845=CARTESIAN_POINT('Ctrl Pts',(-0.198142477397575,2.35416858227091,
5.95633885109385));
#57846=CARTESIAN_POINT('Ctrl Pts',(-0.200459525043095,2.35235108204038,
5.95652170360012));
#57847=CARTESIAN_POINT('Ctrl Pts',(-0.202004881376879,2.35111574503841,
5.95664511866774));
#57848=CARTESIAN_POINT('Ctrl Pts',(-0.207573036532313,2.34657997783755,
5.95709520444008));
#57849=CARTESIAN_POINT('Ctrl Pts',(-0.211526951680161,2.34319661724007,
5.95742519671695));
#57850=CARTESIAN_POINT('Ctrl Pts',(-0.220319556615638,2.33529611781992,
5.95818340135166));
#57851=CARTESIAN_POINT('Ctrl Pts',(-0.225104365213146,2.33072274578182,
5.95861375920701));
#57852=CARTESIAN_POINT('Ctrl Pts',(-0.241371378174606,2.31418660010616,
5.9601398951498));
#57853=CARTESIAN_POINT('Ctrl Pts',(-0.252067788547602,2.30148892782995,
5.96126140185053));
#57854=CARTESIAN_POINT('Ctrl Pts',(-0.272876410845914,2.27252257399,5.96367445293564));
#57855=CARTESIAN_POINT('Ctrl Pts',(-0.282615679658572,2.25605811756274,
5.96496147068477));
#57856=CARTESIAN_POINT('Ctrl Pts',(-0.291331894598258,2.23779768631007,
5.96623694079903));
#57857=CARTESIAN_POINT('Ctrl Pts',(-0.291817507543199,2.23676628804718,
5.96630848695744));
#57858=CARTESIAN_POINT('Ctrl Pts',(-0.29245894457534,2.2353849623668,5.96640362463533));
#57859=CARTESIAN_POINT('Ctrl Pts',(-0.292619624844501,2.23503731875548,
5.96642751080922));
#57860=CARTESIAN_POINT('Ctrl Pts',(-0.292869620597625,2.23449389302969,
5.96646475824669));
#57861=CARTESIAN_POINT('Ctrl Pts',(-0.292959359670112,2.23429830793281,
5.96647814570673));
#57862=CARTESIAN_POINT('Ctrl Pts',(-0.293130906524664,2.23392343372899,
5.96650376991083));
#57863=CARTESIAN_POINT('Ctrl Pts',(-0.29321274516041,2.23374416076038,5.96651600849295));
#57864=CARTESIAN_POINT('Ctrl Pts',(-0.293405776274511,2.2333202845306,5.96654490919947));
#57865=CARTESIAN_POINT('Ctrl Pts',(-0.293516827189713,2.23307561751243,
5.96656156247198));
#57866=CARTESIAN_POINT('Ctrl Pts',(-0.293841166598091,2.23235865288243,
5.96661027980416));
#57867=CARTESIAN_POINT('Ctrl Pts',(-0.29405362331227,2.23188597653412,5.96664229265333));
#57868=CARTESIAN_POINT('Ctrl Pts',(-0.295609461174895,2.22840208009805,
5.96687748651993));
#57869=CARTESIAN_POINT('Ctrl Pts',(-0.296907761050969,2.22537077485921,
5.96707795654666));
#57870=CARTESIAN_POINT('Ctrl Pts',(-0.301031421160604,2.21531920085007,
5.96773074998102));
#57871=CARTESIAN_POINT('Ctrl Pts',(-0.30365624534299,2.2082189302946,5.96817291655553));
#57872=CARTESIAN_POINT('Ctrl Pts',(-0.316779669352195,2.1684678262965,5.97057872956467));
#57873=CARTESIAN_POINT('Ctrl Pts',(-0.32226369604783,2.13439903461908,5.9724110985191));
#57874=CARTESIAN_POINT('Ctrl Pts',(-0.322274982545603,2.10010606710754,
5.97444230798123));
#57875=CARTESIAN_POINT('',(-0.322274999303774,2.10002118378279,6.22472265507673));
#57876=CARTESIAN_POINT('Ctrl Pts',(-0.322274982642247,2.10010577305737,
5.97444232539814));
#57877=CARTESIAN_POINT('Ctrl Pts',(-0.322276324034467,2.09601874782303,
5.9746844044184));
#57878=CARTESIAN_POINT('Ctrl Pts',(-0.32219991927052,2.09193217407,5.97492868233561));
#57879=CARTESIAN_POINT('Ctrl Pts',(-0.321968486419485,2.08579873707773,
5.97529915987549));
#57880=CARTESIAN_POINT('Ctrl Pts',(-0.321871590513878,2.08375004504883,
5.97542355104126));
#57881=CARTESIAN_POINT('Ctrl Pts',(-0.321720677281781,2.08109629533517,
5.97558555916811));
#57882=CARTESIAN_POINT('Ctrl Pts',(-0.321684493673447,2.08049023929307,
5.97562261760034));
#57883=CARTESIAN_POINT('Ctrl Pts',(-0.321619995793277,2.0794589296274,5.9756857815322));
#57884=CARTESIAN_POINT('Ctrl Pts',(-0.321592550045636,2.07903362171208,
5.9757118597827));
#57885=CARTESIAN_POINT('Ctrl Pts',(-0.321539924274289,2.07824253809059,
5.97576042174362));
#57886=CARTESIAN_POINT('Ctrl Pts',(-0.321514963530535,2.07787674808591,
5.97578289854142));
#57887=CARTESIAN_POINT('Ctrl Pts',(-0.32146332831164,2.07713860159609,5.97582830072277));
#57888=CARTESIAN_POINT('Ctrl Pts',(-0.321436630956802,2.07676624732297,
5.97585122679096));
#57889=CARTESIAN_POINT('Ctrl Pts',(-0.321373136224455,2.07590173211162,
5.97590450967321));
#57890=CARTESIAN_POINT('Ctrl Pts',(-0.321335855217238,2.07540960859504,
5.97593488163286));
#57891=CARTESIAN_POINT('Ctrl Pts',(-0.321237566908938,2.0741505683697,5.97601269003489));
#57892=CARTESIAN_POINT('Ctrl Pts',(-0.321174943834661,2.07338378416154,
5.97606017715736));
#57893=CARTESIAN_POINT('Ctrl Pts',(-0.320801147318777,2.06900038282241,
5.97633222167329));
#57894=CARTESIAN_POINT('Ctrl Pts',(-0.320431643059886,2.06538912342834,
5.97655860628214));
#57895=CARTESIAN_POINT('Ctrl Pts',(-0.319933724434097,2.06121969950897,
5.97682271708887));
#57896=CARTESIAN_POINT('Ctrl Pts',(-0.319864719108417,2.06065459112596,
5.97685857187485));
#57897=CARTESIAN_POINT('Ctrl Pts',(-0.319748312806751,2.05972184856381,
5.97691784870096));
#57898=CARTESIAN_POINT('Ctrl Pts',(-0.319701774090159,2.05935410638641,
5.97694124391604));
#57899=CARTESIAN_POINT('Ctrl Pts',(-0.31937029412024,2.05677059219032,5.97710577797865));
#57900=CARTESIAN_POINT('Ctrl Pts',(-0.319062960076768,2.05455779962926,
5.97724760611613));
#57901=CARTESIAN_POINT('Ctrl Pts',(-0.313541684992787,2.01762700297687,
5.97962996163393));
#57902=CARTESIAN_POINT('Ctrl Pts',(-0.3027114338086,1.98398948036205,5.9820637321409));
#57903=CARTESIAN_POINT('Ctrl Pts',(-0.283770011806913,1.94710680351185,
5.98480784499535));
#57904=CARTESIAN_POINT('Ctrl Pts',(-0.280692524035074,1.94152770761205,
5.98522406235335));
#57905=CARTESIAN_POINT('Ctrl Pts',(-0.275908613697531,1.93343226725783,
5.9858258589934));
#57906=CARTESIAN_POINT('Ctrl Pts',(-0.274328902530941,1.93084318642345,
5.98601798574393));
#57907=CARTESIAN_POINT('Ctrl Pts',(-0.272442611369619,1.92784757838102,
5.98623953002309));
#57908=CARTESIAN_POINT('Ctrl Pts',(-0.272171398524418,1.92741911289836,
5.98627119964388));
#57909=CARTESIAN_POINT('Ctrl Pts',(-0.271756191037942,1.92676657598484,
5.98631940142748));
#57910=CARTESIAN_POINT('Ctrl Pts',(-0.271612929613146,1.92654204246659,
5.9863359819238));
#57911=CARTESIAN_POINT('Ctrl Pts',(-0.271363315196208,1.9261518894814,5.98636478268045));
#57912=CARTESIAN_POINT('Ctrl Pts',(-0.271257089111903,1.92598619028251,
5.98637701136242));
#57913=CARTESIAN_POINT('Ctrl Pts',(-0.271016593562798,1.92561180310387,
5.98640463428518));
#57914=CARTESIAN_POINT('Ctrl Pts',(-0.270882235106954,1.92540317326044,
5.98642002244607));
#57915=CARTESIAN_POINT('Ctrl Pts',(-0.270517860199896,1.92483881026177,
5.98646163615303));
#57916=CARTESIAN_POINT('Ctrl Pts',(-0.270287382090383,1.92448337353619,
5.98648783086211));
#57917=CARTESIAN_POINT('Ctrl Pts',(-0.269252307263618,1.92289398468269,
5.98660490806167));
#57918=CARTESIAN_POINT('Ctrl Pts',(-0.268439940157357,1.92166507815052,
5.9866952790142));
#57919=CARTESIAN_POINT('Ctrl Pts',(-0.25113644077913,1.89587540757211,5.98858953312115));
#57920=CARTESIAN_POINT('Ctrl Pts',(-0.231346571480411,1.87369093856763,
5.9901848308886));
#57921=CARTESIAN_POINT('Ctrl Pts',(-0.199261171030816,1.84639972738477,
5.99255832918909));
#57922=CARTESIAN_POINT('Ctrl Pts',(-0.189254396342781,1.83884708486307,
5.9932735083687));
#57923=CARTESIAN_POINT('Ctrl Pts',(-0.174621996600138,1.82908678676636,
5.99430748533453));
#57924=CARTESIAN_POINT('Ctrl Pts',(-0.170344497993436,1.82637697707623,
5.99460835091578));
#57925=CARTESIAN_POINT('Ctrl Pts',(-0.164343236446771,1.82277042811039,
5.99502950813506));
#57926=CARTESIAN_POINT('Ctrl Pts',(-0.162672414698106,1.82178673622255,
5.99514666159192));
#57927=CARTESIAN_POINT('Ctrl Pts',(-0.160168014144757,1.82034254979135,
5.99532215834626));
#57928=CARTESIAN_POINT('Ctrl Pts',(-0.159341085644919,1.81987056454653,
5.99538008869582));
#57929=CARTESIAN_POINT('Ctrl Pts',(-0.15801529474266,1.81912161384015,5.99547294491671));
#57930=CARTESIAN_POINT('Ctrl Pts',(-0.157517763060367,1.81884229425774,
5.99550778631902));
#57931=CARTESIAN_POINT('Ctrl Pts',(-0.15656908219843,1.81831300323682,5.99557421295439));
#57932=CARTESIAN_POINT('Ctrl Pts',(-0.156118069137033,1.81806279044802,
5.99560578943013));
#57933=CARTESIAN_POINT('Ctrl Pts',(-0.155325380996444,1.81762550862425,
5.99566128211725));
#57934=CARTESIAN_POINT('Ctrl Pts',(-0.154983962907371,1.81743797388755,
5.99568518162244));
#57935=CARTESIAN_POINT('Ctrl Pts',(-0.154316466633623,1.81707290409603,
5.9957319038689));
#57936=CARTESIAN_POINT('Ctrl Pts',(-0.153990419873345,1.81689531254961,
5.99575472454909));
#57937=CARTESIAN_POINT('Ctrl Pts',(-0.153215461963583,1.81647494237105,
5.9958089625517));
#57938=CARTESIAN_POINT('Ctrl Pts',(-0.152766280586222,1.81623266643378,
5.99584039770692));
#57939=CARTESIAN_POINT('Ctrl Pts',(-0.151179197877049,1.81538149862372,
5.99595146014532));
#57940=CARTESIAN_POINT('Ctrl Pts',(-0.15003822793166,1.81477838216951,5.99603129198993));
#57941=CARTESIAN_POINT('Ctrl Pts',(-0.132088242759602,1.80542753419985,
5.99728712469225));
#57942=CARTESIAN_POINT('Ctrl Pts',(-0.114546607542374,1.79817374912461,
5.99851644517375));
#57943=CARTESIAN_POINT('Ctrl Pts',(-0.0885519162482108,1.790018321513,6.00033540371106));
#57944=CARTESIAN_POINT('Ctrl Pts',(-0.0805387328308302,1.7878404464921,
6.00089522664238));
#57945=CARTESIAN_POINT('Ctrl Pts',(-0.0700805066005682,1.78542756800238,
6.00162115754897));
#57946=CARTESIAN_POINT('Ctrl Pts',(-0.0677042208196777,1.78490758366534,
6.00178578218591));
#57947=CARTESIAN_POINT('Ctrl Pts',(-0.0572538547405641,1.7827444872967,
6.00250796394472));
#57948=CARTESIAN_POINT('Ctrl Pts',(-0.0491241569203728,1.78138441992741,
6.00306516658279));
#57949=CARTESIAN_POINT('Ctrl Pts',(-0.0298165801534796,1.77891097887452,
6.00436737920277));
#57950=CARTESIAN_POINT('Ctrl Pts',(-0.0186137921955024,1.7780671312962,
6.00510652825681));
#57951=CARTESIAN_POINT('Ctrl Pts',(-0.00636478906222278,1.77778622938642,
6.00588160057922));
#57952=CARTESIAN_POINT('Ctrl Pts',(-0.0053407838913757,1.77776762948839,
6.00594614217272));
#57953=CARTESIAN_POINT('Ctrl Pts',(-0.00357374939333483,1.77774395893557,
6.00605705802779));
#57954=CARTESIAN_POINT('Ctrl Pts',(-0.00283076616661024,1.77773657595665,
6.00610355507108));
#57955=CARTESIAN_POINT('Ctrl Pts',(-0.00177644796941559,1.77772974575061,
6.00616933145193));
#57956=CARTESIAN_POINT('Ctrl Pts',(-0.00146513624856991,1.77772818007296,
6.00618872814567));
#57957=CARTESIAN_POINT('Ctrl Pts',(-0.000929972888969344,1.77772626404852,
6.00622202816027));
#57958=CARTESIAN_POINT('Ctrl Pts',(-0.000706122669313682,1.77772569583411,
6.0062359437676));
#57959=CARTESIAN_POINT('Ctrl Pts',(-0.000277042723912563,1.77772505373371,
6.00626259182007));
#57960=CARTESIAN_POINT('Ctrl Pts',(-7.18138411814191E-5,1.77772494265461,
6.00627532636474));
#57961=CARTESIAN_POINT('Ctrl Pts',(0.000412249114008256,1.77772514304749,
6.00630533652925));
#57962=CARTESIAN_POINT('Ctrl Pts',(0.000691083487634166,1.77772562035113,
6.0063226027857));
#57963=CARTESIAN_POINT('Ctrl Pts',(0.00151654134169048,1.77772810465847,
6.00637365791319));
#57964=CARTESIAN_POINT('Ctrl Pts',(0.00206316422157728,1.77773114052335,
6.00640738942561));
#57965=CARTESIAN_POINT('Ctrl Pts',(0.00692806608651488,1.77777053776774,
6.00670692860615));
#57966=CARTESIAN_POINT('Ctrl Pts',(0.0112454701613375,1.77789230330704,
6.00696806884825));
#57967=CARTESIAN_POINT('Ctrl Pts',(0.0164168488414262,1.77814226794955,
6.00727662576614));
#57968=CARTESIAN_POINT('Ctrl Pts',(0.0172741636417999,1.77818714148329,
6.00732763878128));
#57969=CARTESIAN_POINT('Ctrl Pts',(0.0185942290903376,1.77826152661565,
6.00740598555378));
#57970=CARTESIAN_POINT('Ctrl Pts',(0.0190571062794627,1.77828861177145,
6.00743341947004));
#57971=CARTESIAN_POINT('Ctrl Pts',(0.019972969561048,1.77834418687623,6.00748762836247));
#57972=CARTESIAN_POINT('Ctrl Pts',(0.0204259569467413,1.77837263500097,
6.00751440495122));
#57973=CARTESIAN_POINT('Ctrl Pts',(0.0213271736906037,1.77843114408072,
6.00756760944102));
#57974=CARTESIAN_POINT('Ctrl Pts',(0.0217754032444151,1.77846118546392,
6.00759403804401));
#57975=CARTESIAN_POINT('Ctrl Pts',(0.0529236028462803,1.78061424101814,
6.00942838566713));
#57976=CARTESIAN_POINT('Ctrl Pts',(0.0831638781695995,1.7871224273202,6.01107389418862));
#57977=CARTESIAN_POINT('Ctrl Pts',(0.120068433768491,1.80080384500296,6.01333364628619));
#57978=CARTESIAN_POINT('Ctrl Pts',(0.127989261555435,1.80410559385301,6.01383350366518));
#57979=CARTESIAN_POINT('Ctrl Pts',(0.138838225390564,1.80914508937148,6.01454494020172));
#57980=CARTESIAN_POINT('Ctrl Pts',(0.141885172347559,1.81061923276612,6.01474777655643));
#57981=CARTESIAN_POINT('Ctrl Pts',(0.146193261950573,1.81278792595278,6.01503917722958));
#57982=CARTESIAN_POINT('Ctrl Pts',(0.147473908477938,1.81344338860694,6.01512638915847));
#57983=CARTESIAN_POINT('Ctrl Pts',(0.149429029706652,1.81446063945195,6.01526045566602));
#57984=CARTESIAN_POINT('Ctrl Pts',(0.150106686725002,1.81481629793079,6.01530709500402));
#57985=CARTESIAN_POINT('Ctrl Pts',(0.151218177784307,1.81540470714947,6.01538387702229));
#57986=CARTESIAN_POINT('Ctrl Pts',(0.151652759340992,1.81563604555936,6.01541396973184));
#57987=CARTESIAN_POINT('Ctrl Pts',(0.152491958167897,1.81608524255208,6.01547221991599));
#57988=CARTESIAN_POINT('Ctrl Pts',(0.152896643139389,1.81630297267008,6.015500372781));
#57989=CARTESIAN_POINT('Ctrl Pts',(0.153637709376501,1.81670373010934,6.01555204303792));
#57990=CARTESIAN_POINT('Ctrl Pts',(0.153974233251077,1.81688649313543,6.01557555097874));
#57991=CARTESIAN_POINT('Ctrl Pts',(0.154710508175788,1.8172880583337,6.01562708062456));
#57992=CARTESIAN_POINT('Ctrl Pts',(0.155110122002998,1.81750710920528,6.0156551111789));
#57993=CARTESIAN_POINT('Ctrl Pts',(0.156195902452067,1.81810528517933,6.01573144407577));
#57994=CARTESIAN_POINT('Ctrl Pts',(0.156881149212739,1.81848606572505,6.01577980564082));
#57995=CARTESIAN_POINT('Ctrl Pts',(0.160143880351032,1.82031472509501,6.01601097528115));
#57996=CARTESIAN_POINT('Ctrl Pts',(0.162702683139745,1.82179548642315,6.01619496376859));
#57997=CARTESIAN_POINT('Ctrl Pts',(0.166321641004864,1.8239567559912,6.01645913442091));
#57998=CARTESIAN_POINT('Ctrl Pts',(0.167398791104794,1.82460863213639,6.01653826908407));
#57999=CARTESIAN_POINT('Ctrl Pts',(0.16902587199492,1.82560639178278,6.01665858084509));
#58000=CARTESIAN_POINT('Ctrl Pts',(0.169578631078597,1.82594765918583,6.01669959035282));
#58001=CARTESIAN_POINT('Ctrl Pts',(0.197679134913713,1.84341417103175,6.01879137377047));
#58002=CARTESIAN_POINT('Ctrl Pts',(0.222480638524965,1.86459661297245,6.02100870830197));
#58003=CARTESIAN_POINT('Ctrl Pts',(0.246773618830178,1.89266918962849,6.02350159681502));
#58004=CARTESIAN_POINT('Ctrl Pts',(0.249772337884942,1.89629171369737,6.02381564995278));
#58005=CARTESIAN_POINT('Ctrl Pts',(0.256642968683991,1.90497151389146,6.0245483023688));
#58006=CARTESIAN_POINT('Ctrl Pts',(0.26044657521795,1.9100807629944,6.02496439237164));
#58007=CARTESIAN_POINT('Ctrl Pts',(0.265835920540655,1.91778680039788,6.02556621974879));
#58008=CARTESIAN_POINT('Ctrl Pts',(0.267540171836522,1.92029845616658,6.02575849527237));
#58009=CARTESIAN_POINT('Ctrl Pts',(0.269487578956976,1.92325759520918,6.02598019128351));
#58010=CARTESIAN_POINT('Ctrl Pts',(0.269765399328139,1.92368192889831,6.02601186734955));
#58011=CARTESIAN_POINT('Ctrl Pts',(0.27018759697553,1.92433011352077,6.02606007691514));
#58012=CARTESIAN_POINT('Ctrl Pts',(0.270332698764096,1.92455348805066,6.02607665877204));
#58013=CARTESIAN_POINT('Ctrl Pts',(0.270594917326387,1.92495825366348,6.02610664780295));
#58014=CARTESIAN_POINT('Ctrl Pts',(0.270712128305197,1.92513958185835,6.02612006128768));
#58015=CARTESIAN_POINT('Ctrl Pts',(0.270949306270022,1.9255073119196,6.0261472208323));
#58016=CARTESIAN_POINT('Ctrl Pts',(0.271069262646378,1.92569371895769,6.026160966173));
#58017=CARTESIAN_POINT('Ctrl Pts',(0.271413305684466,1.92622956108312,6.02620041505129));
#58018=CARTESIAN_POINT('Ctrl Pts',(0.271636910702271,1.92657930719593,6.02622608635646));
#58019=CARTESIAN_POINT('Ctrl Pts',(0.272610473426049,1.92810858333926,6.02633800306861));
#58020=CARTESIAN_POINT('Ctrl Pts',(0.273353443216009,1.92929257604979,6.02642379039984));
#58021=CARTESIAN_POINT('Ctrl Pts',(0.287073461453989,1.95147599294181,6.02801585110701));
#58022=CARTESIAN_POINT('Ctrl Pts',(0.297605399935614,1.97389683781789,6.0293748431283));
#58023=CARTESIAN_POINT('Ctrl Pts',(0.31008047671043,2.01100449842006,6.03156493642414));
#58024=CARTESIAN_POINT('Ctrl Pts',(0.313759281967147,2.02499885855254,6.03237789128311));
#58025=CARTESIAN_POINT('Ctrl Pts',(0.318105113879117,2.04761754092978,6.03371481961574));
#58026=CARTESIAN_POINT('Ctrl Pts',(0.31938672821074,2.05610371082636,6.03422120728117));
#58027=CARTESIAN_POINT('Ctrl Pts',(0.32051292859904,2.06630325241381,6.03483981821183));
#58028=CARTESIAN_POINT('Ctrl Pts',(0.320684530268572,2.06797750667553,6.0349416777637));
#58029=CARTESIAN_POINT('Ctrl Pts',(0.320923811497116,2.07050730269682,6.03509609153991));
#58030=CARTESIAN_POINT('Ctrl Pts',(0.321001202462517,2.07136191390072,6.03514834202492));
#58031=CARTESIAN_POINT('Ctrl Pts',(0.32112098689032,2.07274619760191,6.03523312052977));
#58032=CARTESIAN_POINT('Ctrl Pts',(0.321165485515884,2.07327568757455,6.0352655825102));
#58033=CARTESIAN_POINT('Ctrl Pts',(0.321248311683141,2.0742913306554,6.03532791598354));
#58034=CARTESIAN_POINT('Ctrl Pts',(0.321286845675813,2.07477746582335,6.0353577809155));
#58035=CARTESIAN_POINT('Ctrl Pts',(0.321353853909911,2.07564790153094,6.03541130761905));
#58036=CARTESIAN_POINT('Ctrl Pts',(0.321382742606543,2.07603216999382,6.03543495632493));
#58037=CARTESIAN_POINT('Ctrl Pts',(0.321438830393111,2.07679656964346,6.03548203616105));
#58038=CARTESIAN_POINT('Ctrl Pts',(0.321466044554084,2.07717669915171,6.03550546677965));
#58039=CARTESIAN_POINT('Ctrl Pts',(0.321530664410971,2.07810236367373,6.03556256811849));
#58040=CARTESIAN_POINT('Ctrl Pts',(0.321567355950908,2.07864794590456,6.03559626120986));
#58041=CARTESIAN_POINT('Ctrl Pts',(0.321700661992337,2.08070844703493,6.03572365460019));
#58042=CARTESIAN_POINT('Ctrl Pts',(0.321787959928929,2.0822239301215,6.03581764676955));
#58043=CARTESIAN_POINT('Ctrl Pts',(0.323158692612482,2.10935732344249,6.03750593866038));
#58044=CARTESIAN_POINT('Ctrl Pts',(0.321389671727212,2.13503189134735,6.03920166358152));
#58045=CARTESIAN_POINT('Ctrl Pts',(0.313724772733462,2.17532928979751,6.04197348407867));
#58046=CARTESIAN_POINT('Ctrl Pts',(0.309772761142307,2.19021420937721,6.04301977850816));
#58047=CARTESIAN_POINT('Ctrl Pts',(0.30226002210517,2.21207054388735,6.04454815713027));
#58048=CARTESIAN_POINT('Ctrl Pts',(0.299484852913449,2.21928860857097,6.04505129930937));
#58049=CARTESIAN_POINT('Ctrl Pts',(0.295814209527044,2.22789752806881,6.04564372284205));
#58050=CARTESIAN_POINT('Ctrl Pts',(0.295164552344143,2.2293897660107,6.04574612443588));
#58051=CARTESIAN_POINT('Ctrl Pts',(0.294333279016621,2.23126032299449,6.04587406658077));
#58052=CARTESIAN_POINT('Ctrl Pts',(0.29416220613545,2.23164326042592,6.04590023639711));
#58053=CARTESIAN_POINT('Ctrl Pts',(0.293889111114884,2.23225137846412,6.04594175823122));
#58054=CARTESIAN_POINT('Ctrl Pts',(0.293787577336947,2.23247677585536,6.04595714015285));
#58055=CARTESIAN_POINT('Ctrl Pts',(0.293595663647149,2.2329015041803,6.04598610965021));
#58056=CARTESIAN_POINT('Ctrl Pts',(0.293505340767425,2.23310085825089,6.04599970054055));
#58057=CARTESIAN_POINT('Ctrl Pts',(0.29329962404224,2.23355367355041,6.04603055651584));
#58058=CARTESIAN_POINT('Ctrl Pts',(0.293184104910394,2.2338070768361,6.04604781372093));
#58059=CARTESIAN_POINT('Ctrl Pts',(0.292832826822641,2.23457500315665,6.04610008043174));
#58060=CARTESIAN_POINT('Ctrl Pts',(0.292596039246178,2.23508905865577,6.04613502670821));
#58061=CARTESIAN_POINT('Ctrl Pts',(0.290924605397629,2.23869265675996,6.0463797318912));
#58062=CARTESIAN_POINT('Ctrl Pts',(0.289442341057997,2.24176005259815,6.0465866157625));
#58063=CARTESIAN_POINT('Ctrl Pts',(0.276673061714968,2.26714910657841,6.04829189798559));
#58064=CARTESIAN_POINT('Ctrl Pts',(0.262869620789346,2.28811362617499,6.04965855111715));
#58065=CARTESIAN_POINT('Ctrl Pts',(0.232677628683257,2.32406013908515,6.05229237088171));
#58066=CARTESIAN_POINT('Ctrl Pts',(0.216903551347983,2.33936261254836,6.05354461256304));
#58067=CARTESIAN_POINT('Ctrl Pts',(0.19895236730321,2.35353508372282,6.05493302203375));
#58068=CARTESIAN_POINT('Ctrl Pts',(0.198202064817772,2.35412206634907,6.05499098159017));
#58069=CARTESIAN_POINT('Ctrl Pts',(0.196998069755074,2.35505540952141,6.05508387928737));
#58070=CARTESIAN_POINT('Ctrl Pts',(0.196546036534835,2.35540390938515,6.05511873285867));
#58071=CARTESIAN_POINT('Ctrl Pts',(0.195683308370511,2.356065392192,6.05518520761916));
#58072=CARTESIAN_POINT('Ctrl Pts',(0.195272781971566,2.35637859284553,6.05521682010577));
#58073=CARTESIAN_POINT('Ctrl Pts',(0.194551285978017,2.35692630158305,6.05527234572342));
#58074=CARTESIAN_POINT('Ctrl Pts',(0.194240639878214,2.35716123568374,6.05529624205379));
#58075=CARTESIAN_POINT('Ctrl Pts',(0.193633016628128,2.35761903726646,6.05534296276148));
#58076=CARTESIAN_POINT('Ctrl Pts',(0.193336078578046,2.3578419558739,6.0553657850865));
#58077=CARTESIAN_POINT('Ctrl Pts',(0.192630003943509,2.35837011780096,6.05542003100266));
#58078=CARTESIAN_POINT('Ctrl Pts',(0.192220527000308,2.3586749025064,6.05545147243882));
#58079=CARTESIAN_POINT('Ctrl Pts',(0.190772753070647,2.35974718367091,6.05556257812688));
#58080=CARTESIAN_POINT('Ctrl Pts',(0.189730580083967,2.3605094041341,6.05564244714957));
#58081=CARTESIAN_POINT('Ctrl Pts',(0.173247512178866,2.37241335235415,6.0569040280374));
#58082=CARTESIAN_POINT('Ctrl Pts',(0.15685648537718,2.382169353956,6.05813960272788));
#58083=CARTESIAN_POINT('Ctrl Pts',(0.119684304392901,2.40005053932184,6.06089426569416));
#58084=CARTESIAN_POINT('Ctrl Pts',(0.098724491135488,2.40758428832935,6.06241991181727));
#58085=CARTESIAN_POINT('Ctrl Pts',(0.0710101032122141,2.41441822708487,
6.06430826499847));
#58086=CARTESIAN_POINT('Ctrl Pts',(0.0648195163537652,2.41575258956753,
6.06472174196745));
#58087=CARTESIAN_POINT('Ctrl Pts',(0.05567603529061,2.41744315343383,6.0653165470208));
#58088=CARTESIAN_POINT('Ctrl Pts',(0.0527514027849231,2.4179422394241,6.0655044342247));
#58089=CARTESIAN_POINT('Ctrl Pts',(0.0493221151375749,2.41847881988596,
6.06572165091937));
#58090=CARTESIAN_POINT('Ctrl Pts',(0.0488238733228427,2.41855558252769,
6.06575313424284));
#58091=CARTESIAN_POINT('Ctrl Pts',(0.0480627397245179,2.41867102045701,
6.06580111103935));
#58092=CARTESIAN_POINT('Ctrl Pts',(0.0477999797004034,2.41871053978619,
6.06581765215867));
#58093=CARTESIAN_POINT('Ctrl Pts',(0.0473425580156136,2.41877875798385,
6.0658464096939));
#58094=CARTESIAN_POINT('Ctrl Pts',(0.0471479194930042,2.41880760346854,
6.06585863444783));
#58095=CARTESIAN_POINT('Ctrl Pts',(0.0467072948921429,2.41887249181483,
6.06588628192731));
#58096=CARTESIAN_POINT('Ctrl Pts',(0.0464612939664794,2.41890842823027,
6.06590169850582));
#58097=CARTESIAN_POINT('Ctrl Pts',(0.0457939625917339,2.41900512507688,
6.06594346836437));
#58098=CARTESIAN_POINT('Ctrl Pts',(0.045372551070656,2.41906533570641,6.06596979041004));
#58099=CARTESIAN_POINT('Ctrl Pts',(0.0434736757502484,2.41933280599869,
6.06608815407462));
#58100=CARTESIAN_POINT('Ctrl Pts',(0.0419948721830814,2.41953064388627,
6.06617967033556));
#58101=CARTESIAN_POINT('Ctrl Pts',(0.00853123491329284,2.4237711584285,
6.0682366874628));
#58102=CARTESIAN_POINT('Ctrl Pts',(-0.0238853703800827,2.42300288438291,
6.06995659374557));
#58103=CARTESIAN_POINT('Ctrl Pts',(-0.072591374857377,2.41446366609711,
6.07276110104687));
#58104=CARTESIAN_POINT('Ctrl Pts',(-0.0892624662103829,2.41014349417944,
6.07375989293959));
#58105=CARTESIAN_POINT('Ctrl Pts',(-0.106618269922248,2.40413007230692,
6.07487666012262));
#58106=CARTESIAN_POINT('Ctrl Pts',(-0.107726438239217,2.40373931390203,
6.07494830081459));
#58107=CARTESIAN_POINT('Ctrl Pts',(-0.109332175599828,2.40316321164182,
6.0750526042093));
#58108=CARTESIAN_POINT('Ctrl Pts',(-0.109831471566688,2.40298268162148,
6.07508510669631));
#58109=CARTESIAN_POINT('Ctrl Pts',(-0.110703619843708,2.40266490056629,
6.07514200375382));
#58110=CARTESIAN_POINT('Ctrl Pts',(-0.111076669707779,2.40252819195184,
6.07516638019371));
#58111=CARTESIAN_POINT('Ctrl Pts',(-0.111798115605101,2.40226229510442,
6.0752135989404));
#58112=CARTESIAN_POINT('Ctrl Pts',(-0.112146543078011,2.40213319342386,
6.07523643832512));
#58113=CARTESIAN_POINT('Ctrl Pts',(-0.112974078990658,2.40182494055626,
6.07529076623788));
#58114=CARTESIAN_POINT('Ctrl Pts',(-0.113452984627335,2.40164525114762,
6.07532227273767));
#58115=CARTESIAN_POINT('Ctrl Pts',(-0.115145050046982,2.40100577442701,
6.07543382708968));
#58116=CARTESIAN_POINT('Ctrl Pts',(-0.116355846731803,2.40053980708236,
6.07551408189172));
#58117=CARTESIAN_POINT('Ctrl Pts',(-0.136351290076403,2.39270574499538,
6.07684665428916));
#58118=CARTESIAN_POINT('Ctrl Pts',(-0.154402304294605,2.38359827180811,
6.07815981129278));
#58119=CARTESIAN_POINT('Ctrl Pts',(-0.180215954593104,2.36737580437865,
6.08020128533362));
#58120=CARTESIAN_POINT('Ctrl Pts',(-0.188682130013069,2.36147017666878,
6.08089989494506));
#58121=CARTESIAN_POINT('Ctrl Pts',(-0.205208739096896,2.3487207126804,6.08231211659649));
#58122=CARTESIAN_POINT('Ctrl Pts',(-0.213245753435008,2.34186543318844,
6.08302486799576));
#58123=CARTESIAN_POINT('Ctrl Pts',(-0.227032239669349,2.32888369114118,
6.08427850967839));
#58124=CARTESIAN_POINT('Ctrl Pts',(-0.232906681989655,2.32290331266854,
6.08482398972139));
#58125=CARTESIAN_POINT('Ctrl Pts',(-0.239422553371044,2.31573069357209,
6.08543567064522));
#58126=CARTESIAN_POINT('Ctrl Pts',(-0.240297375151487,2.31475582144961,
6.08551793974294));
#58127=CARTESIAN_POINT('Ctrl Pts',(-0.241423824373539,2.31348504264521,
6.08562402943166));
#58128=CARTESIAN_POINT('Ctrl Pts',(-0.241680878315509,2.31319399491729,
6.08564824966583));
#58129=CARTESIAN_POINT('Ctrl Pts',(-0.242096118861859,2.31272212525919,
6.08568739099263));
#58130=CARTESIAN_POINT('Ctrl Pts',(-0.242254629426003,2.31254159090714,
6.08570233636578));
#58131=CARTESIAN_POINT('Ctrl Pts',(-0.242558253511869,2.31219499973033,
6.08573097111408));
#58132=CARTESIAN_POINT('Ctrl Pts',(-0.242703398001503,2.31202897173744,
6.08574466278412));
#58133=CARTESIAN_POINT('Ctrl Pts',(-0.243036808975878,2.31164679839394,
6.08577612131313));
#58134=CARTESIAN_POINT('Ctrl Pts',(-0.243224958136835,2.3114305501304,6.08579387935271));
#58135=CARTESIAN_POINT('Ctrl Pts',(-0.243806779978318,2.31076003178779,
6.08584881138185));
#58136=CARTESIAN_POINT('Ctrl Pts',(-0.244199473255355,2.31030490778423,
6.08588591275705));
#58137=CARTESIAN_POINT('Ctrl Pts',(-0.247432273563176,2.30653689024694,
6.08619158415615));
#58138=CARTESIAN_POINT('Ctrl Pts',(-0.250206267961081,2.30316752958681,
6.08645540300492));
#58139=CARTESIAN_POINT('Ctrl Pts',(-0.253417410859009,2.29910162918703,
6.08676407404153));
#58140=CARTESIAN_POINT('Ctrl Pts',(-0.25392125269123,2.29845866151078,6.08681260498745));
#58141=CARTESIAN_POINT('Ctrl Pts',(-0.254498918147973,2.29771568406699,
6.0868683705174));
#58142=CARTESIAN_POINT('Ctrl Pts',(-0.25457513041202,2.29761754486977,6.08687573024442));
#58143=CARTESIAN_POINT('Ctrl Pts',(-0.254837199113164,2.2972796735276,6.08690104660015));
#58144=CARTESIAN_POINT('Ctrl Pts',(-0.255022774353042,2.29703972239507,
6.08691898860585));
#58145=CARTESIAN_POINT('Ctrl Pts',(-0.272519743352753,2.27434979452356,
6.08861211490864));
#58146=CARTESIAN_POINT('Ctrl Pts',(-0.286795492931976,2.24971173398175,
6.09013876506786));
#58147=CARTESIAN_POINT('Ctrl Pts',(-0.304046051141138,2.2081408845776,6.09269533336683));
#58148=CARTESIAN_POINT('Ctrl Pts',(-0.309225792538832,2.19229160802325,
6.09366408858299));
#58149=CARTESIAN_POINT('Ctrl Pts',(-0.313434583055251,2.1749754102828,6.09474757643626));
#58150=CARTESIAN_POINT('Ctrl Pts',(-0.313705243810199,2.17383474758697,
6.09481905284651));
#58151=CARTESIAN_POINT('Ctrl Pts',(-0.314089316520008,2.17217588399112,
6.09492316056475));
#58152=CARTESIAN_POINT('Ctrl Pts',(-0.314207684440214,2.17165883068618,
6.09495563250657));
#58153=CARTESIAN_POINT('Ctrl Pts',(-0.314412462385804,2.17075405933997,
6.09501249404458));
#58154=CARTESIAN_POINT('Ctrl Pts',(-0.314499433304771,2.17036646833032,
6.09503686557836));
#58155=CARTESIAN_POINT('Ctrl Pts',(-0.314666401092002,2.16961587333682,
6.09508408791751));
#58156=CARTESIAN_POINT('Ctrl Pts',(-0.314746486996248,2.16925288960298,
6.09510693582506));
#58157=CARTESIAN_POINT('Ctrl Pts',(-0.31493539689231,2.16838957220406,6.09516130464812));
#58158=CARTESIAN_POINT('Ctrl Pts',(-0.315043656579309,2.167889117289,6.09519284359864));
#58159=CARTESIAN_POINT('Ctrl Pts',(-0.315422653256835,2.16611668967211,
6.09530462216546));
#58160=CARTESIAN_POINT('Ctrl Pts',(-0.3156868805191,2.1648433514663,6.09538506982508));
#58161=CARTESIAN_POINT('Ctrl Pts',(-0.320174180133562,2.14254089876369,
6.09679672931513));
#58162=CARTESIAN_POINT('Ctrl Pts',(-0.322294390262843,2.12114782869986,
6.0981971628962));
#58163=CARTESIAN_POINT('Ctrl Pts',(-0.322252498381139,2.07514179083036,
6.10128594209211));
#58164=CARTESIAN_POINT('Ctrl Pts',(-0.319421715827119,2.05065997744838,
6.10297727197978));
#58165=CARTESIAN_POINT('Ctrl Pts',(-0.313587547175297,2.02566810382857,
6.10463535462289));
#58166=CARTESIAN_POINT('Ctrl Pts',(-0.313332547194403,2.02460042792881,
6.10470604126003));
#58167=CARTESIAN_POINT('Ctrl Pts',(-0.312278628154533,2.02028540029798,
6.10499106618463));
#58168=CARTESIAN_POINT('Ctrl Pts',(-0.311434605938142,2.01704912657215,
6.10520332941835));
#58169=CARTESIAN_POINT('Ctrl Pts',(-0.310391688961403,2.01329080772112,
6.10544760274731));
#58170=CARTESIAN_POINT('Ctrl Pts',(-0.310241670753992,2.01275557129131,
6.10548233755754));
#58171=CARTESIAN_POINT('Ctrl Pts',(-0.310013924409518,2.01195103147772,
6.10553446640724));
#58172=CARTESIAN_POINT('Ctrl Pts',(-0.309937229503655,2.01168144048583,
6.10555192012439));
#58173=CARTESIAN_POINT('Ctrl Pts',(-0.309799968195203,2.0112013326895,6.10558297764037));
#58174=CARTESIAN_POINT('Ctrl Pts',(-0.309739538902464,2.01099077771695,
6.10559658943409));
#58175=CARTESIAN_POINT('Ctrl Pts',(-0.309610757202732,2.01054378039886,
6.10562546793786));
#58176=CARTESIAN_POINT('Ctrl Pts',(-0.309542348802191,2.0103073553742,6.10564073127614));
#58177=CARTESIAN_POINT('Ctrl Pts',(-0.309357993143648,2.00967293013661,
6.10568166003039));
#58178=CARTESIAN_POINT('Ctrl Pts',(-0.309241548198942,2.00927507319344,
6.10570729632664));
#58179=CARTESIAN_POINT('Ctrl Pts',(-0.308679484388917,2.00736832693394,
6.1058300169887));
#58180=CARTESIAN_POINT('Ctrl Pts',(-0.308223577986725,2.00586245622988,
6.10592650888078));
#58181=CARTESIAN_POINT('Ctrl Pts',(-0.304339793046374,1.99336496555509,
6.10672421156539));
#58182=CARTESIAN_POINT('Ctrl Pts',(-0.300335754018257,1.98255964340394,
6.10739400217946));
#58183=CARTESIAN_POINT('Ctrl Pts',(-0.288099967351573,1.95428924479531,
6.10914954923612));
#58184=CARTESIAN_POINT('Ctrl Pts',(-0.278864724840168,1.93731094009641,
6.11020925435597));
#58185=CARTESIAN_POINT('Ctrl Pts',(-0.257997196607783,1.90600307688698,
6.11233577532785));
#58186=CARTESIAN_POINT('Ctrl Pts',(-0.246546215926454,1.89164411839782,
6.11339596981487));
#58187=CARTESIAN_POINT('Ctrl Pts',(-0.233053395332642,1.87740407849933,
6.11458755156693));
#58188=CARTESIAN_POINT('Ctrl Pts',(-0.232163328989578,1.8764759119415,6.11466590073906));
#58189=CARTESIAN_POINT('Ctrl Pts',(-0.230912850802078,1.87518743223455,
6.11477563323072));
#58190=CARTESIAN_POINT('Ctrl Pts',(-0.230557095112029,1.87482260064643,
6.11480681337896));
#58191=CARTESIAN_POINT('Ctrl Pts',(-0.229940785522465,1.87419355971777,
6.11486076451862));
#58192=CARTESIAN_POINT('Ctrl Pts',(-0.229680637073817,1.87392895304547,
6.11488351769808));
#58193=CARTESIAN_POINT('Ctrl Pts',(-0.229140783950723,1.87338174200713,
6.11493069355465));
#58194=CARTESIAN_POINT('Ctrl Pts',(-0.228861012213215,1.87309920491146,
6.11495511916866));
#58195=CARTESIAN_POINT('Ctrl Pts',(-0.228205124685474,1.87243928156132,
6.11501232932334));
#58196=CARTESIAN_POINT('Ctrl Pts',(-0.227828595302568,1.87206230968517,
6.11504513214394));
#58197=CARTESIAN_POINT('Ctrl Pts',(-0.226611480104256,1.87084979286035,
6.11515103813267));
#58198=CARTESIAN_POINT('Ctrl Pts',(-0.225767226719683,1.87001795803512,
6.11522430445236));
#58199=CARTESIAN_POINT('Ctrl Pts',(-0.223792376335082,1.86809351035422,
6.11539524481828));
#58200=CARTESIAN_POINT('Ctrl Pts',(-0.222658341224862,1.86700448376102,
6.11549307299862));
#58201=CARTESIAN_POINT('Ctrl Pts',(-0.210819650012635,1.85580101924174,
6.11651101464629));
#58202=CARTESIAN_POINT('Ctrl Pts',(-0.199443175942011,1.84642480858418,
6.11746246721005));
#58203=CARTESIAN_POINT('Ctrl Pts',(-0.162347505265138,1.81989616912389,
6.12048368240245));
#58204=CARTESIAN_POINT('Ctrl Pts',(-0.134778971525478,1.80563739888518,
6.12263443974411));
#58205=CARTESIAN_POINT('Ctrl Pts',(-0.10231325515177,1.79437717859305,6.12484157555323));
#58206=CARTESIAN_POINT('Ctrl Pts',(-0.0990035264729396,1.79328903617023,
6.12506282975967));
#58207=CARTESIAN_POINT('Ctrl Pts',(-0.0951324524187147,1.79208553640912,
6.12531673954882));
#58208=CARTESIAN_POINT('Ctrl Pts',(-0.094587809726223,1.79191779237569,
6.12535235206415));
#58209=CARTESIAN_POINT('Ctrl Pts',(-0.0937755978687378,1.79166999681326,
6.12540529116005));
#58210=CARTESIAN_POINT('Ctrl Pts',(-0.0935083686859163,1.79158884811361,
6.12542268166413));
#58211=CARTESIAN_POINT('Ctrl Pts',(-0.0930314525777255,1.79144470123993,
6.12545366904471));
#58212=CARTESIAN_POINT('Ctrl Pts',(-0.0928218071158267,1.79138156943168,
6.12546727377751));
#58213=CARTESIAN_POINT('Ctrl Pts',(-0.0923757752453353,1.79124774875767,
6.12549618258839));
#58214=CARTESIAN_POINT('Ctrl Pts',(-0.0921393726370167,1.79117711789698,
6.12551148320236));
#58215=CARTESIAN_POINT('Ctrl Pts',(-0.0915029618571355,1.79098777096134,
6.12555261636274));
#58216=CARTESIAN_POINT('Ctrl Pts',(-0.0911028021387213,1.79086955961731,
6.12557841928132));
#58217=CARTESIAN_POINT('Ctrl Pts',(-0.0891639944751465,1.7903009072697,
6.12570314829454));
#58218=CARTESIAN_POINT('Ctrl Pts',(-0.087622194656767,1.78986116463411,
6.12580145817532));
#58219=CARTESIAN_POINT('Ctrl Pts',(-0.0745794032770317,1.78624620892881,
6.12662620682416));
#58220=CARTESIAN_POINT('Ctrl Pts',(-0.0629121295655456,1.78370004582771,
6.12731893360064));
#58221=CARTESIAN_POINT('Ctrl Pts',(-0.01967727693028,1.77675280710321,6.12981034467774));
#58222=CARTESIAN_POINT('Ctrl Pts',(0.0123483058771805,1.77638983346874,
6.13152979185127));
#58223=CARTESIAN_POINT('Ctrl Pts',(0.0496733722488915,1.78152299729853,
6.13376209380974));
#58224=CARTESIAN_POINT('Ctrl Pts',(0.0554160184057503,1.78247188550634,
6.13411136692855));
#58225=CARTESIAN_POINT('Ctrl Pts',(0.062098464152659,1.78376285768748,6.1345257013214));
#58226=CARTESIAN_POINT('Ctrl Pts',(0.0630664904390666,1.78395448559134,
6.13458591669315));
#58227=CARTESIAN_POINT('Ctrl Pts',(0.0645247807302468,1.78425013149964,
6.13467692719652));
#58228=CARTESIAN_POINT('Ctrl Pts',(0.0650157133332328,1.78435085331722,
6.13470761695353));
#58229=CARTESIAN_POINT('Ctrl Pts',(0.0658912836991643,1.78453261837151,
6.13476244364955));
#58230=CARTESIAN_POINT('Ctrl Pts',(0.0662760127161906,1.78461322114691,
6.13478656645093));
#58231=CARTESIAN_POINT('Ctrl Pts',(0.0670872480887549,1.78478472920762,
6.13483749890691));
#58232=CARTESIAN_POINT('Ctrl Pts',(0.0675137190157128,1.78487579664753,
6.13486431371254));
#58233=CARTESIAN_POINT('Ctrl Pts',(0.0686407959578311,1.78511886257096,
6.13493528455893));
#58234=CARTESIAN_POINT('Ctrl Pts',(0.0693410789654432,1.7852723330672,6.13497948772036));
#58235=CARTESIAN_POINT('Ctrl Pts',(0.0725210370095364,1.78598036502446,
6.13518070432379));
#58236=CARTESIAN_POINT('Ctrl Pts',(0.0749945575184244,1.78656189174418,
6.13533858148531));
#58237=CARTESIAN_POINT('Ctrl Pts',(0.0857612650868999,1.78922789448097,
6.13603191459942));
#58238=CARTESIAN_POINT('Ctrl Pts',(0.0939758539606996,1.7916125603886,6.13657697597359));
#58239=CARTESIAN_POINT('Ctrl Pts',(0.11574516496817,1.79888269075009,6.1380659913772));
#58240=CARTESIAN_POINT('Ctrl Pts',(0.129082476472,1.80435458012504,6.1390266835851));
#58241=CARTESIAN_POINT('Ctrl Pts',(0.1584904971171,1.81878998915011,6.14123700957637));
#58242=CARTESIAN_POINT('Ctrl Pts',(0.174251876602522,1.82827469863625,6.14249019169553));
#58243=CARTESIAN_POINT('Ctrl Pts',(0.190264851916607,1.83987991184667,6.14378919008863));
#58244=CARTESIAN_POINT('Ctrl Pts',(0.191404076532268,1.84071703923454,6.14388174293532));
#58245=CARTESIAN_POINT('Ctrl Pts',(0.193569150051231,1.84233002906218,6.14405784722488));
#58246=CARTESIAN_POINT('Ctrl Pts',(0.19459593395165,1.84310458867143,6.14414145571172));
#58247=CARTESIAN_POINT('Ctrl Pts',(0.195905010449885,1.84410444928828,6.14424814021547));
#58248=CARTESIAN_POINT('Ctrl Pts',(0.196191584954809,1.84432409580013,6.14427150043006));
#58249=CARTESIAN_POINT('Ctrl Pts',(0.197079354728163,1.84500690300454,6.14434388296792));
#58250=CARTESIAN_POINT('Ctrl Pts',(0.197679288094204,1.84547170951711,6.14439281972307));
#58251=CARTESIAN_POINT('Ctrl Pts',(0.201200631414062,1.84821987798304,6.14468016220897));
#58252=CARTESIAN_POINT('Ctrl Pts',(0.204084254296424,1.85055152035375,6.1449158970472));
#58253=CARTESIAN_POINT('Ctrl Pts',(0.2073723218429,1.8533053852159,6.14518457005795));
#58254=CARTESIAN_POINT('Ctrl Pts',(0.207816497727555,1.8536794443926,6.1452208616136));
#58255=CARTESIAN_POINT('Ctrl Pts',(0.208474439840365,1.85423657155294,6.14527461177801));
#58256=CARTESIAN_POINT('Ctrl Pts',(0.208688978099588,1.85441871966698,6.14529213719708));
#58257=CARTESIAN_POINT('Ctrl Pts',(0.209066299364539,1.85473992593625,6.1453229577456));
#58258=CARTESIAN_POINT('Ctrl Pts',(0.209229182371642,1.85487886524237,6.14533626161611));
#58259=CARTESIAN_POINT('Ctrl Pts',(0.209573492832958,1.85517315552479,6.14536438216025));
#58260=CARTESIAN_POINT('Ctrl Pts',(0.209754885581102,1.8553285454949,6.14537919582944));
#58261=CARTESIAN_POINT('Ctrl Pts',(0.210126415708694,1.85564753334101,6.14540953555669));
#58262=CARTESIAN_POINT('Ctrl Pts',(0.210316535243675,1.85581115188232,6.14542506006956));
#58263=CARTESIAN_POINT('Ctrl Pts',(0.210787480414418,1.85621740943749,6.14546351406734));
#58264=CARTESIAN_POINT('Ctrl Pts',(0.211068079185067,1.85646031265279,6.14548642417412));
#58265=CARTESIAN_POINT('Ctrl Pts',(0.211848953993099,1.85713864821505,6.14555017808704));
#58266=CARTESIAN_POINT('Ctrl Pts',(0.21234830987487,1.85757514399296,6.14559094492608));
#58267=CARTESIAN_POINT('Ctrl Pts',(0.216774543820778,1.86146836270738,6.14595231101492));
#58268=CARTESIAN_POINT('Ctrl Pts',(0.22061832218819,1.86501891950113,6.14626622065885));
#58269=CARTESIAN_POINT('Ctrl Pts',(0.228919635561087,1.87307033490035,6.1469489179583));
#58270=CARTESIAN_POINT('Ctrl Pts',(0.233334411963596,1.87761220020752,6.14731522148948));
#58271=CARTESIAN_POINT('Ctrl Pts',(0.257402471648043,1.90387949229667,6.1493507933882));
#58272=CARTESIAN_POINT('Ctrl Pts',(0.274154946726946,1.92807422356698,6.15093270075099));
#58273=CARTESIAN_POINT('Ctrl Pts',(0.291601912712039,1.96246667060929,6.15318173199054));
#58274=CARTESIAN_POINT('Ctrl Pts',(0.295436405075282,1.97090934319422,6.15373250469504));
#58275=CARTESIAN_POINT('Ctrl Pts',(0.29932781992931,1.98056243536318,6.15436545921748));
#58276=CARTESIAN_POINT('Ctrl Pts',(0.299748500421382,1.9816221639291,6.15443498552988));
#58277=CARTESIAN_POINT('Ctrl Pts',(0.300352383037549,1.98316725316324,6.15453642074973));
#58278=CARTESIAN_POINT('Ctrl Pts',(0.300540053984974,1.98365086731954,6.15456817935076));
#58279=CARTESIAN_POINT('Ctrl Pts',(0.300869216756015,1.98450520578921,6.15462430037405));
#58280=CARTESIAN_POINT('Ctrl Pts',(0.301011193422248,1.98487574315788,6.15464864647198));
#58281=CARTESIAN_POINT('Ctrl Pts',(0.301303327870427,1.98564240427087,6.15469903201226));
#58282=CARTESIAN_POINT('Ctrl Pts',(0.301453389587099,1.98603856358196,6.15472507461606));
#58283=CARTESIAN_POINT('Ctrl Pts',(0.301835614107753,1.98705366464322,6.15479182281734));
#58284=CARTESIAN_POINT('Ctrl Pts',(0.302066653615032,1.98767302471025,6.15483256588615));
#58285=CARTESIAN_POINT('Ctrl Pts',(0.303002421146999,1.99020535305112,6.15499922122754));
#58286=CARTESIAN_POINT('Ctrl Pts',(0.303690883495235,1.99212424417632,6.15512567438918));
#58287=CARTESIAN_POINT('Ctrl Pts',(0.314693320219725,2.02373064189522,6.15721161241558));
#58288=CARTESIAN_POINT('Ctrl Pts',(0.320626025351641,2.05475741142396,6.15932935833572));
#58289=CARTESIAN_POINT('Ctrl Pts',(0.322723830933223,2.1034948798078,6.16262606891827));
#58290=CARTESIAN_POINT('Ctrl Pts',(0.322066676492338,2.12088300378392,6.16379047740456));
#58291=CARTESIAN_POINT('Ctrl Pts',(0.319883851859226,2.1392000871647,6.16495250446753));
#58292=CARTESIAN_POINT('Ctrl Pts',(0.319751645760659,2.14026425988876,6.16501977621116));
#58293=CARTESIAN_POINT('Ctrl Pts',(0.319566238746471,2.14169813111846,6.16511007812119));
#58294=CARTESIAN_POINT('Ctrl Pts',(0.319517705201432,2.14206841037539,6.16513336682239));
#58295=CARTESIAN_POINT('Ctrl Pts',(0.319440442900471,2.14265002404014,6.16516989835721));
#58296=CARTESIAN_POINT('Ctrl Pts',(0.319412147986425,2.14286141423722,6.16518316573174));
#58297=CARTESIAN_POINT('Ctrl Pts',(0.319354886969042,2.14328600335469,6.16520979333015));
#58298=CARTESIAN_POINT('Ctrl Pts',(0.319325917435808,2.14349919966461,6.16522315317109));
#58299=CARTESIAN_POINT('Ctrl Pts',(0.319259276128592,2.14398598069271,6.16525363326509));
#58300=CARTESIAN_POINT('Ctrl Pts',(0.319221466239346,2.14425954569449,6.16527074556021));
#58301=CARTESIAN_POINT('Ctrl Pts',(0.319141430067438,2.14483319161268,6.16530659346751));
#58302=CARTESIAN_POINT('Ctrl Pts',(0.319099132057455,2.14513326242987,6.16532532501048));
#58303=CARTESIAN_POINT('Ctrl Pts',(0.318986495932055,2.14592425269514,6.16537464913859));
#58304=CARTESIAN_POINT('Ctrl Pts',(0.318915447437252,2.14641507261807,6.16540520212951));
#58305=CARTESIAN_POINT('Ctrl Pts',(0.31869904851986,2.14788605147193,6.16549661438319));
#58306=CARTESIAN_POINT('Ctrl Pts',(0.318550308793114,2.14886571680875,6.16555728870091));
#58307=CARTESIAN_POINT('Ctrl Pts',(0.316763054360369,2.16028230868027,6.16626212187127));
#58308=CARTESIAN_POINT('Ctrl Pts',(0.314616609181587,2.17063447073129,6.16687947007845));
#58309=CARTESIAN_POINT('Ctrl Pts',(0.30490258971354,2.20811040165076,6.16909479674247));
#58310=CARTESIAN_POINT('Ctrl Pts',(0.29430119535565,2.23431449233291,6.17061649384455));
#58311=CARTESIAN_POINT('Ctrl Pts',(0.27945710958026,2.26052661951239,6.17236261068925));
#58312=CARTESIAN_POINT('Ctrl Pts',(0.27846870563566,2.26223517324694,6.17247746389227));
#58313=CARTESIAN_POINT('Ctrl Pts',(0.276159650424283,2.26614332683492,6.17274269964716));
#58314=CARTESIAN_POINT('Ctrl Pts',(0.274828315617226,2.26833643102073,6.1728934014094));
#58315=CARTESIAN_POINT('Ctrl Pts',(0.27007960422049,2.27595245969209,6.17342366610002));
#58316=CARTESIAN_POINT('Ctrl Pts',(0.266526930772546,2.28128885006375,6.17380768783157));
#58317=CARTESIAN_POINT('Ctrl Pts',(0.262222287329415,2.28735449304122,6.17426038829708));
#58318=CARTESIAN_POINT('Ctrl Pts',(0.261622869962691,2.28819061588986,6.1743231572484));
#58319=CARTESIAN_POINT('Ctrl Pts',(0.260724547062876,2.28943109303871,6.17441683438047));
#58320=CARTESIAN_POINT('Ctrl Pts',(0.260428678015473,2.28983764672363,6.17444762509177));
#58321=CARTESIAN_POINT('Ctrl Pts',(0.259899701467144,2.29056094949178,6.17450256469765));
#58322=CARTESIAN_POINT('Ctrl Pts',(0.259666962819982,2.29087796811468,6.17452669923447));
#58323=CARTESIAN_POINT('Ctrl Pts',(0.25917547098953,2.291544877874,6.17457758706424));
#58324=CARTESIAN_POINT('Ctrl Pts',(0.258916588410107,2.29189467226977,6.17460434536989));
#58325=CARTESIAN_POINT('Ctrl Pts',(0.258231779284392,2.29281605722242,6.17467500809318));
#58326=CARTESIAN_POINT('Ctrl Pts',(0.257804665177576,2.29338675847847,6.1747189588991));
#58327=CARTESIAN_POINT('Ctrl Pts',(0.255870594628274,2.2959532302734,6.17491743807886));
#58328=CARTESIAN_POINT('Ctrl Pts',(0.254342364850452,2.29793279295081,6.17507280165207));
#58329=CARTESIAN_POINT('Ctrl Pts',(0.242875458509469,2.31243412501182,6.1762281480485));
#58330=CARTESIAN_POINT('Ctrl Pts',(0.232041893106022,2.32421678787079,6.17726469585986));
#58331=CARTESIAN_POINT('Ctrl Pts',(0.217556859123327,2.33779227316138,6.17858516935142));
#58332=CARTESIAN_POINT('Ctrl Pts',(0.214685798179649,2.34038751829849,6.17884393306726));
#58333=CARTESIAN_POINT('Ctrl Pts',(0.190799921314123,2.36120946110694,6.18097107783662));
#58334=CARTESIAN_POINT('Ctrl Pts',(0.167552267100266,2.37669726776595,6.1828943681863));
#58335=CARTESIAN_POINT('Ctrl Pts',(0.14125560781912,2.38967272776466,6.18474907791554));
#58336=CARTESIAN_POINT('Ctrl Pts',(0.139902695280505,2.39032855872838,6.18484363868768));
#58337=CARTESIAN_POINT('Ctrl Pts',(0.138159735427634,2.39115845412936,6.18496431306058));
#58338=CARTESIAN_POINT('Ctrl Pts',(0.137773892054862,2.39134123047982,6.18499095516205));
#58339=CARTESIAN_POINT('Ctrl Pts',(0.137162542943741,2.39162934417616,6.18503305317577));
#58340=CARTESIAN_POINT('Ctrl Pts',(0.136937278168955,2.39173518714768,6.18504854042471));
#58341=CARTESIAN_POINT('Ctrl Pts',(0.136517835007061,2.39193167397696,6.18507733148648));
#58342=CARTESIAN_POINT('Ctrl Pts',(0.136323690338754,2.39202238441391,6.18509063936819));
#58343=CARTESIAN_POINT('Ctrl Pts',(0.135886401403803,2.39222616830484,6.18512057254085));
#58344=CARTESIAN_POINT('Ctrl Pts',(0.135643206935435,2.39233913173253,6.18513719091932));
#58345=CARTESIAN_POINT('Ctrl Pts',(0.135134956191531,2.39257444260048,6.18517186224845));
#58346=CARTESIAN_POINT('Ctrl Pts',(0.134869873912707,2.39269673377103,6.18518991171519));
#58347=CARTESIAN_POINT('Ctrl Pts',(0.134178237582412,2.39301466927063,6.1852369185287));
#58348=CARTESIAN_POINT('Ctrl Pts',(0.133751419825575,2.39320974327198,6.18526584113607));
#58349=CARTESIAN_POINT('Ctrl Pts',(0.132487892979433,2.39378389610956,6.18535121255284));
#58350=CARTESIAN_POINT('Ctrl Pts',(0.131649979129677,2.39416033458195,6.18540750421858));
#58351=CARTESIAN_POINT('Ctrl Pts',(0.122366759348874,2.39828327300989,6.18602771841384));
#58352=CARTESIAN_POINT('Ctrl Pts',(0.113764811994164,2.40166892016873,6.18657104877395));
#58353=CARTESIAN_POINT('Ctrl Pts',(0.0783342367324629,2.41388242650221,
6.18872935709145));
#58354=CARTESIAN_POINT('Ctrl Pts',(0.0505460948361024,2.41953671657172,
6.19025251467767));
#58355=CARTESIAN_POINT('Ctrl Pts',(0.0206910924660686,2.42161452727039,
6.19197820487626));
#58356=CARTESIAN_POINT('Ctrl Pts',(0.0190061446707322,2.42171849776017,
6.19207585086633));
#58357=CARTESIAN_POINT('Ctrl Pts',(0.0138822380994547,2.42199427760851,
6.19237366253869));
#58358=CARTESIAN_POINT('Ctrl Pts',(0.0104413441416143,2.4221242128769,6.19257484892087));
#58359=CARTESIAN_POINT('Ctrl Pts',(-0.000136555521104034,2.42235399599426,
6.19319781080413));
#58360=CARTESIAN_POINT('Ctrl Pts',(-0.00727493791641535,2.42227190503922,
6.19362452448265));
#58361=CARTESIAN_POINT('Ctrl Pts',(-0.015464741360703,2.42190548944949,
6.19412336769333));
#58362=CARTESIAN_POINT('Ctrl Pts',(-0.0165249087877676,2.4218528075229,
6.19418812025241));
#58363=CARTESIAN_POINT('Ctrl Pts',(-0.0180878574252477,2.42176739871311,
6.19428384958939));
#58364=CARTESIAN_POINT('Ctrl Pts',(-0.0185908606579843,2.42173872840595,
6.19431469909012));
#58365=CARTESIAN_POINT('Ctrl Pts',(-0.0194876045951519,2.42168550562084,
6.19436977075608));
#58366=CARTESIAN_POINT('Ctrl Pts',(-0.019881372197351,2.42166140939931,
6.19439397855766));
#58367=CARTESIAN_POINT('Ctrl Pts',(-0.0207045761275696,2.42160951686937,
6.19444464046621));
#58368=CARTESIAN_POINT('Ctrl Pts',(-0.0211340027505667,2.42158158333221,
6.19447109883476));
#58369=CARTESIAN_POINT('Ctrl Pts',(-0.0222530168256028,2.42150654210776,
6.19454012491064));
#58370=CARTESIAN_POINT('Ctrl Pts',(-0.022942508260371,2.42145807608265,
6.19458273519188));
#58371=CARTESIAN_POINT('Ctrl Pts',(-0.0259229626274103,2.42123893487744,
6.19476727261138));
#58372=CARTESIAN_POINT('Ctrl Pts',(-0.0282121750117122,2.42104598738231,
6.19490989760952));
#58373=CARTESIAN_POINT('Ctrl Pts',(-0.0443069212725498,2.41951596477287,
6.19591909880909));
#58374=CARTESIAN_POINT('Ctrl Pts',(-0.058013717022465,2.41731352317646,
6.19681296385267));
#58375=CARTESIAN_POINT('Ctrl Pts',(-0.0853943256030159,2.41108042698548,
6.19866772861216));
#58376=CARTESIAN_POINT('Ctrl Pts',(-0.0990292777717138,2.40701200967548,
6.19962775076814));
#58377=CARTESIAN_POINT('Ctrl Pts',(-0.119053531608282,2.39956398881161,
6.20107355519886));
#58378=CARTESIAN_POINT('Ctrl Pts',(-0.125672115479725,2.3968481927999,6.20155742903898));
#58379=CARTESIAN_POINT('Ctrl Pts',(-0.13582566999223,2.39228139149973,6.20230487024037));
#58380=CARTESIAN_POINT('Ctrl Pts',(-0.139425916812929,2.39058121037036,
6.20257092174548));
#58381=CARTESIAN_POINT('Ctrl Pts',(-0.151662645588858,2.38452273563978,
6.20347680230383));
#58382=CARTESIAN_POINT('Ctrl Pts',(-0.160134857578551,2.37984212461508,
6.20410688688518));
#58383=CARTESIAN_POINT('Ctrl Pts',(-0.169004072429104,2.3744072286998,6.2047597472065));
#58384=CARTESIAN_POINT('Ctrl Pts',(-0.16962237869707,2.37402545927299,6.2048052235714));
#58385=CARTESIAN_POINT('Ctrl Pts',(-0.170482029679533,2.37349064853897,
6.20486839335763));
#58386=CARTESIAN_POINT('Ctrl Pts',(-0.17072446415343,2.37333937627609,6.20488620179406));
#58387=CARTESIAN_POINT('Ctrl Pts',(-0.171142188317985,2.37307795564847,
6.20491687496185));
#58388=CARTESIAN_POINT('Ctrl Pts',(-0.171317573109749,2.37296796080814,
6.20492974983965));
#58389=CARTESIAN_POINT('Ctrl Pts',(-0.171677408627946,2.37274180190721,
6.20495615774185));
#58390=CARTESIAN_POINT('Ctrl Pts',(-0.171861847190943,2.37262561989136,
6.20496968945391));
#58391=CARTESIAN_POINT('Ctrl Pts',(-0.17229538727339,2.3723519084127,6.20500148786805));
#58392=CARTESIAN_POINT('Ctrl Pts',(-0.172544391626592,2.37219422369256,
6.20501974423289));
#58393=CARTESIAN_POINT('Ctrl Pts',(-0.173070877623897,2.37185980793827,
6.20505833058906));
#58394=CARTESIAN_POINT('Ctrl Pts',(-0.173348305949448,2.37168299299085,
6.20507865501474));
#58395=CARTESIAN_POINT('Ctrl Pts',(-0.174096244706551,2.3712046929443,6.20513342777145));
#58396=CARTESIAN_POINT('Ctrl Pts',(-0.174566245173121,2.37090240669463,
6.20516782385659));
#58397=CARTESIAN_POINT('Ctrl Pts',(-0.176014790128062,2.36996542307415,
6.20527377008675));
#58398=CARTESIAN_POINT('Ctrl Pts',(-0.176990689963075,2.36932662653336,
6.20534505845735));
#58399=CARTESIAN_POINT('Ctrl Pts',(-0.190327293992514,2.36049306530224,
6.20631837449763));
#58400=CARTESIAN_POINT('Ctrl Pts',(-0.202113182387467,2.35145873517464,
6.20716814245826));
#58401=CARTESIAN_POINT('Ctrl Pts',(-0.231657197921143,2.32538788719773,
6.20938918311929));
#58402=CARTESIAN_POINT('Ctrl Pts',(-0.248158216252713,2.30708025181392,
6.21073517352927));
#58403=CARTESIAN_POINT('Ctrl Pts',(-0.268076790689056,2.2791396122804,6.21273221293303));
#58404=CARTESIAN_POINT('Ctrl Pts',(-0.273370966253454,2.27095160814391,
6.21331054495667));
#58405=CARTESIAN_POINT('Ctrl Pts',(-0.278809954789398,2.26163930603782,
6.21396631955806));
#58406=CARTESIAN_POINT('Ctrl Pts',(-0.279329858391319,2.2607391872492,6.21402968384572));
#58407=CARTESIAN_POINT('Ctrl Pts',(-0.280101160555895,2.25938877446129,
6.21412471963403));
#58408=CARTESIAN_POINT('Ctrl Pts',(-0.280355851257774,2.25894036060636,
6.21415627245991));
#58409=CARTESIAN_POINT('Ctrl Pts',(-0.280792742654014,2.25816684288156,
6.21421069447979));
#58410=CARTESIAN_POINT('Ctrl Pts',(-0.280975458276061,2.2578420297606,6.21423354512098));
#58411=CARTESIAN_POINT('Ctrl Pts',(-0.28135149304452,2.25717083171431,6.21428076003648));
#58412=CARTESIAN_POINT('Ctrl Pts',(-0.281544736823294,2.256824405451,6.21430512696485));
#58413=CARTESIAN_POINT('Ctrl Pts',(-0.281993217969672,2.25601691693269,
6.21436191950979));
#58414=CARTESIAN_POINT('Ctrl Pts',(-0.282247964445309,2.25555558463549,
6.21439436261762));
#58415=CARTESIAN_POINT('Ctrl Pts',(-0.283056882239348,2.25408214855741,
6.21449797208943));
#58416=CARTESIAN_POINT('Ctrl Pts',(-0.28360674522256,2.25306770102113,6.21456929184038));
#58417=CARTESIAN_POINT('Ctrl Pts',(-0.295863117904717,2.23016303361312,
6.21617935198832));
#58418=CARTESIAN_POINT('Ctrl Pts',(-0.305004471569212,2.20700079237407,
6.21781281550682));
#58419=CARTESIAN_POINT('Ctrl Pts',(-0.31783436978374,2.15888022072901,6.22117310277374));
#58420=CARTESIAN_POINT('Ctrl Pts',(-0.321442388459736,2.13406720704661,
6.22288731729675));
#58421=CARTESIAN_POINT('Ctrl Pts',(-0.322180928912625,2.10787908649388,
6.22453982131179));
#58422=CARTESIAN_POINT('Ctrl Pts',(-0.322208166065209,2.10667298951083,
6.22461556572644));
#58423=CARTESIAN_POINT('Ctrl Pts',(-0.322235274014918,2.10507515450673,
6.2247154072277));
#58424=CARTESIAN_POINT('Ctrl Pts',(-0.322241203734308,2.10468354913219,
6.2247398367413));
#58425=CARTESIAN_POINT('Ctrl Pts',(-0.32224930866881,2.10407501515372,6.22477773551545));
#58426=CARTESIAN_POINT('Ctrl Pts',(-0.322251978718531,2.10385809521546,
6.2247912325156));
#58427=CARTESIAN_POINT('Ctrl Pts',(-0.322256864196161,2.10342571607582,
6.22481811045619));
#58428=CARTESIAN_POINT('Ctrl Pts',(-0.322259082556228,2.1032102589536,6.22483149140035));
#58429=CARTESIAN_POINT('Ctrl Pts',(-0.322263047337864,2.1027836208533,6.22485796311304));
#58430=CARTESIAN_POINT('Ctrl Pts',(-0.322264802252337,2.10257244133396,
6.22487105430052));
#58431=CARTESIAN_POINT('Ctrl Pts',(-0.322268314639747,2.10209306824478,
6.22490074427885));
#58432=CARTESIAN_POINT('Ctrl Pts',(-0.322269944911836,2.10182487346972,
6.22491733592495));
#58433=CARTESIAN_POINT('Ctrl Pts',(-0.322273682472704,2.10105110390097,
6.22496515051638));
#58434=CARTESIAN_POINT('Ctrl Pts',(-0.322274934869778,2.10054552339395,
6.22499632600572));
#58435=CARTESIAN_POINT('Ctrl Pts',(-0.322274997525276,2.1000399384962,6.22502743709318));
#58436=CARTESIAN_POINT('',(-0.322274881329742,2.10027656626812,6.34972265506687));
#58437=CARTESIAN_POINT('Ctrl Pts',(-0.322274999303774,2.10002118378279,
6.22472265507673));
#58438=CARTESIAN_POINT('Ctrl Pts',(-0.322276158268471,2.08238951947228,
6.22581786979066));
#58439=CARTESIAN_POINT('Ctrl Pts',(-0.320826057348452,2.06470156024196,
6.22691308450459));
#58440=CARTESIAN_POINT('Ctrl Pts',(-0.317923029073763,2.04721625998887,
6.22800829921852));
#58441=CARTESIAN_POINT('Ctrl Pts',(-0.31502554512302,2.02976435388827,6.22910142224591));
#58442=CARTESIAN_POINT('Ctrl Pts',(-0.310680702994432,2.01251510674329,
6.23019454527331));
#58443=CARTESIAN_POINT('Ctrl Pts',(-0.304938651877089,1.9957234723613,6.2312876683007));
#58444=CARTESIAN_POINT('Ctrl Pts',(-0.299197597929198,1.97893475402875,
6.23238060149542));
#58445=CARTESIAN_POINT('Ctrl Pts',(-0.292060016039921,1.96260424113098,
6.23347353469014));
#58446=CARTESIAN_POINT('Ctrl Pts',(-0.283626232167341,1.94697276042626,
6.23456646788487));
#58447=CARTESIAN_POINT('Ctrl Pts',(-0.275194890595358,1.93134580636999,
6.2356590845821));
#58448=CARTESIAN_POINT('Ctrl Pts',(-0.265468469318602,1.91641816256849,
6.23675170127934));
#58449=CARTESIAN_POINT('Ctrl Pts',(-0.254593111913849,1.9024056605289,6.23784431797657));
#58450=CARTESIAN_POINT('Ctrl Pts',(-0.243691529540873,1.88835936857261,
6.23893956942291));
#58451=CARTESIAN_POINT('Ctrl Pts',(-0.231635973261083,1.87523322977712,
6.24003482086925));
#58452=CARTESIAN_POINT('Ctrl Pts',(-0.218613162004877,1.86321009095988,
6.24113007231559));
#58453=CARTESIAN_POINT('Ctrl Pts',(-0.205721904410726,1.8513084073269,6.2422142597654));
#58454=CARTESIAN_POINT('Ctrl Pts',(-0.191883510059295,1.84048790191718,
6.2432984472152));
#58455=CARTESIAN_POINT('Ctrl Pts',(-0.177308771851876,1.83088520098408,
6.244382634665));
#58456=CARTESIAN_POINT('Ctrl Pts',(-0.162558307939585,1.82116672154669,
6.24547989402053));
#58457=CARTESIAN_POINT('Ctrl Pts',(-0.146960238062366,1.81263413867367,
6.24657715337606));
#58458=CARTESIAN_POINT('Ctrl Pts',(-0.130730780769772,1.80543143653077,
6.24767441273159));
#58459=CARTESIAN_POINT('Ctrl Pts',(-0.114532370010416,1.79824251297131,
6.24876957305827));
#58460=CARTESIAN_POINT('Ctrl Pts',(-0.0977056422412874,1.79237878939909,
6.24986473338495));
#58461=CARTESIAN_POINT('Ctrl Pts',(-0.0804919229730219,1.78793874645976,
6.25095989371163));
#58462=CARTESIAN_POINT('Ctrl Pts',(-0.0630802086934335,1.78344763342115,
6.25206765075131));
#58463=CARTESIAN_POINT('Ctrl Pts',(-0.0452732803213705,1.78041349834926,
6.25317540779099));
#58464=CARTESIAN_POINT('Ctrl Pts',(-0.0273374283460662,1.77888656110897,
6.25428316483067));
#58465=CARTESIAN_POINT('Ctrl Pts',(-0.00961411907978619,1.77737771831872,
6.2553777947726));
#58466=CARTESIAN_POINT('Ctrl Pts',(0.00823428241176009,1.7773405276635,
6.25647242471453));
#58467=CARTESIAN_POINT('Ctrl Pts',(0.0259463163571276,1.77877116522252,
6.25756705465645));
#58468=CARTESIAN_POINT('Ctrl Pts',(0.0439769615409925,1.78022753766925,
6.25868137524501));
#58469=CARTESIAN_POINT('Ctrl Pts',(0.0618654546753276,1.78320505426578,
6.25979569583357));
#58470=CARTESIAN_POINT('Ctrl Pts',(0.0793435882414551,1.78764480053956,
6.26091001642212));
#58471=CARTESIAN_POINT('Ctrl Pts',(0.0968217218075841,1.79208454681334,
6.26202433701068));
#58472=CARTESIAN_POINT('Ctrl Pts',(0.113888723803027,1.79798619566923,6.26313865759923));
#58473=CARTESIAN_POINT('Ctrl Pts',(0.130296099377664,1.80523890671941,6.26425297818779));
#58474=CARTESIAN_POINT('Ctrl Pts',(0.146452263531704,1.8123805723536,6.26535023754332));
#58475=CARTESIAN_POINT('Ctrl Pts',(0.162070129045757,1.82087686749704,6.26644749689885));
#58476=CARTESIAN_POINT('Ctrl Pts',(0.176911588447618,1.83062393295257,6.26754475625438));
#58477=CARTESIAN_POINT('Ctrl Pts',(0.191724656520408,1.84035235252326,6.26863991658106));
#58478=CARTESIAN_POINT('Ctrl Pts',(0.205763592067393,1.85132642698334,6.26973507690774));
#58479=CARTESIAN_POINT('Ctrl Pts',(0.218814956939098,1.86339655487559,6.27083023723442));
#58480=CARTESIAN_POINT('Ctrl Pts',(0.232016440741833,1.87560551535082,6.2719379942741));
#58481=CARTESIAN_POINT('Ctrl Pts',(0.244206807913172,1.88893546741038,6.27304575131378));
#58482=CARTESIAN_POINT('Ctrl Pts',(0.255199684838193,1.90318969416342,6.27415350835346));
#58483=CARTESIAN_POINT('Ctrl Pts',(0.26606229441685,1.91727500605403,6.27524813829539));
#58484=CARTESIAN_POINT('Ctrl Pts',(0.275755227213166,1.93226212961909,6.27634276823731));
#58485=CARTESIAN_POINT('Ctrl Pts',(0.284140165549627,1.9479291548441,6.27743739817924));
#58486=CARTESIAN_POINT('Ctrl Pts',(0.29267593555208,1.96387800486268,6.2785517187678));
#58487=CARTESIAN_POINT('Ctrl Pts',(0.29985575084529,1.98053075370649,6.27966603935635));
#58488=CARTESIAN_POINT('Ctrl Pts',(0.305583962196553,1.99762999622323,6.28078035994491));
#58489=CARTESIAN_POINT('Ctrl Pts',(0.311312173547817,2.01472923873997,6.28189468053347));
#58490=CARTESIAN_POINT('Ctrl Pts',(0.315588638085686,2.03227414875362,6.28300900112202));
#58491=CARTESIAN_POINT('Ctrl Pts',(0.318372037640385,2.04999578744036,6.28412332171058));
#58492=CARTESIAN_POINT('Ctrl Pts',(0.321112820887983,2.06744609217674,6.28522058106611));
#58493=CARTESIAN_POINT('Ctrl Pts',(0.322423216610124,2.08517707120868,6.28631784042164));
#58494=CARTESIAN_POINT('Ctrl Pts',(0.322261659602295,2.10293229865033,6.28741509977716));
#58495=CARTESIAN_POINT('Ctrl Pts',(0.322100411648855,2.12065356079979,6.28851026010384));
#58496=CARTESIAN_POINT('Ctrl Pts',(0.320472742837832,2.13839821396037,6.28960542043052));
#58497=CARTESIAN_POINT('Ctrl Pts',(0.317388902826077,2.15590581354259,6.2907005807572));
#58498=CARTESIAN_POINT('Ctrl Pts',(0.314269591982681,2.17361478839553,6.29180833779688));
#58499=CARTESIAN_POINT('Ctrl Pts',(0.309660395642225,2.191080411281,6.29291609483656));
#58500=CARTESIAN_POINT('Ctrl Pts',(0.303625829483311,2.20803948951921,6.29402385187624));
#58501=CARTESIAN_POINT('Ctrl Pts',(0.297662773896685,2.2247975999731,6.29511848181817));
#58502=CARTESIAN_POINT('Ctrl Pts',(0.290308291730793,2.24106039220014,6.2962131117601));
#58503=CARTESIAN_POINT('Ctrl Pts',(0.281674095040921,2.25659144232007,6.29730774170203));
#58504=CARTESIAN_POINT('Ctrl Pts',(0.272884582924865,2.27240187125833,6.29842206229058));
#58505=CARTESIAN_POINT('Ctrl Pts',(0.262769217289018,2.28745322235227,6.29953638287914));
#58506=CARTESIAN_POINT('Ctrl Pts',(0.251492652336189,2.30152573395452,6.30065070346769));
#58507=CARTESIAN_POINT('Ctrl Pts',(0.24021608738336,2.31559824555678,6.30176502405625));
#58508=CARTESIAN_POINT('Ctrl Pts',(0.227778940438234,2.32869135031448,6.30287934464481));
#58509=CARTESIAN_POINT('Ctrl Pts',(0.21438497380719,2.34062472572595,6.30399366523336));
#58510=CARTESIAN_POINT('Ctrl Pts',(0.201196080642618,2.35237539061337,6.30509092458889));
#58511=CARTESIAN_POINT('Ctrl Pts',(0.186996896892048,2.36307529412683,6.30618818394442));
#58512=CARTESIAN_POINT('Ctrl Pts',(0.171980530035207,2.37255067953283,6.30728544329995));
#58513=CARTESIAN_POINT('Ctrl Pts',(0.156992889100883,2.38200793877093,6.30838060362663));
#58514=CARTESIAN_POINT('Ctrl Pts',(0.141191780478856,2.39024486707358,6.30947576395331));
#58515=CARTESIAN_POINT('Ctrl Pts',(0.124801738967505,2.39712909917355,6.31057092427999));
#58516=CARTESIAN_POINT('Ctrl Pts',(0.108223176520971,2.40409251483585,6.31167868131967));
#58517=CARTESIAN_POINT('Ctrl Pts',(0.0910427268256701,2.40967147727965,
6.31278643835936));
#58518=CARTESIAN_POINT('Ctrl Pts',(0.0735166105016287,2.41377776148948,
6.31389419539904));
#58519=CARTESIAN_POINT('Ctrl Pts',(0.0561981814537302,2.41783538557594,
6.31498882534096));
#58520=CARTESIAN_POINT('Ctrl Pts',(0.0385430204904939,2.42045494857589,
6.31608345528289));
#58521=CARTESIAN_POINT('Ctrl Pts',(0.0208103887975029,2.42160239946726,
6.31717808522482));
#58522=CARTESIAN_POINT('Ctrl Pts',(0.00275877534540055,2.42277049116988,
6.31829240581338));
#58523=CARTESIAN_POINT('Ctrl Pts',(-0.0153723003312898,2.42241287894167,
6.31940672640193));
#58524=CARTESIAN_POINT('Ctrl Pts',(-0.0333089284096789,2.42054904603383,
6.32052104699049));
#58525=CARTESIAN_POINT('Ctrl Pts',(-0.0512455564880679,2.41868521312599,
6.32163536757905));
#58526=CARTESIAN_POINT('Ctrl Pts',(-0.0689869257586935,2.41531537147781,
6.3227496881676));
#58527=CARTESIAN_POINT('Ctrl Pts',(-0.0862711176153947,2.41051323625635,
6.32386400875616));
#58528=CARTESIAN_POINT('Ctrl Pts',(-0.10329067321931,2.40578462596917,6.32496126811169));
#58529=CARTESIAN_POINT('Ctrl Pts',(-0.119973618395755,2.39963774915087,
6.32605852746721));
#58530=CARTESIAN_POINT('Ctrl Pts',(-0.136069322804202,2.39214091636846,
6.32715578682274));
#58531=CARTESIAN_POINT('Ctrl Pts',(-0.152134236545231,2.38465842483382,
6.32825094714942));
#58532=CARTESIAN_POINT('Ctrl Pts',(-0.167613418944239,2.37583136791738,
6.3293461074761));
#58533=CARTESIAN_POINT('Ctrl Pts',(-0.182274030171178,2.36577688678694,
6.33044126780278));
#58534=CARTESIAN_POINT('Ctrl Pts',(-0.197103270143636,2.35560675737187,
6.33154902484246));
#58535=CARTESIAN_POINT('Ctrl Pts',(-0.211094249505374,2.34418112083898,
6.33265678188215));
#58536=CARTESIAN_POINT('Ctrl Pts',(-0.224034090232527,2.33166765427803,
6.33376453892183));
#58537=CARTESIAN_POINT('Ctrl Pts',(-0.23682059178146,2.31930247429337,6.33485916886375));
#58538=CARTESIAN_POINT('Ctrl Pts',(-0.248580224891392,2.30587571563507,
6.33595379880568));
#58539=CARTESIAN_POINT('Ctrl Pts',(-0.25914401608899,2.29158693731638,6.33704842874761));
#58540=CARTESIAN_POINT('Ctrl Pts',(-0.269897833040104,2.27704112666752,
6.33816274933617));
#58541=CARTESIAN_POINT('Ctrl Pts',(-0.279411825147348,2.26160261165204,
6.33927706992472));
#58542=CARTESIAN_POINT('Ctrl Pts',(-0.287554101940797,2.2455122471891,6.34039139051328));
#58543=CARTESIAN_POINT('Ctrl Pts',(-0.295696378734246,2.22942188272616,
6.34150571110184));
#58544=CARTESIAN_POINT('Ctrl Pts',(-0.302466679293908,2.21268046562178,
6.34262003169039));
#58545=CARTESIAN_POINT('Ctrl Pts',(-0.307785203377992,2.19554812508139,
6.34373435227895));
#58546=CARTESIAN_POINT('Ctrl Pts',(-0.314114228816402,2.17516069853496,
6.34506038996159));
#58547=CARTESIAN_POINT('Ctrl Pts',(-0.318421557416576,2.15411748845562,
6.34638642764423));
#58548=CARTESIAN_POINT('Ctrl Pts',(-0.320603011129514,2.13278543700622,
6.34771246532687));
#58549=CARTESIAN_POINT('Ctrl Pts',(-0.321705326679427,2.12200608749046,
6.34838252857354));
#58550=CARTESIAN_POINT('Ctrl Pts',(-0.32226554723971,2.11115331843988,6.3490525918202));
#58551=CARTESIAN_POINT('Ctrl Pts',(-0.322274881329742,2.10027656626812,
6.34972265506687));
#58552=CARTESIAN_POINT('',(-0.32227496222964,2.09984397152879,6.47472265507269));
#58553=CARTESIAN_POINT('Ctrl Pts',(-0.322274881329823,2.10027656617378,
6.34972265507268));
#58554=CARTESIAN_POINT('Ctrl Pts',(-0.322290035910069,2.0826173546965,6.35081055230423));
#58555=CARTESIAN_POINT('Ctrl Pts',(-0.320849399698483,2.0649328324212,6.35189844953578));
#58556=CARTESIAN_POINT('Ctrl Pts',(-0.317966904445043,2.04748121000407,
6.35298634676733));
#58557=CARTESIAN_POINT('Ctrl Pts',(-0.315083192672738,2.03002222236131,
6.35407470313147));
#58558=CARTESIAN_POINT('Ctrl Pts',(-0.310756513550684,2.01279710640944,
6.35516305949561));
#58559=CARTESIAN_POINT('Ctrl Pts',(-0.305052384133251,1.99605665697304,
6.35625141585975));
#58560=CARTESIAN_POINT('Ctrl Pts',(-0.2993465896174,1.97931132081445,6.35734008992714));
#58561=CARTESIAN_POINT('Ctrl Pts',(-0.292262834855402,1.96305165988339,
6.35842876399452));
#58562=CARTESIAN_POINT('Ctrl Pts',(-0.283915241013496,1.94750963458222,
6.35951743806191));
#58563=CARTESIAN_POINT('Ctrl Pts',(-0.275549064599905,1.9319330111915,6.36060853562573));
#58564=CARTESIAN_POINT('Ctrl Pts',(-0.265913864312675,1.91707786596012,
6.36169963318956));
#58565=CARTESIAN_POINT('Ctrl Pts',(-0.255167702714323,1.90314823059852,
6.36279073075338));
#58566=CARTESIAN_POINT('Ctrl Pts',(-0.252495469959852,1.8996843679411,6.36306205243616));
#58567=CARTESIAN_POINT('Ctrl Pts',(-0.249754728417259,1.8962775673472,6.36333337411895));
#58568=CARTESIAN_POINT('Ctrl Pts',(-0.246948266213006,1.89293061684694,
6.36360469580174));
#58569=CARTESIAN_POINT('Ctrl Pts',(-0.235598576509175,1.87939512380717,
6.36470195515727));
#58570=CARTESIAN_POINT('Ctrl Pts',(-0.223097178713936,1.86675313790524,
6.3657992145128));
#58571=CARTESIAN_POINT('Ctrl Pts',(-0.209610004229396,1.85520453077732,
6.36689647386832));
#58572=CARTESIAN_POINT('Ctrl Pts',(-0.196148630361804,1.84367801583699,
6.367991634195));
#58573=CARTESIAN_POINT('Ctrl Pts',(-0.181705762025049,1.83324127421161,
6.36908679452169));
#58574=CARTESIAN_POINT('Ctrl Pts',(-0.166484416736886,1.82405776943574,
6.37018195484837));
#58575=CARTESIAN_POINT('Ctrl Pts',(-0.151087993048431,1.81476863448759,
6.37128971188805));
#58576=CARTESIAN_POINT('Ctrl Pts',(-0.134895678978682,1.80676228458587,
6.37239746892772));
#58577=CARTESIAN_POINT('Ctrl Pts',(-0.118148231707899,1.80016309271656,
6.3735052259674));
#58578=CARTESIAN_POINT('Ctrl Pts',(-0.101599244360684,1.79364210232434,
6.37459985590933));
#58579=CARTESIAN_POINT('Ctrl Pts',(-0.0845089737811362,1.7884953100742,
6.37569448585126));
#58580=CARTESIAN_POINT('Ctrl Pts',(-0.0671290249930131,1.78479392514025,
6.37678911579319));
#58581=CARTESIAN_POINT('Ctrl Pts',(-0.0494364386486706,1.78102595819536,
6.37790343638174));
#58582=CARTESIAN_POINT('Ctrl Pts',(-0.0314444485246837,1.77875613814127,
6.3790177569703));
#58583=CARTESIAN_POINT('Ctrl Pts',(-0.0134269008111419,1.77800482308021,
6.38013207755886));
#58584=CARTESIAN_POINT('Ctrl Pts',(0.00459064690239998,1.77725350801914,
6.38124639814741));
#58585=CARTESIAN_POINT('Ctrl Pts',(0.0226329188654116,1.77802060562909,
6.38236071873597));
#58586=CARTESIAN_POINT('Ctrl Pts',(0.0404300862316696,1.78027107770441,
6.38347503932452));
#58587=CARTESIAN_POINT('Ctrl Pts',(0.0579547632367289,1.78248709306333,
6.38457229868005));
#58588=CARTESIAN_POINT('Ctrl Pts',(0.0753516038425314,1.78615515676448,
6.38566955803558));
#58589=CARTESIAN_POINT('Ctrl Pts',(0.0923627307326406,1.79124394484219,
6.38676681739111));
#58590=CARTESIAN_POINT('Ctrl Pts',(0.109341315775737,1.79632299819956,6.38786197771779));
#58591=CARTESIAN_POINT('Ctrl Pts',(0.125934900594545,1.80281722366599,6.38895713804447));
#58592=CARTESIAN_POINT('Ctrl Pts',(0.141896145071832,1.8106444062425,6.39005229837115));
#58593=CARTESIAN_POINT('Ctrl Pts',(0.15804097839077,1.81856161835178,6.39116005541083));
#58594=CARTESIAN_POINT('Ctrl Pts',(0.173538052919404,1.82784242406768,6.39226781245051));
#58595=CARTESIAN_POINT('Ctrl Pts',(0.188152467412437,1.83835171578699,6.39337556949019));
#58596=CARTESIAN_POINT('Ctrl Pts',(0.202593698760813,1.84873647072182,6.39447019943212));
#58597=CARTESIAN_POINT('Ctrl Pts',(0.216172486101175,1.86032022457424,6.39556482937405));
#58598=CARTESIAN_POINT('Ctrl Pts',(0.228692757139418,1.87292997014804,6.39665945931598));
#58599=CARTESIAN_POINT('Ctrl Pts',(0.24143824788276,1.88576654493111,6.39777377990453));
#58600=CARTESIAN_POINT('Ctrl Pts',(0.253086142572723,1.89966583775454,6.39888810049309));
#58601=CARTESIAN_POINT('Ctrl Pts',(0.263471085861674,1.91440861404723,6.40000242108165));
#58602=CARTESIAN_POINT('Ctrl Pts',(0.273856029150626,1.92915139033992,6.4011167416702));
#58603=CARTESIAN_POINT('Ctrl Pts',(0.282977647562523,1.94473689943903,6.40223106225876));
#58604=CARTESIAN_POINT('Ctrl Pts',(0.290719338618049,1.96091929760573,6.40334538284732));
#58605=CARTESIAN_POINT('Ctrl Pts',(0.298342497541543,1.97685392895477,6.40444264220285));
#58606=CARTESIAN_POINT('Ctrl Pts',(0.304675548068079,1.99346709317499,6.40553990155837));
#58607=CARTESIAN_POINT('Ctrl Pts',(0.309605234297894,2.01052500617297,6.4066371609139));
#58608=CARTESIAN_POINT('Ctrl Pts',(0.314525490165093,2.02755028782334,6.40773232124058));
#58609=CARTESIAN_POINT('Ctrl Pts',(0.31804743640729,2.0450179126251,6.40882748156726));
#58610=CARTESIAN_POINT('Ctrl Pts',(0.320106311193014,2.06267540811474,6.40992264189395));
#58611=CARTESIAN_POINT('Ctrl Pts',(0.322188867492893,2.0805360030023,6.41103039893363));
#58612=CARTESIAN_POINT('Ctrl Pts',(0.322774246336576,2.09859008855908,6.4121381559733));
#58613=CARTESIAN_POINT('Ctrl Pts',(0.321848892327374,2.11656701942543,6.41324591301298));
#58614=CARTESIAN_POINT('Ctrl Pts',(0.320934503910896,2.13433092079134,6.41434054295491));
#58615=CARTESIAN_POINT('Ctrl Pts',(0.318545119212261,2.1520187035724,6.41543517289684));
#58616=CARTESIAN_POINT('Ctrl Pts',(0.314720068304024,2.16937185475184,6.41652980283877));
#58617=CARTESIAN_POINT('Ctrl Pts',(0.310826210831224,2.18703716144127,6.41764412342732));
#58618=CARTESIAN_POINT('Ctrl Pts',(0.305444652426788,2.20435485819457,6.41875844401588));
#58619=CARTESIAN_POINT('Ctrl Pts',(0.298670219605893,2.22106723564023,6.41987276460443));
#58620=CARTESIAN_POINT('Ctrl Pts',(0.291895786784999,2.23777961308589,6.42098708519299));
#58621=CARTESIAN_POINT('Ctrl Pts',(0.283728908549072,2.2538859508512,6.42210140578155));
#58622=CARTESIAN_POINT('Ctrl Pts',(0.274313175686482,2.2691551278259,6.4232157263701));
#58623=CARTESIAN_POINT('Ctrl Pts',(0.265041606015477,2.2841905202065,6.42431298572563));
#58624=CARTESIAN_POINT('Ctrl Pts',(0.254501154771622,2.29850846845181,6.42541024508116));
#58625=CARTESIAN_POINT('Ctrl Pts',(0.242827084341463,2.31188719341957,6.42650750443669));
#58626=CARTESIAN_POINT('Ctrl Pts',(0.231175346106956,2.32524032523152,6.42760266476337));
#58627=CARTESIAN_POINT('Ctrl Pts',(0.218394747565007,2.33765718161538,6.42869782509005));
#58628=CARTESIAN_POINT('Ctrl Pts',(0.204662515333758,2.34894664175734,6.42979298541673));
#58629=CARTESIAN_POINT('Ctrl Pts',(0.190772332723877,2.36036595511428,6.43090074245641));
#58630=CARTESIAN_POINT('Ctrl Pts',(0.175909010485664,2.37063115485541,6.43200849949609));
#58631=CARTESIAN_POINT('Ctrl Pts',(0.160292774302096,2.37958433813706,6.43311625653577));
#58632=CARTESIAN_POINT('Ctrl Pts',(0.144861593010141,2.38843142476762,6.4342108864777));
#58633=CARTESIAN_POINT('Ctrl Pts',(0.128695971448153,2.39599710374989,6.43530551641963));
#58634=CARTESIAN_POINT('Ctrl Pts',(0.112034562068085,2.40217450674604,6.43640014636155));
#58635=CARTESIAN_POINT('Ctrl Pts',(0.0950734405096114,2.40846303136862,
6.43751446695011));
#58636=CARTESIAN_POINT('Ctrl Pts',(0.0775992762138262,2.41331250287217,
6.43862878753866));
#58637=CARTESIAN_POINT('Ctrl Pts',(0.0598800871405084,2.41666315034914,
6.43974310812722));
#58638=CARTESIAN_POINT('Ctrl Pts',(0.0421608980671892,2.42001379782612,
6.44085742871578));
#58639=CARTESIAN_POINT('Ctrl Pts',(0.024197522144825,2.42186559203785,6.44197174930433));
#58640=CARTESIAN_POINT('Ctrl Pts',(0.00626201842926354,2.42221415665702,
6.44308606989289));
#58641=CARTESIAN_POINT('Ctrl Pts',(-0.0113988768733321,2.42255738444381,
6.44418332924842));
#58642=CARTESIAN_POINT('Ctrl Pts',(-0.0291434008242062,2.42144534841178,
6.44528058860395));
#58643=CARTESIAN_POINT('Ctrl Pts',(-0.0467118575758495,2.41887172654033,
6.44637784795948));
#58644=CARTESIAN_POINT('Ctrl Pts',(-0.0642467063228147,2.41630302794115,
6.44747300828616));
#58645=CARTESIAN_POINT('Ctrl Pts',(-0.0816053904080379,2.41227834057728,
6.44856816861284));
#58646=CARTESIAN_POINT('Ctrl Pts',(-0.0985312760586869,2.40684322261254,
6.44966332893952));
#58647=CARTESIAN_POINT('Ctrl Pts',(-0.115651846011373,2.40134558903299,
6.4507710859792));
#58648=CARTESIAN_POINT('Ctrl Pts',(-0.132328794636532,2.39440497967673,
6.45187884301888));
#58649=CARTESIAN_POINT('Ctrl Pts',(-0.148310142254628,2.38612108857862,
6.45298660005856));
#58650=CARTESIAN_POINT('Ctrl Pts',(-0.164102108352333,2.37793536291237,
6.45408123000049));
#58651=CARTESIAN_POINT('Ctrl Pts',(-0.179214209745205,2.3684384576038,6.45517585994242));
#58652=CARTESIAN_POINT('Ctrl Pts',(-0.193427402736963,2.35777318614517,
6.45627048988434));
#58653=CARTESIAN_POINT('Ctrl Pts',(-0.207896268399406,2.346916063465,6.4573848104729));
#58654=CARTESIAN_POINT('Ctrl Pts',(-0.221432871737814,2.33484857981022,
6.45849913106146));
#58655=CARTESIAN_POINT('Ctrl Pts',(-0.233841873338553,2.32176373440785,
6.45961345165001));
#58656=CARTESIAN_POINT('Ctrl Pts',(-0.246250874939294,2.30867888900548,
6.46072777223857));
#58657=CARTESIAN_POINT('Ctrl Pts',(-0.25753179663213,2.29457737057338,6.46184209282713));
#58658=CARTESIAN_POINT('Ctrl Pts',(-0.26753368823998,2.27968556225171,6.46295641341568));
#58659=CARTESIAN_POINT('Ctrl Pts',(-0.277547582711622,2.26477588287585,
6.46407207125511));
#58660=CARTESIAN_POINT('Ctrl Pts',(-0.286340890299472,2.24898295014912,
6.46518772909454));
#58661=CARTESIAN_POINT('Ctrl Pts',(-0.293764094382879,2.23252861002971,
6.46630338693396));
#58662=CARTESIAN_POINT('Ctrl Pts',(-0.301170835693589,2.21611076143852,
6.46741657052895));
#58663=CARTESIAN_POINT('Ctrl Pts',(-0.307213145628115,2.1990350556288,6.46852975412393));
#58664=CARTESIAN_POINT('Ctrl Pts',(-0.311786712349425,2.18154889102457,
6.46964293771892));
#58665=CARTESIAN_POINT('Ctrl Pts',(-0.316353640034259,2.16408810951666,
6.47075450540516));
#58666=CARTESIAN_POINT('Ctrl Pts',(-0.319455832526156,2.14621875250001,
6.47186607309139));
#58667=CARTESIAN_POINT('Ctrl Pts',(-0.321038463309149,2.12820426742712,
6.47297764077763));
#58668=CARTESIAN_POINT('Ctrl Pts',(-0.32186663700003,2.11877748086864,6.47355931220932));
#58669=CARTESIAN_POINT('Ctrl Pts',(-0.322279545747959,2.10931117441553,
6.474140983641));
#58670=CARTESIAN_POINT('Ctrl Pts',(-0.32227496222964,2.09984397152879,6.47472265507269));
#58671=CARTESIAN_POINT('',(-0.322274913684313,2.10027657538795,6.72483363319554));
#58672=CARTESIAN_POINT('Ctrl Pts',(-0.322274953602036,2.09982706704832,
6.47445952331017));
#58673=CARTESIAN_POINT('Ctrl Pts',(-0.322258535437458,2.06923045040549,
6.47642514822576));
#58674=CARTESIAN_POINT('Ctrl Pts',(-0.317884570239021,2.03879330021116,
6.47852897207899));
#58675=CARTESIAN_POINT('Ctrl Pts',(-0.306838273958802,2.00106826228417,
6.48115616092435));
#58676=CARTESIAN_POINT('Ctrl Pts',(-0.304048970120985,1.99280175273676,
6.48173152784109));
#58677=CARTESIAN_POINT('Ctrl Pts',(-0.299669851892031,1.98137662812439,
6.48251722348514));
#58678=CARTESIAN_POINT('Ctrl Pts',(-0.298358508655174,1.97811592673419,
6.48274032867299));
#58679=CARTESIAN_POINT('Ctrl Pts',(-0.296789597914498,1.97439192923526,
6.48299329123514));
#58680=CARTESIAN_POINT('Ctrl Pts',(-0.296583978079407,1.97390718962834,
6.48302618223395));
#58681=CARTESIAN_POINT('Ctrl Pts',(-0.296270956595319,1.97317425721332,
6.48307585650819));
#58682=CARTESIAN_POINT('Ctrl Pts',(-0.296164430304366,1.97292569504783,
6.48309269273285));
#58683=CARTESIAN_POINT('Ctrl Pts',(-0.295979655634586,1.97249604716068,
6.48312177701995));
#58684=CARTESIAN_POINT('Ctrl Pts',(-0.295901553980528,1.97231489949139,
6.48313403404696));
#58685=CARTESIAN_POINT('Ctrl Pts',(-0.295738245746892,1.97193707965653,
6.48315958707906));
#58686=CARTESIAN_POINT('Ctrl Pts',(-0.295653009551372,1.97174042137837,
6.48317288118724));
#58687=CARTESIAN_POINT('Ctrl Pts',(-0.295416618790474,1.97119650469471,
6.48320963251142));
#58688=CARTESIAN_POINT('Ctrl Pts',(-0.295265047562389,1.97084942604879,
6.4832330641785));
#58689=CARTESIAN_POINT('Ctrl Pts',(-0.29466772673854,1.96948818576826,6.48332488864361));
#58690=CARTESIAN_POINT('Ctrl Pts',(-0.294217354368152,1.96847604283693,
6.48339300196234));
#58691=CARTESIAN_POINT('Ctrl Pts',(-0.285824346810446,1.94987290028494,
6.48464228601582));
#58692=CARTESIAN_POINT('Ctrl Pts',(-0.276321100630202,1.93302516984495,
6.48573132495378));
#58693=CARTESIAN_POINT('Ctrl Pts',(-0.2559928205353,1.90352692961752,6.48773743356918));
#58694=CARTESIAN_POINT('Ctrl Pts',(-0.245588722195322,1.89066737900363,
6.48865389446295));
#58695=CARTESIAN_POINT('Ctrl Pts',(-0.229112108465112,1.87322989638084,
6.49002771021757));
#58696=CARTESIAN_POINT('Ctrl Pts',(-0.223791753930463,1.86797784995627,
6.49046104336544));
#58697=CARTESIAN_POINT('Ctrl Pts',(-0.214934076170592,1.85982219755152,
6.49117118992359));
#58698=CARTESIAN_POINT('Ctrl Pts',(-0.21150901550838,1.85680056091025,6.49144323596642));
#58699=CARTESIAN_POINT('Ctrl Pts',(-0.206648876172002,1.85269321663257,
6.49182646327429));
#58700=CARTESIAN_POINT('Ctrl Pts',(-0.205267076805797,1.8515451145531,6.49193511236472));
#58701=CARTESIAN_POINT('Ctrl Pts',(-0.202861230213319,1.84957992699118,
6.49212379498689));
#58702=CARTESIAN_POINT('Ctrl Pts',(-0.201841657451197,1.84875741418385,
6.49220360823545));
#58703=CARTESIAN_POINT('Ctrl Pts',(-0.200384138285469,1.84759619811764,
6.49231750594974));
#58704=CARTESIAN_POINT('Ctrl Pts',(-0.199950280702594,1.84725236435923,
6.49235138491155));
#58705=CARTESIAN_POINT('Ctrl Pts',(-0.199226535766194,1.84668182358617,
6.49240786027095));
#58706=CARTESIAN_POINT('Ctrl Pts',(-0.198937140967943,1.8464544912708,6.49243043169911));
#58707=CARTESIAN_POINT('Ctrl Pts',(-0.198331873373952,1.84598070123244,
6.4924776178057));
#58708=CARTESIAN_POINT('Ctrl Pts',(-0.198015929278044,1.84573433599436,
6.49250223610215));
#58709=CARTESIAN_POINT('Ctrl Pts',(-0.19731868441456,1.84519272976638,6.49255653839377));
#58710=CARTESIAN_POINT('Ctrl Pts',(-0.196937179235094,1.84489775458869,
6.49258623284264));
#58711=CARTESIAN_POINT('Ctrl Pts',(-0.195602738664758,1.84387075880675,
6.49269003865474));
#58712=CARTESIAN_POINT('Ctrl Pts',(-0.194646381290574,1.84314321937085,
6.49276432639079));
#58713=CARTESIAN_POINT('Ctrl Pts',(-0.180235987978609,1.83230735216395,
6.4938821646308));
#58714=CARTESIAN_POINT('Ctrl Pts',(-0.166016803468828,1.82326434614998,
6.49496739069357));
#58715=CARTESIAN_POINT('Ctrl Pts',(-0.144090960856552,1.81162001856537,
6.49661471952838));
#58716=CARTESIAN_POINT('Ctrl Pts',(-0.136886087578603,1.80813118064035,
6.49715183037116));
#58717=CARTESIAN_POINT('Ctrl Pts',(-0.115848529602402,1.79889451791394,
6.49870228580871));
#58718=CARTESIAN_POINT('Ctrl Pts',(-0.101734891721652,1.79383758986947,
6.49972179280312));
#58719=CARTESIAN_POINT('Ctrl Pts',(-0.0800274595650272,1.78772738605329,
6.50122249589078));
#58720=CARTESIAN_POINT('Ctrl Pts',(-0.0726636081286285,1.78593217676732,
6.50172015116792));
#58721=CARTESIAN_POINT('Ctrl Pts',(-0.0620125190637705,1.78373033076195,
6.50241752456368));
#58722=CARTESIAN_POINT('Ctrl Pts',(-0.05877202844937,1.7831121539632,6.50262674672557));
#58723=CARTESIAN_POINT('Ctrl Pts',(-0.0550119404651455,1.78245452193384,
6.50286567132796));
#58724=CARTESIAN_POINT('Ctrl Pts',(-0.0545011960429062,1.78236646292809,
6.50289804337469));
#58725=CARTESIAN_POINT('Ctrl Pts',(-0.0537253352431158,1.78223462086409,
6.50294709254412));
#58726=CARTESIAN_POINT('Ctrl Pts',(-0.053460375936724,1.78218993717891,
6.5029638206315));
#58727=CARTESIAN_POINT('Ctrl Pts',(-0.0530009923093842,1.78211305582627,
6.50299278444998));
#58728=CARTESIAN_POINT('Ctrl Pts',(-0.0528065947318616,1.78208070518534,
6.50300502891636));
#58729=CARTESIAN_POINT('Ctrl Pts',(-0.0523998692832992,1.78201340338304,
6.50303062171758));
#58730=CARTESIAN_POINT('Ctrl Pts',(-0.0521875367374543,1.78197848667289,
6.50304396803739));
#58731=CARTESIAN_POINT('Ctrl Pts',(-0.0515972307284654,1.78188202179442,
6.50308103226511));
#58732=CARTESIAN_POINT('Ctrl Pts',(-0.0512191807084466,1.78182093436617,
6.50310472388172));
#58733=CARTESIAN_POINT('Ctrl Pts',(-0.04971551085765,1.78158071241237,6.50319877832356));
#58734=CARTESIAN_POINT('Ctrl Pts',(-0.0485890356039956,1.78140687320974,
6.50326884406176));
#58735=CARTESIAN_POINT('Ctrl Pts',(-0.0285911448495527,1.7784293045431,
6.50450606799246));
#58736=CARTESIAN_POINT('Ctrl Pts',(-0.00950519058157107,1.77730037052134,
6.50558339937685));
#58737=CARTESIAN_POINT('Ctrl Pts',(0.0261406239477286,1.77835946023586,
6.50758081032869));
#58738=CARTESIAN_POINT('Ctrl Pts',(0.0426472997564674,1.7801294745042,6.50850026678078));
#58739=CARTESIAN_POINT('Ctrl Pts',(0.0652822655045629,1.78434042508229,
6.50981815591815));
#58740=CARTESIAN_POINT('Ctrl Pts',(0.0715835665926123,1.78570948538023,
6.51019113565383));
#58741=CARTESIAN_POINT('Ctrl Pts',(0.0830062286094235,1.78855258482769,
6.51088193881122));
#58742=CARTESIAN_POINT('Ctrl Pts',(0.0881402302758181,1.78996641884462,
6.51119794356894));
#58743=CARTESIAN_POINT('Ctrl Pts',(0.0951629383555637,1.79208890841296,
6.51163896932012));
#58744=CARTESIAN_POINT('Ctrl Pts',(0.0970836986178495,1.79268911450801,
6.51176050624991));
#58745=CARTESIAN_POINT('Ctrl Pts',(0.0999299768158749,1.79360787698679,
6.51194201829872));
#58746=CARTESIAN_POINT('Ctrl Pts',(0.100859892107893,1.79391273230977,6.51200154596951));
#58747=CARTESIAN_POINT('Ctrl Pts',(0.10234016164324,1.79440548905383,6.51209666952114));
#58748=CARTESIAN_POINT('Ctrl Pts',(0.102891425711614,1.79459065450831,6.51213217535216));
#58749=CARTESIAN_POINT('Ctrl Pts',(0.103938687112864,1.79494557899081,6.51219978300012));
#58750=CARTESIAN_POINT('Ctrl Pts',(0.104434777803806,1.79511505836474,6.51223187550116));
#58751=CARTESIAN_POINT('Ctrl Pts',(0.105299999353866,1.79541300336072,6.51228796450383));
#58752=CARTESIAN_POINT('Ctrl Pts',(0.105669315148705,1.79554093178313,6.51231194316407));
#58753=CARTESIAN_POINT('Ctrl Pts',(0.106387095461984,1.79579102922956,6.51235861968455));
#58754=CARTESIAN_POINT('Ctrl Pts',(0.106735584688907,1.79591312600278,6.51238131511682));
#58755=CARTESIAN_POINT('Ctrl Pts',(0.107557869691453,1.79620280965626,6.51243494618325));
#58756=CARTESIAN_POINT('Ctrl Pts',(0.108031483787504,1.79637090603926,6.51246589871753));
#58757=CARTESIAN_POINT('Ctrl Pts',(0.109677097008734,1.7969593092355,6.51257366472926));
#58758=CARTESIAN_POINT('Ctrl Pts',(0.110847040786707,1.79738529555498,6.51265066713543));
#58759=CARTESIAN_POINT('Ctrl Pts',(0.125970494214967,1.80299134069976,6.51365113396894));
#58760=CARTESIAN_POINT('Ctrl Pts',(0.139549262891696,1.80912442907278,6.51460691548829));
#58761=CARTESIAN_POINT('Ctrl Pts',(0.161232773616753,1.82078673270039,6.51623139714973));
#58762=CARTESIAN_POINT('Ctrl Pts',(0.169597284621658,1.82578694934071,6.51688407825055));
#58763=CARTESIAN_POINT('Ctrl Pts',(0.191846725374177,1.84049527943609,6.51868369222193));
#58764=CARTESIAN_POINT('Ctrl Pts',(0.205213832211823,1.85093137361952,6.51983812182962));
#58765=CARTESIAN_POINT('Ctrl Pts',(0.223591584026318,1.86776770935582,6.52148528083735));
#58766=CARTESIAN_POINT('Ctrl Pts',(0.229281610023606,1.87338358233888,6.52200466386139));
#58767=CARTESIAN_POINT('Ctrl Pts',(0.235629694593427,1.8801331230414,6.52258934544858));
#58768=CARTESIAN_POINT('Ctrl Pts',(0.23649646410194,1.88106571955683,6.52266929577331));
#58769=CARTESIAN_POINT('Ctrl Pts',(0.237617638417225,1.88228646985619,6.52277283730607));
#58770=CARTESIAN_POINT('Ctrl Pts',(0.237877070936153,1.88256995970852,6.52279680495517));
#58771=CARTESIAN_POINT('Ctrl Pts',(0.23829726499828,1.88303077083446,6.52283563785442));
#58772=CARTESIAN_POINT('Ctrl Pts',(0.238458336180257,1.88320780729604,6.52285052669038));
#58773=CARTESIAN_POINT('Ctrl Pts',(0.238767640019753,1.88354853091216,6.52287912346315));
#58774=CARTESIAN_POINT('Ctrl Pts',(0.238915901214033,1.88371219050025,6.52289283354896));
#58775=CARTESIAN_POINT('Ctrl Pts',(0.23925752753382,1.88409007798021,6.52292443077763));
#58776=CARTESIAN_POINT('Ctrl Pts',(0.239450773809236,1.88430441397214,6.52294230884464));
#58777=CARTESIAN_POINT('Ctrl Pts',(0.240067585764723,1.88499039151306,6.52299938867727));
#58778=CARTESIAN_POINT('Ctrl Pts',(0.240490051211414,1.88546302705351,6.52303850760051));
#58779=CARTESIAN_POINT('Ctrl Pts',(0.244258333778891,1.88970393187527,6.52338768601719));
#58780=CARTESIAN_POINT('Ctrl Pts',(0.247516957569114,1.89354920079565,6.52369139449247));
#58781=CARTESIAN_POINT('Ctrl Pts',(0.260255767829884,1.90931680336318,6.52489331831766));
#58782=CARTESIAN_POINT('Ctrl Pts',(0.268976405466718,1.92182892003565,6.52575090668255));
#58783=CARTESIAN_POINT('Ctrl Pts',(0.28519040748839,1.94901268437145,6.52752279820172));
#58784=CARTESIAN_POINT('Ctrl Pts',(0.292510850531186,1.96373513391884,6.52843431397889));
#58785=CARTESIAN_POINT('Ctrl Pts',(0.302262763897536,1.98779700759307,6.52992210082112));
#58786=CARTESIAN_POINT('Ctrl Pts',(0.30545303041204,1.99679771049169,6.53047790248133));
#58787=CARTESIAN_POINT('Ctrl Pts',(0.309152562993284,2.00891947100515,6.53123307982606));
#58788=CARTESIAN_POINT('Ctrl Pts',(0.31002243276866,2.01192582602131,6.53142088461074));
#58789=CARTESIAN_POINT('Ctrl Pts',(0.311206592101632,2.01625350740349,6.53169216576253));
#58790=CARTESIAN_POINT('Ctrl Pts',(0.311556545343067,2.01756495310482,6.5317744955639));
#58791=CARTESIAN_POINT('Ctrl Pts',(0.312082893156295,2.01958867119098,6.53190174273652));
#58792=CARTESIAN_POINT('Ctrl Pts',(0.312265160002553,2.02029941131785,6.53194647090718));
#58793=CARTESIAN_POINT('Ctrl Pts',(0.312599963579255,2.02162373987984,6.53202988725153));
#58794=CARTESIAN_POINT('Ctrl Pts',(0.312753125180324,2.02223716786835,6.53206855510158));
#58795=CARTESIAN_POINT('Ctrl Pts',(0.313003454131965,2.02325246411535,6.53213260511041));
#58796=CARTESIAN_POINT('Ctrl Pts',(0.313101655540057,2.02365407765664,6.53215795386647));
#58797=CARTESIAN_POINT('Ctrl Pts',(0.313292756809693,2.02444219318942,6.53220772341406));
#58798=CARTESIAN_POINT('Ctrl Pts',(0.313385714968459,2.02482868039672,6.53223214227674));
#58799=CARTESIAN_POINT('Ctrl Pts',(0.31359930839239,2.02572400876739,6.53228873913749));
#58800=CARTESIAN_POINT('Ctrl Pts',(0.313719420419001,2.02623297251077,6.53232093391327));
#58801=CARTESIAN_POINT('Ctrl Pts',(0.314039521674849,2.0276042949426,6.53240773634923));
#58802=CARTESIAN_POINT('Ctrl Pts',(0.314237196322276,2.02846718440467,6.5324624182604));
#58803=CARTESIAN_POINT('Ctrl Pts',(0.315643664618939,2.03472504656623,6.5328594491829));
#58804=CARTESIAN_POINT('Ctrl Pts',(0.316716943648237,2.0401492351897,6.5332061171858));
#58805=CARTESIAN_POINT('Ctrl Pts',(0.323018217033364,2.07694206435334,6.53557655859086));
#58806=CARTESIAN_POINT('Ctrl Pts',(0.323716403297786,2.10890391905077,6.53775339437791));
#58807=CARTESIAN_POINT('Ctrl Pts',(0.318482233527883,2.15028676631206,6.54055209572546));
#58808=CARTESIAN_POINT('Ctrl Pts',(0.316782394627325,2.16007196335346,6.54121011226145));
#58809=CARTESIAN_POINT('Ctrl Pts',(0.313815489197909,2.17345264175993,6.54209177099681));
#58810=CARTESIAN_POINT('Ctrl Pts',(0.31293271615149,2.17712697391358,6.5423319330912));
#58811=CARTESIAN_POINT('Ctrl Pts',(0.311851162671223,2.1813038441737,6.54260205793298));
#58812=CARTESIAN_POINT('Ctrl Pts',(0.311715551264867,2.1818222332028,6.54263553192139));
#58813=CARTESIAN_POINT('Ctrl Pts',(0.311509061546128,2.18260359783216,6.54268590746918));
#58814=CARTESIAN_POINT('Ctrl Pts',(0.311439142580097,2.18286682249523,6.54270286424847));
#58815=CARTESIAN_POINT('Ctrl Pts',(0.311313093962704,2.18333894612362,6.54273325329548));
#58816=CARTESIAN_POINT('Ctrl Pts',(0.31125708780089,2.183547876743,6.54274669269961));
#58817=CARTESIAN_POINT('Ctrl Pts',(0.311135745278638,2.18399872873202,6.5427756746269));
#58818=CARTESIAN_POINT('Ctrl Pts',(0.311070337288588,2.18424062962062,6.54279121287173));
#58819=CARTESIAN_POINT('Ctrl Pts',(0.310893615555975,2.18489119404949,6.5428329701236));
#58820=CARTESIAN_POINT('Ctrl Pts',(0.31078177773036,2.18529971662458,6.54285915863868));
#58821=CARTESIAN_POINT('Ctrl Pts',(0.310265278141255,2.18717189240875,6.54297902892264));
#58822=CARTESIAN_POINT('Ctrl Pts',(0.3098510712756,2.18863292553078,6.5430721643837));
#58823=CARTESIAN_POINT('Ctrl Pts',(0.300471281894778,2.2208487460776,6.54511782978115));
#58824=CARTESIAN_POINT('Ctrl Pts',(0.286978505556387,2.25010516858085,6.54682814663942));
#58825=CARTESIAN_POINT('Ctrl Pts',(0.260088425521228,2.29105556364028,6.54960532502415));
#58826=CARTESIAN_POINT('Ctrl Pts',(0.249688055047145,2.3044601903934,6.55058818622405));
#58827=CARTESIAN_POINT('Ctrl Pts',(0.237612149603963,2.31772146431123,6.55167646404756));
#58828=CARTESIAN_POINT('Ctrl Pts',(0.236937459741789,2.31845550988153,6.55173710189994));
#58829=CARTESIAN_POINT('Ctrl Pts',(0.235858702922028,2.31961829375068,6.55183380007201));
#58830=CARTESIAN_POINT('Ctrl Pts',(0.235456844062191,2.32004907923247,6.55186976635934));
#58831=CARTESIAN_POINT('Ctrl Pts',(0.234691415113194,2.3208651079101,6.55193816790806));
#58832=CARTESIAN_POINT('Ctrl Pts',(0.234328071608558,2.32125056174142,6.55197059339633));
#58833=CARTESIAN_POINT('Ctrl Pts',(0.23369431536455,2.32191957128155,6.5520270751825));
#58834=CARTESIAN_POINT('Ctrl Pts',(0.23342433199294,2.32220353368691,6.55205111291031));
#58835=CARTESIAN_POINT('Ctrl Pts',(0.232899831868157,2.3227531802419,6.55209776562651));
#58836=CARTESIAN_POINT('Ctrl Pts',(0.23264537654844,2.32301892242809,6.55212037793161));
#58837=CARTESIAN_POINT('Ctrl Pts',(0.23204591774514,2.32364282906568,6.55217360084294));
#58838=CARTESIAN_POINT('Ctrl Pts',(0.231700539930969,2.32400063108384,6.55220422772685));
#58839=CARTESIAN_POINT('Ctrl Pts',(0.23050853290654,2.32522981145031,6.55230980327229));
#58840=CARTESIAN_POINT('Ctrl Pts',(0.229657813119754,2.32609719263374,6.55238493083617));
#58841=CARTESIAN_POINT('Ctrl Pts',(0.219514719096297,2.33632262945309,6.55327813385003));
#58842=CARTESIAN_POINT('Ctrl Pts',(0.209662526328,2.34510536846211,6.5541214233853));
#58843=CARTESIAN_POINT('Ctrl Pts',(0.179920484911499,2.36851074168235,6.55660396240831));
#58844=CARTESIAN_POINT('Ctrl Pts',(0.15885390277515,2.38148642155011,6.55829536378963));
#58845=CARTESIAN_POINT('Ctrl Pts',(0.128516911978139,2.39567312370475,6.56053704943688));
#58846=CARTESIAN_POINT('Ctrl Pts',(0.120364697394606,2.39908453260391,6.56112114291632));
#58847=CARTESIAN_POINT('Ctrl Pts',(0.108405332242408,2.40352073661635,6.5619424633761));
#58848=CARTESIAN_POINT('Ctrl Pts',(0.104703856327779,2.40481742000188,6.56219187496208));
#58849=CARTESIAN_POINT('Ctrl Pts',(0.100466144879292,2.40621564542868,6.5624712701139));
#58850=CARTESIAN_POINT('Ctrl Pts',(0.0999524268810275,2.40638371389958,
6.56250503783142));
#58851=CARTESIAN_POINT('Ctrl Pts',(0.0991783045902107,2.40663482226382,
6.56255576631305));
#58852=CARTESIAN_POINT('Ctrl Pts',(0.0989182167833165,2.40671882354348,
6.56257278345768));
#58853=CARTESIAN_POINT('Ctrl Pts',(0.0984501231351375,2.40686934772098,
6.56260336205983));
#58854=CARTESIAN_POINT('Ctrl Pts',(0.0982421569839919,2.40693598991992,
6.56261693055362));
#58855=CARTESIAN_POINT('Ctrl Pts',(0.0977953665679315,2.40707866210356,
6.56264604413695));
#58856=CARTESIAN_POINT('Ctrl Pts',(0.0975565220298319,2.40715462466311,
6.56266158518031));
#58857=CARTESIAN_POINT('Ctrl Pts',(0.0969136241461207,2.40735826756444,
6.56270335723016));
#58858=CARTESIAN_POINT('Ctrl Pts',(0.0965094054311341,2.40748543031101,
6.56272955770777));
#58859=CARTESIAN_POINT('Ctrl Pts',(0.0946537190578215,2.40806518901736,
6.56284955274681));
#58860=CARTESIAN_POINT('Ctrl Pts',(0.0931992799997537,2.40850831696512,
6.56294279961969));
#58861=CARTESIAN_POINT('Ctrl Pts',(0.0610437557669386,2.41805707192222,
6.56498780904822));
#58862=CARTESIAN_POINT('Ctrl Pts',(0.0291528022426285,2.42254855126251,
6.56669756083612));
#58863=CARTESIAN_POINT('Ctrl Pts',(-0.0185596787889771,2.42212193200753,
6.56940236004781));
#58864=CARTESIAN_POINT('Ctrl Pts',(-0.0342047289446672,2.42083787323481,
6.57031018052081));
#58865=CARTESIAN_POINT('Ctrl Pts',(-0.0521360208321992,2.41803950179141,
6.57140475643834));
#58866=CARTESIAN_POINT('Ctrl Pts',(-0.0545745251660122,2.41763014662507,
6.57155474737915));
#58867=CARTESIAN_POINT('Ctrl Pts',(-0.0577067638734682,2.41706719955389,
6.57174895348593));
#58868=CARTESIAN_POINT('Ctrl Pts',(-0.0584050799225414,2.416939310052,6.57179234973643));
#58869=CARTESIAN_POINT('Ctrl Pts',(-0.0595301196962569,2.41672942598826,
6.57186242608498));
#58870=CARTESIAN_POINT('Ctrl Pts',(-0.0599571127946968,2.41664887345497,
6.57188906018629));
#58871=CARTESIAN_POINT('Ctrl Pts',(-0.0607703984588084,2.41649374256094,
6.57193986184309));
#58872=CARTESIAN_POINT('Ctrl Pts',(-0.0611567202126165,2.41641931985852,
6.57196402439151));
#58873=CARTESIAN_POINT('Ctrl Pts',(-0.0620376499397637,2.41624794015645,
6.57201919360008));
#58874=CARTESIAN_POINT('Ctrl Pts',(-0.0625321677823352,2.4161505300503,
6.57205021467716));
#58875=CARTESIAN_POINT('Ctrl Pts',(-0.0640413036967127,2.41584958117044,
6.57214504069386));
#58876=CARTESIAN_POINT('Ctrl Pts',(-0.0650551642646875,2.41564231666113,
6.5722089645422));
#58877=CARTESIAN_POINT('Ctrl Pts',(-0.0724680185498928,2.41408966731579,
6.57267796594517));
#58878=CARTESIAN_POINT('Ctrl Pts',(-0.0788253440380896,2.41255477578564,
6.57308908740827));
#58879=CARTESIAN_POINT('Ctrl Pts',(-0.0874050759989636,2.41020491052734,
6.57365670544542));
#58880=CARTESIAN_POINT('Ctrl Pts',(-0.0896719671096978,2.40955721875744,
6.57380790384475));
#58881=CARTESIAN_POINT('Ctrl Pts',(-0.115608626024277,2.40183784704886,
6.57555196700301));
#58882=CARTESIAN_POINT('Ctrl Pts',(-0.138394098259906,2.39209272466296,
6.57722910029268));
#58883=CARTESIAN_POINT('Ctrl Pts',(-0.161202130629033,2.37906542832811,
6.57900264634036));
#58884=CARTESIAN_POINT('Ctrl Pts',(-0.162559634867899,2.3782768502201,6.57910855095055));
#58885=CARTESIAN_POINT('Ctrl Pts',(-0.169442264934589,2.37421116034017,
6.57964710563233));
#58886=CARTESIAN_POINT('Ctrl Pts',(-0.17487449945034,2.37077916729813,6.58007752232645));
#58887=CARTESIAN_POINT('Ctrl Pts',(-0.185428670054059,2.36366104693505,
6.580919950602));
#58888=CARTESIAN_POINT('Ctrl Pts',(-0.190552393365375,2.359982183553,6.58133198139306));
#58889=CARTESIAN_POINT('Ctrl Pts',(-0.19800028162625,2.35429598903102,6.58193180361376));
#58890=CARTESIAN_POINT('Ctrl Pts',(-0.200408850120782,2.35240217123401,
6.58212592018641));
#58891=CARTESIAN_POINT('Ctrl Pts',(-0.203185321176402,2.35015427120927,
6.58234949314189));
#58892=CARTESIAN_POINT('Ctrl Pts',(-0.2035797368622,2.34983339427173,6.5823812484604));
#58893=CARTESIAN_POINT('Ctrl Pts',(-0.204179825980537,2.34934282700711,
6.58242955370517));
#58894=CARTESIAN_POINT('Ctrl Pts',(-0.204386048644261,2.34917381451139,
6.58244615228252));
#58895=CARTESIAN_POINT('Ctrl Pts',(-0.204744160587552,2.34887957546118,
6.58247497292661));
#58896=CARTESIAN_POINT('Ctrl Pts',(-0.204896144490074,2.34875446599054,
6.58248720345338));
#58897=CARTESIAN_POINT('Ctrl Pts',(-0.205239296216202,2.34847146393095,
6.58251481531334));
#58898=CARTESIAN_POINT('Ctrl Pts',(-0.205430396120943,2.34831349026966,
6.58253019059712));
#58899=CARTESIAN_POINT('Ctrl Pts',(-0.205946783532397,2.34788561200102,
6.58257173357458));
#58900=CARTESIAN_POINT('Ctrl Pts',(-0.206271724094448,2.34761528654023,
6.58259787061055));
#58901=CARTESIAN_POINT('Ctrl Pts',(-0.2077202289483,2.3464054123774,6.58271436919698));
#58902=CARTESIAN_POINT('Ctrl Pts',(-0.208837935277838,2.34545883105568,
6.58280422536109));
#58903=CARTESIAN_POINT('Ctrl Pts',(-0.231494546378991,2.32600424418803,
6.58462582276576));
#58904=CARTESIAN_POINT('Ctrl Pts',(-0.250504147151153,2.30473377200297,
6.586164726351));
#58905=CARTESIAN_POINT('Ctrl Pts',(-0.278262413253177,2.26392091465782,
6.58893944405263));
#58906=CARTESIAN_POINT('Ctrl Pts',(-0.288324958338725,2.24549417838805,
6.59014109462002));
#58907=CARTESIAN_POINT('Ctrl Pts',(-0.297017964400265,2.22507225552453,
6.59148983028058));
#58908=CARTESIAN_POINT('Ctrl Pts',(-0.297501169991604,2.22391849766322,
6.59156606624788));
#58909=CARTESIAN_POINT('Ctrl Pts',(-0.298185125033141,2.22225834743568,
6.59167582698931));
#58910=CARTESIAN_POINT('Ctrl Pts',(-0.298391330660344,2.22175420358135,
6.5917091668934));
#58911=CARTESIAN_POINT('Ctrl Pts',(-0.298746615801498,2.22087925748714,
6.59176704418544));
#58912=CARTESIAN_POINT('Ctrl Pts',(-0.298896285929663,2.22050869511624,
6.59179156155729));
#58913=CARTESIAN_POINT('Ctrl Pts',(-0.299182501635492,2.21979625147667,
6.59183870836425));
#58914=CARTESIAN_POINT('Ctrl Pts',(-0.299319151535049,2.2194544125402,6.59186133423539));
#58915=CARTESIAN_POINT('Ctrl Pts',(-0.299639336338036,2.21864944969625,
6.59191462408014));
#58916=CARTESIAN_POINT('Ctrl Pts',(-0.299822383334796,2.21818613387922,
6.59194530443323));
#58917=CARTESIAN_POINT('Ctrl Pts',(-0.300358861613304,2.21681896991571,
6.59203586171084));
#58918=CARTESIAN_POINT('Ctrl Pts',(-0.300709282892866,2.21591395356405,
6.59209583963814));
#58919=CARTESIAN_POINT('Ctrl Pts',(-0.303746584613286,2.20796318773336,
6.59262306135422));
#58920=CARTESIAN_POINT('Ctrl Pts',(-0.306189299510039,2.20082725323033,
6.59309841502821));
#58921=CARTESIAN_POINT('Ctrl Pts',(-0.309906926140884,2.18858062828711,
6.59391882785019));
#58922=CARTESIAN_POINT('Ctrl Pts',(-0.311311005847503,2.18351217512201,
6.5942596549374));
#58923=CARTESIAN_POINT('Ctrl Pts',(-0.313297705766731,2.17559215671941,
6.59479406257193));
#58924=CARTESIAN_POINT('Ctrl Pts',(-0.313966813338072,2.17276308130807,
6.59498530914165));
#58925=CARTESIAN_POINT('Ctrl Pts',(-0.319715117439977,2.14690120075679,
6.59673634378382));
#58926=CARTESIAN_POINT('Ctrl Pts',(-0.322289258550463,2.12338728256337,
6.59835561527569));
#58927=CARTESIAN_POINT('Ctrl Pts',(-0.322272956104475,2.09653565802172,
6.60014663846072));
#58928=CARTESIAN_POINT('Ctrl Pts',(-0.322221242681646,2.09326711248847,
6.60036354200454));
#58929=CARTESIAN_POINT('Ctrl Pts',(-0.322093711926189,2.0891591616064,6.60063434088577));
#58930=CARTESIAN_POINT('Ctrl Pts',(-0.32206432218159,2.08831858567874,6.60068965684094));
#58931=CARTESIAN_POINT('Ctrl Pts',(-0.322004108188569,2.08677003044707,
6.60079137646901));
#58932=CARTESIAN_POINT('Ctrl Pts',(-0.321974238931584,2.08606202081072,
6.60083781150307));
#58933=CARTESIAN_POINT('Ctrl Pts',(-0.321892349648388,2.08426195246846,
6.60095567785508));
#58934=CARTESIAN_POINT('Ctrl Pts',(-0.321837107006106,2.08317004116589,
6.60102699546791));
#58935=CARTESIAN_POINT('Ctrl Pts',(-0.321725315800544,2.08116286548787,
6.60115773884758));
#58936=CARTESIAN_POINT('Ctrl Pts',(-0.32167041545863,2.0802475237296,6.60121722680186));
#58937=CARTESIAN_POINT('Ctrl Pts',(-0.321602822166345,2.07919569345824,
6.60128542019758));
#58938=CARTESIAN_POINT('Ctrl Pts',(-0.321593948640068,2.07905897341921,
6.60129428097452));
#58939=CARTESIAN_POINT('Ctrl Pts',(-0.321556524191658,2.07848798525191,
6.60133127301996));
#58940=CARTESIAN_POINT('Ctrl Pts',(-0.321527180665637,2.07805376738307,
6.60135937166211));
#58941=CARTESIAN_POINT('Ctrl Pts',(-0.321215225898136,2.07357250055268,
6.60164901324086));
#58942=CARTESIAN_POINT('Ctrl Pts',(-0.320857083298464,2.06953083586833,
6.60190733662367));
#58943=CARTESIAN_POINT('Ctrl Pts',(-0.320365218657665,2.06496301213095,
6.60219518875027));
#58944=CARTESIAN_POINT('Ctrl Pts',(-0.320306407405511,2.0644293768773,6.60222875345477));
#58945=CARTESIAN_POINT('Ctrl Pts',(-0.320215306413238,2.06362130407119,
6.60227948091063));
#58946=CARTESIAN_POINT('Ctrl Pts',(-0.320183997097856,2.06334676027073,
6.60229669833238));
#58947=CARTESIAN_POINT('Ctrl Pts',(-0.320128891534884,2.06286901176374,
6.60232662878567));
#58948=CARTESIAN_POINT('Ctrl Pts',(-0.320105254876724,2.06266578936656,
6.60233935084768));
#58949=CARTESIAN_POINT('Ctrl Pts',(-0.320055285274006,2.06223969867003,
6.60236600448215));
#58950=CARTESIAN_POINT('Ctrl Pts',(-0.320028913063907,2.06201683541559,
6.60237993374532));
#58951=CARTESIAN_POINT('Ctrl Pts',(-0.319965043463828,2.06148188228979,
6.60241334133741));
#58952=CARTESIAN_POINT('Ctrl Pts',(-0.319927322089582,2.06116981826796,
6.60243280694771));
#58953=CARTESIAN_POINT('Ctrl Pts',(-0.319796734203696,2.06010259016257,
6.60249930143886));
#58954=CARTESIAN_POINT('Ctrl Pts',(-0.319701649116596,2.05934769257635,
6.60254620577905));
#58955=CARTESIAN_POINT('Ctrl Pts',(-0.317380790370106,2.04143386617511,
6.60365631158666));
#58956=CARTESIAN_POINT('Ctrl Pts',(-0.313779010516772,2.02447860488013,
6.60464357552217));
#58957=CARTESIAN_POINT('Ctrl Pts',(-0.301976775891885,1.98490629694215,
6.60696501134263));
#58958=CARTESIAN_POINT('Ctrl Pts',(-0.292577119968493,1.96275893268245,
6.60828353327848));
#58959=CARTESIAN_POINT('Ctrl Pts',(-0.27632343650692,1.93389751449061,6.61021633595446));
#58960=CARTESIAN_POINT('Ctrl Pts',(-0.27150322067352,1.9261303524574,6.61075951804212));
#58961=CARTESIAN_POINT('Ctrl Pts',(-0.265720380824297,1.91764006659532,
6.6113842601));
#58962=CARTESIAN_POINT('Ctrl Pts',(-0.265075935290741,1.91670457022946,
6.61145353242008));
#58963=CARTESIAN_POINT('Ctrl Pts',(-0.264130465538938,1.91534751261913,
6.61155466492517));
#58964=CARTESIAN_POINT('Ctrl Pts',(-0.263833344695421,1.91492323175601,
6.61158637607559));
#58965=CARTESIAN_POINT('Ctrl Pts',(-0.263306876457105,1.91417529284326,
6.61164244183178));
#58966=CARTESIAN_POINT('Ctrl Pts',(-0.263077951375463,1.91385133769661,
6.61166678021621));
#58967=CARTESIAN_POINT('Ctrl Pts',(-0.262603128364511,1.91318203424247,
6.61171717773355));
#58968=CARTESIAN_POINT('Ctrl Pts',(-0.262357146043624,1.91283674699953,
6.61174324008208));
#58969=CARTESIAN_POINT('Ctrl Pts',(-0.261725029852129,1.91195313544969,
6.61181009689063));
#58970=CARTESIAN_POINT('Ctrl Pts',(-0.261337917462433,1.91141551653376,
6.61185092905998));
#58971=CARTESIAN_POINT('Ctrl Pts',(-0.259745921143715,1.90921887890045,
6.61201840020462));
#58972=CARTESIAN_POINT('Ctrl Pts',(-0.258526896249008,1.9075702119671,6.61214558676522));
#58973=CARTESIAN_POINT('Ctrl Pts',(-0.250350834270083,1.89673044630774,
6.61299191475865));
#58974=CARTESIAN_POINT('Ctrl Pts',(-0.242921479923631,1.88790767896034,
6.61372974241548));
#58975=CARTESIAN_POINT('Ctrl Pts',(-0.21250712649406,1.85548790827707,6.61663963451552));
#58976=CARTESIAN_POINT('Ctrl Pts',(-0.18643512863399,1.83507184396763,6.61893723242836));
#58977=CARTESIAN_POINT('Ctrl Pts',(-0.153399672977918,1.81653160745439,
6.6213936917021));
#58978=CARTESIAN_POINT('Ctrl Pts',(-0.149017447459071,1.81420357537402,
6.62171083030969));
#58979=CARTESIAN_POINT('Ctrl Pts',(-0.144074989921747,1.811722536583,6.62205747633366));
#58980=CARTESIAN_POINT('Ctrl Pts',(-0.143566377095639,1.81146890286419,
6.62209302012971));
#58981=CARTESIAN_POINT('Ctrl Pts',(-0.142802288471738,1.81109038975963,
6.62214622205551));
#58982=CARTESIAN_POINT('Ctrl Pts',(-0.142547317389401,1.81096450254575,
6.62216394259694));
#58983=CARTESIAN_POINT('Ctrl Pts',(-0.142106757929065,1.81074770928801,
6.62219450492392));
#58984=CARTESIAN_POINT('Ctrl Pts',(-0.141921248686971,1.81065664427376,
6.62220735668772));
#58985=CARTESIAN_POINT('Ctrl Pts',(-0.141535610414867,1.81046779760793,
6.6222340368884));
#58986=CARTESIAN_POINT('Ctrl Pts',(-0.141335467871401,1.81037004512766,
6.62224786341812));
#58987=CARTESIAN_POINT('Ctrl Pts',(-0.140860870605367,1.8101388541247,6.62228060261706));
#58988=CARTESIAN_POINT('Ctrl Pts',(-0.140586326462323,1.81000559734797,
6.62229950385664));
#58989=CARTESIAN_POINT('Ctrl Pts',(-0.139674574356821,1.80956465503476,
6.62236215067675));
#58990=CARTESIAN_POINT('Ctrl Pts',(-0.139036536613415,1.80925867539049,
6.62240579042705));
#58991=CARTESIAN_POINT('Ctrl Pts',(-0.12167629344045,1.80100355200804,6.623587888039));
#58992=CARTESIAN_POINT('Ctrl Pts',(-0.104298022489748,1.79450671783784,
6.62463905094674));
#58993=CARTESIAN_POINT('Ctrl Pts',(-0.0623097354637593,1.78281409790137,
6.62708428286339));
#58994=CARTESIAN_POINT('Ctrl Pts',(-0.0374643903824467,1.77893034319031,
6.62846567043877));
#58995=CARTESIAN_POINT('Ctrl Pts',(-0.0119401907742147,1.77794590747969,
6.62997025003553));
#58996=CARTESIAN_POINT('Ctrl Pts',(-0.0114598428059394,1.77792845722683,
6.62999859253812));
#58997=CARTESIAN_POINT('Ctrl Pts',(-0.0043846379138922,1.77768727486621,
6.63041647095283));
#58998=CARTESIAN_POINT('Ctrl Pts',(0.00221513620775677,1.77766507862802,
6.63081159301556));
#58999=CARTESIAN_POINT('Ctrl Pts',(0.00984781068270887,1.77787382464165,
6.63127629289522));
#59000=CARTESIAN_POINT('Ctrl Pts',(0.0108848641264693,1.77790719983255,
6.63133959609801));
#59001=CARTESIAN_POINT('Ctrl Pts',(0.0124259545084263,1.77796424752613,
6.63143391660346));
#59002=CARTESIAN_POINT('Ctrl Pts',(0.0129301333053778,1.77798409687565,
6.63146481404263));
#59003=CARTESIAN_POINT('Ctrl Pts',(0.0138274128395668,1.77802153314783,
6.63151987337695));
#59004=CARTESIAN_POINT('Ctrl Pts',(0.0142205327627943,1.7780386561898,6.63154402068141));
#59005=CARTESIAN_POINT('Ctrl Pts',(0.015047406020875,1.77807618951689,6.63159486308492));
#59006=CARTESIAN_POINT('Ctrl Pts',(0.0154811511396879,1.77809675655505,
6.63162156305284));
#59007=CARTESIAN_POINT('Ctrl Pts',(0.0166226138978508,1.77815319407498,
6.63169190761134));
#59008=CARTESIAN_POINT('Ctrl Pts',(0.0173302542044033,1.77819052212011,
6.63173559783877));
#59009=CARTESIAN_POINT('Ctrl Pts',(0.0204938978501519,1.77836786954533,
6.63193128900987));
#59010=CARTESIAN_POINT('Ctrl Pts',(0.0229483208069975,1.77853367015751,
6.63208409663153));
#59011=CARTESIAN_POINT('Ctrl Pts',(0.0408958379445197,1.77995264285547,
6.63320895506484));
#59012=CARTESIAN_POINT('Ctrl Pts',(0.0562798272310379,1.78229693999802,
6.63421550780486));
#59013=CARTESIAN_POINT('Ctrl Pts',(0.0996759653945203,1.79216113708756,
6.63717156661772));
#59014=CARTESIAN_POINT('Ctrl Pts',(0.126922666148529,1.80235826977959,6.63918181129921));
#59015=CARTESIAN_POINT('Ctrl Pts',(0.153117495314163,1.81642143922152,6.64110327697467));
#59016=CARTESIAN_POINT('Ctrl Pts',(0.153794026069427,1.81678777379333,6.64115288408811));
#59017=CARTESIAN_POINT('Ctrl Pts',(0.157714359585299,1.81892878472342,6.64144021118266));
#59018=CARTESIAN_POINT('Ctrl Pts',(0.160928909144305,1.82075685079156,6.64167527713365));
#59019=CARTESIAN_POINT('Ctrl Pts',(0.16461079709705,1.82293539066012,6.64194326977046));
#59020=CARTESIAN_POINT('Ctrl Pts',(0.165109350714285,1.82323220095402,6.64197953100254));
#59021=CARTESIAN_POINT('Ctrl Pts',(0.165848453949092,1.82367492857575,6.64203324497753));
#59022=CARTESIAN_POINT('Ctrl Pts',(0.166089614960133,1.82381981501425,6.64205076440057));
#59023=CARTESIAN_POINT('Ctrl Pts',(0.166518313202314,1.82407813600565,6.642081895075));
#59024=CARTESIAN_POINT('Ctrl Pts',(0.166705924357836,1.82419144602289,6.64209551446522));
#59025=CARTESIAN_POINT('Ctrl Pts',(0.167099207688071,1.82442952211529,6.64212405517522));
#59026=CARTESIAN_POINT('Ctrl Pts',(0.167304855174735,1.82455432672221,6.64213897385418));
#59027=CARTESIAN_POINT('Ctrl Pts',(0.167849442914818,1.82488566436172,6.64217846758175));
#59028=CARTESIAN_POINT('Ctrl Pts',(0.168188143043823,1.82509259430858,6.64220301653856));
#59029=CARTESIAN_POINT('Ctrl Pts',(0.16893231785014,1.82554914041771,6.64225692604055));
#59030=CARTESIAN_POINT('Ctrl Pts',(0.169337624246516,1.82579903107213,6.64228626875434));
#59031=CARTESIAN_POINT('Ctrl Pts',(0.170538942534619,1.82654338036977,6.6423731895107));
#59032=CARTESIAN_POINT('Ctrl Pts',(0.171333361490152,1.82704041868715,6.64243060350788));
#59033=CARTESIAN_POINT('Ctrl Pts',(0.180213610300974,1.83265050250469,6.64307178761961));
#59034=CARTESIAN_POINT('Ctrl Pts',(0.188070955387116,1.83811824545422,6.64363350236649));
#59035=CARTESIAN_POINT('Ctrl Pts',(0.214489214360279,1.8583054220564,6.64554510701098));
#59036=CARTESIAN_POINT('Ctrl Pts',(0.231663114120729,1.8747130369459,6.64683466922115));
#59037=CARTESIAN_POINT('Ctrl Pts',(0.250542492395792,1.89721435963641,6.64850486760126));
#59038=CARTESIAN_POINT('Ctrl Pts',(0.254083828913118,1.90166956822271,6.64883110578064));
#59039=CARTESIAN_POINT('Ctrl Pts',(0.263867026515596,1.91466974084824,6.64977473248237));
#59040=CARTESIAN_POINT('Ctrl Pts',(0.269808047179066,1.92343076709371,6.65040102299436));
#59041=CARTESIAN_POINT('Ctrl Pts',(0.275919907296202,1.93347441651751,6.65111583007051));
#59042=CARTESIAN_POINT('Ctrl Pts',(0.276527163216149,1.93448476462156,6.65118769829599));
#59043=CARTESIAN_POINT('Ctrl Pts',(0.277373085198512,1.93590985354051,6.65128902259934));
#59044=CARTESIAN_POINT('Ctrl Pts',(0.277616396628106,1.93632183750737,6.65131830949718));
#59045=CARTESIAN_POINT('Ctrl Pts',(0.278061261086454,1.9370789441438,6.6513721212519));
#59046=CARTESIAN_POINT('Ctrl Pts',(0.278263091613831,1.93742390335133,6.65139663597726));
#59047=CARTESIAN_POINT('Ctrl Pts',(0.278671020541204,1.93812410121668,6.65144638940773));
#59048=CARTESIAN_POINT('Ctrl Pts',(0.278877082571272,1.93847936011012,6.65147162937053));
#59049=CARTESIAN_POINT('Ctrl Pts',(0.279383141225968,1.939355680066,6.65153388114936));
#59050=CARTESIAN_POINT('Ctrl Pts',(0.279682358944881,1.93987718708582,6.65157092101362));
#59051=CARTESIAN_POINT('Ctrl Pts',(0.280771240981623,1.94178736509621,6.6517065682485));
#59052=CARTESIAN_POINT('Ctrl Pts',(0.281552026293484,1.94318104722937,6.65180549435269));
#59053=CARTESIAN_POINT('Ctrl Pts',(0.2918637822684,1.9619125381584,6.65313465414971));
#59054=CARTESIAN_POINT('Ctrl Pts',(0.299787065605716,1.98008306812772,6.6544230829428));
#59055=CARTESIAN_POINT('Ctrl Pts',(0.313669554506166,2.02208473169073,6.65738506005834));
#59056=CARTESIAN_POINT('Ctrl Pts',(0.318676531929856,2.04610509787584,6.65907000627506));
#59057=CARTESIAN_POINT('Ctrl Pts',(0.321440352670845,2.07613147534416,6.6610336213089));
#59058=CARTESIAN_POINT('Ctrl Pts',(0.321811972000446,2.08181562717994,6.6613987755048));
#59059=CARTESIAN_POINT('Ctrl Pts',(0.322058145387035,2.08816128093234,6.66179694577708));
#59060=CARTESIAN_POINT('Ctrl Pts',(0.322081531968261,2.08881558843204,6.66183788921779));
#59061=CARTESIAN_POINT('Ctrl Pts',(0.322112479369901,2.08976223797089,6.66189695908852));
#59062=CARTESIAN_POINT('Ctrl Pts',(0.322121636314034,2.09005452076652,6.66191517418997));
#59063=CARTESIAN_POINT('Ctrl Pts',(0.322137028731784,2.09056817161309,6.66194714404775));
#59064=CARTESIAN_POINT('Ctrl Pts',(0.322143433868209,2.09078953401528,6.6619609083776));
#59065=CARTESIAN_POINT('Ctrl Pts',(0.322156240369632,2.09124849114401,6.66198941846315));
#59066=CARTESIAN_POINT('Ctrl Pts',(0.322162607055424,2.09148608594818,6.66200416221949));
#59067=CARTESIAN_POINT('Ctrl Pts',(0.322178193742005,2.09209282274428,6.66204177380023));
#59068=CARTESIAN_POINT('Ctrl Pts',(0.322187042198194,2.0924619752037,6.66206462069132));
#59069=CARTESIAN_POINT('Ctrl Pts',(0.322220808277631,2.09397954941442,6.66215839504681));
#59070=CARTESIAN_POINT('Ctrl Pts',(0.322240220687506,2.09512810333524,6.66222901724266));
#59071=CARTESIAN_POINT('Ctrl Pts',(0.322424833033489,2.11110663858217,6.66320694538956));
#59072=CARTESIAN_POINT('Ctrl Pts',(0.321572294807177,2.1259328754125,6.66406005642422));
#59073=CARTESIAN_POINT('Ctrl Pts',(0.317636179035466,2.15688975863748,6.66582242766279));
#59074=CARTESIAN_POINT('Ctrl Pts',(0.314336799815608,2.17294913113394,6.66672643266804));
#59075=CARTESIAN_POINT('Ctrl Pts',(0.304757378828396,2.20641466622414,6.66869333684917));
#59076=CARTESIAN_POINT('Ctrl Pts',(0.298172274796948,2.22367006161451,6.66975912745724));
#59077=CARTESIAN_POINT('Ctrl Pts',(0.289588998660437,2.24142504502064,6.67095699769655));
#59078=CARTESIAN_POINT('Ctrl Pts',(0.289022002074959,2.24258020110023,6.67103539770377));
#59079=CARTESIAN_POINT('Ctrl Pts',(0.288220779409782,2.24418813318997,6.67114519001482));
#59080=CARTESIAN_POINT('Ctrl Pts',(0.287992368980336,2.24464380678333,6.67117637885386));
#59081=CARTESIAN_POINT('Ctrl Pts',(0.287595793671669,2.24543030223995,6.67123034095924));
#59082=CARTESIAN_POINT('Ctrl Pts',(0.287428136144098,2.24576137999518,6.67125309639639));
#59083=CARTESIAN_POINT('Ctrl Pts',(0.287079671705101,2.24644656295273,6.6713002730786));
#59084=CARTESIAN_POINT('Ctrl Pts',(0.286898780676985,2.24680062449059,6.67132469725388));
#59085=CARTESIAN_POINT('Ctrl Pts',(0.286474013425777,2.24762824591477,6.67138189733892));
#59086=CARTESIAN_POINT('Ctrl Pts',(0.286229617952679,2.24810153666108,6.6714146915096));
#59087=CARTESIAN_POINT('Ctrl Pts',(0.285437999652594,2.24962528831241,6.6715205419012));
#59088=CARTESIAN_POINT('Ctrl Pts',(0.284886163545573,2.25067332978498,6.67159376103359));
#59089=CARTESIAN_POINT('Ctrl Pts',(0.279984447835828,2.25985941915393,6.67223922408107));
#59090=CARTESIAN_POINT('Ctrl Pts',(0.27529308552387,2.26780945705125,6.67282362664537));
#59091=CARTESIAN_POINT('Ctrl Pts',(0.26594508137182,2.2822014219522,6.67393219226125));
#59092=CARTESIAN_POINT('Ctrl Pts',(0.261378616761615,2.28869379424179,6.67445292578714));
#59093=CARTESIAN_POINT('Ctrl Pts',(0.24395391162551,2.31161965387523,6.67636543473339));
#59094=CARTESIAN_POINT('Ctrl Pts',(0.229747551353077,2.32696335852053,6.67779353296056));
#59095=CARTESIAN_POINT('Ctrl Pts',(0.210392584851175,2.3441752460367,6.67952672896297));
#59096=CARTESIAN_POINT('Ctrl Pts',(0.20654713192356,2.34743661188732,6.67986173134638));
#59097=CARTESIAN_POINT('Ctrl Pts',(0.201388699498098,2.35160743538036,6.68029749026662));
#59098=CARTESIAN_POINT('Ctrl Pts',(0.200143377555439,2.35259916550958,6.68040167525754));
#59099=CARTESIAN_POINT('Ctrl Pts',(0.194303158707849,2.35717980240808,6.6808853886833));
#59100=CARTESIAN_POINT('Ctrl Pts',(0.189618412515926,2.3606530961014,6.68125944002314));
#59101=CARTESIAN_POINT('Ctrl Pts',(0.184301917989786,2.36437551469702,6.68166638845782));
#59102=CARTESIAN_POINT('Ctrl Pts',(0.183761021906018,2.36475176409661,6.68170759354653));
#59103=CARTESIAN_POINT('Ctrl Pts',(0.182999470483632,2.36527804397849,6.6817653266783));
#59104=CARTESIAN_POINT('Ctrl Pts',(0.182779781593757,2.36542946003816,6.68178194850408));
#59105=CARTESIAN_POINT('Ctrl Pts',(0.182376562742072,2.36570663236852,6.68181239592652));
#59106=CARTESIAN_POINT('Ctrl Pts',(0.182193090199527,2.36583247169365,6.68182622721691));
#59107=CARTESIAN_POINT('Ctrl Pts',(0.181818800492192,2.36608861832693,6.6818543966148));
#59108=CARTESIAN_POINT('Ctrl Pts',(0.181627973458669,2.36621891043587,6.68186873367684));
#59109=CARTESIAN_POINT('Ctrl Pts',(0.18115621237406,2.36654027420806,6.68190411696132));
#59110=CARTESIAN_POINT('Ctrl Pts',(0.180875115170277,2.3667311076183,6.68192514689624));
#59111=CARTESIAN_POINT('Ctrl Pts',(0.179826078021078,2.36744086504932,6.6820034337586));
#59112=CARTESIAN_POINT('Ctrl Pts',(0.179056192895018,2.36795692652046,6.68206049834049));
#59113=CARTESIAN_POINT('Ctrl Pts',(0.177146055461729,2.36922540165571,6.68220114596431));
#59114=CARTESIAN_POINT('Ctrl Pts',(0.176003213337471,2.3699739078248,6.68228447858582));
#59115=CARTESIAN_POINT('Ctrl Pts',(0.17153821047989,2.37285786496532,6.68260702888197));
#59116=CARTESIAN_POINT('Ctrl Pts',(0.168181526489185,2.37493953762409,6.68284304666794));
#59117=CARTESIAN_POINT('Ctrl Pts',(0.160226638593374,2.37967259856458,6.68338945740611));
#59118=CARTESIAN_POINT('Ctrl Pts',(0.15559945994752,2.38227318607562,6.68369745468987));
#59119=CARTESIAN_POINT('Ctrl Pts',(0.139412597132232,2.39085154053913,6.68474861856945));
#59120=CARTESIAN_POINT('Ctrl Pts',(0.127556222363953,2.39624303039463,6.68547379218808));
#59121=CARTESIAN_POINT('Ctrl Pts',(0.111614060275958,2.40235735455902,6.6864282262624));
#59122=CARTESIAN_POINT('Ctrl Pts',(0.107795127994884,2.40373982015107,6.68665532603328));
#59123=CARTESIAN_POINT('Ctrl Pts',(0.0916133909093569,2.4092540342703,6.6876142318097));
#59124=CARTESIAN_POINT('Ctrl Pts',(0.0790327281646841,2.41270570911318,
6.68835215218976));
#59125=CARTESIAN_POINT('Ctrl Pts',(0.0570537308224934,2.41732459719919,
6.6896610448679));
#59126=CARTESIAN_POINT('Ctrl Pts',(0.0477492413629225,2.41885735344982,
6.6902208958949));
#59127=CARTESIAN_POINT('Ctrl Pts',(0.0372546255473993,2.42011650970681,
6.69086367596115));
#59128=CARTESIAN_POINT('Ctrl Pts',(0.0361169583365184,2.42024686131027,
6.69093350163627));
#59129=CARTESIAN_POINT('Ctrl Pts',(0.0344620323983008,2.42042754876007,
6.69103529352009));
#59130=CARTESIAN_POINT('Ctrl Pts',(0.0339452995903808,2.42048270204822,
6.69106710791667));
#59131=CARTESIAN_POINT('Ctrl Pts',(0.0330336200962892,2.42057778017967,
6.69112329398979));
#59132=CARTESIAN_POINT('Ctrl Pts',(0.0326387278411285,2.42061822568947,
6.6911476492208));
#59133=CARTESIAN_POINT('Ctrl Pts',(0.0318226280977629,2.42070028860927,
6.69119802099171));
#59134=CARTESIAN_POINT('Ctrl Pts',(0.0314014115239478,2.42074180601334,
6.69122404062985));
#59135=CARTESIAN_POINT('Ctrl Pts',(0.0303237923561696,2.42084587892096,
6.69129066243472));
#59136=CARTESIAN_POINT('Ctrl Pts',(0.0296672796847925,2.42090724969874,
6.69133130179642));
#59137=CARTESIAN_POINT('Ctrl Pts',(0.0269937487641927,2.42114889696245,
6.69149701209792));
#59138=CARTESIAN_POINT('Ctrl Pts',(0.0249752750714482,2.42131217192448,
6.69162261622494));
#59139=CARTESIAN_POINT('Ctrl Pts',(-0.00838774946760224,2.4236946494542,
6.693707222624));
#59140=CARTESIAN_POINT('Ctrl Pts',(-0.0398832638499902,2.42133618663887,
6.69582444754338));
#59141=CARTESIAN_POINT('Ctrl Pts',(-0.0783202357909937,2.41271530721903,
6.69848659044372));
#59142=CARTESIAN_POINT('Ctrl Pts',(-0.0860435463694925,2.41067899904203,
6.69902414060131));
#59143=CARTESIAN_POINT('Ctrl Pts',(-0.103123955083956,2.40548972772596,
6.70020932019838));
#59144=CARTESIAN_POINT('Ctrl Pts',(-0.112428837767536,2.40218922000245,
6.7008524737216));
#59145=CARTESIAN_POINT('Ctrl Pts',(-0.122244345139656,2.39819126108725,
6.70151769108359));
#59146=CARTESIAN_POINT('Ctrl Pts',(-0.122919221312364,2.397913700866,6.70156335962871));
#59147=CARTESIAN_POINT('Ctrl Pts',(-0.123857547549199,2.39752405868474,
6.70162675330342));
#59148=CARTESIAN_POINT('Ctrl Pts',(-0.124121793275338,2.39741391698577,
6.70164459450796));
#59149=CARTESIAN_POINT('Ctrl Pts',(-0.124577001556301,2.39722346681187,
6.70167530902859));
#59150=CARTESIAN_POINT('Ctrl Pts',(-0.124768033479432,2.39714332629667,
6.70168819255405));
#59151=CARTESIAN_POINT('Ctrl Pts',(-0.125163981208132,2.39697677163485,
6.70171488314916));
#59152=CARTESIAN_POINT('Ctrl Pts',(-0.125368884519984,2.39689032971282,
6.70172868840381));
#59153=CARTESIAN_POINT('Ctrl Pts',(-0.125776123986787,2.39671803209559,
6.70175611200294));
#59154=CARTESIAN_POINT('Ctrl Pts',(-0.12597846236604,2.3966321812555,6.70176973066547));
#59155=CARTESIAN_POINT('Ctrl Pts',(-0.126450733484886,2.39643122935603,
6.70180150187544));
#59156=CARTESIAN_POINT('Ctrl Pts',(-0.126720597705499,2.39631596625084,
6.70181964456846));
#59157=CARTESIAN_POINT('Ctrl Pts',(-0.128260115953721,2.39565592684532,
6.70192307862415));
#59158=CARTESIAN_POINT('Ctrl Pts',(-0.129526439399022,2.39510334813591,
6.70200790072098));
#59159=CARTESIAN_POINT('Ctrl Pts',(-0.132881910086661,2.39361337938705,
6.70223207588046));
#59160=CARTESIAN_POINT('Ctrl Pts',(-0.134964726741288,2.39266182152779,
6.70237062099168));
#59161=CARTESIAN_POINT('Ctrl Pts',(-0.144659581858135,2.38810710504971,
6.70301346580374));
#59162=CARTESIAN_POINT('Ctrl Pts',(-0.152139225106059,2.38422839071104,
6.7035035330709));
#59163=CARTESIAN_POINT('Ctrl Pts',(-0.166729677598269,2.37592098985497,
6.70446422972996));
#59164=CARTESIAN_POINT('Ctrl Pts',(-0.173836777819929,2.37149947106736,
6.70493461024682));
#59165=CARTESIAN_POINT('Ctrl Pts',(-0.199887121818747,2.35385009469461,
6.70669647172027));
#59166=CARTESIAN_POINT('Ctrl Pts',(-0.217560234037594,2.33887690996202,
6.70797574497701));
#59167=CARTESIAN_POINT('Ctrl Pts',(-0.238669612388335,2.31669023517607,
6.70977562260539));
#59168=CARTESIAN_POINT('Ctrl Pts',(-0.243665423848541,2.31105683894828,
6.71022516727129));
#59169=CARTESIAN_POINT('Ctrl Pts',(-0.249076957457928,2.3045061999595,6.71074213040877));
#59170=CARTESIAN_POINT('Ctrl Pts',(-0.249691367760026,2.30375558248127,
6.71080128374122));
#59171=CARTESIAN_POINT('Ctrl Pts',(-0.250616094032689,2.30261539202133,
6.71089101637054));
#59172=CARTESIAN_POINT('Ctrl Pts',(-0.250928914858841,2.30222785009866,
6.71092149470974));
#59173=CARTESIAN_POINT('Ctrl Pts',(-0.251471380539031,2.3015526132297,6.71097456301667));
#59174=CARTESIAN_POINT('Ctrl Pts',(-0.251701433758816,2.30126524630909,
6.71099713654655));
#59175=CARTESIAN_POINT('Ctrl Pts',(-0.252180237198817,2.3006650525851,6.71104426046144));
#59176=CARTESIAN_POINT('Ctrl Pts',(-0.252428898729361,2.30035215608191,
6.7110688143414));
#59177=CARTESIAN_POINT('Ctrl Pts',(-0.253015152701141,2.29961163533312,
6.71112689482671));
#59178=CARTESIAN_POINT('Ctrl Pts',(-0.253352243281556,2.29918361698476,
6.71116044135962));
#59179=CARTESIAN_POINT('Ctrl Pts',(-0.254460152590617,2.29776949444762,
6.7112711985098));
#59180=CARTESIAN_POINT('Ctrl Pts',(-0.255226304829458,2.29677976380397,
6.71134859394398));
#59181=CARTESIAN_POINT('Ctrl Pts',(-0.259652769490427,2.29099222946145,
6.71180049157234));
#59182=CARTESIAN_POINT('Ctrl Pts',(-0.26318330106082,2.28609711046256,6.71218004372892));
#59183=CARTESIAN_POINT('Ctrl Pts',(-0.275331984213955,2.2682151819066,6.7135584033772));
#59184=CARTESIAN_POINT('Ctrl Pts',(-0.283142080295269,2.25470777824621,
6.7145860116383));
#59185=CARTESIAN_POINT('Ctrl Pts',(-0.292412910025094,2.23560181715299,
6.7160119995205));
#59186=CARTESIAN_POINT('Ctrl Pts',(-0.294747514937318,2.230449465473,6.71639380496975));
#59187=CARTESIAN_POINT('Ctrl Pts',(-0.298048129211772,2.2226235787422,6.71696824444314));
#59188=CARTESIAN_POINT('Ctrl Pts',(-0.299116375467834,2.21999426351854,
6.71716032889619));
#59189=CARTESIAN_POINT('Ctrl Pts',(-0.301325466768272,2.21434405896533,
6.71757084737076));
#59190=CARTESIAN_POINT('Ctrl Pts',(-0.302455927953545,2.2113194169866,6.71778924527279));
#59191=CARTESIAN_POINT('Ctrl Pts',(-0.304326815530602,2.20607468465119,
6.71816519606519));
#59192=CARTESIAN_POINT('Ctrl Pts',(-0.305088865559112,2.20386257106296,
6.71832293016905));
#59193=CARTESIAN_POINT('Ctrl Pts',(-0.310348052728714,2.18803845453742,
6.71944461680408));
#59194=CARTESIAN_POINT('Ctrl Pts',(-0.313957232983756,2.17414612796845,
6.72039514285422));
#59195=CARTESIAN_POINT('Ctrl Pts',(-0.316797686513221,2.1591710768528,6.72135363078277));
#59196=CARTESIAN_POINT('Ctrl Pts',(-0.316962188056315,2.15828346167526,
6.72141019770417));
#59197=CARTESIAN_POINT('Ctrl Pts',(-0.317178704001938,2.1570871555029,6.72148609610303));
#59198=CARTESIAN_POINT('Ctrl Pts',(-0.317233999390033,2.15677907386341,
6.7215056115936));
#59199=CARTESIAN_POINT('Ctrl Pts',(-0.317326424413128,2.1562597723572,6.72153845501799));
#59200=CARTESIAN_POINT('Ctrl Pts',(-0.317363792057402,2.15604859595089,
6.7215517965172));
#59201=CARTESIAN_POINT('Ctrl Pts',(-0.317435122519377,2.15564312643118,
6.72157738496654));
#59202=CARTESIAN_POINT('Ctrl Pts',(-0.317469117512383,2.15544884087231,
6.72158963365203));
#59203=CARTESIAN_POINT('Ctrl Pts',(-0.317538950072604,2.1550475697773,6.72161490635898));
#59204=CARTESIAN_POINT('Ctrl Pts',(-0.317574763509821,2.1548405810863,6.72162792894951));
#59205=CARTESIAN_POINT('Ctrl Pts',(-0.317655207364524,2.15437292339899,
6.72165732032001));
#59206=CARTESIAN_POINT('Ctrl Pts',(-0.317699719421908,2.1541122337848,6.72167368234888));
#59207=CARTESIAN_POINT('Ctrl Pts',(-0.317811374478801,2.1534534272156,6.72171497754669));
#59208=CARTESIAN_POINT('Ctrl Pts',(-0.31787809057946,2.15305523690371,6.72173988666838));
#59209=CARTESIAN_POINT('Ctrl Pts',(-0.318065972638084,2.15192079940594,
6.72181071217877));
#59210=CARTESIAN_POINT('Ctrl Pts',(-0.31818533119747,2.15118424950437,6.72185652863981));
#59211=CARTESIAN_POINT('Ctrl Pts',(-0.320931852769821,2.13385479954498,
6.72293068408991));
#59212=CARTESIAN_POINT('Ctrl Pts',(-0.322260476271441,2.11707992411669,
6.72388901335813));
#59213=CARTESIAN_POINT('Ctrl Pts',(-0.322274881577486,2.10027627742869,
6.72483370602588));
#59214=CARTESIAN_POINT('',(-0.322274855983169,2.09970202152027,6.97470119816725));
#59215=CARTESIAN_POINT('Ctrl Pts',(-0.322274881319243,2.10027657850254,
6.72483368909966));
#59216=CARTESIAN_POINT('Ctrl Pts',(-0.322292341980155,2.07993106223288,
6.7259775041476));
#59217=CARTESIAN_POINT('Ctrl Pts',(-0.320383196143773,2.05962956821057,
6.72709872414235));
#59218=CARTESIAN_POINT('Ctrl Pts',(-0.314408027524657,2.02828985983309,
6.72893409671193));
#59219=CARTESIAN_POINT('Ctrl Pts',(-0.311634562382442,2.01706263284682,
6.72961273384056));
#59220=CARTESIAN_POINT('Ctrl Pts',(-0.307665440760797,2.00404495838612,
6.73043554183747));
#59221=CARTESIAN_POINT('Ctrl Pts',(-0.307047721710094,2.00208631485001,
6.73056030725184));
#59222=CARTESIAN_POINT('Ctrl Pts',(-0.306205916898104,1.99950347510119,
6.73072615883518));
#59223=CARTESIAN_POINT('Ctrl Pts',(-0.305998555478583,1.99887384564408,
6.73076669379932));
#59224=CARTESIAN_POINT('Ctrl Pts',(-0.305655368292431,1.9978425173206,6.73083326315196));
#59225=CARTESIAN_POINT('Ctrl Pts',(-0.305520688992642,1.99744043668135,
6.73085925964289));
#59226=CARTESIAN_POINT('Ctrl Pts',(-0.305258496270871,1.99666276854238,
6.73090962407456));
#59227=CARTESIAN_POINT('Ctrl Pts',(-0.305131082178761,1.99628714815867,
6.7309339886917));
#59228=CARTESIAN_POINT('Ctrl Pts',(-0.304835751619087,1.99542176025312,
6.73099021056599));
#59229=CARTESIAN_POINT('Ctrl Pts',(-0.304667348007322,1.99493216121512,
6.73102208391396));
#59230=CARTESIAN_POINT('Ctrl Pts',(-0.304213610614897,1.99362327609867,
6.73110746989048));
#59231=CARTESIAN_POINT('Ctrl Pts',(-0.303926148677729,1.99280473705577,
6.73116105304204));
#59232=CARTESIAN_POINT('Ctrl Pts',(-0.301896082869726,1.98709799843725,
6.73153593476974));
#59233=CARTESIAN_POINT('Ctrl Pts',(-0.300039021659239,1.98225159352048,
6.7318610300894));
#59234=CARTESIAN_POINT('Ctrl Pts',(-0.297424160138748,1.97589161079522,
6.73229698323918));
#59235=CARTESIAN_POINT('Ctrl Pts',(-0.296770233209781,1.97433595655503,
6.73240436742688));
#59236=CARTESIAN_POINT('Ctrl Pts',(-0.295892459109921,1.97229285139125,
6.73254639524188));
#59237=CARTESIAN_POINT('Ctrl Pts',(-0.295679561348259,1.97180070140844,
6.73258068391327));
#59238=CARTESIAN_POINT('Ctrl Pts',(-0.285421723617948,1.94824941523974,
6.73422520285443));
#59239=CARTESIAN_POINT('Ctrl Pts',(-0.272714391273855,1.92644812541136,
6.73592668510302));
#59240=CARTESIAN_POINT('Ctrl Pts',(-0.253385692743078,1.90073587753876,
6.73810112892537));
#59241=CARTESIAN_POINT('Ctrl Pts',(-0.248983097329683,1.89526133038115,
6.73857446766915));
#59242=CARTESIAN_POINT('Ctrl Pts',(-0.237351756600428,1.88172858428139,
6.73976429583988));
#59243=CARTESIAN_POINT('Ctrl Pts',(-0.229888776992585,1.87388172872463,
6.74047327355406));
#59244=CARTESIAN_POINT('Ctrl Pts',(-0.221344368608981,1.86575914393208,
6.74121502202174));
#59245=CARTESIAN_POINT('Ctrl Pts',(-0.22064147300544,1.86509693783851,6.74127555320187));
#59246=CARTESIAN_POINT('Ctrl Pts',(-0.219742810914166,1.86425789038692,
6.74135231217217));
#59247=CARTESIAN_POINT('Ctrl Pts',(-0.219549799208646,1.86407812551204,
6.7413687613954));
#59248=CARTESIAN_POINT('Ctrl Pts',(-0.219202822383161,1.86375575705495,
6.74139826573993));
#59249=CARTESIAN_POINT('Ctrl Pts',(-0.219048938544433,1.86361306679814,
6.74141132750304));
#59250=CARTESIAN_POINT('Ctrl Pts',(-0.218750220566145,1.86333661986971,
6.74143663738265));
#59251=CARTESIAN_POINT('Ctrl Pts',(-0.218605403207598,1.86320284591739,
6.74144888681532));
#59252=CARTESIAN_POINT('Ctrl Pts',(-0.218302518173839,1.86292357279012,
6.74147446317797));
#59253=CARTESIAN_POINT('Ctrl Pts',(-0.218144428248557,1.86277809923107,
6.74148778814097));
#59254=CARTESIAN_POINT('Ctrl Pts',(-0.217754655672758,1.86242015157136,
6.74152058094793));
#59255=CARTESIAN_POINT('Ctrl Pts',(-0.217522806788386,1.86220785762477,
6.74154003498747));
#59256=CARTESIAN_POINT('Ctrl Pts',(-0.216617077183814,1.86138095349516,
6.7416158317742));
#59257=CARTESIAN_POINT('Ctrl Pts',(-0.215940890815322,1.86076885820684,
6.74167198502214));
#59258=CARTESIAN_POINT('Ctrl Pts',(-0.204038278570644,1.85008599691239,
6.7426530360272));
#59259=CARTESIAN_POINT('Ctrl Pts',(-0.192119436851868,1.84081110647185,
6.74352098036951));
#59260=CARTESIAN_POINT('Ctrl Pts',(-0.17009659507384,1.82603078979801,6.74501901412576));
#59261=CARTESIAN_POINT('Ctrl Pts',(-0.160267412040684,1.82016729002085,
6.74565476331232));
#59262=CARTESIAN_POINT('Ctrl Pts',(-0.138480307197349,1.80869563526606,
6.74703380160354));
#59263=CARTESIAN_POINT('Ctrl Pts',(-0.126448068382314,1.80327474235609,
6.74777758986689));
#59264=CARTESIAN_POINT('Ctrl Pts',(-0.106073331073699,1.79556014540796,
6.74904200571659));
#59265=CARTESIAN_POINT('Ctrl Pts',(-0.0979101866706216,1.79283757927498,
6.74954967417675));
#59266=CARTESIAN_POINT('Ctrl Pts',(-0.0871822558279221,1.78973072679797,
6.75022293167715));
#59267=CARTESIAN_POINT('Ctrl Pts',(-0.0847077139084813,1.78904603195827,
6.75037862882173));
#59268=CARTESIAN_POINT('Ctrl Pts',(-0.0815295559684236,1.78820740081492,
6.75057919512504));
#59269=CARTESIAN_POINT('Ctrl Pts',(-0.080833194380414,1.78802614199899,
6.75062317740628));
#59270=CARTESIAN_POINT('Ctrl Pts',(-0.0797132685617597,1.78773863330169,
6.75069397270331));
#59271=CARTESIAN_POINT('Ctrl Pts',(-0.0792900825184149,1.78763090881404,
6.75072073798875));
#59272=CARTESIAN_POINT('Ctrl Pts',(-0.0784856693940366,1.78742788073499,
6.75077164166492));
#59273=CARTESIAN_POINT('Ctrl Pts',(-0.0781044840931819,1.78733241356928,
6.75079577472103));
#59274=CARTESIAN_POINT('Ctrl Pts',(-0.0772377915514198,1.78711703581432,
6.75085067196637));
#59275=CARTESIAN_POINT('Ctrl Pts',(-0.0767521787467464,1.78699755787775,
6.75088145005175));
#59276=CARTESIAN_POINT('Ctrl Pts',(-0.0753123219047789,1.78664685442312,
6.75097276493727));
#59277=CARTESIAN_POINT('Ctrl Pts',(-0.0743573035177538,1.78641886049538,
6.75103340566745));
#59278=CARTESIAN_POINT('Ctrl Pts',(-0.0678261979626444,1.78489118636413,
6.75144863373122));
#59279=CARTESIAN_POINT('Ctrl Pts',(-0.0622176806293128,1.78373601060769,
6.75180783457533));
#59280=CARTESIAN_POINT('Ctrl Pts',(-0.0562352626013929,1.78266910855679,
6.75219409180155));
#59281=CARTESIAN_POINT('Ctrl Pts',(-0.0558887772316407,1.78260790179655,
6.75221647367286));
#59282=CARTESIAN_POINT('Ctrl Pts',(-0.0324493027619221,1.77850688242696,
6.75373132976085));
#59283=CARTESIAN_POINT('Ctrl Pts',(-0.00898823194892534,1.77699901746954,
6.75530395830445));
#59284=CARTESIAN_POINT('Ctrl Pts',(0.0280152198955742,1.77865687080403,
6.75781059379957));
#59285=CARTESIAN_POINT('Ctrl Pts',(0.0415546743414955,1.78012579328335,
6.75873148107395));
#59286=CARTESIAN_POINT('Ctrl Pts',(0.0602374623161578,1.78335936000663,
6.75997838322112));
#59287=CARTESIAN_POINT('Ctrl Pts',(0.065490330798409,1.78440394396361,6.76032620013949));
#59288=CARTESIAN_POINT('Ctrl Pts',(0.0723782998198994,1.78595308678523,
6.76077655527912));
#59289=CARTESIAN_POINT('Ctrl Pts',(0.0740386049570744,1.78634036400982,
6.76088466699732));
#59290=CARTESIAN_POINT('Ctrl Pts',(0.0767649041583947,1.78699914562723,
6.76106137266218));
#59291=CARTESIAN_POINT('Ctrl Pts',(0.077832697882508,1.78726295938607,6.76113037436944));
#59292=CARTESIAN_POINT('Ctrl Pts',(0.0792524377324671,1.78762144837189,
6.76122182316244));
#59293=CARTESIAN_POINT('Ctrl Pts',(0.0796055877380693,1.78771125731494,
6.76124454595599));
#59294=CARTESIAN_POINT('Ctrl Pts',(0.0801570843221477,1.78785250370413,
6.76127999198451));
#59295=CARTESIAN_POINT('Ctrl Pts',(0.0803555340441774,1.78790353132429,
6.76129273893185));
#59296=CARTESIAN_POINT('Ctrl Pts',(0.0807660394355996,1.78800950257269,
6.76131909022812));
#59297=CARTESIAN_POINT('Ctrl Pts',(0.0809780861113127,1.78806447271735,
6.76133269281748));
#59298=CARTESIAN_POINT('Ctrl Pts',(0.0814613381350981,1.78819027503527,
6.76136367223391));
#59299=CARTESIAN_POINT('Ctrl Pts',(0.0817325067575552,1.78826124473545,
6.76138104093861));
#59300=CARTESIAN_POINT('Ctrl Pts',(0.0825596615257031,1.7884788794588,6.76143397687228));
#59301=CARTESIAN_POINT('Ctrl Pts',(0.083115351874641,1.78862667977282,6.76146947846353));
#59302=CARTESIAN_POINT('Ctrl Pts',(0.0871341297739221,1.7897071032596,6.7617258036703));
#59303=CARTESIAN_POINT('Ctrl Pts',(0.0905820022436709,1.79069603653874,
6.76194343533742));
#59304=CARTESIAN_POINT('Ctrl Pts',(0.103475462442264,1.7946283010598,6.76275116110119));
#59305=CARTESIAN_POINT('Ctrl Pts',(0.112801091684172,1.79794868829559,6.7633230028282));
#59306=CARTESIAN_POINT('Ctrl Pts',(0.141635186479585,1.80973723614822,6.76509399090638));
#59307=CARTESIAN_POINT('Ctrl Pts',(0.160466451628482,1.81970807859022,6.76625821981235));
#59308=CARTESIAN_POINT('Ctrl Pts',(0.186006574408517,1.83665427667127,6.76800308841223));
#59309=CARTESIAN_POINT('Ctrl Pts',(0.193602572730806,1.84218720149462,6.76854532625982));
#59310=CARTESIAN_POINT('Ctrl Pts',(0.20628775483523,1.85230416378483,6.76950261112197));
#59311=CARTESIAN_POINT('Ctrl Pts',(0.211492624015434,1.85673322348962,6.76991175343408));
#59312=CARTESIAN_POINT('Ctrl Pts',(0.21726448581017,1.86197007965197,6.77038634432576));
#59313=CARTESIAN_POINT('Ctrl Pts',(0.217973541898985,1.86261921986852,6.77044501806585));
#59314=CARTESIAN_POINT('Ctrl Pts',(0.219038965016669,1.86360341230984,6.77053374863671));
#59315=CARTESIAN_POINT('Ctrl Pts',(0.219397495396707,1.86393612331279,6.77056370558625));
#59316=CARTESIAN_POINT('Ctrl Pts',(0.220014731474875,1.86451153024235,6.7706154484375));
#59317=CARTESIAN_POINT('Ctrl Pts',(0.220273797189978,1.86475384014901,6.77063721776757));
#59318=CARTESIAN_POINT('Ctrl Pts',(0.220808319819621,1.86525544812339,6.770682241432));
#59319=CARTESIAN_POINT('Ctrl Pts',(0.221083721186264,1.8655148043866,6.77070549825435));
#59320=CARTESIAN_POINT('Ctrl Pts',(0.221748671071617,1.86614322660808,6.77076179543896));
#59321=CARTESIAN_POINT('Ctrl Pts',(0.222137754707119,1.86651278083923,6.77079485687244));
#59322=CARTESIAN_POINT('Ctrl Pts',(0.223575895791958,1.86788558536415,6.77091750722796));
#59323=CARTESIAN_POINT('Ctrl Pts',(0.224619082267808,1.86889493637861,6.77100736093444));
#59324=CARTESIAN_POINT('Ctrl Pts',(0.242252503340233,1.88618859956074,6.77254151569527));
#59325=CARTESIAN_POINT('Ctrl Pts',(0.257036192194062,1.90421038442269,6.77406789104859));
#59326=CARTESIAN_POINT('Ctrl Pts',(0.278439762049603,1.93695210442297,6.77670327256075));
#59327=CARTESIAN_POINT('Ctrl Pts',(0.286134086416015,1.95086713285716,6.77778576052273));
#59328=CARTESIAN_POINT('Ctrl Pts',(0.296045782475372,1.9724091118301,6.77936535156051));
#59329=CARTESIAN_POINT('Ctrl Pts',(0.299059829220571,1.97964312217989,6.77988039487894));
#59330=CARTESIAN_POINT('Ctrl Pts',(0.302583432206568,1.98905254199192,6.78052480271146));
#59331=CARTESIAN_POINT('Ctrl Pts',(0.303338090653373,1.99113276316231,6.78066569849326));
#59332=CARTESIAN_POINT('Ctrl Pts',(0.304367841520667,1.99406514370936,6.78086195440985));
#59333=CARTESIAN_POINT('Ctrl Pts',(0.304660881200354,1.99491087478021,6.78091828314932));
#59334=CARTESIAN_POINT('Ctrl Pts',(0.305161429082977,1.99637517921468,6.78101532523165));
#59335=CARTESIAN_POINT('Ctrl Pts',(0.305370587516357,1.99699317702071,6.78105613195548));
#59336=CARTESIAN_POINT('Ctrl Pts',(0.305673202820218,1.99789633335023,6.78111554596668));
#59337=CARTESIAN_POINT('Ctrl Pts',(0.30576813873378,1.99818098899159,6.78113423988265));
#59338=CARTESIAN_POINT('Ctrl Pts',(0.305932910277509,1.99867734839268,6.78116678035159));
#59339=CARTESIAN_POINT('Ctrl Pts',(0.306002923974494,1.99888899248922,6.78118063749877));
#59340=CARTESIAN_POINT('Ctrl Pts',(0.306137338614457,1.99929673227065,6.78120729915661));
#59341=CARTESIAN_POINT('Ctrl Pts',(0.306201770640241,1.9994928167607,6.78122010552555));
#59342=CARTESIAN_POINT('Ctrl Pts',(0.30635421635015,1.99995825846805,6.78125046755219));
#59343=CARTESIAN_POINT('Ctrl Pts',(0.306442063409475,2.00022767067453,6.78126801330627));
#59344=CARTESIAN_POINT('Ctrl Pts',(0.306749625091868,2.0011751489905,6.78132961900819));
#59345=CARTESIAN_POINT('Ctrl Pts',(0.306967447514603,2.00185383420496,6.78137356801362));
#59346=CARTESIAN_POINT('Ctrl Pts',(0.309853077375612,2.01094838633347,6.78196016409799));
#59347=CARTESIAN_POINT('Ctrl Pts',(0.31217650115249,2.0194705994882,6.78248317402636));
#59348=CARTESIAN_POINT('Ctrl Pts',(0.319665781305849,2.05218308000831,6.78442784987435));
#59349=CARTESIAN_POINT('Ctrl Pts',(0.322392088917836,2.07684418030572,6.78577123025557));
#59350=CARTESIAN_POINT('Ctrl Pts',(0.322188812319144,2.118412714764,6.78813102960269));
#59351=CARTESIAN_POINT('Ctrl Pts',(0.3207872500352,2.13521470559871,6.78910989030885));
#59352=CARTESIAN_POINT('Ctrl Pts',(0.317888527833361,2.15300451201013,6.7902056407977));
#59353=CARTESIAN_POINT('Ctrl Pts',(0.317690453446088,2.15417905638807,6.7902782566166));
#59354=CARTESIAN_POINT('Ctrl Pts',(0.317394174823475,2.15587842569497,6.79038372066029));
#59355=CARTESIAN_POINT('Ctrl Pts',(0.317301168882254,2.15640415667803,6.7904164035814));
#59356=CARTESIAN_POINT('Ctrl Pts',(0.317136586631268,2.15732119405874,6.79047351081591));
#59357=CARTESIAN_POINT('Ctrl Pts',(0.317065591214247,2.15771260463813,6.79049791659506));
#59358=CARTESIAN_POINT('Ctrl Pts',(0.31692702171328,2.15846858997967,6.79054511559125));
#59359=CARTESIAN_POINT('Ctrl Pts',(0.316859542747316,2.15883318174668,6.79056790574401));
#59360=CARTESIAN_POINT('Ctrl Pts',(0.316698035873523,2.15969747264203,6.79062199661888));
#59361=CARTESIAN_POINT('Ctrl Pts',(0.316603454475463,2.16019706616992,6.79065331494687));
#59362=CARTESIAN_POINT('Ctrl Pts',(0.316266717042569,2.16195301763072,6.79076357463993));
#59363=CARTESIAN_POINT('Ctrl Pts',(0.316018264212374,2.16320814275396,6.79084271670036));
#59364=CARTESIAN_POINT('Ctrl Pts',(0.312238252707394,2.18172432446622,6.79201522237486));
#59365=CARTESIAN_POINT('Ctrl Pts',(0.307305162130927,2.19866581049313,6.79315439192311));
#59366=CARTESIAN_POINT('Ctrl Pts',(0.293527889532114,2.23469126497403,6.79572051521411));
#59367=CARTESIAN_POINT('Ctrl Pts',(0.284151298061953,2.25348721669295,6.79715601492943));
#59368=CARTESIAN_POINT('Ctrl Pts',(0.269753047903673,2.27644319869376,6.79896557159278));
#59369=CARTESIAN_POINT('Ctrl Pts',(0.266340814353595,2.28155298971093,6.7993719763893));
#59370=CARTESIAN_POINT('Ctrl Pts',(0.259797692651815,2.29076937367466,6.80010769002199));
#59371=CARTESIAN_POINT('Ctrl Pts',(0.256710150033287,2.29490433867707,6.80043881622971));
#59372=CARTESIAN_POINT('Ctrl Pts',(0.252923175368309,2.29972979619699,6.80082478543587));
#59373=CARTESIAN_POINT('Ctrl Pts',(0.25231843076531,2.30049322602366,6.80088583511165));
#59374=CARTESIAN_POINT('Ctrl Pts',(0.251493508429981,2.30152496440155,6.80096830803059));
#59375=CARTESIAN_POINT('Ctrl Pts',(0.251276352473662,2.30179566583477,6.80098994371064));
#59376=CARTESIAN_POINT('Ctrl Pts',(0.250930674640275,2.3022251563981,6.80102426491124));
#59377=CARTESIAN_POINT('Ctrl Pts',(0.250802439104796,2.30238417402382,6.80103697100736));
#59378=CARTESIAN_POINT('Ctrl Pts',(0.250535444734357,2.30271461515251,6.80106337172469));
#59379=CARTESIAN_POINT('Ctrl Pts',(0.250396661510784,2.3028860176778,6.80107706441354));
#59380=CARTESIAN_POINT('Ctrl Pts',(0.250077028247968,2.30327994931401,6.80110853073044));
#59381=CARTESIAN_POINT('Ctrl Pts',(0.249896056552528,2.30350238025995,6.80112629552463));
#59382=CARTESIAN_POINT('Ctrl Pts',(0.24941228093658,2.30409536678504,6.80117364965696));
#59383=CARTESIAN_POINT('Ctrl Pts',(0.249108946684217,2.30446549174358,6.80120320081684));
#59384=CARTESIAN_POINT('Ctrl Pts',(0.247030885342589,2.30698962948522,6.80140470089151));
#59385=CARTESIAN_POINT('Ctrl Pts',(0.245228996862376,2.30912126956893,6.80157472009918));
#59386=CARTESIAN_POINT('Ctrl Pts',(0.221389415797427,2.33659162209649,6.80376787697726));
#59387=CARTESIAN_POINT('Ctrl Pts',(0.195547219496606,2.35836209614145,6.80554796599594));
#59388=CARTESIAN_POINT('Ctrl Pts',(0.154406560414664,2.38324850156204,6.80829840060562));
#59389=CARTESIAN_POINT('Ctrl Pts',(0.141519497075983,2.38990213221643,6.8091471784033));
#59390=CARTESIAN_POINT('Ctrl Pts',(0.127219863668643,2.39610385604822,6.81009533823911));
#59391=CARTESIAN_POINT('Ctrl Pts',(0.126207770222817,2.39653665197878,6.81016247331863));
#59392=CARTESIAN_POINT('Ctrl Pts',(0.12471716954825,2.39716505590014,6.81026139525233));
#59393=CARTESIAN_POINT('Ctrl Pts',(0.124240369743966,2.39736471436474,6.81029304439665));
#59394=CARTESIAN_POINT('Ctrl Pts',(0.123398239717564,2.39771497477697,6.81034895649544));
#59395=CARTESIAN_POINT('Ctrl Pts',(0.123033108108095,2.39786605392165,6.81037320321135));
#59396=CARTESIAN_POINT('Ctrl Pts',(0.12232021182031,2.39815949190292,6.8104205521335));
#59397=CARTESIAN_POINT('Ctrl Pts',(0.12197247404919,2.39830191485144,6.81044365212389));
#59398=CARTESIAN_POINT('Ctrl Pts',(0.121136179867646,2.3986427290243,6.8104992167175));
#59399=CARTESIAN_POINT('Ctrl Pts',(0.120647385285245,2.39884052953133,6.81053170122564));
#59400=CARTESIAN_POINT('Ctrl Pts',(0.119150204066588,2.39944212193575,6.81063122815866));
#59401=CARTESIAN_POINT('Ctrl Pts',(0.11814026731536,2.39984201291814,6.81069840188693));
#59402=CARTESIAN_POINT('Ctrl Pts',(0.106259712374632,2.40447685354085,6.81148908428356));
#59403=CARTESIAN_POINT('Ctrl Pts',(0.0951701630401514,2.40812313236201,
6.8122322551355));
#59404=CARTESIAN_POINT('Ctrl Pts',(0.062759138451729,2.41686319684023,6.81442167471014));
#59405=CARTESIAN_POINT('Ctrl Pts',(0.041085348085757,2.42039472754361,6.81591081071072));
#59406=CARTESIAN_POINT('Ctrl Pts',(0.00242777394123436,2.4227048382318,
6.81852494522203));
#59407=CARTESIAN_POINT('Ctrl Pts',(-0.014424059179768,2.4223917037847,6.81964869117217));
#59408=CARTESIAN_POINT('Ctrl Pts',(-0.031878476210447,2.42069523865256,
6.82074888976668));
#59409=CARTESIAN_POINT('Ctrl Pts',(-0.0325804383976772,2.42062468463301,
6.82079302614161));
#59410=CARTESIAN_POINT('Ctrl Pts',(-0.0335853418388151,2.42052034778143,
6.82085604684138));
#59411=CARTESIAN_POINT('Ctrl Pts',(-0.0338884693153122,2.42048844000629,
6.82087503563732));
#59412=CARTESIAN_POINT('Ctrl Pts',(-0.0344129678737063,2.42043247783264,
6.8209078543737));
#59413=CARTESIAN_POINT('Ctrl Pts',(-0.0346343597642312,2.42040862399872,
6.82092169568889));
#59414=CARTESIAN_POINT('Ctrl Pts',(-0.0350612630779742,2.42036217972936,
6.82094836302101));
#59415=CARTESIAN_POINT('Ctrl Pts',(-0.0352667770187361,2.42033962104131,
6.82096119082727));
#59416=CARTESIAN_POINT('Ctrl Pts',(-0.0357552482891056,2.42028552715295,
6.82099165680791));
#59417=CARTESIAN_POINT('Ctrl Pts',(-0.0360381863900791,2.42025381466427,
6.82100928491814));
#59418=CARTESIAN_POINT('Ctrl Pts',(-0.036887200113352,2.42015751545781,
6.82106212637427));
#59419=CARTESIAN_POINT('Ctrl Pts',(-0.0374531506814395,2.42009180206938,
6.82109727656668));
#59420=CARTESIAN_POINT('Ctrl Pts',(-0.0429892991701606,2.41943410748912,
6.82144042067905));
#59421=CARTESIAN_POINT('Ctrl Pts',(-0.0479455764284708,2.41872787347188,
6.82174213051543));
#59422=CARTESIAN_POINT('Ctrl Pts',(-0.0662573599042714,2.41568170930456,
6.82284309040585));
#59423=CARTESIAN_POINT('Ctrl Pts',(-0.07947865079888,2.41261508945703,6.82361101719858));
#59424=CARTESIAN_POINT('Ctrl Pts',(-0.108737676633516,2.40385148298188,
6.8253246971275));
#59425=CARTESIAN_POINT('Ctrl Pts',(-0.12459569211984,2.39770035930134,6.82626459498531));
#59426=CARTESIAN_POINT('Ctrl Pts',(-0.153305656229379,2.38386643671697,
6.82808393367285));
#59427=CARTESIAN_POINT('Ctrl Pts',(-0.166250747039522,2.37648395363061,
6.82895410287386));
#59428=CARTESIAN_POINT('Ctrl Pts',(-0.179677563983831,2.36754197372882,
6.82993440911893));
#59429=CARTESIAN_POINT('Ctrl Pts',(-0.180712775149128,2.36684382611399,
6.83001050998267));
#59430=CARTESIAN_POINT('Ctrl Pts',(-0.182193374894341,2.36583274068711,
6.83012011071171));
#59431=CARTESIAN_POINT('Ctrl Pts',(-0.182642077491884,2.36552465685943,
6.83015342645639));
#59432=CARTESIAN_POINT('Ctrl Pts',(-0.183418827037244,2.36498843215475,
6.83021127530816));
#59433=CARTESIAN_POINT('Ctrl Pts',(-0.183747235113236,2.3647608144599,6.83023578845402));
#59434=CARTESIAN_POINT('Ctrl Pts',(-0.18437747314091,2.36432226281163,6.83028293666907));
#59435=CARTESIAN_POINT('Ctrl Pts',(-0.184679366747797,2.36411142102449,
6.8303055681922));
#59436=CARTESIAN_POINT('Ctrl Pts',(-0.185389122664073,2.36361391721632,
6.83035888588452));
#59437=CARTESIAN_POINT('Ctrl Pts',(-0.185796681613986,2.36332682591992,
6.83038958847558));
#59438=CARTESIAN_POINT('Ctrl Pts',(-0.186996818953137,2.36247725594961,
6.83048025427954));
#59439=CARTESIAN_POINT('Ctrl Pts',(-0.187787515677048,2.36191214006249,
6.83054031883728));
#59440=CARTESIAN_POINT('Ctrl Pts',(-0.194721389368632,2.35690891693216,
6.83106998258677));
#59441=CARTESIAN_POINT('Ctrl Pts',(-0.200708342372131,2.35225930449738,
6.8315477745733));
#59442=CARTESIAN_POINT('Ctrl Pts',(-0.210527541120479,2.34406250737537,
6.83236783588203));
#59443=CARTESIAN_POINT('Ctrl Pts',(-0.21444776180887,2.34062523939864,6.83270573019566));
#59444=CARTESIAN_POINT('Ctrl Pts',(-0.237697555721537,2.3192201564564,6.8347740198608));
#59445=CARTESIAN_POINT('Ctrl Pts',(-0.254842425256783,2.29902927550685,
6.83658859195294));
#59446=CARTESIAN_POINT('Ctrl Pts',(-0.273875175313273,2.27006474872148,
6.83890116622805));
#59447=CARTESIAN_POINT('Ctrl Pts',(-0.278151177437159,2.26297722292027,
6.83944610281646));
#59448=CARTESIAN_POINT('Ctrl Pts',(-0.283802239828319,2.25273884881567,
6.84019655784098));
#59449=CARTESIAN_POINT('Ctrl Pts',(-0.285406881337291,2.24971900907254,
6.84041355413997));
#59450=CARTESIAN_POINT('Ctrl Pts',(-0.287201255395476,2.24620837199312,
6.84066034763926));
#59451=CARTESIAN_POINT('Ctrl Pts',(-0.287438146261026,2.24574210518857,
6.84069301554226));
#59452=CARTESIAN_POINT('Ctrl Pts',(-0.287795471898968,2.24503452937019,
6.84074242118496));
#59453=CARTESIAN_POINT('Ctrl Pts',(-0.28791673908383,2.2447936452742,6.8407592110165));
#59454=CARTESIAN_POINT('Ctrl Pts',(-0.288135542048399,2.24435765519145,
6.84078954598172));
#59455=CARTESIAN_POINT('Ctrl Pts',(-0.2882331818201,2.2441626029962,6.84080309764972));
#59456=CARTESIAN_POINT('Ctrl Pts',(-0.288429017856206,2.24377039262779,
6.84083030806667));
#59457=CARTESIAN_POINT('Ctrl Pts',(-0.288527209592251,2.24357323379884,
6.84084396651655));
#59458=CARTESIAN_POINT('Ctrl Pts',(-0.288806761486751,2.24301047757681,
6.84088289604643));
#59459=CARTESIAN_POINT('Ctrl Pts',(-0.288987630252294,2.24264463446878,
6.84090813623155));
#59460=CARTESIAN_POINT('Ctrl Pts',(-0.28975856074101,2.24107778943558,6.84101595104108));
#59461=CARTESIAN_POINT('Ctrl Pts',(-0.290341845169806,2.23987344024012,
6.84109810783992));
#59462=CARTESIAN_POINT('Ctrl Pts',(-0.301583658052285,2.21628832188976,
6.84269377026068));
#59463=CARTESIAN_POINT('Ctrl Pts',(-0.30963420551681,2.19275112314791,6.84405818746292));
#59464=CARTESIAN_POINT('Ctrl Pts',(-0.317976313350995,2.15441227793425,
6.84625322047779));
#59465=CARTESIAN_POINT('Ctrl Pts',(-0.32009434862226,2.14011479458717,6.84706532725283));
#59466=CARTESIAN_POINT('Ctrl Pts',(-0.321930825274427,2.11718079129356,
6.84840088056807));
#59467=CARTESIAN_POINT('Ctrl Pts',(-0.322273821431241,2.10861398800965,
6.8489067771116));
#59468=CARTESIAN_POINT('Ctrl Pts',(-0.322275339951301,2.0975438245451,6.8495741530653));
#59469=CARTESIAN_POINT('Ctrl Pts',(-0.322246583978123,2.0950435789177,6.84972577132713));
#59470=CARTESIAN_POINT('Ctrl Pts',(-0.322171516039962,2.09179975378732,
6.84992371478668));
#59471=CARTESIAN_POINT('Ctrl Pts',(-0.322151715013854,2.09105560038719,
6.84996920843145));
#59472=CARTESIAN_POINT('Ctrl Pts',(-0.322116040958226,2.08986948364505,
6.85004185791066));
#59473=CARTESIAN_POINT('Ctrl Pts',(-0.322101836077988,2.08942746972945,
6.8500689614242));
#59474=CARTESIAN_POINT('Ctrl Pts',(-0.322074663913055,2.08863290037682,
6.85011773786434));
#59475=CARTESIAN_POINT('Ctrl Pts',(-0.322062027425214,2.08828033372048,
6.85013940038503));
#59476=CARTESIAN_POINT('Ctrl Pts',(-0.322031109308002,2.08745553505984,
6.85019012369995));
#59477=CARTESIAN_POINT('Ctrl Pts',(-0.322012367856535,2.08698332198871,
6.85021919886788));
#59478=CARTESIAN_POINT('Ctrl Pts',(-0.321955643363727,2.08562925018755,
6.85030267353166));
#59479=CARTESIAN_POINT('Ctrl Pts',(-0.321915076134098,2.08474750916423,
6.85035715393022));
#59480=CARTESIAN_POINT('Ctrl Pts',(-0.321626381809608,2.07898811737928,
6.85071383130632));
#59481=CARTESIAN_POINT('Ctrl Pts',(-0.321271037165977,2.07411670145508,
6.85101937526794));
#59482=CARTESIAN_POINT('Ctrl Pts',(-0.319875621343921,2.05955618433568,
6.85194486541953));
#59483=CARTESIAN_POINT('Ctrl Pts',(-0.318506783384072,2.04990495970286,
6.85257477945267));
#59484=CARTESIAN_POINT('Ctrl Pts',(-0.313632911979409,2.02403595594415,
6.85430675114566));
#59485=CARTESIAN_POINT('Ctrl Pts',(-0.309309905902645,2.00800305556802,
6.85542847676373));
#59486=CARTESIAN_POINT('Ctrl Pts',(-0.29740141106219,1.97439103594679,6.85784107566176));
#59487=CARTESIAN_POINT('Ctrl Pts',(-0.289444329073496,1.95700567954791,
6.85912741669602));
#59488=CARTESIAN_POINT('Ctrl Pts',(-0.279866330954978,1.94019987637498,
6.86034676044441));
#59489=CARTESIAN_POINT('Ctrl Pts',(-0.279737808378602,1.93997499796166,
6.86036307149682));
#59490=CARTESIAN_POINT('Ctrl Pts',(-0.279140736230509,1.93893320675976,
6.86043861149927));
#59491=CARTESIAN_POINT('Ctrl Pts',(-0.278668872009114,1.93811818405514,
6.86049764012618));
#59492=CARTESIAN_POINT('Ctrl Pts',(-0.278014773839143,1.93699973497293,
6.86057853770992));
#59493=CARTESIAN_POINT('Ctrl Pts',(-0.277835608558162,1.93669453318488,
6.86060060199568));
#59494=CARTESIAN_POINT('Ctrl Pts',(-0.277549635772109,1.9362092214014,6.86063566886617));
#59495=CARTESIAN_POINT('Ctrl Pts',(-0.277443155497015,1.93602892041693,
6.86064869273221));
#59496=CARTESIAN_POINT('Ctrl Pts',(-0.277235163384659,1.935677514048,6.86067406816989));
#59497=CARTESIAN_POINT('Ctrl Pts',(-0.277133669126158,1.93550639938528,
6.86068642078655));
#59498=CARTESIAN_POINT('Ctrl Pts',(-0.276887669849256,1.93509252981834,
6.86071628877096));
#59499=CARTESIAN_POINT('Ctrl Pts',(-0.276743003584368,1.9348498701035,6.86073379354769));
#59500=CARTESIAN_POINT('Ctrl Pts',(-0.27629720933969,1.93410433611787,6.86078755246351));
#59501=CARTESIAN_POINT('Ctrl Pts',(-0.275995026260432,1.93360208932785,
6.8608237379404));
#59502=CARTESIAN_POINT('Ctrl Pts',(-0.272680379048862,1.92812681305507,
6.86121791432844));
#59503=CARTESIAN_POINT('Ctrl Pts',(-0.269535001026556,1.92323497202769,
6.86156736514408));
#59504=CARTESIAN_POINT('Ctrl Pts',(-0.262668591950594,1.91316586886582,
6.8622867595852));
#59505=CARTESIAN_POINT('Ctrl Pts',(-0.258922885183182,1.90800851508295,
6.86265530016712));
#59506=CARTESIAN_POINT('Ctrl Pts',(-0.237973409018472,1.88089312125577,
6.8646126627787));
#59507=CARTESIAN_POINT('Ctrl Pts',(-0.218127423927669,1.86112826977649,
6.86612226118976));
#59508=CARTESIAN_POINT('Ctrl Pts',(-0.194072972230402,1.84270124329628,
6.86787988325165));
#59509=CARTESIAN_POINT('Ctrl Pts',(-0.192145979192528,1.84125902712357,
6.86802015094564));
#59510=CARTESIAN_POINT('Ctrl Pts',(-0.188736364265365,1.83876627061052,
6.86826757304807));
#59511=CARTESIAN_POINT('Ctrl Pts',(-0.187260663703092,1.83770642360667,
6.86837441148749));
#59512=CARTESIAN_POINT('Ctrl Pts',(-0.180429728434084,1.832887481177,6.86886799676653));
#59513=CARTESIAN_POINT('Ctrl Pts',(-0.174970057487257,1.82927974889284,
6.86925984125394));
#59514=CARTESIAN_POINT('Ctrl Pts',(-0.16852416354373,1.82529679071907,6.86972099830477));
#59515=CARTESIAN_POINT('Ctrl Pts',(-0.167641066644662,1.82475698079259,
6.8697841451864));
#59516=CARTESIAN_POINT('Ctrl Pts',(-0.166324057272614,1.82396062296709,
6.86987827748827));
#59517=CARTESIAN_POINT('Ctrl Pts',(-0.165892112478669,1.82370082028145,
6.8699091437479));
#59518=CARTESIAN_POINT('Ctrl Pts',(-0.165121942260404,1.82324004155807,
6.86996416806702));
#59519=CARTESIAN_POINT('Ctrl Pts',(-0.164783954231261,1.82303866905584,
6.8699883116039));
#59520=CARTESIAN_POINT('Ctrl Pts',(-0.164071916458155,1.82261620333812,
6.8700391670955));
#59521=CARTESIAN_POINT('Ctrl Pts',(-0.163697786888806,1.8223952468246,6.87006588396085));
#59522=CARTESIAN_POINT('Ctrl Pts',(-0.162711274003919,1.82181531167767,
6.87013632067883));
#59523=CARTESIAN_POINT('Ctrl Pts',(-0.162098152025379,1.82145759999231,
6.87018008638548));
#59524=CARTESIAN_POINT('Ctrl Pts',(-0.159344794585676,1.81986338759023,
6.87037658114278));
#59525=CARTESIAN_POINT('Ctrl Pts',(-0.157191603775599,1.81864953469204,
6.87053012503778));
#59526=CARTESIAN_POINT('Ctrl Pts',(-0.14128666908987,1.80992275937943,6.87166369552062));
#59527=CARTESIAN_POINT('Ctrl Pts',(-0.127019277660994,1.80339807582073,
6.87267880649944));
#59528=CARTESIAN_POINT('Ctrl Pts',(-0.085328135570271,1.78789331312937,
6.87563456593586));
#59529=CARTESIAN_POINT('Ctrl Pts',(-0.0570974322106372,1.78151724541543,
6.87763399856384));
#59530=CARTESIAN_POINT('Ctrl Pts',(-0.0277340098856623,1.77891988188452,
6.8795391927951));
#59531=CARTESIAN_POINT('Ctrl Pts',(-0.0270716332813282,1.77886335581295,
6.87958207315246));
#59532=CARTESIAN_POINT('Ctrl Pts',(-0.0226198282752288,1.77849731805119,
6.87986959953397));
#59533=CARTESIAN_POINT('Ctrl Pts',(-0.0188251486561185,1.77825281966406,
6.88011142264051));
#59534=CARTESIAN_POINT('Ctrl Pts',(-0.0144424466234604,1.77804824335031,
6.88038628197067));
#59535=CARTESIAN_POINT('Ctrl Pts',(-0.0138579835002017,1.77802255641059,
6.8804228453553));
#59536=CARTESIAN_POINT('Ctrl Pts',(-0.0129913996345142,1.77798683435746,
6.88047691980647));
#59537=CARTESIAN_POINT('Ctrl Pts',(-0.0127093345773721,1.77797557836764,
6.88049449885556));
#59538=CARTESIAN_POINT('Ctrl Pts',(-0.0122081325580716,1.77795623711976,
6.88052569613782));
#59539=CARTESIAN_POINT('Ctrl Pts',(-0.011989002192633,1.77794800491513,
6.88053932264051));
#59540=CARTESIAN_POINT('Ctrl Pts',(-0.0115250607254074,1.77793104991664,
6.88056814441545));
#59541=CARTESIAN_POINT('Ctrl Pts',(-0.011280248717201,1.77792238261196,
6.88058333649427));
#59542=CARTESIAN_POINT('Ctrl Pts',(-0.0106262935710699,1.77789997656651,
6.88062387474249));
#59543=CARTESIAN_POINT('Ctrl Pts',(-0.0102171320334495,1.77788673819862,
6.88064919275271));
#59544=CARTESIAN_POINT('Ctrl Pts',(-0.00829096335637178,1.77782809105331,
6.8807681696053));
#59545=CARTESIAN_POINT('Ctrl Pts',(-0.00677364064662362,1.77779261803498,
6.88086127890078));
#59546=CARTESIAN_POINT('Ctrl Pts',(0.00552489325638143,1.77759201051274,
6.8816114035902));
#59547=CARTESIAN_POINT('Ctrl Pts',(0.0163091749536936,1.77795730168867,
6.88224082061855));
#59548=CARTESIAN_POINT('Ctrl Pts',(0.0589632798324055,1.78155092872221,
6.88468784954465));
#59549=CARTESIAN_POINT('Ctrl Pts',(0.0902907587631205,1.78897876182508,
6.88640991858218));
#59550=CARTESIAN_POINT('Ctrl Pts',(0.121136138778605,1.80135525637921,6.8883696450711));
#59551=CARTESIAN_POINT('Ctrl Pts',(0.122259334126513,1.80181330986426,6.88844135895844));
#59552=CARTESIAN_POINT('Ctrl Pts',(0.128646470044153,1.80446022009727,6.88885123935213));
#59553=CARTESIAN_POINT('Ctrl Pts',(0.133853921971374,1.80678199723371,6.88919349808833));
#59554=CARTESIAN_POINT('Ctrl Pts',(0.139881487167089,1.80966345967125,6.88960023588085));
#59555=CARTESIAN_POINT('Ctrl Pts',(0.140764205308178,1.81009040103376,6.88966007096946));
#59556=CARTESIAN_POINT('Ctrl Pts',(0.142093904676987,1.81074103696969,6.88975061768401));
#59557=CARTESIAN_POINT('Ctrl Pts',(0.142542341989202,1.810961756552,6.88978122553538));
#59558=CARTESIAN_POINT('Ctrl Pts',(0.143342395495558,1.81135785534634,6.88983596087808));
#59559=CARTESIAN_POINT('Ctrl Pts',(0.14369420857446,1.8115328364672,6.88986007441029));
#59560=CARTESIAN_POINT('Ctrl Pts',(0.144436477512356,1.81190371328301,6.88991104429282));
#59561=CARTESIAN_POINT('Ctrl Pts',(0.14482685654768,1.81209976020187,6.88993790590811));
#59562=CARTESIAN_POINT('Ctrl Pts',(0.145847000538548,1.8126146727144,6.89000824625368));
#59563=CARTESIAN_POINT('Ctrl Pts',(0.14647611605023,1.81293481346686,6.8900517697257));
#59564=CARTESIAN_POINT('Ctrl Pts',(0.149285543638173,1.81437609900589,6.89024678613384));
#59565=CARTESIAN_POINT('Ctrl Pts',(0.151454025335213,1.81552001118883,6.89039908039086));
#59566=CARTESIAN_POINT('Ctrl Pts',(0.167273529946703,1.824097219141,6.89152341526636));
#59567=CARTESIAN_POINT('Ctrl Pts',(0.18038189828198,1.8324836042563,6.89252996350282));
#59568=CARTESIAN_POINT('Ctrl Pts',(0.212522953705439,1.85648594887202,6.89519450315251));
#59569=CARTESIAN_POINT('Ctrl Pts',(0.230465225751054,1.87339290239737,6.89688705799964));
#59570=CARTESIAN_POINT('Ctrl Pts',(0.251873065757921,1.89876503393261,6.89908019706598));
#59571=CARTESIAN_POINT('Ctrl Pts',(0.257168373819225,1.90557774958595,6.8996397013343));
#59572=CARTESIAN_POINT('Ctrl Pts',(0.262596811378652,1.91317229024472,6.90022548506959));
#59573=CARTESIAN_POINT('Ctrl Pts',(0.263007268821166,1.91375055691784,6.90026985767464));
#59574=CARTESIAN_POINT('Ctrl Pts',(0.263578714845979,1.91456128599946,6.90033174106603));
#59575=CARTESIAN_POINT('Ctrl Pts',(0.263741307412986,1.91479260723279,6.90034936086878));
#59576=CARTESIAN_POINT('Ctrl Pts',(0.264021968994568,1.9151930248978,6.90037979631037));
#59577=CARTESIAN_POINT('Ctrl Pts',(0.264140180146376,1.91536202072439,6.90039262173551));
#59578=CARTESIAN_POINT('Ctrl Pts',(0.264385899180326,1.91571402199706,6.90041929437713));
#59579=CARTESIAN_POINT('Ctrl Pts',(0.264513379156064,1.91589704613556,6.90043313960832));
#59580=CARTESIAN_POINT('Ctrl Pts',(0.264815812444016,1.91633221488298,6.90046600387927));
#59581=CARTESIAN_POINT('Ctrl Pts',(0.264990596386728,1.91658447819595,6.90048501124917));
#59582=CARTESIAN_POINT('Ctrl Pts',(0.26554081044429,1.91738102288873,6.90054489222762));
#59583=CARTESIAN_POINT('Ctrl Pts',(0.265914929071084,1.91792621460541,6.90058567679077));
#59584=CARTESIAN_POINT('Ctrl Pts',(0.270630306686199,1.92484332589904,6.90110064693492));
#59585=CARTESIAN_POINT('Ctrl Pts',(0.274743640307383,1.93136851370839,6.90155983601539));
#59586=CARTESIAN_POINT('Ctrl Pts',(0.282395221631989,1.94453114631521,6.90244773380957));
#59587=CARTESIAN_POINT('Ctrl Pts',(0.2859430615527,1.95115711960808,6.90287665316356));
#59588=CARTESIAN_POINT('Ctrl Pts',(0.299347135989773,1.97844247609117,6.90459463499572));
#59589=CARTESIAN_POINT('Ctrl Pts',(0.307221120035105,1.99999935510897,6.90584813836431));
#59590=CARTESIAN_POINT('Ctrl Pts',(0.313940419517456,2.0270130230886,6.90745168833202));
#59591=CARTESIAN_POINT('Ctrl Pts',(0.315024538895809,2.03184413135056,6.90773943658765));
#59592=CARTESIAN_POINT('Ctrl Pts',(0.317482117308508,2.0441121309603,6.90847467088267));
#59593=CARTESIAN_POINT('Ctrl Pts',(0.318705837155645,2.05157558416667,6.90892617765654));
#59594=CARTESIAN_POINT('Ctrl Pts',(0.319789255054213,2.06003812682986,6.9094452538242));
#59595=CARTESIAN_POINT('Ctrl Pts',(0.319908236213122,2.06100205997668,6.90950448202995));
#59596=CARTESIAN_POINT('Ctrl Pts',(0.320081671634351,2.06246138690652,6.90959430920316));
#59597=CARTESIAN_POINT('Ctrl Pts',(0.320139337840275,2.06295639931097,6.90962480691013));
#59598=CARTESIAN_POINT('Ctrl Pts',(0.320237610987965,2.06381735639922,6.90967789950418));
#59599=CARTESIAN_POINT('Ctrl Pts',(0.320278739543545,2.06418324157894,6.90970047791583));
#59600=CARTESIAN_POINT('Ctrl Pts',(0.320363198621967,2.06494637990663,6.90974760284944));
#59601=CARTESIAN_POINT('Ctrl Pts',(0.320406417445705,2.06534364458988,6.90977215285043));
#59602=CARTESIAN_POINT('Ctrl Pts',(0.320506776338543,2.06628237264813,6.90983020770833));
#59603=CARTESIAN_POINT('Ctrl Pts',(0.320563283199028,2.06682390119348,6.90986373244416));
#59604=CARTESIAN_POINT('Ctrl Pts',(0.320741504644544,2.0685748456329,6.90997224178341));
#59605=CARTESIAN_POINT('Ctrl Pts',(0.320857748162699,2.06978479674563,6.91004739829891));
#59606=CARTESIAN_POINT('Ctrl Pts',(0.321114770830753,2.07262902584098,6.91022448740044));
#59607=CARTESIAN_POINT('Ctrl Pts',(0.321249922033687,2.0742637666848,6.91032659521263));
#59608=CARTESIAN_POINT('Ctrl Pts',(0.322558293768807,2.09171045168674,6.9114199002776));
#59609=CARTESIAN_POINT('Ctrl Pts',(0.322575423068484,2.10758494703581,6.91244755852085));
#59610=CARTESIAN_POINT('Ctrl Pts',(0.320082331425727,2.14183866310184,6.91473105829981));
#59611=CARTESIAN_POINT('Ctrl Pts',(0.317154786697315,2.16013276498108,6.91599282916249));
#59612=CARTESIAN_POINT('Ctrl Pts',(0.30926222505182,2.19174159439278,6.91818319896648));
#59613=CARTESIAN_POINT('Ctrl Pts',(0.304956284510689,2.20517325489084,6.9191164632231));
#59614=CARTESIAN_POINT('Ctrl Pts',(0.29945626199369,2.21911306402177,6.92005873773542));
#59615=CARTESIAN_POINT('Ctrl Pts',(0.299124680872261,2.21994332080568,6.92011475550323));
#59616=CARTESIAN_POINT('Ctrl Pts',(0.29867282324115,2.22106121368575,6.92019002890422));
#59617=CARTESIAN_POINT('Ctrl Pts',(0.298555582100099,2.22135006057178,6.92020946476912));
#59618=CARTESIAN_POINT('Ctrl Pts',(0.298357111768316,2.22183700308775,6.92024220643058));
#59619=CARTESIAN_POINT('Ctrl Pts',(0.298276104263787,2.22203518791711,6.92025552562627));
#59620=CARTESIAN_POINT('Ctrl Pts',(0.298120056766718,2.22241587444413,6.92028109710688));
#59621=CARTESIAN_POINT('Ctrl Pts',(0.298045047213376,2.22259838658941,6.92029335107687));
#59622=CARTESIAN_POINT('Ctrl Pts',(0.297866654957414,2.22303131668672,6.92032240476938));
#59623=CARTESIAN_POINT('Ctrl Pts',(0.297763124195144,2.22328167297707,6.92033919535156));
#59624=CARTESIAN_POINT('Ctrl Pts',(0.297460611141861,2.22401060062407,6.92038805184601));
#59625=CARTESIAN_POINT('Ctrl Pts',(0.297260788745861,2.22448882572775,6.92042006685903));
#59626=CARTESIAN_POINT('Ctrl Pts',(0.296019576436037,2.22743932915773,6.92061736656948));
#59627=CARTESIAN_POINT('Ctrl Pts',(0.294948465540441,2.22989909949198,6.92078088197342));
#59628=CARTESIAN_POINT('Ctrl Pts',(0.291478915804195,2.2376025524802,6.92129078241875));
#59629=CARTESIAN_POINT('Ctrl Pts',(0.288970291683267,2.24279565801502,6.92163129037745));
#59630=CARTESIAN_POINT('Ctrl Pts',(0.276234500829984,2.26744804906988,6.9232450976797));
#59631=CARTESIAN_POINT('Ctrl Pts',(0.264173269128736,2.28589509884087,6.92444808012059));
#59632=CARTESIAN_POINT('Ctrl Pts',(0.237678598725944,2.31857124291158,6.92681640327721));
#59633=CARTESIAN_POINT('Ctrl Pts',(0.223601777943976,2.33295185625463,6.92797111173281));
#59634=CARTESIAN_POINT('Ctrl Pts',(0.207290181620077,2.34676636359385,6.92926939203645));
#59635=CARTESIAN_POINT('Ctrl Pts',(0.206295471013514,2.34759853828308,6.92934840367674));
#59636=CARTESIAN_POINT('Ctrl Pts',(0.204901541170681,2.34875046856641,6.92945891545481));
#59637=CARTESIAN_POINT('Ctrl Pts',(0.204506533438807,2.34907531985769,6.92949020858004));
#59638=CARTESIAN_POINT('Ctrl Pts',(0.203823218801629,2.34963455120821,6.92954430232737));
#59639=CARTESIAN_POINT('Ctrl Pts',(0.203535275908072,2.34986937615228,6.92956708491375));
#59640=CARTESIAN_POINT('Ctrl Pts',(0.202938582970869,2.3503542790381,6.92961427182778));
#59641=CARTESIAN_POINT('Ctrl Pts',(0.202629775377135,2.35060428491811,6.92963867900566));
#59642=CARTESIAN_POINT('Ctrl Pts',(0.201907179833363,2.35118707834066,6.92969575951856));
#59643=CARTESIAN_POINT('Ctrl Pts',(0.201493031062161,2.35151941480049,6.92972845088862));
#59644=CARTESIAN_POINT('Ctrl Pts',(0.200189704809308,2.35255999279017,6.92983125748689));
#59645=CARTESIAN_POINT('Ctrl Pts',(0.199297607590355,2.3532645482998,6.9299015197753));
#59646=CARTESIAN_POINT('Ctrl Pts',(0.192490649627179,2.35858227387704,6.93043686572223));
#59647=CARTESIAN_POINT('Ctrl Pts',(0.186420506963353,2.3629920568123,6.93090992055428));
#59648=CARTESIAN_POINT('Ctrl Pts',(0.174726979381646,2.37087871208087,6.93181432129725));
#59649=CARTESIAN_POINT('Ctrl Pts',(0.169139604457566,2.37440222082553,6.93224367080748));
#59650=CARTESIAN_POINT('Ctrl Pts',(0.14931448806461,2.38606869595261,6.93375664156678));
#59651=CARTESIAN_POINT('Ctrl Pts',(0.134567556897141,2.39329440062634,6.93486542684595));
#59652=CARTESIAN_POINT('Ctrl Pts',(0.101268433777865,2.40656842744533,6.9372909766152));
#59653=CARTESIAN_POINT('Ctrl Pts',(0.0825832733741295,2.41212127601144,
6.93860343936805));
#59654=CARTESIAN_POINT('Ctrl Pts',(0.062460643711344,2.41616607650144,6.93989636197436));
#59655=CARTESIAN_POINT('Ctrl Pts',(0.0614108320279248,2.41637166391644,
6.93996346946841));
#59656=CARTESIAN_POINT('Ctrl Pts',(0.0599935040764152,2.41664190230448,
6.94005358673988));
#59657=CARTESIAN_POINT('Ctrl Pts',(0.0596268861248823,2.41671114486353,
6.94007685370341));
#59658=CARTESIAN_POINT('Ctrl Pts',(0.0590505768257732,2.41681895533253,
6.94011335920189));
#59659=CARTESIAN_POINT('Ctrl Pts',(0.0588409675050555,2.41685795180989,
6.94012662221829));
#59660=CARTESIAN_POINT('Ctrl Pts',(0.0584370502230526,2.41693268341788,
6.94015215213424));
#59661=CARTESIAN_POINT('Ctrl Pts',(0.0582427495707399,2.41696844760936,
6.94016442059113));
#59662=CARTESIAN_POINT('Ctrl Pts',(0.0577800154651128,2.41705318148768,
6.94019360883034));
#59663=CARTESIAN_POINT('Ctrl Pts',(0.0575115528697855,2.41710198890331,
6.94021051922052));
#59664=CARTESIAN_POINT('Ctrl Pts',(0.0569543651722057,2.41720255666255,
6.94024556790815));
#59665=CARTESIAN_POINT('Ctrl Pts',(0.0566656305711251,2.41725426392566,
6.94026370317271));
#59666=CARTESIAN_POINT('Ctrl Pts',(0.0550166961769833,2.41754723603684,
6.94036712002625));
#59667=CARTESIAN_POINT('Ctrl Pts',(0.0536549994686444,2.41778015225312,
6.94045193243892));
#59668=CARTESIAN_POINT('Ctrl Pts',(0.0428446834331676,2.41955777307926,
6.94112087597888));
#59669=CARTESIAN_POINT('Ctrl Pts',(0.0333319879555434,2.42068965443206,
6.94168312635542));
#59670=CARTESIAN_POINT('Ctrl Pts',(0.00709862688728745,2.42263082072342,
6.94319573480625));
#59671=CARTESIAN_POINT('Ctrl Pts',(-0.00965646364775639,2.42256448958444,
6.94412089556285));
#59672=CARTESIAN_POINT('Ctrl Pts',(-0.0331721590932399,2.42063670125974,
6.94544289408972));
#59673=CARTESIAN_POINT('Ctrl Pts',(-0.0399931148771294,2.4198575197543,
6.9458290004088));
#59674=CARTESIAN_POINT('Ctrl Pts',(-0.0516428523980954,2.41814825121427,
6.94649833002995));
#59675=CARTESIAN_POINT('Ctrl Pts',(-0.0564848021687353,2.41732437422424,
6.94677947390256));
#59676=CARTESIAN_POINT('Ctrl Pts',(-0.0725254988566162,2.41421622027278,
6.947723872382));
#59677=CARTESIAN_POINT('Ctrl Pts',(-0.0836203602850281,2.41144722106272,
6.9483987061421));
#59678=CARTESIAN_POINT('Ctrl Pts',(-0.0956921648825162,2.40774279492059,
6.94916630417527));
#59679=CARTESIAN_POINT('Ctrl Pts',(-0.0968384180018671,2.40738402525708,
6.94923952370293));
#59680=CARTESIAN_POINT('Ctrl Pts',(-0.0984419545824516,2.4068722693139,
6.94934243072406));
#59681=CARTESIAN_POINT('Ctrl Pts',(-0.0989009508320979,2.40672464853088,
6.94937194182115));
#59682=CARTESIAN_POINT('Ctrl Pts',(-0.0997407191295573,2.40645248419772,
6.94942603605397));
#59683=CARTESIAN_POINT('Ctrl Pts',(-0.100121594124359,2.4063282594067,6.94945060865386));
#59684=CARTESIAN_POINT('Ctrl Pts',(-0.100891324790674,2.40607561795556,
6.94950034661922));
#59685=CARTESIAN_POINT('Ctrl Pts',(-0.101280169238756,2.40594716969013,
6.94952551298922));
#59686=CARTESIAN_POINT('Ctrl Pts',(-0.102058141513457,2.40568853387949,
6.94957594516013));
#59687=CARTESIAN_POINT('Ctrl Pts',(-0.102447267617827,2.40555834361007,
6.94960121101185));
#59688=CARTESIAN_POINT('Ctrl Pts',(-0.103374142362199,2.40524626872766,
6.94966149027512));
#59689=CARTESIAN_POINT('Ctrl Pts',(-0.103911659801901,2.40506370618593,
6.94969652608011));
#59690=CARTESIAN_POINT('Ctrl Pts',(-0.107521907810104,2.40382687198106,
6.94993237568279));
#59691=CARTESIAN_POINT('Ctrl Pts',(-0.110578936456974,2.40272764387393,
6.95013467575528));
#59692=CARTESIAN_POINT('Ctrl Pts',(-0.119015080409722,2.39954939487083,
6.95070037825136));
#59693=CARTESIAN_POINT('Ctrl Pts',(-0.124355584241294,2.39737200805112,
6.95106701001202));
#59694=CARTESIAN_POINT('Ctrl Pts',(-0.139427699016517,2.39074991268826,
6.95212669889253));
#59695=CARTESIAN_POINT('Ctrl Pts',(-0.148999692873216,2.38596267197528,
6.9528303803244));
#59696=CARTESIAN_POINT('Ctrl Pts',(-0.165942334182022,2.37640729519951,
6.9541288497474));
#59697=CARTESIAN_POINT('Ctrl Pts',(-0.173390669436343,2.3717968304015,6.9547196486308));
#59698=CARTESIAN_POINT('Ctrl Pts',(-0.198777682056132,2.35461382338246,
6.95679344974949));
#59699=CARTESIAN_POINT('Ctrl Pts',(-0.215617196123676,2.34052069462305,
6.95828286081767));
#59700=CARTESIAN_POINT('Ctrl Pts',(-0.231745221586659,2.32395714283031,
6.95974119456232));
#59701=CARTESIAN_POINT('Ctrl Pts',(-0.232587269943504,2.32308252178152,
6.95981742489979));
#59702=CARTESIAN_POINT('Ctrl Pts',(-0.23369509726322,2.32191874935333,6.95991781068218));
#59703=CARTESIAN_POINT('Ctrl Pts',(-0.23396530485812,2.32163385555001,6.95994230306239));
#59704=CARTESIAN_POINT('Ctrl Pts',(-0.234384129806912,2.32119064733504,
6.95998027720748));
#59705=CARTESIAN_POINT('Ctrl Pts',(-0.234533107797189,2.32103267659218,
6.95999378689288));
#59706=CARTESIAN_POINT('Ctrl Pts',(-0.234816737187704,2.32073131688219,
6.96001951089539));
#59707=CARTESIAN_POINT('Ctrl Pts',(-0.234951416065557,2.3205879561652,6.96003172731854));
#59708=CARTESIAN_POINT('Ctrl Pts',(-0.23526724784478,2.32025114745237,6.96006037960331));
#59709=CARTESIAN_POINT('Ctrl Pts',(-0.2354482931548,2.32005759953758,6.96007680708775));
#59710=CARTESIAN_POINT('Ctrl Pts',(-0.235821767381931,2.31965734544828,
6.96011070180902));
#59711=CARTESIAN_POINT('Ctrl Pts',(-0.236014163853594,2.31945060911844,
6.96012816655049));
#59712=CARTESIAN_POINT('Ctrl Pts',(-0.236510062692875,2.31891634305834,
6.96017319221157));
#59713=CARTESIAN_POINT('Ctrl Pts',(-0.236813157803925,2.31858843361338,
6.96020072230402));
#59714=CARTESIAN_POINT('Ctrl Pts',(-0.240470518039745,2.31461511055141,
6.96053305964955));
#59715=CARTESIAN_POINT('Ctrl Pts',(-0.243741205637736,2.31089321219542,
6.96083168738644));
#59716=CARTESIAN_POINT('Ctrl Pts',(-0.254233219154438,2.29838342891621,
6.96180022949518));
#59717=CARTESIAN_POINT('Ctrl Pts',(-0.261075748884775,2.28928817513233,
6.96244940082143));
#59718=CARTESIAN_POINT('Ctrl Pts',(-0.269950742157918,2.27609168038358,
6.96334567196271));
#59719=CARTESIAN_POINT('Ctrl Pts',(-0.272398480622213,2.27228102566769,
6.96359947493373));
#59720=CARTESIAN_POINT('Ctrl Pts',(-0.277286795834698,2.26430609135024,
6.96412281761958));
#59721=CARTESIAN_POINT('Ctrl Pts',(-0.279715754307783,2.26013605352149,
6.96439223218429));
#59722=CARTESIAN_POINT('Ctrl Pts',(-0.293866292507904,2.23453741633889,
6.9660285358304));
#59723=CARTESIAN_POINT('Ctrl Pts',(-0.303212357072985,2.21189160382883,
6.96741091003816));
#59724=CARTESIAN_POINT('Ctrl Pts',(-0.310307931684961,2.18701870239421,
6.96898029825098));
#59725=CARTESIAN_POINT('Ctrl Pts',(-0.31069528767595,2.18562537674433,6.96906834488947));
#59726=CARTESIAN_POINT('Ctrl Pts',(-0.311213277066018,2.18371235784494,
6.96918942906307));
#59727=CARTESIAN_POINT('Ctrl Pts',(-0.311352015812389,2.18319486115274,
6.96922220362307));
#59728=CARTESIAN_POINT('Ctrl Pts',(-0.31158645398836,2.18231160461384,6.96927817728737));
#59729=CARTESIAN_POINT('Ctrl Pts',(-0.311682801746273,2.181946016723,6.9693013553528));
#59730=CARTESIAN_POINT('Ctrl Pts',(-0.311868319561988,2.18123701596273,
6.96934632542909));
#59731=CARTESIAN_POINT('Ctrl Pts',(-0.311957566309265,2.18089362354218,
6.96936811492308));
#59732=CARTESIAN_POINT('Ctrl Pts',(-0.312168638996795,2.18007594049113,
6.96942002163478));
#59733=CARTESIAN_POINT('Ctrl Pts',(-0.312289951087387,2.17960151923348,
6.96945015541383));
#59734=CARTESIAN_POINT('Ctrl Pts',(-0.31253896927483,2.17861834043678,6.96951264066866));
#59735=CARTESIAN_POINT('Ctrl Pts',(-0.312666515419028,2.17810954422419,
6.96954499721795));
#59736=CARTESIAN_POINT('Ctrl Pts',(-0.312995530133078,2.17678334764678,
6.96962938984752));
#59737=CARTESIAN_POINT('Ctrl Pts',(-0.313195038014143,2.1759654691349,6.96968148904755));
#59738=CARTESIAN_POINT('Ctrl Pts',(-0.319317992010291,2.1504303815822,6.97130979865669));
#59739=CARTESIAN_POINT('Ctrl Pts',(-0.322298355976539,2.12510622756114,
6.97298570556493));
#59740=CARTESIAN_POINT('Ctrl Pts',(-0.322274862187325,2.09970196117587,
6.97470119138623));
#59741=CARTESIAN_POINT('',(-0.3219654526091,2.10024677492677,7.22472265507269));
#59742=CARTESIAN_POINT('Ctrl Pts',(-0.322274862242446,2.09970202078479,
6.97470118736099));
#59743=CARTESIAN_POINT('Ctrl Pts',(-0.322254792744558,2.07799616233327,
6.97616692902254));
#59744=CARTESIAN_POINT('Ctrl Pts',(-0.320041910222358,2.05634574280106,
6.97765048953118));
#59745=CARTESIAN_POINT('Ctrl Pts',(-0.314997195943813,2.03181606877893,
6.97925888435003));
#59746=CARTESIAN_POINT('Ctrl Pts',(-0.31427524269446,2.02856222364379,6.9794706346778));
#59747=CARTESIAN_POINT('Ctrl Pts',(-0.313397127533594,2.02487593948198,
6.97970824887217));
#59748=CARTESIAN_POINT('Ctrl Pts',(-0.313290400305139,2.02443208949767,
6.97973682125599));
#59749=CARTESIAN_POINT('Ctrl Pts',(-0.313091214045297,2.02361140226623,
6.97978958036946));
#59750=CARTESIAN_POINT('Ctrl Pts',(-0.312999017050846,2.0232345031602,6.97981378185102));
#59751=CARTESIAN_POINT('Ctrl Pts',(-0.312848648111069,2.02262457311482,
6.97985290027779));
#59752=CARTESIAN_POINT('Ctrl Pts',(-0.312790896299247,2.02239144052486,
6.97986784145167));
#59753=CARTESIAN_POINT('Ctrl Pts',(-0.312679612762009,2.02194435299197,
6.97989647332939));
#59754=CARTESIAN_POINT('Ctrl Pts',(-0.3126261221968,2.02173038912028,6.97991016631736));
#59755=CARTESIAN_POINT('Ctrl Pts',(-0.312502571952335,2.02123833170854,
6.97994163491793));
#59756=CARTESIAN_POINT('Ctrl Pts',(-0.31243236048083,2.0209602758432,6.97995940169246));
#59757=CARTESIAN_POINT('Ctrl Pts',(-0.312213660337644,2.02009901062124,
6.98001438565315));
#59758=CARTESIAN_POINT('Ctrl Pts',(-0.31206390805354,2.01951611894747,6.98005153002816));
#59759=CARTESIAN_POINT('Ctrl Pts',(-0.31081035419789,2.01469292018172,6.98035834787495));
#59760=CARTESIAN_POINT('Ctrl Pts',(-0.309621749147266,2.01047485702557,
6.98062323055529));
#59761=CARTESIAN_POINT('Ctrl Pts',(-0.302498597866835,1.98703850955839,
6.98208238234991));
#59762=CARTESIAN_POINT('Ctrl Pts',(-0.294860426573917,1.9683822720351,6.98319811786653));
#59763=CARTESIAN_POINT('Ctrl Pts',(-0.283385561392874,1.94645776178699,
6.98458152913997));
#59764=CARTESIAN_POINT('Ctrl Pts',(-0.281151386680398,1.94240402142001,
6.98484045433555));
#59765=CARTESIAN_POINT('Ctrl Pts',(-0.276632149757246,1.93460636838058,
6.98534674806971));
#59766=CARTESIAN_POINT('Ctrl Pts',(-0.274356444052104,1.93085822492165,
6.98559395237056));
#59767=CARTESIAN_POINT('Ctrl Pts',(-0.265021826999951,1.916168168351,6.98658141772468));
#59768=CARTESIAN_POINT('Ctrl Pts',(-0.257379771736471,1.90561298929361,
6.98733341773803));
#59769=CARTESIAN_POINT('Ctrl Pts',(-0.246245651698839,1.89204616962227,
6.98838041746954));
#59770=CARTESIAN_POINT('Ctrl Pts',(-0.243296964569347,1.88860392525328,
6.98865357757056));
#59771=CARTESIAN_POINT('Ctrl Pts',(-0.239863908470939,1.8847632353686,6.98896750425641));
#59772=CARTESIAN_POINT('Ctrl Pts',(-0.239449707636792,1.88430253376502,
6.98900531366845));
#59773=CARTESIAN_POINT('Ctrl Pts',(-0.238744922490738,1.8835231568928,6.98906953814448));
#59774=CARTESIAN_POINT('Ctrl Pts',(-0.238455021080262,1.88320386411302,
6.98909592438253));
#59775=CARTESIAN_POINT('Ctrl Pts',(-0.237879247311214,1.88257226814362,
6.98914826857364));
#59776=CARTESIAN_POINT('Ctrl Pts',(-0.237593398657462,1.88225994444465,
6.98917422549375));
#59777=CARTESIAN_POINT('Ctrl Pts',(-0.237038388916846,1.88165592442344,
6.98922456671188));
#59778=CARTESIAN_POINT('Ctrl Pts',(-0.236769302659316,1.88136416013001,
6.98924894779716));
#59779=CARTESIAN_POINT('Ctrl Pts',(-0.236146874516471,1.88069177168446,
6.98930528483119));
#59780=CARTESIAN_POINT('Ctrl Pts',(-0.23579315087413,1.88031150383642,6.98933725708172));
#59781=CARTESIAN_POINT('Ctrl Pts',(-0.234657732686394,1.87909678255724,
6.98943974608736));
#59782=CARTESIAN_POINT('Ctrl Pts',(-0.233872522470797,1.8782656405398,6.98951041389108));
#59783=CARTESIAN_POINT('Ctrl Pts',(-0.226611118696692,1.87066095286541,
6.99016205137652));
#59784=CARTESIAN_POINT('Ctrl Pts',(-0.219847387035011,1.86416935179256,
6.99075558471187));
#59785=CARTESIAN_POINT('Ctrl Pts',(-0.202537593674635,1.84894851597665,
6.99224502900062));
#59786=CARTESIAN_POINT('Ctrl Pts',(-0.191700482554144,1.84057914690088,
6.99315340432819));
#59787=CARTESIAN_POINT('Ctrl Pts',(-0.17348095558115,1.82827486697669,6.9946330472514));
#59788=CARTESIAN_POINT('Ctrl Pts',(-0.16641926340663,1.82389347177389,6.99519588975997));
#59789=CARTESIAN_POINT('Ctrl Pts',(-0.152166532422991,1.81579604058651,
6.99630466136703));
#59790=CARTESIAN_POINT('Ctrl Pts',(-0.144988726235248,1.81206802614663,
6.9968502549413));
#59791=CARTESIAN_POINT('Ctrl Pts',(-0.130487550700357,1.80521631336783,
6.99791911633876));
#59792=CARTESIAN_POINT('Ctrl Pts',(-0.12317308996342,1.80208586322981,6.99844224554016));
#59793=CARTESIAN_POINT('Ctrl Pts',(-0.113671559665417,1.79842926089034,
6.99909529680369));
#59794=CARTESIAN_POINT('Ctrl Pts',(-0.111585065740821,1.79765101638616,
6.99923710103793));
#59795=CARTESIAN_POINT('Ctrl Pts',(-0.108218436434433,1.79643489125952,
6.99946315122764));
#59796=CARTESIAN_POINT('Ctrl Pts',(-0.106943357078685,1.79598334953672,
6.99954813544767));
#59797=CARTESIAN_POINT('Ctrl Pts',(-0.105389961834506,1.79544423071917,
6.99965087243873));
#59798=CARTESIAN_POINT('Ctrl Pts',(-0.105114346584899,1.79534899507577,
6.99966907041602));
#59799=CARTESIAN_POINT('Ctrl Pts',(-0.104581751369334,1.79516577179543,
6.99970417672085));
#59800=CARTESIAN_POINT('Ctrl Pts',(-0.10432478882804,1.79507773475549,6.99972108795617));
#59801=CARTESIAN_POINT('Ctrl Pts',(-0.103861152295083,1.79491954453971,
6.99975155250005));
#59802=CARTESIAN_POINT('Ctrl Pts',(-0.103654518868025,1.79484927662042,
6.99976511261138));
#59803=CARTESIAN_POINT('Ctrl Pts',(-0.103240246777219,1.79470886828655,
6.99979226405422));
#59804=CARTESIAN_POINT('Ctrl Pts',(-0.10303260887135,1.79463873007968,6.99980585523009));
#59805=CARTESIAN_POINT('Ctrl Pts',(-0.102443256551049,1.79444032175268,
6.99984438292737));
#59806=CARTESIAN_POINT('Ctrl Pts',(-0.102061371327203,1.79431255460784,
6.99986928957191));
#59807=CARTESIAN_POINT('Ctrl Pts',(-0.100451880764203,1.7937774204431,6.9999740194041));
#59808=CARTESIAN_POINT('Ctrl Pts',(-0.099222046459794,1.79337672265726,
7.00005345373485));
#59809=CARTESIAN_POINT('Ctrl Pts',(-0.0772259307896723,1.78635627036069,
7.00146419388377));
#59810=CARTESIAN_POINT('Ctrl Pts',(-0.0558396019943225,1.78185146262231,
7.00267957198056));
#59811=CARTESIAN_POINT('Ctrl Pts',(-0.0175874211049619,1.77777398462785,
7.00482988239314));
#59812=CARTESIAN_POINT('Ctrl Pts',(-0.000904172467797171,1.77729571242723,
7.00576005327469));
#59813=CARTESIAN_POINT('Ctrl Pts',(0.0269410660454354,1.77865732786812,
7.00737321285849));
#59814=CARTESIAN_POINT('Ctrl Pts',(0.0381045312832558,1.77978923199218,
7.00803602404254));
#59815=CARTESIAN_POINT('Ctrl Pts',(0.0503120790039915,1.78167442793353,
7.0087871611806));
#59816=CARTESIAN_POINT('Ctrl Pts',(0.0514377380760737,1.78185438212276,
7.0088566684155));
#59817=CARTESIAN_POINT('Ctrl Pts',(0.0530860746424093,1.78212687118067,
7.00895881689084));
#59818=CARTESIAN_POINT('Ctrl Pts',(0.0536095246281474,1.78221473254704,
7.00899130974107));
#59819=CARTESIAN_POINT('Ctrl Pts',(0.0545243936914246,1.78237061856081,
7.0090481955905));
#59820=CARTESIAN_POINT('Ctrl Pts',(0.0549159095393933,1.78243807479794,
7.00907257048062));
#59821=CARTESIAN_POINT('Ctrl Pts',(0.0556734053631594,1.78257003030272,
7.00911979035278));
#59822=CARTESIAN_POINT('Ctrl Pts',(0.0560394006742645,1.78263443901863,
7.00914263242039));
#59823=CARTESIAN_POINT('Ctrl Pts',(0.0569090578074398,1.78278903459385,
7.00919697321516));
#59824=CARTESIAN_POINT('Ctrl Pts',(0.0574126167115783,1.78287978797948,
7.00922848993396));
#59825=CARTESIAN_POINT('Ctrl Pts',(0.0591931611535906,1.78320506476013,
7.00934011486137));
#59826=CARTESIAN_POINT('Ctrl Pts',(0.0604689303352418,1.78344610299987,
7.00942043036366));
#59827=CARTESIAN_POINT('Ctrl Pts',(0.0818068747996287,1.78761129851937,
7.01076947578114));
#59828=CARTESIAN_POINT('Ctrl Pts',(0.101448431137458,1.79342701559916,7.0121007371681));
#59829=CARTESIAN_POINT('Ctrl Pts',(0.135864813987744,1.8072889776216,7.01458661498581));
#59830=CARTESIAN_POINT('Ctrl Pts',(0.150818733051426,1.81470597713951,7.01572364862022));
#59831=CARTESIAN_POINT('Ctrl Pts',(0.171358997214046,1.82696180547616,7.01732719211138));
#59832=CARTESIAN_POINT('Ctrl Pts',(0.177459528211848,1.83088684558264,7.01780892246554));
#59833=CARTESIAN_POINT('Ctrl Pts',(0.186804858036504,1.8373556779254,7.01855002469984));
#59834=CARTESIAN_POINT('Ctrl Pts',(0.190142007627846,1.83976142603937,7.0188153163938));
#59835=CARTESIAN_POINT('Ctrl Pts',(0.194557739821838,1.84307502810489,7.01916626420745));
#59836=CARTESIAN_POINT('Ctrl Pts',(0.195677609977771,1.84392690803876,7.01925525969968));
#59837=CARTESIAN_POINT('Ctrl Pts',(0.197542998685717,1.84536528339368,7.01940343737787));
#59838=CARTESIAN_POINT('Ctrl Pts',(0.198291559967675,1.84594777597882,7.01946288214594));
#59839=CARTESIAN_POINT('Ctrl Pts',(0.19931025359011,1.84674771735716,7.01954374213382));
#59840=CARTESIAN_POINT('Ctrl Pts',(0.199582613126948,1.84696230243286,7.01956535739938));
#59841=CARTESIAN_POINT('Ctrl Pts',(0.200035895414153,1.84732061904196,7.01960132448628));
#59842=CARTESIAN_POINT('Ctrl Pts',(0.200217010015924,1.84746410568679,7.01961569378468));
#59843=CARTESIAN_POINT('Ctrl Pts',(0.200572208129372,1.84774613095406,7.01964387074479));
#59844=CARTESIAN_POINT('Ctrl Pts',(0.200746302468499,1.8478846550322,7.01965767938979));
#59845=CARTESIAN_POINT('Ctrl Pts',(0.20112886694132,1.84818970295575,7.01968801961105));
#59846=CARTESIAN_POINT('Ctrl Pts',(0.201337274452864,1.84835630599656,7.01970454549394));
#59847=CARTESIAN_POINT('Ctrl Pts',(0.202059612325509,1.84893522187206,7.01976181664903));
#59848=CARTESIAN_POINT('Ctrl Pts',(0.202572489442351,1.84934885540107,7.01980246760025));
#59849=CARTESIAN_POINT('Ctrl Pts',(0.207611232228897,1.85343815031116,7.0202017542648));
#59850=CARTESIAN_POINT('Ctrl Pts',(0.212038176777069,1.85723469882466,7.02055186820207));
#59851=CARTESIAN_POINT('Ctrl Pts',(0.216491383011562,1.86126858577677,7.0209062581015));
#59852=CARTESIAN_POINT('Ctrl Pts',(0.216622678369134,1.86138771558939,7.02091670871348));
#59853=CARTESIAN_POINT('Ctrl Pts',(0.217056353430299,1.86178186020601,7.02095123453494));
#59854=CARTESIAN_POINT('Ctrl Pts',(0.217358309353345,1.86205734293598,7.02097528506401));
#59855=CARTESIAN_POINT('Ctrl Pts',(0.218655209722032,1.86324506978252,7.02107863431232));
#59856=CARTESIAN_POINT('Ctrl Pts',(0.219644952947361,1.86416299598713,7.02115763907955));
#59857=CARTESIAN_POINT('Ctrl Pts',(0.226692960356299,1.87078244676926,7.02172143991755));
#59858=CARTESIAN_POINT('Ctrl Pts',(0.232534557943049,1.87671077091138,7.02219520868321));
#59859=CARTESIAN_POINT('Ctrl Pts',(0.247872276352638,1.89353176996463,7.02347881856043));
#59860=CARTESIAN_POINT('Ctrl Pts',(0.256875600910535,1.90484690750524,7.02427846625861));
#59861=CARTESIAN_POINT('Ctrl Pts',(0.272266173905734,1.92710824065107,7.02580309642709));
#59862=CARTESIAN_POINT('Ctrl Pts',(0.278826239208303,1.93790028804703,7.02652332578263));
#59863=CARTESIAN_POINT('Ctrl Pts',(0.288176330987927,1.95553715483856,7.02769673061448));
#59864=CARTESIAN_POINT('Ctrl Pts',(0.291393227305255,1.96214106630717,7.0281352146176));
#59865=CARTESIAN_POINT('Ctrl Pts',(0.29485569520998,1.96991290647565,7.02865251066988));
#59866=CARTESIAN_POINT('Ctrl Pts',(0.295324026915276,1.9709796451325,7.02872353832026));
#59867=CARTESIAN_POINT('Ctrl Pts',(0.295998891375999,1.97253973972819,7.02882746058706));
#59868=CARTESIAN_POINT('Ctrl Pts',(0.296210000059583,1.97303111600225,7.02886019901778));
#59869=CARTESIAN_POINT('Ctrl Pts',(0.296576059324835,1.97388903685823,7.02891737103253));
#59870=CARTESIAN_POINT('Ctrl Pts',(0.296731556348385,1.97425534820932,7.02894178595786));
#59871=CARTESIAN_POINT('Ctrl Pts',(0.297030531716962,1.97496330075563,7.0289889793721));
#59872=CARTESIAN_POINT('Ctrl Pts',(0.297174100185118,1.97530490343493,7.02901175475345));
#59873=CARTESIAN_POINT('Ctrl Pts',(0.297512923641364,1.97611499888253,7.02906577425903));
#59874=CARTESIAN_POINT('Ctrl Pts',(0.297707661215579,1.97658370575829,7.02909703587927));
#59875=CARTESIAN_POINT('Ctrl Pts',(0.298387361061039,1.97823062064229,7.02920690665641));
#59876=CARTESIAN_POINT('Ctrl Pts',(0.298866437925924,1.97941123105248,7.02928571464882));
#59877=CARTESIAN_POINT('Ctrl Pts',(0.305665512298149,1.99645589853904,7.03042421643172));
#59878=CARTESIAN_POINT('Ctrl Pts',(0.31072080174336,2.0127922077944,7.03152683671944));
#59879=CARTESIAN_POINT('Ctrl Pts',(0.319603290784243,2.05238341187556,7.0342222451962));
#59880=CARTESIAN_POINT('Ctrl Pts',(0.322224013824275,2.07580928575558,7.03583815506516));
#59881=CARTESIAN_POINT('Ctrl Pts',(0.322293176912857,2.10815679139511,7.03798389968668));
#59882=CARTESIAN_POINT('Ctrl Pts',(0.321947877706716,2.11700060934334,7.03856089700817));
#59883=CARTESIAN_POINT('Ctrl Pts',(0.32116725132738,2.12671282266034,7.03917617712368));
#59884=CARTESIAN_POINT('Ctrl Pts',(0.321091751784266,2.12760552842893,7.03923255874372));
#59885=CARTESIAN_POINT('Ctrl Pts',(0.320953571610498,2.12916204789581,7.03933055129066));
#59886=CARTESIAN_POINT('Ctrl Pts',(0.320892552122379,2.12982599836106,7.03937225124895));
#59887=CARTESIAN_POINT('Ctrl Pts',(0.320801231452367,2.13078692297071,7.03943245365061));
#59888=CARTESIAN_POINT('Ctrl Pts',(0.320772577993986,2.13108404632893,7.03945104790475));
#59889=CARTESIAN_POINT('Ctrl Pts',(0.32072193331689,2.13160168068814,7.03948340541087));
#59890=CARTESIAN_POINT('Ctrl Pts',(0.32070012743129,2.13182220921936,7.03949717916308));
#59891=CARTESIAN_POINT('Ctrl Pts',(0.320657370066782,2.13225011769745,7.03952388280717));
#59892=CARTESIAN_POINT('Ctrl Pts',(0.320636444926637,2.13245749921168,7.03953681417184));
#59893=CARTESIAN_POINT('Ctrl Pts',(0.320585815996408,2.13295443720816,7.03956777661595));
#59894=CARTESIAN_POINT('Ctrl Pts',(0.320555921019732,2.13324397464996,7.03958579685738));
#59895=CARTESIAN_POINT('Ctrl Pts',(0.320446709358328,2.13428786108203,7.03965069613542));
#59896=CARTESIAN_POINT('Ctrl Pts',(0.320365121052315,2.13504197763636,7.03969744803567));
#59897=CARTESIAN_POINT('Ctrl Pts',(0.318922930098314,2.14794589568213,7.04049527859276));
#59898=CARTESIAN_POINT('Ctrl Pts',(0.316874517048569,2.1600105221783,7.04120861049668));
#59899=CARTESIAN_POINT('Ctrl Pts',(0.30942305302643,2.19255340371752,7.04311333347171));
#59900=CARTESIAN_POINT('Ctrl Pts',(0.302681830683638,2.21266113052972,7.0442717244115));
#59901=CARTESIAN_POINT('Ctrl Pts',(0.287284903905455,2.24696585816649,7.04640569301412));
#59902=CARTESIAN_POINT('Ctrl Pts',(0.279414150299898,2.26142861548592,7.04736068426978));
#59903=CARTESIAN_POINT('Ctrl Pts',(0.269643080645295,2.27651098181804,7.048450619341));
#59904=CARTESIAN_POINT('Ctrl Pts',(0.268801867576734,2.27778940773735,7.04854377105531));
#59905=CARTESIAN_POINT('Ctrl Pts',(0.267623517663034,2.27955271390534,7.0486733376551));
#59906=CARTESIAN_POINT('Ctrl Pts',(0.267294096329676,2.28004274586078,7.04870946191507));
#59907=CARTESIAN_POINT('Ctrl Pts',(0.266733118802135,2.28087229707631,7.04877081493999));
#59908=CARTESIAN_POINT('Ctrl Pts',(0.266502255628791,2.2812122850633,7.04879601745041));
#59909=CARTESIAN_POINT('Ctrl Pts',(0.266045709841255,2.28188187229255,7.04884576583939));
#59910=CARTESIAN_POINT('Ctrl Pts',(0.265820063438153,2.28221149542505,7.04887031031383));
#59911=CARTESIAN_POINT('Ctrl Pts',(0.265323248928546,2.28293435262041,7.0489242559801));
#59912=CARTESIAN_POINT('Ctrl Pts',(0.265051818583454,2.2833274045317,7.04895366712411));
#59913=CARTESIAN_POINT('Ctrl Pts',(0.264110263514108,2.28468438635085,7.04905547918036));
#59914=CARTESIAN_POINT('Ctrl Pts',(0.263435752274419,2.28564524831094,7.04912804754129));
#59915=CARTESIAN_POINT('Ctrl Pts',(0.256730594076715,2.29508682408247,7.04984587661982));
#59916=CARTESIAN_POINT('Ctrl Pts',(0.250298408644388,2.30327354321823,7.05050668382026));
#59917=CARTESIAN_POINT('Ctrl Pts',(0.225153041468552,2.33227144318951,7.05299752426387));
#59918=CARTESIAN_POINT('Ctrl Pts',(0.204150559004003,2.35093034998928,7.05491988664511));
#59919=CARTESIAN_POINT('Ctrl Pts',(0.171892839572546,2.37282857960462,7.05752651879063));
#59920=CARTESIAN_POINT('Ctrl Pts',(0.162464046834826,2.37854635231268,7.05825146107769));
#59921=CARTESIAN_POINT('Ctrl Pts',(0.151867060814155,2.38425094465483,7.05901267943664));
#59922=CARTESIAN_POINT('Ctrl Pts',(0.150971987795774,2.38472734793461,7.05907657070885));
#59923=CARTESIAN_POINT('Ctrl Pts',(0.14942704564438,2.38554031099556,7.05918613545004));
#59924=CARTESIAN_POINT('Ctrl Pts',(0.148778257268236,2.3858788928244,7.05923193070509));
#59925=CARTESIAN_POINT('Ctrl Pts',(0.147850811300943,2.38635888471757,7.05929708181036));
#59926=CARTESIAN_POINT('Ctrl Pts',(0.147573098735881,2.38650210084832,7.05931655055731));
#59927=CARTESIAN_POINT('Ctrl Pts',(0.147095884659297,2.38674732177676,7.05934993599278));
#59928=CARTESIAN_POINT('Ctrl Pts',(0.14689648462927,2.38684952263256,7.05936386512978));
#59929=CARTESIAN_POINT('Ctrl Pts',(0.146514463445131,2.38704482166296,7.05939051148031));
#59930=CARTESIAN_POINT('Ctrl Pts',(0.146331860317846,2.38713795342769,7.05940323084658));
#59931=CARTESIAN_POINT('Ctrl Pts',(0.145901520745474,2.38735691931166,7.05943316586396));
#59932=CARTESIAN_POINT('Ctrl Pts',(0.145653709699228,2.38748260762058,7.05945037226648));
#59933=CARTESIAN_POINT('Ctrl Pts',(0.144921289292561,2.38785289682239,7.05950113422942));
#59934=CARTESIAN_POINT('Ctrl Pts',(0.144436221058027,2.38809659552977,7.05953463335479));
#59935=CARTESIAN_POINT('Ctrl Pts',(0.140181081151138,2.39022093361568,7.05982747000392));
#59936=CARTESIAN_POINT('Ctrl Pts',(0.136374866212024,2.39202880991834,7.06008236690488));
#59937=CARTESIAN_POINT('Ctrl Pts',(0.132254320782541,2.39388784332185,7.06035197954533));
#59938=CARTESIAN_POINT('Ctrl Pts',(0.131974384628198,2.39401365890281,7.06037026508446));
#59939=CARTESIAN_POINT('Ctrl Pts',(0.131051192966086,2.39442699756022,7.06043046742698));
#59940=CARTESIAN_POINT('Ctrl Pts',(0.130407170009668,2.39471281291533,7.06047230362381));
#59941=CARTESIAN_POINT('Ctrl Pts',(0.103852017062125,2.40639381636734,7.06219092124355));
#59942=CARTESIAN_POINT('Ctrl Pts',(0.0765503682063327,2.41432923185706,
7.0637158310133));
#59943=CARTESIAN_POINT('Ctrl Pts',(0.0333218479986648,2.42091810897705,
7.06619663437679));
#59944=CARTESIAN_POINT('Ctrl Pts',(0.0179384048535991,2.42214422122447,
7.0670899545166));
#59945=CARTESIAN_POINT('Ctrl Pts',(7.96595485979168E-5,2.42228428702588,
7.06816724825204));
#59946=CARTESIAN_POINT('Ctrl Pts',(-0.00236828513133685,2.42227559436703,
7.06831575554552));
#59947=CARTESIAN_POINT('Ctrl Pts',(-0.00552313522269598,2.42222844532618,
7.06850830501083));
#59948=CARTESIAN_POINT('Ctrl Pts',(-0.00623038693984165,2.42221554628234,
7.06855154548899));
#59949=CARTESIAN_POINT('Ctrl Pts',(-0.00737143835275037,2.42219097727389,
7.06862143075003));
#59950=CARTESIAN_POINT('Ctrl Pts',(-0.00780526965702664,2.4221807593615,
7.06864802999268));
#59951=CARTESIAN_POINT('Ctrl Pts',(-0.00863250842986229,2.42215960378743,
7.06869880513676));
#59952=CARTESIAN_POINT('Ctrl Pts',(-0.00902591937755676,2.42214882165154,
7.06872297611904));
#59953=CARTESIAN_POINT('Ctrl Pts',(-0.00992419464094185,2.42212255604658,
7.06877822047647));
#59954=CARTESIAN_POINT('Ctrl Pts',(-0.0104290433625144,2.42210660627061,
7.06880930841204));
#59955=CARTESIAN_POINT('Ctrl Pts',(-0.0119735212883351,2.42205417645872,
7.06890453741189));
#59956=CARTESIAN_POINT('Ctrl Pts',(-0.0130130054638803,2.42201384975603,
7.06896879886838));
#59957=CARTESIAN_POINT('Ctrl Pts',(-0.0207030291127939,2.42167821982743,
7.06944547540725));
#59958=CARTESIAN_POINT('Ctrl Pts',(-0.0273427632544859,2.42118196582502,
7.06986415895268));
#59959=CARTESIAN_POINT('Ctrl Pts',(-0.0358116689572604,2.42028449808203,
7.0704078687766));
#59960=CARTESIAN_POINT('Ctrl Pts',(-0.0376595818808863,2.42007247775069,
7.07052709518816));
#59961=CARTESIAN_POINT('Ctrl Pts',(-0.0418092754205066,2.41955992918412,
7.07079615898283));
#59962=CARTESIAN_POINT('Ctrl Pts',(-0.0441098366241475,2.41925050625653,
7.07094624719358));
#59963=CARTESIAN_POINT('Ctrl Pts',(-0.0684693614032441,2.41570585212978,
7.07254517118954));
#59964=CARTESIAN_POINT('Ctrl Pts',(-0.0901369512278037,2.41021497589176,
7.07405822799484));
#59965=CARTESIAN_POINT('Ctrl Pts',(-0.115653584872897,2.40084772983796,
7.07589449045489));
#59966=CARTESIAN_POINT('Ctrl Pts',(-0.120207120565101,2.39905744980875,
7.07622412330533));
#59967=CARTESIAN_POINT('Ctrl Pts',(-0.135336391650622,2.39270777545903,
7.07732271935609));
#59968=CARTESIAN_POINT('Ctrl Pts',(-0.145709373346801,2.38768493202435,
7.07808178952665));
#59969=CARTESIAN_POINT('Ctrl Pts',(-0.156700950913653,2.38161510128957,
7.07887623940425));
#59970=CARTESIAN_POINT('Ctrl Pts',(-0.157607285925889,2.38110886998203,
7.0789416697534));
#59971=CARTESIAN_POINT('Ctrl Pts',(-0.159165080916036,2.38022886484133,
7.07905397518339));
#59972=CARTESIAN_POINT('Ctrl Pts',(-0.159817703220184,2.37985718042873,
7.07910097711435));
#59973=CARTESIAN_POINT('Ctrl Pts',(-0.160740188345622,2.37932752324656,
7.07916734095207));
#59974=CARTESIAN_POINT('Ctrl Pts',(-0.161011123383687,2.37917143754537,
7.0791868230639));
#59975=CARTESIAN_POINT('Ctrl Pts',(-0.161475854312515,2.3789028044352,7.07922022435599));
#59976=CARTESIAN_POINT('Ctrl Pts',(-0.16166976038697,2.37879044894924,7.07923415601498));
#59977=CARTESIAN_POINT('Ctrl Pts',(-0.162040762312015,2.37857496113782,
7.07926080210328));
#59978=CARTESIAN_POINT('Ctrl Pts',(-0.162217876736977,2.37847186229695,
7.07927351869513));
#59979=CARTESIAN_POINT('Ctrl Pts',(-0.16263474548547,2.37822866907277,7.07930343994072));
#59980=CARTESIAN_POINT('Ctrl Pts',(-0.162874417783053,2.37808843335584,
7.07932063536708));
#59981=CARTESIAN_POINT('Ctrl Pts',(-0.163700383119109,2.37760371502831,
7.07937987046904));
#59982=CARTESIAN_POINT('Ctrl Pts',(-0.16428577215988,2.37725768360229,7.07942181014637));
#59983=CARTESIAN_POINT('Ctrl Pts',(-0.17105001857142,2.37323030077992,7.07990599145593));
#59984=CARTESIAN_POINT('Ctrl Pts',(-0.177105628573264,2.36934461405321,
7.08033522524814));
#59985=CARTESIAN_POINT('Ctrl Pts',(-0.187664495926979,2.36205908285699,
7.08108545653552));
#59986=CARTESIAN_POINT('Ctrl Pts',(-0.192217844814387,2.35873776629691,
7.08140961719347));
#59987=CARTESIAN_POINT('Ctrl Pts',(-0.202302524056698,2.35096853369105,
7.0821345884973));
#59988=CARTESIAN_POINT('Ctrl Pts',(-0.207778731450337,2.34645389117074,
7.08253331290991));
#59989=CARTESIAN_POINT('Ctrl Pts',(-0.223264097021067,2.33280428871435,
7.08368919425291));
#59990=CARTESIAN_POINT('Ctrl Pts',(-0.232851590242998,2.32321474087947,
7.0844419604639));
#59991=CARTESIAN_POINT('Ctrl Pts',(-0.251933419974083,2.30155735618141,
7.08608001480512));
#59992=CARTESIAN_POINT('Ctrl Pts',(-0.261226325242482,2.28935821004901,
7.08696804258917));
#59993=CARTESIAN_POINT('Ctrl Pts',(-0.270952073854046,2.27450529312675,
7.08803903124635));
#59994=CARTESIAN_POINT('Ctrl Pts',(-0.272264872822716,2.27244988308826,
7.08818699249668));
#59995=CARTESIAN_POINT('Ctrl Pts',(-0.273927660473173,2.26978018578954,
7.08837893193387));
#59996=CARTESIAN_POINT('Ctrl Pts',(-0.274299156291246,2.26917933533512,
7.08842211471879));
#59997=CARTESIAN_POINT('Ctrl Pts',(-0.274895554537778,2.26820760342883,
7.08849192920926));
#59998=CARTESIAN_POINT('Ctrl Pts',(-0.275121690404882,2.26783747859686,
7.08851851554316));
#59999=CARTESIAN_POINT('Ctrl Pts',(-0.275551613073455,2.26713060487741,
7.08856928093525));
#60000=CARTESIAN_POINT('Ctrl Pts',(-0.275755531635995,2.26679393671245,
7.08859345510692));
#60001=CARTESIAN_POINT('Ctrl Pts',(-0.276219929132113,2.26602404016256,
7.08864872761308));
#60002=CARTESIAN_POINT('Ctrl Pts',(-0.27648000607169,2.26559057159031,7.08867984056168));
#60003=CARTESIAN_POINT('Ctrl Pts',(-0.277273213120687,2.26426146022828,
7.08877522056662));
#60004=CARTESIAN_POINT('Ctrl Pts',(-0.277803014988361,2.26336384806036,
7.0888396085735));
#60005=CARTESIAN_POINT('Ctrl Pts',(-0.281706971019057,2.25667569500715,
7.08931919253454));
#60006=CARTESIAN_POINT('Ctrl Pts',(-0.284903902327578,2.25078410558769,
7.08974074312677));
#60007=CARTESIAN_POINT('Ctrl Pts',(-0.288795207152222,2.24304665213507,
7.09029379543921));
#60008=CARTESIAN_POINT('Ctrl Pts',(-0.289659727893182,2.24128785558589,
7.09041946800069));
#60009=CARTESIAN_POINT('Ctrl Pts',(-0.291530681329827,2.23739219843099,
7.09069773826261));
#60010=CARTESIAN_POINT('Ctrl Pts',(-0.292529765694621,2.23525195040702,
7.09085056001177));
#60011=CARTESIAN_POINT('Ctrl Pts',(-0.305097009313708,2.20753951564825,
7.09282849154357));
#60012=CARTESIAN_POINT('Ctrl Pts',(-0.313298970645674,2.18057466656254,
7.09475910487376));
#60013=CARTESIAN_POINT('Ctrl Pts',(-0.319636665225482,2.14248482875779,
7.09733682916207));
#60014=CARTESIAN_POINT('Ctrl Pts',(-0.320856640142542,2.13199412749797,
7.09802995583749));
#60015=CARTESIAN_POINT('Ctrl Pts',(-0.321659466671179,2.11996525965469,
7.09879224077578));
#60016=CARTESIAN_POINT('Ctrl Pts',(-0.321748881939039,2.11846838571895,
7.0988865248788));
#60017=CARTESIAN_POINT('Ctrl Pts',(-0.321849314519228,2.11656383228518,
7.09900571040348));
#60018=CARTESIAN_POINT('Ctrl Pts',(-0.321870008559195,2.11615671349427,
7.09903114244822));
#60019=CARTESIAN_POINT('Ctrl Pts',(-0.32190188266075,2.1155052694972,7.09907176367977));
#60020=CARTESIAN_POINT('Ctrl Pts',(-0.321913557060609,2.11526097061979,
7.09908698058751));
#60021=CARTESIAN_POINT('Ctrl Pts',(-0.321935175041236,2.11479752745301,
7.0991158159427));
#60022=CARTESIAN_POINT('Ctrl Pts',(-0.321945172890431,2.11457838812704,
7.09912943730214));
#60023=CARTESIAN_POINT('Ctrl Pts',(-0.321967555510945,2.11407653726298,
7.09916060098398));
#60024=CARTESIAN_POINT('Ctrl Pts',(-0.321979791658115,2.11379381993052,
7.09917813482476));
#60025=CARTESIAN_POINT('Ctrl Pts',(-0.32201632914032,2.11292307091952,7.09923207043524));
#60026=CARTESIAN_POINT('Ctrl Pts',(-0.322039392263881,2.112334984322,7.0992684028843));
#60027=CARTESIAN_POINT('Ctrl Pts',(-0.322202278613281,2.10786915782674,
7.09954360923591));
#60028=CARTESIAN_POINT('Ctrl Pts',(-0.322273676964038,2.103989033816,7.09977873866915));
#60029=CARTESIAN_POINT('Ctrl Pts',(-0.322277943000648,2.0913013741075,7.10053731914127));
#60030=CARTESIAN_POINT('Ctrl Pts',(-0.321919891811834,2.08249722386882,
7.10104757242948));
#60031=CARTESIAN_POINT('Ctrl Pts',(-0.319211921990328,2.04940199492332,
7.10294069795412));
#60032=CARTESIAN_POINT('Ctrl Pts',(-0.314467639224258,2.02539044210436,
7.1042693866788));
#60033=CARTESIAN_POINT('Ctrl Pts',(-0.30567200480236,1.99779105241879,7.10593111732195));
#60034=CARTESIAN_POINT('Ctrl Pts',(-0.304192581746576,1.99346871691982,
7.10619522486907));
#60035=CARTESIAN_POINT('Ctrl Pts',(-0.299517386227723,1.98070199020298,
7.1069889409143));
#60036=CARTESIAN_POINT('Ctrl Pts',(-0.296058353421467,1.97235945827574,
7.10752575666223));
#60037=CARTESIAN_POINT('Ctrl Pts',(-0.291776683206179,1.96314670199933,
7.10814361298504));
#60038=CARTESIAN_POINT('Ctrl Pts',(-0.291294000854892,1.96212228950569,
7.10821266981727));
#60039=CARTESIAN_POINT('Ctrl Pts',(-0.290582974552082,1.96063365493668,
7.10831354542218));
#60040=CARTESIAN_POINT('Ctrl Pts',(-0.290358892421207,1.96016739713914,
7.10834521623515));
#60041=CARTESIAN_POINT('Ctrl Pts',(-0.28996104752605,1.95934466305481,7.10840123504849));
#60042=CARTESIAN_POINT('Ctrl Pts',(-0.289787747158715,1.95898796332222,
7.10842556691501));
#60043=CARTESIAN_POINT('Ctrl Pts',(-0.289427701710891,1.95825035777583,
7.10847597480966));
#60044=CARTESIAN_POINT('Ctrl Pts',(-0.289240862124544,1.95786949918107,
7.10850205409969));
#60045=CARTESIAN_POINT('Ctrl Pts',(-0.288759771102451,1.9568937082195,7.10856900405214));
#60046=CARTESIAN_POINT('Ctrl Pts',(-0.288464433838895,1.95629931609841,
7.10860991262841));
#60047=CARTESIAN_POINT('Ctrl Pts',(-0.287244703520973,1.95386341461201,
7.10877808621948));
#60048=CARTESIAN_POINT('Ctrl Pts',(-0.286304512078766,1.95202991067064,
7.10890590462081));
#60049=CARTESIAN_POINT('Ctrl Pts',(-0.279946029491782,1.93991749142864,
7.10975866922158));
#60050=CARTESIAN_POINT('Ctrl Pts',(-0.273993429947364,1.92993020715675,
7.11050260852844));
#60051=CARTESIAN_POINT('Ctrl Pts',(-0.248903020062674,1.89258139615628,
7.11344902178578));
#60052=CARTESIAN_POINT('Ctrl Pts',(-0.226103662915226,1.86793995548581,
7.11578066242824));
#60053=CARTESIAN_POINT('Ctrl Pts',(-0.199486445672673,1.8468860819622,7.11797424850297));
#60054=CARTESIAN_POINT('Ctrl Pts',(-0.199040537904893,1.8465352849186,7.1180108583174));
#60055=CARTESIAN_POINT('Ctrl Pts',(-0.195517071114537,1.8437783944682,7.11829903657008));
#60056=CARTESIAN_POINT('Ctrl Pts',(-0.192396748829027,1.84142712694815,
7.11854761752251));
#60057=CARTESIAN_POINT('Ctrl Pts',(-0.188756945138123,1.83878679392749,
7.11882933053229));
#60058=CARTESIAN_POINT('Ctrl Pts',(-0.188278660338053,1.83844184310379,
7.11886618752649));
#60059=CARTESIAN_POINT('Ctrl Pts',(-0.187569272479577,1.83793316910757,
7.11892061199511));
#60060=CARTESIAN_POINT('Ctrl Pts',(-0.187338899510602,1.83776843713208,
7.11893824872901));
#60061=CARTESIAN_POINT('Ctrl Pts',(-0.186929677403547,1.83747663063074,
7.11896951064209));
#60062=CARTESIAN_POINT('Ctrl Pts',(-0.18675091567227,1.83734943507416,7.11898314421709));
#60063=CARTESIAN_POINT('Ctrl Pts',(-0.186372702278239,1.83708090364854,
7.11901194131849));
#60064=CARTESIAN_POINT('Ctrl Pts',(-0.18617322020817,1.83693961252398,7.11902710173152));
#60065=CARTESIAN_POINT('Ctrl Pts',(-0.185641118671591,1.83656363881565,
7.11906746653094));
#60066=CARTESIAN_POINT('Ctrl Pts',(-0.185308213614012,1.8363293582759,7.11909264318052));
#60067=CARTESIAN_POINT('Ctrl Pts',(-0.183751792665983,1.83523843720898,
7.11920999506939));
#60068=CARTESIAN_POINT('Ctrl Pts',(-0.182522749359586,1.83438966020019,
7.11930163885746));
#60069=CARTESIAN_POINT('Ctrl Pts',(-0.172622625957208,1.82765380720749,
7.1200320548807));
#60070=CARTESIAN_POINT('Ctrl Pts',(-0.16367399107364,1.82218370598194,7.12064473475317));
#60071=CARTESIAN_POINT('Ctrl Pts',(-0.130445673127193,1.80403604933509,
7.12281205583066));
#60072=CARTESIAN_POINT('Ctrl Pts',(-0.104843479137785,1.79402826287495,
7.12429384654248));
#60073=CARTESIAN_POINT('Ctrl Pts',(-0.0670853146933372,1.78457331872525,
7.12654263421604));
#60074=CARTESIAN_POINT('Ctrl Pts',(-0.0557460321925753,1.78237323090294,
7.12722404940653));
#60075=CARTESIAN_POINT('Ctrl Pts',(-0.0431215920958387,1.78062067494908,
7.12799881170899));
#60076=CARTESIAN_POINT('Ctrl Pts',(-0.0419282327445183,1.78046182041535,
7.12807220085131));
#60077=CARTESIAN_POINT('Ctrl Pts',(-0.0402552827254262,1.78024865793598,
7.12817530636383));
#60078=CARTESIAN_POINT('Ctrl Pts',(-0.0397764072498257,1.78018873384238,
7.1282048454214));
#60079=CARTESIAN_POINT('Ctrl Pts',(-0.0388996485715129,1.78008102031784,
7.12825897495029));
#60080=CARTESIAN_POINT('Ctrl Pts',(-0.0385018067514579,1.78003289685589,
7.1282835548352));
#60081=CARTESIAN_POINT('Ctrl Pts',(-0.037697380447532,1.77993711443681,
7.12833329121868));
#60082=CARTESIAN_POINT('Ctrl Pts',(-0.0372907929166976,1.77988948788141,
7.12835844869064));
#60083=CARTESIAN_POINT('Ctrl Pts',(-0.0362931625080061,1.77977455466068,
7.1284202234262));
#60084=CARTESIAN_POINT('Ctrl Pts',(-0.0357020236072169,1.77970810970246,
7.12845686778367));
#60085=CARTESIAN_POINT('Ctrl Pts',(-0.0335647189203274,1.77947386368942,
7.12858950544548));
#60086=CARTESIAN_POINT('Ctrl Pts',(-0.032017546546237,1.7793156209114,7.12868579922816));
#60087=CARTESIAN_POINT('Ctrl Pts',(-0.0231794226756824,1.7784762656267,
7.12923751714671));
#60088=CARTESIAN_POINT('Ctrl Pts',(-0.0158685849866832,1.7780326549048,
7.12970035524123));
#60089=CARTESIAN_POINT('Ctrl Pts',(-0.00289208019701325,1.77768828797407,
7.13053411471465));
#60090=CARTESIAN_POINT('Ctrl Pts',(0.00276796796728354,1.77768720740032,
7.13090188141825));
#60091=CARTESIAN_POINT('Ctrl Pts',(0.0352027912077775,1.77853540294144,
7.13303191850251));
#60092=CARTESIAN_POINT('Ctrl Pts',(0.061784958986285,1.78257114794478,7.13487763144612));
#60093=CARTESIAN_POINT('Ctrl Pts',(0.0972662818958669,1.79258794082323,
7.13732734817175));
#60094=CARTESIAN_POINT('Ctrl Pts',(0.106840108412954,1.79578273889988,7.13798535614099));
#60095=CARTESIAN_POINT('Ctrl Pts',(0.116932834428128,1.79968612255806,7.13866458056378));
#60096=CARTESIAN_POINT('Ctrl Pts',(0.117615486753771,1.79995282029013,7.13871044896925));
#60097=CARTESIAN_POINT('Ctrl Pts',(0.118564030454495,1.80032713073458,7.138774075309));
#60098=CARTESIAN_POINT('Ctrl Pts',(0.118830690286628,1.8004327705857,7.13879195042558));
#60099=CARTESIAN_POINT('Ctrl Pts',(0.119289838085621,1.80061537593076,7.13882270775962));
#60100=CARTESIAN_POINT('Ctrl Pts',(0.119482392858993,1.80069217117353,7.13883560025157));
#60101=CARTESIAN_POINT('Ctrl Pts',(0.119881274915942,1.80085170071506,7.1388622940213));
#60102=CARTESIAN_POINT('Ctrl Pts',(0.120087590361259,1.80093446256378,7.13887609350972));
#60103=CARTESIAN_POINT('Ctrl Pts',(0.120574576572685,1.80113039851237,7.13890864851831));
#60104=CARTESIAN_POINT('Ctrl Pts',(0.12085517478159,1.80124375497848,7.13892739296166));
#60105=CARTESIAN_POINT('Ctrl Pts',(0.121778037864629,1.80161808746332,7.13898899854824));
#60106=CARTESIAN_POINT('Ctrl Pts',(0.122419625975329,1.80188074293622,7.13903175864886));
#60107=CARTESIAN_POINT('Ctrl Pts',(0.123927931981081,1.80250390852192,7.13913213174345));
#60108=CARTESIAN_POINT('Ctrl Pts',(0.124793937513339,1.8028661413107,7.13918964366859));
#60109=CARTESIAN_POINT('Ctrl Pts',(0.134494618900455,1.80697363391175,7.13983267776966));
#60110=CARTESIAN_POINT('Ctrl Pts',(0.143160325168732,1.81110830088701,7.14039601304263));
#60111=CARTESIAN_POINT('Ctrl Pts',(0.177722036964782,1.82953662072146,7.14264763419519));
#60112=CARTESIAN_POINT('Ctrl Pts',(0.201776009326334,1.84697392182734,7.14423964867464));
#60113=CARTESIAN_POINT('Ctrl Pts',(0.230604817933909,1.87463296325583,7.14655866757371));
#60114=CARTESIAN_POINT('Ctrl Pts',(0.237741562551963,1.88217484460242,7.14717337216882));
#60115=CARTESIAN_POINT('Ctrl Pts',(0.245265900505138,1.89093735371872,7.14787560113998));
#60116=CARTESIAN_POINT('Ctrl Pts',(0.246025331195607,1.89183158651262,7.14794712972961));
#60117=CARTESIAN_POINT('Ctrl Pts',(0.247117402617992,1.89313182844161,7.14805094794052));
#60118=CARTESIAN_POINT('Ctrl Pts',(0.247453966939947,1.89353454206306,7.14808307704597));
#60119=CARTESIAN_POINT('Ctrl Pts',(0.248043919009222,1.89424395965151,7.14813963125053));
#60120=CARTESIAN_POINT('Ctrl Pts',(0.248297726024389,1.89455031480625,7.14816403921836));
#60121=CARTESIAN_POINT('Ctrl Pts',(0.248813660907834,1.89517542119086,7.14821381385264));
#60122=CARTESIAN_POINT('Ctrl Pts',(0.249075745001279,1.89549420744576,7.14823918222942));
#60123=CARTESIAN_POINT('Ctrl Pts',(0.249728483834574,1.89629128305521,7.14830257444544));
#60124=CARTESIAN_POINT('Ctrl Pts',(0.250118376256505,1.89677019202898,7.14834062899051));
#60125=CARTESIAN_POINT('Ctrl Pts',(0.250960873299347,1.897811136724,7.14842327229059));
#60126=CARTESIAN_POINT('Ctrl Pts',(0.251412970754599,1.89837357692311,7.14846788120274));
#60127=CARTESIAN_POINT('Ctrl Pts',(0.25269068172186,1.89997411596522,7.14859470146078));
#60128=CARTESIAN_POINT('Ctrl Pts',(0.253511773554806,1.901015790834,7.14867709293906));
#60129=CARTESIAN_POINT('Ctrl Pts',(0.273077032596814,1.92615484604641,7.15066210033693));
#60130=CARTESIAN_POINT('Ctrl Pts',(0.288305116808705,1.95278424782804,7.15271337312039));
#60131=CARTESIAN_POINT('Ctrl Pts',(0.300805321201804,1.98429018158299,7.15500565593547));
#60132=CARTESIAN_POINT('Ctrl Pts',(0.302002508421689,1.9874518385644,7.1552340245765));
#60133=CARTESIAN_POINT('Ctrl Pts',(0.308290016881722,2.0048797202458,7.15648216933656));
#60134=CARTESIAN_POINT('Ctrl Pts',(0.312420146394423,2.01947436860702,7.15748931116751));
#60135=CARTESIAN_POINT('Ctrl Pts',(0.315694341713643,2.03519961990106,7.15849948684836));
#60136=CARTESIAN_POINT('Ctrl Pts',(0.315876379523323,2.03609288335539,7.15855661456581));
#60137=CARTESIAN_POINT('Ctrl Pts',(0.31611607956451,2.0372951465529,7.15863315070452));
#60138=CARTESIAN_POINT('Ctrl Pts',(0.316177081344159,2.03760346452093,7.15865274703949));
#60139=CARTESIAN_POINT('Ctrl Pts',(0.316279018192595,2.038122666324,7.15868569382008));
#60140=CARTESIAN_POINT('Ctrl Pts',(0.316320193447893,2.03833350188774,7.15869905800062));
#60141=CARTESIAN_POINT('Ctrl Pts',(0.316398753785029,2.03873791468038,7.15872466396509));
#60142=CARTESIAN_POINT('Ctrl Pts',(0.316436171767975,2.03893148363099,7.15873690753517));
#60143=CARTESIAN_POINT('Ctrl Pts',(0.316524305927,2.03938967104083,7.15876585918351));
#60144=CARTESIAN_POINT('Ctrl Pts',(0.316574867840449,2.03965431852916,7.15878255831355));
#60145=CARTESIAN_POINT('Ctrl Pts',(0.316722372208424,2.0404316625897,7.15883154093794));
#60146=CARTESIAN_POINT('Ctrl Pts',(0.316818402084771,2.04094453464202,7.15886377236693));
#60147=CARTESIAN_POINT('Ctrl Pts',(0.317528596811942,2.0447891026014,7.15910475479407));
#60148=CARTESIAN_POINT('Ctrl Pts',(0.318091466890424,2.04813022175631,7.15931064142299));
#60149=CARTESIAN_POINT('Ctrl Pts',(0.319823245807952,2.05950171179576,7.1600012918486));
#60150=CARTESIAN_POINT('Ctrl Pts',(0.320741611420546,2.06756761233605,7.16047420936283));
#60151=CARTESIAN_POINT('Ctrl Pts',(0.323881355451705,2.1090211348548,7.16285667348626));
#60152=CARTESIAN_POINT('Ctrl Pts',(0.321198429221979,2.1425710082323,7.16464967167782));
#60153=CARTESIAN_POINT('Ctrl Pts',(0.313318833953293,2.17544936214753,7.16665056897304));
#60154=CARTESIAN_POINT('Ctrl Pts',(0.313236765231017,2.17578935851811,7.1666712845979));
#60155=CARTESIAN_POINT('Ctrl Pts',(0.311800040832471,2.18169926013288,7.16703179500768));
#60156=CARTESIAN_POINT('Ctrl Pts',(0.310297640138955,2.18723189099882,7.16737590616462));
#60157=CARTESIAN_POINT('Ctrl Pts',(0.308365982052197,2.19366195326035,7.16778465049679));
#60158=CARTESIAN_POINT('Ctrl Pts',(0.30807909327924,2.19460133522471,7.16784458681572));
#60159=CARTESIAN_POINT('Ctrl Pts',(0.307639639309348,2.19601707204352,7.1679352570114));
#60160=CARTESIAN_POINT('Ctrl Pts',(0.307490250286527,2.19649441316712,7.16796588668877));
#60161=CARTESIAN_POINT('Ctrl Pts',(0.307221508568814,2.19734615925498,7.16802064635261));
#60162=CARTESIAN_POINT('Ctrl Pts',(0.307102580912326,2.19772069813407,7.16804476233239));
#60163=CARTESIAN_POINT('Ctrl Pts',(0.306852745720532,2.19850254364545,7.16809518079205));
#60164=CARTESIAN_POINT('Ctrl Pts',(0.30672171163757,2.19890980875607,7.16812148739707));
#60165=CARTESIAN_POINT('Ctrl Pts',(0.306389328207243,2.19993587263861,7.16818787464146));
#60166=CARTESIAN_POINT('Ctrl Pts',(0.306186915577639,2.2005543226244,7.16822799026202));
#60167=CARTESIAN_POINT('Ctrl Pts',(0.305733974676915,2.20192418623585,7.16831707287149));
#60168=CARTESIAN_POINT('Ctrl Pts',(0.305482547092245,2.20267529603392,7.16836606940177));
#60169=CARTESIAN_POINT('Ctrl Pts',(0.30474431457889,2.20485396154392,7.16850863330048));
#60170=CARTESIAN_POINT('Ctrl Pts',(0.304250258802843,2.20627902151181,7.16860244015751));
#60171=CARTESIAN_POINT('Ctrl Pts',(0.302540715828281,2.21110041995744,7.16892173382152));
#60172=CARTESIAN_POINT('Ctrl Pts',(0.301278250510866,2.21447970178233,7.16914876989356));
#60173=CARTESIAN_POINT('Ctrl Pts',(0.295638752613398,2.22883529978783,7.17012750251643));
#60174=CARTESIAN_POINT('Ctrl Pts',(0.290716989389823,2.23958647770634,7.17089697834695));
#60175=CARTESIAN_POINT('Ctrl Pts',(0.270049185383439,2.27887408868154,7.17384286216314));
#60176=CARTESIAN_POINT('Ctrl Pts',(0.250599239559919,2.30523748408877,7.1761193685785));
#60177=CARTESIAN_POINT('Ctrl Pts',(0.226488499113328,2.32927339904247,7.17827201546946));
#60178=CARTESIAN_POINT('Ctrl Pts',(0.225441494859509,2.33030298376181,7.17836435233834));
#60179=CARTESIAN_POINT('Ctrl Pts',(0.22408377294486,2.3316199847557,7.17848258713693));
#60180=CARTESIAN_POINT('Ctrl Pts',(0.223779497287755,2.33191397377896,7.17850898810828));
#60181=CARTESIAN_POINT('Ctrl Pts',(0.223295927562847,2.33237935768715,7.17855079198686));
#60182=CARTESIAN_POINT('Ctrl Pts',(0.223117014412688,2.33255114496775,7.17856622549574));
#60183=CARTESIAN_POINT('Ctrl Pts',(0.222795758114769,2.33285889404903,7.17859387799154));
#60184=CARTESIAN_POINT('Ctrl Pts',(0.222653489772382,2.33299493098383,7.17860610286065));
#60185=CARTESIAN_POINT('Ctrl Pts',(0.222318309545093,2.33331484284125,7.17863485494019));
#60186=CARTESIAN_POINT('Ctrl Pts',(0.222125294429452,2.33349860861445,7.17865137358169));
#60187=CARTESIAN_POINT('Ctrl Pts',(0.221563812790055,2.33403185764265,7.17869931577494));
#60188=CARTESIAN_POINT('Ctrl Pts',(0.221194745726188,2.33438071166631,7.17873069057425));
#60189=CARTESIAN_POINT('Ctrl Pts',(0.218603498120495,2.33681847016637,7.1789500236647));
#60190=CARTESIAN_POINT('Ctrl Pts',(0.216352492677694,2.33887669989179,7.17913566870703));
#60191=CARTESIAN_POINT('Ctrl Pts',(0.209329151504021,2.3451178252093,7.17970129097684));
#60192=CARTESIAN_POINT('Ctrl Pts',(0.204462004820493,2.34919217784713,7.18007439744852));
#60193=CARTESIAN_POINT('Ctrl Pts',(0.188122383355537,2.36206899489701,7.1812785256904));
#60194=CARTESIAN_POINT('Ctrl Pts',(0.176177346588848,2.37024393572151,7.18208447508553));
#60195=CARTESIAN_POINT('Ctrl Pts',(0.147385652487123,2.38722535685445,7.18395283498972));
#60196=CARTESIAN_POINT('Ctrl Pts',(0.130231043386789,2.39539926367027,7.18501474082521));
#60197=CARTESIAN_POINT('Ctrl Pts',(0.11085954001258,2.40261237200339,7.18622681780977));
#60198=CARTESIAN_POINT('Ctrl Pts',(0.10925630645183,2.40319489549231,7.18632720113826));
#60199=CARTESIAN_POINT('Ctrl Pts',(0.101584536312963,2.40591362813335,7.18680802332566));
#60200=CARTESIAN_POINT('Ctrl Pts',(0.0954578942667162,2.40788041106997,
7.18719344223938));
#60201=CARTESIAN_POINT('Ctrl Pts',(0.0882872019016843,2.40994774773028,
7.18764765319786));
#60202=CARTESIAN_POINT('Ctrl Pts',(0.0872962442046343,2.41022830633561,
7.1877104901779));
#60203=CARTESIAN_POINT('Ctrl Pts',(0.0858192992364137,2.41063882010222,
7.18780424925866));
#60204=CARTESIAN_POINT('Ctrl Pts',(0.0853343182806539,2.41077239709307,
7.18783505358634));
#60205=CARTESIAN_POINT('Ctrl Pts',(0.084469598281967,2.41100838779882,7.18789000844686));
#60206=CARTESIAN_POINT('Ctrl Pts',(0.0840899799342798,2.41111124310705,
7.1879141445922));
#60207=CARTESIAN_POINT('Ctrl Pts',(0.0833560756061799,2.4113086486802,7.18796082702655));
#60208=CARTESIAN_POINT('Ctrl Pts',(0.0830018145008967,2.41140328975678,
7.1879833703278));
#60209=CARTESIAN_POINT('Ctrl Pts',(0.082035653744319,2.41165963439264,7.18804487754866));
#60210=CARTESIAN_POINT('Ctrl Pts',(0.0814234403976755,2.41182013972752,
7.18808388021184));
#60211=CARTESIAN_POINT('Ctrl Pts',(0.0790414342392191,2.41243714225304,
7.18823574482878));
#60212=CARTESIAN_POINT('Ctrl Pts',(0.0772682701159036,2.41288037713807,
7.18834903447287));
#60213=CARTESIAN_POINT('Ctrl Pts',(0.0728376085493974,2.41394794190226,
7.18863275465341));
#60214=CARTESIAN_POINT('Ctrl Pts',(0.0701758074652522,2.41455362460552,
7.18880377672876));
#60215=CARTESIAN_POINT('Ctrl Pts',(0.0596396439274277,2.41681069938714,
7.18948312548077));
#60216=CARTESIAN_POINT('Ctrl Pts',(0.0517128472239275,2.41820067527034,
7.18999958319172));
#60217=CARTESIAN_POINT('Ctrl Pts',(0.032605481168604,2.42081837204902,7.19125731425797));
#60218=CARTESIAN_POINT('Ctrl Pts',(0.021396757741781,2.42176029519217,7.19200570697803));
#60219=CARTESIAN_POINT('Ctrl Pts',(-0.0164326227418953,2.42295379152613,
7.19455264444582));
#60220=CARTESIAN_POINT('Ctrl Pts',(-0.0430306160610507,2.42049607370513,
7.19638649478743));
#60221=CARTESIAN_POINT('Ctrl Pts',(-0.0703810063063582,2.41449899351517,
7.19815564912526));
#60222=CARTESIAN_POINT('Ctrl Pts',(-0.0717351724495111,2.41419288370309,
7.19824290998145));
#60223=CARTESIAN_POINT('Ctrl Pts',(-0.0734905773858463,2.41378413291825,
7.19835555540831));
#60224=CARTESIAN_POINT('Ctrl Pts',(-0.0738936292391306,2.41368946204519,
7.19838138719749));
#60225=CARTESIAN_POINT('Ctrl Pts',(-0.0745119826531165,2.41354296213611,
7.19842096697865));
#60226=CARTESIAN_POINT('Ctrl Pts',(-0.0747274131820014,2.41349168790226,
7.19843474686019));
#60227=CARTESIAN_POINT('Ctrl Pts',(-0.0751548315140514,2.41338949321313,
7.19846206737511));
#60228=CARTESIAN_POINT('Ctrl Pts',(-0.0753668191636071,2.41333858001526,
7.19847560825721));
#60229=CARTESIAN_POINT('Ctrl Pts',(-0.0758389769710143,2.41322467471814,
7.19850574701212));
#60230=CARTESIAN_POINT('Ctrl Pts',(-0.0760991197051235,2.41316157373096,
7.19852233845807));
#60231=CARTESIAN_POINT('Ctrl Pts',(-0.0768580096499789,2.41297649369226,
7.19857069914261));
#60232=CARTESIAN_POINT('Ctrl Pts',(-0.0773565472843937,2.41285364605851,
7.19860241830899));
#60233=CARTESIAN_POINT('Ctrl Pts',(-0.0809409877734502,2.41196129091386,
7.19883012729805));
#60234=CARTESIAN_POINT('Ctrl Pts',(-0.0840157813233215,2.41114729770155,
7.19902359793514));
#60235=CARTESIAN_POINT('Ctrl Pts',(-0.0914916249952602,2.40904930179883,
7.19949055579906));
#60236=CARTESIAN_POINT('Ctrl Pts',(-0.0958783945567755,2.40771663296007,
7.19976163194437));
#60237=CARTESIAN_POINT('Ctrl Pts',(-0.114111452681419,2.40174975711589,
7.20088171396187));
#60238=CARTESIAN_POINT('Ctrl Pts',(-0.127663939002439,2.39627069405924,
7.20169867588525));
#60239=CARTESIAN_POINT('Ctrl Pts',(-0.154204702977334,2.38337994355875,
7.20334821530274));
#60240=CARTESIAN_POINT('Ctrl Pts',(-0.167142213809476,2.37594697780071,
7.20417905263917));
#60241=CARTESIAN_POINT('Ctrl Pts',(-0.183300197286749,2.36510931582671,
7.2052954717734));
#60242=CARTESIAN_POINT('Ctrl Pts',(-0.187027678167634,2.36249296534632,
7.20555881678487));
#60243=CARTESIAN_POINT('Ctrl Pts',(-0.197927452028649,2.3544922710342,7.20634836907675));
#60244=CARTESIAN_POINT('Ctrl Pts',(-0.204931320866296,2.34888696867695,
7.2068816840926));
#60245=CARTESIAN_POINT('Ctrl Pts',(-0.212459121869228,2.34232897561804,
7.2074888831766));
#60246=CARTESIAN_POINT('Ctrl Pts',(-0.213223131211375,2.34165700314452,
7.20755091396228));
#60247=CARTESIAN_POINT('Ctrl Pts',(-0.214365411281454,2.34064269432955,
7.20764427345308));
#60248=CARTESIAN_POINT('Ctrl Pts',(-0.214746077159248,2.34030305497026,
7.20767548924522));
#60249=CARTESIAN_POINT('Ctrl Pts',(-0.215402343392353,2.33971471355354,
7.20772948536364));
#60250=CARTESIAN_POINT('Ctrl Pts',(-0.215678324238804,2.33946643582065,
7.20775224780742));
#60251=CARTESIAN_POINT('Ctrl Pts',(-0.216232205412781,2.33896641933254,
7.20779804278728));
#60252=CARTESIAN_POINT('Ctrl Pts',(-0.216510096595333,2.33871467130599,
7.20782107569694));
#60253=CARTESIAN_POINT('Ctrl Pts',(-0.217073276123506,2.33820268162525,
7.2078678704868));
#60254=CARTESIAN_POINT('Ctrl Pts',(-0.217358537272114,2.3379424111278,7.20789163356988));
#60255=CARTESIAN_POINT('Ctrl Pts',(-0.218260045614617,2.33711690653498,
7.20796692462412));
#60256=CARTESIAN_POINT('Ctrl Pts',(-0.218874557278458,2.3365497897515,7.2080185327248));
#60257=CARTESIAN_POINT('Ctrl Pts',(-0.222667778699551,2.33302168910037,
7.20833888492995));
#60258=CARTESIAN_POINT('Ctrl Pts',(-0.225788427638567,2.32999919615949,
7.20861026591442));
#60259=CARTESIAN_POINT('Ctrl Pts',(-0.234845730527272,2.32086476756189,
7.20942202879155));
#60260=CARTESIAN_POINT('Ctrl Pts',(-0.240601795031474,2.31457986302706,
7.20996998163263));
#60261=CARTESIAN_POINT('Ctrl Pts',(-0.24966590761539,2.303859226455,7.21088781990901));
#60262=CARTESIAN_POINT('Ctrl Pts',(-0.253121022527009,2.29955298261628,
7.21125231329694));
#60263=CARTESIAN_POINT('Ctrl Pts',(-0.27552916716822,2.27010602979294,7.21371474962178));
#60264=CARTESIAN_POINT('Ctrl Pts',(-0.290819687747357,2.24239475184208,
7.21590979668551));
#60265=CARTESIAN_POINT('Ctrl Pts',(-0.302391678940644,2.21145780564612,
7.21799977192156));
#60266=CARTESIAN_POINT('Ctrl Pts',(-0.302923353477104,2.21000460025734,
7.21809711887514));
#60267=CARTESIAN_POINT('Ctrl Pts',(-0.303588233500547,2.20814592955057,
7.21822052514394));
#60268=CARTESIAN_POINT('Ctrl Pts',(-0.303731117227819,2.207743983734,7.21824714682433));
#60269=CARTESIAN_POINT('Ctrl Pts',(-0.303956903541944,2.20710480644401,
7.21828937549967));
#60270=CARTESIAN_POINT('Ctrl Pts',(-0.304040326829884,2.20686776144576,
7.21830501342331));
#60271=CARTESIAN_POINT('Ctrl Pts',(-0.304195705405711,2.20642460287695,
7.21833420545718));
#60272=CARTESIAN_POINT('Ctrl Pts',(-0.304267727977743,2.20621851531857,
7.21834776349157));
#60273=CARTESIAN_POINT('Ctrl Pts',(-0.304429143692553,2.20575512418161,
7.21837820976048));
#60274=CARTESIAN_POINT('Ctrl Pts',(-0.304518419857189,2.20549778096738,
7.21839509093392));
#60275=CARTESIAN_POINT('Ctrl Pts',(-0.304782404824621,2.20473370343698,
7.21844513330403));
#60276=CARTESIAN_POINT('Ctrl Pts',(-0.30495617691483,2.2042266429354,7.21847823895089));
#60277=CARTESIAN_POINT('Ctrl Pts',(-0.306346400221008,2.2001367808294,7.21874444627241));
#60278=CARTESIAN_POINT('Ctrl Pts',(-0.30750099835517,2.196533055817,7.21897396368596));
#60279=CARTESIAN_POINT('Ctrl Pts',(-0.311460670305453,2.18338132334846,
7.21979619343975));
#60280=CARTESIAN_POINT('Ctrl Pts',(-0.313886840694076,2.17372435827734,
7.22037084623118));
#60281=CARTESIAN_POINT('Ctrl Pts',(-0.320111158949036,2.14299066923983,
7.22215240170525));
#60282=CARTESIAN_POINT('Ctrl Pts',(-0.322259181944044,2.12164123795382,
7.22332463650292));
#60283=CARTESIAN_POINT('Ctrl Pts',(-0.322274912962847,2.10023685394134,
7.22454439956175));
#60284=CARTESIAN_POINT('',(-0.321882949708748,2.09979413277033,7.34972265507269));
#60285=CARTESIAN_POINT('Ctrl Pts',(-0.3219654526091,2.10024677492677,7.22472265507269));
#60286=CARTESIAN_POINT('Ctrl Pts',(-0.321458228780833,2.02894014117497,
7.22911504031661));
#60287=CARTESIAN_POINT('Ctrl Pts',(-0.262891613614646,1.84935084621839,
7.24013087340147));
#60288=CARTESIAN_POINT('Ctrl Pts',(0.034383760505689,1.72048342076356,7.25777015432727));
#60289=CARTESIAN_POINT('Ctrl Pts',(0.337716885669452,1.92347129968311,7.27764049785004));
#60290=CARTESIAN_POINT('Ctrl Pts',(0.331240744233873,2.28840022893095,7.29751084137284));
#60291=CARTESIAN_POINT('Ctrl Pts',(0.0208963143190576,2.48049759650978,
7.31738118489562));
#60292=CARTESIAN_POINT('Ctrl Pts',(-0.267716732443814,2.34302254774173,
7.33478512279558));
#60293=CARTESIAN_POINT('Ctrl Pts',(-0.32148895242199,2.1673236380514,7.3455656128546));
#60294=CARTESIAN_POINT('Ctrl Pts',(-0.321882949708748,2.09979413277033,
7.34972265507269));
#60295=CARTESIAN_POINT('',(-0.322274866683432,2.10029313678766,7.59976792125168));
#60296=CARTESIAN_POINT('Ctrl Pts',(-0.32227492433765,2.09977916485371,7.34949702710362));
#60297=CARTESIAN_POINT('Ctrl Pts',(-0.322261526895343,2.08022765877105,
7.35077232927699));
#60298=CARTESIAN_POINT('Ctrl Pts',(-0.320468946951427,2.0607191748254,7.35209519898572));
#60299=CARTESIAN_POINT('Ctrl Pts',(-0.313453942902018,2.02271891291142,
7.35470899680524));
#60300=CARTESIAN_POINT('Ctrl Pts',(-0.308325470672367,2.0042851036715,7.35599397997341));
#60301=CARTESIAN_POINT('Ctrl Pts',(-0.301330739653725,1.98571299797414,
7.35723962346725));
#60302=CARTESIAN_POINT('Ctrl Pts',(-0.301065055575812,1.98501493214401,
7.35728636570966));
#60303=CARTESIAN_POINT('Ctrl Pts',(-0.300684958015297,1.98402660228161,
7.35735242747226));
#60304=CARTESIAN_POINT('Ctrl Pts',(-0.300572548783337,1.98373557777692,
7.35737186572807));
#60305=CARTESIAN_POINT('Ctrl Pts',(-0.300378713467072,1.98323590327112,
7.35740521500175));
#60306=CARTESIAN_POINT('Ctrl Pts',(-0.300297492295101,1.98302717447438,
7.35741913839949));
#60307=CARTESIAN_POINT('Ctrl Pts',(-0.300141482836316,1.98262748206851,
7.35744578541107));
#60308=CARTESIAN_POINT('Ctrl Pts',(-0.300066729973869,1.98243650546134,
7.35745851115518));
#60309=CARTESIAN_POINT('Ctrl Pts',(-0.299890118738951,1.9819865696529,7.35748847778705));
#60310=CARTESIAN_POINT('Ctrl Pts',(-0.299788106970629,1.98172767026954,
7.35750570937793));
#60311=CARTESIAN_POINT('Ctrl Pts',(-0.299485520503827,1.98096263175371,
7.3575565946343));
#60312=CARTESIAN_POINT('Ctrl Pts',(-0.299283997157887,1.98045686516639,
7.3575901914773));
#60313=CARTESIAN_POINT('Ctrl Pts',(-0.297495480792886,1.97600106535583,
7.35788581698478));
#60314=CARTESIAN_POINT('Ctrl Pts',(-0.295831558408913,1.97208209588234,
7.35814331137904));
#60315=CARTESIAN_POINT('Ctrl Pts',(-0.29397869153214,1.96794781665378,7.35841343419876));
#60316=CARTESIAN_POINT('Ctrl Pts',(-0.293866688269368,1.96769875386821,
7.35842970137416));
#60317=CARTESIAN_POINT('Ctrl Pts',(-0.293703563278234,1.96733724033889,
7.35845330491927));
#60318=CARTESIAN_POINT('Ctrl Pts',(-0.293652693554999,1.96722467679861,
7.35846065314043));
#60319=CARTESIAN_POINT('Ctrl Pts',(-0.293200061794657,1.96622463448198,
7.35852592653383));
#60320=CARTESIAN_POINT('Ctrl Pts',(-0.292794337953979,1.96533894267379,
7.35858366605395));
#60321=CARTESIAN_POINT('Ctrl Pts',(-0.292167466632221,1.96398671538254,
7.35867173229371));
#60322=CARTESIAN_POINT('Ctrl Pts',(-0.291949207105771,1.96351885614851,
7.35870218639288));
#60323=CARTESIAN_POINT('Ctrl Pts',(-0.290771418524515,1.96100991222749,
7.35886542374839));
#60324=CARTESIAN_POINT('Ctrl Pts',(-0.289791587259936,1.95897837493863,
7.35899732995153));
#60325=CARTESIAN_POINT('Ctrl Pts',(-0.276973670951746,1.93310015156548,
7.36067617644098));
#60326=CARTESIAN_POINT('Ctrl Pts',(-0.262245586195704,1.91079782598986,
7.36211581844594));
#60327=CARTESIAN_POINT('Ctrl Pts',(-0.24084272486558,1.88576713348248,7.36399246416441));
#60328=CARTESIAN_POINT('Ctrl Pts',(-0.236605073266455,1.88109597406637,
7.36435522998365));
#60329=CARTESIAN_POINT('Ctrl Pts',(-0.227816800433414,1.87196216183603,
7.36509426499083));
#60330=CARTESIAN_POINT('Ctrl Pts',(-0.223265442835,1.86750422730543,7.36547046707366));
#60331=CARTESIAN_POINT('Ctrl Pts',(-0.216897506407837,1.86162650673583,
7.36599019398776));
#60332=CARTESIAN_POINT('Ctrl Pts',(-0.215193244512747,1.86008685388274,
7.36612866865216));
#60333=CARTESIAN_POINT('Ctrl Pts',(-0.212279073396333,1.85751018737441,
7.36636449914988));
#60334=CARTESIAN_POINT('Ctrl Pts',(-0.211077649320833,1.85646367818252,
7.3664614568349));
#60335=CARTESIAN_POINT('Ctrl Pts',(-0.209413159194657,1.85503538126217,
7.36659543929197));
#60336=CARTESIAN_POINT('Ctrl Pts',(-0.208956699348618,1.85464590187465,
7.36663214642671));
#60337=CARTESIAN_POINT('Ctrl Pts',(-0.208219933323152,1.85402079542729,
7.36669133923831));
#60338=CARTESIAN_POINT('Ctrl Pts',(-0.207940307135927,1.85378436608983,
7.36671379194235));
#60339=CARTESIAN_POINT('Ctrl Pts',(-0.207356961395593,1.85329283855796,
7.3667606055309));
#60340=CARTESIAN_POINT('Ctrl Pts',(-0.207053172801086,1.8530378235908,7.36678496976293));
#60341=CARTESIAN_POINT('Ctrl Pts',(-0.206351776221203,1.85245124095413,
7.36684118892952));
#60342=CARTESIAN_POINT('Ctrl Pts',(-0.205953839282455,1.85212006992372,
7.3668730599499));
#60343=CARTESIAN_POINT('Ctrl Pts',(-0.204681255525725,1.85106618029524,
7.36697490402675));
#60344=CARTESIAN_POINT('Ctrl Pts',(-0.203803596628387,1.85034712718464,
7.36704502546367));
#60345=CARTESIAN_POINT('Ctrl Pts',(-0.195856494145233,1.8439060166101,7.36767895228184));
#60346=CARTESIAN_POINT('Ctrl Pts',(-0.188552215527339,1.83848149261084,
7.36825457976716));
#60347=CARTESIAN_POINT('Ctrl Pts',(-0.167723009508977,1.82433928251443,
7.36987952474492));
#60348=CARTESIAN_POINT('Ctrl Pts',(-0.153761059997696,1.81631485004823,
7.37095176845409));
#60349=CARTESIAN_POINT('Ctrl Pts',(-0.127699142116004,1.80382699188026,
7.37290251104633));
#60350=CARTESIAN_POINT('Ctrl Pts',(-0.115817745704351,1.79898209588476,
7.37377406913718));
#60351=CARTESIAN_POINT('Ctrl Pts',(-0.0952859930722547,1.79200595013497,
7.37522549140947));
#60352=CARTESIAN_POINT('Ctrl Pts',(-0.0867779253147608,1.78950141303003,
7.37581163260688));
#60353=CARTESIAN_POINT('Ctrl Pts',(-0.0744120500520206,1.78640937235369,
7.37663215051821));
#60354=CARTESIAN_POINT('Ctrl Pts',(-0.0706304143673872,1.78553603885967,
7.37687892080602));
#60355=CARTESIAN_POINT('Ctrl Pts',(-0.066306250351506,1.78461936089861,
7.37715567121209));
#60356=CARTESIAN_POINT('Ctrl Pts',(-0.0657784934869911,1.78450886516372,
7.37718935655519));
#60357=CARTESIAN_POINT('Ctrl Pts',(-0.0649830671551264,1.78434441053295,
7.37723998608531));
#60358=CARTESIAN_POINT('Ctrl Pts',(-0.0647156057062469,1.78428946714106,
7.37725698632624));
#60359=CARTESIAN_POINT('Ctrl Pts',(-0.0642341231477217,1.7841911959269,
7.3772875466632));
#60360=CARTESIAN_POINT('Ctrl Pts',(-0.0640201282999115,1.78414774580501,
7.37730111375834));
#60361=CARTESIAN_POINT('Ctrl Pts',(-0.0635602291084476,1.78405485315791,
7.37733023775003));
#60362=CARTESIAN_POINT('Ctrl Pts',(-0.0633143119057035,1.78400548035397,
7.37734579057241));
#60363=CARTESIAN_POINT('Ctrl Pts',(-0.0626519814308786,1.78387330846248,
7.37738762491545));
#60364=CARTESIAN_POINT('Ctrl Pts',(-0.0622354599460625,1.78379104470323,
7.37741387575172));
#60365=CARTESIAN_POINT('Ctrl Pts',(-0.0603190239079019,1.78341647839241,
7.37753439723656));
#60366=CARTESIAN_POINT('Ctrl Pts',(-0.0588171728557488,1.78313401698438,
7.37762811434973));
#60367=CARTESIAN_POINT('Ctrl Pts',(-0.0288296998344187,1.77771466201601,
7.37948581521866));
#60368=CARTESIAN_POINT('Ctrl Pts',(0.000222891550511969,1.77642687310158,
7.3810505465331));
#60369=CARTESIAN_POINT('Ctrl Pts',(0.0425923321829934,1.78026312012273,
7.3834449487952));
#60370=CARTESIAN_POINT('Ctrl Pts',(0.0560316428543165,1.78234266440841,
7.38421986580922));
#60371=CARTESIAN_POINT('Ctrl Pts',(0.0739291284730726,1.78628334695308,
7.38529947857499));
#60372=CARTESIAN_POINT('Ctrl Pts',(0.0785361515495423,1.78740485622242,
7.38558165384037));
#60373=CARTESIAN_POINT('Ctrl Pts',(0.0849010629692599,1.78910388170572,
7.38597822965838));
#60374=CARTESIAN_POINT('Ctrl Pts',(0.0866813775760356,1.78959554541157,
7.38608989283481));
#60375=CARTESIAN_POINT('Ctrl Pts',(0.0897453161601677,1.79047011792881,
7.38628338747504));
#60376=CARTESIAN_POINT('Ctrl Pts',(0.0910309725165503,1.79084578019089,
7.38636498328308));
#60377=CARTESIAN_POINT('Ctrl Pts',(0.0928494995379397,1.79138947169846,
7.38648098400849));
#60378=CARTESIAN_POINT('Ctrl Pts',(0.0933843446142382,1.79155089249964,
7.38651517287877));
#60379=CARTESIAN_POINT('Ctrl Pts',(0.0942704159147848,1.79182083223603,
7.38657193363579));
#60380=CARTESIAN_POINT('Ctrl Pts',(0.0946218825030613,1.79192856330026,
7.38659447968531));
#60381=CARTESIAN_POINT('Ctrl Pts',(0.0953548527065584,1.79215460498317,
7.38664156467746));
#60382=CARTESIAN_POINT('Ctrl Pts',(0.0957363220272728,1.79227302391541,
7.38666610713915));
#60383=CARTESIAN_POINT('Ctrl Pts',(0.0965733761510479,1.79253457643338,
7.38672004300031));
#60384=CARTESIAN_POINT('Ctrl Pts',(0.097028864352117,1.79267801388635,7.3867494463382));
#60385=CARTESIAN_POINT('Ctrl Pts',(0.0986022926192273,1.79317734769137,
7.38685120380645));
#60386=CARTESIAN_POINT('Ctrl Pts',(0.0997185968205904,1.79353833278979,
7.38692372514454));
#60387=CARTESIAN_POINT('Ctrl Pts',(0.12516221009088,1.80191990226256,7.38858426778419));
#60388=CARTESIAN_POINT('Ctrl Pts',(0.148443742406816,1.8128045452929,7.39027366115344));
#60389=CARTESIAN_POINT('Ctrl Pts',(0.183464851425994,1.83458278099478,7.39305887087783));
#60390=CARTESIAN_POINT('Ctrl Pts',(0.196124457419223,1.84379524243491,7.39412327804836));
#60391=CARTESIAN_POINT('Ctrl Pts',(0.214491405840648,1.85932300563061,7.39571576287857));
#60392=CARTESIAN_POINT('Ctrl Pts',(0.22070265019479,1.8650056453983,7.39626363823343));
#60393=CARTESIAN_POINT('Ctrl Pts',(0.227618231980305,1.87184908418765,7.39687779162366));
#60394=CARTESIAN_POINT('Ctrl Pts',(0.228545970845989,1.8727784357365,7.39696027073779));
#60395=CARTESIAN_POINT('Ctrl Pts',(0.229740926924612,1.87399019228399,7.39706659086489));
#60396=CARTESIAN_POINT('Ctrl Pts',(0.230013332592185,1.87426742919633,7.39709083365577));
#60397=CARTESIAN_POINT('Ctrl Pts',(0.230453363141809,1.87471688745468,7.39713000252832));
#60398=CARTESIAN_POINT('Ctrl Pts',(0.230621297046185,1.87488880363003,7.39714495295291));
#60399=CARTESIAN_POINT('Ctrl Pts',(0.230942943047865,1.87521881461686,7.39717359116464));
#60400=CARTESIAN_POINT('Ctrl Pts',(0.231096684701733,1.87537687882599,7.39718728125961));
#60401=CARTESIAN_POINT('Ctrl Pts',(0.231449791351423,1.87574065956226,7.39721872772094));
#60402=CARTESIAN_POINT('Ctrl Pts',(0.231649044939236,1.87594648480675,7.39723647529021));
#60403=CARTESIAN_POINT('Ctrl Pts',(0.232264966565486,1.87658442028152,7.39729134510506));
#60404=CARTESIAN_POINT('Ctrl Pts',(0.232680704992113,1.87701743231214,7.39732839497164));
#60405=CARTESIAN_POINT('Ctrl Pts',(0.236093581268659,1.88059204900149,7.39763268164981));
#60406=CARTESIAN_POINT('Ctrl Pts',(0.239028335869683,1.88379295285257,7.39789521493852));
#60407=CARTESIAN_POINT('Ctrl Pts',(0.24260398846304,1.88785471245867,7.39821766138594));
#60408=CARTESIAN_POINT('Ctrl Pts',(0.243306313639451,1.88866056675538,7.39828112420555));
#60409=CARTESIAN_POINT('Ctrl Pts',(0.245074101451898,1.89070943493942,7.39844123404827));
#60410=CARTESIAN_POINT('Ctrl Pts',(0.246134136028889,1.8919571123703,7.3985375876602));
#60411=CARTESIAN_POINT('Ctrl Pts',(0.264412197142547,1.91380593389285,7.40020614956665));
#60412=CARTESIAN_POINT('Ctrl Pts',(0.279000303184931,1.93647274494139,7.40165739095483));
#60413=CARTESIAN_POINT('Ctrl Pts',(0.297124752025477,1.97428097870768,7.40403862586409));
#60414=CARTESIAN_POINT('Ctrl Pts',(0.302678281025226,1.98831221643822,7.40491322212158));
#60415=CARTESIAN_POINT('Ctrl Pts',(0.307710577184216,2.00419856029788,7.40591861884607));
#60416=CARTESIAN_POINT('Ctrl Pts',(0.308180528578827,2.0057212811669,7.40601512261245));
#60417=CARTESIAN_POINT('Ctrl Pts',(0.308876459743618,2.00803702886921,7.40616211532462));
#60418=CARTESIAN_POINT('Ctrl Pts',(0.309110725779828,2.00882755552749,7.40621233470371));
#60419=CARTESIAN_POINT('Ctrl Pts',(0.309536888972073,2.01028615972665,7.40630507303871));
#60420=CARTESIAN_POINT('Ctrl Pts',(0.309729663776775,2.01095397742793,7.40634756318936));
#60421=CARTESIAN_POINT('Ctrl Pts',(0.310037633506612,2.01203395780428,7.40641632791855));
#60422=CARTESIAN_POINT('Ctrl Pts',(0.310154171274403,2.0124457379207,7.40644255871901));
#60423=CARTESIAN_POINT('Ctrl Pts',(0.310376138366452,2.01323605149106,7.4064929256906));
#60424=CARTESIAN_POINT('Ctrl Pts',(0.31048169633051,2.01361454827525,7.40651705762646));
#60425=CARTESIAN_POINT('Ctrl Pts',(0.310719982902284,2.01447504579175,7.40657194422518));
#60426=CARTESIAN_POINT('Ctrl Pts',(0.310852282445289,2.01495716337526,7.40660271276375));
#60427=CARTESIAN_POINT('Ctrl Pts',(0.311240896900857,2.01638635062781,7.406693973734));
#60428=CARTESIAN_POINT('Ctrl Pts',(0.311494007582491,2.01733427874208,7.40675456991313));
#60429=CARTESIAN_POINT('Ctrl Pts',(0.313191139698531,2.02380870742002,7.40716891497506));
#60430=CARTESIAN_POINT('Ctrl Pts',(0.314492261299111,2.02937129556919,7.40752725518391));
#60431=CARTESIAN_POINT('Ctrl Pts',(0.322073452769963,2.06616645044225,7.40991501907185));
#60432=CARTESIAN_POINT('Ctrl Pts',(0.323839053401613,2.09814453984804,7.41209741555548));
#60433=CARTESIAN_POINT('Ctrl Pts',(0.319774007427222,2.14184258940461,7.41504018461208));
#60434=CARTESIAN_POINT('Ctrl Pts',(0.317987028940872,2.15376369778721,7.41583561941497));
#60435=CARTESIAN_POINT('Ctrl Pts',(0.315208850233183,2.16713532403285,7.41670001334998));
#60436=CARTESIAN_POINT('Ctrl Pts',(0.314869302333308,2.16871021542138,7.4168013714739));
#60437=CARTESIAN_POINT('Ctrl Pts',(0.314426803136517,2.17069042209416,7.41692819173013));
#60438=CARTESIAN_POINT('Ctrl Pts',(0.314334861747314,2.17109813641367,7.41695426999124));
#60439=CARTESIAN_POINT('Ctrl Pts',(0.314187348941903,2.1717464029843,7.41699568009487));
#60440=CARTESIAN_POINT('Ctrl Pts',(0.314132294206982,2.17198707046107,7.41701104156667));
#60441=CARTESIAN_POINT('Ctrl Pts',(0.314027899205345,2.17244102477784,7.41703999400814));
#60442=CARTESIAN_POINT('Ctrl Pts',(0.313978618571107,2.17265432286305,7.41705358824294));
#60443=CARTESIAN_POINT('Ctrl Pts',(0.313866032424949,2.17313936811134,7.41708448032186));
#60444=CARTESIAN_POINT('Ctrl Pts',(0.313802591432197,2.17341108288094,7.41710177021502));
#60445=CARTESIAN_POINT('Ctrl Pts',(0.313608795213759,2.17423626137171,7.41715423264765));
#60446=CARTESIAN_POINT('Ctrl Pts',(0.313477327155475,2.17478946656445,7.4171893412582));
#60447=CARTESIAN_POINT('Ctrl Pts',(0.312535906159033,2.17870478227281,7.41743739826131));
#60448=CARTESIAN_POINT('Ctrl Pts',(0.311673307312672,2.18205417262405,7.41764738195327));
#60449=CARTESIAN_POINT('Ctrl Pts',(0.303264346761115,2.21265690653161,7.41955097657269));
#60450=CARTESIAN_POINT('Ctrl Pts',(0.292214438948206,2.23882383662416,7.42107755472311));
#60451=CARTESIAN_POINT('Ctrl Pts',(0.26923611032039,2.27794655281542,7.42363947516003));
#60452=CARTESIAN_POINT('Ctrl Pts',(0.259427175492304,2.29196479429241,7.42462390033303));
#60453=CARTESIAN_POINT('Ctrl Pts',(0.247466119363986,2.30645730495474,7.42575643688147));
#60454=CARTESIAN_POINT('Ctrl Pts',(0.246367322318854,2.30776727683412,7.42585989821044));
#60455=CARTESIAN_POINT('Ctrl Pts',(0.244695015922741,2.3097290594753,7.42601652744217));
#60456=CARTESIAN_POINT('Ctrl Pts',(0.244129199863142,2.31038741159343,7.42606938097697));
#60457=CARTESIAN_POINT('Ctrl Pts',(0.24321003398437,2.31144820121549,7.42615501812706));
#60458=CARTESIAN_POINT('Ctrl Pts',(0.242858326274361,2.31185206107502,7.42618773385038));
#60459=CARTESIAN_POINT('Ctrl Pts',(0.242182203720644,2.31262454457155,7.42625052759352));
#60460=CARTESIAN_POINT('Ctrl Pts',(0.241857949567405,2.31299330735982,7.42628059888398));
#60461=CARTESIAN_POINT('Ctrl Pts',(0.241277497750128,2.31365040013009,7.4263343535673));
#60462=CARTESIAN_POINT('Ctrl Pts',(0.24102162234473,2.31393901457315,7.42635802345106));
#60463=CARTESIAN_POINT('Ctrl Pts',(0.240512675459503,2.31451100885014,7.42640505207505));
#60464=CARTESIAN_POINT('Ctrl Pts',(0.240259619718885,2.31479440194104,7.42642841013404));
#60465=CARTESIAN_POINT('Ctrl Pts',(0.23964396653593,2.31548141291726,7.42648517660794));
#60466=CARTESIAN_POINT('Ctrl Pts',(0.239280850744737,2.3158845628363,7.42651860685005));
#60467=CARTESIAN_POINT('Ctrl Pts',(0.237916682786574,2.31739146268785,7.42664401033311));
#60468=CARTESIAN_POINT('Ctrl Pts',(0.236909009562826,2.31848916921896,7.42673626390827));
#60469=CARTESIAN_POINT('Ctrl Pts',(0.218762569928013,2.33798381975717,7.42839103011352));
#60470=CARTESIAN_POINT('Ctrl Pts',(0.199540319895566,2.35431575926016,7.4300506923714));
#60471=CARTESIAN_POINT('Ctrl Pts',(0.165499797724477,2.37698283545666,7.43281276530607));
#60472=CARTESIAN_POINT('Ctrl Pts',(0.151755063936069,2.38474568469427,7.43388594890604));
#60473=CARTESIAN_POINT('Ctrl Pts',(0.131738306342143,2.3941882692157,7.43535050661704));
#60474=CARTESIAN_POINT('Ctrl Pts',(0.125899863970404,2.39673381125721,7.43576648652181));
#60475=CARTESIAN_POINT('Ctrl Pts',(0.117206728503596,2.40022116530097,7.43636578380568));
#60476=CARTESIAN_POINT('Ctrl Pts',(0.114408445075333,2.40129864683227,7.43655570224769));
#60477=CARTESIAN_POINT('Ctrl Pts',(0.111121139626074,2.40251202212807,7.43677499326239));
#60478=CARTESIAN_POINT('Ctrl Pts',(0.110646452993243,2.40268596540325,7.43680656648272));
#60479=CARTESIAN_POINT('Ctrl Pts',(0.109921364433264,2.40294973185579,7.43685465185827));
#60480=CARTESIAN_POINT('Ctrl Pts',(0.109671260088295,2.40304036216689,7.43687121199087));
#60481=CARTESIAN_POINT('Ctrl Pts',(0.109235939529656,2.40319749977158,7.43689999038019));
#60482=CARTESIAN_POINT('Ctrl Pts',(0.109050775118479,2.4032641469073,7.43691221701533));
#60483=CARTESIAN_POINT('Ctrl Pts',(0.108631762250848,2.40341453088364,7.43693985255746));
#60484=CARTESIAN_POINT('Ctrl Pts',(0.10839787845273,2.40349816682973,7.43695525534996));
#60485=CARTESIAN_POINT('Ctrl Pts',(0.107763847112237,2.40372406759573,7.43699694944475));
#60486=CARTESIAN_POINT('Ctrl Pts',(0.107363512904892,2.40386581262615,7.43702320970577));
#60487=CARTESIAN_POINT('Ctrl Pts',(0.105564184375826,2.40449889521849,7.43714094762509));
#60488=CARTESIAN_POINT('Ctrl Pts',(0.104162060550437,2.40498137574661,7.43723190667217));
#60489=CARTESIAN_POINT('Ctrl Pts',(0.072038281751541,2.41578800860379,7.43929895379844));
#60490=CARTESIAN_POINT('Ctrl Pts',(0.0399310982912344,2.42143106456642,
7.44102682020046));
#60491=CARTESIAN_POINT('Ctrl Pts',(-0.00785175016274551,2.42254589197846,
7.44373876415127));
#60492=CARTESIAN_POINT('Ctrl Pts',(-0.0232245135824139,2.4218043386661,
7.44462980949059));
#60493=CARTESIAN_POINT('Ctrl Pts',(-0.0409110140993787,2.41967708374758,
7.44570439295655));
#60494=CARTESIAN_POINT('Ctrl Pts',(-0.0433341118570751,2.41935764150812,
7.44585266583824));
#60495=CARTESIAN_POINT('Ctrl Pts',(-0.0464530958618366,2.41891030919293,
7.44604495344453));
#60496=CARTESIAN_POINT('Ctrl Pts',(-0.0471525635412023,2.41880763975104,
7.4460881691795));
#60497=CARTESIAN_POINT('Ctrl Pts',(-0.0482807359620205,2.41863825005176,
7.44615802408864));
#60498=CARTESIAN_POINT('Ctrl Pts',(-0.0487096563519322,2.41857296375595,
7.4461846177949));
#60499=CARTESIAN_POINT('Ctrl Pts',(-0.0495274213639583,2.41844680099558,
7.44623538875211));
#60500=CARTESIAN_POINT('Ctrl Pts',(-0.049916289143771,2.41838607791047,
7.44625956109785));
#60501=CARTESIAN_POINT('Ctrl Pts',(-0.0508041250859461,2.41824577263861,
7.44631481750648));
#60502=CARTESIAN_POINT('Ctrl Pts',(-0.05130301836948,2.41816572918785,7.44634591615278));
#60503=CARTESIAN_POINT('Ctrl Pts',(-0.0528293236139818,2.41791716243199,
7.44644120979776));
#60504=CARTESIAN_POINT('Ctrl Pts',(-0.0538561013263279,2.41774483459452,
7.44650552542752));
#60505=CARTESIAN_POINT('Ctrl Pts',(-0.0614607330363169,2.41643060226578,
7.44698344451386));
#60506=CARTESIAN_POINT('Ctrl Pts',(-0.0680020980278876,2.41508959309327,
7.44740335318742));
#60507=CARTESIAN_POINT('Ctrl Pts',(-0.0763225056268109,2.41311271514275,
7.44794939112691));
#60508=CARTESIAN_POINT('Ctrl Pts',(-0.0781444245685719,2.41266299097908,
7.44806969422149));
#60509=CARTESIAN_POINT('Ctrl Pts',(-0.0817246995185879,2.41174598472427,
7.44830756008916));
#60510=CARTESIAN_POINT('Ctrl Pts',(-0.083483234745857,2.41127967298985,
7.44842509022123));
#60511=CARTESIAN_POINT('Ctrl Pts',(-0.112843499242343,2.40322750602925,
7.45039899757463));
#60512=CARTESIAN_POINT('Ctrl Pts',(-0.139315655900175,2.39201244060027,
7.45236792164115));
#60513=CARTESIAN_POINT('Ctrl Pts',(-0.173115774615028,2.37203930138863,
7.45498959912348));
#60514=CARTESIAN_POINT('Ctrl Pts',(-0.182005952877563,2.36617350799146,
7.45568883829962));
#60515=CARTESIAN_POINT('Ctrl Pts',(-0.191805300488816,2.35898681879531,
7.45645727735599));
#60516=CARTESIAN_POINT('Ctrl Pts',(-0.193014002410747,2.35808727339693,
7.45655201516556));
#60517=CARTESIAN_POINT('Ctrl Pts',(-0.194542227019738,2.356933190266,7.45667169193729));
#60518=CARTESIAN_POINT('Ctrl Pts',(-0.194867609153495,2.35668649606329,
7.45669716682055));
#60519=CARTESIAN_POINT('Ctrl Pts',(-0.195387258846602,2.35629095691814,
7.45673784035899));
#60520=CARTESIAN_POINT('Ctrl Pts',(-0.195581825884623,2.35614250897147,
7.45675306685999));
#60521=CARTESIAN_POINT('Ctrl Pts',(-0.195950449892836,2.35586059665337,
7.4567819097855));
#60522=CARTESIAN_POINT('Ctrl Pts',(-0.196124538258917,2.35572717733169,
7.45679552914569));
#60523=CARTESIAN_POINT('Ctrl Pts',(-0.196522703474639,2.35542138235988,
7.45682667386535));
#60524=CARTESIAN_POINT('Ctrl Pts',(-0.19674668946289,2.35524888978107,7.45684419078004));
#60525=CARTESIAN_POINT('Ctrl Pts',(-0.197435160396986,2.35471725068142,
7.45689802344901));
#60526=CARTESIAN_POINT('Ctrl Pts',(-0.197898894374068,2.35435712683947,
7.45693427026667));
#60527=CARTESIAN_POINT('Ctrl Pts',(-0.201395177642832,2.35162665380411,
7.4572074714067));
#60528=CARTESIAN_POINT('Ctrl Pts',(-0.204386188379017,2.34920328985304,
7.45744074210153));
#60529=CARTESIAN_POINT('Ctrl Pts',(-0.228711538102684,2.32876184085922,
7.45934090498066));
#60530=CARTESIAN_POINT('Ctrl Pts',(-0.247667265827999,2.30809212563943,
7.46084937356339));
#60531=CARTESIAN_POINT('Ctrl Pts',(-0.271443359884391,2.27424160842031,
7.46318549050736));
#60532=CARTESIAN_POINT('Ctrl Pts',(-0.278468973331682,2.26277779984589,
7.4639561390373));
#60533=CARTESIAN_POINT('Ctrl Pts',(-0.287482427280929,2.24576991684566,
7.46509724704549));
#60534=CARTESIAN_POINT('Ctrl Pts',(-0.290066573691369,2.24055742919544,
7.46544656587996));
#60535=CARTESIAN_POINT('Ctrl Pts',(-0.292896224973288,2.23443895201392,
7.46585718806442));
#60536=CARTESIAN_POINT('Ctrl Pts',(-0.293280698861437,2.23359813647496,
7.46591362865117));
#60537=CARTESIAN_POINT('Ctrl Pts',(-0.293859878024684,2.2323169661157,7.46599965084002));
#60538=CARTESIAN_POINT('Ctrl Pts',(-0.294057225576128,2.23187780524878,
7.46602914158545));
#60539=CARTESIAN_POINT('Ctrl Pts',(-0.294413147627628,2.23108099476309,
7.46608265725775));
#60540=CARTESIAN_POINT('Ctrl Pts',(-0.294572056674591,2.23072349486014,
7.46610667065653));
#60541=CARTESIAN_POINT('Ctrl Pts',(-0.294911848864742,2.22995529392316,
7.46615827754153));
#60542=CARTESIAN_POINT('Ctrl Pts',(-0.295092525739823,2.22954450304324,
7.46618587802615));
#60543=CARTESIAN_POINT('Ctrl Pts',(-0.295574530191809,2.22844236639545,
7.46625994057599));
#60544=CARTESIAN_POINT('Ctrl Pts',(-0.295874288674136,2.2277503411717,7.46630645610841));
#60545=CARTESIAN_POINT('Ctrl Pts',(-0.297223172016263,2.22460608236259,
7.4665178625672));
#60546=CARTESIAN_POINT('Ctrl Pts',(-0.298244233745826,2.222141991528,7.46668370469839));
#60547=CARTESIAN_POINT('Ctrl Pts',(-0.299475739143415,2.21906250099698,
7.46689122679276));
#60548=CARTESIAN_POINT('Ctrl Pts',(-0.299715084313064,2.21845870885847,
7.46693192773647));
#60549=CARTESIAN_POINT('Ctrl Pts',(-0.311966751852016,2.18727679492721,
7.46903452546429));
#60550=CARTESIAN_POINT('Ctrl Pts',(-0.319232292372442,2.15504722634259,
7.47127041119508));
#60551=CARTESIAN_POINT('Ctrl Pts',(-0.322020786084112,2.11482461997514,
7.47398440293776));
#60552=CARTESIAN_POINT('Ctrl Pts',(-0.322278183387271,2.10734437814288,
7.47448450862746));
#60553=CARTESIAN_POINT('Ctrl Pts',(-0.32227471063135,2.0992569169113,7.47501614503034));
#60554=CARTESIAN_POINT('Ctrl Pts',(-0.322272749041375,2.09865221691015,
7.47505584039782));
#60555=CARTESIAN_POINT('Ctrl Pts',(-0.322259178914493,2.09641237956066,
7.47520266167197));
#60556=CARTESIAN_POINT('Ctrl Pts',(-0.322236827622263,2.09477730615424,
7.4753094217966));
#60557=CARTESIAN_POINT('Ctrl Pts',(-0.322179229564705,2.09207106305374,
7.47548535647127));
#60558=CARTESIAN_POINT('Ctrl Pts',(-0.322151082943541,2.09099978769373,
7.47555480197062));
#60559=CARTESIAN_POINT('Ctrl Pts',(-0.32198193068935,2.08558969215906,7.47590444358153));
#60560=CARTESIAN_POINT('Ctrl Pts',(-0.321758603911821,2.08125363840353,
7.47618120513538));
#60561=CARTESIAN_POINT('Ctrl Pts',(-0.3214047372209,2.07632446825163,7.47649088283619));
#60562=CARTESIAN_POINT('Ctrl Pts',(-0.321360083558188,2.07572588578635,
7.47652840594408));
#60563=CARTESIAN_POINT('Ctrl Pts',(-0.32129164870998,2.07484181733002,7.4765836988531));
#60564=CARTESIAN_POINT('Ctrl Pts',(-0.321269159140845,2.07455623706101,
7.47660154061435));
#60565=CARTESIAN_POINT('Ctrl Pts',(-0.321228684833388,2.07405089047564,
7.4766330774373));
#60566=CARTESIAN_POINT('Ctrl Pts',(-0.321210855306483,2.07383111237841,
7.47664678126998));
#60567=CARTESIAN_POINT('Ctrl Pts',(-0.321173121353051,2.07337182876216,
7.47667539435594));
#60568=CARTESIAN_POINT('Ctrl Pts',(-0.321153174622573,2.07313232771745,
7.4766903011586));
#60569=CARTESIAN_POINT('Ctrl Pts',(-0.321100267017823,2.07250554199368,
7.47672927694563));
#60570=CARTESIAN_POINT('Ctrl Pts',(-0.321066873260514,2.07211829276273,
7.47675332148254));
#60571=CARTESIAN_POINT('Ctrl Pts',(-0.320917583532146,2.07042289957278,
7.47685843545395));
#60572=CARTESIAN_POINT('Ctrl Pts',(-0.320794390675278,2.06911538668003,
7.4769390993658));
#60573=CARTESIAN_POINT('Ctrl Pts',(-0.319822549819421,2.05943472772793,
7.4775335894894));
#60574=CARTESIAN_POINT('Ctrl Pts',(-0.318654112941115,2.0510961313201,7.47803051485388));
#60575=CARTESIAN_POINT('Ctrl Pts',(-0.314329149005187,2.027110162878,7.4794403800165));
#60576=CARTESIAN_POINT('Ctrl Pts',(-0.310335574272976,2.01163915384284,
7.48032616214036));
#60577=CARTESIAN_POINT('Ctrl Pts',(-0.297284708618472,1.97314335527495,
7.48259947086348));
#60578=CARTESIAN_POINT('Ctrl Pts',(-0.286697875668781,1.95075226935366,
7.4839945729806));
#60579=CARTESIAN_POINT('Ctrl Pts',(-0.272832694084156,1.92846005943784,
7.48558619437701));
#60580=CARTESIAN_POINT('Ctrl Pts',(-0.271995563643761,1.92713576601158,
7.48568153045452));
#60581=CARTESIAN_POINT('Ctrl Pts',(-0.270849335729347,1.92535143859102,
7.48581107009117));
#60582=CARTESIAN_POINT('Ctrl Pts',(-0.270548649270705,1.92488600558778,
7.48584496064615));
#60583=CARTESIAN_POINT('Ctrl Pts',(-0.270038034241506,1.92410007824352,
7.48590235975522));
#60584=CARTESIAN_POINT('Ctrl Pts',(-0.269828731039281,1.92377917740904,
7.48592584491846));
#60585=CARTESIAN_POINT('Ctrl Pts',(-0.269425268453555,1.92316299812767,
7.48597103399035));
#60586=CARTESIAN_POINT('Ctrl Pts',(-0.269231194518096,1.92286766413426,
7.48599273467583));
#60587=CARTESIAN_POINT('Ctrl Pts',(-0.268773272006708,1.92217330707748,
7.48604385334323));
#60588=CARTESIAN_POINT('Ctrl Pts',(-0.268509020519237,1.92177455188203,
7.48607328643624));
#60589=CARTESIAN_POINT('Ctrl Pts',(-0.267739590108587,1.9206190775345,7.48615879861507));
#60590=CARTESIAN_POINT('Ctrl Pts',(-0.267232096282438,1.91986391215137,
7.48621496489547));
#60591=CARTESIAN_POINT('Ctrl Pts',(-0.263653355716719,1.91458705017719,
7.48660941580433));
#60592=CARTESIAN_POINT('Ctrl Pts',(-0.26047086313411,1.91014221773362,7.48695191335197));
#60593=CARTESIAN_POINT('Ctrl Pts',(-0.250142239746943,1.89646549082929,
7.48803936477488));
#60594=CARTESIAN_POINT('Ctrl Pts',(-0.24260730075123,1.88754039879937,7.48879918587341));
#60595=CARTESIAN_POINT('Ctrl Pts',(-0.213860096148085,1.85701727220393,
7.49158026631161));
#60596=CARTESIAN_POINT('Ctrl Pts',(-0.190117817070804,1.83802321876545,
7.49368525504334));
#60597=CARTESIAN_POINT('Ctrl Pts',(-0.160910778273966,1.82074666665782,
7.49586774973772));
#60598=CARTESIAN_POINT('Ctrl Pts',(-0.157713210773484,1.81892839212649,
7.49610154944893));
#60599=CARTESIAN_POINT('Ctrl Pts',(-0.153976653499718,1.81688747575884,
7.49636825370207));
#60600=CARTESIAN_POINT('Ctrl Pts',(-0.153467502293264,1.81661115590509,
7.49640445726968));
#60601=CARTESIAN_POINT('Ctrl Pts',(-0.152710134902788,1.81620276715513,
7.49645810241774));
#60602=CARTESIAN_POINT('Ctrl Pts',(-0.152462490044769,1.81606964973214,
7.49647561043107));
#60603=CARTESIAN_POINT('Ctrl Pts',(-0.152021502629277,1.81583334750356,
7.49650672838327));
#60604=CARTESIAN_POINT('Ctrl Pts',(-0.151828229115562,1.81573003588593,
7.49652034643599));
#60605=CARTESIAN_POINT('Ctrl Pts',(-0.151418121047094,1.81551135599188,
7.49654919982685));
#60606=CARTESIAN_POINT('Ctrl Pts',(-0.151201260561406,1.81539603875452,
7.49656443187123));
#60607=CARTESIAN_POINT('Ctrl Pts',(-0.150620038808862,1.81508782142063,
7.49660518909658));
#60608=CARTESIAN_POINT('Ctrl Pts',(-0.15025543733087,1.81489537157278,7.4966306855814));
#60609=CARTESIAN_POINT('Ctrl Pts',(-0.148519522585434,1.81398334784071,
7.49675174698456));
#60610=CARTESIAN_POINT('Ctrl Pts',(-0.147143373848165,1.81327294920144,
7.49684673866733));
#60611=CARTESIAN_POINT('Ctrl Pts',(-0.135788546076031,1.80751461458152,
7.49762294409451));
#60612=CARTESIAN_POINT('Ctrl Pts',(-0.125557267455462,1.80297868711241,
7.49827449733968));
#60613=CARTESIAN_POINT('Ctrl Pts',(-0.0824529427827286,1.7864954440634,
7.50090808862388));
#60614=CARTESIAN_POINT('Ctrl Pts',(-0.0479838896690525,1.77940478345643,
7.50278448911669));
#60615=CARTESIAN_POINT('Ctrl Pts',(-0.00928726900057291,1.77783686879122,
7.50510314487613));
#60616=CARTESIAN_POINT('Ctrl Pts',(-0.00552501174200246,1.77775039348909,
7.50533038893702));
#60617=CARTESIAN_POINT('Ctrl Pts',(-0.000983001639697015,1.77772555712258,
7.50560719164472));
#60618=CARTESIAN_POINT('Ctrl Pts',(-0.000203775976239631,1.77772412240012,
7.50565476701871));
#60619=CARTESIAN_POINT('Ctrl Pts',(0.00107203310947944,1.77772640043957,
7.50573280663182));
#60620=CARTESIAN_POINT('Ctrl Pts',(0.00156861940101777,1.7777284349226,
7.50576321827106));
#60621=CARTESIAN_POINT('Ctrl Pts',(0.00245775825731967,1.77773413280312,
7.5058177357273));
#60622=CARTESIAN_POINT('Ctrl Pts',(0.00285031338416871,1.77773736572904,
7.50584182801245));
#60623=CARTESIAN_POINT('Ctrl Pts',(0.00368154973764707,1.77774573038595,
7.50589289218606));
#60624=CARTESIAN_POINT('Ctrl Pts',(0.0041202280146117,1.77775104063623,
7.50591986961889));
#60625=CARTESIAN_POINT('Ctrl Pts',(0.00528744962038929,1.77776755376991,
7.50599172746481));
#60626=CARTESIAN_POINT('Ctrl Pts',(0.00601596499620415,1.77778033163982,
7.5060366571325));
#60627=CARTESIAN_POINT('Ctrl Pts',(0.00940372142326487,1.77785124461056,
7.50624596699108));
#60628=CARTESIAN_POINT('Ctrl Pts',(0.0120621591330603,1.77793982827692,
7.50641129822334));
#60629=CARTESIAN_POINT('Ctrl Pts',(0.0325425236953344,1.77887619666149,
7.50769367321661));
#60630=CARTESIAN_POINT('Ctrl Pts',(0.0502644214661067,1.78116961752135,
7.50885664924497));
#60631=CARTESIAN_POINT('Ctrl Pts',(0.084688649647664,1.78856648065074,7.511210923269));
#60632=CARTESIAN_POINT('Ctrl Pts',(0.10135050723683,1.79358353913651,7.51239655913679));
#60633=CARTESIAN_POINT('Ctrl Pts',(0.126732013946108,1.80352417784261,7.51422485677772));
#60634=CARTESIAN_POINT('Ctrl Pts',(0.13576764884014,1.80755154919271,7.5148799230681));
#60635=CARTESIAN_POINT('Ctrl Pts',(0.147830730121591,1.81360816494451,7.51574766435115));
#60636=CARTESIAN_POINT('Ctrl Pts',(0.151029679621281,1.81528216329809,7.51597707884198));
#60637=CARTESIAN_POINT('Ctrl Pts',(0.154705915595677,1.81728532533884,7.51623932295906));
#60638=CARTESIAN_POINT('Ctrl Pts',(0.155211110196343,1.8175623628606,7.51627532994188));
#60639=CARTESIAN_POINT('Ctrl Pts',(0.155961175529324,1.81797630232479,7.51632874037461));
#60640=CARTESIAN_POINT('Ctrl Pts',(0.156206611343792,1.81811216965465,7.5163462094178));
#60641=CARTESIAN_POINT('Ctrl Pts',(0.15664340465935,1.81835471351617,7.51637728397507));
#60642=CARTESIAN_POINT('Ctrl Pts',(0.156834830674453,1.81846126463625,7.5163908975176));
#60643=CARTESIAN_POINT('Ctrl Pts',(0.157240953385629,1.81868786249397,7.516419768848));
#60644=CARTESIAN_POINT('Ctrl Pts',(0.157455620722199,1.81880795951202,7.51643502328626));
#60645=CARTESIAN_POINT('Ctrl Pts',(0.158023893143474,1.81912673795696,7.5164753890674));
#60646=CARTESIAN_POINT('Ctrl Pts',(0.15837726244995,1.81932584216203,7.51650047319099));
#60647=CARTESIAN_POINT('Ctrl Pts',(0.160025257669488,1.82025850025271,7.51661738415348));
#60648=CARTESIAN_POINT('Ctrl Pts',(0.161315196117022,1.82100036294766,7.51670868363776));
#60649=CARTESIAN_POINT('Ctrl Pts',(0.171640689189943,1.82703426015247,7.51743818624322));
#60650=CARTESIAN_POINT('Ctrl Pts',(0.180419584255306,1.83275546090998,7.51805034015976));
#60651=CARTESIAN_POINT('Ctrl Pts',(0.209374302340331,1.85370369233939,7.52009621756664));
#60652=CARTESIAN_POINT('Ctrl Pts',(0.228031324597575,1.87086839377805,7.52146865531097));
#60653=CARTESIAN_POINT('Ctrl Pts',(0.247034115806452,1.8929962827731,7.52314091686641));
#60654=CARTESIAN_POINT('Ctrl Pts',(0.249521611401101,1.8960015752848,7.52336605420259));
#60655=CARTESIAN_POINT('Ctrl Pts',(0.258081153194738,1.90673371152912,7.52416471678739));
#60656=CARTESIAN_POINT('Ctrl Pts',(0.263853298654219,1.91469175103825,7.52474768380718));
#60657=CARTESIAN_POINT('Ctrl Pts',(0.269824951733037,1.92377072868257,7.52540846569277));
#60658=CARTESIAN_POINT('Ctrl Pts',(0.270393137505785,1.92464375746289,7.52547196104456));
#60659=CARTESIAN_POINT('Ctrl Pts',(0.271236568907388,1.92595355270691,7.52556716143676));
#60660=CARTESIAN_POINT('Ctrl Pts',(0.271515017542906,1.92638825681486,7.52559874722855));
#60661=CARTESIAN_POINT('Ctrl Pts',(0.27199275710952,1.9271380472721,7.52565321096264));
#60662=CARTESIAN_POINT('Ctrl Pts',(0.272192548569439,1.92745281479456,7.52567607028625));
#60663=CARTESIAN_POINT('Ctrl Pts',(0.272603746965568,1.92810314122026,7.52572328900514));
#60664=CARTESIAN_POINT('Ctrl Pts',(0.2728150815016,1.92843874498858,7.52574765102988));
#60665=CARTESIAN_POINT('Ctrl Pts',(0.273305525353882,1.92922077808542,7.52580440798869));
#60666=CARTESIAN_POINT('Ctrl Pts',(0.27358416064105,1.92966750202092,7.52583682034686));
#60667=CARTESIAN_POINT('Ctrl Pts',(0.274450590248883,1.93106422186664,7.52593813314234));
#60668=CARTESIAN_POINT('Ctrl Pts',(0.275034535720964,1.93201658494995,7.52600717489425));
#60669=CARTESIAN_POINT('Ctrl Pts',(0.284427550475583,1.94751602871191,7.52713023977432));
#60670=CARTESIAN_POINT('Ctrl Pts',(0.292075055211723,1.96273242974542,7.52822689351689));
#60671=CARTESIAN_POINT('Ctrl Pts',(0.307202067195499,1.9998880943741,7.53088937974676));
#60672=CARTESIAN_POINT('Ctrl Pts',(0.313589000834757,2.02217110125456,7.53247717853517));
#60673=CARTESIAN_POINT('Ctrl Pts',(0.319302345149324,2.05512338869548,7.53470131759485));
#60674=CARTESIAN_POINT('Ctrl Pts',(0.320576932530829,2.06538240071531,7.53537590430649));
#60675=CARTESIAN_POINT('Ctrl Pts',(0.321412060614349,2.07642023987314,7.53607073093546));
#60676=CARTESIAN_POINT('Ctrl Pts',(0.321465096523879,2.07715466048096,7.53611681545331));
#60677=CARTESIAN_POINT('Ctrl Pts',(0.321535333763853,2.07817599104091,7.53618069317203));
#60678=CARTESIAN_POINT('Ctrl Pts',(0.32155466854812,2.07846274478563,7.53619860475853));
#60679=CARTESIAN_POINT('Ctrl Pts',(0.321587299286734,2.07895653068464,7.53622940815392));
#60680=CARTESIAN_POINT('Ctrl Pts',(0.321600778931337,2.07916354985433,7.53624231030758));
#60681=CARTESIAN_POINT('Ctrl Pts',(0.321628281901789,2.07959232308535,7.53626900761201));
#60682=CARTESIAN_POINT('Ctrl Pts',(0.32164227576583,2.07981407825817,7.53628280100086));
#60683=CARTESIAN_POINT('Ctrl Pts',(0.321669634198054,2.08025486858505,7.53631019091756));
#60684=CARTESIAN_POINT('Ctrl Pts',(0.321683004426913,2.08047390353233,7.53632378778158));
#60685=CARTESIAN_POINT('Ctrl Pts',(0.321727579013203,2.08121661020578,7.53636984671027));
#60686=CARTESIAN_POINT('Ctrl Pts',(0.32175772865227,2.08174034798887,7.53640224960014));
#60687=CARTESIAN_POINT('Ctrl Pts',(0.321979725704294,2.08576810659435,7.5366508674772));
#60688=CARTESIAN_POINT('Ctrl Pts',(0.322115616753237,2.08927514783993,7.53686400586497));
#60689=CARTESIAN_POINT('Ctrl Pts',(0.322389338252756,2.10149660401304,7.53759730453807));
#60690=CARTESIAN_POINT('Ctrl Pts',(0.322230998615781,2.11021441198464,7.53810369316131));
#60691=CARTESIAN_POINT('Ctrl Pts',(0.320589753881509,2.13812872716889,7.53970135358148));
#60692=CARTESIAN_POINT('Ctrl Pts',(0.317741294467233,2.15720243738382,7.54075888617756));
#60693=CARTESIAN_POINT('Ctrl Pts',(0.308724619168357,2.19440629439183,7.54291889424128));
#60694=CARTESIAN_POINT('Ctrl Pts',(0.302612471913952,2.21246763174207,7.54401698247043));
#60695=CARTESIAN_POINT('Ctrl Pts',(0.294423087930708,2.23106444239101,7.54525121573497));
#60696=CARTESIAN_POINT('Ctrl Pts',(0.293895628593212,2.23224296648183,7.54532988031166));
#60697=CARTESIAN_POINT('Ctrl Pts',(0.293149782878248,2.23388293764343,7.54543998389657));
#60698=CARTESIAN_POINT('Ctrl Pts',(0.292937355710624,2.23434709456529,7.54547121790912));
#60699=CARTESIAN_POINT('Ctrl Pts',(0.292568507967334,2.23514799901131,7.54552523702457));
#60700=CARTESIAN_POINT('Ctrl Pts',(0.292412606084908,2.23548498548457,7.5455480042089));
#60701=CARTESIAN_POINT('Ctrl Pts',(0.292088607567802,2.23618215353597,7.54559518525006));
#60702=CARTESIAN_POINT('Ctrl Pts',(0.291920426326473,2.23654229492635,7.54561960200237));
#60703=CARTESIAN_POINT('Ctrl Pts',(0.291525610134593,2.2373836861714,7.54567675000832));
#60704=CARTESIAN_POINT('Ctrl Pts',(0.291298449564691,2.23786468679899,7.54570949942449));
#60705=CARTESIAN_POINT('Ctrl Pts',(0.290576536256193,2.23938355048045,7.54581316566862));
#60706=CARTESIAN_POINT('Ctrl Pts',(0.290077423923666,2.24041932075781,7.54588423373395));
#60707=CARTESIAN_POINT('Ctrl Pts',(0.27806365433372,2.26501318432381,7.54758073827031));
#60708=CARTESIAN_POINT('Ctrl Pts',(0.26372477522185,2.28707592514208,7.54931284549977));
#60709=CARTESIAN_POINT('Ctrl Pts',(0.237958722599989,2.31778274584016,7.552021529374));
#60710=CARTESIAN_POINT('Ctrl Pts',(0.228363106651417,2.32782447021078,7.55296467383625));
#60711=CARTESIAN_POINT('Ctrl Pts',(0.210555839783719,2.34420044536229,7.55457347628032));
#60712=CARTESIAN_POINT('Ctrl Pts',(0.202629784659497,2.35081634590742,7.55524714752603));
#60713=CARTESIAN_POINT('Ctrl Pts',(0.193811942350944,2.35748523942902,7.55594111347248));
#60714=CARTESIAN_POINT('Ctrl Pts',(0.193223285908746,2.35792727527178,7.555987186263));
#60715=CARTESIAN_POINT('Ctrl Pts',(0.192402727725433,2.35853906585154,7.55605105034629));
#60716=CARTESIAN_POINT('Ctrl Pts',(0.192172111484596,2.3587105289251,7.55606895995923));
#60717=CARTESIAN_POINT('Ctrl Pts',(0.191774622924526,2.35900523674641,7.55609976086153));
#60718=CARTESIAN_POINT('Ctrl Pts',(0.1916078609171,2.35912862886071,7.55611266249185));
#60719=CARTESIAN_POINT('Ctrl Pts',(0.19126223084712,2.35938385464388,7.55613935960183));
#60720=CARTESIAN_POINT('Ctrl Pts',(0.191083345884996,2.35951566412101,7.55615315331808));
#60721=CARTESIAN_POINT('Ctrl Pts',(0.190727518720663,2.35977728420069,7.55618054416707));
#60722=CARTESIAN_POINT('Ctrl Pts',(0.190550579750975,2.35990709944379,7.55619414163548));
#60723=CARTESIAN_POINT('Ctrl Pts',(0.189950141585274,2.3603466816438,7.55624020713036));
#60724=CARTESIAN_POINT('Ctrl Pts',(0.18952601564226,2.36065559716829,7.55627261595687));
#60725=CARTESIAN_POINT('Ctrl Pts',(0.186257526027512,2.36302403238353,7.55652138921393));
#60726=CARTESIAN_POINT('Ctrl Pts',(0.183380286502167,2.36503807386133,7.55673467272383));
#60727=CARTESIAN_POINT('Ctrl Pts',(0.17644450716106,2.36972601979594,7.5572368347689));
#60728=CARTESIAN_POINT('Ctrl Pts',(0.172357203899732,2.37235599708269,7.55752325645542));
#60729=CARTESIAN_POINT('Ctrl Pts',(0.153136519010056,2.38411748056163,7.55883428460118));
#60730=CARTESIAN_POINT('Ctrl Pts',(0.137326822676004,2.39208727429661,7.55981306731855));
#60731=CARTESIAN_POINT('Ctrl Pts',(0.0984474439200499,2.40782826487582,
7.56215992032219));
#60732=CARTESIAN_POINT('Ctrl Pts',(0.0749997813105582,2.41436431793709,
7.56353438164212));
#60733=CARTESIAN_POINT('Ctrl Pts',(0.0496295329358651,2.41843387559515,
7.56509357448261));
#60734=CARTESIAN_POINT('Ctrl Pts',(0.0482150226277544,2.41865111824052,
7.56518070924072));
#60735=CARTESIAN_POINT('Ctrl Pts',(0.046271449059068,2.41893637778122,7.56530072715308));
#60736=CARTESIAN_POINT('Ctrl Pts',(0.045743579333687,2.41901251545133,7.56533335327366));
#60737=CARTESIAN_POINT('Ctrl Pts',(0.0448418510773135,2.41914029274495,
7.56538913785444));
#60738=CARTESIAN_POINT('Ctrl Pts',(0.0444680851611076,2.41919258678972,
7.5654122755827));
#60739=CARTESIAN_POINT('Ctrl Pts',(0.0437425393052485,2.41929279967722,
7.56545721954621));
#60740=CARTESIAN_POINT('Ctrl Pts',(0.0433907701738959,2.41934079403162,
7.56547902336126));
#60741=CARTESIAN_POINT('Ctrl Pts',(0.0425519838049881,2.4194538240735,7.5655310465413));
#60742=CARTESIAN_POINT('Ctrl Pts',(0.0420648968123182,2.41951832731916,
7.56556128268018));
#60743=CARTESIAN_POINT('Ctrl Pts',(0.0410552397786087,2.41964968396805,
7.56562401227821));
#60744=CARTESIAN_POINT('Ctrl Pts',(0.0405326498266147,2.4197163703455,7.5656565109245));
#60745=CARTESIAN_POINT('Ctrl Pts',(0.0375243938921511,2.42009275209141,
7.56584376423246));
#60746=CARTESIAN_POINT('Ctrl Pts',(0.0350354039826819,2.42037473367361,
7.56599939083861));
#60747=CARTESIAN_POINT('Ctrl Pts',(0.0214036742884474,2.42175834263087,
7.56685573187668));
#60748=CARTESIAN_POINT('Ctrl Pts',(0.0102137971727213,2.4223075825396,7.56757368229564));
#60749=CARTESIAN_POINT('Ctrl Pts',(-0.0191384516478878,2.4222182378215,
7.56949671374057));
#60750=CARTESIAN_POINT('Ctrl Pts',(-0.03725727032625,2.42062852560138,7.57072531935603));
#60751=CARTESIAN_POINT('Ctrl Pts',(-0.0736300222395724,2.41431169295863,
7.57322266100388));
#60752=CARTESIAN_POINT('Ctrl Pts',(-0.0918029673777799,2.4094925133396,
7.57448625858238));
#60753=CARTESIAN_POINT('Ctrl Pts',(-0.11001898473321,2.40291477039152,7.57570678831306));
#60754=CARTESIAN_POINT('Ctrl Pts',(-0.110582361969647,2.40270955775722,
7.57574448743863));
#60755=CARTESIAN_POINT('Ctrl Pts',(-0.111792221333861,2.40226503283002,
7.57582533651021));
#60756=CARTESIAN_POINT('Ctrl Pts',(-0.112438516919302,2.40202521543123,
7.57586845747046));
#60757=CARTESIAN_POINT('Ctrl Pts',(-0.113338564281399,2.40168795028591,
7.57592840908233));
#60758=CARTESIAN_POINT('Ctrl Pts',(-0.113592963878698,2.40159225464138,
7.57594534335488));
#60759=CARTESIAN_POINT('Ctrl Pts',(-0.114056599141817,2.4014171824842,7.57597618482715));
#60760=CARTESIAN_POINT('Ctrl Pts',(-0.114265873544572,2.4013379097433,7.57599009826335));
#60761=CARTESIAN_POINT('Ctrl Pts',(-0.114689445478729,2.4011769568133,7.57601824324527));
#60762=CARTESIAN_POINT('Ctrl Pts',(-0.114903738595512,2.40109526578328,
7.57603247411396));
#60763=CARTESIAN_POINT('Ctrl Pts',(-0.115333917545817,2.40093075043041,
7.57606102546662));
#60764=CARTESIAN_POINT('Ctrl Pts',(-0.115549801810046,2.40084792236865,
7.57607534571319));
#60765=CARTESIAN_POINT('Ctrl Pts',(-0.116067207556463,2.40064877082858,
7.57610964758216));
#60766=CARTESIAN_POINT('Ctrl Pts',(-0.116368644315582,2.40053222571464,
7.57612961595105));
#60767=CARTESIAN_POINT('Ctrl Pts',(-0.118475865847565,2.39971386060581,
7.57626910057416));
#60768=CARTESIAN_POINT('Ctrl Pts',(-0.120275516164659,2.39899620344473,
7.57638768050341));
#60769=CARTESIAN_POINT('Ctrl Pts',(-0.125403971786671,2.3968973008883,7.57672433096375));
#60770=CARTESIAN_POINT('Ctrl Pts',(-0.128716329096655,2.39547634832763,
7.57694022925628));
#60771=CARTESIAN_POINT('Ctrl Pts',(-0.141106012973778,2.38991345309271,
7.57774447849008));
#60772=CARTESIAN_POINT('Ctrl Pts',(-0.150013793721498,2.38540604470241,
7.57831602093122));
#60773=CARTESIAN_POINT('Ctrl Pts',(-0.166038142563203,2.37633968588535,
7.57935671772759));
#60774=CARTESIAN_POINT('Ctrl Pts',(-0.173211914282338,2.37190057928035,
7.57982760159066));
#60775=CARTESIAN_POINT('Ctrl Pts',(-0.202006409449512,2.35248008775026,
7.58176890483647));
#60776=CARTESIAN_POINT('Ctrl Pts',(-0.221923980034108,2.3351643447647,7.58324605302351));
#60777=CARTESIAN_POINT('Ctrl Pts',(-0.240572010170563,2.3144499349627,7.58493572957001));
#60778=CARTESIAN_POINT('Ctrl Pts',(-0.241619355069264,2.31326920499904,
7.5850317675072));
#60779=CARTESIAN_POINT('Ctrl Pts',(-0.243064385402854,2.3116158349032,7.58516589031185));
#60780=CARTESIAN_POINT('Ctrl Pts',(-0.243469460672147,2.31114965958932,
7.58520366761837));
#60781=CARTESIAN_POINT('Ctrl Pts',(-0.244116861893139,2.31040026686489,
7.58526433445649));
#60782=CARTESIAN_POINT('Ctrl Pts',(-0.244360042202338,2.31011778680147,
7.5852871886055));
#60783=CARTESIAN_POINT('Ctrl Pts',(-0.244860990891138,2.30953383520275,
7.58533440505151));
#60784=CARTESIAN_POINT('Ctrl Pts',(-0.245118693769062,2.30923230849398,
7.58535876999264));
#60785=CARTESIAN_POINT('Ctrl Pts',(-0.245717358807478,2.30852921310653,
7.58541554812993));
#60786=CARTESIAN_POINT('Ctrl Pts',(-0.246057893582275,2.30812728350399,
7.58544797879015));
#60787=CARTESIAN_POINT('Ctrl Pts',(-0.246768631135511,2.30728422505712,
7.58551594756151));
#60788=CARTESIAN_POINT('Ctrl Pts',(-0.247138639737531,2.30684293561013,
7.58555149346543));
#60789=CARTESIAN_POINT('Ctrl Pts',(-0.248125469814401,2.30565956822895,
7.58564673093253));
#60790=CARTESIAN_POINT('Ctrl Pts',(-0.248740140926261,2.30491571202373,
7.5857065097549));
#60791=CARTESIAN_POINT('Ctrl Pts',(-0.253227412591613,2.29943541331254,
7.5861463076778));
#60792=CARTESIAN_POINT('Ctrl Pts',(-0.256967553582593,2.29459258647957,
7.58653161471535));
#60793=CARTESIAN_POINT('Ctrl Pts',(-0.268390840917365,2.27889740462174,
7.58777106381338));
#60794=CARTESIAN_POINT('Ctrl Pts',(-0.275540736382772,2.26767574343762,
7.58864434037639));
#60795=CARTESIAN_POINT('Ctrl Pts',(-0.284324466800438,2.25180343556272,
7.58985733119353));
#60796=CARTESIAN_POINT('Ctrl Pts',(-0.286576119062603,2.24750868295947,
7.59018335983897));
#60797=CARTESIAN_POINT('Ctrl Pts',(-0.290933053726064,2.23872176636475,
7.59084500210653));
#60798=CARTESIAN_POINT('Ctrl Pts',(-0.293033262153102,2.23422844981656,
7.59118058048565));
#60799=CARTESIAN_POINT('Ctrl Pts',(-0.30314404845961,2.21122737811287,7.59288088150922));
#60800=CARTESIAN_POINT('Ctrl Pts',(-0.309509492590652,2.1920430044328,7.59424532760991));
#60801=CARTESIAN_POINT('Ctrl Pts',(-0.314310947131777,2.17121276232323,
7.59559366311978));
#60802=CARTESIAN_POINT('Ctrl Pts',(-0.314575144575699,2.17003647284579,
7.59566935628951));
#60803=CARTESIAN_POINT('Ctrl Pts',(-0.314916399814976,2.16847620070052,
7.5957691407845));
#60804=CARTESIAN_POINT('Ctrl Pts',(-0.314999363060229,2.1680935401512,7.59579356406139));
#60805=CARTESIAN_POINT('Ctrl Pts',(-0.315127203680706,2.16749865315473,
7.5958314553584));
#60806=CARTESIAN_POINT('Ctrl Pts',(-0.315172564164754,2.16728653264813,
7.59584495110018));
#60807=CARTESIAN_POINT('Ctrl Pts',(-0.315258657106847,2.16688193664784,
7.59587066339529));
#60808=CARTESIAN_POINT('Ctrl Pts',(-0.315299427203429,2.16668947095373,
7.59588288202449));
#60809=CARTESIAN_POINT('Ctrl Pts',(-0.315394787604303,2.16623725557477,
7.59591156113053));
#60810=CARTESIAN_POINT('Ctrl Pts',(-0.315449233195827,2.16597747609163,
7.5959280131785));
#60811=CARTESIAN_POINT('Ctrl Pts',(-0.315561059876289,2.16544060807013,
7.59596196664057));
#60812=CARTESIAN_POINT('Ctrl Pts',(-0.315618397114836,2.16516351048668,
7.59597946553258));
#60813=CARTESIAN_POINT('Ctrl Pts',(-0.315765540141842,2.16444765208037,
7.59602460679799));
#60814=CARTESIAN_POINT('Ctrl Pts',(-0.315854796796701,2.16400877710048,
7.59605221812197));
#60815=CARTESIAN_POINT('Ctrl Pts',(-0.316609741036623,2.16025668453382,
7.59628774401639));
#60816=CARTESIAN_POINT('Ctrl Pts',(-0.317224222368816,2.15693321588249,
7.59649281634104));
#60817=CARTESIAN_POINT('Ctrl Pts',(-0.320756986632099,2.13598819890224,
7.5977664681049));
#60818=CARTESIAN_POINT('Ctrl Pts',(-0.322258617410972,2.11815760258075,
7.5987687044119));
#60819=CARTESIAN_POINT('Ctrl Pts',(-0.322274866683432,2.10029313678766,
7.59976792125168));
#60820=CARTESIAN_POINT('',(-0.322274884703664,2.09971229684994,7.84976773360871));
#60821=CARTESIAN_POINT('Ctrl Pts',(-0.322274866567678,2.10029326402016,
7.59976791413516));
#60822=CARTESIAN_POINT('Ctrl Pts',(-0.322282627172534,2.09176494918208,
7.60024493013726));
#60823=CARTESIAN_POINT('Ctrl Pts',(-0.321951858909869,2.08323959832138,
7.60072047059375));
#60824=CARTESIAN_POINT('Ctrl Pts',(-0.320114986704937,2.05987875615432,
7.60203851720321));
#60825=CARTESIAN_POINT('Ctrl Pts',(-0.317917443161926,2.04512058209853,
7.60288873575766));
#60826=CARTESIAN_POINT('Ctrl Pts',(-0.313824600351961,2.02656930827139,
7.60401283891559));
#60827=CARTESIAN_POINT('Ctrl Pts',(-0.312866208813105,2.02258760168286,
7.60425735170267));
#60828=CARTESIAN_POINT('Ctrl Pts',(-0.311413820421765,2.01702196652574,
7.60460418843131));
#60829=CARTESIAN_POINT('Ctrl Pts',(-0.31098304858881,2.01542184134173,7.60470449569615));
#60830=CARTESIAN_POINT('Ctrl Pts',(-0.310313100591616,2.01300761512598,
7.60485676073409));
#60831=CARTESIAN_POINT('Ctrl Pts',(-0.310083013916828,2.01219100340156,
7.6049084248884));
#60832=CARTESIAN_POINT('Ctrl Pts',(-0.309651932135624,2.01068385485919,
7.60500407797423));
#60833=CARTESIAN_POINT('Ctrl Pts',(-0.309451844431036,2.00999306236091,
7.60504803722253));
#60834=CARTESIAN_POINT('Ctrl Pts',(-0.309126576618208,2.0088839977207,7.60511880426135));
#60835=CARTESIAN_POINT('Ctrl Pts',(-0.309002855106537,2.00846529742173,
7.60514556439013));
#60836=CARTESIAN_POINT('Ctrl Pts',(-0.308766157524181,2.00767021053095,
7.60519646399146));
#60837=CARTESIAN_POINT('Ctrl Pts',(-0.308653343006841,2.00729377634606,
7.60522059814218));
#60838=CARTESIAN_POINT('Ctrl Pts',(-0.308395354779793,2.00643862430486,
7.60527550576607));
#60839=CARTESIAN_POINT('Ctrl Pts',(-0.308249754647873,2.00596003707599,
7.60530629315531));
#60840=CARTESIAN_POINT('Ctrl Pts',(-0.30781487220525,2.00454244138303,7.60539766059838));
#60841=CARTESIAN_POINT('Ctrl Pts',(-0.307522411175606,2.0036044210643,7.60545834476044));
#60842=CARTESIAN_POINT('Ctrl Pts',(-0.305492471747742,1.99719699118218,
7.60587443567609));
#60843=CARTESIAN_POINT('Ctrl Pts',(-0.303613556244517,1.99177379918732,
7.6062344776727));
#60844=CARTESIAN_POINT('Ctrl Pts',(-0.301468200117906,1.98607800371821,
7.60662137106605));
#60845=CARTESIAN_POINT('Ctrl Pts',(-0.301344912325454,1.98575228346607,
7.60664352658161));
#60846=CARTESIAN_POINT('Ctrl Pts',(-0.293042496448928,1.96392464795292,
7.60813029886089));
#60847=CARTESIAN_POINT('Ctrl Pts',(-0.282586417274222,1.94336353475165,
7.60967188986564));
#60848=CARTESIAN_POINT('Ctrl Pts',(-0.265874628036835,1.91770924492085,
7.61174374413981));
#60849=CARTESIAN_POINT('Ctrl Pts',(-0.261490345514521,1.91147403405841,
7.61225964928539));
#60850=CARTESIAN_POINT('Ctrl Pts',(-0.250889714718192,1.89748026786927,
7.6134390402329));
#60851=CARTESIAN_POINT('Ctrl Pts',(-0.244526749046959,1.88984150594009,
7.61409919278889));
#60852=CARTESIAN_POINT('Ctrl Pts',(-0.23560385684265,1.88008459196654,7.61495262560708));
#60853=CARTESIAN_POINT('Ctrl Pts',(-0.233350190940766,1.87769468204636,
7.61516252906186));
#60854=CARTESIAN_POINT('Ctrl Pts',(-0.230152089300836,1.87440547723299,
7.61545210991204));
#60855=CARTESIAN_POINT('Ctrl Pts',(-0.229238223255117,1.87347691056317,
7.61553393976824));
#60856=CARTESIAN_POINT('Ctrl Pts',(-0.228115317688583,1.87234969682733,
7.61563334319043));
#60857=CARTESIAN_POINT('Ctrl Pts',(-0.227911627488441,1.87214577301291,
7.615651328959));
#60858=CARTESIAN_POINT('Ctrl Pts',(-0.227517165797678,1.87175191707393,
7.61568607123645));
#60859=CARTESIAN_POINT('Ctrl Pts',(-0.227326429468672,1.87156195028338,
7.61570283048679));
#60860=CARTESIAN_POINT('Ctrl Pts',(-0.226995609761852,1.87123328993824,
7.61573182893887));
#60861=CARTESIAN_POINT('Ctrl Pts',(-0.226855637421857,1.87109448618632,
7.61574407694198));
#60862=CARTESIAN_POINT('Ctrl Pts',(-0.226562780386366,1.87080460657884,
7.61576965793466));
#60863=CARTESIAN_POINT('Ctrl Pts',(-0.226409872381463,1.87065355570506,
7.61578298894362));
#60864=CARTESIAN_POINT('Ctrl Pts',(-0.225984988272528,1.87023467101025,
7.61581996146411));
#60865=CARTESIAN_POINT('Ctrl Pts',(-0.225712686126458,1.86996716613611,
7.61584357690281));
#60866=CARTESIAN_POINT('Ctrl Pts',(-0.224631552848655,1.86890884768716,
7.61593702607609));
#60867=CARTESIAN_POINT('Ctrl Pts',(-0.223819023335212,1.86812179900863,
7.6160065674809));
#60868=CARTESIAN_POINT('Ctrl Pts',(-0.209391213088773,1.85429294046512,
7.61722961883035));
#60869=CARTESIAN_POINT('Ctrl Pts',(-0.194659164794283,1.84246422384312,
7.61829535380736));
#60870=CARTESIAN_POINT('Ctrl Pts',(-0.167965688585287,1.82463849064139,
7.62009370560276));
#60871=CARTESIAN_POINT('Ctrl Pts',(-0.156513830330996,1.81797190364002,
7.62082906162481));
#60872=CARTESIAN_POINT('Ctrl Pts',(-0.133489201985662,1.8064036992444,7.62228830139366));
#60873=CARTESIAN_POINT('Ctrl Pts',(-0.121976232835162,1.80143692946991,
7.62300942403435));
#60874=CARTESIAN_POINT('Ctrl Pts',(-0.106731420851478,1.79588943422921,
7.62397206999624));
#60875=CARTESIAN_POINT('Ctrl Pts',(-0.103237326017269,1.79468559604599,
7.6241931708423));
#60876=CARTESIAN_POINT('Ctrl Pts',(-0.0975213145023391,1.79282556823799,
7.62455601876995));
#60877=CARTESIAN_POINT('Ctrl Pts',(-0.0953116096362679,1.79213276409057,
7.62469656347766));
#60878=CARTESIAN_POINT('Ctrl Pts',(-0.0926018226668458,1.79131513953503,
7.62486930877767));
#60879=CARTESIAN_POINT('Ctrl Pts',(-0.0921086180276386,1.79116761322408,
7.62490076574525));
#60880=CARTESIAN_POINT('Ctrl Pts',(-0.0911523278631431,1.79088406430516,
7.62496179022892));
#60881=CARTESIAN_POINT('Ctrl Pts',(-0.0906892858261045,1.79074789894379,
7.62499135299994));
#60882=CARTESIAN_POINT('Ctrl Pts',(-0.0898862006454022,1.79051369691227,
7.62504265115158));
#60883=CARTESIAN_POINT('Ctrl Pts',(-0.0895462977544971,1.79041517895375,
7.62506437079241));
#60884=CARTESIAN_POINT('Ctrl Pts',(-0.0888400215349069,1.79021173127658,
7.62510951818272));
#60885=CARTESIAN_POINT('Ctrl Pts',(-0.0884736231336985,1.79010689121468,
7.62513294881542));
#60886=CARTESIAN_POINT('Ctrl Pts',(-0.0875810556523122,1.78985320681173,
7.62519005021932));
#60887=CARTESIAN_POINT('Ctrl Pts',(-0.0870546934337768,1.78970505163731,
7.62522374336172));
#60888=CARTESIAN_POINT('Ctrl Pts',(-0.0850656938766144,1.78915066722938,
7.62535113714026));
#60889=CARTESIAN_POINT('Ctrl Pts',(-0.0836005876066289,1.78875343924163,
7.62544512964909));
#60890=CARTESIAN_POINT('Ctrl Pts',(-0.0569263426189914,1.78172329113667,
7.62715934229412));
#60891=CARTESIAN_POINT('Ctrl Pts',(-0.0310126781057647,1.77816415002519,
7.62888461008634));
#60892=CARTESIAN_POINT('Ctrl Pts',(0.0107898038386987,1.77752076425262,
7.6317106256321));
#60893=CARTESIAN_POINT('Ctrl Pts',(0.0265363553429475,1.77843330420052,
7.63278180849565));
#60894=CARTESIAN_POINT('Ctrl Pts',(0.0473904299778287,1.78118465379786,
7.63416827861842));
#60895=CARTESIAN_POINT('Ctrl Pts',(0.052609849427483,1.782004263736,7.63451243056053));
#60896=CARTESIAN_POINT('Ctrl Pts',(0.060879218885872,1.78351200927402,7.63505074558761));
#60897=CARTESIAN_POINT('Ctrl Pts',(0.063943219805935,1.78411680324568,7.63524867083693));
#60898=CARTESIAN_POINT('Ctrl Pts',(0.0674968135246448,1.78487206445999,
7.6354760530861));
#60899=CARTESIAN_POINT('Ctrl Pts',(0.0679952969282747,1.78497924640143,
7.63550789945115));
#60900=CARTESIAN_POINT('Ctrl Pts',(0.0687565049252962,1.78514480934257,
7.63555645192006));
#60901=CARTESIAN_POINT('Ctrl Pts',(0.0690194113359994,1.78520233655002,
7.63557320668361));
#60902=CARTESIAN_POINT('Ctrl Pts',(0.0694747555877969,1.78530256941549,
7.63560220014495));
#60903=CARTESIAN_POINT('Ctrl Pts',(0.0696672259412174,1.78534512221979,
7.63561444763467));
#60904=CARTESIAN_POINT('Ctrl Pts',(0.070069517538475,1.78543445110896,7.6356400303097));
#60905=CARTESIAN_POINT('Ctrl Pts',(0.0702793303757291,1.78548126039962,
7.63565336350943));
#60906=CARTESIAN_POINT('Ctrl Pts',(0.0707963099453595,1.78559714179906,
7.63568619399884));
#60907=CARTESIAN_POINT('Ctrl Pts',(0.0711034233863667,1.78566645433312,
7.635705677421));
#60908=CARTESIAN_POINT('Ctrl Pts',(0.0723030486474282,1.78593904623824,
7.63578170720328));
#60909=CARTESIAN_POINT('Ctrl Pts',(0.0731948055165846,1.78614568026774,
7.63583806258971));
#60910=CARTESIAN_POINT('Ctrl Pts',(0.0899864871920014,1.79011203591269,
7.63689637351517));
#60911=CARTESIAN_POINT('Ctrl Pts',(0.105581208741519,1.79507232211674,7.63783145380563));
#60912=CARTESIAN_POINT('Ctrl Pts',(0.137222385028771,1.80785717085118,7.63975289566128));
#60913=CARTESIAN_POINT('Ctrl Pts',(0.153130457127615,1.81587242733715,7.64073415353935));
#60914=CARTESIAN_POINT('Ctrl Pts',(0.174727180110384,1.82909696602539,7.64217534513245));
#60915=CARTESIAN_POINT('Ctrl Pts',(0.181017677694464,1.83325924299381,7.64260927791923));
#60916=CARTESIAN_POINT('Ctrl Pts',(0.194073658011579,1.84257274184813,7.64354752861949));
#60917=CARTESIAN_POINT('Ctrl Pts',(0.200792768955453,1.84777862434406,7.64405344031565));
#60918=CARTESIAN_POINT('Ctrl Pts',(0.208166112695658,1.85397290633075,7.64463905229903));
#60919=CARTESIAN_POINT('Ctrl Pts',(0.209030422120792,1.85470682057848,7.6447081899481));
#60920=CARTESIAN_POINT('Ctrl Pts',(0.210293358067197,1.85579074432932,7.64480994713881));
#60921=CARTESIAN_POINT('Ctrl Pts',(0.210695028700754,1.85613720686034,7.64484242025708));
#60922=CARTESIAN_POINT('Ctrl Pts',(0.211395994881534,1.85674485253725,7.64489928316279));
#60923=CARTESIAN_POINT('Ctrl Pts',(0.211695667121723,1.85700560101377,7.6449236548852));
#60924=CARTESIAN_POINT('Ctrl Pts',(0.212274821677775,1.85751141496069,7.64497087708462));
#60925=CARTESIAN_POINT('Ctrl Pts',(0.212554363750437,1.857756411351,7.64499372466289));
#60926=CARTESIAN_POINT('Ctrl Pts',(0.213217953092829,1.85834002760045,7.645048091906));
#60927=CARTESIAN_POINT('Ctrl Pts',(0.213601617603051,1.85867907936986,7.64507962960342));
#60928=CARTESIAN_POINT('Ctrl Pts',(0.214956805069971,1.8598824486145,7.64519139950662));
#60929=CARTESIAN_POINT('Ctrl Pts',(0.215923893206026,1.86075172144294,7.6452718397134));
#60930=CARTESIAN_POINT('Ctrl Pts',(0.232673910789583,1.87599185414803,7.64667705901706));
#60931=CARTESIAN_POINT('Ctrl Pts',(0.246992743009958,1.89188690915617,7.64807035270954));
#60932=CARTESIAN_POINT('Ctrl Pts',(0.269513355504437,1.92251242015414,7.65062206910837));
#60933=CARTESIAN_POINT('Ctrl Pts',(0.278335080892861,1.93669396118157,7.6517600312076));
#60934=CARTESIAN_POINT('Ctrl Pts',(0.29012781088824,1.95940658105974,7.65347159965461));
#60935=CARTESIAN_POINT('Ctrl Pts',(0.293906238454361,1.96748658240961,7.65406030247668));
#60936=CARTESIAN_POINT('Ctrl Pts',(0.298715390051944,1.97899207300769,7.65486129222814));
#60937=CARTESIAN_POINT('Ctrl Pts',(0.300031544497606,1.98229325613311,7.65508694159062));
#60938=CARTESIAN_POINT('Ctrl Pts',(0.301479659184068,1.98610764898124,7.65534236059185));
#60939=CARTESIAN_POINT('Ctrl Pts',(0.301665222182729,1.98660006059487,7.65537523261527));
#60940=CARTESIAN_POINT('Ctrl Pts',(0.301926520519513,1.98729862439793,7.65542172179269));
#60941=CARTESIAN_POINT('Ctrl Pts',(0.302003251182413,1.98750439950132,7.65543539825272));
#60942=CARTESIAN_POINT('Ctrl Pts',(0.302157223648336,1.9879186133441,7.65546289216664));
#60943=CARTESIAN_POINT('Ctrl Pts',(0.302234460370589,1.98812705419416,7.65547670931627));
#60944=CARTESIAN_POINT('Ctrl Pts',(0.30238331287976,1.9885300457749,7.65550338722137));
#60945=CARTESIAN_POINT('Ctrl Pts',(0.302454956426713,1.98872458521033,7.6555162496574));
#60946=CARTESIAN_POINT('Ctrl Pts',(0.302625284311501,1.98918846988976,7.65554688265321));
#60947=CARTESIAN_POINT('Ctrl Pts',(0.302723797054619,1.98945787857878,7.65556464288974));
#60948=CARTESIAN_POINT('Ctrl Pts',(0.303072787575791,1.9904162490999,7.65562771481072));
#60949=CARTESIAN_POINT('Ctrl Pts',(0.303321276580222,1.99110594034042,7.65567290849936));
#60950=CARTESIAN_POINT('Ctrl Pts',(0.306958275080049,2.00130962170744,7.65633872033921));
#60951=CARTESIAN_POINT('Ctrl Pts',(0.309900483222269,2.01097803085273,7.65693361398019));
#60952=CARTESIAN_POINT('Ctrl Pts',(0.31706126377891,2.03921108816337,7.65861076261609));
#60953=CARTESIAN_POINT('Ctrl Pts',(0.320096628769684,2.05803134278968,7.65965768632261));
#60954=CARTESIAN_POINT('Ctrl Pts',(0.32289076322274,2.09710043748009,7.66185883407635));
#60955=CARTESIAN_POINT('Ctrl Pts',(0.322440930026884,2.11727788974356,7.6630120298648));
#60956=CARTESIAN_POINT('Ctrl Pts',(0.319881450294143,2.13925543779138,7.66435018529346));
#60957=CARTESIAN_POINT('Ctrl Pts',(0.319633091555802,2.14122885089238,7.66447103743562));
#60958=CARTESIAN_POINT('Ctrl Pts',(0.31927785080493,2.14385506622871,7.66463283617608));
#60959=CARTESIAN_POINT('Ctrl Pts',(0.319187199544413,2.14451004926154,7.66467326951541));
#60960=CARTESIAN_POINT('Ctrl Pts',(0.319035159339379,2.14558423219985,7.66473971449814));
#60961=CARTESIAN_POINT('Ctrl Pts',(0.318974958047902,2.14600360046319,7.66476568852064));
#60962=CARTESIAN_POINT('Ctrl Pts',(0.318856773448181,2.14681550058235,7.66481603970489));
#60963=CARTESIAN_POINT('Ctrl Pts',(0.318798891776286,2.14720804665027,7.66484041360587));
#60964=CARTESIAN_POINT('Ctrl Pts',(0.318663679155768,2.14811345151512,7.66489670055097));
#60965=CARTESIAN_POINT('Ctrl Pts',(0.318585834954727,2.1486262315111,7.6649286298051));
#60966=CARTESIAN_POINT('Ctrl Pts',(0.318332984257065,2.15026515276589,7.66503084457905));
#60967=CARTESIAN_POINT('Ctrl Pts',(0.318153243375403,2.15139054509174,7.66510128000994));
#60968=CARTESIAN_POINT('Ctrl Pts',(0.316459783595278,2.16164410621306,7.66574532391633));
#60969=CARTESIAN_POINT('Ctrl Pts',(0.314559713562472,2.17070324404687,7.66633117520644));
#60970=CARTESIAN_POINT('Ctrl Pts',(0.310352786517696,2.18719315707374,7.6674302968538));
#60971=CARTESIAN_POINT('Ctrl Pts',(0.308161508710353,2.19464654772916,7.66793972644221));
#60972=CARTESIAN_POINT('Ctrl Pts',(0.298538275863968,2.22348455142405,7.66995762257628));
#60973=CARTESIAN_POINT('Ctrl Pts',(0.289131803603431,2.24413963968149,7.67151123890643));
#60974=CARTESIAN_POINT('Ctrl Pts',(0.272619389909045,2.27215573413383,7.67367717072749));
#60975=CARTESIAN_POINT('Ctrl Pts',(0.26720929408885,2.28043880847528,7.67432480367485));
#60976=CARTESIAN_POINT('Ctrl Pts',(0.260867972785904,2.28923527152023,7.67501013469854));
#60977=CARTESIAN_POINT('Ctrl Pts',(0.260306192193256,2.29000729873281,7.67507026059871));
#60978=CARTESIAN_POINT('Ctrl Pts',(0.259325266363233,2.29134282065335,7.67517421604834));
#60979=CARTESIAN_POINT('Ctrl Pts',(0.258907698395762,2.29190745822746,7.67521814934222));
#60980=CARTESIAN_POINT('Ctrl Pts',(0.258308662744803,2.29271196338546,7.67528071589409));
#60981=CARTESIAN_POINT('Ctrl Pts',(0.258128703517364,2.29295294375339,7.6752994530861));
#60982=CARTESIAN_POINT('Ctrl Pts',(0.257814694324563,2.2933722026742,7.67533204482165));
#60983=CARTESIAN_POINT('Ctrl Pts',(0.257680796320666,2.29355059438157,7.6753459100532));
#60984=CARTESIAN_POINT('Ctrl Pts',(0.257422744005917,2.29389365389967,7.67537256916636));
#60985=CARTESIAN_POINT('Ctrl Pts',(0.257298617096428,2.29405834121462,7.67538536494083));
#60986=CARTESIAN_POINT('Ctrl Pts',(0.257003954595633,2.29444850956187,7.67541567542274));
#60987=CARTESIAN_POINT('Ctrl Pts',(0.256833279880444,2.29467388601427,7.675433180306));
#60988=CARTESIAN_POINT('Ctrl Pts',(0.256233593242599,2.29546361262195,7.67549450638565));
#60989=CARTESIAN_POINT('Ctrl Pts',(0.255803011989643,2.29602677685642,7.67553821796193));
#60990=CARTESIAN_POINT('Ctrl Pts',(0.250117198696013,2.3034127085152,7.6761112905374));
#60991=CARTESIAN_POINT('Ctrl Pts',(0.244591840034279,2.31002429735919,7.67662196977456));
#60992=CARTESIAN_POINT('Ctrl Pts',(0.218866253677617,2.33841275828205,7.6788445624055));
#60993=CARTESIAN_POINT('Ctrl Pts',(0.195978364654515,2.3575574639317,7.68043916532117));
#60994=CARTESIAN_POINT('Ctrl Pts',(0.161446403587191,2.37913732276244,7.68278696891977));
#60995=CARTESIAN_POINT('Ctrl Pts',(0.151809872449005,2.38449307467799,7.68343513773508));
#60996=CARTESIAN_POINT('Ctrl Pts',(0.140136153002332,2.39021884200434,7.68422152465313));
#60997=CARTESIAN_POINT('Ctrl Pts',(0.138345570024417,2.39107665762414,7.68434216549759));
#60998=CARTESIAN_POINT('Ctrl Pts',(0.135949624369565,2.39219738276677,7.68450365968567));
#60999=CARTESIAN_POINT('Ctrl Pts',(0.135351189781173,2.39247506949584,7.68454400152066));
#61000=CARTESIAN_POINT('Ctrl Pts',(0.134367356869488,2.3929279232953,7.68461033453553));
#61001=CARTESIAN_POINT('Ctrl Pts',(0.133982456554868,2.39310417289934,7.684636288343));
#61002=CARTESIAN_POINT('Ctrl Pts',(0.133235995958048,2.39344420689029,7.68468662775838));
#61003=CARTESIAN_POINT('Ctrl Pts',(0.132874477993955,2.39360808277702,7.6847110101623));
#61004=CARTESIAN_POINT('Ctrl Pts',(0.132039126491449,2.39398488831605,7.6847673563651));
#61005=CARTESIAN_POINT('Ctrl Pts',(0.131565079966595,2.3941973405916,7.68479933648259));
#61006=CARTESIAN_POINT('Ctrl Pts',(0.130292630787299,2.39476392052288,7.68488519210596));
#61007=CARTESIAN_POINT('Ctrl Pts',(0.129493302917554,2.39511594832361,7.68493913936043));
#61008=CARTESIAN_POINT('Ctrl Pts',(0.123833053926022,2.39758132535605,7.68532126866551));
#61009=CARTESIAN_POINT('Ctrl Pts',(0.118922321009848,2.39957761367977,7.68565341456002));
#61010=CARTESIAN_POINT('Ctrl Pts',(0.112486785114604,2.4020105885899,7.68608982877782));
#61011=CARTESIAN_POINT('Ctrl Pts',(0.111004680896542,2.40255847885103,7.68619041031641));
#61012=CARTESIAN_POINT('Ctrl Pts',(0.104348801382813,2.40496347310704,7.6866424533139));
#61013=CARTESIAN_POINT('Ctrl Pts',(0.099132284114397,2.40669883751386,7.68699770113815));
#61014=CARTESIAN_POINT('Ctrl Pts',(0.0658731152984475,2.41682591571437,
7.68926820793129));
#61015=CARTESIAN_POINT('Ctrl Pts',(0.0368463247491426,2.42149631890393,
7.69129150223799));
#61016=CARTESIAN_POINT('Ctrl Pts',(-0.000754476213337938,2.42238220977441,
7.69378110817522));
#61017=CARTESIAN_POINT('Ctrl Pts',(-0.00910512026353613,2.42225453034135,
7.69432447945846));
#61018=CARTESIAN_POINT('Ctrl Pts',(-0.01874709040981,2.4217319228053,7.69493398291066));
#61019=CARTESIAN_POINT('Ctrl Pts',(-0.0200516356364027,2.42165325367172,
7.69501606672404));
#61020=CARTESIAN_POINT('Ctrl Pts',(-0.0217428297209001,2.42154093909962,
7.69512195306316));
#61021=CARTESIAN_POINT('Ctrl Pts',(-0.0221299227381875,2.42151452950793,
7.69514615335335));
#61022=CARTESIAN_POINT('Ctrl Pts',(-0.0227565565787065,2.4214706400921,
7.69518527032531));
#61023=CARTESIAN_POINT('Ctrl Pts',(-0.022996125731761,2.42145359153504,
7.69520021123239));
#61024=CARTESIAN_POINT('Ctrl Pts',(-0.0234556528949428,2.4214203736771,
7.695228842928));
#61025=CARTESIAN_POINT('Ctrl Pts',(-0.0236756126656092,2.42140424644455,
7.69524253599996));
#61026=CARTESIAN_POINT('Ctrl Pts',(-0.0241815579501206,2.4213666288356,
7.69527400524159));
#61027=CARTESIAN_POINT('Ctrl Pts',(-0.024467532290785,2.42134498243971,
7.695291772572));
#61028=CARTESIAN_POINT('Ctrl Pts',(-0.025353559332595,2.42127672634035,
7.69534675983841));
#61029=CARTESIAN_POINT('Ctrl Pts',(-0.0259535150184322,2.42122881709272,
7.69538390695073));
#61030=CARTESIAN_POINT('Ctrl Pts',(-0.0309211943292435,2.4208181165863,
7.69569079793071));
#61031=CARTESIAN_POINT('Ctrl Pts',(-0.0352814940747872,2.42036792129348,
7.69595574847398));
#61032=CARTESIAN_POINT('Ctrl Pts',(-0.0398140977481186,2.41980626494128,
7.69622781639151));
#61033=CARTESIAN_POINT('Ctrl Pts',(-0.0399966664845369,2.41978348322828,
7.69623876933111));
#61034=CARTESIAN_POINT('Ctrl Pts',(-0.0685396888196573,2.41619693611508,
7.69795029059364));
#61035=CARTESIAN_POINT('Ctrl Pts',(-0.0963035101548373,2.40887582910447,
7.69948957840477));
#61036=CARTESIAN_POINT('Ctrl Pts',(-0.13730168874294,2.39198876011352,7.70200256126843));
#61037=CARTESIAN_POINT('Ctrl Pts',(-0.151402187655715,2.38493239541957,
7.70291419626693));
#61038=CARTESIAN_POINT('Ctrl Pts',(-0.167059228957503,2.3756057605764,7.70401332021529));
#61039=CARTESIAN_POINT('Ctrl Pts',(-0.169174272798061,2.3743125701388,7.70416369835424));
#61040=CARTESIAN_POINT('Ctrl Pts',(-0.171876080648981,2.37261748563579,
7.70435833660206));
#61041=CARTESIAN_POINT('Ctrl Pts',(-0.172476764307002,2.37223784882908,
7.70440177327053));
#61042=CARTESIAN_POINT('Ctrl Pts',(-0.173442855206537,2.371622790916,7.70447189920152));
#61043=CARTESIAN_POINT('Ctrl Pts',(-0.173809052608442,2.37138861029088,
7.70449854234858));
#61044=CARTESIAN_POINT('Ctrl Pts',(-0.174505763414764,2.3709410801583,7.70454935092744));
#61045=CARTESIAN_POINT('Ctrl Pts',(-0.174836362388252,2.37072786477749,
7.70457351132938));
#61046=CARTESIAN_POINT('Ctrl Pts',(-0.175589406401248,2.37024024449193,
7.70462866124025));
#61047=CARTESIAN_POINT('Ctrl Pts',(-0.176011599351105,2.36996545385044,
7.70465966512925));
#61048=CARTESIAN_POINT('Ctrl Pts',(-0.177297957180039,2.36912390826298,
7.70475438769765));
#61049=CARTESIAN_POINT('Ctrl Pts',(-0.178160035407185,2.36855398966096,
7.70481822490645));
#61050=CARTESIAN_POINT('Ctrl Pts',(-0.184431644300477,2.36436435014612,
7.70528527566721));
#61051=CARTESIAN_POINT('Ctrl Pts',(-0.18973281568978,2.36058585866802,7.70569447673474));
#61052=CARTESIAN_POINT('Ctrl Pts',(-0.196355075678692,2.35555650413883,
7.7062250027743));
#61053=CARTESIAN_POINT('Ctrl Pts',(-0.197785238188114,2.35445125643444,
7.70634076801978));
#61054=CARTESIAN_POINT('Ctrl Pts',(-0.204139354505823,2.34945477802752,
7.70686047278658));
#61055=CARTESIAN_POINT('Ctrl Pts',(-0.208958066600866,2.34543243628884,
7.70726920031167));
#61056=CARTESIAN_POINT('Ctrl Pts',(-0.231300447782583,2.32564737507268,
7.70923411880967));
#61057=CARTESIAN_POINT('Ctrl Pts',(-0.247176887376128,2.30813467009008,
7.71084974170074));
#61058=CARTESIAN_POINT('Ctrl Pts',(-0.266191809007985,2.28188300157065,
7.71301940431304));
#61059=CARTESIAN_POINT('Ctrl Pts',(-0.271086553062576,2.27450390153318,
7.71360463705952));
#61060=CARTESIAN_POINT('Ctrl Pts',(-0.277691097829145,2.26359715716246,
7.71442550875905));
#61061=CARTESIAN_POINT('Ctrl Pts',(-0.279649990149578,2.26022565977059,
7.71467344857037));
#61062=CARTESIAN_POINT('Ctrl Pts',(-0.281809978508257,2.25634769904972,
7.71495137026948));
#61063=CARTESIAN_POINT('Ctrl Pts',(-0.282071451878627,2.25587547283041,
7.71498509223173));
#61064=CARTESIAN_POINT('Ctrl Pts',(-0.282463461444175,2.25516327913916,
7.71503576575282));
#61065=CARTESIAN_POINT('Ctrl Pts',(-0.282594879330144,2.2549238019865,7.71505277351064));
#61066=CARTESIAN_POINT('Ctrl Pts',(-0.282830805813152,2.25449258426823,
7.71508334196713));
#61067=CARTESIAN_POINT('Ctrl Pts',(-0.282935423783227,2.25430090498878,
7.71509690968145));
#61068=CARTESIAN_POINT('Ctrl Pts',(-0.283159748678892,2.25388890545698,
7.71512602903156));
#61069=CARTESIAN_POINT('Ctrl Pts',(-0.28327939296606,2.25366855246422,7.71514157660566));
#61070=CARTESIAN_POINT('Ctrl Pts',(-0.283600758804313,2.25307503119626,
7.71518338319139));
#61071=CARTESIAN_POINT('Ctrl Pts',(-0.283802001821224,2.25270160227473,
7.715209611588));
#61072=CARTESIAN_POINT('Ctrl Pts',(-0.284723167831009,2.25098416461056,
7.71532989823764));
#61073=CARTESIAN_POINT('Ctrl Pts',(-0.28543430007864,2.24963542634218,7.71542340556752));
#61074=CARTESIAN_POINT('Ctrl Pts',(-0.300856923577085,2.21987473000819,
7.71746687796392));
#61075=CARTESIAN_POINT('Ctrl Pts',(-0.311268623925318,2.18942870693895,
7.71917530570832));
#61076=CARTESIAN_POINT('Ctrl Pts',(-0.320075159774721,2.14124543488957,
7.72195175980088));
#61077=CARTESIAN_POINT('Ctrl Pts',(-0.321802671577201,2.12433537806756,
7.72293636262128));
#61078=CARTESIAN_POINT('Ctrl Pts',(-0.322224436732959,2.10589581504815,
7.72405550158802));
#61079=CARTESIAN_POINT('Ctrl Pts',(-0.322248031643791,2.1044220189982,7.72414524873119));
#61080=CARTESIAN_POINT('Ctrl Pts',(-0.322266841072826,2.10236595246547,
7.72427088711324));
#61081=CARTESIAN_POINT('Ctrl Pts',(-0.322270589364442,2.10178376282133,
7.72430651099395));
#61082=CARTESIAN_POINT('Ctrl Pts',(-0.322274276684768,2.10079478700175,
7.72436710941423));
#61083=CARTESIAN_POINT('Ctrl Pts',(-0.322275023155283,2.10038800376921,
7.72439205861316));
#61084=CARTESIAN_POINT('Ctrl Pts',(-0.322274975684238,2.09957330169344,
7.72444207515811));
#61085=CARTESIAN_POINT('Ctrl Pts',(-0.322274177427816,2.09916538361351,
7.72446714259294));
#61086=CARTESIAN_POINT('Ctrl Pts',(-0.322270338419107,2.09816966763754,
7.72452839141201));
#61087=CARTESIAN_POINT('Ctrl Pts',(-0.322266463987034,2.09758187607652,
7.72456459884681));
#61088=CARTESIAN_POINT('Ctrl Pts',(-0.322246901720612,2.09548461458602,
7.7246939723881));
#61089=CARTESIAN_POINT('Ctrl Pts',(-0.322222216542256,2.09397526630236,
7.72478741982268));
#61090=CARTESIAN_POINT('Ctrl Pts',(-0.321749558177897,2.07376186946427,
7.72604356066092));
#61091=CARTESIAN_POINT('Ctrl Pts',(-0.31968436819104,2.05513463260738,7.72725805362947));
#61092=CARTESIAN_POINT('Ctrl Pts',(-0.310084166221126,2.00713544075561,
7.73052644916394));
#61093=CARTESIAN_POINT('Ctrl Pts',(-0.300006792080827,1.97845991596012,
7.73262950984543));
#61094=CARTESIAN_POINT('Ctrl Pts',(-0.285390834993922,1.95028198303144,
7.73463711044471));
#61095=CARTESIAN_POINT('Ctrl Pts',(-0.284692807219456,1.94895888299198,
7.73473119228828));
#61096=CARTESIAN_POINT('Ctrl Pts',(-0.28378412276943,1.94726516812631,7.73485134174637));
#61097=CARTESIAN_POINT('Ctrl Pts',(-0.283581923420975,1.9468900724403,7.73487793232737));
#61098=CARTESIAN_POINT('Ctrl Pts',(-0.283260531620537,1.9462966860919,7.73491996750274));
#61099=CARTESIAN_POINT('Ctrl Pts',(-0.283141830321619,1.94607813214683,
7.73493544327615));
#61100=CARTESIAN_POINT('Ctrl Pts',(-0.282928771256614,1.94568692624474,
7.73496313260724));
#61101=CARTESIAN_POINT('Ctrl Pts',(-0.282834509062742,1.94551422453788,
7.7349753521463));
#61102=CARTESIAN_POINT('Ctrl Pts',(-0.282612635268746,1.94510860402726,
7.73500404214789));
#61103=CARTESIAN_POINT('Ctrl Pts',(-0.282484894055848,1.94487575691916,
7.73502050416059));
#61104=CARTESIAN_POINT('Ctrl Pts',(-0.282114144152394,1.94420192937727,
7.73506812192688));
#61105=CARTESIAN_POINT('Ctrl Pts',(-0.28187038827982,1.9437613576617,7.73509922993938));
#61106=CARTESIAN_POINT('Ctrl Pts',(-0.280189839225027,1.94074061647781,
7.73531235229594));
#61107=CARTESIAN_POINT('Ctrl Pts',(-0.27871861205453,1.93817962418204,7.73549220017288));
#61108=CARTESIAN_POINT('Ctrl Pts',(-0.273994511379368,1.93021192009098,
7.7360502531131));
#61109=CARTESIAN_POINT('Ctrl Pts',(-0.270617787235335,1.92488001687209,
7.7364215247782));
#61110=CARTESIAN_POINT('Ctrl Pts',(-0.258383994817622,1.90676254116668,
7.73768775441519));
#61111=CARTESIAN_POINT('Ctrl Pts',(-0.248759537234503,1.89452065582141,
7.73855244538971));
#61112=CARTESIAN_POINT('Ctrl Pts',(-0.227423412915464,1.87108914866398,
7.74032418162177));
#61113=CARTESIAN_POINT('Ctrl Pts',(-0.215678380409823,1.85999090158165,
7.74122950041062));
#61114=CARTESIAN_POINT('Ctrl Pts',(-0.19553047000612,1.84363032168451,7.74273954613139));
#61115=CARTESIAN_POINT('Ctrl Pts',(-0.187630317063021,1.83779318982994,
7.74332203418941));
#61116=CARTESIAN_POINT('Ctrl Pts',(-0.178611654321421,1.83174613306845,
7.74398229859104));
#61117=CARTESIAN_POINT('Ctrl Pts',(-0.177743876704504,1.83117036168348,
7.74404578045392));
#61118=CARTESIAN_POINT('Ctrl Pts',(-0.176441835193752,1.83031551608606,
7.74414096390663));
#61119=CARTESIAN_POINT('Ctrl Pts',(-0.176009660903805,1.83003325883712,
7.74417254630693));
#61120=CARTESIAN_POINT('Ctrl Pts',(-0.175264190211969,1.82954893559221,
7.74422700574909));
#61121=CARTESIAN_POINT('Ctrl Pts',(-0.174951216939581,1.82934637209262,
7.74424986417901));
#61122=CARTESIAN_POINT('Ctrl Pts',(-0.174304563642449,1.82892943350893,
7.74429708250409));
#61123=CARTESIAN_POINT('Ctrl Pts',(-0.173970838069511,1.82871513049273,
7.74432144503122));
#61124=CARTESIAN_POINT('Ctrl Pts',(-0.173193129765183,1.82821774766822,
7.74437820564126));
#61125=CARTESIAN_POINT('Ctrl Pts',(-0.172748848121884,1.82793513944702,
7.74441062115514));
#61126=CARTESIAN_POINT('Ctrl Pts',(-0.171330767636939,1.82703797030089,
7.74451405575814));
#61127=CARTESIAN_POINT('Ctrl Pts',(-0.17035437494087,1.82642754436919,7.74458522750354));
#61128=CARTESIAN_POINT('Ctrl Pts',(-0.149232484045475,1.81337937984627,
7.74612395229316));
#61129=CARTESIAN_POINT('Ctrl Pts',(-0.12778487432275,1.80319652752802,7.74767705029028));
#61130=CARTESIAN_POINT('Ctrl Pts',(-0.0841474590898502,1.78809112455826,
7.7507879369035));
#61131=CARTESIAN_POINT('Ctrl Pts',(-0.0621607463559797,1.78297621808199,
7.75233154489361));
#61132=CARTESIAN_POINT('Ctrl Pts',(-0.0393030596261878,1.78013015745656,
7.75382047173914));
#61133=CARTESIAN_POINT('Ctrl Pts',(-0.0387862756358132,1.78006708282181,
7.75385407231093));
#61134=CARTESIAN_POINT('Ctrl Pts',(-0.0343386619931378,1.77953517648902,
7.75414270215606));
#61135=CARTESIAN_POINT('Ctrl Pts',(-0.0303994324227468,1.7791375296862,
7.75439466285182));
#61136=CARTESIAN_POINT('Ctrl Pts',(-0.0258636736898057,1.77876395523703,
7.75467979869705));
#61137=CARTESIAN_POINT('Ctrl Pts',(-0.0252735476693131,1.77871698788587,
7.75471679961649));
#61138=CARTESIAN_POINT('Ctrl Pts',(-0.0244004638428416,1.77864992072209,
7.75477139556526));
#61139=CARTESIAN_POINT('Ctrl Pts',(-0.0241176077816137,1.77862856834492,
7.75478906048402));
#61140=CARTESIAN_POINT('Ctrl Pts',(-0.0236158733734507,1.77859135931309,
7.75482035404235));
#61141=CARTESIAN_POINT('Ctrl Pts',(-0.023397007028472,1.77857535277048,
7.75483399113954));
#61142=CARTESIAN_POINT('Ctrl Pts',(-0.0229345523295774,1.77854200652439,
7.7548627765025));
#61143=CARTESIAN_POINT('Ctrl Pts',(-0.0226909612358904,1.77852472017422,
7.75487792169359));
#61144=CARTESIAN_POINT('Ctrl Pts',(-0.0220423638416082,1.77847943357468,
7.75491820312795));
#61145=CARTESIAN_POINT('Ctrl Pts',(-0.0216373222189689,1.77845192158921,
7.75494331183649));
#61146=CARTESIAN_POINT('Ctrl Pts',(-0.0197533042653283,1.77832752784366,
7.7550598907854));
#61147=CARTESIAN_POINT('Ctrl Pts',(-0.0182736920653518,1.77824008212772,
7.75515083806837));
#61148=CARTESIAN_POINT('Ctrl Pts',(-0.00646758888353097,1.77762403844278,
7.75587205036314));
#61149=CARTESIAN_POINT('Ctrl Pts',(0.0038794469008034,1.77758243324402,
7.75647691100931));
#61150=CARTESIAN_POINT('Ctrl Pts',(0.0435014725895693,1.77933137914622,
7.75874871504159));
#61151=CARTESIAN_POINT('Ctrl Pts',(0.0724776566637045,1.78461470851599,
7.76033005174923));
#61152=CARTESIAN_POINT('Ctrl Pts',(0.109685900557101,1.79680554651173,7.76260798048083));
#61153=CARTESIAN_POINT('Ctrl Pts',(0.118884766532973,1.80029304965327,7.76319133893898));
#61154=CARTESIAN_POINT('Ctrl Pts',(0.128865459385863,1.80460881123032,7.76385254375402));
#61155=CARTESIAN_POINT('Ctrl Pts',(0.129819694152113,1.80502693683003,7.76391605012076));
#61156=CARTESIAN_POINT('Ctrl Pts',(0.13124374586941,1.80565917485821,7.76401126434545));
#61157=CARTESIAN_POINT('Ctrl Pts',(0.13171510941765,1.80586980413228,7.76404285290647));
#61158=CARTESIAN_POINT('Ctrl Pts',(0.132525991113844,1.80623448754287,7.76409732014512));
#61159=CARTESIAN_POINT('Ctrl Pts',(0.132865752816791,1.8063880003194,7.76412018019851));
#61160=CARTESIAN_POINT('Ctrl Pts',(0.133566378863496,1.80670602571804,7.76416739923939));
#61161=CARTESIAN_POINT('Ctrl Pts',(0.133927207328215,1.80687061551613,7.76419176085427));
#61162=CARTESIAN_POINT('Ctrl Pts',(0.134766306408868,1.80725523840757,7.76424851483342));
#61163=CARTESIAN_POINT('Ctrl Pts',(0.135244342480983,1.80747577774731,7.76428092461616));
#61164=CARTESIAN_POINT('Ctrl Pts',(0.136732234250004,1.8081666353005,7.76438204177389));
#61165=CARTESIAN_POINT('Ctrl Pts',(0.137740185050097,1.80864101522819,7.76445088945287));
#61166=CARTESIAN_POINT('Ctrl Pts',(0.143828822133454,1.81154521506301,7.76486890237278));
#61167=CARTESIAN_POINT('Ctrl Pts',(0.14884728945677,1.81410251664506,7.76522248547441));
#61168=CARTESIAN_POINT('Ctrl Pts',(0.166135537625027,1.82349081874894,7.76647356544263));
#61169=CARTESIAN_POINT('Ctrl Pts',(0.178022466737198,1.83099022604891,7.76739422079178));
#61170=CARTESIAN_POINT('Ctrl Pts',(0.211479762072975,1.85528914297911,7.77015802566485));
#61171=CARTESIAN_POINT('Ctrl Pts',(0.231447870817435,1.87408188193071,7.77204784094079));
#61172=CARTESIAN_POINT('Ctrl Pts',(0.251178104135047,1.89804788902278,7.77404508414141));
#61173=CARTESIAN_POINT('Ctrl Pts',(0.253499323255273,1.90096937117097,7.77428230650393));
#61174=CARTESIAN_POINT('Ctrl Pts',(0.256123343070602,1.90439236414173,7.77455249206801));
#61175=CARTESIAN_POINT('Ctrl Pts',(0.256476034371073,1.9048550336863,7.77458885072494));
#61176=CARTESIAN_POINT('Ctrl Pts',(0.256997610600598,1.9055431073641,7.77464268096086));
#61177=CARTESIAN_POINT('Ctrl Pts',(0.257167453526111,1.9057677786865,7.77466021963864));
#61178=CARTESIAN_POINT('Ctrl Pts',(0.25746896459633,1.90616771180441,7.77469137180001));
#61179=CARTESIAN_POINT('Ctrl Pts',(0.257600748396059,1.90634288522152,7.77470499346462));
#61180=CARTESIAN_POINT('Ctrl Pts',(0.257879642140193,1.90671439271894,7.77473383303792));
#61181=CARTESIAN_POINT('Ctrl Pts',(0.258026706241336,1.90691075980373,7.77474904769641));
#61182=CARTESIAN_POINT('Ctrl Pts',(0.258414618013022,1.90742995288603,7.77478919908587));
#61183=CARTESIAN_POINT('Ctrl Pts',(0.258655085941057,1.90775306408344,7.77481410910981));
#61184=CARTESIAN_POINT('Ctrl Pts',(0.259758560345059,1.90924159539474,7.77492851451173));
#61185=CARTESIAN_POINT('Ctrl Pts',(0.260614317756808,1.91041240503098,7.77501751045227));
#61186=CARTESIAN_POINT('Ctrl Pts',(0.267325429512785,1.91972556388609,7.77571797421593));
#61187=CARTESIAN_POINT('Ctrl Pts',(0.272806346021825,1.92813232211608,7.77630552164729));
#61188=CARTESIAN_POINT('Ctrl Pts',(0.289315307935573,1.95623963039215,7.77817544973955));
#61189=CARTESIAN_POINT('Ctrl Pts',(0.298669039715419,1.97684442666317,7.77940730875144));
#61190=CARTESIAN_POINT('Ctrl Pts',(0.311068185546339,2.01411116006017,7.78163674768107));
#61191=CARTESIAN_POINT('Ctrl Pts',(0.315101211316615,2.03034789996888,7.78260776830101));
#61192=CARTESIAN_POINT('Ctrl Pts',(0.318067016899126,2.04807542151478,7.78369965197339));
#61193=CARTESIAN_POINT('Ctrl Pts',(0.318269200547256,2.0493294464078,7.78377704731128));
#61194=CARTESIAN_POINT('Ctrl Pts',(0.318541685889781,2.05108551429919,7.78388565704629));
#61195=CARTESIAN_POINT('Ctrl Pts',(0.318618226389089,2.05158658895598,7.78391667373389));
#61196=CARTESIAN_POINT('Ctrl Pts',(0.318748647138123,2.05245409849474,7.7839704187687));
#61197=CARTESIAN_POINT('Ctrl Pts',(0.318803078585654,2.05282045056614,7.78399312962639));
#61198=CARTESIAN_POINT('Ctrl Pts',(0.318914699932508,2.05358073411826,7.78404029074662));
#61199=CARTESIAN_POINT('Ctrl Pts',(0.318971791732013,2.05397467919619,7.78406474407294));
#61200=CARTESIAN_POINT('Ctrl Pts',(0.319103971868309,2.05489880825572,7.78412214670083));
#61201=CARTESIAN_POINT('Ctrl Pts',(0.319178468800585,2.05542907441529,7.78415511464611));
#61202=CARTESIAN_POINT('Ctrl Pts',(0.319411080886695,2.05711529111568,7.7842600484781));
#61203=CARTESIAN_POINT('Ctrl Pts',(0.319564239165475,2.05827190588451,7.78433217077017));
#61204=CARTESIAN_POINT('Ctrl Pts',(0.319907435102527,2.06097640924704,7.78450116414507));
#61205=CARTESIAN_POINT('Ctrl Pts',(0.320092523125963,2.06252488598625,7.78459818993511));
#61206=CARTESIAN_POINT('Ctrl Pts',(0.32188521623478,2.07850632743434,7.785602416623));
#61207=CARTESIAN_POINT('Ctrl Pts',(0.322526540231538,2.09302887188142,7.78654007058299));
#61208=CARTESIAN_POINT('Ctrl Pts',(0.321674641207534,2.12941387095035,7.78894944602776));
#61209=CARTESIAN_POINT('Ctrl Pts',(0.318936951345095,2.1511747464266,7.79044779904293));
#61210=CARTESIAN_POINT('Ctrl Pts',(0.312848697030029,2.17754900199409,7.79225948446135));
#61211=CARTESIAN_POINT('Ctrl Pts',(0.311558161917351,2.18258130013824,7.7926046746758));
#61212=CARTESIAN_POINT('Ctrl Pts',(0.309412804020751,2.19017860799573,7.79312308482443));
#61213=CARTESIAN_POINT('Ctrl Pts',(0.308646468176721,2.19276757615912,7.7932992553002));
#61214=CARTESIAN_POINT('Ctrl Pts',(0.307788388571434,2.19553807424186,7.79348703670735));
#61215=CARTESIAN_POINT('Ctrl Pts',(0.307728932355303,2.19572941011571,7.7935000014288));
#61216=CARTESIAN_POINT('Ctrl Pts',(0.307591503259304,2.19617021921587,7.79352986120156));
#61217=CARTESIAN_POINT('Ctrl Pts',(0.307513405134188,2.1964196536242,7.79354675088289));
#61218=CARTESIAN_POINT('Ctrl Pts',(0.306153450925803,2.20074469634268,7.79383948928161));
#61219=CARTESIAN_POINT('Ctrl Pts',(0.304790898013345,2.20479476246311,7.79411179324649));
#61220=CARTESIAN_POINT('Ctrl Pts',(0.303164109932842,2.20932975390627,7.79441369604927));
#61221=CARTESIAN_POINT('Ctrl Pts',(0.302978790013457,2.20984227534452,7.79444777184432));
#61222=CARTESIAN_POINT('Ctrl Pts',(0.302696833853365,2.21061591167039,7.79449913950461));
#61223=CARTESIAN_POINT('Ctrl Pts',(0.302601159055137,2.21087737226075,7.79451648799274));
#61224=CARTESIAN_POINT('Ctrl Pts',(0.302434407635974,2.21133124798399,7.7945465825807));
#61225=CARTESIAN_POINT('Ctrl Pts',(0.302363486115709,2.21152371929007,7.79455933795447));
#61226=CARTESIAN_POINT('Ctrl Pts',(0.3022147513561,2.21192618030643,7.79458599569032));
#61227=CARTESIAN_POINT('Ctrl Pts',(0.302136903039917,2.21213615651077,7.79459989585083));
#61228=CARTESIAN_POINT('Ctrl Pts',(0.301981259876219,2.21255462598113,7.79462758236381));
#61229=CARTESIAN_POINT('Ctrl Pts',(0.301903467707945,2.21276312044642,7.79464136889677));
#61230=CARTESIAN_POINT('Ctrl Pts',(0.301631485066761,2.21348977504726,7.79468939189644));
#61231=CARTESIAN_POINT('Ctrl Pts',(0.301436174642718,2.21400751927559,7.79472356151797));
#61232=CARTESIAN_POINT('Ctrl Pts',(0.299666496691615,2.21866238118381,7.79503036792827));
#61233=CARTESIAN_POINT('Ctrl Pts',(0.298008286421634,2.22276740592593,7.79529808048655));
#61234=CARTESIAN_POINT('Ctrl Pts',(0.292937673050119,2.23461132767112,7.79606574579406));
#61235=CARTESIAN_POINT('Ctrl Pts',(0.289304453078017,2.2422520476952,7.79655501470293));
#61236=CARTESIAN_POINT('Ctrl Pts',(0.277746558924407,2.2642788663434,7.79797239992448));
#61237=CARTESIAN_POINT('Ctrl Pts',(0.269018651123098,2.27821251223945,7.79887907141783));
#61238=CARTESIAN_POINT('Ctrl Pts',(0.246707911063124,2.30843092604645,7.80098954235841));
#61239=CARTESIAN_POINT('Ctrl Pts',(0.232507740680082,2.32416108773845,7.80220099347435));
#61240=CARTESIAN_POINT('Ctrl Pts',(0.215909414530784,2.33926134355247,7.80356386064021));
#61241=CARTESIAN_POINT('Ctrl Pts',(0.214942481842434,2.34013037130609,7.80364306359823));
#61242=CARTESIAN_POINT('Ctrl Pts',(0.213587487072899,2.34133342723037,7.80375380032486));
#61243=CARTESIAN_POINT('Ctrl Pts',(0.213203838107999,2.34167242528703,7.80378512596495));
#61244=CARTESIAN_POINT('Ctrl Pts',(0.212540261190554,2.34225596206613,7.80383926077788));
#61245=CARTESIAN_POINT('Ctrl Pts',(0.212260714144713,2.34250093404446,7.80386205185047));
#61246=CARTESIAN_POINT('Ctrl Pts',(0.211681533731948,2.34300671122778,7.80390924207554));
#61247=CARTESIAN_POINT('Ctrl Pts',(0.211381840817271,2.34326744705232,7.80393364405347));
#61248=CARTESIAN_POINT('Ctrl Pts',(0.210680797992579,2.34387508771395,7.80399068775535));
#61249=CARTESIAN_POINT('Ctrl Pts',(0.210279072955018,2.34422155621912,7.8040233474448));
#61250=CARTESIAN_POINT('Ctrl Pts',(0.209015848393551,2.34530559908987,7.80412595773305));
#61251=CARTESIAN_POINT('Ctrl Pts',(0.208151316940547,2.34603961272067,7.80419605459133));
#61252=CARTESIAN_POINT('Ctrl Pts',(0.200781098066636,2.35223050530183,7.80479258925983));
#61253=CARTESIAN_POINT('Ctrl Pts',(0.194066507643606,2.35743241013519,7.80532930185445));
#61254=CARTESIAN_POINT('Ctrl Pts',(0.181019659289397,2.36673929792265,7.80636118000203));
#61255=CARTESIAN_POINT('Ctrl Pts',(0.174733230890601,2.37089897509574,7.8068538961858));
#61256=CARTESIAN_POINT('Ctrl Pts',(0.153149799494756,2.38411656192535,7.80852888650995));
#61257=CARTESIAN_POINT('Ctrl Pts',(0.137251281498932,2.39212854808915,7.80973767408629));
#61258=CARTESIAN_POINT('Ctrl Pts',(0.10560827789721,2.40491913236995,7.8120411096631));
#61259=CARTESIAN_POINT('Ctrl Pts',(0.0899947172923275,2.40988688402467,
7.81313327882749));
#61260=CARTESIAN_POINT('Ctrl Pts',(0.0731782221931669,2.41385818805318,
7.81422001269156));
#61261=CARTESIAN_POINT('Ctrl Pts',(0.0722859806585192,2.41406488415594,
7.81427740821395));
#61262=CARTESIAN_POINT('Ctrl Pts',(0.0710857753133844,2.41433753727323,
7.81435424870901));
#61263=CARTESIAN_POINT('Ctrl Pts',(0.0707785895888558,2.41440684796736,
7.81437388347206));
#61264=CARTESIAN_POINT('Ctrl Pts',(0.0702615142085858,2.41452272011223,
7.81440687939338));
#61265=CARTESIAN_POINT('Ctrl Pts',(0.0700516795127248,2.41456952179725,
7.81442025436745));
#61266=CARTESIAN_POINT('Ctrl Pts',(0.069649367517086,2.41465883124986,7.81444586875617));
#61267=CARTESIAN_POINT('Ctrl Pts',(0.0694568994500815,2.41470137209441,
7.81445810998107));
#61268=CARTESIAN_POINT('Ctrl Pts',(0.0690015932658903,2.4148015694989,7.81448703785629));
#61269=CARTESIAN_POINT('Ctrl Pts',(0.068738722207993,2.41485907340059,7.81450371560332));
#61270=CARTESIAN_POINT('Ctrl Pts',(0.0679777301039346,2.41502454446437,
7.81455192849065));
#61271=CARTESIAN_POINT('Ctrl Pts',(0.0674794216712453,2.41513165988902,
7.81458341476739));
#61272=CARTESIAN_POINT('Ctrl Pts',(0.0639306184851298,2.41588570028342,
7.81480706505685));
#61273=CARTESIAN_POINT('Ctrl Pts',(0.0608709965770389,2.41648953086046,
7.81499680913416));
#61274=CARTESIAN_POINT('Ctrl Pts',(0.0524138916075015,2.41803139301057,
7.81551402478171));
#61275=CARTESIAN_POINT('Ctrl Pts',(0.0470003206310586,2.41887640251969,
7.81583701016565));
#61276=CARTESIAN_POINT('Ctrl Pts',(0.0260955798092798,2.42159544026768,
7.81706218971309));
#61277=CARTESIAN_POINT('Ctrl Pts',(0.0104967851393392,2.42248177316093,
7.81793086150959));
#61278=CARTESIAN_POINT('Ctrl Pts',(-0.0311254436506786,2.42182227345409,
7.82025774231299));
#61279=CARTESIAN_POINT('Ctrl Pts',(-0.0569949724175114,2.41826039531,7.82172144340392));
#61280=CARTESIAN_POINT('Ctrl Pts',(-0.0836205209930331,2.41124120296321,
7.82339137909399));
#61281=CARTESIAN_POINT('Ctrl Pts',(-0.0850849650266446,2.41084405504504,
7.82348373086133));
#61282=CARTESIAN_POINT('Ctrl Pts',(-0.087073165000146,2.41028976531911,
7.82360981513051));
#61283=CARTESIAN_POINT('Ctrl Pts',(-0.087599422318235,2.41014160592967,
7.82364325563485));
#61284=CARTESIAN_POINT('Ctrl Pts',(-0.0884918496502678,2.40988790455496,
7.82370007914616));
#61285=CARTESIAN_POINT('Ctrl Pts',(-0.0888582153931184,2.40978305053556,
7.82372343972041));
#61286=CARTESIAN_POINT('Ctrl Pts',(-0.0895644599052865,2.409579567143,7.82376853595656));
#61287=CARTESIAN_POINT('Ctrl Pts',(-0.0899043640735989,2.4094810271883,
7.82379026867599));
#61288=CARTESIAN_POINT('Ctrl Pts',(-0.0907075025220222,2.4092467584632,
7.82384168759514));
#61289=CARTESIAN_POINT('Ctrl Pts',(-0.0911705945694027,2.40911054869678,
7.82387138946149));
#61290=CARTESIAN_POINT('Ctrl Pts',(-0.0921270068576774,2.40882690189701,
7.82393284344144));
#61291=CARTESIAN_POINT('Ctrl Pts',(-0.0926202829979628,2.40867932211327,
7.82396460015662));
#61292=CARTESIAN_POINT('Ctrl Pts',(-0.0953313940116427,2.40786112042951,
7.82413947939449));
#61293=CARTESIAN_POINT('Ctrl Pts',(-0.0975422548252596,2.4071677916532,
7.8242833441271));
#61294=CARTESIAN_POINT('Ctrl Pts',(-0.10326193876419,2.40530611479243,7.82465887785764));
#61295=CARTESIAN_POINT('Ctrl Pts',(-0.106758390033697,2.40410112800867,
7.8248917377807));
#61296=CARTESIAN_POINT('Ctrl Pts',(-0.122024532935296,2.39854421102713,
7.82592332641025));
#61297=CARTESIAN_POINT('Ctrl Pts',(-0.133553760828635,2.39356764433169,
7.82674224145896));
#61298=CARTESIAN_POINT('Ctrl Pts',(-0.156552798271399,2.38200451497779,
7.82845473999739));
#61299=CARTESIAN_POINT('Ctrl Pts',(-0.167967363648404,2.37535841787191,
7.8293484479648));
#61300=CARTESIAN_POINT('Ctrl Pts',(-0.194637220954538,2.35755324445342,
7.83151783137158));
#61301=CARTESIAN_POINT('Ctrl Pts',(-0.209384019391688,2.34571494708776,
7.8327892954898));
#61302=CARTESIAN_POINT('Ctrl Pts',(-0.223828972014007,2.33186860541699,
7.83405051977083));
#61303=CARTESIAN_POINT('Ctrl Pts',(-0.224642633234347,2.33108038929128,
7.8341216133455));
#61304=CARTESIAN_POINT('Ctrl Pts',(-0.225725065035867,2.33002068716734,
7.83421623790147));
#61305=CARTESIAN_POINT('Ctrl Pts',(-0.225997520919612,2.32975300227019,
7.83424005961378));
#61306=CARTESIAN_POINT('Ctrl Pts',(-0.226422585834484,2.3293338929733,7.83427722979112));
#61307=CARTESIAN_POINT('Ctrl Pts',(-0.226575519197391,2.32918280027819,
7.83429060427191));
#61308=CARTESIAN_POINT('Ctrl Pts',(-0.226868386514299,2.328892878177,7.8343162182744));
#61309=CARTESIAN_POINT('Ctrl Pts',(-0.227008343269147,2.32875407442538,
7.83432845960528));
#61310=CARTESIAN_POINT('Ctrl Pts',(-0.227339068855871,2.32842547102381,
7.83435738856153));
#61311=CARTESIAN_POINT('Ctrl Pts',(-0.227529727135925,2.3282355610141,7.83437406728155));
#61312=CARTESIAN_POINT('Ctrl Pts',(-0.227924005593286,2.32784184492002,
7.83440856255477));
#61313=CARTESIAN_POINT('Ctrl Pts',(-0.228127590914905,2.32763800404839,
7.83442637633619));
#61314=CARTESIAN_POINT('Ctrl Pts',(-0.229248898328521,2.32651227412544,
7.83452450502748));
#61315=CARTESIAN_POINT('Ctrl Pts',(-0.230161323089784,2.3255850908257,7.83460440538622));
#61316=CARTESIAN_POINT('Ctrl Pts',(-0.233356934308235,2.32229821771889,
7.83488453724095));
#61317=CARTESIAN_POINT('Ctrl Pts',(-0.235609732292113,2.31990910018318,
7.83508255678206));
#61318=CARTESIAN_POINT('Ctrl Pts',(-0.244540977625731,2.31014258110534,
7.83587185224763));
#61319=CARTESIAN_POINT('Ctrl Pts',(-0.250913126686691,2.30249155800404,
7.83644489805314));
#61320=CARTESIAN_POINT('Ctrl Pts',(-0.261526996009817,2.28847547709734,
7.83744196561603));
#61321=CARTESIAN_POINT('Ctrl Pts',(-0.265915241467133,2.28223189876138,
7.83786920841151));
#61322=CARTESIAN_POINT('Ctrl Pts',(-0.282611472057146,2.25658742244511,
7.83958028896554));
#61323=CARTESIAN_POINT('Ctrl Pts',(-0.293049622222281,2.23605386273079,
7.84085943326052));
#61324=CARTESIAN_POINT('Ctrl Pts',(-0.301339757035058,2.21426131099904,
7.84223922115728));
#61325=CARTESIAN_POINT('Ctrl Pts',(-0.301462776026184,2.21393634639763,
7.84225979950111));
#61326=CARTESIAN_POINT('Ctrl Pts',(-0.303612089474638,2.20823091098701,
7.84262115785176));
#61327=CARTESIAN_POINT('Ctrl Pts',(-0.305494466068497,2.20279764505322,
7.84296627853491));
#61328=CARTESIAN_POINT('Ctrl Pts',(-0.307527308421526,2.19637996020461,
7.84337611627586));
#61329=CARTESIAN_POINT('Ctrl Pts',(-0.30781988841825,2.19544138732548,7.84343610752144));
#61330=CARTESIAN_POINT('Ctrl Pts',(-0.308254890759444,2.19402312649331,
7.84352684471022));
#61331=CARTESIAN_POINT('Ctrl Pts',(-0.308400499835402,2.19354441559765,
7.84355748622322));
#61332=CARTESIAN_POINT('Ctrl Pts',(-0.308658479176102,2.19268912179596,
7.84361225908258));
#61333=CARTESIAN_POINT('Ctrl Pts',(-0.308771276825858,2.19231266799182,
7.84363637639647));
#61334=CARTESIAN_POINT('Ctrl Pts',(-0.309007915036776,2.19151761922301,
7.84368733076293));
#61335=CARTESIAN_POINT('Ctrl Pts',(-0.309131594148688,2.19109897738026,
7.84371417303347));
#61336=CARTESIAN_POINT('Ctrl Pts',(-0.309456698058431,2.18999024640339,
7.84378529366064));
#61337=CARTESIAN_POINT('Ctrl Pts',(-0.309656664210244,2.18929973526148,
7.8438296194956));
#61338=CARTESIAN_POINT('Ctrl Pts',(-0.310087463381698,2.18779327837854,
7.84392639587658));
#61339=CARTESIAN_POINT('Ctrl Pts',(-0.310317389244331,2.18697708080565,
7.84397887564971));
#61340=CARTESIAN_POINT('Ctrl Pts',(-0.310986797476033,2.18456435111375,
7.84413415057298));
#61341=CARTESIAN_POINT('Ctrl Pts',(-0.311417194025377,2.18296534688794,
7.84423723966543));
#61342=CARTESIAN_POINT('Ctrl Pts',(-0.312868146516092,2.1774043738214,7.84459642798809));
#61343=CARTESIAN_POINT('Ctrl Pts',(-0.313825532676101,2.17342647180308,
7.84485454297649));
#61344=CARTESIAN_POINT('Ctrl Pts',(-0.317894230765282,2.15498460924081,
7.84605701148127));
#61345=CARTESIAN_POINT('Ctrl Pts',(-0.320082583443454,2.14033719035447,
7.84702967888952));
#61346=CARTESIAN_POINT('Ctrl Pts',(-0.321943102381381,2.11698286673872,
7.84859929369352));
#61347=CARTESIAN_POINT('Ctrl Pts',(-0.322282578411479,2.1083490653952,7.84918328118932));
#61348=CARTESIAN_POINT('Ctrl Pts',(-0.322274871694426,2.0997124250686,7.84976774768668));
#61349=CARTESIAN_POINT('',(-0.321883070004627,2.10020594158585,8.09972265507268));
#61350=CARTESIAN_POINT('Ctrl Pts',(-0.322274871581366,2.09971229839457,
7.84976775625908));
#61351=CARTESIAN_POINT('Ctrl Pts',(-0.322258932177978,2.08185744780233,
7.85097604578122));
#61352=CARTESIAN_POINT('Ctrl Pts',(-0.320759214031128,2.06403261792786,
7.85218492979292));
#61353=CARTESIAN_POINT('Ctrl Pts',(-0.317227215097624,2.04308309014836,
7.85354975638942));
#61354=CARTESIAN_POINT('Ctrl Pts',(-0.316611681255006,2.0397531232916,7.85376492348035));
#61355=CARTESIAN_POINT('Ctrl Pts',(-0.315854814762916,2.03599129032254,
7.85400550858418));
#61356=CARTESIAN_POINT('Ctrl Pts',(-0.315764952135085,2.0355494458331,7.85403372735028));
#61357=CARTESIAN_POINT('Ctrl Pts',(-0.315616929148595,2.03482937433395,
7.85407964998335));
#61358=CARTESIAN_POINT('Ctrl Pts',(-0.315559327852224,2.03455103498279,
7.85409738517302));
#61359=CARTESIAN_POINT('Ctrl Pts',(-0.315447040121666,2.03401203566707,
7.8541316977061));
#61360=CARTESIAN_POINT('Ctrl Pts',(-0.315392398681621,2.03375136670536,
7.85414827759786));
#61361=CARTESIAN_POINT('Ctrl Pts',(-0.315296814488741,2.03329817740091,
7.8541770776898));
#61362=CARTESIAN_POINT('Ctrl Pts',(-0.315256018611684,2.03310562733237,
7.85418930631074));
#61363=CARTESIAN_POINT('Ctrl Pts',(-0.315169995147034,2.032701436713,7.85421495933809));
#61364=CARTESIAN_POINT('Ctrl Pts',(-0.315124730916052,2.03248980501274,
7.85422838156139));
#61365=CARTESIAN_POINT('Ctrl Pts',(-0.314997493993823,2.0318978283478,7.854265899938));
#61366=CARTESIAN_POINT('Ctrl Pts',(-0.314915045304004,2.03151758436582,
7.85428996870754));
#61367=CARTESIAN_POINT('Ctrl Pts',(-0.314578371219292,2.02997834709904,
7.8543872800327));
#61368=CARTESIAN_POINT('Ctrl Pts',(-0.314318430502202,2.02882059382544,
7.85446019883639));
#61369=CARTESIAN_POINT('Ctrl Pts',(-0.309515824382371,2.00796964281188,
7.85576892476597));
#61370=CARTESIAN_POINT('Ctrl Pts',(-0.303136182553172,1.98874194307644,
7.85690426773417));
#61371=CARTESIAN_POINT('Ctrl Pts',(-0.292999455965349,1.96569781215525,
7.85831268057875));
#61372=CARTESIAN_POINT('Ctrl Pts',(-0.290898593475207,1.96120602613415,
7.8585894997276));
#61373=CARTESIAN_POINT('Ctrl Pts',(-0.286540373701567,1.95242191886493,
7.85913816899843));
#61374=CARTESIAN_POINT('Ctrl Pts',(-0.284288125615973,1.94812855309445,
7.85940991992784));
#61375=CARTESIAN_POINT('Ctrl Pts',(-0.275495460623045,1.93224894047294,
7.86043294951374));
#61376=CARTESIAN_POINT('Ctrl Pts',(-0.268337097808095,1.92102145748324,
7.86119341598281));
#61377=CARTESIAN_POINT('Ctrl Pts',(-0.256910170231663,1.90533196326534,
7.86233884940617));
#61378=CARTESIAN_POINT('Ctrl Pts',(-0.2531749733236,1.9004983571356,7.86270409391885));
#61379=CARTESIAN_POINT('Ctrl Pts',(-0.248698624034314,1.89503394112871,
7.86313288381852));
#61380=CARTESIAN_POINT('Ctrl Pts',(-0.248089079704336,1.89429657419839,
7.86319108844901));
#61381=CARTESIAN_POINT('Ctrl Pts',(-0.247109567352257,1.8931223427714,7.86328433414638));
#61382=CARTESIAN_POINT('Ctrl Pts',(-0.246741699692676,1.89268372721,7.86331928979842));
#61383=CARTESIAN_POINT('Ctrl Pts',(-0.246034663581908,1.8918452622313,7.86338635328193));
#61384=CARTESIAN_POINT('Ctrl Pts',(-0.245695683866944,1.89144525547607,
7.86341845333226));
#61385=CARTESIAN_POINT('Ctrl Pts',(-0.24509880589746,1.89074439554351,7.86347488391181));
#61386=CARTESIAN_POINT('Ctrl Pts',(-0.244841325437408,1.89044318669011,
7.86349919720603));
#61387=CARTESIAN_POINT('Ctrl Pts',(-0.244340103315882,1.88985902586917,
7.86354646937504));
#61388=CARTESIAN_POINT('Ctrl Pts',(-0.24409642394058,1.8895760210559,7.86356942565344));
#61389=CARTESIAN_POINT('Ctrl Pts',(-0.24344602015584,1.88882330395995,7.8636306293497));
#61390=CARTESIAN_POINT('Ctrl Pts',(-0.243038429856108,1.88835434499014,
7.86366891265978));
#61391=CARTESIAN_POINT('Ctrl Pts',(-0.24157557931191,1.8866810389704,7.86380606034529));
#61392=CARTESIAN_POINT('Ctrl Pts',(-0.240512715969049,1.88548339699866,
7.86390524162596));
#61393=CARTESIAN_POINT('Ctrl Pts',(-0.221774834238887,1.86468373663772,
7.86564587480005));
#61394=CARTESIAN_POINT('Ctrl Pts',(-0.20177052469913,1.84732256586555,7.86739519596161));
#61395=CARTESIAN_POINT('Ctrl Pts',(-0.172347192043686,1.82752975350544,
7.86979298453034));
#61396=CARTESIAN_POINT('Ctrl Pts',(-0.164603854095112,1.82278318159002,
7.87040856968137));
#61397=CARTESIAN_POINT('Ctrl Pts',(-0.147342991688531,1.8131809930222,7.87173644584256));
#61398=CARTESIAN_POINT('Ctrl Pts',(-0.137762692351258,1.80845826870893,
7.87244597945534));
#61399=CARTESIAN_POINT('Ctrl Pts',(-0.125567137491608,1.8031820508526,7.87330155634401));
#61400=CARTESIAN_POINT('Ctrl Pts',(-0.123156768891748,1.80217385571919,
7.87346840191766));
#61401=CARTESIAN_POINT('Ctrl Pts',(-0.119319230421289,1.80062327029458,
7.87373018491216));
#61402=CARTESIAN_POINT('Ctrl Pts',(-0.117900062024642,1.80006153859348,
7.87382616988519));
#61403=CARTESIAN_POINT('Ctrl Pts',(-0.116195186491908,1.79940068935003,
7.87394044609689));
#61404=CARTESIAN_POINT('Ctrl Pts',(-0.115913294594358,1.79929187728765,
7.87395930736223));
#61405=CARTESIAN_POINT('Ctrl Pts',(-0.115423052440332,1.79910343248774,
7.87399205021005));
#61406=CARTESIAN_POINT('Ctrl Pts',(-0.115214772386363,1.7990236195314,7.87400594255496));
#61407=CARTESIAN_POINT('Ctrl Pts',(-0.114796930297791,1.79886399965439,
7.87403377542652));
#61408=CARTESIAN_POINT('Ctrl Pts',(-0.114587367160357,1.79878419497256,
7.8740477158247));
#61409=CARTESIAN_POINT('Ctrl Pts',(-0.114186269614117,1.79863193037106,
7.8740743611343));
#61410=CARTESIAN_POINT('Ctrl Pts',(-0.113994749690766,1.7985594343759,7.87408706824206));
#61411=CARTESIAN_POINT('Ctrl Pts',(-0.113543937295348,1.79838927953756,
7.87411694232161));
#61412=CARTESIAN_POINT('Ctrl Pts',(-0.1132845872233,1.79829177224778,7.87413410013843));
#61413=CARTESIAN_POINT('Ctrl Pts',(-0.112519621679996,1.79800529521695,
7.87418462460534));
#61414=CARTESIAN_POINT('Ctrl Pts',(-0.112013653656151,1.79781725994929,
7.87421793556288));
#61415=CARTESIAN_POINT('Ctrl Pts',(-0.107632552538369,1.79620160638566,
7.87450546291387));
#61416=CARTESIAN_POINT('Ctrl Pts',(-0.103730563266756,1.79484724402656,
7.87475541420429));
#61417=CARTESIAN_POINT('Ctrl Pts',(-0.099557752997718,1.79348817936978,
7.87501731675413));
#61418=CARTESIAN_POINT('Ctrl Pts',(-0.0993120098759176,1.79340846870266,
7.87503272084469));
#61419=CARTESIAN_POINT('Ctrl Pts',(-0.0846749539895292,1.78868015293434,
7.87594906517088));
#61420=CARTESIAN_POINT('Ctrl Pts',(-0.0699727079321773,1.78504950584,7.87680324809009));
#61421=CARTESIAN_POINT('Ctrl Pts',(-0.0371963059840335,1.7793652691963,
7.87866722719831));
#61422=CARTESIAN_POINT('Ctrl Pts',(-0.0190952416640365,1.77778029876138,
7.87967193504103));
#61423=CARTESIAN_POINT('Ctrl Pts',(0.0102113351150218,1.7776932464846,7.88135666728746));
#61424=CARTESIAN_POINT('Ctrl Pts',(0.0213730601444318,1.77824066885499,
7.88201142037582));
#61425=CARTESIAN_POINT('Ctrl Pts',(0.0349971557098768,1.77962091173683,
7.8828370401502));
#61426=CARTESIAN_POINT('Ctrl Pts',(0.0375080976576649,1.77990516537533,
7.88299029258626));
#61427=CARTESIAN_POINT('Ctrl Pts',(0.0405394914810656,1.78028449483028,
7.88317670621085));
#61428=CARTESIAN_POINT('Ctrl Pts',(0.0410634350588698,1.78035136647965,
7.8832089762678));
#61429=CARTESIAN_POINT('Ctrl Pts',(0.0420754214693971,1.78048305691186,
7.88327140378583));
#61430=CARTESIAN_POINT('Ctrl Pts',(0.0425634851191913,1.78054770662511,
7.88330155583706));
#61431=CARTESIAN_POINT('Ctrl Pts',(0.0434033807515645,1.78066091954123,
7.88335352071114));
#61432=CARTESIAN_POINT('Ctrl Pts',(0.0437552851259638,1.78070894658507,
7.88337531654926));
#61433=CARTESIAN_POINT('Ctrl Pts',(0.0444805795560989,1.7808091545632,7.88342028730183));
#61434=CARTESIAN_POINT('Ctrl Pts',(0.0448539587654445,1.78086140918169,
7.88344346451782));
#61435=CARTESIAN_POINT('Ctrl Pts',(0.0457538841185101,1.78098896471327,
7.88349939076852));
#61436=CARTESIAN_POINT('Ctrl Pts',(0.0462803358973223,1.78106491404918,
7.88353216028183));
#61437=CARTESIAN_POINT('Ctrl Pts',(0.0482137010783108,1.78134872153592,
7.8836527006894));
#61438=CARTESIAN_POINT('Ctrl Pts',(0.0496194062492849,1.78156458636344,
7.88374072482089));
#61439=CARTESIAN_POINT('Ctrl Pts',(0.0749922357072826,1.7856330082916,7.88533659576262));
#61440=CARTESIAN_POINT('Ctrl Pts',(0.0984446508668024,1.79217111215096,
7.88693453538845));
#61441=CARTESIAN_POINT('Ctrl Pts',(0.137371964881999,1.80793063132598,7.88976775531084));
#61442=CARTESIAN_POINT('Ctrl Pts',(0.153230639388537,1.81592961670599,7.8909774892196));
#61443=CARTESIAN_POINT('Ctrl Pts',(0.172469956947232,1.82771591963494,7.89246428407692));
#61444=CARTESIAN_POINT('Ctrl Pts',(0.176531704672809,1.83033155766143,7.89277920322749));
#61445=CARTESIAN_POINT('Ctrl Pts',(0.183427389747883,1.83499476568953,7.89331368558763));
#61446=CARTESIAN_POINT('Ctrl Pts',(0.18628958747963,1.83699890952607,7.89353548195043));
#61447=CARTESIAN_POINT('Ctrl Pts',(0.189543088370175,1.83935681882906,7.89378701588884));
#61448=CARTESIAN_POINT('Ctrl Pts',(0.189966661559608,1.83966537351916,7.89381975147414));
#61449=CARTESIAN_POINT('Ctrl Pts',(0.190566489631344,1.84010456567569,7.89386609007485));
#61450=CARTESIAN_POINT('Ctrl Pts',(0.19074336372377,1.84023434994392,7.89387975183531));
#61451=CARTESIAN_POINT('Ctrl Pts',(0.191099087100104,1.84049592702523,7.89390722301798));
#61452=CARTESIAN_POINT('Ctrl Pts',(0.191277933162101,1.84062772455903,7.89392103212303));
#61453=CARTESIAN_POINT('Ctrl Pts',(0.191623565235151,1.84088298409545,7.89394771410498));
#61454=CARTESIAN_POINT('Ctrl Pts',(0.191790367860852,1.84100642193073,7.89396058862522));
#61455=CARTESIAN_POINT('Ctrl Pts',(0.19218806724616,1.84130132364875,7.89399127965306));
#61456=CARTESIAN_POINT('Ctrl Pts',(0.192418854411754,1.84147293602784,7.89400908574712));
#61457=CARTESIAN_POINT('Ctrl Pts',(0.193240617378158,1.84208570553367,7.89407247450046));
#61458=CARTESIAN_POINT('Ctrl Pts',(0.193830314057742,1.8425285863009,7.89411793760893));
#61459=CARTESIAN_POINT('Ctrl Pts',(0.202724822756754,1.84925651870783,7.89480338037994));
#61460=CARTESIAN_POINT('Ctrl Pts',(0.210722707799278,1.85593927249584,7.89541599658786));
#61461=CARTESIAN_POINT('Ctrl Pts',(0.228586565704996,1.87239981988116,7.89681263473243));
#61462=CARTESIAN_POINT('Ctrl Pts',(0.238172226417083,1.88245071754785,7.89758496006825));
#61463=CARTESIAN_POINT('Ctrl Pts',(0.263848382977891,1.91311157436162,7.89982070972837));
#61464=CARTESIAN_POINT('Ctrl Pts',(0.278117328138475,1.93509479545138,7.90129274457144));
#61465=CARTESIAN_POINT('Ctrl Pts',(0.29008272192339,1.95959160908565,7.90295046925214));
#61466=CARTESIAN_POINT('Ctrl Pts',(0.290582590157954,1.96062905596628,7.90302068287719));
#61467=CARTESIAN_POINT('Ctrl Pts',(0.291305358697669,1.96214991130708,7.90312363373724));
#61468=CARTESIAN_POINT('Ctrl Pts',(0.291532642641951,1.96263123634737,7.90315621892845));
#61469=CARTESIAN_POINT('Ctrl Pts',(0.291927584997375,1.96347301081714,7.90321321224776));
#61470=CARTESIAN_POINT('Ctrl Pts',(0.292095771331766,1.96383321247255,7.90323760206043));
#61471=CARTESIAN_POINT('Ctrl Pts',(0.292419717669013,1.96453036450791,7.90328481144513));
#61472=CARTESIAN_POINT('Ctrl Pts',(0.292575562896564,1.96486727481489,7.90330762802961));
#61473=CARTESIAN_POINT('Ctrl Pts',(0.292944182258829,1.9656677927261,7.90336184632108));
#61474=CARTESIAN_POINT('Ctrl Pts',(0.293156437975896,1.96613163667662,7.90339326583043));
#61475=CARTESIAN_POINT('Ctrl Pts',(0.29390119940669,1.96776943490269,7.90350422058128));
#61476=CARTESIAN_POINT('Ctrl Pts',(0.294427756465662,1.96894606643142,7.90358395986331));
#61477=CARTESIAN_POINT('Ctrl Pts',(0.302496790197261,1.98727102548914,7.90482633082116));
#61478=CARTESIAN_POINT('Ctrl Pts',(0.308535654506631,2.00503865699358,7.90604102274337));
#61479=CARTESIAN_POINT('Ctrl Pts',(0.317501653290525,2.04159242584183,7.90855253286967));
#61480=CARTESIAN_POINT('Ctrl Pts',(0.320381002975282,2.0603173631063,7.90984497495856));
#61481=CARTESIAN_POINT('Ctrl Pts',(0.322157595687597,2.08776815255019,7.91168669990593));
#61482=CARTESIAN_POINT('Ctrl Pts',(0.322369319103746,2.09636962812861,7.91225580190674));
#61483=CARTESIAN_POINT('Ctrl Pts',(0.322171496127166,2.10919606604382,7.91308342685875));
#61484=CARTESIAN_POINT('Ctrl Pts',(0.322023176726636,2.11342082261824,7.91335260906187));
#61485=CARTESIAN_POINT('Ctrl Pts',(0.321761789542182,2.11818863581479,7.91365161772659));
#61486=CARTESIAN_POINT('Ctrl Pts',(0.321730409049222,2.11873551669189,7.91368584372121));
#61487=CARTESIAN_POINT('Ctrl Pts',(0.321681055505062,2.11955890924342,7.91373726514261));
#61488=CARTESIAN_POINT('Ctrl Pts',(0.321664120151505,2.11983547857213,7.91375451842785));
#61489=CARTESIAN_POINT('Ctrl Pts',(0.321634463203355,2.12030977503769,7.91378407416897));
#61490=CARTESIAN_POINT('Ctrl Pts',(0.321621915959067,2.12050751222978,7.91379638647316));
#61491=CARTESIAN_POINT('Ctrl Pts',(0.321595603366356,2.12091621900285,7.9138218149182));
#61492=CARTESIAN_POINT('Ctrl Pts',(0.321581812813738,2.12112718604032,7.91383492958663));
#61493=CARTESIAN_POINT('Ctrl Pts',(0.321543705029712,2.12170147399554,7.9138706002601));
#61494=CARTESIAN_POINT('Ctrl Pts',(0.321518979522512,2.12206476892519,7.91389313321644));
#61495=CARTESIAN_POINT('Ctrl Pts',(0.321423564658934,2.12343248962119,7.91397784539681));
#61496=CARTESIAN_POINT('Ctrl Pts',(0.321348782927495,2.12443663770256,7.91403979708322));
#61497=CARTESIAN_POINT('Ctrl Pts',(0.319855870133592,2.14328957994406,7.91519867320213));
#61498=CARTESIAN_POINT('Ctrl Pts',(0.316957151100179,2.16099288480806,7.91621576110948));
#61499=CARTESIAN_POINT('Ctrl Pts',(0.305065577006273,2.20842838594641,7.91896009332865));
#61500=CARTESIAN_POINT('Ctrl Pts',(0.29323380259033,2.23724233499828,7.92066539462707));
#61501=CARTESIAN_POINT('Ctrl Pts',(0.276447241611424,2.26565672543972,7.92266108121648));
#61502=CARTESIAN_POINT('Ctrl Pts',(0.275407105148127,2.26738026833172,7.92278338833579));
#61503=CARTESIAN_POINT('Ctrl Pts',(0.27400307467952,2.26965827469059,7.92294675948895));
#61504=CARTESIAN_POINT('Ctrl Pts',(0.273653503179996,2.27022154767181,7.92298729650321));
#61505=CARTESIAN_POINT('Ctrl Pts',(0.273077483030194,2.27114334255704,7.92305386836502));
#61506=CARTESIAN_POINT('Ctrl Pts',(0.27285205913344,2.27150250512346,7.9230798653094));
#61507=CARTESIAN_POINT('Ctrl Pts',(0.272414409501804,2.27219675503421,7.9231302300102));
#61508=CARTESIAN_POINT('Ctrl Pts',(0.272202272617804,2.27253189771168,7.92315459444175));
#61509=CARTESIAN_POINT('Ctrl Pts',(0.271711807710557,2.27330359842089,7.9232108150113));
#61510=CARTESIAN_POINT('Ctrl Pts',(0.271433045861665,2.27373987822097,7.92324268723768));
#61511=CARTESIAN_POINT('Ctrl Pts',(0.270539973869678,2.27513019651722,7.9233445389832));
#61512=CARTESIAN_POINT('Ctrl Pts',(0.269921680961147,2.2760816551714,7.92341466691436));
#61513=CARTESIAN_POINT('Ctrl Pts',(0.264300602926611,2.28463245881778,7.9240488014076));
#61514=CARTESIAN_POINT('Ctrl Pts',(0.258983579072112,2.29201935412604,7.92462463863247));
#61515=CARTESIAN_POINT('Ctrl Pts',(0.249886318203063,2.30359181178599,7.92557471837433));
#61516=CARTESIAN_POINT('Ctrl Pts',(0.246296043712791,2.30792078077566,7.92594177541064));
#61517=CARTESIAN_POINT('Ctrl Pts',(0.225474136926969,2.33173034383116,7.92802627813301));
#61518=CARTESIAN_POINT('Ctrl Pts',(0.206049340942353,2.34916058980704,7.92981807853498));
#61519=CARTESIAN_POINT('Ctrl Pts',(0.177424243971776,2.36918691121252,7.93213627465463));
#61520=CARTESIAN_POINT('Ctrl Pts',(0.169895068998796,2.37400119232201,7.93271909344267));
#61521=CARTESIAN_POINT('Ctrl Pts',(0.161003271363964,2.37917908293114,7.93336889858684));
#61522=CARTESIAN_POINT('Ctrl Pts',(0.15982735262647,2.37985394626998,7.93345408126176));
#61523=CARTESIAN_POINT('Ctrl Pts',(0.15830568088081,2.38071451860004,7.93356330836455));
#61524=CARTESIAN_POINT('Ctrl Pts',(0.157963821577807,2.38090703200243,7.93358778254492));
#61525=CARTESIAN_POINT('Ctrl Pts',(0.157409703889777,2.38121774440651,7.93362734667651));
#61526=CARTESIAN_POINT('Ctrl Pts',(0.157197663226957,2.38133632777278,7.93364246137268));
#61527=CARTESIAN_POINT('Ctrl Pts',(0.156793569883267,2.38156171678587,7.93367121798969));
#61528=CARTESIAN_POINT('Ctrl Pts',(0.156601543653029,2.38166856488058,7.93368486256854));
#61529=CARTESIAN_POINT('Ctrl Pts',(0.156163475179066,2.38191173044604,7.93371594307616));
#61530=CARTESIAN_POINT('Ctrl Pts',(0.155917363996643,2.38204792207862,7.9337333708238));
#61531=CARTESIAN_POINT('Ctrl Pts',(0.155149764107383,2.38247138048533,7.93378762288085));
#61532=CARTESIAN_POINT('Ctrl Pts',(0.154627653655933,2.38275752657373,7.93382437552342));
#61533=CARTESIAN_POINT('Ctrl Pts',(0.150559087996966,2.38497269175915,7.93410963925556));
#61534=CARTESIAN_POINT('Ctrl Pts',(0.14697726624696,2.38683647064676,7.93435409292421));
#61535=CARTESIAN_POINT('Ctrl Pts',(0.142956236081539,2.38883367984733,7.93462221551448));
#61536=CARTESIAN_POINT('Ctrl Pts',(0.142550876936337,2.38903395568328,7.93464917444293));
#61537=CARTESIAN_POINT('Ctrl Pts',(0.141334512184778,2.38963174382366,7.93472986333274));
#61538=CARTESIAN_POINT('Ctrl Pts',(0.140522249355728,2.39002670365849,7.93478347040678));
#61539=CARTESIAN_POINT('Ctrl Pts',(0.138267128069659,2.39111155017826,7.93493157003802));
#61540=CARTESIAN_POINT('Ctrl Pts',(0.136820762216312,2.39179412700156,7.93502572992031));
#61541=CARTESIAN_POINT('Ctrl Pts',(0.132740678451923,2.39368261469346,7.93528919456026));
#61542=CARTESIAN_POINT('Ctrl Pts',(0.130095652471343,2.39486384650226,7.93545748973609));
#61543=CARTESIAN_POINT('Ctrl Pts',(0.107461645344667,2.40460801559988,7.93687934773295));
#61544=CARTESIAN_POINT('Ctrl Pts',(0.0866683002105105,2.41116357892471,
7.93806878319673));
#61545=CARTESIAN_POINT('Ctrl Pts',(0.0549097768024357,2.41774242499981,
7.9398999275065));
#61546=CARTESIAN_POINT('Ctrl Pts',(0.0443468393510754,2.41938795235659,
7.94051059119462));
#61547=CARTESIAN_POINT('Ctrl Pts',(0.0260817354073458,2.42130973074655,
7.94158585419155));
#61548=CARTESIAN_POINT('Ctrl Pts',(0.0184154012885111,2.4218401133452,7.94204287624618));
#61549=CARTESIAN_POINT('Ctrl Pts',(0.00913806175046046,2.42214939654715,
7.9426056456217));
#61550=CARTESIAN_POINT('Ctrl Pts',(0.00753789751668553,2.42219080965365,
7.94270305724656));
#61551=CARTESIAN_POINT('Ctrl Pts',(0.00533588394085926,2.42223138588347,
7.94283760223657));
#61552=CARTESIAN_POINT('Ctrl Pts',(0.00473422794086623,2.42224078696507,
7.94287441478547));
#61553=CARTESIAN_POINT('Ctrl Pts',(0.00372178955027446,2.42225377059293,
7.94293644798275));
#61554=CARTESIAN_POINT('Ctrl Pts',(0.00331101857959443,2.42225825285368,
7.94296164039817));
#61555=CARTESIAN_POINT('Ctrl Pts',(0.00250066928757386,2.42226554570591,
7.94301138663945));
#61556=CARTESIAN_POINT('Ctrl Pts',(0.00210109200908594,2.42226839855328,
7.94303593909606));
#61557=CARTESIAN_POINT('Ctrl Pts',(0.00122335238087326,2.42227303281044,
7.94308992360258));
#61558=CARTESIAN_POINT('Ctrl Pts',(0.000745189921370165,2.42227449318234,
7.94311936565926));
#61559=CARTESIAN_POINT('Ctrl Pts',(-0.000909951061609263,2.42227586458622,
7.94322139406877));
#61560=CARTESIAN_POINT('Ctrl Pts',(-0.002086913932684,2.42227039211981,
7.94329414882692));
#61561=CARTESIAN_POINT('Ctrl Pts',(-0.0137774730839854,2.42215199107151,
7.9440188673165));
#61562=CARTESIAN_POINT('Ctrl Pts',(-0.0242785074332012,2.42153108221361,
7.9446867072892));
#61563=CARTESIAN_POINT('Ctrl Pts',(-0.0404548765975516,2.41977764674232,
7.94574310583009));
#61564=CARTESIAN_POINT('Ctrl Pts',(-0.0461622976310948,2.41900372557221,
7.94612114172282));
#61565=CARTESIAN_POINT('Ctrl Pts',(-0.0724682015490074,2.41471593984277,
7.94788663715116));
#61566=CARTESIAN_POINT('Ctrl Pts',(-0.0927143413632195,2.40935692994802,
7.94931567080794));
#61567=CARTESIAN_POINT('Ctrl Pts',(-0.124781816505537,2.39743584391792,
7.95161010768108));
#61568=CARTESIAN_POINT('Ctrl Pts',(-0.136968519178387,2.39202448964841,
7.95248872204807));
#61569=CARTESIAN_POINT('Ctrl Pts',(-0.149380189184174,2.38556467289061,
7.95336617278646));
#61570=CARTESIAN_POINT('Ctrl Pts',(-0.149972758908458,2.38525391308138,
7.95340802074615));
#61571=CARTESIAN_POINT('Ctrl Pts',(-0.150828075396917,2.38480195971763,
7.95346835555974));
#61572=CARTESIAN_POINT('Ctrl Pts',(-0.15109159572406,2.38466224598675,7.95348693507904));
#61573=CARTESIAN_POINT('Ctrl Pts',(-0.151550532338594,2.38441810924009,
7.95351927545306));
#61574=CARTESIAN_POINT('Ctrl Pts',(-0.151746035254182,2.38431385035144,
7.95353304677546));
#61575=CARTESIAN_POINT('Ctrl Pts',(-0.152125306120398,2.38411108801945,
7.95355975215387));
#61576=CARTESIAN_POINT('Ctrl Pts',(-0.152309085463493,2.38401260814218,
7.95357268767051));
#61577=CARTESIAN_POINT('Ctrl Pts',(-0.1527494200689,2.38377610041267,7.95360366984434));
#61578=CARTESIAN_POINT('Ctrl Pts',(-0.153005884541916,2.38363790260454,
7.9536217056325));
#61579=CARTESIAN_POINT('Ctrl Pts',(-0.153786694861446,2.38321578990748,
7.95367658896102));
#61580=CARTESIAN_POINT('Ctrl Pts',(-0.154310444212702,2.38293076536419,
7.9537133663687));
#61581=CARTESIAN_POINT('Ctrl Pts',(-0.160050479431413,2.37978635651616,
7.95411605489116));
#61582=CARTESIAN_POINT('Ctrl Pts',(-0.165187836793753,2.37678430380563,
7.95447307178854));
#61583=CARTESIAN_POINT('Ctrl Pts',(-0.170360685129585,2.37356613999067,
7.95483211706501));
#61584=CARTESIAN_POINT('Ctrl Pts',(-0.170481797560588,2.37349068117173,
7.95484052317632));
#61585=CARTESIAN_POINT('Ctrl Pts',(-0.182947339921855,2.36571255607436,
7.95570570353242));
#61586=CARTESIAN_POINT('Ctrl Pts',(-0.194757159022596,2.35718206897935,
7.95652368609568));
#61587=CARTESIAN_POINT('Ctrl Pts',(-0.215347442424132,2.34007478333718,
7.95802167416347));
#61588=CARTESIAN_POINT('Ctrl Pts',(-0.224292416405225,2.33173978105501,
7.95870150368423));
#61589=CARTESIAN_POINT('Ctrl Pts',(-0.243749195134019,2.31142544222842,
7.9602949519516));
#61590=CARTESIAN_POINT('Ctrl Pts',(-0.253888320057476,2.29913565459063,
7.96121557017588));
#61591=CARTESIAN_POINT('Ctrl Pts',(-0.264518388113055,2.2841125160232,7.96232540748322));
#61592=CARTESIAN_POINT('Ctrl Pts',(-0.265935288851899,2.28205992917191,
7.96247669224427));
#61593=CARTESIAN_POINT('Ctrl Pts',(-0.267725928230209,2.279400418427,7.96267234201996));
#61594=CARTESIAN_POINT('Ctrl Pts',(-0.268121701952594,2.27880837706252,
7.96271587294973));
#61595=CARTESIAN_POINT('Ctrl Pts',(-0.268756070509483,2.2778525778087,7.96278611451706));
#61596=CARTESIAN_POINT('Ctrl Pts',(-0.268995898340527,2.27748963784382,
7.96281277876174));
#61597=CARTESIAN_POINT('Ctrl Pts',(-0.269451159659886,2.27679763255968,
7.96286360355131));
#61598=CARTESIAN_POINT('Ctrl Pts',(-0.269666727203407,2.27646865602137,
7.96288775901338));
#61599=CARTESIAN_POINT('Ctrl Pts',(-0.270156660806904,2.2757179767614,7.96294286423652));
#61600=CARTESIAN_POINT('Ctrl Pts',(-0.27043064220822,2.27529602529929,7.96297382829223));
#61601=CARTESIAN_POINT('Ctrl Pts',(-0.271262646656974,2.27400808453257,
7.96306831135616));
#61602=CARTESIAN_POINT('Ctrl Pts',(-0.271817502237051,2.27314006582006,
7.96313194801796));
#61603=CARTESIAN_POINT('Ctrl Pts',(-0.275810554755725,2.26682681232695,
7.96359451411695));
#61604=CARTESIAN_POINT('Ctrl Pts',(-0.279088802291413,2.26128260356565,
7.96399930246104));
#61605=CARTESIAN_POINT('Ctrl Pts',(-0.283036697898372,2.2541246726383,7.96452065743821));
#61606=CARTESIAN_POINT('Ctrl Pts',(-0.283862494322685,2.25259839844246,
7.96463175155426));
#61607=CARTESIAN_POINT('Ctrl Pts',(-0.286775971722933,2.24710808762827,
7.96503112148844));
#61608=CARTESIAN_POINT('Ctrl Pts',(-0.28879319864089,2.24310741718386,7.96532166545972));
#61609=CARTESIAN_POINT('Ctrl Pts',(-0.30174725267772,2.21602617207257,7.96728485773741));
#61610=CARTESIAN_POINT('Ctrl Pts',(-0.309989515824185,2.19175892271045,
7.96903713270421));
#61611=CARTESIAN_POINT('Ctrl Pts',(-0.31763907958223,2.15564304431348,7.97150799990326));
#61612=CARTESIAN_POINT('Ctrl Pts',(-0.319406302270793,2.14438926152066,
7.97225792046781));
#61613=CARTESIAN_POINT('Ctrl Pts',(-0.32068021565817,2.1320380932898,7.97304347750477));
#61614=CARTESIAN_POINT('Ctrl Pts',(-0.320781142646429,2.13101126771642,
7.97310850305196));
#61615=CARTESIAN_POINT('Ctrl Pts',(-0.320946673354063,2.1292398198769,7.97322017580404));
#61616=CARTESIAN_POINT('Ctrl Pts',(-0.321013620552848,2.12849543208073,
7.97326694799747));
#61617=CARTESIAN_POINT('Ctrl Pts',(-0.321104849460066,2.12743990996202,
7.97333304460863));
#61618=CARTESIAN_POINT('Ctrl Pts',(-0.321131269090855,2.12712897011615,
7.97335248793103));
#61619=CARTESIAN_POINT('Ctrl Pts',(-0.321175876291508,2.12659477926577,
7.97338584321219));
#61620=CARTESIAN_POINT('Ctrl Pts',(-0.321194282787789,2.1263715471935,7.9733997675622));
#61621=CARTESIAN_POINT('Ctrl Pts',(-0.321229095117471,2.12594390347759,
7.97342641445788));
#61622=CARTESIAN_POINT('Ctrl Pts',(-0.321245538554226,2.12573949566795,
7.97343913913755));
#61623=CARTESIAN_POINT('Ctrl Pts',(-0.321283829968317,2.12525774381251,
7.97346910049723));
#61624=CARTESIAN_POINT('Ctrl Pts',(-0.321305513989276,2.12498038636707,
7.97348632788842));
#61625=CARTESIAN_POINT('Ctrl Pts',(-0.321368550280487,2.12416043525954,
7.97353719258001));
#61626=CARTESIAN_POINT('Ctrl Pts',(-0.321408887730428,2.12361776110019,
7.9735707731226));
#61627=CARTESIAN_POINT('Ctrl Pts',(-0.321752120898366,2.11883632461891,
7.97386593130243));
#61628=CARTESIAN_POINT('Ctrl Pts',(-0.321972541793684,2.1145918126738,7.97412299043251));
#61629=CARTESIAN_POINT('Ctrl Pts',(-0.322138624691726,2.10942001207882,
7.97443152541405));
#61630=CARTESIAN_POINT('Ctrl Pts',(-0.32216431984864,2.10849595194501,7.9744864703627));
#61631=CARTESIAN_POINT('Ctrl Pts',(-0.322189581817633,2.10742103305464,
7.97455018702444));
#61632=CARTESIAN_POINT('Ctrl Pts',(-0.32219301886017,2.10727027931688,7.97455911853231));
#61633=CARTESIAN_POINT('Ctrl Pts',(-0.322203769155405,2.10678377117518,
7.97458792755029));
#61634=CARTESIAN_POINT('Ctrl Pts',(-0.322210663417825,2.10644800673407,
7.97460778787639));
#61635=CARTESIAN_POINT('Ctrl Pts',(-0.322243049164172,2.10474073498525,
7.97470866180329));
#61636=CARTESIAN_POINT('Ctrl Pts',(-0.322260309064804,2.10336906707049,
7.97478934413744));
#61637=CARTESIAN_POINT('Ctrl Pts',(-0.322272586116957,2.10138814841775,
7.97490539229644));
#61638=CARTESIAN_POINT('Ctrl Pts',(-0.322274634324835,2.10077897251971,
7.97494101537436));
#61639=CARTESIAN_POINT('Ctrl Pts',(-0.322278855065594,2.09276771086691,
7.97540869041609));
#61640=CARTESIAN_POINT('Ctrl Pts',(-0.32202773443698,2.08536728885032,7.97583171717467));
#61641=CARTESIAN_POINT('Ctrl Pts',(-0.319167646610688,2.04360284295726,
7.97819942833365));
#61642=CARTESIAN_POINT('Ctrl Pts',(-0.311315845336575,2.00982780241766,
7.98006769064258));
#61643=CARTESIAN_POINT('Ctrl Pts',(-0.298120433186201,1.97758461131722,
7.98217448017197));
#61644=CARTESIAN_POINT('Ctrl Pts',(-0.29797586204607,1.97723312455924,7.98219748383168));
#61645=CARTESIAN_POINT('Ctrl Pts',(-0.29718658971003,1.97532382365179,7.98232264548775));
#61646=CARTESIAN_POINT('Ctrl Pts',(-0.296530302786638,1.97377085354978,
7.98242518812886));
#61647=CARTESIAN_POINT('Ctrl Pts',(-0.295610154105342,1.97164028873369,
7.9825669159028));
#61648=CARTESIAN_POINT('Ctrl Pts',(-0.295356717537208,1.97105819885271,
7.98260574538362));
#61649=CARTESIAN_POINT('Ctrl Pts',(-0.294950410957761,1.97013248232345,
7.98266767100056));
#61650=CARTESIAN_POINT('Ctrl Pts',(-0.294798655657859,1.96978836575791,
7.98269072896484));
#61651=CARTESIAN_POINT('Ctrl Pts',(-0.294502278353795,1.96911948174347,
7.98273562339036));
#61652=CARTESIAN_POINT('Ctrl Pts',(-0.294357720570051,1.9687946862588,7.98275745762591));
#61653=CARTESIAN_POINT('Ctrl Pts',(-0.294010706762027,1.96801846831673,
7.98280972140552));
#61654=CARTESIAN_POINT('Ctrl Pts',(-0.293807748541964,1.96756727259281,
7.98284016816148));
#61655=CARTESIAN_POINT('Ctrl Pts',(-0.293196067167288,1.96621577287938,
7.98293157021642));
#61656=CARTESIAN_POINT('Ctrl Pts',(-0.292784241760667,1.96531688684037,
7.98299263219577));
#61657=CARTESIAN_POINT('Ctrl Pts',(-0.289106971866324,1.95738712978435,
7.98353372389257));
#61658=CARTESIAN_POINT('Ctrl Pts',(-0.285593214855551,1.95047484898909,
7.98402232911353));
#61659=CARTESIAN_POINT('Ctrl Pts',(-0.278630521139103,1.93792028600481,
7.9849428633235));
#61660=CARTESIAN_POINT('Ctrl Pts',(-0.275250490306978,1.93224434677021,
7.98537225044948));
#61661=CARTESIAN_POINT('Ctrl Pts',(-0.262805660311028,1.91273606082892,
7.98689421936328));
#61662=CARTESIAN_POINT('Ctrl Pts',(-0.252853611858638,1.89950170830973,
7.98801248217074));
#61663=CARTESIAN_POINT('Ctrl Pts',(-0.229217042412051,1.87264324352422,
7.99043323637256));
#61664=CARTESIAN_POINT('Ctrl Pts',(-0.215232663582003,1.85936202528794,
7.99173128890212));
#61665=CARTESIAN_POINT('Ctrl Pts',(-0.200099249302323,1.84737088557421,
7.99294818405348));
#61666=CARTESIAN_POINT('Ctrl Pts',(-0.200053524706638,1.84733467535221,
7.99295185920715));
#61667=CARTESIAN_POINT('Ctrl Pts',(-0.199163638787225,1.84663034989125,
7.99302335312529));
#61668=CARTESIAN_POINT('Ctrl Pts',(-0.198316130541619,1.84596644501931,
7.99309089226384));
#61669=CARTESIAN_POINT('Ctrl Pts',(-0.197169705419999,1.84507761419416,
7.99318149583913));
#61670=CARTESIAN_POINT('Ctrl Pts',(-0.196873713084509,1.84484895332363,
7.99320482100931));
#61671=CARTESIAN_POINT('Ctrl Pts',(-0.196408224745283,1.84449064515518,
7.99324139622688));
#61672=CARTESIAN_POINT('Ctrl Pts',(-0.196238998095383,1.8443606509397,7.99325467091501));
#61673=CARTESIAN_POINT('Ctrl Pts',(-0.195912887889294,1.8441106586911,7.99328020932289));
#61674=CARTESIAN_POINT('Ctrl Pts',(-0.195756024315178,1.843990637708,7.9932924746267));
#61675=CARTESIAN_POINT('Ctrl Pts',(-0.195382519217882,1.84370540185631,
7.99332163423241));
#61676=CARTESIAN_POINT('Ctrl Pts',(-0.195165778664042,1.84354031760658,
7.99333851919561));
#61677=CARTESIAN_POINT('Ctrl Pts',(-0.194521775168591,1.8430510902317,7.99338858374208));
#61678=CARTESIAN_POINT('Ctrl Pts',(-0.194093909494702,1.84272773652661,
7.99342170770138));
#61679=CARTESIAN_POINT('Ctrl Pts',(-0.190633811872276,1.84012635921396,
7.99368848219602));
#61680=CARTESIAN_POINT('Ctrl Pts',(-0.187562231108778,1.83790083567827,
7.9939185313181));
#61681=CARTESIAN_POINT('Ctrl Pts',(-0.176256844167683,1.83001004291888,
7.99474381544702));
#61682=CARTESIAN_POINT('Ctrl Pts',(-0.167799374888341,1.82467390653016,
7.99532083149949));
#61683=CARTESIAN_POINT('Ctrl Pts',(-0.131743415463936,1.80420458645057,
7.99767598523277));
#61684=CARTESIAN_POINT('Ctrl Pts',(-0.102254432046472,1.79276176038056,
7.99937736302653));
#61685=CARTESIAN_POINT('Ctrl Pts',(-0.0712554161033839,1.7857008621921,
8.0012616863351));
#61686=CARTESIAN_POINT('Ctrl Pts',(-0.070936776215713,1.78562879246045,
8.00128106287805));
#61687=CARTESIAN_POINT('Ctrl Pts',(-0.0652971462924663,1.78436223601831,
8.00162414610145));
#61688=CARTESIAN_POINT('Ctrl Pts',(-0.0599470543503156,1.78330257246682,
8.00195178608463));
#61689=CARTESIAN_POINT('Ctrl Pts',(-0.0537042533029964,1.78222994854732,
8.00233746201053));
#61690=CARTESIAN_POINT('Ctrl Pts',(-0.052835018429724,1.78208426709833,
8.0023912375245));
#61691=CARTESIAN_POINT('Ctrl Pts',(-0.051450222259879,1.78185801512595,
8.00247703128507));
#61692=CARTESIAN_POINT('Ctrl Pts',(-0.0509350397262251,1.78177512725556,
8.00250897597185));
#61693=CARTESIAN_POINT('Ctrl Pts',(-0.0500272355011672,1.78163133132422,
8.00256531420451));
#61694=CARTESIAN_POINT('Ctrl Pts',(-0.0496346972491237,1.78156989728824,
8.00258969102141));
#61695=CARTESIAN_POINT('Ctrl Pts',(-0.0488245968536997,1.78144464719917,
8.00264003193276));
#61696=CARTESIAN_POINT('Ctrl Pts',(-0.0484070210244022,1.78138092591806,
8.00266599897939));
#61697=CARTESIAN_POINT('Ctrl Pts',(-0.0473410933620343,1.78122041120201,
8.00273233102465));
#61698=CARTESIAN_POINT('Ctrl Pts',(-0.0466925715596229,1.78112477502017,
8.0027727325874));
#61699=CARTESIAN_POINT('Ctrl Pts',(-0.0440700350332399,1.78074620687141,
8.00293629400941));
#61700=CARTESIAN_POINT('Ctrl Pts',(-0.0420937385077417,1.7804796261488,
8.00305996976343));
#61701=CARTESIAN_POINT('Ctrl Pts',(-0.0291818473656847,1.77885982292568,
8.00387084785819));
#61702=CARTESIAN_POINT('Ctrl Pts',(-0.0181866238236534,1.77805001437369,
8.00457509382631));
#61703=CARTESIAN_POINT('Ctrl Pts',(0.0236713919595222,1.77711819757734,
8.00731002993426));
#61704=CARTESIAN_POINT('Ctrl Pts',(0.0544482356536206,1.78086375105238,
8.00945064021308));
#61705=CARTESIAN_POINT('Ctrl Pts',(0.0848024713733795,1.78908187636469,
8.01151772230319));
#61706=CARTESIAN_POINT('Ctrl Pts',(0.0853836944600332,1.78924098808699,
8.01155727803791));
#61707=CARTESIAN_POINT('Ctrl Pts',(0.0874214974412825,1.78980499205283,
8.01169586829089));
#61708=CARTESIAN_POINT('Ctrl Pts',(0.0888756922704561,1.79021850822738,
8.01179459794157));
#61709=CARTESIAN_POINT('Ctrl Pts',(0.0912164185633628,1.79090195856612,
8.01195318682969));
#61710=CARTESIAN_POINT('Ctrl Pts',(0.0921047757328037,1.79116550620301,
8.01201329776371));
#61711=CARTESIAN_POINT('Ctrl Pts',(0.0931326345568202,1.79147526909201,
8.01208274931372));
#61712=CARTESIAN_POINT('Ctrl Pts',(0.0932732468130623,1.79151774989402,
8.01209224821875));
#61713=CARTESIAN_POINT('Ctrl Pts',(0.0939233130916909,1.79171462852633,
8.01213615264867));
#61714=CARTESIAN_POINT('Ctrl Pts',(0.0944324162780242,1.7918701933109,8.01217050803259));
#61715=CARTESIAN_POINT('Ctrl Pts',(0.0987115379628434,1.79318935017212,
8.01245901828756));
#61716=CARTESIAN_POINT('Ctrl Pts',(0.102460494093283,1.79442088876476,8.0127101250091));
#61717=CARTESIAN_POINT('Ctrl Pts',(0.106744475737754,1.79591589602634,8.01299439628836));
#61718=CARTESIAN_POINT('Ctrl Pts',(0.107302328235808,1.79611229745454,8.01303136101743));
#61719=CARTESIAN_POINT('Ctrl Pts',(0.108126836695061,1.79640513309702,8.01308591385298));
#61720=CARTESIAN_POINT('Ctrl Pts',(0.108393907101428,1.79650038397341,8.01310357169027));
#61721=CARTESIAN_POINT('Ctrl Pts',(0.108867439755196,1.79666997455176,8.01313485729367));
#61722=CARTESIAN_POINT('Ctrl Pts',(0.109073951774108,1.79674417264828,8.01314849350185));
#61723=CARTESIAN_POINT('Ctrl Pts',(0.109510182437678,1.79690141004515,8.01317728179479));
#61724=CARTESIAN_POINT('Ctrl Pts',(0.109739881873043,1.79698449937735,8.01319243079518));
#61725=CARTESIAN_POINT('Ctrl Pts',(0.110351352779289,1.79720647364527,8.01323273309103));
#61726=CARTESIAN_POINT('Ctrl Pts',(0.110732958053222,1.79734582000635,8.01325785880126));
#61727=CARTESIAN_POINT('Ctrl Pts',(0.112508245611008,1.79799788822094,8.01337463068625));
#61728=CARTESIAN_POINT('Ctrl Pts',(0.113898665957808,1.79851952809187,8.01346575179029));
#61729=CARTESIAN_POINT('Ctrl Pts',(0.124973839897785,1.80276212593847,8.01418925166488));
#61730=CARTESIAN_POINT('Ctrl Pts',(0.134478457384338,1.8069395855513,8.01479605597399));
#61731=CARTESIAN_POINT('Ctrl Pts',(0.167085939366902,1.82319248850407,8.01688267436618));
#61732=CARTESIAN_POINT('Ctrl Pts',(0.18891050529078,1.83760135536174,8.01829597067789));
#61733=CARTESIAN_POINT('Ctrl Pts',(0.218614898526131,1.86285880727917,8.02053678631184));
#61734=CARTESIAN_POINT('Ctrl Pts',(0.227952779632836,1.87182049459948,8.02129706269674));
#61735=CARTESIAN_POINT('Ctrl Pts',(0.23754737208645,1.88220678292567,8.02215638969351));
#61736=CARTESIAN_POINT('Ctrl Pts',(0.238363311768323,1.88310009006638,8.02223012804065));
#61737=CARTESIAN_POINT('Ctrl Pts',(0.239506906854062,1.88436636715142,8.0223344226344));
#61738=CARTESIAN_POINT('Ctrl Pts',(0.239838767164566,1.88473553984249,8.02236480146124));
#61739=CARTESIAN_POINT('Ctrl Pts',(0.240414954124197,1.8853794961803,8.0224177450542));
#61740=CARTESIAN_POINT('Ctrl Pts',(0.240659666557461,1.88565393468273,8.02244029357517));
#61741=CARTESIAN_POINT('Ctrl Pts',(0.241164201206696,1.88622171009245,8.02248691326849));
#61742=CARTESIAN_POINT('Ctrl Pts',(0.241423959064496,1.88651510318767,8.02251098708016));
#61743=CARTESIAN_POINT('Ctrl Pts',(0.242034173186306,1.88720687004315,8.02256771031642));
#61744=CARTESIAN_POINT('Ctrl Pts',(0.242384181224886,1.88760563606022,8.02260037834183));
#61745=CARTESIAN_POINT('Ctrl Pts',(0.243121531211282,1.88844989910624,8.022669480765));
#61746=CARTESIAN_POINT('Ctrl Pts',(0.243508636633396,1.88889559927798,8.02270592482671));
#61747=CARTESIAN_POINT('Ctrl Pts',(0.24454814620666,1.8900991192603,8.02280423857034));
#61748=CARTESIAN_POINT('Ctrl Pts',(0.245198247520846,1.89085891143797,8.02286620306268));
#61749=CARTESIAN_POINT('Ctrl Pts',(0.256941257899232,1.90471332015096,8.02399429765951));
#61750=CARTESIAN_POINT('Ctrl Pts',(0.26697240246131,1.91866809131453,8.02510386989432));
#61751=CARTESIAN_POINT('Ctrl Pts',(0.292275155676151,1.96055068692588,8.02835748734154));
#61752=CARTESIAN_POINT('Ctrl Pts',(0.304592873076093,1.99002722309371,8.03057428696961));
#61753=CARTESIAN_POINT('Ctrl Pts',(0.312780121345811,2.02233289139819,8.03268311463891));
#61754=CARTESIAN_POINT('Ctrl Pts',(0.313150509496931,2.02384001904503,8.03278075101568));
#61755=CARTESIAN_POINT('Ctrl Pts',(0.313608926693887,2.02576524329903,8.03290447308806));
#61756=CARTESIAN_POINT('Ctrl Pts',(0.313707023389319,2.02618088671783,8.0329311246088));
#61757=CARTESIAN_POINT('Ctrl Pts',(0.313861556033892,2.02684152493356,8.03297338999459));
#61758=CARTESIAN_POINT('Ctrl Pts',(0.313918531566079,2.02708639104738,8.03298903487884));
#61759=CARTESIAN_POINT('Ctrl Pts',(0.314024444384473,2.02754400225804,8.03301823317692));
#61760=CARTESIAN_POINT('Ctrl Pts',(0.314073451676662,2.02775672881094,8.03303179053127));
#61761=CARTESIAN_POINT('Ctrl Pts',(0.314183089369426,2.02823485462372,8.03306222665873));
#61762=CARTESIAN_POINT('Ctrl Pts',(0.314243599508734,2.02850028038028,8.03307909839138));
#61763=CARTESIAN_POINT('Ctrl Pts',(0.314422085626569,2.0292878072633,8.03312908553812));
#61764=CARTESIAN_POINT('Ctrl Pts',(0.314539098022451,2.02981012924671,8.03316214558673));
#61765=CARTESIAN_POINT('Ctrl Pts',(0.315467961716257,2.03400537746912,8.03342694803447));
#61766=CARTESIAN_POINT('Ctrl Pts',(0.316216794712723,2.03769216089017,8.03365514847465));
#61767=CARTESIAN_POINT('Ctrl Pts',(0.318691461989134,2.05107286658834,8.03446989314532));
#61768=CARTESIAN_POINT('Ctrl Pts',(0.320037544871541,2.060832196817,8.03503876440866));
#61769=CARTESIAN_POINT('Ctrl Pts',(0.323858630121932,2.10259862205488,8.03742265182372));
#61770=CARTESIAN_POINT('Ctrl Pts',(0.321992567900392,2.13481397971778,8.03915598276016));
#61771=CARTESIAN_POINT('Ctrl Pts',(0.314298964755468,2.17145571713681,8.04137948920178));
#61772=CARTESIAN_POINT('Ctrl Pts',(0.313070388406846,2.17665954300122,8.04170079662869));
#61773=CARTESIAN_POINT('Ctrl Pts',(0.311490622949169,2.18267729123685,8.04207963299852));
#61774=CARTESIAN_POINT('Ctrl Pts',(0.311264791433999,2.18352348329259,8.04213307174817));
#61775=CARTESIAN_POINT('Ctrl Pts',(0.310899336081152,2.18487077847462,8.04221842849841));
#61776=CARTESIAN_POINT('Ctrl Pts',(0.310761942299494,2.18537248636313,8.04225027411254));
#61777=CARTESIAN_POINT('Ctrl Pts',(0.310517538020945,2.18625654671252,8.04230649661029));
#61778=CARTESIAN_POINT('Ctrl Pts',(0.310411034223105,2.18663903912014,8.04233085698053));
#61779=CARTESIAN_POINT('Ctrl Pts',(0.310191897641845,2.18742044429211,8.04238069645845));
#61780=CARTESIAN_POINT('Ctrl Pts',(0.310079201565583,2.18781933839864,8.04240617758718));
#61781=CARTESIAN_POINT('Ctrl Pts',(0.30979157556242,2.1888299506696,8.04247083418969));
#61782=CARTESIAN_POINT('Ctrl Pts',(0.309615603721355,2.18944136821627,8.04251004356273));
#61783=CARTESIAN_POINT('Ctrl Pts',(0.309231061084397,2.19076273472439,8.04259498245305));
#61784=CARTESIAN_POINT('Ctrl Pts',(0.309021853783321,2.19147249326278,8.04264073260259));
#61785=CARTESIAN_POINT('Ctrl Pts',(0.308417408890938,2.19349739750329,8.04277161897104));
#61786=CARTESIAN_POINT('Ctrl Pts',(0.308016210753199,2.19481073391865,8.04285694980391));
#61787=CARTESIAN_POINT('Ctrl Pts',(0.306658432921034,2.19915587718971,8.04314074315344));
#61788=CARTESIAN_POINT('Ctrl Pts',(0.305665410158883,2.20217601641843,8.0433403937669));
#61789=CARTESIAN_POINT('Ctrl Pts',(0.301466364047907,2.2143374141486,8.04415429729472));
#61790=CARTESIAN_POINT('Ctrl Pts',(0.297893890697003,2.22334590420502,8.04478036189242));
#61791=CARTESIAN_POINT('Ctrl Pts',(0.287139829580337,2.24725927601229,8.04650493511214));
#61792=CARTESIAN_POINT('Ctrl Pts',(0.27920815999822,2.26179399088306,8.04762314863608));
#61793=CARTESIAN_POINT('Ctrl Pts',(0.259706423815186,2.29179213334084,8.05004403844249));
#61794=CARTESIAN_POINT('Ctrl Pts',(0.24778955565927,2.3069593492444,8.05134227725306));
#61795=CARTESIAN_POINT('Ctrl Pts',(0.234465770358515,2.32110407120128,8.05256695714794));
#61796=CARTESIAN_POINT('Ctrl Pts',(0.234342724542055,2.32123448019273,8.05257824934252));
#61797=CARTESIAN_POINT('Ctrl Pts',(0.233544093234559,2.32207948848807,8.05265142592055));
#61798=CARTESIAN_POINT('Ctrl Pts',(0.232865338646995,2.32279110576569,8.0527130825534));
#61799=CARTESIAN_POINT('Ctrl Pts',(0.231933435417272,2.3237592165674,8.05279699169251));
#61800=CARTESIAN_POINT('Ctrl Pts',(0.23168310718535,2.32401839949272,8.05281945874867));
#61801=CARTESIAN_POINT('Ctrl Pts',(0.231285739549084,2.32442844446465,8.05285500690835));
#61802=CARTESIAN_POINT('Ctrl Pts',(0.231138986952012,2.32457958214185,8.05286811034594));
#61803=CARTESIAN_POINT('Ctrl Pts',(0.230853725020348,2.32487279212537,8.05289353264205));
#61804=CARTESIAN_POINT('Ctrl Pts',(0.23071523372932,2.32501487932895,8.05290585268387));
#61805=CARTESIAN_POINT('Ctrl Pts',(0.230381672973994,2.32535646925533,8.05293547276838));
#61806=CARTESIAN_POINT('Ctrl Pts',(0.230186475649989,2.32555584653644,8.05295276261958));
#61807=CARTESIAN_POINT('Ctrl Pts',(0.229592710226044,2.32616075332619,8.0530052248007));
#61808=CARTESIAN_POINT('Ctrl Pts',(0.229193324893439,2.32656548450716,8.05304033320261));
#61809=CARTESIAN_POINT('Ctrl Pts',(0.225301149129364,2.33048893406631,8.05338076666994));
#61810=CARTESIAN_POINT('Ctrl Pts',(0.221728436540492,2.33392790250292,8.053679899582));
#61811=CARTESIAN_POINT('Ctrl Pts',(0.211340187973619,2.34347532539091,8.05451749462918));
#61812=CARTESIAN_POINT('Ctrl Pts',(0.204341613830049,2.34937810610984,8.05504414396834));
#61813=CARTESIAN_POINT('Ctrl Pts',(0.17297161656457,2.37362770444534,8.05729360379517));
#61814=CARTESIAN_POINT('Ctrl Pts',(0.146318762130083,2.38875967756152,8.05894600705478));
#61815=CARTESIAN_POINT('Ctrl Pts',(0.11653239710867,2.40047237841021,8.06083799351339));
#61816=CARTESIAN_POINT('Ctrl Pts',(0.115125136911787,2.40101437259044,8.0609274338485));
#61817=CARTESIAN_POINT('Ctrl Pts',(0.109117322363898,2.40327993877601,8.06130957430957));
#61818=CARTESIAN_POINT('Ctrl Pts',(0.104481671834036,2.40490799850585,8.06160520877488));
#61819=CARTESIAN_POINT('Ctrl Pts',(0.099000307656386,2.40669339951746,8.06195629870211));
#61820=CARTESIAN_POINT('Ctrl Pts',(0.0981887732054333,2.40695417739159,
8.06200831703418));
#61821=CARTESIAN_POINT('Ctrl Pts',(0.0968869307338629,2.40736681950774,
8.06209182828128));
#61822=CARTESIAN_POINT('Ctrl Pts',(0.0963972741225356,2.40752073851736,
8.06212325366222));
#61823=CARTESIAN_POINT('Ctrl Pts',(0.0955292675201147,2.40779131148993,
8.06217898766003));
#61824=CARTESIAN_POINT('Ctrl Pts',(0.0951510654583473,2.4079084395101,8.06220328067417));
#61825=CARTESIAN_POINT('Ctrl Pts',(0.094373727649485,2.4081476096914,8.06225323015188));
#61826=CARTESIAN_POINT('Ctrl Pts',(0.0939745688870358,2.40826957395901,
8.06227888911364));
#61827=CARTESIAN_POINT('Ctrl Pts',(0.0929773829730055,2.40857215062055,
8.06234301676043));
#61828=CARTESIAN_POINT('Ctrl Pts',(0.0923790673796352,2.40875179964559,
8.06238151687857));
#61829=CARTESIAN_POINT('Ctrl Pts',(0.0910694708266693,2.40914086899944,
8.06246583854892));
#61830=CARTESIAN_POINT('Ctrl Pts',(0.0903579832691287,2.40934957612252,
8.062511683191));
#61831=CARTESIAN_POINT('Ctrl Pts',(0.0883229911429242,2.4099388994536,8.0626429071377));
#61832=CARTESIAN_POINT('Ctrl Pts',(0.0869977707612186,2.41031348656928,
8.06272848228498));
#61833=CARTESIAN_POINT('Ctrl Pts',(0.0825937519070526,2.41152789925992,
8.06301328618101));
#61834=CARTESIAN_POINT('Ctrl Pts',(0.0795049592836114,2.41233046624247,
8.06321371261066));
#61835=CARTESIAN_POINT('Ctrl Pts',(0.066965101686883,2.41539065667375,8.06403034295932));
#61836=CARTESIAN_POINT('Ctrl Pts',(0.0574268727891681,2.41726599951836,
8.0646584268736));
#61837=CARTESIAN_POINT('Ctrl Pts',(0.0314433697613744,2.42116459415678,
8.06638685156063));
#61838=CARTESIAN_POINT('Ctrl Pts',(0.0149036741358159,2.42235567102332,
8.06750687707209));
#61839=CARTESIAN_POINT('Ctrl Pts',(-0.0208089795883369,2.42217251997626,
8.06992318325287));
#61840=CARTESIAN_POINT('Ctrl Pts',(-0.0399208290263174,2.42036644504946,
8.07121497634501));
#61841=CARTESIAN_POINT('Ctrl Pts',(-0.059876679886445,2.41666582780565,
8.07249429183234));
#61842=CARTESIAN_POINT('Ctrl Pts',(-0.0609913324165863,2.41645303088322,
8.07256550815842));
#61843=CARTESIAN_POINT('Ctrl Pts',(-0.06247992346075,2.41616068840008,8.0726602720277));
#61844=CARTESIAN_POINT('Ctrl Pts',(-0.0628548606445195,2.41608636196811,
8.07268411136308));
#61845=CARTESIAN_POINT('Ctrl Pts',(-0.0634405261655854,2.41596917809562,
8.07272130266208));
#61846=CARTESIAN_POINT('Ctrl Pts',(-0.063651343789003,2.41592677680295,
8.0727346806908));
#61847=CARTESIAN_POINT('Ctrl Pts',(-0.0640553143773882,2.41584510630179,
8.07276029747395));
#61848=CARTESIAN_POINT('Ctrl Pts',(-0.0642484723543551,2.4158058711854,
8.07277253804542));
#61849=CARTESIAN_POINT('Ctrl Pts',(-0.0647051517315274,2.41571267209139,
8.07280145924154));
#61850=CARTESIAN_POINT('Ctrl Pts',(-0.0649686413212397,2.41565855544532,
8.07281813097552));
#61851=CARTESIAN_POINT('Ctrl Pts',(-0.0657409614018235,2.41549892497306,
8.07286695503118));
#61852=CARTESIAN_POINT('Ctrl Pts',(-0.0662496078596602,2.41539250963293,
8.0728990557993));
#61853=CARTESIAN_POINT('Ctrl Pts',(-0.0700190274722311,2.41459437772303,
8.07313655498883));
#61854=CARTESIAN_POINT('Ctrl Pts',(-0.0732693029911311,2.41385330659291,
8.0733391818633));
#61855=CARTESIAN_POINT('Ctrl Pts',(-0.0840935240639338,2.41120802882875,
8.07400850584284));
#61856=CARTESIAN_POINT('Ctrl Pts',(-0.0916101244380889,2.40907889321617,
8.07446430428317));
#61857=CARTESIAN_POINT('Ctrl Pts',(-0.112143208152841,2.40244769105528,
8.07570282561714));
#61858=CARTESIAN_POINT('Ctrl Pts',(-0.12495999630363,2.39738147408969,8.07646887047718));
#61859=CARTESIAN_POINT('Ctrl Pts',(-0.152490164970555,2.38440415157265,
8.07817055229565));
#61860=CARTESIAN_POINT('Ctrl Pts',(-0.166991450120111,2.37613903100072,
8.07910612718435));
#61861=CARTESIAN_POINT('Ctrl Pts',(-0.188398332358233,2.36163288361778,
8.0806146686472));
#61862=CARTESIAN_POINT('Ctrl Pts',(-0.195784282584122,2.3561526646729,8.08116107127087));
#61863=CARTESIAN_POINT('Ctrl Pts',(-0.20380932385925,2.34964821181058,8.08178929736777));
#61864=CARTESIAN_POINT('Ctrl Pts',(-0.204689412312811,2.34892712706179,
8.08185867785068));
#61865=CARTESIAN_POINT('Ctrl Pts',(-0.205964830487254,2.34787079874053,
8.08195993927896));
#61866=CARTESIAN_POINT('Ctrl Pts',(-0.206363205824805,2.34753923233027,
8.08199167064877));
#61867=CARTESIAN_POINT('Ctrl Pts',(-0.20706509940704,2.34695217680815,8.08204775994896));
#61868=CARTESIAN_POINT('Ctrl Pts',(-0.207368949718518,2.34669708493036,
8.08207210161414));
#61869=CARTESIAN_POINT('Ctrl Pts',(-0.207952346974062,2.34620546522189,
8.08211895500641));
#61870=CARTESIAN_POINT('Ctrl Pts',(-0.208231963494635,2.34596902059925,
8.08214146329741));
#61871=CARTESIAN_POINT('Ctrl Pts',(-0.208968140815141,2.34534435170966,
8.08220086086279));
#61872=CARTESIAN_POINT('Ctrl Pts',(-0.209424021156393,2.34495533092078,
8.08223778289992));
#61873=CARTESIAN_POINT('Ctrl Pts',(-0.211084180373076,2.34353062917742,
8.08237275439994));
#61874=CARTESIAN_POINT('Ctrl Pts',(-0.21228186790583,2.34248733361709,8.08247111871724));
#61875=CARTESIAN_POINT('Ctrl Pts',(-0.215185716620661,2.33991981389111,
8.08271206880286));
#61876=CARTESIAN_POINT('Ctrl Pts',(-0.216883433752606,2.33838621072542,
8.08285504530595));
#61877=CARTESIAN_POINT('Ctrl Pts',(-0.223221122955843,2.33253742747787,
8.08339689057492));
#61878=CARTESIAN_POINT('Ctrl Pts',(-0.227749570916298,2.3281040307674,8.08380074562501));
#61879=CARTESIAN_POINT('Ctrl Pts',(-0.236537295890935,2.31897807334195,
8.08461905831328));
#61880=CARTESIAN_POINT('Ctrl Pts',(-0.240794744729038,2.31428759168804,
8.0850333334376));
#61881=CARTESIAN_POINT('Ctrl Pts',(-0.261778803401388,2.2897537385695,8.08716705776583));
#61882=CARTESIAN_POINT('Ctrl Pts',(-0.276201077863411,2.26806967271759,
8.08895650022701));
#61883=CARTESIAN_POINT('Ctrl Pts',(-0.291873112809776,2.23693306167294,
8.0912621531797));
#61884=CARTESIAN_POINT('Ctrl Pts',(-0.295547939101266,2.22881004235692,
8.09184088793663));
#61885=CARTESIAN_POINT('Ctrl Pts',(-0.299148800702242,2.21988194518528,
8.09244501478758));
#61886=CARTESIAN_POINT('Ctrl Pts',(-0.299413751203288,2.21921867033464,
8.09248970855261));
#61887=CARTESIAN_POINT('Ctrl Pts',(-0.299780831841562,2.21829078123557,
8.0925519661125));
#61888=CARTESIAN_POINT('Ctrl Pts',(-0.299884818498321,2.21802691091733,
8.09256964065442));
#61889=CARTESIAN_POINT('Ctrl Pts',(-0.300063901101739,2.21757071704998,
8.09260014502208));
#61890=CARTESIAN_POINT('Ctrl Pts',(-0.300139160585324,2.21737845856768,
8.09261298473829));
#61891=CARTESIAN_POINT('Ctrl Pts',(-0.300295278239088,2.21697850728355,
8.09263966135788));
#61892=CARTESIAN_POINT('Ctrl Pts',(-0.300376105613391,2.21677080318206,
8.09265349631855));
#61893=CARTESIAN_POINT('Ctrl Pts',(-0.30056737738462,2.2162777746808,8.09268629212091));
#61894=CARTESIAN_POINT('Ctrl Pts',(-0.300677631433077,2.21599237556941,
8.0927052414243));
#61895=CARTESIAN_POINT('Ctrl Pts',(-0.301043123260012,2.21504225554338,
8.09276820977808));
#61896=CARTESIAN_POINT('Ctrl Pts',(-0.301296566809617,2.21437683976274,
8.09281212149621));
#61897=CARTESIAN_POINT('Ctrl Pts',(-0.30552105533322,2.20317396645069,8.09354834292224));
#61898=CARTESIAN_POINT('Ctrl Pts',(-0.308939832790488,2.19243497996905,
8.09420852233683));
#61899=CARTESIAN_POINT('Ctrl Pts',(-0.318734983840597,2.15497962738738,
8.0964267746084));
#61900=CARTESIAN_POINT('Ctrl Pts',(-0.322258489260165,2.12764421150429,
8.09791182346188));
#61901=CARTESIAN_POINT('Ctrl Pts',(-0.322274942115673,2.10019315625606,
8.09949688950528));
#61902=CARTESIAN_POINT('',(-0.321965306320612,2.09975328274957,8.22472265507268));
#61903=CARTESIAN_POINT('Ctrl Pts',(-0.321883070004627,2.10020594158585,
8.09972265507268));
#61904=CARTESIAN_POINT('Ctrl Pts',(-0.321488885205279,2.0326703045558,8.10388007865086));
#61905=CARTESIAN_POINT('Ctrl Pts',(-0.267709080667653,1.85696506890364,
8.11466095006996));
#61906=CARTESIAN_POINT('Ctrl Pts',(0.0209181958432102,1.71950360581931,
8.13206526932999));
#61907=CARTESIAN_POINT('Ctrl Pts',(0.331251578158445,1.9116188202888,8.15193561285278));
#61908=CARTESIAN_POINT('Ctrl Pts',(0.337706733343549,2.27654812136149,8.17180595637557));
#61909=CARTESIAN_POINT('Ctrl Pts',(0.0343619353062186,2.47951855594141,
8.19167629989838));
#61910=CARTESIAN_POINT('Ctrl Pts',(-0.262899600533858,2.35063682153811,
8.20931519946406));
#61911=CARTESIAN_POINT('Ctrl Pts',(-0.321458260237508,2.17105380698424,
8.22033065118884));
#61912=CARTESIAN_POINT('Ctrl Pts',(-0.321965306320612,2.09975328274957,
8.22472265507268));
#61913=CARTESIAN_POINT('',(-0.322274858416085,2.100295336748,8.47470128209576));
#61914=CARTESIAN_POINT('Ctrl Pts',(-0.322274896144014,2.09974127163842,
8.22454451420393));
#61915=CARTESIAN_POINT('Ctrl Pts',(-0.322255995347832,2.07619823179053,
8.22610054604818));
#61916=CARTESIAN_POINT('Ctrl Pts',(-0.319657178017348,2.05272766680074,
8.22771693421608));
#61917=CARTESIAN_POINT('Ctrl Pts',(-0.31282525226628,2.02213862653997,8.22980782044883));
#61918=CARTESIAN_POINT('Ctrl Pts',(-0.310848803978768,2.01458880939707,
8.2303218442946));
#61919=CARTESIAN_POINT('Ctrl Pts',(-0.307505365589767,2.00348028881086,
8.23106819917312));
#61920=CARTESIAN_POINT('Ctrl Pts',(-0.306346311450068,1.9998623690893,8.23130966313781));
#61921=CARTESIAN_POINT('Ctrl Pts',(-0.30495080866007,1.99575764893316,8.23158109427415));
#61922=CARTESIAN_POINT('Ctrl Pts',(-0.304776849216764,1.99525012816356,
8.23161461050934));
#61923=CARTESIAN_POINT('Ctrl Pts',(-0.304512624828613,1.99448549296031,
8.2316650368354));
#61924=CARTESIAN_POINT('Ctrl Pts',(-0.304423300925214,1.99422805792199,
8.23168200231245));
#61925=CARTESIAN_POINT('Ctrl Pts',(-0.304262480994648,1.99376645973344,
8.23171240078252));
#61926=CARTESIAN_POINT('Ctrl Pts',(-0.304191106073464,1.99356225572985,
8.23172584093098));
#61927=CARTESIAN_POINT('Ctrl Pts',(-0.304036637645502,1.99312174525002,
8.23175481750411));
#61928=CARTESIAN_POINT('Ctrl Pts',(-0.303953474467364,1.99288546443444,
8.23177034966491));
#61929=CARTESIAN_POINT('Ctrl Pts',(-0.303729090229062,1.99225031595683,
8.23181207474879));
#61930=CARTESIAN_POINT('Ctrl Pts',(-0.303587358358929,1.9918516273249,8.23183823726004));
#61931=CARTESIAN_POINT('Ctrl Pts',(-0.302934708263323,1.99002713011228,
8.23195783675143));
#61932=CARTESIAN_POINT('Ctrl Pts',(-0.302414517224714,1.98860462503037,
8.2320507304143));
#61933=CARTESIAN_POINT('Ctrl Pts',(-0.290661122720945,1.95715321580582,
8.2340978292654));
#61934=CARTESIAN_POINT('Ctrl Pts',(-0.275017226733627,1.92895780443477,
8.23580937968716));
#61935=CARTESIAN_POINT('Ctrl Pts',(-0.251173373899254,1.89795383644452,
8.23802673896079));
#61936=CARTESIAN_POINT('Ctrl Pts',(-0.246701086865196,1.89251679079154,
8.23842950892459));
#61937=CARTESIAN_POINT('Ctrl Pts',(-0.235223364088875,1.87945928945521,
8.2394389324722));
#61938=CARTESIAN_POINT('Ctrl Pts',(-0.228022512535002,1.87202207205858,
8.24005196337986));
#61939=CARTESIAN_POINT('Ctrl Pts',(-0.219650645401829,1.86416943955152,
8.24074999282841));
#61940=CARTESIAN_POINT('Ctrl Pts',(-0.218820219059982,1.86339870890864,
8.24081907704328));
#61941=CARTESIAN_POINT('Ctrl Pts',(-0.217680088669632,1.86235167400246,
8.24091372229927));
#61942=CARTESIAN_POINT('Ctrl Pts',(-0.21737388246518,1.86207155892554,8.24093912138518));
#61943=CARTESIAN_POINT('Ctrl Pts',(-0.216796467180539,1.86154538892985,
8.24098697967823));
#61944=CARTESIAN_POINT('Ctrl Pts',(-0.216525377875889,1.86129920306684,
8.24100943329567));
#61945=CARTESIAN_POINT('Ctrl Pts',(-0.215959565466856,1.86078712562081,
8.24105626664384));
#61946=CARTESIAN_POINT('Ctrl Pts',(-0.215664769695718,1.86052131557226,
8.24108064975591));
#61947=CARTESIAN_POINT('Ctrl Pts',(-0.214982988143061,1.8599088498866,8.24113700087975));
#61948=CARTESIAN_POINT('Ctrl Pts',(-0.214595654431348,1.85956258475887,
8.2411689852191));
#61949=CARTESIAN_POINT('Ctrl Pts',(-0.21335242771577,1.85845657329933,8.24127155140891));
#61950=CARTESIAN_POINT('Ctrl Pts',(-0.212493331604829,1.85770045529584,
8.24134228462895));
#61951=CARTESIAN_POINT('Ctrl Pts',(-0.204537251833345,1.85077291088792,
8.24199607719296));
#61952=CARTESIAN_POINT('Ctrl Pts',(-0.197177991955495,1.84491091934045,
8.2425917920397));
#61953=CARTESIAN_POINT('Ctrl Pts',(-0.186368396457859,1.83704809381521,
8.24345565035917));
#61954=CARTESIAN_POINT('Ctrl Pts',(-0.183120607179277,1.83477608442076,
8.24371382080624));
#61955=CARTESIAN_POINT('Ctrl Pts',(-0.168256252022952,1.82478083104544,
8.2448889410407));
#61956=CARTESIAN_POINT('Ctrl Pts',(-0.156188414067491,1.81775741242609,
8.24582637186048));
#61957=CARTESIAN_POINT('Ctrl Pts',(-0.132347121462362,1.80588026165995,
8.24762772974648));
#61958=CARTESIAN_POINT('Ctrl Pts',(-0.120665092825832,1.8008977847092,8.24848893588757));
#61959=CARTESIAN_POINT('Ctrl Pts',(-0.0997302592355138,1.79339564059978,
8.24996822128051));
#61960=CARTESIAN_POINT('Ctrl Pts',(-0.0906013623910445,1.79057506674255,
8.25059286368307));
#61961=CARTESIAN_POINT('Ctrl Pts',(-0.0804540240822051,1.78792756949624,
8.25125546823024));
#61962=CARTESIAN_POINT('Ctrl Pts',(-0.0795472261459676,1.78769519578758,
8.25131440545272));
#61963=CARTESIAN_POINT('Ctrl Pts',(-0.0779686028522084,1.78729798357846,
8.25141651440416));
#61964=CARTESIAN_POINT('Ctrl Pts',(-0.0772972408954239,1.78713135236047,
8.25145978484391));
#61965=CARTESIAN_POINT('Ctrl Pts',(-0.0763316572703518,1.78689499342699,
8.25152179092407));
#61966=CARTESIAN_POINT('Ctrl Pts',(-0.0760378717655394,1.78682351764239,
8.25154062648893));
#61967=CARTESIAN_POINT('Ctrl Pts',(-0.0755279623172703,1.78670022035226,
8.25157326554582));
#61968=CARTESIAN_POINT('Ctrl Pts',(-0.0753118849150722,1.78664820885966,
8.25158708007219));
#61969=CARTESIAN_POINT('Ctrl Pts',(-0.0748940856722545,1.78654809848911,
8.25161375927465));
#61970=CARTESIAN_POINT('Ctrl Pts',(-0.0746923717178264,1.78649997091347,
8.25162662561923));
#61971=CARTESIAN_POINT('Ctrl Pts',(-0.0742112904962405,1.78638567888054,
8.25165727739857));
#61972=CARTESIAN_POINT('Ctrl Pts',(-0.0739318804191332,1.78631969282802,
8.25167505248091));
#61973=CARTESIAN_POINT('Ctrl Pts',(-0.0729373210322925,1.78608621834283,
8.25173822675518));
#61974=CARTESIAN_POINT('Ctrl Pts',(-0.0722216807667435,1.7859207998511,
8.25178350745024));
#61975=CARTESIAN_POINT('Ctrl Pts',(-0.0615599619685552,1.78349473705332,
8.25245556306786));
#61976=CARTESIAN_POINT('Ctrl Pts',(-0.0515114270030518,1.78170480426918,
8.2530560977969));
#61977=CARTESIAN_POINT('Ctrl Pts',(-0.0241580255962727,1.77816211978753,
8.25464352260644));
#61978=CARTESIAN_POINT('Ctrl Pts',(-0.00676900199513222,1.77732759733156,
8.25560345244038));
#61979=CARTESIAN_POINT('Ctrl Pts',(0.0220277845513836,1.77827556342132,
8.25721874264397));
#61980=CARTESIAN_POINT('Ctrl Pts',(0.0334236257123433,1.77925918005283,
8.25786436917472));
#61981=CARTESIAN_POINT('Ctrl Pts',(0.051242427986826,1.78175721916992,8.25890481099587));
#61982=CARTESIAN_POINT('Ctrl Pts',(0.0577125837788584,1.78286674166639,
8.25928904260863));
#61983=CARTESIAN_POINT('Ctrl Pts',(0.067506178420532,1.78485580832934,8.25988319018327));
#61984=CARTESIAN_POINT('Ctrl Pts',(0.070857068035082,1.78559227071052,8.26008873558658));
#61985=CARTESIAN_POINT('Ctrl Pts',(0.0756095789940844,1.78671661579665,
8.26038375458923));
#61986=CARTESIAN_POINT('Ctrl Pts',(0.0770213913476366,1.78706072087082,
8.26047183681467));
#61987=CARTESIAN_POINT('Ctrl Pts',(0.0794998507213796,1.78768259069385,
8.26062726653322));
#61988=CARTESIAN_POINT('Ctrl Pts',(0.0805674971549476,1.78795630309947,
8.26069448315496));
#61989=CARTESIAN_POINT('Ctrl Pts',(0.0821331235687456,1.78836625318486,
8.26079344395835));
#61990=CARTESIAN_POINT('Ctrl Pts',(0.0826322216510079,1.78849822138338,
8.26082504988412));
#61991=CARTESIAN_POINT('Ctrl Pts',(0.0834915754548075,1.78872765664655,
8.26087957140916));
#61992=CARTESIAN_POINT('Ctrl Pts',(0.083851984000042,1.78882455160146,8.26090246841936));
#61993=CARTESIAN_POINT('Ctrl Pts',(0.0845679481265212,1.78901837097817,
8.2609480160272));
#61994=CARTESIAN_POINT('Ctrl Pts',(0.0849235074327807,1.78911527968882,
8.26097066608611));
#61995=CARTESIAN_POINT('Ctrl Pts',(0.0857607867220597,1.78934502613618,
8.26102407494874));
#61996=CARTESIAN_POINT('Ctrl Pts',(0.0862423644823651,1.78947837452197,
8.26105485031326));
#61997=CARTESIAN_POINT('Ctrl Pts',(0.087664063633908,1.789875603934,8.2611458716149));
#61998=CARTESIAN_POINT('Ctrl Pts',(0.0886032917876881,1.79014263646177,
8.26120622002157));
#61999=CARTESIAN_POINT('Ctrl Pts',(0.0969406660654781,1.79255404727747,
8.26174387036586));
#62000=CARTESIAN_POINT('Ctrl Pts',(0.10426037610646,1.794958586243,8.26222963917548));
#62001=CARTESIAN_POINT('Ctrl Pts',(0.114717113164343,1.79881398516656,8.26294457310198));
#62002=CARTESIAN_POINT('Ctrl Pts',(0.117928374047243,1.80005679070078,8.26316704928007));
#62003=CARTESIAN_POINT('Ctrl Pts',(0.145521566749939,1.81124737832489,8.26510394805226));
#62004=CARTESIAN_POINT('Ctrl Pts',(0.168617334283851,1.82409702523694,8.26690873278305));
#62005=CARTESIAN_POINT('Ctrl Pts',(0.200420973227003,1.84728962164024,8.26954757731479));
#62006=CARTESIAN_POINT('Ctrl Pts',(0.210479180620339,1.85560338473454,8.270407131995));
#62007=CARTESIAN_POINT('Ctrl Pts',(0.220560879729639,1.8650220261108,8.27127321558611));
#62008=CARTESIAN_POINT('Ctrl Pts',(0.221112802813991,1.86554130781846,8.27132064328367));
#62009=CARTESIAN_POINT('Ctrl Pts',(0.221890695934833,1.86627838532623,8.27138750200485));
#62010=CARTESIAN_POINT('Ctrl Pts',(0.222118181917902,1.86649456671921,8.27140705566144));
#62011=CARTESIAN_POINT('Ctrl Pts',(0.22250773376119,1.86686584471434,8.27144054190119));
#62012=CARTESIAN_POINT('Ctrl Pts',(0.222669953814464,1.86702077857953,8.27145448712507));
#62013=CARTESIAN_POINT('Ctrl Pts',(0.222979894059801,1.86731741713022,8.27148113208948));
#62014=CARTESIAN_POINT('Ctrl Pts',(0.223127640820691,1.86745909300031,8.27149383404484));
#62015=CARTESIAN_POINT('Ctrl Pts',(0.223474816027414,1.86779263833444,8.27152368244175));
#62016=CARTESIAN_POINT('Ctrl Pts',(0.223674132903451,1.86798462447203,8.2715408197679));
#62017=CARTESIAN_POINT('Ctrl Pts',(0.224260551239826,1.86855093271814,8.27159124420043));
#62018=CARTESIAN_POINT('Ctrl Pts',(0.224646964538702,1.86892597090661,8.27162447592548));
#62019=CARTESIAN_POINT('Ctrl Pts',(0.227963786366516,1.87216133679109,8.27190978795215));
#62020=CARTESIAN_POINT('Ctrl Pts',(0.230840536355453,1.87507646869592,8.2721576753221));
#62021=CARTESIAN_POINT('Ctrl Pts',(0.254331126491047,1.89980606264411,8.27419371474141));
#62022=CARTESIAN_POINT('Ctrl Pts',(0.271862949925925,1.92434975671978,8.27580295489753));
#62023=CARTESIAN_POINT('Ctrl Pts',(0.291060358721008,1.9611579636798,8.27816189879016));
#62024=CARTESIAN_POINT('Ctrl Pts',(0.295825432924316,1.97162352570644,8.27882566702504));
#62025=CARTESIAN_POINT('Ctrl Pts',(0.301326912092194,1.9856494244943,8.27972045744278));
#62026=CARTESIAN_POINT('Ctrl Pts',(0.302577093982221,1.98899971732683,8.27993453052497));
#62027=CARTESIAN_POINT('Ctrl Pts',(0.304271690262339,1.99378248898462,8.28024092505828));
#62028=CARTESIAN_POINT('Ctrl Pts',(0.304762280734173,1.99519841000071,8.2803317286314));
#62029=CARTESIAN_POINT('Ctrl Pts',(0.30549586282019,1.99736435851528,8.28047079957808));
#62030=CARTESIAN_POINT('Ctrl Pts',(0.305746011003941,1.99811195437565,8.28051883145515));
#62031=CARTESIAN_POINT('Ctrl Pts',(0.306196819816607,1.99947585735974,8.28060651859447));
#62032=CARTESIAN_POINT('Ctrl Pts',(0.306398369558215,2.00009186798982,8.28064614440556));
#62033=CARTESIAN_POINT('Ctrl Pts',(0.306729676281944,2.00111489590947,8.28071198968264));
#62034=CARTESIAN_POINT('Ctrl Pts',(0.306860485345735,2.00152157264853,8.28073817446935));
#62035=CARTESIAN_POINT('Ctrl Pts',(0.307110109638165,2.00230296467212,8.28078850542785));
#62036=CARTESIAN_POINT('Ctrl Pts',(0.307229048700757,2.00267763984534,8.28081264747702));
#62037=CARTESIAN_POINT('Ctrl Pts',(0.307498109728462,2.00353062941936,8.28086762929784));
#62038=CARTESIAN_POINT('Ctrl Pts',(0.307647801462758,2.00400907752602,8.28089848312788));
#62039=CARTESIAN_POINT('Ctrl Pts',(0.308089057640011,2.00543106500771,8.28099022630835));
#62040=CARTESIAN_POINT('Ctrl Pts',(0.308377400126561,2.00637559100586,8.28105122104512));
#62041=CARTESIAN_POINT('Ctrl Pts',(0.310339149882183,2.01290910078152,8.28147354218179));
#62042=CARTESIAN_POINT('Ctrl Pts',(0.311864770852018,2.01854099071496,8.28183966233875));
#62043=CARTESIAN_POINT('Ctrl Pts',(0.321019348210053,2.05637689265291,8.28431529201753));
#62044=CARTESIAN_POINT('Ctrl Pts',(0.323799612953773,2.08954634954697,8.2865913944019));
#62045=CARTESIAN_POINT('Ctrl Pts',(0.320730677539727,2.1333077457305,8.28952219706427));
#62046=CARTESIAN_POINT('Ctrl Pts',(0.319435873417244,2.1440266764052,8.29023140140384));
#62047=CARTESIAN_POINT('Ctrl Pts',(0.317348062861834,2.15615770208835,8.29100985918171));
#62048=CARTESIAN_POINT('Ctrl Pts',(0.317079986355857,2.15765208560087,8.29110532855341));
#62049=CARTESIAN_POINT('Ctrl Pts',(0.316726215694184,2.15954701958721,8.29122579694933));
#62050=CARTESIAN_POINT('Ctrl Pts',(0.316650310758013,2.15994934487509,8.29125134049104));
#62051=CARTESIAN_POINT('Ctrl Pts',(0.316527763073654,2.16059216815155,8.29129209786023));
#62052=CARTESIAN_POINT('Ctrl Pts',(0.316481612760247,2.16083275781478,8.29130733973422));
#62053=CARTESIAN_POINT('Ctrl Pts',(0.316393632298905,2.16128860539198,8.29133619485268));
#62054=CARTESIAN_POINT('Ctrl Pts',(0.316351857127204,2.16150387144435,8.29134981107063));
#62055=CARTESIAN_POINT('Ctrl Pts',(0.316255804313102,2.16199614132562,8.29138092569395));
#62056=CARTESIAN_POINT('Ctrl Pts',(0.3162013825176,2.16227311616107,8.29139841571307));
#62057=CARTESIAN_POINT('Ctrl Pts',(0.31603306901943,2.1631238231516,8.29145208503395));
#62058=CARTESIAN_POINT('Ctrl Pts',(0.315917978380196,2.16369732107371,8.29148819600614));
#62059=CARTESIAN_POINT('Ctrl Pts',(0.315043511355309,2.16799412617874,8.2917582473801));
#62060=CARTESIAN_POINT('Ctrl Pts',(0.314219857622185,2.17170424948038,8.29198859868031));
#62061=CARTESIAN_POINT('Ctrl Pts',(0.306117238230526,2.20537572071285,8.29406048866452));
#62062=CARTESIAN_POINT('Ctrl Pts',(0.29463850933332,2.23416612043077,8.29570948487915));
#62063=CARTESIAN_POINT('Ctrl Pts',(0.272021860239076,2.27341973789832,8.29828754604229));
#62064=CARTESIAN_POINT('Ctrl Pts',(0.263968165960037,2.28544817587149,8.2991283592283));
#62065=CARTESIAN_POINT('Ctrl Pts',(0.254184382675395,2.29812595845684,8.30009484875323));
#62066=CARTESIAN_POINT('Ctrl Pts',(0.25322503670252,2.29935063698686,8.30018908140717));
#62067=CARTESIAN_POINT('Ctrl Pts',(0.251752675637069,2.30120244103574,8.30033292084229));
#62068=CARTESIAN_POINT('Ctrl Pts',(0.251246091442515,2.30183466869024,8.30038227191472));
#62069=CARTESIAN_POINT('Ctrl Pts',(0.25030747279461,2.30299707491932,8.30047346054869));
#62070=CARTESIAN_POINT('Ctrl Pts',(0.249876123208658,2.30352780252703,8.30051527048573));
#62071=CARTESIAN_POINT('Ctrl Pts',(0.249173402209867,2.30438682117714,8.30058322974469));
#62072=CARTESIAN_POINT('Ctrl Pts',(0.248903062038938,2.3047159562531,8.30060933728236));
#62073=CARTESIAN_POINT('Ctrl Pts',(0.248381790471071,2.30534803756207,8.30065960802339));
#62074=CARTESIAN_POINT('Ctrl Pts',(0.248130955176592,2.3056510623585,8.30068376729336));
#62075=CARTESIAN_POINT('Ctrl Pts',(0.247557736704661,2.30634097080579,8.30073890699828));
#62076=CARTESIAN_POINT('Ctrl Pts',(0.247235000817604,2.30672755888255,8.30076990179382));
#62077=CARTESIAN_POINT('Ctrl Pts',(0.246247686062536,2.30790459158825,8.30086456965716));
#62078=CARTESIAN_POINT('Ctrl Pts',(0.245580217643585,2.30869259391986,8.30092836105402));
#62079=CARTESIAN_POINT('Ctrl Pts',(0.240688526905232,2.31441167948182,8.30139438356912));
#62080=CARTESIAN_POINT('Ctrl Pts',(0.236320188553444,2.31921700179485,8.30180257258702));
#62081=CARTESIAN_POINT('Ctrl Pts',(0.230559261812351,2.32518180105656,8.3023315934675));
#62082=CARTESIAN_POINT('Ctrl Pts',(0.229297765532181,2.32646622541267,8.3024468902202));
#62083=CARTESIAN_POINT('Ctrl Pts',(0.223608901927806,2.33216222321378,8.30296442255023));
#62084=CARTESIAN_POINT('Ctrl Pts',(0.219064741631382,2.33645479486463,8.30337140916914));
#62085=CARTESIAN_POINT('Ctrl Pts',(0.196763273493759,2.35632663462441,8.30533777969493));
#62086=CARTESIAN_POINT('Ctrl Pts',(0.177454028160258,2.37005372547209,8.30695707265761));
#62087=CARTESIAN_POINT('Ctrl Pts',(0.149082864337998,2.38585650783233,8.30913077668616));
#62088=CARTESIAN_POINT('Ctrl Pts',(0.141169058535459,2.38984645238553,8.30971651174549));
#62089=CARTESIAN_POINT('Ctrl Pts',(0.129558740692125,2.39511155589719,8.31053718738767));
#62090=CARTESIAN_POINT('Ctrl Pts',(0.125988193025744,2.39665346163708,8.31078448009236));
#62091=CARTESIAN_POINT('Ctrl Pts',(0.121891378278172,2.39833531225558,8.31106175375366));
#62092=CARTESIAN_POINT('Ctrl Pts',(0.121391820428101,2.39853892975686,8.31109545548291));
#62093=CARTESIAN_POINT('Ctrl Pts',(0.120638593145714,2.39884373851871,8.31114610469839));
#62094=CARTESIAN_POINT('Ctrl Pts',(0.120385305673937,2.39894586196691,8.31116310830342));
#62095=CARTESIAN_POINT('Ctrl Pts',(0.119931112370513,2.39912831816193,8.31119354815077));
#62096=CARTESIAN_POINT('Ctrl Pts',(0.119730255867269,2.39920877037899,8.31120699163204));
#62097=CARTESIAN_POINT('Ctrl Pts',(0.119297092820497,2.39938176597631,8.31123594506605));
#62098=CARTESIAN_POINT('Ctrl Pts',(0.119064760226522,2.39947424100869,8.31125145081788));
#62099=CARTESIAN_POINT('Ctrl Pts',(0.118440710375996,2.39972178973153,8.31129303631262));
#62100=CARTESIAN_POINT('Ctrl Pts',(0.118048794587964,2.39987636655022,8.31131908599037));
#62101=CARTESIAN_POINT('Ctrl Pts',(0.116262508225279,2.40057685720457,8.31143751674716));
#62102=CARTESIAN_POINT('Ctrl Pts',(0.114864617323409,2.40111382863789,8.31152936731556));
#62103=CARTESIAN_POINT('Ctrl Pts',(0.0833370490654287,2.41297299891607,
8.31358341059271));
#62104=CARTESIAN_POINT('Ctrl Pts',(0.0516778241459738,2.41973018248313,
8.3153008581447));
#62105=CARTESIAN_POINT('Ctrl Pts',(0.00400927344428922,2.42262534987356,
8.31800903592352));
#62106=CARTESIAN_POINT('Ctrl Pts',(-0.0115648770916579,2.42244278508247,
8.31891017150142));
#62107=CARTESIAN_POINT('Ctrl Pts',(-0.0295162987467325,2.42092993248103,
8.3199967787625));
#62108=CARTESIAN_POINT('Ctrl Pts',(-0.0319663677915664,2.4206951578455,
8.32014608800993));
#62109=CARTESIAN_POINT('Ctrl Pts',(-0.035118162808726,2.42035666468081,
8.32033953309254));
#62110=CARTESIAN_POINT('Ctrl Pts',(-0.0358226134232033,2.42027865729606,
8.32038285794817));
#62111=CARTESIAN_POINT('Ctrl Pts',(-0.0369582616171983,2.42014910761688,
8.32045284671485));
#62112=CARTESIAN_POINT('Ctrl Pts',(-0.0373896250489441,2.42009901615817,
8.3204794648386));
#62113=CARTESIAN_POINT('Ctrl Pts',(-0.038211652044458,2.42000187515843,
8.32053025431114));
#62114=CARTESIAN_POINT('Ctrl Pts',(-0.0386023335506537,2.41995498167576,
8.3205544206931));
#62115=CARTESIAN_POINT('Ctrl Pts',(-0.0394937355143449,2.41984633031453,
8.32060962419098));
#62116=CARTESIAN_POINT('Ctrl Pts',(-0.0399943978858773,2.41978411200947,
8.32064067578934));
#62117=CARTESIAN_POINT('Ctrl Pts',(-0.041524001538584,2.41959037679496,
8.32073568565396));
#62118=CARTESIAN_POINT('Ctrl Pts',(-0.0425524481596547,2.41945506845101,
8.32079976350455));
#62119=CARTESIAN_POINT('Ctrl Pts',(-0.0501122391539524,2.41842330508963,
8.32127225138458));
#62120=CARTESIAN_POINT('Ctrl Pts',(-0.0566149458339473,2.41733164874971,
8.32168680680054));
#62121=CARTESIAN_POINT('Ctrl Pts',(-0.064876279194895,2.41568275534116,
8.32222447841607));
#62122=CARTESIAN_POINT('Ctrl Pts',(-0.0666701970753574,2.41530876649616,
8.32234189744928));
#62123=CARTESIAN_POINT('Ctrl Pts',(-0.072661012976683,2.41400641449459,
8.32273625455804));
#62124=CARTESIAN_POINT('Ctrl Pts',(-0.0768423816233633,2.41300941986759,
8.32301519030779));
#62125=CARTESIAN_POINT('Ctrl Pts',(-0.105648435930526,2.40552900275532,
8.32496203457186));
#62126=CARTESIAN_POINT('Ctrl Pts',(-0.129447740793255,2.39623060791731,
8.32670900758343));
#62127=CARTESIAN_POINT('Ctrl Pts',(-0.161937044286073,2.37886747709717,
8.3291745575876));
#62128=CARTESIAN_POINT('Ctrl Pts',(-0.171683579581393,2.37297524388826,
8.32992430557303));
#62129=CARTESIAN_POINT('Ctrl Pts',(-0.181952223863904,2.3659993009728,8.33070969475765));
#62130=CARTESIAN_POINT('Ctrl Pts',(-0.182802791802399,2.36541548421857,
8.33077471261378));
#62131=CARTESIAN_POINT('Ctrl Pts',(-0.184264653831585,2.3644017236102,8.3308863733415));
#62132=CARTESIAN_POINT('Ctrl Pts',(-0.184877276955737,2.36397372329758,
8.3309331411664));
#62133=CARTESIAN_POINT('Ctrl Pts',(-0.185743592255013,2.36336398944111,
8.33099923269483));
#62134=CARTESIAN_POINT('Ctrl Pts',(-0.185998511843769,2.36318401659677,
8.33101867527838));
#62135=CARTESIAN_POINT('Ctrl Pts',(-0.186435962630036,2.36287422397991,
8.33105202968345));
#62136=CARTESIAN_POINT('Ctrl Pts',(-0.18661862027742,2.36274458388653,8.33106595389455));
#62137=CARTESIAN_POINT('Ctrl Pts',(-0.186968250658633,2.3624958874427,8.33109260080698));
#62138=CARTESIAN_POINT('Ctrl Pts',(-0.187135244663637,2.36237686232584,
8.33110532564177));
#62139=CARTESIAN_POINT('Ctrl Pts',(-0.187528526363154,2.36209598399671,
8.33113528776981));
#62140=CARTESIAN_POINT('Ctrl Pts',(-0.187754718737168,2.36193399668699,
8.33115251577308));
#62141=CARTESIAN_POINT('Ctrl Pts',(-0.188422738581413,2.36145428542849,
8.33120338346171));
#62142=CARTESIAN_POINT('Ctrl Pts',(-0.188863974165728,2.36113573301246,
8.33123696637981));
#62143=CARTESIAN_POINT('Ctrl Pts',(-0.192744428215652,2.35831923835979,
8.33153219260575));
#62144=CARTESIAN_POINT('Ctrl Pts',(-0.196134920719671,2.35575445378477,
8.33178931511299));
#62145=CARTESIAN_POINT('Ctrl Pts',(-0.200199106889556,2.35255166962367,
8.33209784960425));
#62146=CARTESIAN_POINT('Ctrl Pts',(-0.200921890638701,2.35197702698514,
8.33215273267425));
#62147=CARTESIAN_POINT('Ctrl Pts',(-0.201730786758905,2.35132822800901,
8.33221418134362));
#62148=CARTESIAN_POINT('Ctrl Pts',(-0.201819333610174,2.35125712945452,
8.33222090826365));
#62149=CARTESIAN_POINT('Ctrl Pts',(-0.217084600729435,2.33898663128751,
8.33338067948435));
#62150=CARTESIAN_POINT('Ctrl Pts',(-0.231126217796276,2.32543551820192,
8.3344605382151));
#62151=CARTESIAN_POINT('Ctrl Pts',(-0.260778874754767,2.29111589421998,
8.33699638420464));
#62152=CARTESIAN_POINT('Ctrl Pts',(-0.275275200653457,2.26957061701527,
8.33845637976977));
#62153=CARTESIAN_POINT('Ctrl Pts',(-0.287564354508336,2.24549657303681,
8.34009997474716));
#62154=CARTESIAN_POINT('Ctrl Pts',(-0.288084159677424,2.24446462417411,
8.34017042873191));
#62155=CARTESIAN_POINT('Ctrl Pts',(-0.288833072790938,2.2429577200604,8.3402733177258));
#62156=CARTESIAN_POINT('Ctrl Pts',(-0.289066586456472,2.24248495447557,
8.34030559860681));
#62157=CARTESIAN_POINT('Ctrl Pts',(-0.289473756932274,2.24165548723899,
8.34036223838518));
#62158=CARTESIAN_POINT('Ctrl Pts',(-0.289647917755419,2.24129903310028,
8.34038657964588));
#62159=CARTESIAN_POINT('Ctrl Pts',(-0.289984367652972,2.24060718675741,
8.34043382615094));
#62160=CARTESIAN_POINT('Ctrl Pts',(-0.290146734237677,2.24027183274031,
8.34045672865102));
#62161=CARTESIAN_POINT('Ctrl Pts',(-0.290532301513119,2.23947194346743,
8.34051135869919));
#62162=CARTESIAN_POINT('Ctrl Pts',(-0.290754969650857,2.23900715397236,
8.34054310468744));
#62163=CARTESIAN_POINT('Ctrl Pts',(-0.291422828228239,2.23760446455367,
8.34063891898839));
#62164=CARTESIAN_POINT('Ctrl Pts',(-0.29186459914382,2.23666495236097,8.34070310556189));
#62165=CARTESIAN_POINT('Ctrl Pts',(-0.296386475694923,2.22692637069945,
8.3413685785848));
#62166=CARTESIAN_POINT('Ctrl Pts',(-0.300071533507521,2.21795036559158,
8.34198337493987));
#62167=CARTESIAN_POINT('Ctrl Pts',(-0.304702522471836,2.20504135540363,
8.34287080321147));
#62168=CARTESIAN_POINT('Ctrl Pts',(-0.305988146833679,2.2012351988422,8.34313281083461));
#62169=CARTESIAN_POINT('Ctrl Pts',(-0.314529584705017,2.17429696507946,
8.3449890988564));
#62170=CARTESIAN_POINT('Ctrl Pts',(-0.319225504080827,2.15043574997385,
8.34665142814623));
#62171=CARTESIAN_POINT('Ctrl Pts',(-0.321918916382813,2.11751334094391,
8.34886255247666));
#62172=CARTESIAN_POINT('Ctrl Pts',(-0.322276976597949,2.10872244622439,
8.34944413543821));
#62173=CARTESIAN_POINT('Ctrl Pts',(-0.322274112328226,2.09603013592404,
8.35026164780834));
#62174=CARTESIAN_POINT('Ctrl Pts',(-0.322202543125355,2.09213311512152,
8.35050962374752));
#62175=CARTESIAN_POINT('Ctrl Pts',(-0.322038789492845,2.08764925349233,
8.35079072369609));
#62176=CARTESIAN_POINT('Ctrl Pts',(-0.32201566754641,2.08706041944243,8.35082755472705));
#62177=CARTESIAN_POINT('Ctrl Pts',(-0.321979045376265,2.08618876815533,
8.350881948255));
#62178=CARTESIAN_POINT('Ctrl Pts',(-0.32196678749655,2.08590590417565,8.35089957989809));
#62179=CARTESIAN_POINT('Ctrl Pts',(-0.32194436986702,2.08540388867636,8.35093083609994));
#62180=CARTESIAN_POINT('Ctrl Pts',(-0.321934359105089,2.08518473140471,
8.35094446904338));
#62181=CARTESIAN_POINT('Ctrl Pts',(-0.321912718568679,2.08472135390612,
8.35097326828698));
#62182=CARTESIAN_POINT('Ctrl Pts',(-0.321901034695205,2.08447713731783,
8.35098843146677));
#62183=CARTESIAN_POINT('Ctrl Pts',(-0.321869147169632,2.08382614457258,
8.35102881141952));
#62184=CARTESIAN_POINT('Ctrl Pts',(-0.321848450236824,2.08341939133873,
8.35105400041887));
#62185=CARTESIAN_POINT('Ctrl Pts',(-0.32174814382633,2.08151907384536,8.35117149336452));
#62186=CARTESIAN_POINT('Ctrl Pts',(-0.321658906930937,2.08002600483372,
8.35126326430161));
#62187=CARTESIAN_POINT('Ctrl Pts',(-0.320859447470214,2.06805039015372,
8.35199537142328));
#62188=CARTESIAN_POINT('Ctrl Pts',(-0.31964730836709,2.05760648607181,8.3526094877765));
#62189=CARTESIAN_POINT('Ctrl Pts',(-0.313399767065271,2.0199598011947,8.35479375427832));
#62190=CARTESIAN_POINT('Ctrl Pts',(-0.305380696477646,1.99337634306458,
8.35628978082287));
#62191=CARTESIAN_POINT('Ctrl Pts',(-0.29251938846195,1.96469343297168,8.35810796097955));
#62192=CARTESIAN_POINT('Ctrl Pts',(-0.290912543196602,1.96127238765257,
8.3583281322873));
#62193=CARTESIAN_POINT('Ctrl Pts',(-0.285875503296402,1.95102085177581,
8.35899908790642));
#62194=CARTESIAN_POINT('Ctrl Pts',(-0.282262344403604,1.94428376946158,
8.35945536209082));
#62195=CARTESIAN_POINT('Ctrl Pts',(-0.2779226613954,1.93684020385766,8.35997957399958));
#62196=CARTESIAN_POINT('Ctrl Pts',(-0.27742815590886,1.93600078332297,8.36003898418915));
#62197=CARTESIAN_POINT('Ctrl Pts',(-0.276674560084789,1.93473472064,8.36012904111841));
#62198=CARTESIAN_POINT('Ctrl Pts',(-0.276418269242805,1.93430641175822,
8.36015958585972));
#62199=CARTESIAN_POINT('Ctrl Pts',(-0.275971095500023,1.93356302759901,
8.36021273745393));
#62200=CARTESIAN_POINT('Ctrl Pts',(-0.275780664954729,1.93324768016969,
8.36023532774009));
#62201=CARTESIAN_POINT('Ctrl Pts',(-0.275382614641563,1.93259106730347,
8.36028245525117));
#62202=CARTESIAN_POINT('Ctrl Pts',(-0.27517490032497,1.93224986014218,8.36030699591665));
#62203=CARTESIAN_POINT('Ctrl Pts',(-0.274683013387382,1.93144522164978,
8.36036498894045));
#62204=CARTESIAN_POINT('Ctrl Pts',(-0.274398302162044,1.93098212250452,
8.3603984610604));
#62205=CARTESIAN_POINT('Ctrl Pts',(-0.273457757713399,1.92946091331325,
8.36050872638518));
#62206=CARTESIAN_POINT('Ctrl Pts',(-0.272796971398159,1.92840589267734,
8.36058570214581));
#62207=CARTESIAN_POINT('Ctrl Pts',(-0.271234714189636,1.92594340282012,
8.36076656173354));
#62208=CARTESIAN_POINT('Ctrl Pts',(-0.270328380099697,1.9245390757275,8.36087062514322));
#62209=CARTESIAN_POINT('Ctrl Pts',(-0.264722303532908,1.91599923762277,
8.36150916704484));
#62210=CARTESIAN_POINT('Ctrl Pts',(-0.259751634075699,1.90904648453232,
8.3620537711795));
#62211=CARTESIAN_POINT('Ctrl Pts',(-0.245685032853088,1.89093772043069,
8.3635413631272));
#62212=CARTESIAN_POINT('Ctrl Pts',(-0.236109014993976,1.88018046450449,
8.36450105773741));
#62213=CARTESIAN_POINT('Ctrl Pts',(-0.210723619630669,1.8552425705878,8.36690194105967));
#62214=CARTESIAN_POINT('Ctrl Pts',(-0.194169971108228,1.8419132634194,8.36835205146717));
#62215=CARTESIAN_POINT('Ctrl Pts',(-0.176315920496391,1.8302336395527,8.36973294610763));
#62216=CARTESIAN_POINT('Ctrl Pts',(-0.176205410938968,1.83016144418298,
8.36974148657233));
#62217=CARTESIAN_POINT('Ctrl Pts',(-0.175903749687777,1.82996463465255,
8.36976478131237));
#62218=CARTESIAN_POINT('Ctrl Pts',(-0.175712509591243,1.8298401553408,8.36977952899657));
#62219=CARTESIAN_POINT('Ctrl Pts',(-0.171899896619578,1.82736426382098,
8.37007313877608));
#62220=CARTESIAN_POINT('Ctrl Pts',(-0.168231536846383,1.82508551576612,
8.3703483885368));
#62221=CARTESIAN_POINT('Ctrl Pts',(-0.164048256972519,1.8226020119296,8.37065324280955));
#62222=CARTESIAN_POINT('Ctrl Pts',(-0.163577527748032,1.82232416952954,
8.37068741999957));
#62223=CARTESIAN_POINT('Ctrl Pts',(-0.162865609188858,1.82190640655792,
8.37073891457079));
#62224=CARTESIAN_POINT('Ctrl Pts',(-0.162624944383984,1.82176560091257,
8.37075628896612));
#62225=CARTESIAN_POINT('Ctrl Pts',(-0.162206825123207,1.82152169990013,
8.37078641604224));
#62226=CARTESIAN_POINT('Ctrl Pts',(-0.162029454883633,1.82141846167825,
8.3707991780456));
#62227=CARTESIAN_POINT('Ctrl Pts',(-0.161658411584607,1.82120297042727,
8.37082583684298));
#62228=CARTESIAN_POINT('Ctrl Pts',(-0.161464720298202,1.82109074982354,
8.37083973145648));
#62229=CARTESIAN_POINT('Ctrl Pts',(-0.161001374931853,1.82082294181753,
8.37087291831654));
#62230=CARTESIAN_POINT('Ctrl Pts',(-0.160731611086281,1.82066754262183,
8.37089219827109));
#62231=CARTESIAN_POINT('Ctrl Pts',(-0.159817226633964,1.82014256877044,
8.3709574093419));
#62232=CARTESIAN_POINT('Ctrl Pts',(-0.159171547042178,1.81977482914385,
8.37100322233764));
#62233=CARTESIAN_POINT('Ctrl Pts',(-0.157632852281189,1.81890551672235,
8.37111185406888));
#62234=CARTESIAN_POINT('Ctrl Pts',(-0.156738700406101,1.81840595797006,
8.37117454781781));
#62235=CARTESIAN_POINT('Ctrl Pts',(-0.146015241581794,1.81248171037654,
8.37192144240463));
#62236=CARTESIAN_POINT('Ctrl Pts',(-0.13591015483748,1.80756931447792,8.37257542789105));
#62237=CARTESIAN_POINT('Ctrl Pts',(-0.114987700837369,1.79871776199675,
8.37387164294198));
#62238=CARTESIAN_POINT('Ctrl Pts',(-0.104175069907032,1.79481033373575,
8.37451241336183));
#62239=CARTESIAN_POINT('Ctrl Pts',(-0.0681977911061162,1.78394448654688,
8.37661313558764));
#62240=CARTESIAN_POINT('Ctrl Pts',(-0.0423996271884223,1.77946289505241,
8.37808015783452));
#62241=CARTESIAN_POINT('Ctrl Pts',(-0.0148020113481421,1.77806139810893,
8.37975573076812));
#62242=CARTESIAN_POINT('Ctrl Pts',(-0.0132583878551417,1.77799413367224,
8.37984976039698));
#62243=CARTESIAN_POINT('Ctrl Pts',(-0.0111638324911713,1.77791794841732,
8.37997778829323));
#62244=CARTESIAN_POINT('Ctrl Pts',(-0.0106132562710758,1.77789933577686,
8.38001148284188));
#62245=CARTESIAN_POINT('Ctrl Pts',(-0.00968059233818868,1.77787020029484,
8.38006863115311));
#62246=CARTESIAN_POINT('Ctrl Pts',(-0.00929852734156827,1.77785894531533,
8.38009206194372));
#62247=CARTESIAN_POINT('Ctrl Pts',(-0.00856297469243163,1.77783858684496,
8.38013720988414));
#62248=CARTESIAN_POINT('Ctrl Pts',(-0.00820949009489424,1.77782938536787,
8.3801589239324));
#62249=CARTESIAN_POINT('Ctrl Pts',(-0.00737591060267823,1.77780905943351,
8.38021017063445));
#62250=CARTESIAN_POINT('Ctrl Pts',(-0.0068958055477118,1.77779842628839,
8.38023971863681));
#62251=CARTESIAN_POINT('Ctrl Pts',(-0.00549721487744029,1.77777057836495,
8.38032588936334));
#62252=CARTESIAN_POINT('Ctrl Pts',(-0.00457868290780011,1.77775621778919,
8.38038260136456));
#62253=CARTESIAN_POINT('Ctrl Pts',(0.0020123287590675,1.77768135817776,
8.38079041227238));
#62254=CARTESIAN_POINT('Ctrl Pts',(0.00768516421377774,1.77776671808107,
8.38114605540946));
#62255=CARTESIAN_POINT('Ctrl Pts',(0.0261250649637962,1.7785313776521,8.38231823212648));
#62256=CARTESIAN_POINT('Ctrl Pts',(0.0388533011378991,1.77982044408159,
8.38315311713507));
#62257=CARTESIAN_POINT('Ctrl Pts',(0.0796599171670877,1.78642236011341,
8.38590523017834));
#62258=CARTESIAN_POINT('Ctrl Pts',(0.107116888338767,1.79470906028241,8.38788587532245));
#62259=CARTESIAN_POINT('Ctrl Pts',(0.136780512800453,1.8081637392716,8.3899855218027));
#62260=CARTESIAN_POINT('Ctrl Pts',(0.140407643486822,1.80989138397474,8.39024125840119));
#62261=CARTESIAN_POINT('Ctrl Pts',(0.14453358337266,1.81195213532323,8.39053021461082));
#62262=CARTESIAN_POINT('Ctrl Pts',(0.145064712788122,1.81221925327693,8.39056737415495));
#62263=CARTESIAN_POINT('Ctrl Pts',(0.145845894700233,1.81261484093938,8.39062196936374));
#62264=CARTESIAN_POINT('Ctrl Pts',(0.146096519265338,1.81274216858507,8.39063947606104));
#62265=CARTESIAN_POINT('Ctrl Pts',(0.14654274463031,1.81296960456806,8.39067062954465));
#62266=CARTESIAN_POINT('Ctrl Pts',(0.146738409723914,1.81306958505861,8.39068428438318));
#62267=CARTESIAN_POINT('Ctrl Pts',(0.147150279987368,1.81328057304923,8.39071301547411));
#62268=CARTESIAN_POINT('Ctrl Pts',(0.147366461313003,1.81339162473445,8.39072808883609));
#62269=CARTESIAN_POINT('Ctrl Pts',(0.147938790227462,1.81368644708487,8.39076797695414));
#62270=CARTESIAN_POINT('Ctrl Pts',(0.148294722433425,1.81387063845286,8.39079276512074));
#62271=CARTESIAN_POINT('Ctrl Pts',(0.149891275716121,1.81470061818552,8.39090387564516));
#62272=CARTESIAN_POINT('Ctrl Pts',(0.151128052745254,1.81535382728715,8.39098973571893));
#62273=CARTESIAN_POINT('Ctrl Pts',(0.160656583402995,1.82046597308272,8.39164988801422));
#62274=CARTESIAN_POINT('Ctrl Pts',(0.168754472454573,1.82527873234048,8.3922030728907));
#62275=CARTESIAN_POINT('Ctrl Pts',(0.200645091961242,1.8461752214554,8.39439686892825));
#62276=CARTESIAN_POINT('Ctrl Pts',(0.222449475160951,1.86504917268763,8.39594460023162));
#62277=CARTESIAN_POINT('Ctrl Pts',(0.249012395592701,1.89510043033793,8.39826316738812));
#62278=CARTESIAN_POINT('Ctrl Pts',(0.25609982618789,1.90403101956672,8.39893606448791));
#62279=CARTESIAN_POINT('Ctrl Pts',(0.26339430895806,1.91429578825574,8.39970155486363));
#62280=CARTESIAN_POINT('Ctrl Pts',(0.26408409927393,1.91527803405993,8.39977472404634));
#62281=CARTESIAN_POINT('Ctrl Pts',(0.265043186872483,1.9166601051141,8.39987757214404));
#62282=CARTESIAN_POINT('Ctrl Pts',(0.265317104500601,1.91705672458457,8.39990707493418));
#62283=CARTESIAN_POINT('Ctrl Pts',(0.265817034317198,1.91778408312762,8.39996115868353));
#62284=CARTESIAN_POINT('Ctrl Pts',(0.266043321968399,1.91811463245067,8.39998572912189));
#62285=CARTESIAN_POINT('Ctrl Pts',(0.266499715445926,1.91878398242116,8.4000354675717));
#62286=CARTESIAN_POINT('Ctrl Pts',(0.266729792870285,1.91912280145688,8.40006063659699));
#62287=CARTESIAN_POINT('Ctrl Pts',(0.267286287777501,1.91994568359164,8.4001217448425));
#62288=CARTESIAN_POINT('Ctrl Pts',(0.267612036032181,1.92043019559317,8.40015770924133));
#62289=CARTESIAN_POINT('Ctrl Pts',(0.268763226097576,1.92215254424173,8.40028550107465));
#62290=CARTESIAN_POINT('Ctrl Pts',(0.26958140090896,1.92339519432673,8.40037760104398));
#62291=CARTESIAN_POINT('Ctrl Pts',(0.280262733450074,1.93986526874697,8.4015970931591));
#62292=CARTESIAN_POINT('Ctrl Pts',(0.288829797175336,1.95589074399111,8.40277306604974));
#62293=CARTESIAN_POINT('Ctrl Pts',(0.304123502124761,1.99141015214696,8.40535141409662));
#62294=CARTESIAN_POINT('Ctrl Pts',(0.310422819527596,2.01100293492122,8.40675790509365));
#62295=CARTESIAN_POINT('Ctrl Pts',(0.315502735721852,2.0342008423504,8.40834194451299));
#62296=CARTESIAN_POINT('Ctrl Pts',(0.316143264527338,2.03735063632381,8.40855524728323));
#62297=CARTESIAN_POINT('Ctrl Pts',(0.316942815293981,2.04160757229913,8.4088407193618));
#62298=CARTESIAN_POINT('Ctrl Pts',(0.31714333796636,2.04270665816837,8.40891417353523));
#62299=CARTESIAN_POINT('Ctrl Pts',(0.317738036289297,2.04606507845205,8.40913781640207));
#62300=CARTESIAN_POINT('Ctrl Pts',(0.318113821739515,2.04832764351941,8.40928737142928));
#62301=CARTESIAN_POINT('Ctrl Pts',(0.318547934559806,2.05112588990915,8.40947081292755));
#62302=CARTESIAN_POINT('Ctrl Pts',(0.318629105927412,2.05165790537173,8.40950562189478));
#62303=CARTESIAN_POINT('Ctrl Pts',(0.319345581933388,2.05643405909756,8.40981749600457));
#62304=CARTESIAN_POINT('Ctrl Pts',(0.319897426308408,2.06069054819696,8.41009103224958));
#62305=CARTESIAN_POINT('Ctrl Pts',(0.320423449612298,2.06549947362142,8.41039417013517));
#62306=CARTESIAN_POINT('Ctrl Pts',(0.320481406564421,2.06604206368645,8.41042828865567));
#62307=CARTESIAN_POINT('Ctrl Pts',(0.320566871198163,2.06686189011352,8.4104797097972));
#62308=CARTESIAN_POINT('Ctrl Pts',(0.320595397591823,2.06713901582408,8.41049706920583));
#62309=CARTESIAN_POINT('Ctrl Pts',(0.320644308151127,2.06762029388172,8.41052717748673));
#62310=CARTESIAN_POINT('Ctrl Pts',(0.320664856717466,2.06782442875524,8.41053993565342));
#62311=CARTESIAN_POINT('Ctrl Pts',(0.320707422895147,2.06825138336867,8.41056659382704));
#62312=CARTESIAN_POINT('Ctrl Pts',(0.320729403220996,2.06847420630827,8.41058049164128));
#62313=CARTESIAN_POINT('Ctrl Pts',(0.320781417591502,2.06900718069372,8.41061369906985));
#62314=CARTESIAN_POINT('Ctrl Pts',(0.320811234171217,2.06931735421999,8.41063299635232));
#62315=CARTESIAN_POINT('Ctrl Pts',(0.320908662582816,2.07034654392444,8.41069693426005));
#62316=CARTESIAN_POINT('Ctrl Pts',(0.320974308035185,2.07106575069344,8.41074146474658));
#62317=CARTESIAN_POINT('Ctrl Pts',(0.321125059428692,2.07278104982611,8.41084732506675));
#62318=CARTESIAN_POINT('Ctrl Pts',(0.321207949788138,2.07377733624378,8.41090853460866));
#62319=CARTESIAN_POINT('Ctrl Pts',(0.322126593262677,2.08547746936625,8.41162428623593));
#62320=CARTESIAN_POINT('Ctrl Pts',(0.322431683697765,2.09621749507579,8.41225115407617));
#62321=CARTESIAN_POINT('Ctrl Pts',(0.321724317202829,2.12899278310915,8.41412562405545));
#62322=CARTESIAN_POINT('Ctrl Pts',(0.318988739280889,2.15092524378861,8.41533045696976));
#62323=CARTESIAN_POINT('Ctrl Pts',(0.313972921640174,2.17267914297819,8.41659862160365));
#62324=CARTESIAN_POINT('Ctrl Pts',(0.313909932427393,2.17295072083493,8.41661446456874));
#62325=CARTESIAN_POINT('Ctrl Pts',(0.312661413783001,2.17830214749635,8.41692687132574));
#62326=CARTESIAN_POINT('Ctrl Pts',(0.311353112126086,2.18335239884336,8.41722565788024));
#62327=CARTESIAN_POINT('Ctrl Pts',(0.308971055259537,2.19170666106868,8.41772843339678));
#62328=CARTESIAN_POINT('Ctrl Pts',(0.307965406128891,2.19502911209026,8.41793066015776));
#62329=CARTESIAN_POINT('Ctrl Pts',(0.306336575709194,2.2001127588084,8.41824403041404));
#62330=CARTESIAN_POINT('Ctrl Pts',(0.305751406570611,2.20188591304335,8.41835407804502));
#62331=CARTESIAN_POINT('Ctrl Pts',(0.305035311241287,2.20399405564536,8.41848585311103));
#62332=CARTESIAN_POINT('Ctrl Pts',(0.3049191839852,2.2043340593957,8.41850713512105));
#62333=CARTESIAN_POINT('Ctrl Pts',(0.302948696563384,2.21007197169169,8.41886678806722));
#62334=CARTESIAN_POINT('Ctrl Pts',(0.300951926554263,2.21541959711119,8.41920943974378));
#62335=CARTESIAN_POINT('Ctrl Pts',(0.298446908288367,2.22162064269975,8.41961660319025));
#62336=CARTESIAN_POINT('Ctrl Pts',(0.298075354254859,2.2225284495538,8.41967645979995));
#62337=CARTESIAN_POINT('Ctrl Pts',(0.297508201564514,2.22389630954061,8.41976703276733));
#62338=CARTESIAN_POINT('Ctrl Pts',(0.29731566507344,2.22435763271075,8.4197976452602));
#62339=CARTESIAN_POINT('Ctrl Pts',(0.29696987114851,2.22518077190033,8.41985238577364));
#62340=CARTESIAN_POINT('Ctrl Pts',(0.29681702353858,2.22554275988305,8.41987649982497));
#62341=CARTESIAN_POINT('Ctrl Pts',(0.29649286871903,2.22630655255101,8.41992746755679));
#62342=CARTESIAN_POINT('Ctrl Pts',(0.296321406006372,2.22670829001284,8.41995432649574));
#62343=CARTESIAN_POINT('Ctrl Pts',(0.295870789081046,2.22775816924708,8.42002465259536));
#62344=CARTESIAN_POINT('Ctrl Pts',(0.295590322883945,2.22840574226066,8.42006816446474));
#62345=CARTESIAN_POINT('Ctrl Pts',(0.294328378687823,2.23129342141016,8.42026279880509));
#62346=CARTESIAN_POINT('Ctrl Pts',(0.293323567647281,2.23352318577301,8.42041471837392));
#62347=CARTESIAN_POINT('Ctrl Pts',(0.290622543758115,2.23933933762203,8.42081537344335));
#62348=CARTESIAN_POINT('Ctrl Pts',(0.288885357859103,2.24290612901568,8.42106550621722));
#62349=CARTESIAN_POINT('Ctrl Pts',(0.280277445407858,2.25978121043864,8.42227065807382));
#62350=CARTESIAN_POINT('Ctrl Pts',(0.272551238605597,2.27263023996599,8.4232549979425));
#62351=CARTESIAN_POINT('Ctrl Pts',(0.255821728664446,2.29651380919368,8.42520855876348));
#62352=CARTESIAN_POINT('Ctrl Pts',(0.246924422897168,2.30758310271861,8.426173585409));
#62353=CARTESIAN_POINT('Ctrl Pts',(0.226962375438949,2.32931195581173,8.4281619160929));
#62354=CARTESIAN_POINT('Ctrl Pts',(0.215804750006076,2.33984230020496,8.42918118325994));
#62355=CARTESIAN_POINT('Ctrl Pts',(0.20323530841813,2.35011479461538,8.43020205794527));
#62356=CARTESIAN_POINT('Ctrl Pts',(0.202529379716162,2.35068675966678,8.43025899241625));
#62357=CARTESIAN_POINT('Ctrl Pts',(0.201576344870802,2.35145228437,8.43033530885438));
#62358=CARTESIAN_POINT('Ctrl Pts',(0.201331369852359,2.35164847236129,8.43035487738665));
#62359=CARTESIAN_POINT('Ctrl Pts',(0.200918333549415,2.35197826287601,8.43038778861869));
#62360=CARTESIAN_POINT('Ctrl Pts',(0.200750425323612,2.35211205534701,8.43040114499502));
#62361=CARTESIAN_POINT('Ctrl Pts',(0.200428047906117,2.35236840554695,8.43042674490399));
#62362=CARTESIAN_POINT('Ctrl Pts',(0.200273601065332,2.35249098839829,8.43043899020527));
#62363=CARTESIAN_POINT('Ctrl Pts',(0.199907648648315,2.35278089399213,8.43046795921089));
#62364=CARTESIAN_POINT('Ctrl Pts',(0.199696045731322,2.35294809284932,8.43048467393425));
#62365=CARTESIAN_POINT('Ctrl Pts',(0.199081713413944,2.35343225853603,8.43053309748792));
#62366=CARTESIAN_POINT('Ctrl Pts',(0.198678435137737,2.35374853241406,8.43056475679251));
#62367=CARTESIAN_POINT('Ctrl Pts',(0.195754801823926,2.35603017009604,8.43079336338358));
#62368=CARTESIAN_POINT('Ctrl Pts',(0.19320597567093,2.3579589953376,8.43098776625499));
#62369=CARTESIAN_POINT('Ctrl Pts',(0.185764100317055,2.36341844225202,8.4315427451628));
#62370=CARTESIAN_POINT('Ctrl Pts',(0.180799859106272,2.36685013975899,8.43189755566925));
#62371=CARTESIAN_POINT('Ctrl Pts',(0.158872968525616,2.38111483178102,8.43341278685427));
#62372=CARTESIAN_POINT('Ctrl Pts',(0.141012145262795,2.39048555531205,8.43451860139516));
#62373=CARTESIAN_POINT('Ctrl Pts',(0.102815970011274,2.40616645734095,8.43683842911468));
#62374=CARTESIAN_POINT('Ctrl Pts',(0.0824983582121419,2.4122544511575,8.43805086071517));
#62375=CARTESIAN_POINT('Ctrl Pts',(0.0604564839611807,2.41655628160546,
8.43941484745044));
#62376=CARTESIAN_POINT('Ctrl Pts',(0.0591789813705468,2.41679759147346,
8.43949405216134));
#62377=CARTESIAN_POINT('Ctrl Pts',(0.0573964288908414,2.41712314278283,
8.43960479094875));
#62378=CARTESIAN_POINT('Ctrl Pts',(0.0568925735448265,2.41721392278485,
8.4396361168865));
#62379=CARTESIAN_POINT('Ctrl Pts',(0.0560225421013413,2.4173685374466,8.43969025207543));
#62380=CARTESIAN_POINT('Ctrl Pts',(0.0556564668790967,2.41743294012617,
8.43971304322576));
#62381=CARTESIAN_POINT('Ctrl Pts',(0.0548989325062827,2.41756486051501,
8.43976023348141));
#62382=CARTESIAN_POINT('Ctrl Pts',(0.054507458442941,2.41763228802522,8.43978463541195));
#62383=CARTESIAN_POINT('Ctrl Pts',(0.0535929039131717,2.41778807041089,
8.43984167877783));
#62384=CARTESIAN_POINT('Ctrl Pts',(0.0530697291148096,2.41787585767345,
8.43987433817805));
#62385=CARTESIAN_POINT('Ctrl Pts',(0.0514231181477317,2.41814797600156,
8.43997721641948));
#62386=CARTESIAN_POINT('Ctrl Pts',(0.0502989299011547,2.41832764459189,
8.44004758296037));
#62387=CARTESIAN_POINT('Ctrl Pts',(0.0380842663052069,2.42021348188773,
8.44081357653443));
#62388=CARTESIAN_POINT('Ctrl Pts',(0.0269141238935459,2.42134508728867,
8.44152734950925));
#62389=CARTESIAN_POINT('Ctrl Pts',(-0.00094347221127675,2.42270457418021,
8.44334280122242));
#62390=CARTESIAN_POINT('Ctrl Pts',(-0.0176319661942657,2.42222373875657,
8.44446273442364));
#62391=CARTESIAN_POINT('Ctrl Pts',(-0.0559735906195382,2.41813100078004,
8.44707124596398));
#62392=CARTESIAN_POINT('Ctrl Pts',(-0.0774496561311467,2.41359550571066,
8.44855999820637));
#62393=CARTESIAN_POINT('Ctrl Pts',(-0.0994548686942221,2.40654750168359,
8.45001752161645));
#62394=CARTESIAN_POINT('Ctrl Pts',(-0.100605911993593,2.40617167125275,
8.4500935469848));
#62395=CARTESIAN_POINT('Ctrl Pts',(-0.102126997406757,2.40566551305355,
8.45019370336743));
#62396=CARTESIAN_POINT('Ctrl Pts',(-0.102498939531805,2.40554099048795,
8.45021816941118));
#62397=CARTESIAN_POINT('Ctrl Pts',(-0.10307635409797,2.40534650474978,8.45025611198134));
#62398=CARTESIAN_POINT('Ctrl Pts',(-0.10328198314249,2.40527701304859,8.45026961635238));
#62399=CARTESIAN_POINT('Ctrl Pts',(-0.103673838847605,2.40514414538069,
8.45029533588346));
#62400=CARTESIAN_POINT('Ctrl Pts',(-0.103860076437212,2.40508080707297,
8.45030755313817));
#62401=CARTESIAN_POINT('Ctrl Pts',(-0.104297232579509,2.4049316861513,8.45033621560172));
#62402=CARTESIAN_POINT('Ctrl Pts',(-0.104548102947228,2.40484576446814,
8.45035265241376));
#62403=CARTESIAN_POINT('Ctrl Pts',(-0.105066129068437,2.40466762877337,
8.45038656944156));
#62404=CARTESIAN_POINT('Ctrl Pts',(-0.105333270276923,2.40457537273067,
8.45040404715185));
#62405=CARTESIAN_POINT('Ctrl Pts',(-0.106751976128618,2.4040833391314,8.45049679868113));
#62406=CARTESIAN_POINT('Ctrl Pts',(-0.107901407388321,2.40367737475766,
8.45057171000643));
#62407=CARTESIAN_POINT('Ctrl Pts',(-0.110877350222705,2.40260727993817,
8.45076511465639));
#62408=CARTESIAN_POINT('Ctrl Pts',(-0.112700235596778,2.4019331216899,8.45088304779185));
#62409=CARTESIAN_POINT('Ctrl Pts',(-0.120394342735421,2.39900821643135,
8.45137899815008));
#62410=CARTESIAN_POINT('Ctrl Pts',(-0.126205489376465,2.39660225307005,
8.45174905479962));
#62411=CARTESIAN_POINT('Ctrl Pts',(-0.140468669379752,2.39020174849718,
8.45265472868859));
#62412=CARTESIAN_POINT('Ctrl Pts',(-0.148824478333991,2.38600663467383,
8.45318302032387));
#62413=CARTESIAN_POINT('Ctrl Pts',(-0.164822153083709,2.37708361813717,
8.45421110403603));
#62414=CARTESIAN_POINT('Ctrl Pts',(-0.172471870442244,2.37238782826001,
8.45471074376862));
#62415=CARTESIAN_POINT('Ctrl Pts',(-0.188411024728193,2.36166258570287,
8.45578723807841));
#62416=CARTESIAN_POINT('Ctrl Pts',(-0.196628731048234,2.35554480848539,
8.45636447709347));
#62417=CARTESIAN_POINT('Ctrl Pts',(-0.205412272779601,2.34833091844971,
8.4570178570847));
#62418=CARTESIAN_POINT('Ctrl Pts',(-0.206279805775255,2.34761076018854,
8.45708280005337));
#62419=CARTESIAN_POINT('Ctrl Pts',(-0.216161363688582,2.33931988799238,
8.45782736116971));
#62420=CARTESIAN_POINT('Ctrl Pts',(-0.224756929824862,2.33126611890626,
8.45852176521525));
#62421=CARTESIAN_POINT('Ctrl Pts',(-0.233644531959335,2.32197430752714,
8.45930333329821));
#62422=CARTESIAN_POINT('Ctrl Pts',(-0.234392939503212,2.32118388364044,
8.45936966939292));
#62423=CARTESIAN_POINT('Ctrl Pts',(-0.235498305847194,2.32000455043293,
8.45946843090707));
#62424=CARTESIAN_POINT('Ctrl Pts',(-0.235858342044654,2.31961852551825,
8.45950072430516));
#62425=CARTESIAN_POINT('Ctrl Pts',(-0.236473155571586,2.31895607696545,
8.45955608558057));
#62426=CARTESIAN_POINT('Ctrl Pts',(-0.23672840143305,2.31868008802608,8.45957913340888));
#62427=CARTESIAN_POINT('Ctrl Pts',(-0.237224135961085,2.31814218156596,
8.45962402174879));
#62428=CARTESIAN_POINT('Ctrl Pts',(-0.237464675306515,2.31788031127402,
8.45964586005976));
#62429=CARTESIAN_POINT('Ctrl Pts',(-0.238039159366992,2.31725280077638,
8.45969815544192));
#62430=CARTESIAN_POINT('Ctrl Pts',(-0.238372694939274,2.31688678876394,
8.45972862978243));
#62431=CARTESIAN_POINT('Ctrl Pts',(-0.239062910492958,2.316125851389,8.45979192793603));
#62432=CARTESIAN_POINT('Ctrl Pts',(-0.239419458298895,2.3157308086352,8.45982475720346));
#62433=CARTESIAN_POINT('Ctrl Pts',(-0.24034965668487,2.31469503433844,8.45991075044783));
#62434=CARTESIAN_POINT('Ctrl Pts',(-0.240921721004999,2.31405288963972,
8.45996398086783));
#62435=CARTESIAN_POINT('Ctrl Pts',(-0.245480400421749,2.30889432685496,
8.46039095428239));
#62436=CARTESIAN_POINT('Ctrl Pts',(-0.24934200503406,2.30426948722472,8.46076985029906));
#62437=CARTESIAN_POINT('Ctrl Pts',(-0.260117069755862,2.29060370305715,
8.46187939957853));
#62438=CARTESIAN_POINT('Ctrl Pts',(-0.266683675229906,2.2813020461917,8.46262281460333));
#62439=CARTESIAN_POINT('Ctrl Pts',(-0.27495287018226,2.26816446217166,8.46365480892187));
#62440=CARTESIAN_POINT('Ctrl Pts',(-0.277093580512788,2.26461322326421,
8.46393202486914));
#62441=CARTESIAN_POINT('Ctrl Pts',(-0.281392767825059,2.2571596761643,8.46450973788012));
#62442=CARTESIAN_POINT('Ctrl Pts',(-0.283539984604242,2.25325185008603,
8.4648103564494));
#62443=CARTESIAN_POINT('Ctrl Pts',(-0.294565571132059,2.2321604211386,8.46641851296347));
#62444=CARTESIAN_POINT('Ctrl Pts',(-0.301965070820477,2.21424727773257,
8.46773701697062));
#62445=CARTESIAN_POINT('Ctrl Pts',(-0.30921991471604,2.19093900410105,8.46932095262835));
#62446=CARTESIAN_POINT('Ctrl Pts',(-0.310611787633625,2.18606499090623,
8.4696450500948));
#62447=CARTESIAN_POINT('Ctrl Pts',(-0.312048071163627,2.18054551429612,
8.47000255969751));
#62448=CARTESIAN_POINT('Ctrl Pts',(-0.312206120470207,2.17993070090641,
8.47004225081337));
#62449=CARTESIAN_POINT('Ctrl Pts',(-0.312433418700957,2.1790355482132,8.47009984438616));
#62450=CARTESIAN_POINT('Ctrl Pts',(-0.312504107824726,2.17875558136897,
8.47011782947241));
#62451=CARTESIAN_POINT('Ctrl Pts',(-0.31262820011313,2.17826131161598,8.47014953186297));
#62452=CARTESIAN_POINT('Ctrl Pts',(-0.312681759335453,2.17804704851501,
8.47016325824607));
#62453=CARTESIAN_POINT('Ctrl Pts',(-0.312792884789983,2.17760054187807,
8.47019182851542));
#62454=CARTESIAN_POINT('Ctrl Pts',(-0.312850412525768,2.17736828974691,
8.47020667012873));
#62455=CARTESIAN_POINT('Ctrl Pts',(-0.312999579040515,2.17676318493524,
8.47024528835668));
#62456=CARTESIAN_POINT('Ctrl Pts',(-0.31309081060403,2.17639023078829,8.47026904134436));
#62457=CARTESIAN_POINT('Ctrl Pts',(-0.313287658567591,2.17557924081101,
8.47032058713231));
#62458=CARTESIAN_POINT('Ctrl Pts',(-0.31339302345367,2.1751411439136,8.47034836557216));
#62459=CARTESIAN_POINT('Ctrl Pts',(-0.314267400564064,2.17147173764769,
8.47058048559791));
#62460=CARTESIAN_POINT('Ctrl Pts',(-0.314987369257546,2.16822878878098,
8.47078208482908));
#62461=CARTESIAN_POINT('Ctrl Pts',(-0.320037310506056,2.14369556163156,
8.47228454619064));
#62462=CARTESIAN_POINT('Ctrl Pts',(-0.322254947008397,2.12202539477509,
8.47348612124905));
#62463=CARTESIAN_POINT('Ctrl Pts',(-0.322274864620942,2.10029539558797,
8.47470126795611));
#62464=CARTESIAN_POINT('',(-0.322274924948143,2.09973710004718,8.72483341161327));
#62465=CARTESIAN_POINT('Ctrl Pts',(-0.322274864675418,2.1002953361489,8.47470127127996));
#62466=CARTESIAN_POINT('Ctrl Pts',(-0.322298157958911,2.07487738506705,
8.47612264914654));
#62467=CARTESIAN_POINT('Ctrl Pts',(-0.319314602306005,2.04954914401777,
8.47755844204353));
#62468=CARTESIAN_POINT('Ctrl Pts',(-0.313190622656218,2.02401632946606,
8.47915428160579));
#62469=CARTESIAN_POINT('Ctrl Pts',(-0.312991074432553,2.0231984921232,8.47920554819074));
#62470=CARTESIAN_POINT('Ctrl Pts',(-0.312661995217988,2.02187236403647,
8.47928892536041));
#62471=CARTESIAN_POINT('Ctrl Pts',(-0.312534422737548,2.02136358760759,
8.47932097287557));
#62472=CARTESIAN_POINT('Ctrl Pts',(-0.31228535331439,2.02038044514755,8.4793830163082));
#62473=CARTESIAN_POINT('Ctrl Pts',(-0.312164016106489,2.01990603984275,
8.47941300700011));
#62474=CARTESIAN_POINT('Ctrl Pts',(-0.311952899388195,2.01908838111012,
8.47946478816371));
#62475=CARTESIAN_POINT('Ctrl Pts',(-0.311863633140215,2.01874499504009,
8.47948656199237));
#62476=CARTESIAN_POINT('Ctrl Pts',(-0.311678073725247,2.01803600226395,
8.47953157613093));
#62477=CARTESIAN_POINT('Ctrl Pts',(-0.311581703915576,2.01767041631876,
8.47955481889614));
#62478=CARTESIAN_POINT('Ctrl Pts',(-0.311347209606714,2.01678715385805,
8.47961105070911));
#62479=CARTESIAN_POINT('Ctrl Pts',(-0.311208437370691,2.01626965187767,
8.47964406072336));
#62480=CARTESIAN_POINT('Ctrl Pts',(-0.31069030235538,2.01435653375134,8.47976633138556));
#62481=CARTESIAN_POINT('Ctrl Pts',(-0.310302841181847,2.01296314611725,
8.47985585471153));
#62482=CARTESIAN_POINT('Ctrl Pts',(-0.303201636624754,1.98807604272175,
8.48146337717821));
#62483=CARTESIAN_POINT('Ctrl Pts',(-0.293848405738632,1.9654234671219,8.4830727320084));
#62484=CARTESIAN_POINT('Ctrl Pts',(-0.279702605687232,1.93984149803431,
8.48504532844743));
#62485=CARTESIAN_POINT('Ctrl Pts',(-0.277282085069137,1.93568646421829,
8.4853706935095));
#62486=CARTESIAN_POINT('Ctrl Pts',(-0.272413496451516,1.92774324614534,
8.48600116994133));
#62487=CARTESIAN_POINT('Ctrl Pts',(-0.269977041663995,1.9239491555125,8.48630621317142));
#62488=CARTESIAN_POINT('Ctrl Pts',(-0.261177484899353,1.91085882160613,
8.48737014607697));
#62489=CARTESIAN_POINT('Ctrl Pts',(-0.254406851938782,1.90184536906323,
8.48812372579876));
#62490=CARTESIAN_POINT('Ctrl Pts',(-0.243957012551486,1.88935493790551,
8.48918063605117));
#62491=CARTESIAN_POINT('Ctrl Pts',(-0.240646724324148,1.88558095431011,
8.4895017439435));
#62492=CARTESIAN_POINT('Ctrl Pts',(-0.236926435956432,1.88153428805485,
8.48984655820794));
#62493=CARTESIAN_POINT('Ctrl Pts',(-0.236602682444027,1.88118369800704,
8.48987643599668));
#62494=CARTESIAN_POINT('Ctrl Pts',(-0.236077369300966,1.88061736966058,
8.48992470420759));
#62495=CARTESIAN_POINT('Ctrl Pts',(-0.235876291324364,1.88040118856554,
8.48994313049929));
#62496=CARTESIAN_POINT('Ctrl Pts',(-0.235487866938806,1.87998473835891,
8.4899786285144));
#62497=CARTESIAN_POINT('Ctrl Pts',(-0.235300561534521,1.8797844315829,8.48999570332742));
#62498=CARTESIAN_POINT('Ctrl Pts',(-0.234964947855461,1.87942643910998,
8.49002622074851));
#62499=CARTESIAN_POINT('Ctrl Pts',(-0.234816736649928,1.8792686640405,8.4900396707516));
#62500=CARTESIAN_POINT('Ctrl Pts',(-0.234519462130586,1.87895284506744,
8.49006659423363));
#62501=CARTESIAN_POINT('Ctrl Pts',(-0.234370398611091,1.87879480323161,
8.49008006757644));
#62502=CARTESIAN_POINT('Ctrl Pts',(-0.233951096534526,1.87835114559316,
8.49011789147779));
#62503=CARTESIAN_POINT('Ctrl Pts',(-0.233680493737948,1.8780658722056,8.49014221390746));
#62504=CARTESIAN_POINT('Ctrl Pts',(-0.232569402664169,1.87689882900213,
8.49024172596749));
#62505=CARTESIAN_POINT('Ctrl Pts',(-0.231724426237672,1.8760213180857,8.49031657319546));
#62506=CARTESIAN_POINT('Ctrl Pts',(-0.215266184678152,1.8591222105287,8.49175893641388));
#62507=CARTESIAN_POINT('Ctrl Pts',(-0.198028736053994,1.84476167561535,
8.49300375565353));
#62508=CARTESIAN_POINT('Ctrl Pts',(-0.169385222980104,1.82556177567674,
8.49493115286423));
#62509=CARTESIAN_POINT('Ctrl Pts',(-0.158959197454201,1.81939413697203,
8.49560739826756));
#62510=CARTESIAN_POINT('Ctrl Pts',(-0.13957510084302,1.80935492859208,8.49685255649649));
#62511=CARTESIAN_POINT('Ctrl Pts',(-0.130741439654788,1.80527569032136,
8.49741570603977));
#62512=CARTESIAN_POINT('Ctrl Pts',(-0.118131539108899,1.8001312268028,8.49822269578325));
#62513=CARTESIAN_POINT('Ctrl Pts',(-0.114499464785686,1.79872568596785,
8.49845545503784));
#62514=CARTESIAN_POINT('Ctrl Pts',(-0.108578731967018,1.79655700870703,
8.49883586517626));
#62515=CARTESIAN_POINT('Ctrl Pts',(-0.106305351733928,1.79575312375438,
8.49898216099628));
#62516=CARTESIAN_POINT('Ctrl Pts',(-0.103530056554027,1.79480666045679,
8.49916110157431));
#62517=CARTESIAN_POINT('Ctrl Pts',(-0.103036496911362,1.79463967610239,
8.49919293762443));
#62518=CARTESIAN_POINT('Ctrl Pts',(-0.102080694484082,1.79431888386117,
8.49925461613643));
#62519=CARTESIAN_POINT('Ctrl Pts',(-0.101618503365226,1.79416492562182,
8.49928445354622));
#62520=CARTESIAN_POINT('Ctrl Pts',(-0.100819417167313,1.79390075728381,
8.4993360609682));
#62521=CARTESIAN_POINT('Ctrl Pts',(-0.100482685134412,1.79379005362996,
8.4993578146614));
#62522=CARTESIAN_POINT('Ctrl Pts',(-0.0997854205558294,1.79356209568316,
8.4994028733816));
#62523=CARTESIAN_POINT('Ctrl Pts',(-0.0994248625074841,1.79344492163551,
8.49942618101374));
#62524=CARTESIAN_POINT('Ctrl Pts',(-0.0985506143273258,1.79316251333776,
8.49948271405068));
#62525=CARTESIAN_POINT('Ctrl Pts',(-0.0980367156482074,1.79299793293082,
8.49951596090577));
#62526=CARTESIAN_POINT('Ctrl Pts',(-0.0961205360674598,1.79238956208202,
8.49963998907533));
#62527=CARTESIAN_POINT('Ctrl Pts',(-0.0947156521184655,1.79195408767742,
8.49973104289575));
#62528=CARTESIAN_POINT('Ctrl Pts',(-0.0714744453803711,1.7849239879905,
8.50123947653329));
#62529=CARTESIAN_POINT('Ctrl Pts',(-0.0490062202099829,1.78065772378202,
8.50273565493494));
#62530=CARTESIAN_POINT('Ctrl Pts',(-0.00961311279734053,1.77743462748962,
8.50539683366068));
#62531=CARTESIAN_POINT('Ctrl Pts',(0.00713495622397891,1.77737028299389,
8.50653783079707));
#62532=CARTESIAN_POINT('Ctrl Pts',(0.0333573205564837,1.77931312919962,
8.5082868217346));
#62533=CARTESIAN_POINT('Ctrl Pts',(0.0428669914389807,1.78044524774001,
8.50891283919201));
#62534=CARTESIAN_POINT('Ctrl Pts',(0.05367535124866,1.78222328854958,8.50960474027681));
#62535=CARTESIAN_POINT('Ctrl Pts',(0.0550362127610522,1.78245614929647,
8.50969149523809));
#62536=CARTESIAN_POINT('Ctrl Pts',(0.056684313212086,1.78274907364949,8.50979608877205));
#62537=CARTESIAN_POINT('Ctrl Pts',(0.0569729930320736,1.7828007886183,8.50981439166232));
#62538=CARTESIAN_POINT('Ctrl Pts',(0.0575300862652771,1.78290137302047,
8.50984967795719));
#62539=CARTESIAN_POINT('Ctrl Pts',(0.0577985088457912,1.78295018934792,
8.50986666435275));
#62540=CARTESIAN_POINT('Ctrl Pts',(0.0582611970181856,1.78303494265621,
8.50989591721373));
#62541=CARTESIAN_POINT('Ctrl Pts',(0.0584554913431511,1.78307071737125,
8.5099081929619));
#62542=CARTESIAN_POINT('Ctrl Pts',(0.0588594157771167,1.78314547460537,
8.50993369613674));
#62543=CARTESIAN_POINT('Ctrl Pts',(0.0590690394808009,1.78318448638976,
8.5099469218247));
#62544=CARTESIAN_POINT('Ctrl Pts',(0.0596454393599121,1.78329234860351,
8.50998326222909));
#62545=CARTESIAN_POINT('Ctrl Pts',(0.0600121363832061,1.78336162838408,
8.51000635235882));
#62546=CARTESIAN_POINT('Ctrl Pts',(0.0614301271179904,1.78363208002385,
8.51009553052319));
#62547=CARTESIAN_POINT('Ctrl Pts',(0.0624805516175137,1.78383785480682,
8.51016135890689));
#62548=CARTESIAN_POINT('Ctrl Pts',(0.0825881666887994,1.78788099820235,
8.51141733271637));
#62549=CARTESIAN_POINT('Ctrl Pts',(0.101263874154127,1.79343034922647,8.51251377699693));
#62550=CARTESIAN_POINT('Ctrl Pts',(0.134568304867893,1.80670539640465,8.51452126888673));
#62551=CARTESIAN_POINT('Ctrl Pts',(0.149322454176347,1.81393508954759,8.51543178774858));
#62552=CARTESIAN_POINT('Ctrl Pts',(0.169153404684813,1.82560626402644,8.51674939128876));
#62553=CARTESIAN_POINT('Ctrl Pts',(0.174740820852452,1.82913022542743,8.51713173276097));
#62554=CARTESIAN_POINT('Ctrl Pts',(0.186446155509846,1.83702569549574,8.51796125900637));
#62555=CARTESIAN_POINT('Ctrl Pts',(0.192527173766854,1.84144453720802,8.51840986863519));
#62556=CARTESIAN_POINT('Ctrl Pts',(0.199336608998842,1.84676618660709,8.51893544069666));
#62557=CARTESIAN_POINT('Ctrl Pts',(0.20022169960771,1.8474654105113,8.51900422011868));
#62558=CARTESIAN_POINT('Ctrl Pts',(0.201516702376564,1.84849955376657,8.51910554779072));
#62559=CARTESIAN_POINT('Ctrl Pts',(0.201929495922301,1.84883086482685,8.51913795138844));
#62560=CARTESIAN_POINT('Ctrl Pts',(0.202650505000997,1.84941247817276,8.51919473351801));
#62561=CARTESIAN_POINT('Ctrl Pts',(0.202959078489603,1.84966233657509,8.5192190941399));
#62562=CARTESIAN_POINT('Ctrl Pts',(0.203555881700145,1.85014740935363,8.51926632478465));
#62563=CARTESIAN_POINT('Ctrl Pts',(0.20384416757373,1.85038255395146,8.51928919196431));
#62564=CARTESIAN_POINT('Ctrl Pts',(0.204529179163417,1.85094327175224,8.51934365316465));
#62565=CARTESIAN_POINT('Ctrl Pts',(0.204925534695703,1.85126929373405,8.51937526536341));
#62566=CARTESIAN_POINT('Ctrl Pts',(0.206328890910064,1.85242925474074,8.51948755111807));
#62567=CARTESIAN_POINT('Ctrl Pts',(0.207331583152448,1.85326836506218,8.51956843520224));
#62568=CARTESIAN_POINT('Ctrl Pts',(0.223690240677228,1.86712835939027,8.52089895254329));
#62569=CARTESIAN_POINT('Ctrl Pts',(0.237794986637941,1.88155139091264,8.52220913604721));
#62570=CARTESIAN_POINT('Ctrl Pts',(0.264299569133966,1.91428374563332,8.52502915288392));
#62571=CARTESIAN_POINT('Ctrl Pts',(0.276352588634905,1.93274562434885,8.52653916103517));
#62572=CARTESIAN_POINT('Ctrl Pts',(0.28905054417156,1.95736899163948,8.52836514342316));
#62573=CARTESIAN_POINT('Ctrl Pts',(0.291533972804677,1.96251628114577,8.5287370145117));
#62574=CARTESIAN_POINT('Ctrl Pts',(0.294972671495013,1.97015626948368,8.52927196157799));
#62575=CARTESIAN_POINT('Ctrl Pts',(0.296035859308263,1.9725988916549,8.52944049942771));
#62576=CARTESIAN_POINT('Ctrl Pts',(0.29726927942361,1.97553145436602,8.52963963837981));
#62577=CARTESIAN_POINT('Ctrl Pts',(0.297468732389164,1.97600888499204,8.52967195814453));
#62578=CARTESIAN_POINT('Ctrl Pts',(0.297770795324136,1.97673685720115,8.52972108283385));
#62579=CARTESIAN_POINT('Ctrl Pts',(0.297874239639976,1.97698704832085,8.52973793818996));
#62580=CARTESIAN_POINT('Ctrl Pts',(0.298052526644022,1.97741979803185,8.52976704387263));
#62581=CARTESIAN_POINT('Ctrl Pts',(0.298127516838931,1.9776022947206,8.52977930320437));
#62582=CARTESIAN_POINT('Ctrl Pts',(0.298283566009757,1.97798305138086,8.52980484954653));
#62583=CARTESIAN_POINT('Ctrl Pts',(0.29836459468634,1.97818132269577,8.52981813468054));
#62584=CARTESIAN_POINT('Ctrl Pts',(0.298563186448095,1.97866864916119,8.52985074501205));
#62585=CARTESIAN_POINT('Ctrl Pts',(0.298680527785691,1.97895779528616,8.52987005670967));
#62586=CARTESIAN_POINT('Ctrl Pts',(0.299133228380408,1.98007798202666,8.52994473091039));
#62587=CARTESIAN_POINT('Ctrl Pts',(0.299465544823922,1.980910259786,8.52999991093429));
#62588=CARTESIAN_POINT('Ctrl Pts',(0.304984677020462,1.9949019711,8.53092268331537));
#62589=CARTESIAN_POINT('Ctrl Pts',(0.309303830367882,2.00838940012572,8.53174015932404));
#62590=CARTESIAN_POINT('Ctrl Pts',(0.317211088658042,2.04014006726122,8.53359337687551));
#62591=CARTESIAN_POINT('Ctrl Pts',(0.320133031877508,2.05851564408632,8.53461538679904));
#62592=CARTESIAN_POINT('Ctrl Pts',(0.322576716223429,2.09273022512197,8.53655956497202));
#62593=CARTESIAN_POINT('Ctrl Pts',(0.322547057551053,2.10847856355302,8.5374701523147));
#62594=CARTESIAN_POINT('Ctrl Pts',(0.321245661597191,2.1257888931757,8.53851710436484));
#62595=CARTESIAN_POINT('Ctrl Pts',(0.321110869980468,2.12741625678343,8.53861596496862));
#62596=CARTESIAN_POINT('Ctrl Pts',(0.320854578506306,2.13024866638306,8.53878882063849));
#62597=CARTESIAN_POINT('Ctrl Pts',(0.320738641458448,2.13145419175834,8.53886264075579));
#62598=CARTESIAN_POINT('Ctrl Pts',(0.32056081909363,2.1331998863911,8.538969909188));
#62599=CARTESIAN_POINT('Ctrl Pts',(0.320504356582679,2.1337406075844,8.53900318675328));
#62600=CARTESIAN_POINT('Ctrl Pts',(0.320404034035923,2.13467838192459,8.53906099067864));
#62601=CARTESIAN_POINT('Ctrl Pts',(0.320360803362932,2.135075502359,8.5390854971641));
#62602=CARTESIAN_POINT('Ctrl Pts',(0.320276287716734,2.13583867816492,8.53913264767996));
#62603=CARTESIAN_POINT('Ctrl Pts',(0.320235113216692,2.13620474537355,8.53915528819268));
#62604=CARTESIAN_POINT('Ctrl Pts',(0.32013667552013,2.13706661177312,8.53920865013098));
#62605=CARTESIAN_POINT('Ctrl Pts',(0.320078888166211,2.13756234906433,8.53923938804583));
#62606=CARTESIAN_POINT('Ctrl Pts',(0.319904916426641,2.13902523475362,8.53933022633979));
#62607=CARTESIAN_POINT('Ctrl Pts',(0.319785499182839,2.13999198645359,8.53939042860866));
#62608=CARTESIAN_POINT('Ctrl Pts',(0.318690869276193,2.14853512276183,8.53992397292191));
#62609=CARTESIAN_POINT('Ctrl Pts',(0.317451025307856,2.15607458234423,8.54040564037596));
#62610=CARTESIAN_POINT('Ctrl Pts',(0.314982444566395,2.16834496291487,8.5412083176936));
#62611=CARTESIAN_POINT('Ctrl Pts',(0.31391185045856,2.1731048604808,8.54152437327844));
#62612=CARTESIAN_POINT('Ctrl Pts',(0.307207189187937,2.20004236586333,8.54333934688574));
#62613=CARTESIAN_POINT('Ctrl Pts',(0.299332052898711,2.2215929180072,8.5449002552512));
#62614=CARTESIAN_POINT('Ctrl Pts',(0.28593047106801,2.2488669652428,8.54694651120588));
#62615=CARTESIAN_POINT('Ctrl Pts',(0.282382692096742,2.25549158846926,8.54744890952973));
#62616=CARTESIAN_POINT('Ctrl Pts',(0.274731595035463,2.26865099140515,8.5484502763893));
#62617=CARTESIAN_POINT('Ctrl Pts',(0.270618447379577,2.27517501308584,8.54894850228024));
#62618=CARTESIAN_POINT('Ctrl Pts',(0.265902495166367,2.28209194276354,8.54947354487824));
#62619=CARTESIAN_POINT('Ctrl Pts',(0.265528449677218,2.28263694857682,8.54951489216924));
#62620=CARTESIAN_POINT('Ctrl Pts',(0.264978520714319,2.28343296627837,8.54957524520067));
#62621=CARTESIAN_POINT('Ctrl Pts',(0.264803954837154,2.28368487978628,8.54959433944103));
#62622=CARTESIAN_POINT('Ctrl Pts',(0.264501770184818,2.2841196320595,8.5496272821941));
#62623=CARTESIAN_POINT('Ctrl Pts',(0.264374320748109,2.28430258780272,8.54964114231642));
#62624=CARTESIAN_POINT('Ctrl Pts',(0.264128565109189,2.28465459456044,8.54966780301087));
#62625=CARTESIAN_POINT('Ctrl Pts',(0.264010286678735,2.28482366387271,8.54968060545407));
#62626=CARTESIAN_POINT('Ctrl Pts',(0.263729325535709,2.28522445475037,8.54971094839437));
#62627=CARTESIAN_POINT('Ctrl Pts',(0.263566499350684,2.28545607621898,8.54972847901731));
#62628=CARTESIAN_POINT('Ctrl Pts',(0.262993510643645,2.28626887820114,8.54978998110197));
#62629=CARTESIAN_POINT('Ctrl Pts',(0.262581725491865,2.28684892048763,8.54983384211226));
#62630=CARTESIAN_POINT('Ctrl Pts',(0.25708056593167,2.29454377489242,8.55041538694619));
#62631=CARTESIAN_POINT('Ctrl Pts',(0.251704939767702,2.30145062169001,8.55093379330792));
#62632=CARTESIAN_POINT('Ctrl Pts',(0.230145342531506,2.32693859594889,8.55286913108312));
#62633=CARTESIAN_POINT('Ctrl Pts',(0.212131559118262,2.34386141348969,8.55420770103896));
#62634=CARTESIAN_POINT('Ctrl Pts',(0.180029914514718,2.36774381106247,8.55647793074426));
#62635=CARTESIAN_POINT('Ctrl Pts',(0.167056283744873,2.37602468103237,8.55736900477858));
#62636=CARTESIAN_POINT('Ctrl Pts',(0.152125351440082,2.38411555887143,8.55839341339151));
#62637=CARTESIAN_POINT('Ctrl Pts',(0.150702568394904,2.38487279455553,8.55849100464118));
#62638=CARTESIAN_POINT('Ctrl Pts',(0.148210306780509,2.3861753336353,8.55866193856896));
#62639=CARTESIAN_POINT('Ctrl Pts',(0.147143342073657,2.38672539727,8.55873511254563));
#62640=CARTESIAN_POINT('Ctrl Pts',(0.145591531290294,2.38751447581604,8.55884154025076));
#62641=CARTESIAN_POINT('Ctrl Pts',(0.14510910903397,2.38775825662693,8.55887462648465));
#62642=CARTESIAN_POINT('Ctrl Pts',(0.144269583262879,2.38817984334013,8.55893220560762));
#62643=CARTESIAN_POINT('Ctrl Pts',(0.143912757636174,2.38835820250103,8.55895667905511));
#62644=CARTESIAN_POINT('Ctrl Pts',(0.14322512742581,2.38870031996441,8.5590038425264));
#62645=CARTESIAN_POINT('Ctrl Pts',(0.142894370653338,2.38886417345791,8.559026529176));
#62646=CARTESIAN_POINT('Ctrl Pts',(0.14211311447227,2.3892495295305,8.5590801173357));
#62647=CARTESIAN_POINT('Ctrl Pts',(0.141662378548815,2.38947054796294,8.55911103568034));
#62648=CARTESIAN_POINT('Ctrl Pts',(0.140094794417585,2.39023467491219,8.55921857042302));
#62649=CARTESIAN_POINT('Ctrl Pts',(0.138975335402668,2.39077237493402,8.55929537467757));
#62650=CARTESIAN_POINT('Ctrl Pts',(0.124578655756466,2.39758527676272,8.56028330680299));
#62651=CARTESIAN_POINT('Ctrl Pts',(0.110892653860461,2.40295139470231,8.56122587143526));
#62652=CARTESIAN_POINT('Ctrl Pts',(0.0873168228179365,2.41038315704674,
8.56285578520356));
#62653=CARTESIAN_POINT('Ctrl Pts',(0.0776082624895371,2.41295186130109,
8.56352835861894));
#62654=CARTESIAN_POINT('Ctrl Pts',(0.0502986055330913,2.41882843156283,
8.56541342118114));
#62655=CARTESIAN_POINT('Ctrl Pts',(0.0325172825177378,2.42112955149173,
8.56663444467349));
#62656=CARTESIAN_POINT('Ctrl Pts',(0.00985150512526624,2.42216000060252,
8.56812708619422));
#62657=CARTESIAN_POINT('Ctrl Pts',(0.00506208514787253,2.42227084650992,
8.568438765919));
#62658=CARTESIAN_POINT('Ctrl Pts',(-0.00291035897192122,2.42227756838619,
8.56894953175527));
#62659=CARTESIAN_POINT('Ctrl Pts',(-0.00609245613933498,2.42223312234828,
8.56915126012565));
#62660=CARTESIAN_POINT('Ctrl Pts',(-0.00978682072199205,2.42212677234905,
8.56938257943543));
#62661=CARTESIAN_POINT('Ctrl Pts',(-0.0103000924292323,2.42211076888002,
8.56941465277231));
#62662=CARTESIAN_POINT('Ctrl Pts',(-0.0110808771168979,2.42208455636771,
8.56946334176545));
#62663=CARTESIAN_POINT('Ctrl Pts',(-0.0113484162099816,2.42207524080413,
8.56948000725967));
#62664=CARTESIAN_POINT('Ctrl Pts',(-0.011833819865078,2.4220577337432,8.56951021090698));
#62665=CARTESIAN_POINT('Ctrl Pts',(-0.0120516869455893,2.42204965455501,
8.56952375531863));
#62666=CARTESIAN_POINT('Ctrl Pts',(-0.0124908255963676,2.42203292368306,
8.56955103138261));
#62667=CARTESIAN_POINT('Ctrl Pts',(-0.0127120954584672,2.42202426506354,
8.5695647625837));
#62668=CARTESIAN_POINT('Ctrl Pts',(-0.0133469961452603,2.42199876504766,
8.56960412691129));
#62669=CARTESIAN_POINT('Ctrl Pts',(-0.0137606056074492,2.42198135464058,
8.56962972802481));
#62670=CARTESIAN_POINT('Ctrl Pts',(-0.0155607395557798,2.4219021051102,
8.56974096791646));
#62671=CARTESIAN_POINT('Ctrl Pts',(-0.0169469165689319,2.42183210540889,
8.5698261553968));
#62672=CARTESIAN_POINT('Ctrl Pts',(-0.0524099184088968,2.41981151914836,
8.57199443971786));
#62673=CARTESIAN_POINT('Ctrl Pts',(-0.0859689423470034,2.41246843317864,
8.57380206380365));
#62674=CARTESIAN_POINT('Ctrl Pts',(-0.132068625013949,2.39437308028247,
8.57662533821058));
#62675=CARTESIAN_POINT('Ctrl Pts',(-0.145960146760766,2.38773802158973,
8.57752310117291));
#62676=CARTESIAN_POINT('Ctrl Pts',(-0.160380612686434,2.37953660299457,
8.57853144882258));
#62677=CARTESIAN_POINT('Ctrl Pts',(-0.161433863959101,2.37892967006633,
8.57860554856585));
#62678=CARTESIAN_POINT('Ctrl Pts',(-0.162948572271037,2.37804537084887,
8.57871277616127));
#62679=CARTESIAN_POINT('Ctrl Pts',(-0.163412816373294,2.377772779255,8.57874573081852));
#62680=CARTESIAN_POINT('Ctrl Pts',(-0.164219549077923,2.3772963652254,8.57880315568855));
#62681=CARTESIAN_POINT('Ctrl Pts',(-0.1645623476377,2.37709306776647,8.57882760675657));
#62682=CARTESIAN_POINT('Ctrl Pts',(-0.16522235657758,2.37669999123729,8.57887478055871));
#62683=CARTESIAN_POINT('Ctrl Pts',(-0.165539619479028,2.37651030115483,
8.57889750001862));
#62684=CARTESIAN_POINT('Ctrl Pts',(-0.16628874485693,2.3760606510241,8.5789512482236));
#62685=CARTESIAN_POINT('Ctrl Pts',(-0.166720324219239,2.37580022334575,
8.57898229404809));
#62686=CARTESIAN_POINT('Ctrl Pts',(-0.16822326760528,2.37488848627861,8.57909069266373));
#62687=CARTESIAN_POINT('Ctrl Pts',(-0.169291429875897,2.37423194444059,
8.57916823733298));
#62688=CARTESIAN_POINT('Ctrl Pts',(-0.183502144444412,2.36538271508641,
8.58020671063603));
#62689=CARTESIAN_POINT('Ctrl Pts',(-0.196039317029163,2.35626057063135,
8.58120271100038));
#62690=CARTESIAN_POINT('Ctrl Pts',(-0.214319834075695,2.34083065204934,
8.5827841754068));
#62691=CARTESIAN_POINT('Ctrl Pts',(-0.220552173325257,2.33513638651739,
8.583349340232));
#62692=CARTESIAN_POINT('Ctrl Pts',(-0.237526636305793,2.31835823567996,
8.58495827450552));
#62693=CARTESIAN_POINT('Ctrl Pts',(-0.24770669807064,2.30673806021719,8.58600952560816));
#62694=CARTESIAN_POINT('Ctrl Pts',(-0.261760270500657,2.28816107837605,
8.58756139889997));
#62695=CARTESIAN_POINT('Ctrl Pts',(-0.266274420518883,2.28171676650787,
8.58807855988608));
#62696=CARTESIAN_POINT('Ctrl Pts',(-0.272364802746784,2.27230717533677,
8.5887974610413));
#62697=CARTESIAN_POINT('Ctrl Pts',(-0.274137369081325,2.26947286949933,
8.58900951590757));
#62698=CARTESIAN_POINT('Ctrl Pts',(-0.276134441350277,2.26616623105738,
8.58925131015467));
#62699=CARTESIAN_POINT('Ctrl Pts',(-0.27640220731496,2.26572044485839,8.58928379160596));
#62700=CARTESIAN_POINT('Ctrl Pts',(-0.276806881088675,2.26504302046026,
8.58933297262597));
#62701=CARTESIAN_POINT('Ctrl Pts',(-0.276944578130796,2.26481185838983,
8.5893497235749));
#62702=CARTESIAN_POINT('Ctrl Pts',(-0.277182647517975,2.26441105313428,
8.58937871279436));
#62703=CARTESIAN_POINT('Ctrl Pts',(-0.277283153530108,2.26424149063785,
8.58939095984863));
#62704=CARTESIAN_POINT('Ctrl Pts',(-0.277492962631956,2.26388678268848,
8.58941654395893));
#62705=CARTESIAN_POINT('Ctrl Pts',(-0.277602235675585,2.26370162063583,
8.58942987902521));
#62706=CARTESIAN_POINT('Ctrl Pts',(-0.277905164528154,2.26318713524465,
8.58946687585156));
#62707=CARTESIAN_POINT('Ctrl Pts',(-0.278098420969849,2.26285757531793,
8.58949051148097));
#62708=CARTESIAN_POINT('Ctrl Pts',(-0.278862705856799,2.26154891399755,
8.58958412001901));
#62709=CARTESIAN_POINT('Ctrl Pts',(-0.27942916214763,2.26056713163912,8.58965379935056));
#62710=CARTESIAN_POINT('Ctrl Pts',(-0.289476872674266,2.24293822336309,
8.5908955656493));
#62711=CARTESIAN_POINT('Ctrl Pts',(-0.297461900549118,2.22547848241258,
8.59197703886323));
#62712=CARTESIAN_POINT('Ctrl Pts',(-0.309366087925198,2.19180315291237,
8.59397741497382));
#62713=CARTESIAN_POINT('Ctrl Pts',(-0.313672408857621,2.1757943992234,8.59489570014111));
#62714=CARTESIAN_POINT('Ctrl Pts',(-0.318525031848314,2.14997442214091,
8.59639978979804));
#62715=CARTESIAN_POINT('Ctrl Pts',(-0.319887082928467,2.14034684959598,
8.59696521339813));
#62716=CARTESIAN_POINT('Ctrl Pts',(-0.321275281259053,2.12582755222279,
8.59783389740767));
#62717=CARTESIAN_POINT('Ctrl Pts',(-0.321628702471114,2.12097242586813,
8.59812699352486));
#62718=CARTESIAN_POINT('Ctrl Pts',(-0.32191611057508,2.11523059574938,8.5984773035488));
#62719=CARTESIAN_POINT('Ctrl Pts',(-0.321956581193793,2.1143496723443,8.59853115066144));
#62720=CARTESIAN_POINT('Ctrl Pts',(-0.322013178468303,2.11299660299506,
8.59861401810306));
#62721=CARTESIAN_POINT('Ctrl Pts',(-0.322031883638001,2.1125245644011,8.59864295755724));
#62722=CARTESIAN_POINT('Ctrl Pts',(-0.322062743976273,2.1116999580824,8.59869356485156));
#62723=CARTESIAN_POINT('Ctrl Pts',(-0.322075358291699,2.11134740747459,
8.59871521826279));
#62724=CARTESIAN_POINT('Ctrl Pts',(-0.322102485784134,2.110552723335,8.59876406553171));
#62725=CARTESIAN_POINT('Ctrl Pts',(-0.322116667512639,2.11011057988189,
8.59879126973305));
#62726=CARTESIAN_POINT('Ctrl Pts',(-0.322152289030624,2.10892375009722,
8.59886436546013));
#62727=CARTESIAN_POINT('Ctrl Pts',(-0.322172056930501,2.10817901960742,
8.59891030928292));
#62728=CARTESIAN_POINT('Ctrl Pts',(-0.322247036446666,2.10492951209401,
8.59911111672114));
#62729=CARTESIAN_POINT('Ctrl Pts',(-0.322275619572637,2.10242426216178,
8.59926681202063));
#62730=CARTESIAN_POINT('Ctrl Pts',(-0.322272832832555,2.09133812609189,
8.5999598458512));
#62731=CARTESIAN_POINT('Ctrl Pts',(-0.321927971084576,2.08276149861095,
8.60050688914823));
#62732=CARTESIAN_POINT('Ctrl Pts',(-0.320084275941854,2.0597968364723,8.60200185316021));
#62733=CARTESIAN_POINT('Ctrl Pts',(-0.317958670844613,2.04547987579012,
8.60296663528113));
#62734=CARTESIAN_POINT('Ctrl Pts',(-0.309606539234907,2.00716788135307,
8.6056126165525));
#62735=CARTESIAN_POINT('Ctrl Pts',(-0.301563889964951,1.98366667577301,
8.60731034970665));
#62736=CARTESIAN_POINT('Ctrl Pts',(-0.290333431154184,1.96010909948202,
8.60895852370223));
#62737=CARTESIAN_POINT('Ctrl Pts',(-0.289750221951268,1.9589050875445,8.60904258535201));
#62738=CARTESIAN_POINT('Ctrl Pts',(-0.288979344626559,1.9573385808161,8.6091516921087));
#62739=CARTESIAN_POINT('Ctrl Pts',(-0.288798472480428,1.9569727842622,8.60917715088927));
#62740=CARTESIAN_POINT('Ctrl Pts',(-0.288518907869344,1.95641008414183,
8.60921628361089));
#62741=CARTESIAN_POINT('Ctrl Pts',(-0.288420708355805,1.95621293825068,
8.60922998831388));
#62742=CARTESIAN_POINT('Ctrl Pts',(-0.288224852827786,1.95582074553898,
8.60925724018274));
#62743=CARTESIAN_POINT('Ctrl Pts',(-0.288127201545608,1.95562569849688,
8.60927078743857));
#62744=CARTESIAN_POINT('Ctrl Pts',(-0.287908367010099,1.95518970834806,
8.60930105693745));
#62745=CARTESIAN_POINT('Ctrl Pts',(-0.287787079593905,1.95494881874721,
8.60931777248146));
#62746=CARTESIAN_POINT('Ctrl Pts',(-0.287429679258594,1.95424119685872,
8.60936685022283));
#62747=CARTESIAN_POINT('Ctrl Pts',(-0.287192730872771,1.95377488398083,
8.60939916004662));
#62748=CARTESIAN_POINT('Ctrl Pts',(-0.285397468414168,1.95026301606031,
8.60964226594377));
#62749=CARTESIAN_POINT('Ctrl Pts',(-0.283791809350712,1.94724172505508,
8.60985014027847));
#62750=CARTESIAN_POINT('Ctrl Pts',(-0.278135424112408,1.93699552183511,
8.61055269420806));
#62751=CARTESIAN_POINT('Ctrl Pts',(-0.27385421177145,1.92990100805802,8.611034998999));
#62752=CARTESIAN_POINT('Ctrl Pts',(-0.25471416661972,1.90078307138899,8.61303023353306));
#62753=CARTESIAN_POINT('Ctrl Pts',(-0.237436334732314,1.88047597171762,
8.61446972800151));
#62754=CARTESIAN_POINT('Ctrl Pts',(-0.214697841373923,1.85961604274329,
8.61624665156091));
#62755=CARTESIAN_POINT('Ctrl Pts',(-0.211476390761636,1.85677717202346,
8.61649580996712));
#62756=CARTESIAN_POINT('Ctrl Pts',(-0.206808855092645,1.85282679924358,
8.61685398235208));
#62757=CARTESIAN_POINT('Ctrl Pts',(-0.205408501234214,1.85166184111768,
8.61696108820524));
#62758=CARTESIAN_POINT('Ctrl Pts',(-0.198919788094088,1.84635629507863,
8.61745593192391));
#62759=CARTESIAN_POINT('Ctrl Pts',(-0.193715907030422,1.84236003959812,
8.61784879210187));
#62760=CARTESIAN_POINT('Ctrl Pts',(-0.187553576607034,1.83792004188325,
8.61831104705655));
#62761=CARTESIAN_POINT('Ctrl Pts',(-0.186710269714065,1.83731858899306,
8.61837424250285));
#62762=CARTESIAN_POINT('Ctrl Pts',(-0.185452170570876,1.83643042229541,
8.6184684332785));
#62763=CARTESIAN_POINT('Ctrl Pts',(-0.185039575543705,1.83614059550802,
8.61849930922907));
#62764=CARTESIAN_POINT('Ctrl Pts',(-0.184303817899745,1.8356263380448,8.61855434442802));
#62765=CARTESIAN_POINT('Ctrl Pts',(-0.183980920540885,1.83540152815487,
8.61857848913262));
#62766=CARTESIAN_POINT('Ctrl Pts',(-0.183300636776477,1.83492974345595,
8.61862934054027));
#62767=CARTESIAN_POINT('Ctrl Pts',(-0.182943161302258,1.8346828990118,8.61865605214097));
#62768=CARTESIAN_POINT('Ctrl Pts',(-0.182000570671358,1.83403483077372,
8.61872646014563));
#62769=CARTESIAN_POINT('Ctrl Pts',(-0.181414630216673,1.83363481665813,
8.61877020233591));
#62770=CARTESIAN_POINT('Ctrl Pts',(-0.178784421993921,1.83185191124407,
8.61896644638034));
#62771=CARTESIAN_POINT('Ctrl Pts',(-0.176725673175903,1.83049062549386,
8.61911976052625));
#62772=CARTESIAN_POINT('Ctrl Pts',(-0.161515276034905,1.82068242857172,
8.62025060656303));
#62773=CARTESIAN_POINT('Ctrl Pts',(-0.14778219989945,1.81317987803289,8.62126304009206));
#62774=CARTESIAN_POINT('Ctrl Pts',(-0.117525313290562,1.79940153180281,
8.62347199148681));
#62775=CARTESIAN_POINT('Ctrl Pts',(-0.100918428102868,1.79342693035838,
8.6246722434427));
#62776=CARTESIAN_POINT('Ctrl Pts',(-0.069244537682779,1.78488570633752,
8.62688240334311));
#62777=CARTESIAN_POINT('Ctrl Pts',(-0.0543179440716717,1.78197247164592,
8.62789235741758));
#62778=CARTESIAN_POINT('Ctrl Pts',(-0.0383355576014893,1.78001188994944,
8.62890502288658));
#62779=CARTESIAN_POINT('Ctrl Pts',(-0.0374308540527212,1.77990480046906,
8.62896211252217));
#62780=CARTESIAN_POINT('Ctrl Pts',(-0.0362135146670193,1.77976593606299,
8.62903860537103));
#62781=CARTESIAN_POINT('Ctrl Pts',(-0.0359012800986873,1.7797307813113,
8.6290581962319));
#62782=CARTESIAN_POINT('Ctrl Pts',(-0.0353755134088078,1.77967236333363,
8.62909113601298));
#62783=CARTESIAN_POINT('Ctrl Pts',(-0.0351620094043913,1.77964885694529,
8.62910449865661));
#62784=CARTESIAN_POINT('Ctrl Pts',(-0.0347524850985844,1.77960418342912,
8.62913010342618));
#62785=CARTESIAN_POINT('Ctrl Pts',(-0.0345564703069038,1.77958298288507,
8.62914234733483));
#62786=CARTESIAN_POINT('Ctrl Pts',(-0.0340924879393328,1.77953323025312,
8.62917130239016));
#62787=CARTESIAN_POINT('Ctrl Pts',(-0.033824504243271,1.77950483442045,
8.6291880045822));
#62788=CARTESIAN_POINT('Ctrl Pts',(-0.0330373039361792,1.77942242019123,
8.6292370049441));
#62789=CARTESIAN_POINT('Ctrl Pts',(-0.032517988192475,1.77936932682542,
8.62926925099118));
#62790=CARTESIAN_POINT('Ctrl Pts',(-0.0286213198927139,1.77898050704224,
8.62951062744522));
#62791=CARTESIAN_POINT('Ctrl Pts',(-0.0252388215946294,1.77869687376856,
8.62971688288239));
#62792=CARTESIAN_POINT('Ctrl Pts',(-0.0137246983724219,1.77791434134935,
8.63040978726543));
#62793=CARTESIAN_POINT('Ctrl Pts',(-0.00557838692804692,1.77767029018376,
8.63088448994781));
#62794=CARTESIAN_POINT('Ctrl Pts',(0.0304526758666886,1.77795752248239,
8.63294912131454));
#62795=CARTESIAN_POINT('Ctrl Pts',(0.058189563717908,1.78179749128044,8.63445652636926));
#62796=CARTESIAN_POINT('Ctrl Pts',(0.0888553993195147,1.79019174012449,
8.63629530784051));
#62797=CARTESIAN_POINT('Ctrl Pts',(0.0926045416386487,1.79129166338582,
8.63652293621822));
#62798=CARTESIAN_POINT('Ctrl Pts',(0.103536562859958,1.79471596206472,8.6371961567505));
#62799=CARTESIAN_POINT('Ctrl Pts',(0.110658458306603,1.79722474455812,8.63764694817855));
#62800=CARTESIAN_POINT('Ctrl Pts',(0.118589066858118,1.80033560220971,8.63816525394164));
#62801=CARTESIAN_POINT('Ctrl Pts',(0.11949121150046,1.80069418912565,8.63822445485515));
#62802=CARTESIAN_POINT('Ctrl Pts',(0.120853888431524,1.80124297242638,8.63831424756699));
#62803=CARTESIAN_POINT('Ctrl Pts',(0.121315628032383,1.80143017187875,8.63834473821528));
#62804=CARTESIAN_POINT('Ctrl Pts',(0.12211779530301,1.80175755627689,8.63839782195723));
#62805=CARTESIAN_POINT('Ctrl Pts',(0.122458421218158,1.80189725556692,8.63842039858915));
#62806=CARTESIAN_POINT('Ctrl Pts',(0.123168289842822,1.80218981261848,8.6384675231486));
#62807=CARTESIAN_POINT('Ctrl Pts',(0.123537488934966,1.80234277405643,8.63849207456093));
#62808=CARTESIAN_POINT('Ctrl Pts',(0.124409139833329,1.80270580540699,8.63855013874764));
#62809=CARTESIAN_POINT('Ctrl Pts',(0.124911344365616,1.80291646249625,8.63858367141864));
#62810=CARTESIAN_POINT('Ctrl Pts',(0.126564815856991,1.80361496929238,8.6386943368392));
#62811=CARTESIAN_POINT('Ctrl Pts',(0.127713766876184,1.8041082415475,8.63877165398284));
#62812=CARTESIAN_POINT('Ctrl Pts',(0.15405447441484,1.81559894048176,8.64055398776295));
#62813=CARTESIAN_POINT('Ctrl Pts',(0.17773372852645,1.82976529809131,8.64237719618967));
#62814=CARTESIAN_POINT('Ctrl Pts',(0.214126927098644,1.85841000209708,8.64550986373934));
#62815=CARTESIAN_POINT('Ctrl Pts',(0.227881152534135,1.87133789495012,8.64679049860684));
#62816=CARTESIAN_POINT('Ctrl Pts',(0.240840237491832,1.88585626532937,8.6480463317393));
#62817=CARTESIAN_POINT('Ctrl Pts',(0.241251271381388,1.8863194366283,8.6480862179897));
#62818=CARTESIAN_POINT('Ctrl Pts',(0.244046633668339,1.88948772282619,8.64835782922808));
#62819=CARTESIAN_POINT('Ctrl Pts',(0.246386873265539,1.89223164430725,8.64858697783846));
#62820=CARTESIAN_POINT('Ctrl Pts',(0.249047026945283,1.89545884099768,8.64884895068513));
#62821=CARTESIAN_POINT('Ctrl Pts',(0.249412182966242,1.8959042617875,8.64888494497765));
#62822=CARTESIAN_POINT('Ctrl Pts',(0.249953391924104,1.89656805519794,8.64893834025456));
#62823=CARTESIAN_POINT('Ctrl Pts',(0.250130354511707,1.8967856795066,8.64895580677819));
#62824=CARTESIAN_POINT('Ctrl Pts',(0.25044502724324,1.89717369019531,8.64898687853296));
#62825=CARTESIAN_POINT('Ctrl Pts',(0.250582847683207,1.89734398585804,8.64900049178701));
#62826=CARTESIAN_POINT('Ctrl Pts',(0.250871941356647,1.8977019457203,8.64902905632544));
#62827=CARTESIAN_POINT('Ctrl Pts',(0.251023177262946,1.89788963855572,8.64904400489544));
#62828=CARTESIAN_POINT('Ctrl Pts',(0.251425015297271,1.89838949047335,8.64908373851545));
#62829=CARTESIAN_POINT('Ctrl Pts',(0.251675247648462,1.89870194836009,8.64910849682829));
#62830=CARTESIAN_POINT('Ctrl Pts',(0.252224391398879,1.89939027284592,8.64916286584248));
#62831=CARTESIAN_POINT('Ctrl Pts',(0.252523046814001,1.89976634378787,8.6491924584077));
#62832=CARTESIAN_POINT('Ctrl Pts',(0.253408836917653,1.9008868765289,8.64928030299234));
#62833=CARTESIAN_POINT('Ctrl Pts',(0.253993534290668,1.90163327104521,8.64933838677612));
#62834=CARTESIAN_POINT('Ctrl Pts',(0.2605633465122,1.91009662769758,8.64999229315507));
#62835=CARTESIAN_POINT('Ctrl Pts',(0.266198664745275,1.91808007293643,8.65056514777496));
#62836=CARTESIAN_POINT('Ctrl Pts',(0.282950778912228,1.9442619425724,8.65235047111826));
#62837=CARTESIAN_POINT('Ctrl Pts',(0.292629374975802,1.9633119269917,8.65351706044498));
#62838=CARTESIAN_POINT('Ctrl Pts',(0.306963177572893,2.00016529081372,8.65575257943072));
#62839=CARTESIAN_POINT('Ctrl Pts',(0.312116087044209,2.01767890847305,8.65680681817659));
#62840=CARTESIAN_POINT('Ctrl Pts',(0.316018236103701,2.03679160313739,8.65799171126637));
#62841=CARTESIAN_POINT('Ctrl Pts',(0.316267760267555,2.03805219354455,8.65807000482565));
#62842=CARTESIAN_POINT('Ctrl Pts',(0.316605661235126,2.03981453327043,8.65817967187188));
#62843=CARTESIAN_POINT('Ctrl Pts',(0.31670040000447,2.04031506250406,8.6582108425084));
#62844=CARTESIAN_POINT('Ctrl Pts',(0.316862089280427,2.04118053327133,8.65826478164746));
#62845=CARTESIAN_POINT('Ctrl Pts',(0.316929597235285,2.04154537072383,8.65828753235682));
#62846=CARTESIAN_POINT('Ctrl Pts',(0.317068149534322,2.04230145325715,8.65833470731456));
#62847=CARTESIAN_POINT('Ctrl Pts',(0.31713910007669,2.0426927147241,8.65835913450717));
#62848=CARTESIAN_POINT('Ctrl Pts',(0.31730345047005,2.04360868868258,8.65841635570135));
#62849=CARTESIAN_POINT('Ctrl Pts',(0.317396272992565,2.04413350237142,8.6584491680037));
#62850=CARTESIAN_POINT('Ctrl Pts',(0.317691461446308,2.04582696569904,8.6585551349574));
#62851=CARTESIAN_POINT('Ctrl Pts',(0.317888676225886,2.0469964926789,8.65862845302382));
#62852=CARTESIAN_POINT('Ctrl Pts',(0.320697573345813,2.06423365017761,8.65971112310684));
#62853=CARTESIAN_POINT('Ctrl Pts',(0.322094251481028,2.0804728499953,8.66075938610701));
#62854=CARTESIAN_POINT('Ctrl Pts',(0.322511813901921,2.12182534544475,8.66349881246203));
#62855=CARTESIAN_POINT('Ctrl Pts',(0.319836704247099,2.14684613788721,8.66522659305696));
#62856=CARTESIAN_POINT('Ctrl Pts',(0.312287975047061,2.18011950945565,8.6674845439894));
#62857=CARTESIAN_POINT('Ctrl Pts',(0.30991731349674,2.18884936263284,8.66807203137488));
#62858=CARTESIAN_POINT('Ctrl Pts',(0.306965664652279,2.19815176891556,8.66868449319783));
#62859=CARTESIAN_POINT('Ctrl Pts',(0.30674668291707,2.19883401013424,8.66872933095073));
#62860=CARTESIAN_POINT('Ctrl Pts',(0.306437725610052,2.19978565332511,8.66879175617843));
#62861=CARTESIAN_POINT('Ctrl Pts',(0.306349668556235,2.20005566882286,8.66880945518048));
#62862=CARTESIAN_POINT('Ctrl Pts',(0.306196949718405,2.20052186964667,8.66883999036363));
#62863=CARTESIAN_POINT('Ctrl Pts',(0.306132456239882,2.20071810925153,8.66885283648184));
#62864=CARTESIAN_POINT('Ctrl Pts',(0.30599800742989,2.2011258854847,8.66887951497889));
#62865=CARTESIAN_POINT('Ctrl Pts',(0.305928021496317,2.20133741130375,8.66889334543396));
#62866=CARTESIAN_POINT('Ctrl Pts',(0.305763475409961,2.2018330121822,8.66892573036467));
#62867=CARTESIAN_POINT('Ctrl Pts',(0.305668738334773,2.20211702929209,8.66894427433671));
#62868=CARTESIAN_POINT('Ctrl Pts',(0.305367427793272,2.2030161672356,8.66900293410981));
#62869=CARTESIAN_POINT('Ctrl Pts',(0.305159390649157,2.20363080133284,8.66904296384211));
#62870=CARTESIAN_POINT('Ctrl Pts',(0.304661907110309,2.20508610021847,8.66913758977227));
#62871=CARTESIAN_POINT('Ctrl Pts',(0.304370833728097,2.20592620885011,8.66919209259535));
#62872=CARTESIAN_POINT('Ctrl Pts',(0.303349863577725,2.20883402020328,8.66938034964859));
#62873=CARTESIAN_POINT('Ctrl Pts',(0.302602325483185,2.21089552237283,8.6695131300002));
#62874=CARTESIAN_POINT('Ctrl Pts',(0.29915461053368,2.2201088320558,8.67010414988252));
#62875=CARTESIAN_POINT('Ctrl Pts',(0.296221335244625,2.2271713457132,8.6705506811821));
#62876=CARTESIAN_POINT('Ctrl Pts',(0.286376291092042,2.24868129121374,8.67190966754929));
#62877=CARTESIAN_POINT('Ctrl Pts',(0.278637263801769,2.26272318402109,8.67279629043257));
#62878=CARTESIAN_POINT('Ctrl Pts',(0.261703453147865,2.28867074440385,8.67453133740211));
#62879=CARTESIAN_POINT('Ctrl Pts',(0.252657347459537,2.30062292434542,8.67537647152513));
#62880=CARTESIAN_POINT('Ctrl Pts',(0.241070603887207,2.31389990449348,8.67640600982071));
#62881=CARTESIAN_POINT('Ctrl Pts',(0.239302748722093,2.31587588819111,8.67656176004499));
#62882=CARTESIAN_POINT('Ctrl Pts',(0.233214445075489,2.32251427090134,8.67709407076778));
#62883=CARTESIAN_POINT('Ctrl Pts',(0.228780742600018,2.32707034475708,8.67747494837282));
#62884=CARTESIAN_POINT('Ctrl Pts',(0.22347829058257,2.33220612063115,8.67792424948242));
#62885=CARTESIAN_POINT('Ctrl Pts',(0.222737727214367,2.33291658089851,8.67798686443318));
#62886=CARTESIAN_POINT('Ctrl Pts',(0.221629654358644,2.33396949427333,8.67808035602638));
#62887=CARTESIAN_POINT('Ctrl Pts',(0.221264712195126,2.334314649722,8.67811111588517));
#62888=CARTESIAN_POINT('Ctrl Pts',(0.220612650659917,2.33492847553018,8.67816602094904));
#62889=CARTESIAN_POINT('Ctrl Pts',(0.220325843080183,2.33519747684651,8.67819015186363));
#62890=CARTESIAN_POINT('Ctrl Pts',(0.219720387990236,2.33576326334799,8.67824105315812));
#62891=CARTESIAN_POINT('Ctrl Pts',(0.219401630071303,2.33605992875151,8.67826782859273));
#62892=CARTESIAN_POINT('Ctrl Pts',(0.218558577354822,2.33684136839186,8.67833858472978));
#62893=CARTESIAN_POINT('Ctrl Pts',(0.218033273119016,2.337325045701,8.67838261204206));
#62894=CARTESIAN_POINT('Ctrl Pts',(0.21565209318303,2.33950295411902,8.67858191720156));
#62895=CARTESIAN_POINT('Ctrl Pts',(0.213778088120343,2.34117715229746,8.6787380387998));
#62896=CARTESIAN_POINT('Ctrl Pts',(0.205483993376011,2.34841430456749,8.67942599987128));
#62897=CARTESIAN_POINT('Ctrl Pts',(0.198865464501719,2.35374365721168,8.67996732857903));
#62898=CARTESIAN_POINT('Ctrl Pts',(0.180749550684643,2.36718645791379,8.68143036422119));
#62899=CARTESIAN_POINT('Ctrl Pts',(0.168919020419637,2.37481865881849,8.68236773658319));
#62900=CARTESIAN_POINT('Ctrl Pts',(0.143747347497387,2.38881677584888,8.68430995647952));
#62901=CARTESIAN_POINT('Ctrl Pts',(0.130389340437173,2.39508822395324,8.68531364011999));
#62902=CARTESIAN_POINT('Ctrl Pts',(0.113602003427085,2.40160643804579,8.68651514136518));
#62903=CARTESIAN_POINT('Ctrl Pts',(0.110537226817099,2.40274309450574,8.68673210350815));
#62904=CARTESIAN_POINT('Ctrl Pts',(0.106243873291195,2.40426151084052,8.68703227399758));
#62905=CARTESIAN_POINT('Ctrl Pts',(0.105029566409871,2.40468281516359,8.68711675661527));
#62906=CARTESIAN_POINT('Ctrl Pts',(0.102283052369747,2.40561734855506,8.68730685540025));
#62907=CARTESIAN_POINT('Ctrl Pts',(0.100749428044346,2.40612634560497,8.68741231727358));
#62908=CARTESIAN_POINT('Ctrl Pts',(0.0987757888328263,2.40676494157526,
8.68754710284833));
#62909=CARTESIAN_POINT('Ctrl Pts',(0.0983392610149304,2.40690515731545,
8.68757685613368));
#62910=CARTESIAN_POINT('Ctrl Pts',(0.0932633386534025,2.40852363686374,
8.68792213532385));
#62911=CARTESIAN_POINT('Ctrl Pts',(0.0885909960822404,2.4098976067008,8.68823327129162));
#62912=CARTESIAN_POINT('Ctrl Pts',(0.0833431179823502,2.41131241537206,
8.68857395002852));
#62913=CARTESIAN_POINT('Ctrl Pts',(0.082796836798722,2.41145814984909,8.68860930772208));
#62914=CARTESIAN_POINT('Ctrl Pts',(0.0819759555784916,2.41167482857076,
8.68866227748653));
#62915=CARTESIAN_POINT('Ctrl Pts',(0.0817016443932521,2.41174684819992,
8.68867995122046));
#62916=CARTESIAN_POINT('Ctrl Pts',(0.0812274762474998,2.41187067087675,
8.6887104545704));
#62917=CARTESIAN_POINT('Ctrl Pts',(0.0810276645329549,2.41192264398651,
8.6887232940753));
#62918=CARTESIAN_POINT('Ctrl Pts',(0.0806120469780002,2.41203032413868,
8.68874997063392));
#62919=CARTESIAN_POINT('Ctrl Pts',(0.0803962335592368,2.41208599925314,
8.6887638057443));
#62920=CARTESIAN_POINT('Ctrl Pts',(0.0799666240730491,2.41219635385069,
8.68879131320454));
#62921=CARTESIAN_POINT('Ctrl Pts',(0.0797528289626704,2.41225103778283,
8.68880498582793));
#62922=CARTESIAN_POINT('Ctrl Pts',(0.0790194524669056,2.41243781648468,
8.68885183081006));
#62923=CARTESIAN_POINT('Ctrl Pts',(0.0784995940727626,2.41256883526366,
8.68888494097346));
#62924=CARTESIAN_POINT('Ctrl Pts',(0.0742492066112446,2.41362877840991,
8.68915488393508));
#62925=CARTESIAN_POINT('Ctrl Pts',(0.0705024576010375,2.4144922288318,8.68938801496147));
#62926=CARTESIAN_POINT('Ctrl Pts',(0.062545550252067,2.41617656444665,8.68987467350211));
#62927=CARTESIAN_POINT('Ctrl Pts',(0.0583326376750847,2.41698087099498,
8.69012740128338));
#62928=CARTESIAN_POINT('Ctrl Pts',(0.0408897968480715,2.41995140192052,
8.69115808501131));
#62929=CARTESIAN_POINT('Ctrl Pts',(0.0275463330329515,2.42137536593075,
8.69190989759375));
#62930=CARTESIAN_POINT('Ctrl Pts',(-0.00920744555482762,2.42299090349877,
8.69396745206395));
#62931=CARTESIAN_POINT('Ctrl Pts',(-0.0326067896022078,2.42147249786692,
8.69526791844942));
#62932=CARTESIAN_POINT('Ctrl Pts',(-0.0560014621145417,2.41737225806352,
8.69667375113669));
#62933=CARTESIAN_POINT('Ctrl Pts',(-0.0563676828391008,2.41730741919634,
8.69669578307073));
#62934=CARTESIAN_POINT('Ctrl Pts',(-0.0623288190750037,2.41624136266905,
8.69705481836407));
#62935=CARTESIAN_POINT('Ctrl Pts',(-0.0678961103403432,2.41509299138242,
8.69739606797671));
#62936=CARTESIAN_POINT('Ctrl Pts',(-0.0743837459729702,2.4135748613147,
8.69780171258002));
#62937=CARTESIAN_POINT('Ctrl Pts',(-0.0753365840236626,2.41334730633582,
8.69786149228186));
#62938=CARTESIAN_POINT('Ctrl Pts',(-0.0767737800217712,2.41299714366867,
8.69795197142869));
#62939=CARTESIAN_POINT('Ctrl Pts',(-0.0772589206176465,2.41287774677042,
8.6979825673312));
#62940=CARTESIAN_POINT('Ctrl Pts',(-0.078125080418771,2.41266244067464,
8.6980372893661));
#62941=CARTESIAN_POINT('Ctrl Pts',(-0.0785062063791439,2.41256696171676,
8.69806140156535));
#62942=CARTESIAN_POINT('Ctrl Pts',(-0.0793108163144453,2.41236382788214,
8.69811237700117));
#62943=CARTESIAN_POINT('Ctrl Pts',(-0.0797342575422867,2.41225600830862,
8.69813924551946));
#62944=CARTESIAN_POINT('Ctrl Pts',(-0.0808556030816881,2.41196805380572,
8.69821050929332));
#62945=CARTESIAN_POINT('Ctrl Pts',(-0.0815531216571581,2.41178643889611,
8.69825495237002));
#62946=CARTESIAN_POINT('Ctrl Pts',(-0.0847442344969672,2.41094411860663,
8.69845880627202));
#62947=CARTESIAN_POINT('Ctrl Pts',(-0.0872303931161674,2.410255842928,8.69861910877855));
#62948=CARTESIAN_POINT('Ctrl Pts',(-0.105917800988257,2.40483999626897,
8.69983555471317));
#62949=CARTESIAN_POINT('Ctrl Pts',(-0.121730933814442,2.39887693620633,
8.70093260999324));
#62950=CARTESIAN_POINT('Ctrl Pts',(-0.144336276134454,2.38826005966262,
8.70259814290849));
#62951=CARTESIAN_POINT('Ctrl Pts',(-0.151537239450821,2.38454047016076,
8.70314400401242));
#62952=CARTESIAN_POINT('Ctrl Pts',(-0.16617655690857,2.37626521959363,8.7042809203921));
#62953=CARTESIAN_POINT('Ctrl Pts',(-0.173585945467618,2.37167083299168,
8.70487183322863));
#62954=CARTESIAN_POINT('Ctrl Pts',(-0.192890183645024,2.35858820235948,
8.70644131211505));
#62955=CARTESIAN_POINT('Ctrl Pts',(-0.204411054725253,2.3495810804317,8.70741063552269));
#62956=CARTESIAN_POINT('Ctrl Pts',(-0.215959441337407,2.33921438773561,
8.70838660137789));
#62957=CARTESIAN_POINT('Ctrl Pts',(-0.216634003733595,2.33860367154802,
8.7084436235559));
#62958=CARTESIAN_POINT('Ctrl Pts',(-0.217537896780091,2.33777833735934,
8.70852003971562));
#62959=CARTESIAN_POINT('Ctrl Pts',(-0.217769505071698,2.33756623690193,
8.70853962087396));
#62960=CARTESIAN_POINT('Ctrl Pts',(-0.218158966280046,2.33720853098944,
8.7085725482492));
#62961=CARTESIAN_POINT('Ctrl Pts',(-0.218316983725192,2.33706310628248,
8.70858590816913));
#62962=CARTESIAN_POINT('Ctrl Pts',(-0.218619803192187,2.33678385956987,
8.70861151082394));
#62963=CARTESIAN_POINT('Ctrl Pts',(-0.218764626703939,2.33665006360433,
8.70862375533543));
#62964=CARTESIAN_POINT('Ctrl Pts',(-0.219063376292857,2.33637355362213,
8.70864901414304));
#62965=CARTESIAN_POINT('Ctrl Pts',(-0.219217285218453,2.33623082260119,
8.70866202701847));
#62966=CARTESIAN_POINT('Ctrl Pts',(-0.219564391655619,2.33590829403369,
8.7086913751546));
#62967=CARTESIAN_POINT('Ctrl Pts',(-0.219757508271615,2.33572840905674,
8.70870770372155));
#62968=CARTESIAN_POINT('Ctrl Pts',(-0.220657564641559,2.33488795393915,
8.70878380917562));
#62969=CARTESIAN_POINT('Ctrl Pts',(-0.221361758148437,2.33422443046147,
8.70884336210164));
#62970=CARTESIAN_POINT('Ctrl Pts',(-0.229923416863778,2.32608414215394,
8.70956768142848));
#62971=CARTESIAN_POINT('Ctrl Pts',(-0.23740253568767,2.31821757233283,8.71020326249131));
#62972=CARTESIAN_POINT('Ctrl Pts',(-0.249055292319071,2.3046512362283,8.71122819593721));
#62973=CARTESIAN_POINT('Ctrl Pts',(-0.253463360288602,2.29916575733967,
8.71162526417457));
#62974=CARTESIAN_POINT('Ctrl Pts',(-0.272792659146722,2.27342982719718,
8.71343174032465));
#62975=CARTESIAN_POINT('Ctrl Pts',(-0.285489588884242,2.25162237894765,
8.71481676172906));
#62976=CARTESIAN_POINT('Ctrl Pts',(-0.295800567586154,2.22792062984747,
8.71633809485773));
#62977=CARTESIAN_POINT('Ctrl Pts',(-0.296077069642911,2.22727934689565,
8.71637926105461));
#62978=CARTESIAN_POINT('Ctrl Pts',(-0.298928977146458,2.22060542173213,
8.71680775082826));
#62979=CARTESIAN_POINT('Ctrl Pts',(-0.301321567627375,2.21449674539301,
8.71720056617074));
#62980=CARTESIAN_POINT('Ctrl Pts',(-0.303874135358511,2.20734411176951,
8.71766277266108));
#62981=CARTESIAN_POINT('Ctrl Pts',(-0.304217563481681,2.20636692390714,
8.71772596596596));
#62982=CARTESIAN_POINT('Ctrl Pts',(-0.304721155312714,2.20491161689075,
8.71782015416331));
#62983=CARTESIAN_POINT('Ctrl Pts',(-0.304884919655724,2.20443474333623,
8.71785102968665));
#62984=CARTESIAN_POINT('Ctrl Pts',(-0.305174479942624,2.20358507237578,
8.71790606440589));
#62985=CARTESIAN_POINT('Ctrl Pts',(-0.305300713845271,2.20321242440102,
8.71793020905894));
#62986=CARTESIAN_POINT('Ctrl Pts',(-0.305564891805026,2.20242783433434,
8.71798106064633));
#62987=CARTESIAN_POINT('Ctrl Pts',(-0.30570268586448,2.20201584289972,8.71800777247888));
#62988=CARTESIAN_POINT('Ctrl Pts',(-0.306063324250148,2.20093027563092,
8.71807818174809));
#62989=CARTESIAN_POINT('Ctrl Pts',(-0.30628477712196,2.20025624309972,8.71812192497404));
#62990=CARTESIAN_POINT('Ctrl Pts',(-0.30726667673414,2.19723403322372,8.71831818005326));
#62991=CARTESIAN_POINT('Ctrl Pts',(-0.308002341522887,2.1948779474879,8.71847150431057));
#62992=CARTESIAN_POINT('Ctrl Pts',(-0.313198332671817,2.17753933768661,
8.71960247013815));
#62993=CARTESIAN_POINT('Ctrl Pts',(-0.316589686574244,2.16226062690177,
8.72061502137044));
#62994=CARTESIAN_POINT('Ctrl Pts',(-0.321146229598096,2.13121460337009,
8.72269988635691));
#62995=CARTESIAN_POINT('Ctrl Pts',(-0.322287724825793,2.11548544269752,
8.72376975591092));
#62996=CARTESIAN_POINT('Ctrl Pts',(-0.322274893015885,2.09973740411269,
8.72483344686166));
#62997=CARTESIAN_POINT('',(-0.322274962187229,2.10015611604601,8.97472265507268));
#62998=CARTESIAN_POINT('Ctrl Pts',(-0.322274892771064,2.09973710382478,
8.72483346714441));
#62999=CARTESIAN_POINT('Ctrl Pts',(-0.322260696355795,2.08233423288161,
8.72600893253744));
#63000=CARTESIAN_POINT('Ctrl Pts',(-0.320836875012741,2.06495801800556,
8.72717327402486));
#63001=CARTESIAN_POINT('Ctrl Pts',(-0.317940286355703,2.0473182359678,8.72829440674435));
#63002=CARTESIAN_POINT('Ctrl Pts',(-0.31786357071133,2.04685732063037,8.72832365698864));
#63003=CARTESIAN_POINT('Ctrl Pts',(-0.317737437134452,2.04610954261467,
8.72837103834983));
#63004=CARTESIAN_POINT('Ctrl Pts',(-0.317688632838165,2.04582257923291,
8.72838920358338));
#63005=CARTESIAN_POINT('Ctrl Pts',(-0.317602439820313,2.04531989596424,
8.72842099292514));
#63006=CARTESIAN_POINT('Ctrl Pts',(-0.317565220040452,2.04510414789333,
8.72843462657574));
#63007=CARTESIAN_POINT('Ctrl Pts',(-0.317489830078936,2.04466978519519,
8.72846205443247));
#63008=CARTESIAN_POINT('Ctrl Pts',(-0.317451653830905,2.04445117143337,
8.72847584829638));
#63009=CARTESIAN_POINT('Ctrl Pts',(-0.31737727683206,2.04402783731317,8.72850253883455));
#63010=CARTESIAN_POINT('Ctrl Pts',(-0.317341103900015,2.04382311310411,
8.72851543708006));
#63011=CARTESIAN_POINT('Ctrl Pts',(-0.317254163107915,2.04333382695032,
8.72854624169374));
#63012=CARTESIAN_POINT('Ctrl Pts',(-0.317203210348791,2.04304929742896,
8.72856413747114));
#63013=CARTESIAN_POINT('Ctrl Pts',(-0.317047606122362,2.04218706225256,
8.72861831599577));
#63014=CARTESIAN_POINT('Ctrl Pts',(-0.316941758010437,2.04160956961178,
8.72865453106242));
#63015=CARTESIAN_POINT('Ctrl Pts',(-0.315808840250748,2.03552237897722,
8.72903553860515));
#63016=CARTESIAN_POINT('Ctrl Pts',(-0.314639712590034,2.03003967012019,
8.72937244093462));
#63017=CARTESIAN_POINT('Ctrl Pts',(-0.312846623179465,2.02258940917239,
8.72982508042066));
#63018=CARTESIAN_POINT('Ctrl Pts',(-0.31234600957366,2.02059357791735,8.72994582436981));
#63019=CARTESIAN_POINT('Ctrl Pts',(-0.310762677926306,2.01452797041486,
8.73031159170614));
#63020=CARTESIAN_POINT('Ctrl Pts',(-0.30961924938343,2.01047440226361,8.73055439134698));
#63021=CARTESIAN_POINT('Ctrl Pts',(-0.306882044035726,2.00145149075179,
8.73109346529664));
#63022=CARTESIAN_POINT('Ctrl Pts',(-0.30524636004538,1.99649608629821,8.73138858059926));
#63023=CARTESIAN_POINT('Ctrl Pts',(-0.302406289795634,1.98854593456659,
8.73186352575278));
#63024=CARTESIAN_POINT('Ctrl Pts',(-0.301276016993766,1.98552583380336,
8.7320442979145));
#63025=CARTESIAN_POINT('Ctrl Pts',(-0.299068084915275,1.97988555720773,
8.73238334644627));
#63026=CARTESIAN_POINT('Ctrl Pts',(-0.298000834323777,1.9772616539135,8.73254167031454));
#63027=CARTESIAN_POINT('Ctrl Pts',(-0.294703160179138,1.96945077698144,
8.73301556488068));
#63028=CARTESIAN_POINT('Ctrl Pts',(-0.292370899332094,1.96430803774405,
8.73333105765857));
#63029=CARTESIAN_POINT('Ctrl Pts',(-0.283108752483761,1.94523347323296,
8.73452173821856));
#63030=CARTESIAN_POINT('Ctrl Pts',(-0.275308865188227,1.93174959309689,
8.73540663830876));
#63031=CARTESIAN_POINT('Ctrl Pts',(-0.263174894708821,1.91389098056518,
8.73668245830491));
#63032=CARTESIAN_POINT('Ctrl Pts',(-0.259644110619399,1.9089960186471,8.73704377447665));
#63033=CARTESIAN_POINT('Ctrl Pts',(-0.255217113772652,1.90320830901687,
8.73748656098228));
#63034=CARTESIAN_POINT('Ctrl Pts',(-0.254450274820983,1.90221779054555,
8.73756290645172));
#63035=CARTESIAN_POINT('Ctrl Pts',(-0.253341546524175,1.90080277747021,
8.73767279686496));
#63036=CARTESIAN_POINT('Ctrl Pts',(-0.253004318061632,1.90037463163403,
8.73770615633022));
#63037=CARTESIAN_POINT('Ctrl Pts',(-0.252417889532214,1.89963397385541,
8.73776405665592));
#63038=CARTESIAN_POINT('Ctrl Pts',(-0.252169190378016,1.89932106535403,
8.73778857745584));
#63039=CARTESIAN_POINT('Ctrl Pts',(-0.25169036002893,1.8987209057868,8.73783572314968));
#63040=CARTESIAN_POINT('Ctrl Pts',(-0.251460317444367,1.89843358452408,
8.73785834446517));
#63041=CARTESIAN_POINT('Ctrl Pts',(-0.250917944696875,1.89775853903116,
8.7379116118476));
#63042=CARTESIAN_POINT('Ctrl Pts',(-0.250605207932157,1.89737114406246,
8.73794227425981));
#63043=CARTESIAN_POINT('Ctrl Pts',(-0.249680926940995,1.8962316265383,8.73803274401803));
#63044=CARTESIAN_POINT('Ctrl Pts',(-0.249066889553967,1.89548154167325,
8.7380926520914));
#63045=CARTESIAN_POINT('Ctrl Pts',(-0.243666075723224,1.88894450677984,
8.73861790660274));
#63046=CARTESIAN_POINT('Ctrl Pts',(-0.238682108603656,1.88332417427561,
8.73909129644687));
#63047=CARTESIAN_POINT('Ctrl Pts',(-0.217588256326666,1.86114863221881,
8.7410529224041));
#63048=CARTESIAN_POINT('Ctrl Pts',(-0.199919201675758,1.84617601021165,
8.74260890005521));
#63049=CARTESIAN_POINT('Ctrl Pts',(-0.173816208021734,1.82848500097667,
8.74474255100959));
#63050=CARTESIAN_POINT('Ctrl Pts',(-0.166643019397468,1.82402431086632,
8.74531309350797));
#63051=CARTESIAN_POINT('Ctrl Pts',(-0.152020182018295,1.81570926057497,
8.74643595576111));
#63052=CARTESIAN_POINT('Ctrl Pts',(-0.144578284204794,1.81185333076884,
8.74698796541639));
#63053=CARTESIAN_POINT('Ctrl Pts',(-0.134927128523312,1.80732089286679,
8.74767229865384));
#63054=CARTESIAN_POINT('Ctrl Pts',(-0.132849930750197,1.80637219761226,
8.74781777440189));
#63055=CARTESIAN_POINT('Ctrl Pts',(-0.129502643317078,1.80488622223059,
8.74804910533886));
#63056=CARTESIAN_POINT('Ctrl Pts',(-0.128238923441014,1.80433489361735,
8.74813574081585));
#63057=CARTESIAN_POINT('Ctrl Pts',(-0.126702132708159,1.80367613798968,
8.74824021564959));
#63058=CARTESIAN_POINT('Ctrl Pts',(-0.126432428871207,1.80356096316298,
8.74825851799625));
#63059=CARTESIAN_POINT('Ctrl Pts',(-0.125960373451495,1.80336013715884,
8.74829049430182));
#63060=CARTESIAN_POINT('Ctrl Pts',(-0.125758091333839,1.80327432471857,
8.74830417804093));
#63061=CARTESIAN_POINT('Ctrl Pts',(-0.125350936754697,1.80310209209146,
8.74833168322957));
#63062=CARTESIAN_POINT('Ctrl Pts',(-0.125146061997697,1.80301567678846,
8.74834550438119));
#63063=CARTESIAN_POINT('Ctrl Pts',(-0.124750087023205,1.80284913873433,
8.74837218036557));
#63064=CARTESIAN_POINT('Ctrl Pts',(-0.124558999434806,1.80276898845571,
8.74838503689722));
#63065=CARTESIAN_POINT('Ctrl Pts',(-0.124103536938228,1.80257846443069,
8.74841564149292));
#63066=CARTESIAN_POINT('Ctrl Pts',(-0.123839091354566,1.80246825857577,
8.74843337927783));
#63067=CARTESIAN_POINT('Ctrl Pts',(-0.122899429292558,1.80207813075246,
8.74849629679433));
#63068=CARTESIAN_POINT('Ctrl Pts',(-0.12222340129491,1.80180015074258,8.74854135928366));
#63069=CARTESIAN_POINT('Ctrl Pts',(-0.112330754647716,1.79777162673305,
8.74919790441448));
#63070=CARTESIAN_POINT('Ctrl Pts',(-0.102945133706881,1.79444716865806,
8.74978441829878));
#63071=CARTESIAN_POINT('Ctrl Pts',(-0.0857908400194216,1.78925147505316,
8.75081721926188));
#63072=CARTESIAN_POINT('Ctrl Pts',(-0.0780785500121411,1.78722457757065,
8.75126781189534));
#63073=CARTESIAN_POINT('Ctrl Pts',(-0.0443138837009667,1.77967766057423,
8.75321054427306));
#63074=CARTESIAN_POINT('Ctrl Pts',(-0.0177120305236979,1.77711255364482,
8.75467479387227));
#63075=CARTESIAN_POINT('Ctrl Pts',(0.0148563386640629,1.77801250497585,
8.75660263305416));
#63076=CARTESIAN_POINT('Ctrl Pts',(0.0208047252700085,1.77834208521132,
8.75695973339654));
#63077=CARTESIAN_POINT('Ctrl Pts',(0.0278372007182144,1.77892761338925,
8.7573890124909));
#63078=CARTESIAN_POINT('Ctrl Pts',(0.0289336293793941,1.77902456132658,
8.75745614506992));
#63079=CARTESIAN_POINT('Ctrl Pts',(0.0305441895539643,1.77917528881871,
8.75755506400842));
#63080=CARTESIAN_POINT('Ctrl Pts',(0.0310587307676597,1.77922469225601,
8.75758671267006));
#63081=CARTESIAN_POINT('Ctrl Pts',(0.0319664006810245,1.77931404614726,
8.75764262421642));
#63082=CARTESIAN_POINT('Ctrl Pts',(0.032359579890751,1.77935348223007,8.75766687086365));
#63083=CARTESIAN_POINT('Ctrl Pts',(0.0331265157681409,1.77943183129544,
8.7577142198783));
#63084=CARTESIAN_POINT('Ctrl Pts',(0.0335002790241556,1.77947067507485,
8.75773732003031));
#63085=CARTESIAN_POINT('Ctrl Pts',(0.0345037177054995,1.77957673289986,
8.75779940380947));
#63086=CARTESIAN_POINT('Ctrl Pts',(0.0351332619766329,1.77964514904817,
8.75783842525451));
#63087=CARTESIAN_POINT('Ctrl Pts',(0.0374279163017484,1.77990136743283,
8.75798091755415));
#63088=CARTESIAN_POINT('Ctrl Pts',(0.0390917341974001,1.78010029753503,
8.75808473858858));
#63089=CARTESIAN_POINT('Ctrl Pts',(0.0673841753349688,1.78370702663367,
8.75985892414296));
#63090=CARTESIAN_POINT('Ctrl Pts',(0.0934800062884635,1.79041521019778,
8.76164116536206));
#63091=CARTESIAN_POINT('Ctrl Pts',(0.133196876933989,1.80610944923135,8.76452972936043));
#63092=CARTESIAN_POINT('Ctrl Pts',(0.147507000707802,1.81302473610557,8.76560757647378));
#63093=CARTESIAN_POINT('Ctrl Pts',(0.165513696467116,1.82343058250576,8.76697145076985));
#63094=CARTESIAN_POINT('Ctrl Pts',(0.169720679573648,1.82599211119791,8.76729056943461));
#63095=CARTESIAN_POINT('Ctrl Pts',(0.175217492881881,1.82951418450674,8.76770653218142));
#63096=CARTESIAN_POINT('Ctrl Pts',(0.176561005927488,1.83038924794715,8.76780811898252));
#63097=CARTESIAN_POINT('Ctrl Pts',(0.178773970572868,1.83185424342745,8.76797523877158));
#63098=CARTESIAN_POINT('Ctrl Pts',(0.17964715101956,1.83243845469619,8.76804112564475));
#63099=CARTESIAN_POINT('Ctrl Pts',(0.180813073435839,1.83322680901411,8.76812901168384));
#63100=CARTESIAN_POINT('Ctrl Pts',(0.181108343146563,1.83342717505389,8.76815126103359));
#63101=CARTESIAN_POINT('Ctrl Pts',(0.181572373698216,1.83374318677741,8.76818621392171));
#63102=CARTESIAN_POINT('Ctrl Pts',(0.181741357112701,1.83385850268467,8.76819893979343));
#63103=CARTESIAN_POINT('Ctrl Pts',(0.182091513180357,1.83409794156049,8.76822530363758));
#63104=CARTESIAN_POINT('Ctrl Pts',(0.182272667340052,1.8342220878333,8.76823893974835));
#63105=CARTESIAN_POINT('Ctrl Pts',(0.182684697413777,1.83450507445787,8.76826994742903));
#63106=CARTESIAN_POINT('Ctrl Pts',(0.182915492797769,1.83466403060693,8.76828731095464));
#63107=CARTESIAN_POINT('Ctrl Pts',(0.183631540248659,1.83515857360068,8.76834116653154));
#63108=CARTESIAN_POINT('Ctrl Pts',(0.184116081808442,1.83549519447874,8.7683775884164));
#63109=CARTESIAN_POINT('Ctrl Pts',(0.187807285508566,1.83807460628332,8.76865490516783));
#63110=CARTESIAN_POINT('Ctrl Pts',(0.190973955757526,1.8403744235781,8.76889199097375));
#63111=CARTESIAN_POINT('Ctrl Pts',(0.194546229958606,1.84306955195291,8.76915947535224));
#63112=CARTESIAN_POINT('Ctrl Pts',(0.194993458407329,1.84340880390833,8.76919296344005));
#63113=CARTESIAN_POINT('Ctrl Pts',(0.196045023192711,1.84421082143432,8.76927171100662));
#63114=CARTESIAN_POINT('Ctrl Pts',(0.196648613313292,1.84467456473654,8.7693169172034));
#63115=CARTESIAN_POINT('Ctrl Pts',(0.202992241002735,1.849584265379,8.7697921529898));
#63116=CARTESIAN_POINT('Ctrl Pts',(0.208582489825422,1.85422113909048,8.77021206647014));
#63117=CARTESIAN_POINT('Ctrl Pts',(0.229272364076566,1.87259735362667,8.7717908520609));
#63118=CARTESIAN_POINT('Ctrl Pts',(0.24321124562788,1.88757088328228,8.7729099371792));
#63119=CARTESIAN_POINT('Ctrl Pts',(0.260543291125407,1.91014954018143,8.77452207103142));
#63120=CARTESIAN_POINT('Ctrl Pts',(0.265204698588115,1.9167175401006,8.77498284455656));
#63121=CARTESIAN_POINT('Ctrl Pts',(0.274922117527831,1.93155756178613,8.77601551048747));
#63122=CARTESIAN_POINT('Ctrl Pts',(0.279860544777585,1.9398966809335,8.77659048054858));
#63123=CARTESIAN_POINT('Ctrl Pts',(0.284955152850656,1.94945747186269,8.7772492787722));
#63124=CARTESIAN_POINT('Ctrl Pts',(0.285489271375744,1.95047285266493,8.77731923677799));
#63125=CARTESIAN_POINT('Ctrl Pts',(0.286260229435344,1.95195766452471,8.77742153400054));
#63126=CARTESIAN_POINT('Ctrl Pts',(0.286501364179161,1.95242486534765,8.77745372159955));
#63127=CARTESIAN_POINT('Ctrl Pts',(0.286922335528286,1.95324542187343,8.77751025337633));
#63128=CARTESIAN_POINT('Ctrl Pts',(0.287102665797678,1.95359852420242,8.7775345801248));
#63129=CARTESIAN_POINT('Ctrl Pts',(0.287451395209751,1.95428448890782,8.77758183952082));
#63130=CARTESIAN_POINT('Ctrl Pts',(0.287619869010104,1.95461731282687,8.77760476950006));
#63131=CARTESIAN_POINT('Ctrl Pts',(0.288020478083653,1.95541214722366,8.77765953052191));
#63132=CARTESIAN_POINT('Ctrl Pts',(0.288252079560253,1.95587442423281,8.77769138020848));
#63133=CARTESIAN_POINT('Ctrl Pts',(0.289075665002224,1.95752822836355,8.77780532656314));
#63134=CARTESIAN_POINT('Ctrl Pts',(0.289661375319058,1.95872284907736,8.77788764201278));
#63135=CARTESIAN_POINT('Ctrl Pts',(0.299662889516564,1.97944570635287,8.77931577445174));
#63136=CARTESIAN_POINT('Ctrl Pts',(0.307090040568869,1.99986732285151,8.78073238544349));
#63137=CARTESIAN_POINT('Ctrl Pts',(0.31688438347207,2.03853895590807,8.78341212989071));
#63138=CARTESIAN_POINT('Ctrl Pts',(0.319851863138486,2.05654935492758,8.78465750305385));
#63139=CARTESIAN_POINT('Ctrl Pts',(0.322017719441619,2.08406849100827,8.78649255061327));
#63140=CARTESIAN_POINT('Ctrl Pts',(0.322345127745983,2.09345172232237,8.7871059573917));
#63141=CARTESIAN_POINT('Ctrl Pts',(0.322254357045707,2.10376349600042,8.78775742936807));
#63142=CARTESIAN_POINT('Ctrl Pts',(0.322242201653298,2.10469020888693,8.78781577493486));
#63143=CARTESIAN_POINT('Ctrl Pts',(0.322214187898982,2.1062972893788,8.78791659123541));
#63144=CARTESIAN_POINT('Ctrl Pts',(0.322200171904551,2.10697767737924,8.78795916024547));
#63145=CARTESIAN_POINT('Ctrl Pts',(0.322176874657326,2.10795782592793,8.78802031554977));
#63146=CARTESIAN_POINT('Ctrl Pts',(0.32216933012098,2.1082576200331,8.78803899816941));
#63147=CARTESIAN_POINT('Ctrl Pts',(0.322155448658234,2.10878021668604,8.78807152533318));
#63148=CARTESIAN_POINT('Ctrl Pts',(0.322149299038407,2.10900302368569,8.78808538044692));
#63149=CARTESIAN_POINT('Ctrl Pts',(0.322137008366368,2.10943218342938,8.7881120427815));
#63150=CARTESIAN_POINT('Ctrl Pts',(0.322130900200218,2.10963853621049,8.78812485185188));
#63151=CARTESIAN_POINT('Ctrl Pts',(0.322115932129284,2.1101282914895,8.78815522700341));
#63152=CARTESIAN_POINT('Ctrl Pts',(0.322106896469763,2.11041168901096,8.78817278316068));
#63153=CARTESIAN_POINT('Ctrl Pts',(0.322073799759564,2.11140844374886,8.78823446016852));
#63154=CARTESIAN_POINT('Ctrl Pts',(0.322047742638686,2.11212173933942,8.78827846973815));
#63155=CARTESIAN_POINT('Ctrl Pts',(0.321665481461743,2.12171238658769,8.78886855655391));
#63156=CARTESIAN_POINT('Ctrl Pts',(0.320944658955875,2.13057235535916,8.78939474612698));
#63157=CARTESIAN_POINT('Ctrl Pts',(0.316347648893621,2.16789946524014,8.79157348813092));
#63158=CARTESIAN_POINT('Ctrl Pts',(0.309041647680371,2.19581066888568,8.79311950746693));
#63159=CARTESIAN_POINT('Ctrl Pts',(0.29371756233942,2.2331402184187,8.79544024328249));
#63160=CARTESIAN_POINT('Ctrl Pts',(0.288724551688154,2.24364683117515,8.79612270671749));
#63161=CARTESIAN_POINT('Ctrl Pts',(0.282191295736733,2.25567111679856,8.79695002621638));
#63162=CARTESIAN_POINT('Ctrl Pts',(0.281189927467982,2.25747269090075,8.79707523921317));
#63163=CARTESIAN_POINT('Ctrl Pts',(0.279843320442655,2.25984158490248,8.79724159771543));
#63164=CARTESIAN_POINT('Ctrl Pts',(0.279513496203458,2.26041764768951,8.7972821877295));
#63165=CARTESIAN_POINT('Ctrl Pts',(0.278969967835434,2.2613601953682,8.79734882446085));
#63166=CARTESIAN_POINT('Ctrl Pts',(0.27875731451587,2.26172728651821,8.79737483313035));
#63167=CARTESIAN_POINT('Ctrl Pts',(0.278344478827622,2.2624367076563,8.79742520481471));
#63168=CARTESIAN_POINT('Ctrl Pts',(0.278144388115525,2.26277909032073,8.79744956447199));
#63169=CARTESIAN_POINT('Ctrl Pts',(0.27768184869669,2.26356721583485,8.79750575141895));
#63170=CARTESIAN_POINT('Ctrl Pts',(0.277418958272868,2.26401269700056,8.79753759473544));
#63171=CARTESIAN_POINT('Ctrl Pts',(0.276577230343338,2.26543123397116,8.79763926274733));
#63172=CARTESIAN_POINT('Ctrl Pts',(0.275994341886924,2.2664018651085,8.79770923509907));
#63173=CARTESIAN_POINT('Ctrl Pts',(0.270721457989278,2.27507839611782,8.79833841171719));
#63174=CARTESIAN_POINT('Ctrl Pts',(0.265715376629005,2.28258659570454,8.79890924320437));
#63175=CARTESIAN_POINT('Ctrl Pts',(0.257776643450155,2.2934740931857,8.79977863669193));
#63176=CARTESIAN_POINT('Ctrl Pts',(0.255077637659044,2.2970188279369,8.80006866589417));
#63177=CARTESIAN_POINT('Ctrl Pts',(0.238002577770641,2.31850513974181,8.80186971172069));
#63178=CARTESIAN_POINT('Ctrl Pts',(0.221814876426225,2.33492060095534,8.80344146712607));
#63179=CARTESIAN_POINT('Ctrl Pts',(0.193370247451214,2.35818297835718,8.80591021540188));
#63180=CARTESIAN_POINT('Ctrl Pts',(0.182170533410412,2.36620386777425,8.80682068596833));
#63181=CARTESIAN_POINT('Ctrl Pts',(0.169971149655269,2.37380898286792,8.80772458044402));
#63182=CARTESIAN_POINT('Ctrl Pts',(0.169450426986674,2.37413154437732,8.80776300186166));
#63183=CARTESIAN_POINT('Ctrl Pts',(0.16851369083295,2.37470811638072,8.80783182614452));
#63184=CARTESIAN_POINT('Ctrl Pts',(0.168098016439848,2.37496267033908,8.80786226375829));
#63185=CARTESIAN_POINT('Ctrl Pts',(0.167458972517395,2.37535202234476,8.80790889768027));
#63186=CARTESIAN_POINT('Ctrl Pts',(0.167236016443831,2.37548749244037,8.8079251380064));
#63187=CARTESIAN_POINT('Ctrl Pts',(0.166844569762744,2.37572468859786,8.80795359878342));
#63188=CARTESIAN_POINT('Ctrl Pts',(0.1666761509022,2.37582653078125,8.80796582689884));
#63189=CARTESIAN_POINT('Ctrl Pts',(0.16629511898072,2.37605646277275,8.80799345327738));
#63190=CARTESIAN_POINT('Ctrl Pts',(0.166082451614913,2.37618446100748,8.8080088454511));
#63191=CARTESIAN_POINT('Ctrl Pts',(0.165506183125178,2.3765303937591,8.80805048120272));
#63192=CARTESIAN_POINT('Ctrl Pts',(0.165142297933698,2.37674785773928,8.80807669388768));
#63193=CARTESIAN_POINT('Ctrl Pts',(0.16350972488175,2.3777191446436,8.80819395194698));
#63194=CARTESIAN_POINT('Ctrl Pts',(0.162236271300806,2.37846498146501,8.80828448385238));
#63195=CARTESIAN_POINT('Ctrl Pts',(0.137305765971917,2.39283721444691,8.81003962155796));
#63196=CARTESIAN_POINT('Ctrl Pts',(0.112012697052257,2.4034142518641,8.81152574565271));
#63197=CARTESIAN_POINT('Ctrl Pts',(0.0644520308146028,2.41653157999843,
8.81429426335219));
#63198=CARTESIAN_POINT('Ctrl Pts',(0.0426783635898178,2.4201946969691,8.81555308599202));
#63199=CARTESIAN_POINT('Ctrl Pts',(0.019450692515286,2.4216899459763,8.81696744759775));
#63200=CARTESIAN_POINT('Ctrl Pts',(0.0181977863153876,2.42176325347233,
8.81704393754693));
#63201=CARTESIAN_POINT('Ctrl Pts',(0.0163998204168731,2.42185791742771,
8.81715399902614));
#63202=CARTESIAN_POINT('Ctrl Pts',(0.0158550740017596,2.42188521206049,
8.81718738427328));
#63203=CARTESIAN_POINT('Ctrl Pts',(0.0149109352396885,2.42193011580013,
8.81724531496638));
#63204=CARTESIAN_POINT('Ctrl Pts',(0.0145115733687877,2.42194836493581,
8.81726984029324));
#63205=CARTESIAN_POINT('Ctrl Pts',(0.0137445614716117,2.42198198405806,
8.81731698455669));
#63206=CARTESIAN_POINT('Ctrl Pts',(0.0133769168115668,2.42199746757216,
8.81733959989577));
#63207=CARTESIAN_POINT('Ctrl Pts',(0.0125121573914139,2.42203240371802,
8.81739283778809));
#63208=CARTESIAN_POINT('Ctrl Pts',(0.0120150235689858,2.42205133493157,
8.81742347664173));
#63209=CARTESIAN_POINT('Ctrl Pts',(0.0105505746195737,2.42210370662052,
8.81751383152523));
#63210=CARTESIAN_POINT('Ctrl Pts',(0.00958315677007563,2.42213394033701,
8.81757364792153));
#63211=CARTESIAN_POINT('Ctrl Pts',(0.00114818908164743,2.42235951944911,
8.81809632557724));
#63212=CARTESIAN_POINT('Ctrl Pts',(-0.00632337799140969,2.42229951596798,
8.81856714358265));
#63213=CARTESIAN_POINT('Ctrl Pts',(-0.0452221131712706,2.42063405834695,
8.82106213584235));
#63214=CARTESIAN_POINT('Ctrl Pts',(-0.0762890915469068,2.41469109347257,
8.82322720676722));
#63215=CARTESIAN_POINT('Ctrl Pts',(-0.117051324841573,2.40049506249168,
8.8261097325587));
#63216=CARTESIAN_POINT('Ctrl Pts',(-0.127893051336785,2.39604346267437,
8.82687787116214));
#63217=CARTESIAN_POINT('Ctrl Pts',(-0.139095793645375,2.39071294568465,
8.82765609697782));
#63218=CARTESIAN_POINT('Ctrl Pts',(-0.139721080584836,2.39041294093043,
8.82769948064076));
#63219=CARTESIAN_POINT('Ctrl Pts',(-0.140617868455738,2.38997910667554,
8.82776161950276));
#63220=CARTESIAN_POINT('Ctrl Pts',(-0.140890151361558,2.38984691215967,
8.82778047521528));
#63221=CARTESIAN_POINT('Ctrl Pts',(-0.14136209187765,2.38961696087007,8.82781313785937));
#63222=CARTESIAN_POINT('Ctrl Pts',(-0.14156183498671,2.38951938090572,8.82782695586999));
#63223=CARTESIAN_POINT('Ctrl Pts',(-0.141947637480392,2.38933041113613,
8.82785363335594));
#63224=CARTESIAN_POINT('Ctrl Pts',(-0.142133709195218,2.3892390487218,8.82786649451581));
#63225=CARTESIAN_POINT('Ctrl Pts',(-0.142576989772869,2.38902086404293,
8.82789712137573));
#63226=CARTESIAN_POINT('Ctrl Pts',(-0.142834118289561,2.38889387760688,
8.82791487676211));
#63227=CARTESIAN_POINT('Ctrl Pts',(-0.143747520811072,2.38844126371283,
8.82797791528867));
#63228=CARTESIAN_POINT('Ctrl Pts',(-0.14440285995952,2.38811373867302,8.82802308059625));
#63229=CARTESIAN_POINT('Ctrl Pts',(-0.154046628178938,2.38325281170862,
8.82868687305661));
#63230=CARTESIAN_POINT('Ctrl Pts',(-0.162819991638525,2.37830238230672,
8.82927994136813));
#63231=CARTESIAN_POINT('Ctrl Pts',(-0.182365272159847,2.36603250847289,
8.83060895750549));
#63232=CARTESIAN_POINT('Ctrl Pts',(-0.192954204416631,2.35845521681986,
8.83133509974725));
#63233=CARTESIAN_POINT('Ctrl Pts',(-0.212911693850643,2.34226194539666,
8.8327716051899));
#63234=CARTESIAN_POINT('Ctrl Pts',(-0.222285561657763,2.33369071317039,
8.83348073371653));
#63235=CARTESIAN_POINT('Ctrl Pts',(-0.241380749795235,2.314039489622,8.83504697116557));
#63236=CARTESIAN_POINT('Ctrl Pts',(-0.25089653278207,2.30280140706446,8.83590816030668));
#63237=CARTESIAN_POINT('Ctrl Pts',(-0.260264370181138,2.29006538244534,
8.83686991007667));
#63238=CARTESIAN_POINT('Ctrl Pts',(-0.260913280849371,2.2891736023311,8.83693717484378));
#63239=CARTESIAN_POINT('Ctrl Pts',(-0.261859826732141,2.28785865536907,
8.8370362521097));
#63240=CARTESIAN_POINT('Ctrl Pts',(-0.262161045711064,2.28743806806519,
8.83706792627387));
#63241=CARTESIAN_POINT('Ctrl Pts',(-0.2626905925084,2.28669489662663,8.83712386701633));
#63242=CARTESIAN_POINT('Ctrl Pts',(-0.262919342634793,2.28637261355971,
8.83714811730096));
#63243=CARTESIAN_POINT('Ctrl Pts',(-0.263364356188542,2.28574318996892,
8.83719546145926));
#63244=CARTESIAN_POINT('Ctrl Pts',(-0.263580676674741,2.28543609037149,
8.8372185530955));
#63245=CARTESIAN_POINT('Ctrl Pts',(-0.264159823708576,2.28461084281381,
8.83728058500736));
#63246=CARTESIAN_POINT('Ctrl Pts',(-0.264521661105536,2.28409200564671,
8.83731956298646));
#63247=CARTESIAN_POINT('Ctrl Pts',(-0.265833916905219,2.28219851050813,
8.83746173654556));
#63248=CARTESIAN_POINT('Ctrl Pts',(-0.266775153432269,2.28081754879097,
8.83756528027127));
#63249=CARTESIAN_POINT('Ctrl Pts',(-0.267929849436996,2.27909476163688,
8.83769428828531));
#63250=CARTESIAN_POINT('Ctrl Pts',(-0.268153478127074,2.27875975506551,
8.837719366966));
#63251=CARTESIAN_POINT('Ctrl Pts',(-0.287540395923266,2.24959897488626,
8.83990169283422));
#63252=CARTESIAN_POINT('Ctrl Pts',(-0.301931254759561,2.2178795043545,8.84225666039802));
#63253=CARTESIAN_POINT('Ctrl Pts',(-0.31485105909334,2.17032470634958,8.84557219905085));
#63254=CARTESIAN_POINT('Ctrl Pts',(-0.317728279144217,2.15590717156857,
8.84654588727399));
#63255=CARTESIAN_POINT('Ctrl Pts',(-0.319708477482743,2.14059836451964,
8.84751480552321));
#63256=CARTESIAN_POINT('Ctrl Pts',(-0.319802064784626,2.13985444971627,
8.84756172789254));
#63257=CARTESIAN_POINT('Ctrl Pts',(-0.319930975701138,2.13880005213162,
8.8476279992011));
#63258=CARTESIAN_POINT('Ctrl Pts',(-0.319968444333143,2.1384898414066,8.84764746789428));
#63259=CARTESIAN_POINT('Ctrl Pts',(-0.320032006584502,2.13795708881445,
8.84768085326594));
#63260=CARTESIAN_POINT('Ctrl Pts',(-0.320058319333889,2.13773457374957,
8.8476947823928));
#63261=CARTESIAN_POINT('Ctrl Pts',(-0.320108259446001,2.13730844243144,
8.84772142874444));
#63262=CARTESIAN_POINT('Ctrl Pts',(-0.320131924574502,2.13710483137036,
8.8477341481219));
#63263=CARTESIAN_POINT('Ctrl Pts',(-0.320187211364249,2.13662516227013,
8.84776408319475));
#63264=CARTESIAN_POINT('Ctrl Pts',(-0.320218670357147,2.13634908511332,
8.84778128964151));
#63265=CARTESIAN_POINT('Ctrl Pts',(-0.320310533907743,2.13553353585035,
8.84783205182091));
#63266=CARTESIAN_POINT('Ctrl Pts',(-0.320369932914362,2.1349939480032,8.84786555111782));
#63267=CARTESIAN_POINT('Ctrl Pts',(-0.320878396509613,2.13026517998466,
8.84815839263795));
#63268=CARTESIAN_POINT('Ctrl Pts',(-0.32124666110887,2.12606747643924,8.84841329407567));
#63269=CARTESIAN_POINT('Ctrl Pts',(-0.321544051180808,2.12169395446229,
8.84867474294954));
#63270=CARTESIAN_POINT('Ctrl Pts',(-0.321555447073908,2.12152438076493,
8.84868487360629));
#63271=CARTESIAN_POINT('Ctrl Pts',(-0.321633513349248,2.12034883625798,
8.84875505866966));
#63272=CARTESIAN_POINT('Ctrl Pts',(-0.321695597827328,2.11934255496585,
8.84881491357782));
#63273=CARTESIAN_POINT('Ctrl Pts',(-0.321847816361753,2.11667148176497,
8.84897323585806));
#63274=CARTESIAN_POINT('Ctrl Pts',(-0.321929756761703,2.1150062356838,8.84907136647059));
#63275=CARTESIAN_POINT('Ctrl Pts',(-0.32204088584863,2.11232390002778,8.84922861551369));
#63276=CARTESIAN_POINT('Ctrl Pts',(-0.32207818617969,2.11130719671791,8.84928802972966));
#63277=CARTESIAN_POINT('Ctrl Pts',(-0.32221786023398,2.10693507943468,8.84954277943375));
#63278=CARTESIAN_POINT('Ctrl Pts',(-0.322272620580041,2.10357827202705,
8.84973647614376));
#63279=CARTESIAN_POINT('Ctrl Pts',(-0.322290768041176,2.07713063214126,
8.8512517776118));
#63280=CARTESIAN_POINT('Ctrl Pts',(-0.319825063208097,2.05410476171697,
8.85251106920004));
#63281=CARTESIAN_POINT('Ctrl Pts',(-0.313582461707878,2.02538880381381,
8.8541831089166));
#63282=CARTESIAN_POINT('Ctrl Pts',(-0.312065577726141,2.01927912088184,
8.85454453917948));
#63283=CARTESIAN_POINT('Ctrl Pts',(-0.307731685966037,2.00377920850272,
8.85548100968785));
#63284=CARTESIAN_POINT('Ctrl Pts',(-0.304663580332873,1.99446657045809,
8.85606248285969));
#63285=CARTESIAN_POINT('Ctrl Pts',(-0.300805753399857,1.98433601285977,
8.85672165078864));
#63286=CARTESIAN_POINT('Ctrl Pts',(-0.300430593039771,1.98336502271776,
8.85678510402785));
#63287=CARTESIAN_POINT('Ctrl Pts',(-0.299862416655417,1.98191539886184,
8.85688025153368));
#63288=CARTESIAN_POINT('Ctrl Pts',(-0.299672941906687,1.98143537697742,
8.8569118267362));
#63289=CARTESIAN_POINT('Ctrl Pts',(-0.29934461740526,1.98060940314597,8.85696627706987));
#63290=CARTESIAN_POINT('Ctrl Pts',(-0.299206318471468,1.98026323216522,
8.85698913360348));
#63291=CARTESIAN_POINT('Ctrl Pts',(-0.298919632775466,1.97954923794643,
8.85703635109468));
#63292=CARTESIAN_POINT('Ctrl Pts',(-0.298771167029535,1.97918144725447,
8.85706071468962));
#63293=CARTESIAN_POINT('Ctrl Pts',(-0.298423982093608,1.97832592755294,
8.85711748305613));
#63294=CARTESIAN_POINT('Ctrl Pts',(-0.29822474596679,1.97783841077389,8.85714990527332));
#63295=CARTESIAN_POINT('Ctrl Pts',(-0.29758586554852,1.97628599289326,8.85725338233978));
#63296=CARTESIAN_POINT('Ctrl Pts',(-0.297141709289092,1.9752229689639,8.8573245900226));
#63297=CARTESIAN_POINT('Ctrl Pts',(-0.287349671482454,1.95213593403689,
8.85887885290199));
#63298=CARTESIAN_POINT('Ctrl Pts',(-0.275585829744622,1.93122318310951,
8.86044940394228));
#63299=CARTESIAN_POINT('Ctrl Pts',(-0.246663942788651,1.89101663788483,
8.86378722553699));
#63300=CARTESIAN_POINT('Ctrl Pts',(-0.229281848669844,1.87208076536259,
8.86554801978358));
#63301=CARTESIAN_POINT('Ctrl Pts',(-0.208754706573058,1.85447058540916,
8.86725753455761));
#63302=CARTESIAN_POINT('Ctrl Pts',(-0.207663052093727,1.85354660091356,
8.86734744811972));
#63303=CARTESIAN_POINT('Ctrl Pts',(-0.206243786767565,1.85236144998933,
8.86746301827893));
#63304=CARTESIAN_POINT('Ctrl Pts',(-0.205921789298037,1.85209363112531,
8.8674891508703));
#63305=CARTESIAN_POINT('Ctrl Pts',(-0.205427995137265,1.85168454758796,
8.8675290910772));
#63306=CARTESIAN_POINT('Ctrl Pts',(-0.205256574328739,1.8515428330914,8.86754293150418));
#63307=CARTESIAN_POINT('Ctrl Pts',(-0.204918493577907,1.85126392860915,
8.86757017884476));
#63308=CARTESIAN_POINT('Ctrl Pts',(-0.20475184347794,1.85112672941004,8.86758358637682));
#63309=CARTESIAN_POINT('Ctrl Pts',(-0.204380148803442,1.8508213477693,8.86761343815956));
#63310=CARTESIAN_POINT('Ctrl Pts',(-0.204175034968636,1.85065325137634,
8.86762987608733));
#63311=CARTESIAN_POINT('Ctrl Pts',(-0.203581311731131,1.85016790277527,
8.86767735615302));
#63312=CARTESIAN_POINT('Ctrl Pts',(-0.203192166538295,1.84985130271099,
8.867708350976));
#63313=CARTESIAN_POINT('Ctrl Pts',(-0.200538069222985,1.84770226672015,
8.86791890794821));
#63314=CARTESIAN_POINT('Ctrl Pts',(-0.198249005885499,1.84589963297107,
8.86809636279078));
#63315=CARTESIAN_POINT('Ctrl Pts',(-0.19098816397572,1.84033958947094,8.86864749567428));
#63316=CARTESIAN_POINT('Ctrl Pts',(-0.185931422846102,1.83669499787208,
8.86901439166271));
#63317=CARTESIAN_POINT('Ctrl Pts',(-0.168350578715503,1.82478303779293,
8.87024519320756));
#63318=CARTESIAN_POINT('Ctrl Pts',(-0.155355905336822,1.81724410504196,
8.87108090119991));
#63319=CARTESIAN_POINT('Ctrl Pts',(-0.118521572621929,1.79918319523656,
8.8733740149801));
#63320=CARTESIAN_POINT('Ctrl Pts',(-0.0938636196441517,1.79060143293861,
8.87483698948597));
#63321=CARTESIAN_POINT('Ctrl Pts',(-0.0669083229615542,1.78474308615827,
8.87650932755639));
#63322=CARTESIAN_POINT('Ctrl Pts',(-0.0653702207950793,1.78442056546173,
8.87660495715832));
#63323=CARTESIAN_POINT('Ctrl Pts',(-0.0632859993804361,1.78399942128491,
8.87673483624149));
#63324=CARTESIAN_POINT('Ctrl Pts',(-0.0627418764662671,1.78389093591408,
8.87676877061321));
#63325=CARTESIAN_POINT('Ctrl Pts',(-0.061821358498288,1.78370987654059,
8.87682622581015));
#63326=CARTESIAN_POINT('Ctrl Pts',(-0.0614451078126426,1.78363656771305,
8.87684972315053));
#63327=CARTESIAN_POINT('Ctrl Pts',(-0.0607217814529869,1.78349697357264,
8.87689492155951));
#63328=CARTESIAN_POINT('Ctrl Pts',(-0.0603747255848012,1.78343058740698,
8.87691661937788));
#63329=CARTESIAN_POINT('Ctrl Pts',(-0.0595579664270996,1.78327574657764,
8.87696770998058));
#63330=CARTESIAN_POINT('Ctrl Pts',(-0.0590881750887718,1.78318776596906,
8.87699711782385));
#63331=CARTESIAN_POINT('Ctrl Pts',(-0.0577254124541961,1.7829356899484,
8.87708248559026));
#63332=CARTESIAN_POINT('Ctrl Pts',(-0.0568319466828875,1.78277432361056,
8.87713853225449));
#63333=CARTESIAN_POINT('Ctrl Pts',(-0.050598047280674,1.78167561812943,
8.87753013364932));
#63334=CARTESIAN_POINT('Ctrl Pts',(-0.0452356590802402,1.78086945640211,
8.87786983233231));
#63335=CARTESIAN_POINT('Ctrl Pts',(-0.0286035072074248,1.77879664658106,
8.87893308587018));
#63336=CARTESIAN_POINT('Ctrl Pts',(-0.0172862883562451,1.77798929953014,
8.87967049463249));
#63337=CARTESIAN_POINT('Ctrl Pts',(0.0248631475781336,1.7772108452284,8.88246349016681));
#63338=CARTESIAN_POINT('Ctrl Pts',(0.0555967588339537,1.78106448826708,
8.88460965130779));
#63339=CARTESIAN_POINT('Ctrl Pts',(0.0887021012420303,1.79015252929423,
8.8868151246211));
#63340=CARTESIAN_POINT('Ctrl Pts',(0.0920746595262546,1.79113793136097,
8.88703828513017));
#63341=CARTESIAN_POINT('Ctrl Pts',(0.0959763346076498,1.79234752515739,
8.88729414340403));
#63342=CARTESIAN_POINT('Ctrl Pts',(0.096521627993712,1.79251816732877,8.88732984892155));
#63343=CARTESIAN_POINT('Ctrl Pts',(0.0973330608546645,1.79277446549635,
8.88738289918576));
#63344=CARTESIAN_POINT('Ctrl Pts',(0.0975995436049225,1.79285901791535,
8.88740030824783));
#63345=CARTESIAN_POINT('Ctrl Pts',(0.0980745526824929,1.79301041435947,
8.88743131619295));
#63346=CARTESIAN_POINT('Ctrl Pts',(0.09828312074374,1.7930771240954,8.88744492297298));
#63347=CARTESIAN_POINT('Ctrl Pts',(0.0987263746579838,1.79321939540149,
8.8874738227648));
#63348=CARTESIAN_POINT('Ctrl Pts',(0.0989610411599483,1.79329501349921,
8.88748911233976));
#63349=CARTESIAN_POINT('Ctrl Pts',(0.0995918534760068,1.79349908356311,
8.88753018495524));
#63350=CARTESIAN_POINT('Ctrl Pts',(0.0999878391649064,1.7936280347695,8.88755593851882));
#63351=CARTESIAN_POINT('Ctrl Pts',(0.101898567340829,1.79425435504504,8.8876800690918));
#63352=CARTESIAN_POINT('Ctrl Pts',(0.103409888985203,1.79476220328917,8.88777783701345));
#63353=CARTESIAN_POINT('Ctrl Pts',(0.116078997629744,1.79912429186519,8.88859439840179));
#63354=CARTESIAN_POINT('Ctrl Pts',(0.12702238586571,1.80357816318646,8.88928018287624));
#63355=CARTESIAN_POINT('Ctrl Pts',(0.166147476990419,1.82206775399998,8.8917434812219));
#63356=CARTESIAN_POINT('Ctrl Pts',(0.192473461255659,1.83960536062014,8.89344198000537));
#63357=CARTESIAN_POINT('Ctrl Pts',(0.216998486171563,1.86172440113803,8.8953941844975));
#63358=CARTESIAN_POINT('Ctrl Pts',(0.218148091113861,1.86277644670589,8.89548661571909));
#63359=CARTESIAN_POINT('Ctrl Pts',(0.222861208161219,1.86715282441087,8.89586947834959));
#63360=CARTESIAN_POINT('Ctrl Pts',(0.226356575607455,1.87054930365324,8.89616277370531));
#63361=CARTESIAN_POINT('Ctrl Pts',(0.230369594465517,1.87462975266717,8.89651133297455));
#63362=CARTESIAN_POINT('Ctrl Pts',(0.230963330217309,1.87523826279754,8.89656321631688));
#63363=CARTESIAN_POINT('Ctrl Pts',(0.231911188212521,1.87621742876866,8.89664655198655));
#63364=CARTESIAN_POINT('Ctrl Pts',(0.232266848745611,1.87658659535731,8.89667793723287));
#63365=CARTESIAN_POINT('Ctrl Pts',(0.232895569621621,1.87724231561999,8.89673362479218));
#63366=CARTESIAN_POINT('Ctrl Pts',(0.233168986314741,1.87752852740528,8.89675791158907));
#63367=CARTESIAN_POINT('Ctrl Pts',(0.233729849183261,1.87811780670513,8.8968078749422));
#63368=CARTESIAN_POINT('Ctrl Pts',(0.234017234707306,1.87842093068635,8.89683355404813));
#63369=CARTESIAN_POINT('Ctrl Pts',(0.23471540153008,1.87916020539984,8.89689612885302));
#63370=CARTESIAN_POINT('Ctrl Pts',(0.235125556269604,1.87959694336141,8.89693305138742));
#63371=CARTESIAN_POINT('Ctrl Pts',(0.236029585552976,1.88056496054974,8.89701479239995));
#63372=CARTESIAN_POINT('Ctrl Pts',(0.236522888009921,1.8810967674325,8.89705963510838));
#63373=CARTESIAN_POINT('Ctrl Pts',(0.237919617337709,1.88261275084432,8.89718728670297));
#63374=CARTESIAN_POINT('Ctrl Pts',(0.238818717719707,1.88360087710475,8.89727027863465));
#63375=CARTESIAN_POINT('Ctrl Pts',(0.247174704874004,1.89289974765042,8.8980493630745));
#63376=CARTESIAN_POINT('Ctrl Pts',(0.254200282124472,1.9015862480755,8.89876329669453));
#63377=CARTESIAN_POINT('Ctrl Pts',(0.279222252804439,1.93603921425327,8.90154646187504));
#63378=CARTESIAN_POINT('Ctrl Pts',(0.293864757746272,1.96401740517007,8.90372971502152));
#63379=CARTESIAN_POINT('Ctrl Pts',(0.304591832199293,1.99470894525708,8.90585942279916));
#63380=CARTESIAN_POINT('Ctrl Pts',(0.304950154036124,1.99575128747471,8.90593142749199));
#63381=CARTESIAN_POINT('Ctrl Pts',(0.307139853746894,2.00222893045918,8.90637681035773));
#63382=CARTESIAN_POINT('Ctrl Pts',(0.308831351091482,2.00771089703728,8.90674463577063));
#63383=CARTESIAN_POINT('Ctrl Pts',(0.310552385674948,2.01386741670208,8.90714545396255));
#63384=CARTESIAN_POINT('Ctrl Pts',(0.310727108467706,2.0144998816654,8.90718648731425));
#63385=CARTESIAN_POINT('Ctrl Pts',(0.310976975400687,2.01541523742082,8.90724566300259));
#63386=CARTESIAN_POINT('Ctrl Pts',(0.311053666235849,2.01569769865062,8.90726389445221));
#63387=CARTESIAN_POINT('Ctrl Pts',(0.311187718825959,2.01619410320164,8.90729588339691));
#63388=CARTESIAN_POINT('Ctrl Pts',(0.311245244918827,2.01640800156178,8.90730965050072));
#63389=CARTESIAN_POINT('Ctrl Pts',(0.311364014517086,2.01685144301477,8.9073381566845));
#63390=CARTESIAN_POINT('Ctrl Pts',(0.311425224624566,2.01708099413683,8.90735289378404));
#63391=CARTESIAN_POINT('Ctrl Pts',(0.311582741691439,2.01767435190335,8.9073909376204));
#63392=CARTESIAN_POINT('Ctrl Pts',(0.311678665675963,2.01803826124121,8.90741422202649));
#63393=CARTESIAN_POINT('Ctrl Pts',(0.312078701058168,2.01956674394809,8.90751182208519));
#63394=CARTESIAN_POINT('Ctrl Pts',(0.312376929627991,2.02073286761323,8.90758580056656));
#63395=CARTESIAN_POINT('Ctrl Pts',(0.314432149371889,2.02896088461722,8.90810455857716));
#63396=CARTESIAN_POINT('Ctrl Pts',(0.315956190123305,2.03607944859552,8.90853667440967));
#63397=CARTESIAN_POINT('Ctrl Pts',(0.318670169255978,2.05124927929915,8.90943408763561));
#63398=CARTESIAN_POINT('Ctrl Pts',(0.319798908404867,2.05930624162602,8.90989702052615));
#63399=CARTESIAN_POINT('Ctrl Pts',(0.321941336036895,2.08037555605419,8.91109105610421));
#63400=CARTESIAN_POINT('Ctrl Pts',(0.322471822641228,2.09342168576267,8.91181450003036));
#63401=CARTESIAN_POINT('Ctrl Pts',(0.321786860081639,2.12756400069777,8.91373333809356));
#63402=CARTESIAN_POINT('Ctrl Pts',(0.319292234244214,2.14856774392116,8.914942662245));
#63403=CARTESIAN_POINT('Ctrl Pts',(0.314484286871246,2.17044500721736,8.91630310348402));
#63404=CARTESIAN_POINT('Ctrl Pts',(0.31419756013777,2.17171303129051,8.91638230479323));
#63405=CARTESIAN_POINT('Ctrl Pts',(0.313787238746545,2.17347793225166,8.91649303958141));
#63406=CARTESIAN_POINT('Ctrl Pts',(0.313670117674537,2.17397631378644,8.91652436494148));
#63407=CARTESIAN_POINT('Ctrl Pts',(0.313465915068896,2.17483604661298,8.91657849940072));
#63408=CARTESIAN_POINT('Ctrl Pts',(0.313379394776107,2.17519753127945,8.9166012904002));
#63409=CARTESIAN_POINT('Ctrl Pts',(0.313201102241993,2.17593679158553,8.91664796031189));
#63410=CARTESIAN_POINT('Ctrl Pts',(0.313109271429653,2.17631455237787,8.91667184108002));
#63411=CARTESIAN_POINT('Ctrl Pts',(0.312894393844351,2.17719156899034,8.9167273591163));
#63412=CARTESIAN_POINT('Ctrl Pts',(0.312770835552658,2.1776906972888,8.9167590128429));
#63413=CARTESIAN_POINT('Ctrl Pts',(0.312508225395731,2.17874076168891,8.91682572730963));
#63414=CARTESIAN_POINT('Ctrl Pts',(0.312368910060966,2.17929162952068,8.91686079648195));
#63415=CARTESIAN_POINT('Ctrl Pts',(0.311993661246145,2.1807590659377,8.91695440539228));
#63416=CARTESIAN_POINT('Ctrl Pts',(0.311755147069329,2.18167496332411,8.91701302851905));
#63417=CARTESIAN_POINT('Ctrl Pts',(0.311019757524381,2.18444870950738,8.91719117105373));
#63418=CARTESIAN_POINT('Ctrl Pts',(0.310510290512103,2.18630314789058,8.91731109734575));
#63419=CARTESIAN_POINT('Ctrl Pts',(0.301707762110398,2.21725670480012,8.91932696347975));
#63420=CARTESIAN_POINT('Ctrl Pts',(0.289375299231291,2.24504416850141,8.92136748264914));
#63421=CARTESIAN_POINT('Ctrl Pts',(0.265490327263784,2.28329375984226,8.9244152083093));
#63422=CARTESIAN_POINT('Ctrl Pts',(0.256762393972877,2.29533273655835,8.92541211550288));
#63423=CARTESIAN_POINT('Ctrl Pts',(0.245089131575015,2.30929328050275,8.92657983209037));
#63424=CARTESIAN_POINT('Ctrl Pts',(0.242904001756527,2.31182541816605,8.92679210179912));
#63425=CARTESIAN_POINT('Ctrl Pts',(0.240305419965702,2.31474356238312,8.92703682078126));
#63426=CARTESIAN_POINT('Ctrl Pts',(0.239929988045259,2.3151629459221,8.92707199295912));
#63427=CARTESIAN_POINT('Ctrl Pts',(0.239367579638569,2.31578789274175,8.92712440534689));
#63428=CARTESIAN_POINT('Ctrl Pts',(0.239181435446284,2.3159941984758,8.92714170764004));
#63429=CARTESIAN_POINT('Ctrl Pts',(0.238848242056302,2.31636252162515,8.92717259757277));
#63430=CARTESIAN_POINT('Ctrl Pts',(0.238701294854324,2.31652462985372,8.92718619287522));
#63431=CARTESIAN_POINT('Ctrl Pts',(0.238387705128317,2.3168698664483,8.9272151459766));
#63432=CARTESIAN_POINT('Ctrl Pts',(0.238221017112637,2.31705295191832,8.92723050017975));
#63433=CARTESIAN_POINT('Ctrl Pts',(0.237770234739882,2.31754693392924,8.92727192740529));
#63434=CARTESIAN_POINT('Ctrl Pts',(0.237485740450284,2.31785746734467,8.9272979700624));
#63435=CARTESIAN_POINT('Ctrl Pts',(0.236085516971168,2.3193798480159,8.92742564934313));
#63436=CARTESIAN_POINT('Ctrl Pts',(0.234961090739875,2.32058371460265,8.92752663397393));
#63437=CARTESIAN_POINT('Ctrl Pts',(0.228475385859191,2.32742176645885,8.92810070933279));
#63438=CARTESIAN_POINT('Ctrl Pts',(0.22292031983579,2.33286952202615,8.92855994614469));
#63439=CARTESIAN_POINT('Ctrl Pts',(0.204768037342205,2.34942558660646,8.92998287038919));
#63440=CARTESIAN_POINT('Ctrl Pts',(0.191496963064975,2.3597538479926,8.93091339431608));
#63441=CARTESIAN_POINT('Ctrl Pts',(0.169365888073198,2.37435540297082,8.93239684847875));
#63442=CARTESIAN_POINT('Ctrl Pts',(0.161013196783965,2.37933927476415,8.93294276876294));
#63443=CARTESIAN_POINT('Ctrl Pts',(0.13939703375399,2.3909451502094,8.93434359747116));
#63444=CARTESIAN_POINT('Ctrl Pts',(0.125879873193419,2.39704340017954,8.93520957022873));
#63445=CARTESIAN_POINT('Ctrl Pts',(0.110826028632106,2.40262239585278,8.93618502588585));
#63446=CARTESIAN_POINT('Ctrl Pts',(0.109657102572407,2.40304792175766,8.93626083108995));
#63447=CARTESIAN_POINT('Ctrl Pts',(0.108012704879563,2.40363577454573,8.93636756664988));
#63448=CARTESIAN_POINT('Ctrl Pts',(0.107539262275934,2.40380377723791,8.93639830825601));
#63449=CARTESIAN_POINT('Ctrl Pts',(0.10671719027324,2.40409332982125,8.93645170708666));
#63450=CARTESIAN_POINT('Ctrl Pts',(0.106368740282479,2.40421538920717,8.936474347361));
#63451=CARTESIAN_POINT('Ctrl Pts',(0.105650958820011,2.40446543861813,8.93652099780195));
#63452=CARTESIAN_POINT('Ctrl Pts',(0.10528160281724,2.40459335599886,8.93654501033346));
#63453=CARTESIAN_POINT('Ctrl Pts',(0.104416144219568,2.40489132405972,8.93660129259252));
#63454=CARTESIAN_POINT('Ctrl Pts',(0.103919858534033,2.40506083599448,8.93663358008765));
#63455=CARTESIAN_POINT('Ctrl Pts',(0.102872132782956,2.40541584506591,8.93670177202064));
#63456=CARTESIAN_POINT('Ctrl Pts',(0.102320600264549,2.40560106163925,8.93673768561277));
#63457=CARTESIAN_POINT('Ctrl Pts',(0.100839409636644,2.40609401833207,8.93683418114682));
#63458=CARTESIAN_POINT('Ctrl Pts',(0.099908850880177,2.4063990144833,8.93689485339801));
#63459=CARTESIAN_POINT('Ctrl Pts',(0.097060093387592,2.40731835414597,8.93708074836289));
#63460=CARTESIAN_POINT('Ctrl Pts',(0.0951375411472141,2.40791895117248,
8.9372064206804));
#63461=CARTESIAN_POINT('Ctrl Pts',(0.0881062408479981,2.4100433628044,8.93766688828996));
#63462=CARTESIAN_POINT('Ctrl Pts',(0.0829657499102364,2.41145830446664,
8.9380051759722));
#63463=CARTESIAN_POINT('Ctrl Pts',(0.0715603971888622,2.41429529248572,
8.93875964645394));
#63464=CARTESIAN_POINT('Ctrl Pts',(0.065283432379469,2.41565881293745,8.93917743793338));
#63465=CARTESIAN_POINT('Ctrl Pts',(0.0426728059678572,2.4198671829655,8.94069058204958));
#63466=CARTESIAN_POINT('Ctrl Pts',(0.0261668043160319,2.42163830251601,
8.94181195692942));
#63467=CARTESIAN_POINT('Ctrl Pts',(-0.00948715886695256,2.42270077233948,
8.94422528357856));
#63468=CARTESIAN_POINT('Ctrl Pts',(-0.028588996447638,2.42157215106553,
8.94551271211166));
#63469=CARTESIAN_POINT('Ctrl Pts',(-0.0486076322654278,2.418590289491,8.94678852344306));
#63470=CARTESIAN_POINT('Ctrl Pts',(-0.049733987095753,2.41841640204645,
8.94686005046168));
#63471=CARTESIAN_POINT('Ctrl Pts',(-0.0512375521396569,2.41817610770617,
8.94695516647691));
#63472=CARTESIAN_POINT('Ctrl Pts',(-0.0516155829978412,2.41811500099764,
8.94697904996131));
#63473=CARTESIAN_POINT('Ctrl Pts',(-0.0522058678254474,2.41801850463794,
8.9470162941752));
#63474=CARTESIAN_POINT('Ctrl Pts',(-0.0524181952141211,2.41798357620908,
8.94702968109365));
#63475=CARTESIAN_POINT('Ctrl Pts',(-0.05282491475024,2.41791625130544,8.94705530487045));
#63476=CARTESIAN_POINT('Ctrl Pts',(-0.0530193107610832,2.4178838894143,
8.94706754356569));
#63477=CARTESIAN_POINT('Ctrl Pts',(-0.0534786960207722,2.41780698057106,
8.94709644544344));
#63478=CARTESIAN_POINT('Ctrl Pts',(-0.0537436589901876,2.41776228056109,
8.94711309977187));
#63479=CARTESIAN_POINT('Ctrl Pts',(-0.0545195420548629,2.41763038865867,
8.94716182320525));
#63480=CARTESIAN_POINT('Ctrl Pts',(-0.0550303111361263,2.41754229502612,
8.94719384108015));
#63481=CARTESIAN_POINT('Ctrl Pts',(-0.0587908349926369,2.41688436208507,
8.94742916590621));
#63482=CARTESIAN_POINT('Ctrl Pts',(-0.0620320308223173,2.41626585402224,
8.94762975844531));
#63483=CARTESIAN_POINT('Ctrl Pts',(-0.0726883433434493,2.41406220580999,
8.94828357590692));
#63484=CARTESIAN_POINT('Ctrl Pts',(-0.080057468392593,2.41226508582347,
8.94872659776379));
#63485=CARTESIAN_POINT('Ctrl Pts',(-0.101767029822699,2.40615154332826,
8.9500226933532));
#63486=CARTESIAN_POINT('Ctrl Pts',(-0.115877658273491,2.40109418864508,
8.95085379849453));
#63487=CARTESIAN_POINT('Ctrl Pts',(-0.136913215012995,2.39185610721325,
8.95213904616455));
#63488=CARTESIAN_POINT('Ctrl Pts',(-0.14411772392343,2.38836659281184,8.95258795138594));
#63489=CARTESIAN_POINT('Ctrl Pts',(-0.166061897899345,2.37670996447366,
8.95399851793362));
#63490=CARTESIAN_POINT('Ctrl Pts',(-0.180294431458085,2.36765416603103,
8.95497789715423));
#63491=CARTESIAN_POINT('Ctrl Pts',(-0.194606628745201,2.35688631136057,
8.95606675364755));
#63492=CARTESIAN_POINT('Ctrl Pts',(-0.195457105451215,2.35623980331256,
8.95613186500964));
#63493=CARTESIAN_POINT('Ctrl Pts',(-0.196719028445348,2.35527058756554,
8.95622909274544));
#63494=CARTESIAN_POINT('Ctrl Pts',(-0.197132935212526,2.35495108330413,
8.95626108268312));
#63495=CARTESIAN_POINT('Ctrl Pts',(-0.197842023553578,2.35440096237444,
8.95631605856195));
#63496=CARTESIAN_POINT('Ctrl Pts',(-0.198137584889666,2.35417083505584,
8.95633902507114));
#63497=CARTESIAN_POINT('Ctrl Pts',(-0.198729996299828,2.35370791573786,
8.95638516213873));
#63498=CARTESIAN_POINT('Ctrl Pts',(-0.199026840188522,2.35347511676706,
8.95640833295378));
#63499=CARTESIAN_POINT('Ctrl Pts',(-0.199716152667372,2.35293256802114,
8.95646226160738));
#63500=CARTESIAN_POINT('Ctrl Pts',(-0.200108309752366,2.35262242569809,
8.95649303509207));
#63501=CARTESIAN_POINT('Ctrl Pts',(-0.201300525589124,2.35167502897891,
8.9565868756943));
#63502=CARTESIAN_POINT('Ctrl Pts',(-0.202098267919176,2.35103488179819,
8.95665005872169));
#63503=CARTESIAN_POINT('Ctrl Pts',(-0.203921648938973,2.34955738776692,
8.95679538395917));
#63504=CARTESIAN_POINT('Ctrl Pts',(-0.204945196540839,2.34871750044116,
8.95687762835488));
#63505=CARTESIAN_POINT('Ctrl Pts',(-0.208291380710295,2.34593705839446,
8.95714872155706));
#63506=CARTESIAN_POINT('Ctrl Pts',(-0.210591803545795,2.34397013596802,
8.95733864147238));
#63507=CARTESIAN_POINT('Ctrl Pts',(-0.21955526616318,2.33608490035683,8.95809300443898));
#63508=CARTESIAN_POINT('Ctrl Pts',(-0.225998811123837,2.3299241358665,8.95866737650572));
#63509=CARTESIAN_POINT('Ctrl Pts',(-0.256154937521758,2.29859773330147,
8.96151719372327));
#63510=CARTESIAN_POINT('Ctrl Pts',(-0.275963802860107,2.26999977396766,
8.96393974722564));
#63511=CARTESIAN_POINT('Ctrl Pts',(-0.292192277528338,2.23599464477283,
8.96635357884874));
#63512=CARTESIAN_POINT('Ctrl Pts',(-0.29349260337437,2.2331651755648,8.96655100239203));
#63513=CARTESIAN_POINT('Ctrl Pts',(-0.29497158628689,2.22982000772364,8.96678003229308));
#63514=CARTESIAN_POINT('Ctrl Pts',(-0.295190142031184,2.22932227642538,
8.966813997086));
#63515=CARTESIAN_POINT('Ctrl Pts',(-0.295518428274151,2.22856948031794,
8.96686519438217));
#63516=CARTESIAN_POINT('Ctrl Pts',(-0.295629088832514,2.22831482594112,
8.96688248347486));
#63517=CARTESIAN_POINT('Ctrl Pts',(-0.295826354172688,2.22785926507287,
8.96691335886861));
#63518=CARTESIAN_POINT('Ctrl Pts',(-0.295913083379698,2.22765841364295,
8.96692695280361));
#63519=CARTESIAN_POINT('Ctrl Pts',(-0.29609758450565,2.22722993926506,8.9669559127394));
#63520=CARTESIAN_POINT('Ctrl Pts',(-0.296195298223147,2.22700229252641,
8.96697127512441));
#63521=CARTESIAN_POINT('Ctrl Pts',(-0.296458652282342,2.22638679115667,
8.9670127472706));
#63522=CARTESIAN_POINT('Ctrl Pts',(-0.296623794655047,2.22599872198236,
8.96703882655314));
#63523=CARTESIAN_POINT('Ctrl Pts',(-0.297432870103816,2.22408706366514,
8.96716696299609));
#63524=CARTESIAN_POINT('Ctrl Pts',(-0.298065843703337,2.22255882130027,
8.96726836252298));
#63525=CARTESIAN_POINT('Ctrl Pts',(-0.30161367615232,2.21380290202484,8.96784378978326));
#63526=CARTESIAN_POINT('Ctrl Pts',(-0.304277623218085,2.20647562985073,
8.96830391459757));
#63527=CARTESIAN_POINT('Ctrl Pts',(-0.316996295114574,2.16710005743181,
8.97070014466733));
#63528=CARTESIAN_POINT('Ctrl Pts',(-0.322260308621024,2.13372621392319,
8.972489958609));
#63529=CARTESIAN_POINT('Ctrl Pts',(-0.322274969295649,2.10014067867101,
8.97445939472581));
#63530=CARTESIAN_POINT('',(-0.322274881362357,2.09972347173989,9.09972265507268));
#63531=CARTESIAN_POINT('Ctrl Pts',(-0.322274962187229,2.10015611604601,
8.97472265507268));
#63532=CARTESIAN_POINT('Ctrl Pts',(-0.322283729205766,2.0820581008871,8.9758346106162));
#63533=CARTESIAN_POINT('Ctrl Pts',(-0.320763654444053,2.06396370109893,
8.97694656615972));
#63534=CARTESIAN_POINT('Ctrl Pts',(-0.317742702268281,2.04614138156014,
8.97805852170324));
#63535=CARTESIAN_POINT('Ctrl Pts',(-0.314719940415267,2.02830838570335,
8.97917114335484));
#63536=CARTESIAN_POINT('Ctrl Pts',(-0.310194678618889,2.01074851592955,
8.98028376500643));
#63537=CARTESIAN_POINT('Ctrl Pts',(-0.304245854863578,1.99371907309714,
8.98139638665803));
#63538=CARTESIAN_POINT('Ctrl Pts',(-0.298280377608901,1.97664195700577,
8.98251212305041));
#63539=CARTESIAN_POINT('Ctrl Pts',(-0.290883676387714,1.96009891314594,
8.98362785944279));
#63540=CARTESIAN_POINT('Ctrl Pts',(-0.282182837315571,1.94432719585768,
8.98474359583517));
#63541=CARTESIAN_POINT('Ctrl Pts',(-0.277643074226491,1.93609812054632,
8.98532574416009));
#63542=CARTESIAN_POINT('Ctrl Pts',(-0.272749034639811,1.92807859711184,
8.98590789248501));
#63543=CARTESIAN_POINT('Ctrl Pts',(-0.26752335448613,1.92029905278634,8.98649004080994));
#63544=CARTESIAN_POINT('Ctrl Pts',(-0.257673757412418,1.90563581761505,
8.98758730016547));
#63545=CARTESIAN_POINT('Ctrl Pts',(-0.246584156538608,1.89173885726974,
8.98868455952099));
#63546=CARTESIAN_POINT('Ctrl Pts',(-0.234398341562797,1.87882451967361,
8.98978181887652));
#63547=CARTESIAN_POINT('Ctrl Pts',(-0.222235837736759,1.86593488687223,
8.9908769792032));
#63548=CARTESIAN_POINT('Ctrl Pts',(-0.208981760378368,1.85402474602817,
8.99197213952988));
#63549=CARTESIAN_POINT('Ctrl Pts',(-0.194820638675809,1.84327817706523,
8.99306729985656));
#63550=CARTESIAN_POINT('Ctrl Pts',(-0.180496633437845,1.83240799931036,
8.99417505689624));
#63551=CARTESIAN_POINT('Ctrl Pts',(-0.16524513381604,1.822728927404,8.99528281393592));
#63552=CARTESIAN_POINT('Ctrl Pts',(-0.149292342938792,1.81439017530056,
8.9963905709756));
#63553=CARTESIAN_POINT('Ctrl Pts',(-0.133528595180004,1.80615023874066,
8.99748520091753));
#63554=CARTESIAN_POINT('Ctrl Pts',(-0.117080824816662,1.79921931751597,
8.99857983085945));
#63555=CARTESIAN_POINT('Ctrl Pts',(-0.100191661963566,1.79369491271287,
8.99967446080138));
#63556=CARTESIAN_POINT('Ctrl Pts',(-0.0829986900103658,1.78807113267924,
9.00078878138994));
#63557=CARTESIAN_POINT('Ctrl Pts',(-0.0653490595285042,1.78390527915881,
9.00190310197849));
#63558=CARTESIAN_POINT('Ctrl Pts',(-0.0475129112710903,1.78124664882147,
9.00301742256705));
#63559=CARTESIAN_POINT('Ctrl Pts',(-0.0296767630136734,1.77858801848412,
9.0041317431556));
#63560=CARTESIAN_POINT('Ctrl Pts',(-0.0116549354123172,1.77743660794139,
9.00524606374416));
#63561=CARTESIAN_POINT('Ctrl Pts',(0.00628054822842578,1.77778620399035,
9.00636038433272));
#63562=CARTESIAN_POINT('Ctrl Pts',(0.0239414237635632,1.77813044741483,
9.00745764368825));
#63563=CARTESIAN_POINT('Ctrl Pts',(0.0416292381677865,1.77993210664495,
9.00855490304378));
#63564=CARTESIAN_POINT('Ctrl Pts',(0.0590842462719857,1.78318739376806,
9.00965216239931));
#63565=CARTESIAN_POINT('Ctrl Pts',(0.0765058633958602,1.78643645361087,
9.01074732272599));
#63566=CARTESIAN_POINT('Ctrl Pts',(0.0936947946213764,1.79113354471842,
9.01184248305267));
#63567=CARTESIAN_POINT('Ctrl Pts',(0.110396373268946,1.79722315743429,9.01293764337936));
#63568=CARTESIAN_POINT('Ctrl Pts',(0.127290056202733,1.8033828138705,9.01404540041904));
#63569=CARTESIAN_POINT('Ctrl Pts',(0.143684305481806,1.81096709130857,9.01515315745872));
#63570=CARTESIAN_POINT('Ctrl Pts',(0.15933121150109,1.81986656631777,9.0162609144984));
#63571=CARTESIAN_POINT('Ctrl Pts',(0.174792699186319,1.82866058112748,9.01735554444033));
#63572=CARTESIAN_POINT('Ctrl Pts',(0.189523817135947,1.83873832804346,9.01845017438226));
#63573=CARTESIAN_POINT('Ctrl Pts',(0.203311244625655,1.84994857842082,9.01954480432419));
#63574=CARTESIAN_POINT('Ctrl Pts',(0.217346685943797,1.86136048332118,9.02065912491275));
#63575=CARTESIAN_POINT('Ctrl Pts',(0.230403474059228,1.87394555685329,9.0217734455013));
#63576=CARTESIAN_POINT('Ctrl Pts',(0.242293927378484,1.88750334501336,9.02288776608986));
#63577=CARTESIAN_POINT('Ctrl Pts',(0.254184380697738,1.90106113317343,9.02400208667842));
#63578=CARTESIAN_POINT('Ctrl Pts',(0.264908048211737,1.91559092915891,9.02511640726697));
#63579=CARTESIAN_POINT('Ctrl Pts',(0.274322902962821,1.93086064758593,9.02623072785553));
#63580=CARTESIAN_POINT('Ctrl Pts',(0.283593607966985,1.94589657312872,9.02732798721106));
#63581=CARTESIAN_POINT('Ctrl Pts',(0.291653474164235,1.96174407486439,9.02842524656658));
#63582=CARTESIAN_POINT('Ctrl Pts',(0.298365081745992,1.97818270393861,9.02952250592211));
#63583=CARTESIAN_POINT('Ctrl Pts',(0.30506385019554,1.99458988633938,9.03061766624879));
#63584=CARTESIAN_POINT('Ctrl Pts',(0.31041913095044,2.01158526775857,9.03171282657547));
#63585=CARTESIAN_POINT('Ctrl Pts',(0.314339741848481,2.02892467151233,9.03280798690215));
#63586=CARTESIAN_POINT('Ctrl Pts',(0.318305448253605,2.0464635159209,9.03391574394183));
#63587=CARTESIAN_POINT('Ctrl Pts',(0.320802955351907,2.06435360066012,9.03502350098151));
#63588=CARTESIAN_POINT('Ctrl Pts',(0.321790070374446,2.08232724601514,9.03613125802119));
#63589=CARTESIAN_POINT('Ctrl Pts',(0.322765487926393,2.10008790080355,9.03722588796312));
#63590=CARTESIAN_POINT('Ctrl Pts',(0.322266158204137,2.11792935502614,9.03832051790505));
#63591=CARTESIAN_POINT('Ctrl Pts',(0.320303762597408,2.13559038200052,9.03941514784697));
#63592=CARTESIAN_POINT('Ctrl Pts',(0.3183060666239,2.15356910267936,9.04052946843553));
#63593=CARTESIAN_POINT('Ctrl Pts',(0.314792186798191,2.17136001160134,9.04164378902408));
#63594=CARTESIAN_POINT('Ctrl Pts',(0.309829072997926,2.18869679334816,9.04275810961264));
#63595=CARTESIAN_POINT('Ctrl Pts',(0.304865959197661,2.20603357509497,9.0438724302012));
#63596=CARTESIAN_POINT('Ctrl Pts',(0.298453961575723,2.22291546784511,9.04498675078975));
#63597=CARTESIAN_POINT('Ctrl Pts',(0.290711339919773,2.23909742077785,9.04610107137831));
#63598=CARTESIAN_POINT('Ctrl Pts',(0.283087264644172,2.25503161370986,9.04719833073383));
#63599=CARTESIAN_POINT('Ctrl Pts',(0.274125352650181,2.27038703255115,9.04829559008936));
#63600=CARTESIAN_POINT('Ctrl Pts',(0.263936573456107,2.28492879931814,9.04939284944489));
#63601=CARTESIAN_POINT('Ctrl Pts',(0.253767285133859,2.29944274806035,9.05048800977157));
#63602=CARTESIAN_POINT('Ctrl Pts',(0.242376174381177,2.31314547105133,9.05158317009825));
#63603=CARTESIAN_POINT('Ctrl Pts',(0.229919190773728,2.32582812344558,9.05267833042493));
#63604=CARTESIAN_POINT('Ctrl Pts',(0.217318924905658,2.33865665377971,9.05378608746461));
#63605=CARTESIAN_POINT('Ctrl Pts',(0.203628567065381,2.35044082858695,9.05489384450429));
#63606=CARTESIAN_POINT('Ctrl Pts',(0.189050347441566,2.36100027156542,9.05600160154397));
#63607=CARTESIAN_POINT('Ctrl Pts',(0.174644882047434,2.37143458345898,9.0570962314859));
#63608=CARTESIAN_POINT('Ctrl Pts',(0.159373171695866,2.38067263963363,9.05819086142782));
#63609=CARTESIAN_POINT('Ctrl Pts',(0.143461183805843,2.38858285528774,9.05928549136975));
#63610=CARTESIAN_POINT('Ctrl Pts',(0.127262964634619,2.39663536310403,9.06039981195831));
#63611=CARTESIAN_POINT('Ctrl Pts',(0.110401923236308,2.40331137049352,9.06151413254687));
#63612=CARTESIAN_POINT('Ctrl Pts',(0.0931382235613252,2.40852300876408,
9.06262845313543));
#63613=CARTESIAN_POINT('Ctrl Pts',(0.0758745238863453,2.41373464703464,
9.06374277372398));
#63614=CARTESIAN_POINT('Ctrl Pts',(0.0582089960319397,2.41748179821334,
9.06485709431254));
#63615=CARTESIAN_POINT('Ctrl Pts',(0.0404116992755282,2.41973124680998,
9.0659714149011));
#63616=CARTESIAN_POINT('Ctrl Pts',(0.0228868948613931,2.42194625436058,
9.06706867425663));
#63617=CARTESIAN_POINT('Ctrl Pts',(0.00512453887649297,2.42272308397212,
9.06816593361216));
#63618=CARTESIAN_POINT('Ctrl Pts',(-0.0126178092598918,2.42202789710595,
9.06926319296769));
#63619=CARTESIAN_POINT('Ctrl Pts',(-0.0303262167418809,2.42133404011433,
9.07035835329437));
#63620=CARTESIAN_POINT('Ctrl Pts',(-0.0480139256462691,2.41917372179016,
9.07145351362105));
#63621=CARTESIAN_POINT('Ctrl Pts',(-0.0654209171645705,2.41556501584039,
9.07254867394773));
#63622=CARTESIAN_POINT('Ctrl Pts',(-0.0830281267431725,2.41191480196521,
9.07365643098741));
#63623=CARTESIAN_POINT('Ctrl Pts',(-0.100347309977487,2.40678269072537,
9.07476418802709));
#63624=CARTESIAN_POINT('Ctrl Pts',(-0.117117332388186,2.4002410799329,9.07587194506677));
#63625=CARTESIAN_POINT('Ctrl Pts',(-0.133688627356306,2.39377698827257,
9.0769665750087));
#63626=CARTESIAN_POINT('Ctrl Pts',(-0.149723003145249,2.38593698750682,
9.07806120495063));
#63627=CARTESIAN_POINT('Ctrl Pts',(-0.164987500651015,2.37683984585665,
9.07915583489255));
#63628=CARTESIAN_POINT('Ctrl Pts',(-0.180526582118754,2.36757906113889,
9.08027015548111));
#63629=CARTESIAN_POINT('Ctrl Pts',(-0.195267075030213,2.35701583907237,
9.08138447606966));
#63630=CARTESIAN_POINT('Ctrl Pts',(-0.20899426636859,2.34532136525394,9.08249879665822));
#63631=CARTESIAN_POINT('Ctrl Pts',(-0.222721457706969,2.3336268914355,9.08361311724678));
#63632=CARTESIAN_POINT('Ctrl Pts',(-0.235434798931871,2.32080179996489,
9.08472743783533));
#63633=CARTESIAN_POINT('Ctrl Pts',(-0.246960173897901,2.30705518137279,
9.08584175842389));
#63634=CARTESIAN_POINT('Ctrl Pts',(-0.258246551289241,2.29359362148927,
9.08693297174532));
#63635=CARTESIAN_POINT('Ctrl Pts',(-0.268466945430599,2.27916115582596,
9.08802418506674));
#63636=CARTESIAN_POINT('Ctrl Pts',(-0.277453675406663,2.26395314461252,
9.08911539838817));
#63637=CARTESIAN_POINT('Ctrl Pts',(-0.286422256699789,2.24877584594684,
9.09020440800651));
#63638=CARTESIAN_POINT('Ctrl Pts',(-0.294161666304057,2.23282674204478,
9.09129341762485));
#63639=CARTESIAN_POINT('Ctrl Pts',(-0.300546385562578,2.21633161973544,
9.09238242724319));
#63640=CARTESIAN_POINT('Ctrl Pts',(-0.306923858795906,2.19985521775928,
9.09347020094327));
#63641=CARTESIAN_POINT('Ctrl Pts',(-0.311949384609126,2.18283474338672,
9.09455797464335));
#63642=CARTESIAN_POINT('Ctrl Pts',(-0.315545106443843,2.16551687892707,
9.09564574834343));
#63643=CARTESIAN_POINT('Ctrl Pts',(-0.319141554491157,2.14819551685222,
9.09673374173652));
#63644=CARTESIAN_POINT('Ctrl Pts',(-0.32130745995202,2.13057740961706,9.09782173512961));
#63645=CARTESIAN_POINT('Ctrl Pts',(-0.322015914725242,2.11291999569138,
9.0989097285227));
#63646=CARTESIAN_POINT('Ctrl Pts',(-0.32219236239434,2.10852224209124,9.09918070403936));
#63647=CARTESIAN_POINT('Ctrl Pts',(-0.322278655583543,2.10412206985998,
9.09945167955602));
#63648=CARTESIAN_POINT('Ctrl Pts',(-0.322274881362357,2.09972347173989,
9.09972265507268));
#63649=CARTESIAN_POINT('',(-0.322274875432262,2.10028335511254,9.34963671698665));
#63650=CARTESIAN_POINT('Ctrl Pts',(-0.322274874243154,2.09971529566301,
9.09960026516195));
#63651=CARTESIAN_POINT('Ctrl Pts',(-0.322258472261694,2.08114885383066,
9.10084055535965));
#63652=CARTESIAN_POINT('Ctrl Pts',(-0.320637716279971,2.06261890227565,
9.10210934893191));
#63653=CARTESIAN_POINT('Ctrl Pts',(-0.315899320326289,2.0355998352095,9.10394542848056));
#63654=CARTESIAN_POINT('Ctrl Pts',(-0.314008279355452,2.02693435888201,
9.10453159358843));
#63655=CARTESIAN_POINT('Ctrl Pts',(-0.310779179419296,2.01460367167756,
9.10535210223544));
#63656=CARTESIAN_POINT('Ctrl Pts',(-0.309728444291832,2.0108679328407,9.10559884178897));
#63657=CARTESIAN_POINT('Ctrl Pts',(-0.308455099497607,2.00663556387459,
9.10587556140901));
#63658=CARTESIAN_POINT('Ctrl Pts',(-0.308298464016908,2.00611963232959,
9.10590924578666));
#63659=CARTESIAN_POINT('Ctrl Pts',(-0.308060557794192,2.00534302504051,
9.10595987415689));
#63660=CARTESIAN_POINT('Ctrl Pts',(-0.307980250360868,2.00508205877742,
9.10597687419959));
#63661=CARTESIAN_POINT('Ctrl Pts',(-0.307835121556776,2.004612572932,9.10600743432248));
#63662=CARTESIAN_POINT('Ctrl Pts',(-0.307770420056702,2.00440401762833,
9.10602100140136));
#63663=CARTESIAN_POINT('Ctrl Pts',(-0.307630941685702,2.00395603998124,
9.10605012551575));
#63664=CARTESIAN_POINT('Ctrl Pts',(-0.307556097483437,2.00371663985764,
9.10606567847678));
#63665=CARTESIAN_POINT('Ctrl Pts',(-0.307353812000797,2.00307224269368,
9.10610751355303));
#63666=CARTESIAN_POINT('Ctrl Pts',(-0.307225849199085,2.00266740794239,
9.10613376498207));
#63667=CARTESIAN_POINT('Ctrl Pts',(-0.306633619003731,2.00080657897697,
9.1062542926759));
#63668=CARTESIAN_POINT('Ctrl Pts',(-0.30615978903774,1.99935361471708,9.10634801533614));
#63669=CARTESIAN_POINT('Ctrl Pts',(-0.296460502603906,1.97031391943269,
9.10821445833314));
#63670=CARTESIAN_POINT('Ctrl Pts',(-0.283550760047593,1.94409326228964,
9.10978601547487));
#63671=CARTESIAN_POINT('Ctrl Pts',(-0.263185535209028,1.91385855220464,
9.11183830144321));
#63672=CARTESIAN_POINT('Ctrl Pts',(-0.2588694193366,1.90790137640211,9.11225533826638));
#63673=CARTESIAN_POINT('Ctrl Pts',(-0.247369166838068,1.89312073824048,
9.11333196654901));
#63674=CARTESIAN_POINT('Ctrl Pts',(-0.239915280582552,1.88452111563952,
9.11399901409463));
#63675=CARTESIAN_POINT('Ctrl Pts',(-0.230394595692527,1.87464469926597,
9.11482694699622));
#63676=CARTESIAN_POINT('Ctrl Pts',(-0.228747764730766,1.87297325934145,
9.11496933821882));
#63677=CARTESIAN_POINT('Ctrl Pts',(-0.226716233923845,1.8709559172089,9.11514406507556));
#63678=CARTESIAN_POINT('Ctrl Pts',(-0.226348732561406,1.87059273366087,
9.11517563646829));
#63679=CARTESIAN_POINT('Ctrl Pts',(-0.22570160793421,1.86995628096857,9.11523116672119));
#63680=CARTESIAN_POINT('Ctrl Pts',(-0.225422357098112,1.86968263329028,
9.11525510893262));
#63681=CARTESIAN_POINT('Ctrl Pts',(-0.224857883156401,1.86913149552027,
9.11530346448591));
#63682=CARTESIAN_POINT('Ctrl Pts',(-0.224572642723948,1.86885402422718,
9.11532787858507));
#63683=CARTESIAN_POINT('Ctrl Pts',(-0.224020788283589,1.86831918645996,
9.11537507249279));
#63684=CARTESIAN_POINT('Ctrl Pts',(-0.223754242699118,1.86806174998906,
9.11539784919771));
#63685=CARTESIAN_POINT('Ctrl Pts',(-0.223121509272482,1.86745274583675,
9.11545187510309));
#63686=CARTESIAN_POINT('Ctrl Pts',(-0.222754934429039,1.86710158329928,
9.11548314180942));
#63687=CARTESIAN_POINT('Ctrl Pts',(-0.221465036704191,1.86587174938988,
9.11559304743202));
#63688=CARTESIAN_POINT('Ctrl Pts',(-0.220537341401229,1.86499769961032,
9.11567188535008));
#63689=CARTESIAN_POINT('Ctrl Pts',(-0.207067371122049,1.85245665654059,
9.11681371582356));
#63690=CARTESIAN_POINT('Ctrl Pts',(-0.1936217585474,1.84180424973892,9.11791991247994));
#63691=CARTESIAN_POINT('Ctrl Pts',(-0.169364568862311,1.82555034123905,
9.11985990927497));
#63692=CARTESIAN_POINT('Ctrl Pts',(-0.158964284120615,1.81939832252074,
9.1206757329195));
#63693=CARTESIAN_POINT('Ctrl Pts',(-0.137489862973049,1.80827341274372,
9.122312408251));
#63694=CARTESIAN_POINT('Ctrl Pts',(-0.126429791880727,1.80331262613866,
9.12313196302028));
#63695=CARTESIAN_POINT('Ctrl Pts',(-0.109233677734899,1.79673634301453,
9.12434965175588));
#63696=CARTESIAN_POINT('Ctrl Pts',(-0.10328594037938,1.79465942357064,9.12476089698939));
#63697=CARTESIAN_POINT('Ctrl Pts',(-0.0944714051371783,1.79186851352077,
9.12535225067944));
#63698=CARTESIAN_POINT('Ctrl Pts',(-0.0916498562243471,1.79101753332767,
9.12553886560109));
#63699=CARTESIAN_POINT('Ctrl Pts',(-0.0883331904049763,1.79006665826838,
9.12575478217274));
#63700=CARTESIAN_POINT('Ctrl Pts',(-0.0878491407277201,1.78992910919337,
9.12578620857896));
#63701=CARTESIAN_POINT('Ctrl Pts',(-0.087109187900887,1.78972071369493,
9.12583411661762));
#63702=CARTESIAN_POINT('Ctrl Pts',(-0.086853518855257,1.7896490496383,9.12585064568728));
#63703=CARTESIAN_POINT('Ctrl Pts',(-0.0863898251143923,1.78951969411308,
9.12588057946306));
#63704=CARTESIAN_POINT('Ctrl Pts',(-0.0861818318575394,1.78946189592036,
9.12589399036292));
#63705=CARTESIAN_POINT('Ctrl Pts',(-0.0857596294837019,1.78934502909263,
9.12592118024344));
#63706=CARTESIAN_POINT('Ctrl Pts',(-0.0855454182802888,1.78928597326381,
9.12593495843733));
#63707=CARTESIAN_POINT('Ctrl Pts',(-0.0849282911958205,1.78911652423032,
9.12597460383864));
#63708=CARTESIAN_POINT('Ctrl Pts',(-0.0845252196139656,1.78900669234538,
9.12600043830105));
#63709=CARTESIAN_POINT('Ctrl Pts',(-0.0827503053433083,1.78852675634932,
9.12611394201476));
#63710=CARTESIAN_POINT('Ctrl Pts',(-0.0813762102549527,1.78816493602542,
9.12620113708507));
#63711=CARTESIAN_POINT('Ctrl Pts',(-0.0558778029100651,1.78163083717593,
9.1278074235099));
#63712=CARTESIAN_POINT('Ctrl Pts',(-0.0311162946684242,1.77826491360616,
9.12917691824217));
#63713=CARTESIAN_POINT('Ctrl Pts',(0.00506599152502737,1.77756748815989,
9.13120182978354));
#63714=CARTESIAN_POINT('Ctrl Pts',(0.0163459817285308,1.77794227393381,
9.13183571511754));
#63715=CARTESIAN_POINT('Ctrl Pts',(0.034974104765286,1.77954247645762,9.13290912731224));
#63716=CARTESIAN_POINT('Ctrl Pts',(0.0423410168123546,1.78043241763628,
9.13334051791606));
#63717=CARTESIAN_POINT('Ctrl Pts',(0.0558401505882859,1.7825381184018,9.13414878559052));
#63718=CARTESIAN_POINT('Ctrl Pts',(0.0619803548452364,1.78367959880508,
9.13452329825408));
#63719=CARTESIAN_POINT('Ctrl Pts',(0.069003608049313,1.78519757883599,9.13496091425843));
#63720=CARTESIAN_POINT('Ctrl Pts',(0.0699231029898691,1.78540053729659,
9.13501839052465));
#63721=CARTESIAN_POINT('Ctrl Pts',(0.0712244772589702,1.78569377443052,
9.13510000107385));
#63722=CARTESIAN_POINT('Ctrl Pts',(0.0716071076670508,1.78578072668603,
9.13512402856535));
#63723=CARTESIAN_POINT('Ctrl Pts',(0.0723782086693916,1.78595743998373,
9.13517251591159));
#63724=CARTESIAN_POINT('Ctrl Pts',(0.0727666733458124,1.78604722355164,
9.13519697645204));
#63725=CARTESIAN_POINT('Ctrl Pts',(0.073514746327156,1.78622158428419,9.13524414572068));
#63726=CARTESIAN_POINT('Ctrl Pts',(0.0738743780000734,1.78630605939864,
9.13526685113204));
#63727=CARTESIAN_POINT('Ctrl Pts',(0.0747235196489008,1.78650705839744,
9.13532053089127));
#63728=CARTESIAN_POINT('Ctrl Pts',(0.0752129024647078,1.78662411049731,
9.13535152221376));
#63729=CARTESIAN_POINT('Ctrl Pts',(0.0769157755237287,1.78703562763256,
9.13545955097957));
#63730=CARTESIAN_POINT('Ctrl Pts',(0.078127815138552,1.78733599611269,9.13553677857381));
#63731=CARTESIAN_POINT('Ctrl Pts',(0.0939937055300143,1.79136590626235,
9.13655219682045));
#63732=CARTESIAN_POINT('Ctrl Pts',(0.108366944324479,1.79611465005757,9.13752377269832));
#63733=CARTESIAN_POINT('Ctrl Pts',(0.144066310137117,1.81076483023157,9.14007182548812));
#63734=CARTESIAN_POINT('Ctrl Pts',(0.164741442780121,1.82202124665936,9.1416824549965));
#63735=CARTESIAN_POINT('Ctrl Pts',(0.192777070003411,1.84151931887298,9.14396311271342));
#63736=CARTESIAN_POINT('Ctrl Pts',(0.201238381091352,1.84805074723259,9.14466494535187));
#63737=CARTESIAN_POINT('Ctrl Pts',(0.210508180778111,1.85597180381185,9.14543599351815));
#63738=CARTESIAN_POINT('Ctrl Pts',(0.211649021090287,1.85696060649992,9.14553092269137));
#63739=CARTESIAN_POINT('Ctrl Pts',(0.213089782537022,1.85822719928189,9.14565080659364));
#63740=CARTESIAN_POINT('Ctrl Pts',(0.213396156618565,1.85849757157831,9.14567629948603));
#63741=CARTESIAN_POINT('Ctrl Pts',(0.213885252529585,1.85893085162249,9.14571699501363));
#63742=CARTESIAN_POINT('Ctrl Pts',(0.214068303124133,1.85909338500652,9.14573222554726));
#63743=CARTESIAN_POINT('Ctrl Pts',(0.214415005376566,1.8594019343462,9.14576107166391));
#63744=CARTESIAN_POINT('Ctrl Pts',(0.214578691806236,1.85954790757827,9.14577469019254));
#63745=CARTESIAN_POINT('Ctrl Pts',(0.214952945883327,1.85988234854823,9.14580582698294));
#63746=CARTESIAN_POINT('Ctrl Pts',(0.215163414415457,1.86007092593606,9.14582333681536));
#63747=CARTESIAN_POINT('Ctrl Pts',(0.215809973437433,1.86065177035025,9.14587712644387));
#63748=CARTESIAN_POINT('Ctrl Pts',(0.216245244357999,1.86104495406694,9.14591333746357));
#63749=CARTESIAN_POINT('Ctrl Pts',(0.219519015664243,1.8640184489747,9.14618570482448));
#63750=CARTESIAN_POINT('Ctrl Pts',(0.222312466094142,1.86664820283091,9.14641820268445));
#63751=CARTESIAN_POINT('Ctrl Pts',(0.234991758822656,1.87901890144542,9.14747767387963));
#63752=CARTESIAN_POINT('Ctrl Pts',(0.24428982087052,1.88934307640058,9.14826699627979));
#63753=CARTESIAN_POINT('Ctrl Pts',(0.271639667051752,1.92396693480952,9.15074664319979));
#63754=CARTESIAN_POINT('Ctrl Pts',(0.286949783059319,1.95021540284296,9.15240546797203));
#63755=CARTESIAN_POINT('Ctrl Pts',(0.299200252366479,1.98022885415913,9.15435153972689));
#63756=CARTESIAN_POINT('Ctrl Pts',(0.300002762336829,1.98225340502009,9.15448293652728));
#63757=CARTESIAN_POINT('Ctrl Pts',(0.301333525877102,1.98571256229793,9.15470772923827));
#63758=CARTESIAN_POINT('Ctrl Pts',(0.301872209853844,1.98714309490997,9.15480077490439));
#63759=CARTESIAN_POINT('Ctrl Pts',(0.302604440203599,1.98913036621863,9.15493016514653));
#63760=CARTESIAN_POINT('Ctrl Pts',(0.302806672871608,1.98968390061783,9.15496621968648));
#63761=CARTESIAN_POINT('Ctrl Pts',(0.303147268688875,1.99062414435107,9.15502748782927));
#63762=CARTESIAN_POINT('Ctrl Pts',(0.303286413463739,1.99101057061216,9.15505267534497));
#63763=CARTESIAN_POINT('Ctrl Pts',(0.303559496240895,1.99177353563899,9.1551024205723));
#63764=CARTESIAN_POINT('Ctrl Pts',(0.303693473300852,1.99215005972052,9.15512697693167));
#63765=CARTESIAN_POINT('Ctrl Pts',(0.30398629062281,1.99297785456089,9.1551809804028));
#63766=CARTESIAN_POINT('Ctrl Pts',(0.304144826895351,1.99342923116603,9.155210437548));
#63767=CARTESIAN_POINT('Ctrl Pts',(0.304690396410581,1.99499368260546,9.15531257166522));
#63768=CARTESIAN_POINT('Ctrl Pts',(0.305072325606169,1.99610851600007,9.15538541751101));
#63769=CARTESIAN_POINT('Ctrl Pts',(0.308818057608964,2.0072409058005,9.15611352218554));
#63770=CARTESIAN_POINT('Ctrl Pts',(0.311692990637474,2.01741501427231,9.15678482066411));
#63771=CARTESIAN_POINT('Ctrl Pts',(0.320231424730917,2.05451065713549,9.15925675265897));
#63772=CARTESIAN_POINT('Ctrl Pts',(0.322943658201463,2.08198781363458,9.16114487968192));
#63773=CARTESIAN_POINT('Ctrl Pts',(0.321774090001628,2.12177647121397,9.16380844989872));
#63774=CARTESIAN_POINT('Ctrl Pts',(0.320707237087258,2.13405474278516,9.16461825995984));
#63775=CARTESIAN_POINT('Ctrl Pts',(0.318831436977289,2.14699216036942,9.16543887969094));
#63776=CARTESIAN_POINT('Ctrl Pts',(0.318720207620647,2.14774073337185,9.16548624343311));
#63777=CARTESIAN_POINT('Ctrl Pts',(0.318559150032686,2.14879899518658,9.16555302784647));
#63778=CARTESIAN_POINT('Ctrl Pts',(0.318511506067473,2.14910900635726,9.16557257078445));
#63779=CARTESIAN_POINT('Ctrl Pts',(0.318429016241406,2.14964058365201,9.16560604429084));
#63780=CARTESIAN_POINT('Ctrl Pts',(0.318394391586701,2.14986218343634,9.16561998747565));
#63781=CARTESIAN_POINT('Ctrl Pts',(0.318327718604069,2.15028599316591,9.16564663257866));
#63782=CARTESIAN_POINT('Ctrl Pts',(0.318295708968677,2.1504882084556,9.1656593367039));
#63783=CARTESIAN_POINT('Ctrl Pts',(0.318219956239749,2.15096382774621,9.16568919592193));
#63784=CARTESIAN_POINT('Ctrl Pts',(0.318176053374253,2.15123720667924,9.16570634188262));
#63785=CARTESIAN_POINT('Ctrl Pts',(0.318045643331123,2.15204262610709,9.16575680845929));
#63786=CARTESIAN_POINT('Ctrl Pts',(0.317958153056366,2.15257450987804,9.16579007356293));
#63787=CARTESIAN_POINT('Ctrl Pts',(0.317192129240031,2.15715957875916,9.16607631710921));
#63788=CARTESIAN_POINT('Ctrl Pts',(0.3164374213785,2.16119988968931,9.16632507234972));
#63789=CARTESIAN_POINT('Ctrl Pts',(0.313685665327031,2.17451489372656,9.16713660437448));
#63790=CARTESIAN_POINT('Ctrl Pts',(0.311356320299432,2.1837164148254,9.1676841486425));
#63791=CARTESIAN_POINT('Ctrl Pts',(0.3029051775992,2.21182156622319,9.16935176870362));
#63792=CARTESIAN_POINT('Ctrl Pts',(0.29544033066617,2.23027148417016,9.17044205494023));
#63793=CARTESIAN_POINT('Ctrl Pts',(0.278694809583666,2.2626859020224,9.17251158505862));
#63794=CARTESIAN_POINT('Ctrl Pts',(0.269935118322576,2.27684008111278,9.17347644893916));
#63795=CARTESIAN_POINT('Ctrl Pts',(0.25950999006673,2.29109375160174,9.17454748352658));
#63796=CARTESIAN_POINT('Ctrl Pts',(0.258892082961262,2.29193005545316,9.17461070311868));
#63797=CARTESIAN_POINT('Ctrl Pts',(0.257768441672667,2.29343554393617,9.17472520379362));
#63798=CARTESIAN_POINT('Ctrl Pts',(0.257264119796638,2.29410577483576,9.17477642965546));
#63799=CARTESIAN_POINT('Ctrl Pts',(0.25647837765781,2.29514156461832,9.17485598881477));
#63800=CARTESIAN_POINT('Ctrl Pts',(0.256198776730041,2.29550850428091,9.17488425053767));
#63801=CARTESIAN_POINT('Ctrl Pts',(0.255704063766449,2.29615486674713,9.17493417014095));
#63802=CARTESIAN_POINT('Ctrl Pts',(0.255489278707218,2.29643453983288,9.17495581508745));
#63803=CARTESIAN_POINT('Ctrl Pts',(0.255037786703901,2.29702043747325,9.17500125543092));
#63804=CARTESIAN_POINT('Ctrl Pts',(0.254800986398235,2.29732658907866,9.17502505450536));
#63805=CARTESIAN_POINT('Ctrl Pts',(0.254140555110172,2.29817726874747,9.17509133671047));
#63806=CARTESIAN_POINT('Ctrl Pts',(0.253715728087504,2.29872086178636,9.17513386732795));
#63807=CARTESIAN_POINT('Ctrl Pts',(0.252013409770457,2.30088472863147,9.17530387418962));
#63808=CARTESIAN_POINT('Ctrl Pts',(0.250722138563106,2.30249405378318,9.17543190033613));
#63809=CARTESIAN_POINT('Ctrl Pts',(0.225741065353069,2.3330229474704,9.17789154864242));
#63810=CARTESIAN_POINT('Ctrl Pts',(0.197215876685887,2.35761022942843,9.18045858130194));
#63811=CARTESIAN_POINT('Ctrl Pts',(0.155819778857383,2.38230998972758,9.18367961993618));
#63812=CARTESIAN_POINT('Ctrl Pts',(0.146233287374389,2.38739278366106,9.18439249788832));
#63813=CARTESIAN_POINT('Ctrl Pts',(0.135028488436193,2.39262740921821,9.18517464453166));
#63814=CARTESIAN_POINT('Ctrl Pts',(0.133644607389639,2.39326202012556,9.18527038102681));
#63815=CARTESIAN_POINT('Ctrl Pts',(0.131882530920689,2.3940549976001,9.18539113833416));
#63816=CARTESIAN_POINT('Ctrl Pts',(0.131508489727078,2.39422246805738,9.18541670681925));
#63817=CARTESIAN_POINT('Ctrl Pts',(0.130910268484528,2.39448894255419,9.1854574946429));
#63818=CARTESIAN_POINT('Ctrl Pts',(0.130686294764353,2.39458840446138,9.1854727421011));
#63819=CARTESIAN_POINT('Ctrl Pts',(0.130261711679657,2.39477637315822,9.18550160166721));
#63820=CARTESIAN_POINT('Ctrl Pts',(0.130061127108632,2.3948649299553,9.18551521676232));
#63821=CARTESIAN_POINT('Ctrl Pts',(0.129602255386049,2.39506695953797,9.18554632054076));
#63822=CARTESIAN_POINT('Ctrl Pts',(0.129343909918394,2.39518029775141,9.18556380085897));
#63823=CARTESIAN_POINT('Ctrl Pts',(0.12855019057871,2.39552726665042,9.18561741132981));
#63824=CARTESIAN_POINT('Ctrl Pts',(0.128014326303372,2.39575978277213,9.18565347337094));
#63825=CARTESIAN_POINT('Ctrl Pts',(0.124003881406022,2.39748700784234,9.18592239976159));
#63826=CARTESIAN_POINT('Ctrl Pts',(0.120503679033797,2.39892197780236,9.18615170846144));
#63827=CARTESIAN_POINT('Ctrl Pts',(0.115912166306965,2.40071058474788,9.18644653887563));
#63828=CARTESIAN_POINT('Ctrl Pts',(0.114843269962672,2.40112042357502,9.18651475786318));
#63829=CARTESIAN_POINT('Ctrl Pts',(0.111695483025373,2.40230815645427,9.18671449541018));
#63830=CARTESIAN_POINT('Ctrl Pts',(0.109610678126212,2.40307029234126,9.18684530227731));
#63831=CARTESIAN_POINT('Ctrl Pts',(0.106453792041393,2.40418750869589,9.18704138283768));
#63832=CARTESIAN_POINT('Ctrl Pts',(0.105387484032473,2.40455857983375,9.18710727305348));
#63833=CARTESIAN_POINT('Ctrl Pts',(0.0755785433885693,2.41475667998751,
9.18894033688237));
#63834=CARTESIAN_POINT('Ctrl Pts',(0.0455907947716183,2.42047729148712,
9.19056806203115));
#63835=CARTESIAN_POINT('Ctrl Pts',(0.00435261472609193,2.42242999542373,
9.19294955545122));
#63836=CARTESIAN_POINT('Ctrl Pts',(-0.00655612161160735,2.42239265856827,
9.19359116068032));
#63837=CARTESIAN_POINT('Ctrl Pts',(-0.019419547863179,2.42169548033113,
9.19437034970359));
#63838=CARTESIAN_POINT('Ctrl Pts',(-0.0213968101145816,2.42157001904668,
9.19449074248126));
#63839=CARTESIAN_POINT('Ctrl Pts',(-0.0240249457020883,2.4213789122036,
9.19465163356744));
#63840=CARTESIAN_POINT('Ctrl Pts',(-0.0246769854787377,2.42132950316289,
9.19469162167063));
#63841=CARTESIAN_POINT('Ctrl Pts',(-0.0257496132859311,2.42124493952232,
9.19475752200417));
#63842=CARTESIAN_POINT('Ctrl Pts',(-0.0261702928103834,2.42121094241107,
9.19478339781715));
#63843=CARTESIAN_POINT('Ctrl Pts',(-0.0269870214463744,2.42114332358624,
9.19483369320375));
#63844=CARTESIAN_POINT('Ctrl Pts',(-0.0273830777037293,2.42110979534076,
9.19485810979491));
#63845=CARTESIAN_POINT('Ctrl Pts',(-0.0282998566475121,2.42103047672796,
9.19491469119259));
#63846=CARTESIAN_POINT('Ctrl Pts',(-0.0288205309150977,2.42098415204973,
9.19494687274844));
#63847=CARTESIAN_POINT('Ctrl Pts',(-0.0302219295388583,2.42085603152695,
9.19503361677299));
#63848=CARTESIAN_POINT('Ctrl Pts',(-0.0311024289517391,2.42077187669837,
9.19508825333711));
#63849=CARTESIAN_POINT('Ctrl Pts',(-0.0374699062007123,2.42013683352641,
9.19548435933184));
#63850=CARTESIAN_POINT('Ctrl Pts',(-0.0429420022529031,2.41944884476655,
9.19583012526517));
#63851=CARTESIAN_POINT('Ctrl Pts',(-0.079632879734054,2.4138760775783,9.198186634193));
#63852=CARTESIAN_POINT('Ctrl Pts',(-0.110000398399723,2.40456307509838,
9.20034825134858));
#63853=CARTESIAN_POINT('Ctrl Pts',(-0.146611337647609,2.38713520403494,
9.20307014969199));
#63854=CARTESIAN_POINT('Ctrl Pts',(-0.154540518051768,2.38294657077944,
9.20366555098833));
#63855=CARTESIAN_POINT('Ctrl Pts',(-0.166278561583133,2.37610501471716,
9.20454577493825));
#63856=CARTESIAN_POINT('Ctrl Pts',(-0.170221572836756,2.37369172581329,
9.20484122222881));
#63857=CARTESIAN_POINT('Ctrl Pts',(-0.174750431413928,2.37078411838863,
9.20517907187464));
#63858=CARTESIAN_POINT('Ctrl Pts',(-0.175387877025763,2.37037167875161,
9.20522658963348));
#63859=CARTESIAN_POINT('Ctrl Pts',(-0.176286943228662,2.36978544791447,
9.20529355297633));
#63860=CARTESIAN_POINT('Ctrl Pts',(-0.176549770130788,2.36961352512085,
9.20531312170985));
#63861=CARTESIAN_POINT('Ctrl Pts',(-0.176999929400635,2.36931812222151,
9.20534662586448));
#63862=CARTESIAN_POINT('Ctrl Pts',(-0.177187384547364,2.36919483041682,
9.20536057396056));
#63863=CARTESIAN_POINT('Ctrl Pts',(-0.177545574537902,2.36895870773709,
9.20538721874755));
#63864=CARTESIAN_POINT('Ctrl Pts',(-0.177716330449988,2.3688459101373,9.20539991766426));
#63865=CARTESIAN_POINT('Ctrl Pts',(-0.178117578729359,2.36858030502818,
9.20542975089488));
#63866=CARTESIAN_POINT('Ctrl Pts',(-0.178347982535267,2.36842736303955,
9.20544687611678));
#63867=CARTESIAN_POINT('Ctrl Pts',(-0.17902580915851,2.36797616390847,9.20549724149264));
#63868=CARTESIAN_POINT('Ctrl Pts',(-0.179472685500309,2.36767708145655,
9.2055304264486));
#63869=CARTESIAN_POINT('Ctrl Pts',(-0.183299289330032,2.36510214667537,
9.20581443808981));
#63870=CARTESIAN_POINT('Ctrl Pts',(-0.1866365124877,2.36276337949726,9.20606111391321));
#63871=CARTESIAN_POINT('Ctrl Pts',(-0.200885109389166,2.35236931701582,
9.20711408268274));
#63872=CARTESIAN_POINT('Ctrl Pts',(-0.211327327125846,2.34369230024236,
9.20788545526469));
#63873=CARTESIAN_POINT('Ctrl Pts',(-0.233930133501104,2.32236144585911,
9.20963225194391));
#63874=CARTESIAN_POINT('Ctrl Pts',(-0.245666306574055,2.30932266259556,
9.21059983675026));
#63875=CARTESIAN_POINT('Ctrl Pts',(-0.260673406462534,2.28963897554837,
9.21201086642339));
#63876=CARTESIAN_POINT('Ctrl Pts',(-0.264866489011503,2.28373703940968,
9.21242806451234));
#63877=CARTESIAN_POINT('Ctrl Pts',(-0.273055988707078,2.27134640569059,
9.21329791751021));
#63878=CARTESIAN_POINT('Ctrl Pts',(-0.277028051356033,2.2648472274589,9.21375101322573));
#63879=CARTESIAN_POINT('Ctrl Pts',(-0.281547667589517,2.25682672479033,
9.21430919151071));
#63880=CARTESIAN_POINT('Ctrl Pts',(-0.282319022907817,2.25543384411447,
9.21440608928429));
#63881=CARTESIAN_POINT('Ctrl Pts',(-0.283367011184956,2.2535078927868,9.21454003921946));
#63882=CARTESIAN_POINT('Ctrl Pts',(-0.283652531725253,2.25297966339973,
9.21457677430012));
#63883=CARTESIAN_POINT('Ctrl Pts',(-0.284130772403353,2.25208894875669,
9.21463871371018));
#63884=CARTESIAN_POINT('Ctrl Pts',(-0.284324279963388,2.25172688615163,
9.21466388999783));
#63885=CARTESIAN_POINT('Ctrl Pts',(-0.284704868607723,2.25101150039954,
9.21471363297264));
#63886=CARTESIAN_POINT('Ctrl Pts',(-0.284891985112615,2.25065819685023,
9.21473819834659));
#63887=CARTESIAN_POINT('Ctrl Pts',(-0.285301828758954,2.24988085783625,
9.21479224555848));
#63888=CARTESIAN_POINT('Ctrl Pts',(-0.285524268684286,2.24945667274259,
9.21482173749133));
#63889=CARTESIAN_POINT('Ctrl Pts',(-0.286271431098901,2.24802410457041,
9.21492133603052));
#63890=CARTESIAN_POINT('Ctrl Pts',(-0.286791759242231,2.24701345031991,
9.21499159737818));
#63891=CARTESIAN_POINT('Ctrl Pts',(-0.291672960867762,2.23740796174153,
9.21565937862092));
#63892=CARTESIAN_POINT('Ctrl Pts',(-0.295651150585205,2.22862515004463,
9.21627020420648));
#63893=CARTESIAN_POINT('Ctrl Pts',(-0.307746451678849,2.1983834054305,9.21837722942361));
#63894=CARTESIAN_POINT('Ctrl Pts',(-0.313964835083191,2.17624290408021,
9.21993178354173));
#63895=CARTESIAN_POINT('Ctrl Pts',(-0.320771365033645,2.13591432430947,
9.22269576647163));
#63896=CARTESIAN_POINT('Ctrl Pts',(-0.322275132160368,2.11797292193138,
9.22390021191208));
#63897=CARTESIAN_POINT('Ctrl Pts',(-0.322274995589501,2.09939897745547,
9.22506493325287));
#63898=CARTESIAN_POINT('Ctrl Pts',(-0.322273323115425,2.09880032001375,
9.22510238362959));
#63899=CARTESIAN_POINT('Ctrl Pts',(-0.322268353573463,2.09790975499496,
9.22515795787839));
#63900=CARTESIAN_POINT('Ctrl Pts',(-0.322266328030864,2.09761784587171,
9.22517615208023));
#63901=CARTESIAN_POINT('Ctrl Pts',(-0.32226217452405,2.09711728694944,9.22520731303542));
#63902=CARTESIAN_POINT('Ctrl Pts',(-0.322260240543767,2.09690863642755,
9.22522029068208));
#63903=CARTESIAN_POINT('Ctrl Pts',(-0.322255836046731,2.09647852146802,
9.22524701940766));
#63904=CARTESIAN_POINT('Ctrl Pts',(-0.322253339880275,2.09625705818156,
9.22526076893302));
#63905=CARTESIAN_POINT('Ctrl Pts',(-0.322246953047899,2.09573789786962,
9.22529297097684));
#63906=CARTESIAN_POINT('Ctrl Pts',(-0.322242878138978,2.09544020245614,
9.22531141309229));
#63907=CARTESIAN_POINT('Ctrl Pts',(-0.32222835038992,2.09447645366835,9.22537104343758));
#63908=CARTESIAN_POINT('Ctrl Pts',(-0.322216244926181,2.09381042138694,
9.2254121393879));
#63909=CARTESIAN_POINT('Ctrl Pts',(-0.321797515193333,2.07413073331827,
9.22662319427765));
#63910=CARTESIAN_POINT('Ctrl Pts',(-0.31971061374058,2.05518676054616,9.22770078146485));
#63911=CARTESIAN_POINT('Ctrl Pts',(-0.313474902300085,2.0241419544787,9.22947603343592));
#63912=CARTESIAN_POINT('Ctrl Pts',(-0.310258700092123,2.01190634070192,
9.23017811048497));
#63913=CARTESIAN_POINT('Ctrl Pts',(-0.300543368385666,1.98217746120095,
9.23194451258543));
#63914=CARTESIAN_POINT('Ctrl Pts',(-0.293229940625628,1.96500180125661,
9.2330210443297));
#63915=CARTESIAN_POINT('Ctrl Pts',(-0.283869100244403,1.94741831888985,
9.23423099464817));
#63916=CARTESIAN_POINT('Ctrl Pts',(-0.283256865453793,1.94628473211179,
9.23430948825398));
#63917=CARTESIAN_POINT('Ctrl Pts',(-0.282392824214243,1.94470760309457,
9.23441939069695));
#63918=CARTESIAN_POINT('Ctrl Pts',(-0.282146731438201,1.94426093091856,
9.23445059552838));
#63919=CARTESIAN_POINT('Ctrl Pts',(-0.281719695425607,1.94349017089206,
9.23450457781423));
#63920=CARTESIAN_POINT('Ctrl Pts',(-0.281539250083858,1.94316580711323,
9.23452733740783));
#63921=CARTESIAN_POINT('Ctrl Pts',(-0.281164377597431,1.94249467804651,
9.23457451562032));
#63922=CARTESIAN_POINT('Ctrl Pts',(-0.280969868441365,1.94214795947072,
9.23459893715711));
#63923=CARTESIAN_POINT('Ctrl Pts',(-0.280513368757434,1.94133775170132,
9.23465611875502));
#63924=CARTESIAN_POINT('Ctrl Pts',(-0.280250870814821,1.94087455109586,
9.23468889704213));
#63925=CARTESIAN_POINT('Ctrl Pts',(-0.279401386990875,1.93938418447322,
9.23479464539101));
#63926=CARTESIAN_POINT('Ctrl Pts',(-0.278809897653228,1.93835960851158,
9.23486777792404));
#63927=CARTESIAN_POINT('Ctrl Pts',(-0.269436192681703,1.92232703934681,
9.23601906333756));
#63928=CARTESIAN_POINT('Ctrl Pts',(-0.25946065184863,1.908053307656,9.23714183366535));
#63929=CARTESIAN_POINT('Ctrl Pts',(-0.230326005810092,1.87281209831388,
9.24018053548816));
#63930=CARTESIAN_POINT('Ctrl Pts',(-0.209466684786698,1.85344772086862,
9.24214545802994));
#63931=CARTESIAN_POINT('Ctrl Pts',(-0.185590656364188,1.83652677909995,
9.24404169192221));
#63932=CARTESIAN_POINT('Ctrl Pts',(-0.184834272856886,1.83599560329842,
9.24410142186924));
#63933=CARTESIAN_POINT('Ctrl Pts',(-0.18081665974169,1.83319993516573,9.24441683493926));
#63934=CARTESIAN_POINT('Ctrl Pts',(-0.177515896862501,1.83099247415949,
9.24466954884462));
#63935=CARTESIAN_POINT('Ctrl Pts',(-0.173676495061207,1.828526241167,9.24495544707642));
#63936=CARTESIAN_POINT('Ctrl Pts',(-0.173177101425418,1.82820739850611,
9.24499247981865));
#63937=CARTESIAN_POINT('Ctrl Pts',(-0.172437237377411,1.82773789226243,
9.24504711367425));
#63938=CARTESIAN_POINT('Ctrl Pts',(-0.172197446318721,1.82758616843696,
9.24506478481674));
#63939=CARTESIAN_POINT('Ctrl Pts',(-0.171771842888959,1.82731766140926,
9.24509608536871));
#63940=CARTESIAN_POINT('Ctrl Pts',(-0.171586111620487,1.82720075130444,
9.24510972324946));
#63941=CARTESIAN_POINT('Ctrl Pts',(-0.171193504358359,1.8269541809532,9.24513850604796));
#63942=CARTESIAN_POINT('Ctrl Pts',(-0.17098660097096,1.82682456639958,9.24515364789954));
#63943=CARTESIAN_POINT('Ctrl Pts',(-0.170435471189059,1.82648018279805,
9.24519391104559));
#63944=CARTESIAN_POINT('Ctrl Pts',(-0.170090984759505,1.82626582758185,
9.24521900484957));
#63945=CARTESIAN_POINT('Ctrl Pts',(-0.168488331055755,1.82527277662101,
9.24533541492642));
#63946=CARTESIAN_POINT('Ctrl Pts',(-0.167225189226694,1.82450208484835,
9.24542621008789));
#63947=CARTESIAN_POINT('Ctrl Pts',(-0.15711931551246,1.81843121450526,9.24614542535052));
#63948=CARTESIAN_POINT('Ctrl Pts',(-0.148031211999004,1.81354883950229,
9.24674858908856));
#63949=CARTESIAN_POINT('Ctrl Pts',(-0.116389496695447,1.79845908535726,
9.24875690034716));
#63950=CARTESIAN_POINT('Ctrl Pts',(-0.0929026318538538,1.79041536118521,
9.25010214219421));
#63951=CARTESIAN_POINT('Ctrl Pts',(-0.0683257705576937,1.78505090526437,
9.25154099103011));
#63952=CARTESIAN_POINT('Ctrl Pts',(-0.0679256660838118,1.78496437172494,
9.25156442123641));
#63953=CARTESIAN_POINT('Ctrl Pts',(-0.061523656446614,1.78359252501878,
9.25193943147789));
#63954=CARTESIAN_POINT('Ctrl Pts',(-0.0554866577776933,1.78247822843998,
9.25229460043902));
#63955=CARTESIAN_POINT('Ctrl Pts',(-0.0477416910453507,1.78127629969844,
9.25275431304524));
#63956=CARTESIAN_POINT('Ctrl Pts',(-0.0460596181757361,1.78102887650557,
9.25285439507981));
#63957=CARTESIAN_POINT('Ctrl Pts',(-0.0380615186182831,1.77991698628041,
9.25333155553501));
#63958=CARTESIAN_POINT('Ctrl Pts',(-0.0317230610866462,1.77922678774512,
9.25371352670742));
#63959=CARTESIAN_POINT('Ctrl Pts',(-0.0243446696689885,1.77864417276754,
9.25416401019866));
#63960=CARTESIAN_POINT('Ctrl Pts',(-0.0233203476112143,1.77856821565604,
9.25422667886042));
#63961=CARTESIAN_POINT('Ctrl Pts',(-0.0217944049762667,1.77846239406403,
9.25432023516853));
#63962=CARTESIAN_POINT('Ctrl Pts',(-0.021293042442949,1.77842880343801,
9.25435100579226));
#63963=CARTESIAN_POINT('Ctrl Pts',(-0.0203991847801133,1.7783710157292,
9.25440592290483));
#63964=CARTESIAN_POINT('Ctrl Pts',(-0.0200067192086265,1.77834636416311,
9.25443005507973));
#63965=CARTESIAN_POINT('Ctrl Pts',(-0.0191796630295581,1.77829593461542,
9.25448095165898));
#63966=CARTESIAN_POINT('Ctrl Pts',(-0.0187450636472245,1.77827031883149,
9.25450772110336));
#63967=CARTESIAN_POINT('Ctrl Pts',(-0.0175979326795973,1.77820503784865,
9.25457844457243));
#63968=CARTESIAN_POINT('Ctrl Pts',(-0.0168853218916665,1.7781668587729,
9.25462244512944));
#63969=CARTESIAN_POINT('Ctrl Pts',(-0.0136670870658746,1.77800515567262,
9.25482146104727));
#63970=CARTESIAN_POINT('Ctrl Pts',(-0.0111602539462873,1.77790852665464,
9.25497731715918));
#63971=CARTESIAN_POINT('Ctrl Pts',(-0.00016948184314906,1.77761333437575,
9.25566445474171));
#63972=CARTESIAN_POINT('Ctrl Pts',(0.00831861923177028,1.7777206648977,
9.25620520749217));
#63973=CARTESIAN_POINT('Ctrl Pts',(0.0310260047299391,1.778905432777,9.25767980904175));
#63974=CARTESIAN_POINT('Ctrl Pts',(0.0451936281512032,1.7805914925298,9.25863004311568));
#63975=CARTESIAN_POINT('Ctrl Pts',(0.0837792052296277,1.78780236500515,
9.26127765193915));
#63976=CARTESIAN_POINT('Ctrl Pts',(0.107740338692095,1.79524019021462,9.26299382321312));
#63977=CARTESIAN_POINT('Ctrl Pts',(0.131907595360206,1.80595306161003,9.264664710065));
#63978=CARTESIAN_POINT('Ctrl Pts',(0.133209530231184,1.80654057022214,9.26475450708809));
#63979=CARTESIAN_POINT('Ctrl Pts',(0.134887948594719,1.8073114416635,9.2648699489321));
#63980=CARTESIAN_POINT('Ctrl Pts',(0.135268014536934,1.80748689754962,9.26489606846483));
#63981=CARTESIAN_POINT('Ctrl Pts',(0.135849454124314,1.80775669231238,9.26493599302665));
#63982=CARTESIAN_POINT('Ctrl Pts',(0.136051071946451,1.80785049906427,9.26494983082696));
#63983=CARTESIAN_POINT('Ctrl Pts',(0.136448215969172,1.80803577859409,9.26497707569316));
#63984=CARTESIAN_POINT('Ctrl Pts',(0.13664374621373,1.80812723860632,9.26499048337205));
#63985=CARTESIAN_POINT('Ctrl Pts',(0.13707934540302,1.80833152544253,9.26502033930313));
#63986=CARTESIAN_POINT('Ctrl Pts',(0.137319366378446,1.80844445193851,9.26503678122364));
#63987=CARTESIAN_POINT('Ctrl Pts',(0.138013191676665,1.80877193384008,9.26508428410554));
#63988=CARTESIAN_POINT('Ctrl Pts',(0.138466637084566,1.80898725454274,9.26511529768147));
#63989=CARTESIAN_POINT('Ctrl Pts',(0.141503895057553,1.81043821699306,9.26532283186054));
#63990=CARTESIAN_POINT('Ctrl Pts',(0.144071744119346,1.81170724531417,9.26549731831639));
#63991=CARTESIAN_POINT('Ctrl Pts',(0.152078489829783,1.81579787629006,9.26603936614333));
#63992=CARTESIAN_POINT('Ctrl Pts',(0.157454315306971,1.81874057722857,9.26640035519251));
#63993=CARTESIAN_POINT('Ctrl Pts',(0.169999682119959,1.82608037282053,9.2672434206219));
#63994=CARTESIAN_POINT('Ctrl Pts',(0.177087536894045,1.83060832828774,9.26772029051195));
#63995=CARTESIAN_POINT('Ctrl Pts',(0.210408630096527,1.85377900994109,9.27000322078026));
#63996=CARTESIAN_POINT('Ctrl Pts',(0.233923402722349,1.87599943669894,9.27176448193724));
#63997=CARTESIAN_POINT('Ctrl Pts',(0.255014094907295,1.90293873792034,9.27383266479325));
#63998=CARTESIAN_POINT('Ctrl Pts',(0.256255225133291,1.90455540705853,9.27395645884159));
#63999=CARTESIAN_POINT('Ctrl Pts',(0.257893769093772,1.90673217869587,9.27412276002631));
#64000=CARTESIAN_POINT('Ctrl Pts',(0.258304866384437,1.90728196016027,9.2741647300531));
#64001=CARTESIAN_POINT('Ctrl Pts',(0.258944579696721,1.90814320563806,9.27423042857951));
#64002=CARTESIAN_POINT('Ctrl Pts',(0.259174399218538,1.90845377663665,9.27425411010876));
#64003=CARTESIAN_POINT('Ctrl Pts',(0.259612977163245,1.90904869169004,9.27429945494492));
#64004=CARTESIAN_POINT('Ctrl Pts',(0.259821828450057,1.9093329668869,9.27432111459966));
#64005=CARTESIAN_POINT('Ctrl Pts',(0.26030346127108,1.90999079593874,9.27437121813774));
#64006=CARTESIAN_POINT('Ctrl Pts',(0.260575905662381,1.9103645946496,9.27439967503089));
#64007=CARTESIAN_POINT('Ctrl Pts',(0.261342808765185,1.91142157292852,9.2744801044996));
#64008=CARTESIAN_POINT('Ctrl Pts',(0.261835389186077,1.91210610494704,9.27453214946206));
#64009=CARTESIAN_POINT('Ctrl Pts',(0.262933666079342,1.91364507039714,9.27464906316954));
#64010=CARTESIAN_POINT('Ctrl Pts',(0.263537893544775,1.91450053593183,9.27471398770104));
#64011=CARTESIAN_POINT('Ctrl Pts',(0.268324825427074,1.92134847207295,9.27523321509284));
#64012=CARTESIAN_POINT('Ctrl Pts',(0.272306476642403,1.92747826475906,9.27569509443316));
#64013=CARTESIAN_POINT('Ctrl Pts',(0.279091136079439,1.93874409255423,9.27653971044202));
#64014=CARTESIAN_POINT('Ctrl Pts',(0.281969262502211,1.94383131420171,9.2769196055743));
#64015=CARTESIAN_POINT('Ctrl Pts',(0.294778660739563,1.9679821666332,9.27871532824959));
#64016=CARTESIAN_POINT('Ctrl Pts',(0.302924371818978,1.98792935304771,9.28018121119283));
#64017=CARTESIAN_POINT('Ctrl Pts',(0.313265455631432,2.02286806746097,9.28263504820887));
#64018=CARTESIAN_POINT('Ctrl Pts',(0.316505846438503,2.03748000787696,9.28362822331295));
#64019=CARTESIAN_POINT('Ctrl Pts',(0.31885555975502,2.05316900972577,9.28462593138143));
#64020=CARTESIAN_POINT('Ctrl Pts',(0.318986988108309,2.05407276295913,9.28468316228142));
#64021=CARTESIAN_POINT('Ctrl Pts',(0.319158515719454,2.05528852051733,9.28475981570073));
#64022=CARTESIAN_POINT('Ctrl Pts',(0.319202000828369,2.05560003127266,9.28477942685575));
#64023=CARTESIAN_POINT('Ctrl Pts',(0.319274426982014,2.05612447065233,9.28481239258689));
#64024=CARTESIAN_POINT('Ctrl Pts',(0.319303611114518,2.05633736459992,9.2848257609291));
#64025=CARTESIAN_POINT('Ctrl Pts',(0.319359160928617,2.0567456265861,9.284851370135));
#64026=CARTESIAN_POINT('Ctrl Pts',(0.319385560086513,2.05694098820292,9.28486361279413));
#64027=CARTESIAN_POINT('Ctrl Pts',(0.319447597797777,2.05740328172236,9.28489255524443));
#64028=CARTESIAN_POINT('Ctrl Pts',(0.3194830809984,2.05767023383205,9.28490924610476));
#64029=CARTESIAN_POINT('Ctrl Pts',(0.31958624767971,2.05845391109278,9.28495818083918));
#64030=CARTESIAN_POINT('Ctrl Pts',(0.319653012868413,2.05897075941926,9.28499037280276));
#64031=CARTESIAN_POINT('Ctrl Pts',(0.320134106178299,2.06276750054387,9.28522627128089));
#64032=CARTESIAN_POINT('Ctrl Pts',(0.320499216787296,2.06605358546599,9.28542725350824));
#64033=CARTESIAN_POINT('Ctrl Pts',(0.321542105045374,2.07696767212112,9.28608594554629));
#64034=CARTESIAN_POINT('Ctrl Pts',(0.321998636700488,2.08461463118804,9.28653321635976));
#64035=CARTESIAN_POINT('Ctrl Pts',(0.32281194090703,2.11851775518767,9.28848131290178));
#64036=CARTESIAN_POINT('Ctrl Pts',(0.320232143351835,2.14474342978141,9.289903849634));
#64037=CARTESIAN_POINT('Ctrl Pts',(0.313498370728776,2.17483952120189,9.29167315690037));
#64038=CARTESIAN_POINT('Ctrl Pts',(0.312402362596835,2.17929025021266,9.29193816881204));
#64039=CARTESIAN_POINT('Ctrl Pts',(0.308875290159987,2.1924020465289,9.29273095220771));
#64040=CARTESIAN_POINT('Ctrl Pts',(0.306176306637433,2.20098578759863,9.29326585016435));
#64041=CARTESIAN_POINT('Ctrl Pts',(0.302737869754027,2.21050899426926,9.29388163263373));
#64042=CARTESIAN_POINT('Ctrl Pts',(0.302348062437887,2.21157107459621,9.29395062413024));
#64043=CARTESIAN_POINT('Ctrl Pts',(0.301771951168544,2.21311557149981,9.29405142182942));
#64044=CARTESIAN_POINT('Ctrl Pts',(0.30159006267522,2.21359963520379,9.29408308039754));
#64045=CARTESIAN_POINT('Ctrl Pts',(0.301266638796291,2.21445411838799,9.29413908496814));
#64046=CARTESIAN_POINT('Ctrl Pts',(0.301125582968606,2.21482471923403,9.2941634148633));
#64047=CARTESIAN_POINT('Ctrl Pts',(0.300832179275959,2.21559133,9.294213825944));
#64048=CARTESIAN_POINT('Ctrl Pts',(0.300679732678443,2.21598730108409,9.29423991040554));
#64049=CARTESIAN_POINT('Ctrl Pts',(0.300291471339335,2.21698987753377,9.29430607214552));
#64050=CARTESIAN_POINT('Ctrl Pts',(0.300054601022688,2.21759606966093,9.29434618485862));
#64051=CARTESIAN_POINT('Ctrl Pts',(0.299094119402971,2.22003231259936,9.29450783752528));
#64052=CARTESIAN_POINT('Ctrl Pts',(0.29835560073337,2.22185640551228,9.29462987915179));
#64053=CARTESIAN_POINT('Ctrl Pts',(0.296449994918476,2.22644193688992,9.29493927411264));
#64054=CARTESIAN_POINT('Ctrl Pts',(0.295261015388246,2.22919401962474,9.29512736259417));
#64055=CARTESIAN_POINT('Ctrl Pts',(0.290314085929752,2.24021937595996,9.29589079442097));
#64056=CARTESIAN_POINT('Ctrl Pts',(0.286245693683029,2.24834796629056,9.29647654477005));
#64057=CARTESIAN_POINT('Ctrl Pts',(0.273670845445757,2.2710238720236,9.29817669186159));
#64058=CARTESIAN_POINT('Ctrl Pts',(0.264360406265617,2.2850901847439,9.2993142090678));
#64059=CARTESIAN_POINT('Ctrl Pts',(0.244245175457211,2.31084676501312,9.30152571400347));
#64060=CARTESIAN_POINT('Ctrl Pts',(0.233587958237221,2.3225956243493,9.30259608444995));
#64061=CARTESIAN_POINT('Ctrl Pts',(0.221974953148232,2.33364145628118,9.30363371413978));
#64062=CARTESIAN_POINT('Ctrl Pts',(0.221840661888979,2.333768968538,9.3036456968559));
#64063=CARTESIAN_POINT('Ctrl Pts',(0.221528606161668,2.33406476068633,9.30367350341307));
#64064=CARTESIAN_POINT('Ctrl Pts',(0.221350759492087,2.33423295416334,9.30368932237285));
#64065=CARTESIAN_POINT('Ctrl Pts',(0.218048943265193,2.33734843510757,9.30398247804967));
#64066=CARTESIAN_POINT('Ctrl Pts',(0.214866364296733,2.34023336833978,9.30425623660791));
#64067=CARTESIAN_POINT('Ctrl Pts',(0.2112152517576,2.34341238863278,9.30455959725218));
#64068=CARTESIAN_POINT('Ctrl Pts',(0.210802711185122,2.34376974890723,9.30459372343867));
#64069=CARTESIAN_POINT('Ctrl Pts',(0.210178204231378,2.34430795263381,9.30464515417546));
#64070=CARTESIAN_POINT('Ctrl Pts',(0.209966910505311,2.34448956981505,9.3046625155429));
#64071=CARTESIAN_POINT('Ctrl Pts',(0.209599612816335,2.34480445263217,9.30469262628015));
#64072=CARTESIAN_POINT('Ctrl Pts',(0.20944371707812,2.34493784333649,9.30470538494806));
#64073=CARTESIAN_POINT('Ctrl Pts',(0.209117432923521,2.34521648599239,9.30473204320171));
#64074=CARTESIAN_POINT('Ctrl Pts',(0.20894702061857,2.34536170917635,9.30474594059635));
#64075=CARTESIAN_POINT('Ctrl Pts',(0.208539108955493,2.34570859312132,9.30477914533061));
#64076=CARTESIAN_POINT('Ctrl Pts',(0.208301467405451,2.34591008799214,9.30479844034362));
#64077=CARTESIAN_POINT('Ctrl Pts',(0.207494996909642,2.34659188172576,9.30486375485412));
#64078=CARTESIAN_POINT('Ctrl Pts',(0.206924790565097,2.34707055864894,9.30490965572031));
#64079=CARTESIAN_POINT('Ctrl Pts',(0.205564284719224,2.3482046627318,9.30501852679852));
#64080=CARTESIAN_POINT('Ctrl Pts',(0.204772496335225,2.34885830217888,9.30508137128727));
#64081=CARTESIAN_POINT('Ctrl Pts',(0.201911848269049,2.35119693548841,9.30530662675852));
#64082=CARTESIAN_POINT('Ctrl Pts',(0.199825143401271,2.35286005607218,9.30546758454704));
#64083=CARTESIAN_POINT('Ctrl Pts',(0.188523108315542,2.36164056856456,9.30632301050846));
#64084=CARTESIAN_POINT('Ctrl Pts',(0.178946949472971,2.36828117997872,9.30699046576959));
#64085=CARTESIAN_POINT('Ctrl Pts',(0.153545734144269,2.38392903426079,9.30867549964184));
#64086=CARTESIAN_POINT('Ctrl Pts',(0.137280313603271,2.39214057659763,9.30967751877737));
#64087=CARTESIAN_POINT('Ctrl Pts',(0.104939158971385,2.40516731135652,9.3116568457012));
#64088=CARTESIAN_POINT('Ctrl Pts',(0.0890112943534987,2.41018733778611,
9.31262622861209));
#64089=CARTESIAN_POINT('Ctrl Pts',(0.071531320563508,2.41423885390322,9.3137162631697));
#64090=CARTESIAN_POINT('Ctrl Pts',(0.0702929871033947,2.41451817597141,
9.31379361161546));
#64091=CARTESIAN_POINT('Ctrl Pts',(0.0685580627147062,2.4148987527181,9.31390216612746));
#64092=CARTESIAN_POINT('Ctrl Pts',(0.0680628229743746,2.41500616589321,
9.31393317475301));
#64093=CARTESIAN_POINT('Ctrl Pts',(0.0672052247278319,2.41519005464356,
9.31398690962972));
#64094=CARTESIAN_POINT('Ctrl Pts',(0.0668429829217559,2.4152670747306,9.31400961840719));
#64095=CARTESIAN_POINT('Ctrl Pts',(0.0660910884008059,2.41542558889517,
9.31405677884015));
#64096=CARTESIAN_POINT('Ctrl Pts',(0.0657014159944474,2.41550698570709,
9.31408123356577));
#64097=CARTESIAN_POINT('Ctrl Pts',(0.0649284619885563,2.41566695032384,
9.31412976937126));
#64098=CARTESIAN_POINT('Ctrl Pts',(0.0645451861255913,2.41574554256365,
9.31415384962059));
#64099=CARTESIAN_POINT('Ctrl Pts',(0.0633313427595625,2.41599214344634,
9.31423015514773));
#64100=CARTESIAN_POINT('Ctrl Pts',(0.0625002603399509,2.41615757326218,
9.31428246272126));
#64101=CARTESIAN_POINT('Ctrl Pts',(0.0569298591988327,2.41724355838911,
9.31463349473452));
#64102=CARTESIAN_POINT('Ctrl Pts',(0.052171237743816,2.41806075218673,9.31493549621284));
#64103=CARTESIAN_POINT('Ctrl Pts',(0.0378364111312539,2.42019211830719,
9.3158522360954));
#64104=CARTESIAN_POINT('Ctrl Pts',(0.0282183395614718,2.42118262937666,
9.31647681062151));
#64105=CARTESIAN_POINT('Ctrl Pts',(0.00680963320186511,2.4224183556767,
9.31788709111213));
#64106=CARTESIAN_POINT('Ctrl Pts',(-0.00497935150054212,2.42245176032486,
9.31867721899912));
#64107=CARTESIAN_POINT('Ctrl Pts',(-0.0361772342734136,2.42082876753904,
9.32078753453597));
#64108=CARTESIAN_POINT('Ctrl Pts',(-0.05548104489608,2.41805947824297,9.32211492148567));
#64109=CARTESIAN_POINT('Ctrl Pts',(-0.0745369065890626,2.41353698369352,
9.32338709907955));
#64110=CARTESIAN_POINT('Ctrl Pts',(-0.0746559061223345,2.41350867016502,
9.32339504190501));
#64111=CARTESIAN_POINT('Ctrl Pts',(-0.0755791648016716,2.41328844398702,
9.32345665353613));
#64112=CARTESIAN_POINT('Ctrl Pts',(-0.0763827067508067,2.41309350268692,
9.32351020056131));
#64113=CARTESIAN_POINT('Ctrl Pts',(-0.0809182204460799,2.41197467574403,
9.32381198128239));
#64114=CARTESIAN_POINT('Ctrl Pts',(-0.0846343706815731,2.41098711092148,
9.32405748337377));
#64115=CARTESIAN_POINT('Ctrl Pts',(-0.0892476148320064,2.4096723187868,
9.32435929202675));
#64116=CARTESIAN_POINT('Ctrl Pts',(-0.0901619332109386,2.40940734902357,
9.32441896255034));
#64117=CARTESIAN_POINT('Ctrl Pts',(-0.0914160792180088,2.40903786573837,
9.32450059703569));
#64118=CARTESIAN_POINT('Ctrl Pts',(-0.0917569162566877,2.40893683872547,
9.32452276094028));
#64119=CARTESIAN_POINT('Ctrl Pts',(-0.0922985492737435,2.40877531864463,
9.32455794679089));
#64120=CARTESIAN_POINT('Ctrl Pts',(-0.0924994533216363,2.40871519356512,
9.32457099027684));
#64121=CARTESIAN_POINT('Ctrl Pts',(-0.0928907080424122,2.40859768552311,
9.32459637678469));
#64122=CARTESIAN_POINT('Ctrl Pts',(-0.093081063727561,2.40854032269113,
9.32460872089945));
#64123=CARTESIAN_POINT('Ctrl Pts',(-0.0935409338230394,2.4084012785868,
9.32463852545799));
#64124=CARTESIAN_POINT('Ctrl Pts',(-0.0938103951527391,2.40831941991576,
9.3246559754266));
#64125=CARTESIAN_POINT('Ctrl Pts',(-0.0946360549059517,2.40806741314544,
9.32470940201458));
#64126=CARTESIAN_POINT('Ctrl Pts',(-0.0951919041861844,2.40789611124561,
9.32474531120143));
#64127=CARTESIAN_POINT('Ctrl Pts',(-0.0994105648733737,2.40658348613522,
9.3250174229573));
#64128=CARTESIAN_POINT('Ctrl Pts',(-0.103053390348468,2.40537828390361,
9.32524996335253));
#64129=CARTESIAN_POINT('Ctrl Pts',(-0.116655505600875,2.40060698203345,
9.32611212822289));
#64130=CARTESIAN_POINT('Ctrl Pts',(-0.126459525647403,2.39661607235071,
9.32672117577617));
#64131=CARTESIAN_POINT('Ctrl Pts',(-0.143342881597667,2.38875371715189,
9.32777668239566));
#64132=CARTESIAN_POINT('Ctrl Pts',(-0.150505935692425,2.38508570667653,
9.32822673572628));
#64133=CARTESIAN_POINT('Ctrl Pts',(-0.165369889900727,2.37675774494261,
9.32917918994205));
#64134=CARTESIAN_POINT('Ctrl Pts',(-0.17302788853198,2.37203565120332,9.3296811195897));
#64135=CARTESIAN_POINT('Ctrl Pts',(-0.196184954583837,2.35638264124531,
9.33125854023691));
#64136=CARTESIAN_POINT('Ctrl Pts',(-0.21092179052807,2.34440219363547,9.33235257380039));
#64137=CARTESIAN_POINT('Ctrl Pts',(-0.225445235354195,2.33029825732799,
9.33358223559826));
#64138=CARTESIAN_POINT('Ctrl Pts',(-0.226365735707659,2.32939353760302,
9.33366086982803));
#64139=CARTESIAN_POINT('Ctrl Pts',(-0.227642606261134,2.32812338749328,
9.33377093771352));
#64140=CARTESIAN_POINT('Ctrl Pts',(-0.228003589057303,2.32776259455633,
9.33380216654944));
#64141=CARTESIAN_POINT('Ctrl Pts',(-0.228625691729252,2.32713785804182,
9.33385617913084));
#64142=CARTESIAN_POINT('Ctrl Pts',(-0.228887216089035,2.32687431715301,
9.33387894496799));
#64143=CARTESIAN_POINT('Ctrl Pts',(-0.229427781996047,2.32632769709366,
9.33392612550393));
#64144=CARTESIAN_POINT('Ctrl Pts',(-0.229706756302274,2.32604455253384,
9.33395054310217));
#64145=CARTESIAN_POINT('Ctrl Pts',(-0.230258513828674,2.32548247082932,
9.33399897328838));
#64146=CARTESIAN_POINT('Ctrl Pts',(-0.230531315783888,2.32520355299751,
9.33402298498937));
#64147=CARTESIAN_POINT('Ctrl Pts',(-0.23116260062137,2.32455576651155,9.33407870519483));
#64148=CARTESIAN_POINT('Ctrl Pts',(-0.231520707502572,2.32418653436863,
9.3341104300423));
#64149=CARTESIAN_POINT('Ctrl Pts',(-0.233483254752722,2.32215329958119,
9.33428493742793));
#64150=CARTESIAN_POINT('Ctrl Pts',(-0.23507060760306,2.32047296378069,9.33442845856515));
#64151=CARTESIAN_POINT('Ctrl Pts',(-0.245360785143318,2.30934254884466,
9.33537479751482));
#64152=CARTESIAN_POINT('Ctrl Pts',(-0.253508896483958,2.29939755197797,
9.33620084103928));
#64153=CARTESIAN_POINT('Ctrl Pts',(-0.265659212282505,2.28261536638295,
9.33756489605877));
#64154=CARTESIAN_POINT('Ctrl Pts',(-0.270041747005516,2.27606996439986,
9.33809007366851));
#64155=CARTESIAN_POINT('Ctrl Pts',(-0.287328519772448,2.24808590209848,
9.34030086907598));
#64156=CARTESIAN_POINT('Ctrl Pts',(-0.29795412321071,2.22534175292491,9.3420235074827));
#64157=CARTESIAN_POINT('Ctrl Pts',(-0.306915483240647,2.19836493000829,
9.34384834081225));
#64158=CARTESIAN_POINT('Ctrl Pts',(-0.307937833344241,2.1951160679989,9.34406456008923));
#64159=CARTESIAN_POINT('Ctrl Pts',(-0.309069832391499,2.19130900610683,
9.34431331829989));
#64160=CARTESIAN_POINT('Ctrl Pts',(-0.30922969742782,2.19076612876508,9.3443486819231));
#64161=CARTESIAN_POINT('Ctrl Pts',(-0.309466095826875,2.18995548182837,
9.34440132338054));
#64162=CARTESIAN_POINT('Ctrl Pts',(-0.309543712374288,2.18968803324999,
9.34441866409503));
#64163=CARTESIAN_POINT('Ctrl Pts',(-0.309681708947806,2.18921021616435,
9.34444959641043));
#64164=CARTESIAN_POINT('Ctrl Pts',(-0.309742221283587,2.1889998869678,9.3444631957585));
#64165=CARTESIAN_POINT('Ctrl Pts',(-0.30987062967239,2.18855184699738,9.34449212927638));
#64166=CARTESIAN_POINT('Ctrl Pts',(-0.309938466280587,2.18831412039325,
9.34450745990819));
#64167=CARTESIAN_POINT('Ctrl Pts',(-0.310120658846409,2.18767284930989,
9.34454875775674));
#64168=CARTESIAN_POINT('Ctrl Pts',(-0.310234501148351,2.1872691575037,9.34457469493356));
#64169=CARTESIAN_POINT('Ctrl Pts',(-0.310483049340056,2.18638115763045,
9.34463161812143));
#64170=CARTESIAN_POINT('Ctrl Pts',(-0.31061741116021,2.18589675321653,9.34466258437064));
#64171=CARTESIAN_POINT('Ctrl Pts',(-0.311018160631981,2.18443872498491,
9.34475553976064));
#64172=CARTESIAN_POINT('Ctrl Pts',(-0.311281110982906,2.18346415114804,
9.34481733646845));
#64173=CARTESIAN_POINT('Ctrl Pts',(-0.318641213874295,2.15566673697281,
9.34657079076452));
#64174=CARTESIAN_POINT('Ctrl Pts',(-0.322250473770379,2.12803666604931,
9.34807817638457));
#64175=CARTESIAN_POINT('Ctrl Pts',(-0.322274875432262,2.10028335511254,
9.34963671698665));
#64176=CARTESIAN_POINT('',(-0.322274971935003,2.09977570497444,9.59989500205939));
#64177=CARTESIAN_POINT('Ctrl Pts',(-0.322274875630863,2.10028312914261,
9.34963672967643));
#64178=CARTESIAN_POINT('Ctrl Pts',(-0.322293905266275,2.07862243632518,
9.3508531277297));
#64179=CARTESIAN_POINT('Ctrl Pts',(-0.320129274946486,2.05701771372018,
9.35209326684815));
#64180=CARTESIAN_POINT('Ctrl Pts',(-0.315652217724324,2.03499602690769,
9.35345949425794));
#64181=CARTESIAN_POINT('Ctrl Pts',(-0.315486918798168,2.034198456551,9.35350910970234));
#64182=CARTESIAN_POINT('Ctrl Pts',(-0.315212577168667,2.032899552619,9.35359013421058));
#64183=CARTESIAN_POINT('Ctrl Pts',(-0.315105357043244,2.03239783434005,
9.35362148504255));
#64184=CARTESIAN_POINT('Ctrl Pts',(-0.314914592177069,2.0315154973075,9.35367671559367));
#64185=CARTESIAN_POINT('Ctrl Pts',(-0.31483155408659,2.0311347691182,9.35370057906101));
#64186=CARTESIAN_POINT('Ctrl Pts',(-0.314662472793085,2.03036623204061,
9.35374881383568));
#64187=CARTESIAN_POINT('Ctrl Pts',(-0.314576402694029,2.02997842982138,
9.35377318596776));
#64188=CARTESIAN_POINT('Ctrl Pts',(-0.314408409264114,2.0292280707614,9.35382040786416));
#64189=CARTESIAN_POINT('Ctrl Pts',(-0.314326575223432,2.02886549437401,
9.35384325472771));
#64190=CARTESIAN_POINT('Ctrl Pts',(-0.314130533897973,2.02800385142772,
9.35389761854134));
#64191=CARTESIAN_POINT('Ctrl Pts',(-0.314015764540868,2.02750491498554,
9.35392915351871));
#64192=CARTESIAN_POINT('Ctrl Pts',(-0.313605343649847,2.02573995497256,
9.35404090461757));
#64193=CARTESIAN_POINT('Ctrl Pts',(-0.313303223653341,2.02447546211863,
9.35412132864826));
#64194=CARTESIAN_POINT('Ctrl Pts',(-0.307952360392867,2.00266471442149,
9.35551487286207));
#64195=CARTESIAN_POINT('Ctrl Pts',(-0.300901130828245,1.98266710950557,
9.35689523677099));
#64196=CARTESIAN_POINT('Ctrl Pts',(-0.289453561004378,1.9581818922806,9.35870888205722));
#64197=CARTESIAN_POINT('Ctrl Pts',(-0.28681837249172,1.95292533082108,9.35910565754199));
#64198=CARTESIAN_POINT('Ctrl Pts',(-0.281420778202499,1.94285586478276,
9.35987829670385));
#64199=CARTESIAN_POINT('Ctrl Pts',(-0.278674879403395,1.93803628365411,
9.36025394585873));
#64200=CARTESIAN_POINT('Ctrl Pts',(-0.267994925262872,1.92036731081013,
9.36164885612311));
#64201=CARTESIAN_POINT('Ctrl Pts',(-0.259284420180758,1.90800815028088,
9.36266124421665));
#64202=CARTESIAN_POINT('Ctrl Pts',(-0.247935542658628,1.89409400626534,
9.36380890890688));
#64203=CARTESIAN_POINT('Ctrl Pts',(-0.246103352304488,1.89190758561332,
9.36398946988456));
#64204=CARTESIAN_POINT('Ctrl Pts',(-0.243915170828827,1.88936568066,9.36419935710503));
#64205=CARTESIAN_POINT('Ctrl Pts',(-0.243587153879473,1.88898643285974,
9.36423067107927));
#64206=CARTESIAN_POINT('Ctrl Pts',(-0.243084334672872,1.88840781639797,
9.36427844326892));
#64207=CARTESIAN_POINT('Ctrl Pts',(-0.242910171154434,1.88820789751323,
9.36429494850975));
#64208=CARTESIAN_POINT('Ctrl Pts',(-0.242593768694897,1.8878456090236,9.36432485743772));
#64209=CARTESIAN_POINT('Ctrl Pts',(-0.242451613928936,1.88768316806204,
9.36433826726574));
#64210=CARTESIAN_POINT('Ctrl Pts',(-0.242162633106145,1.88735361692522,
9.36436547120151));
#64211=CARTESIAN_POINT('Ctrl Pts',(-0.24201579787261,1.88718651666657,9.36437926449163));
#64212=CARTESIAN_POINT('Ctrl Pts',(-0.24159189763467,1.88670511921467,9.36441900023277));
#64213=CARTESIAN_POINT('Ctrl Pts',(-0.241314391261022,1.88639120863836,
9.36444490970192));
#64214=CARTESIAN_POINT('Ctrl Pts',(-0.240085975021403,1.8850070936514,9.36455914951093));
#64215=CARTESIAN_POINT('Ctrl Pts',(-0.239128533454196,1.88394266999483,
9.36464699809856));
#64216=CARTESIAN_POINT('Ctrl Pts',(-0.221286845089395,1.86437128628977,
9.36626294318893));
#64217=CARTESIAN_POINT('Ctrl Pts',(-0.202305480853914,1.84788555396402,
9.36763976992079));
#64218=CARTESIAN_POINT('Ctrl Pts',(-0.174643391834059,1.829016924532,9.36951361341396));
#64219=CARTESIAN_POINT('Ctrl Pts',(-0.16750083080066,1.82454472941497,9.36998666544951));
#64220=CARTESIAN_POINT('Ctrl Pts',(-0.150794226285885,1.81497445123109,
9.37108238757193));
#64221=CARTESIAN_POINT('Ctrl Pts',(-0.141132380713601,1.81006883346267,
9.37170862185046));
#64222=CARTESIAN_POINT('Ctrl Pts',(-0.12789411421198,1.8041660731153,9.37256890132675));
#64223=CARTESIAN_POINT('Ctrl Pts',(-0.124520554091748,1.80273034677676,
9.37278828283996));
#64224=CARTESIAN_POINT('Ctrl Pts',(-0.118990523464957,1.80048751599635,
9.37314853488349));
#64225=CARTESIAN_POINT('Ctrl Pts',(-0.11684855208458,1.79964539590766,9.37328822471829));
#64226=CARTESIAN_POINT('Ctrl Pts',(-0.114217583312692,1.79864342826637,
9.37346004808157));
#64227=CARTESIAN_POINT('Ctrl Pts',(-0.113736945508574,1.79846169913854,
9.37349144742457));
#64228=CARTESIAN_POINT('Ctrl Pts',(-0.112890786752646,1.79814407747496,
9.37354674381974));
#64229=CARTESIAN_POINT('Ctrl Pts',(-0.112525449031058,1.7980076970926,9.37357062453296));
#64230=CARTESIAN_POINT('Ctrl Pts',(-0.111787317701912,1.79773367844616,
9.37361888568023));
#64231=CARTESIAN_POINT('Ctrl Pts',(-0.1114145153072,1.79759606596267,9.37364326692416));
#64232=CARTESIAN_POINT('Ctrl Pts',(-0.110692761408097,1.79733116089089,
9.37369048223614));
#64233=CARTESIAN_POINT('Ctrl Pts',(-0.110343842296186,1.79720378129619,
9.37371331335844));
#64234=CARTESIAN_POINT('Ctrl Pts',(-0.10951438989669,1.79690259791433,9.37376760157657));
#64235=CARTESIAN_POINT('Ctrl Pts',(-0.109033663008653,1.79672933364461,
9.37379907658278));
#64236=CARTESIAN_POINT('Ctrl Pts',(-0.107333800319685,1.79612123089425,
9.373910413615));
#64237=CARTESIAN_POINT('Ctrl Pts',(-0.106112471378754,1.7956925989336,9.37399048153383));
#64238=CARTESIAN_POINT('Ctrl Pts',(-0.0863832012927313,1.78890171922341,
9.37528517247159));
#64239=CARTESIAN_POINT('Ctrl Pts',(-0.06733963026167,1.78423217539372,9.3765568498142));
#64240=CARTESIAN_POINT('Ctrl Pts',(-0.0299072985257442,1.77859487964436,
9.37908804780099));
#64241=CARTESIAN_POINT('Ctrl Pts',(-0.0116230347082161,1.7774157926223,
9.38033772504611));
#64242=CARTESIAN_POINT('Ctrl Pts',(0.0155271427417528,1.77797716614114,
9.38215476398131));
#64243=CARTESIAN_POINT('Ctrl Pts',(0.0243815822328268,1.77852626540802,
9.3827407513187));
#64244=CARTESIAN_POINT('Ctrl Pts',(0.0369409743264621,1.77982713385704,
9.38355290669376));
#64245=CARTESIAN_POINT('Ctrl Pts',(0.040672336647712,1.78027970992947,9.3837917723761));
#64246=CARTESIAN_POINT('Ctrl Pts',(0.0449276023634252,1.78087153810816,
9.38406075141584));
#64247=CARTESIAN_POINT('Ctrl Pts',(0.0454598999144294,1.78094692893927,
9.38409433692993));
#64248=CARTESIAN_POINT('Ctrl Pts',(0.0462619371237329,1.78106257169552,
9.38414484651368));
#64249=CARTESIAN_POINT('Ctrl Pts',(0.0465318150575613,1.78110183414029,
9.38416182624261));
#64250=CARTESIAN_POINT('Ctrl Pts',(0.0470176651122379,1.78117314657818,
9.38419236444613));
#64251=CARTESIAN_POINT('Ctrl Pts',(0.0472336540090899,1.78120507340084,
9.38420592987459));
#64252=CARTESIAN_POINT('Ctrl Pts',(0.0476658017074738,1.78126940098881,
9.38423305013833));
#64253=CARTESIAN_POINT('Ctrl Pts',(0.0478819590347595,1.78130180201619,
9.38424660489682));
#64254=CARTESIAN_POINT('Ctrl Pts',(0.0484933628282909,1.78139408481404,
9.38428491510517));
#64255=CARTESIAN_POINT('Ctrl Pts',(0.0488885328371591,1.78145448238752,
9.38430964122306));
#64256=CARTESIAN_POINT('Ctrl Pts',(0.0505383924314835,1.78170978849045,
9.38441273191768));
#64257=CARTESIAN_POINT('Ctrl Pts',(0.051792058816934,1.78191137929603,9.3844907225774));
#64258=CARTESIAN_POINT('Ctrl Pts',(0.0746908074174633,1.78573249007612,
9.38590949672349));
#64259=CARTESIAN_POINT('Ctrl Pts',(0.0959154033819419,1.7915468504694,9.38713257838033));
#64260=CARTESIAN_POINT('Ctrl Pts',(0.130295122235821,1.80486137051123,9.38919335073471));
#64261=CARTESIAN_POINT('Ctrl Pts',(0.143812240678983,1.81120658492307,9.3900260020898));
#64262=CARTESIAN_POINT('Ctrl Pts',(0.163894937197353,1.82239447007665,9.39134817235584));
#64263=CARTESIAN_POINT('Ctrl Pts',(0.170798485187874,1.82658777726573,9.39181924967101));
#64264=CARTESIAN_POINT('Ctrl Pts',(0.181845376726697,1.83387956672711,9.39260641226734));
#64265=CARTESIAN_POINT('Ctrl Pts',(0.186084659846815,1.8368264436245,9.39291698534842));
#64266=CARTESIAN_POINT('Ctrl Pts',(0.190972236384032,1.84040111974668,9.39328590247239));
#64267=CARTESIAN_POINT('Ctrl Pts',(0.191691107200913,1.84093148957632,9.39334044458028));
#64268=CARTESIAN_POINT('Ctrl Pts',(0.192719321851519,1.84169671034368,9.39341886565087));
#64269=CARTESIAN_POINT('Ctrl Pts',(0.193030465322343,1.84192914554809,9.39344265027479));
#64270=CARTESIAN_POINT('Ctrl Pts',(0.193658455124436,1.84240004727871,9.39349076508444));
#64271=CARTESIAN_POINT('Ctrl Pts',(0.19397528293384,1.84263853728334,9.39351509616395));
#64272=CARTESIAN_POINT('Ctrl Pts',(0.194589183397091,1.84310242432811,9.39356235161898));
#64273=CARTESIAN_POINT('Ctrl Pts',(0.194886306763208,1.84332775351507,9.39358527330334));
#64274=CARTESIAN_POINT('Ctrl Pts',(0.195594072083972,1.84386643833788,9.39363999482435));
#64275=CARTESIAN_POINT('Ctrl Pts',(0.196004352103471,1.84418026582054,9.39367181324343));
#64276=CARTESIAN_POINT('Ctrl Pts',(0.197240675919896,1.8451306629686,9.39376798911634));
#64277=CARTESIAN_POINT('Ctrl Pts',(0.198064380009028,1.84577025247464,9.39383246606994));
#64278=CARTESIAN_POINT('Ctrl Pts',(0.206653357776954,1.8525064969228,9.39450901333605));
#64279=CARTESIAN_POINT('Ctrl Pts',(0.214136917744299,1.85895230666839,9.39513508877155));
#64280=CARTESIAN_POINT('Ctrl Pts',(0.226309182941974,1.87045135245252,9.3962193882094));
#64281=CARTESIAN_POINT('Ctrl Pts',(0.231153482423853,1.87533027437389,9.39667052080783));
#64282=CARTESIAN_POINT('Ctrl Pts',(0.251870509400426,1.89757513541451,9.39868675085785));
#64283=CARTESIAN_POINT('Ctrl Pts',(0.265968746776228,1.91649225684921,9.40030348969872));
#64284=CARTESIAN_POINT('Ctrl Pts',(0.28154240915932,1.94300550062641,9.40234695746611));
#64285=CARTESIAN_POINT('Ctrl Pts',(0.284992248894844,1.94935858864712,9.40282102421913));
#64286=CARTESIAN_POINT('Ctrl Pts',(0.289678059808428,1.95872602710037,9.40349242003798));
#64287=CARTESIAN_POINT('Ctrl Pts',(0.291086465160418,1.96165121774778,9.40369829552711));
#64288=CARTESIAN_POINT('Ctrl Pts',(0.292670774985091,1.96507310134358,9.40393434035085));
#64289=CARTESIAN_POINT('Ctrl Pts',(0.292889896592284,1.96554941801986,9.40396709036049));
#64290=CARTESIAN_POINT('Ctrl Pts',(0.293220081670156,1.96627179726101,9.4040165948859));
#64291=CARTESIAN_POINT('Ctrl Pts',(0.293331998618923,1.96651746522499,9.40403340180831));
#64292=CARTESIAN_POINT('Ctrl Pts',(0.293525139910082,1.96694284401612,9.40406245337255));
#64293=CARTESIAN_POINT('Ctrl Pts',(0.293606507841787,1.96712248846603,9.40407470691692));
#64294=CARTESIAN_POINT('Ctrl Pts',(0.293776057526267,1.96749773705492,9.40410027039347));
#64295=CARTESIAN_POINT('Ctrl Pts',(0.293864208569767,1.96769335397047,9.40411357839707));
#64296=CARTESIAN_POINT('Ctrl Pts',(0.294080627217723,1.96817489418025,9.40414629355887));
#64297=CARTESIAN_POINT('Ctrl Pts',(0.294208673588825,1.96846091753322,9.40416568704251));
#64298=CARTESIAN_POINT('Ctrl Pts',(0.294704994718336,1.96957392424243,9.4042410051272));
#64299=CARTESIAN_POINT('Ctrl Pts',(0.295070206078204,1.97040228134483,9.40429674323942));
#64300=CARTESIAN_POINT('Ctrl Pts',(0.301844110849039,1.98594364649578,9.40533674853517));
#64301=CARTESIAN_POINT('Ctrl Pts',(0.307149481955308,2.00111587611416,9.40625645772988));
#64302=CARTESIAN_POINT('Ctrl Pts',(0.315761891685831,2.0332715556909,9.4081320705102));
#64303=CARTESIAN_POINT('Ctrl Pts',(0.318878263655718,2.05025149494832,9.40908340975898));
#64304=CARTESIAN_POINT('Ctrl Pts',(0.322160179407236,2.08252846682303,9.41092520354666));
#64305=CARTESIAN_POINT('Ctrl Pts',(0.322625578948256,2.09774571043346,9.41180714661301));
#64306=CARTESIAN_POINT('Ctrl Pts',(0.321950901364855,2.11453816428942,9.4128210172081));
#64307=CARTESIAN_POINT('Ctrl Pts',(0.321874671138459,2.11613806208383,9.41291800755346));
#64308=CARTESIAN_POINT('Ctrl Pts',(0.321720838577729,2.1189288608512,9.41308791065645));
#64309=CARTESIAN_POINT('Ctrl Pts',(0.321648541136978,2.12012003163019,9.41316065695271));
#64310=CARTESIAN_POINT('Ctrl Pts',(0.321534375178657,2.12184274369171,9.41326620421207));
#64311=CARTESIAN_POINT('Ctrl Pts',(0.321497800229628,2.12237463554175,9.4132988389927));
#64312=CARTESIAN_POINT('Ctrl Pts',(0.321431507998527,2.12330495479299,9.41335600245721));
#64313=CARTESIAN_POINT('Ctrl Pts',(0.321402369269883,2.12370342332857,9.41338051292542));
#64314=CARTESIAN_POINT('Ctrl Pts',(0.321344946620158,2.12446909365008,9.41342766205336));
#64315=CARTESIAN_POINT('Ctrl Pts',(0.321316774063191,2.12483630339331,9.41345029717843));
#64316=CARTESIAN_POINT('Ctrl Pts',(0.321248967248624,2.1257006891357,9.41350363260593));
#64317=CARTESIAN_POINT('Ctrl Pts',(0.321208808255606,2.12619782194969,9.41353434935725));
#64318=CARTESIAN_POINT('Ctrl Pts',(0.321086918148299,2.12766428944318,9.41362508429229));
#64319=CARTESIAN_POINT('Ctrl Pts',(0.321001952555254,2.12863334313052,9.41368520403908));
#64320=CARTESIAN_POINT('Ctrl Pts',(0.320214261455708,2.13717263423444,9.41421642369828));
#64321=CARTESIAN_POINT('Ctrl Pts',(0.319248297052032,2.14471562345521,9.41469576945104));
#64322=CARTESIAN_POINT('Ctrl Pts',(0.317395269729055,2.15600111193666,9.41542908976962));
#64323=CARTESIAN_POINT('Ctrl Pts',(0.316706449256916,2.15977378095019,9.41567696340226));
#64324=CARTESIAN_POINT('Ctrl Pts',(0.310558210433744,2.19034898985035,9.41770786880935));
#64325=CARTESIAN_POINT('Ctrl Pts',(0.301773983632801,2.21636767891518,9.41958800651799));
#64326=CARTESIAN_POINT('Ctrl Pts',(0.288278933120266,2.24411362657803,9.42164917565765));
#64327=CARTESIAN_POINT('Ctrl Pts',(0.286693197301422,2.24724297138602,9.42188230031728));
#64328=CARTESIAN_POINT('Ctrl Pts',(0.281510629397849,2.25706914932774,9.4226151341318));
#64329=CARTESIAN_POINT('Ctrl Pts',(0.277727524980031,2.26366549782313,9.42310834655076));
#64330=CARTESIAN_POINT('Ctrl Pts',(0.273066095713724,2.27116539070468,9.423665364877));
#64331=CARTESIAN_POINT('Ctrl Pts',(0.272411892341,2.27220465914063,9.42374246436211));
#64332=CARTESIAN_POINT('Ctrl Pts',(0.271545457693763,2.27356378454799,9.42384315163782));
#64333=CARTESIAN_POINT('Ctrl Pts',(0.27133858407659,2.27388701991723,9.42386708714367));
#64334=CARTESIAN_POINT('Ctrl Pts',(0.271001814037888,2.27441115114478,9.42390588079707));
#64335=CARTESIAN_POINT('Ctrl Pts',(0.27087227120859,2.27461227203914,9.42392076244257));
#64336=CARTESIAN_POINT('Ctrl Pts',(0.27062269629981,2.27499880187041,9.42394935449233));
#64337=CARTESIAN_POINT('Ctrl Pts',(0.270502697916237,2.27518423110806,9.42396306702688));
#64338=CARTESIAN_POINT('Ctrl Pts',(0.270225331889106,2.27561187049936,9.42399468238821));
#64339=CARTESIAN_POINT('Ctrl Pts',(0.270067828685458,2.27585399331703,9.42401257610559));
#64340=CARTESIAN_POINT('Ctrl Pts',(0.269562871587066,2.27662796344427,9.42406975576439));
#64341=CARTESIAN_POINT('Ctrl Pts',(0.269214167780233,2.27715899946471,9.42410895845359));
#64342=CARTESIAN_POINT('Ctrl Pts',(0.266061789665223,2.2819289099315,9.42446085589621));
#64343=CARTESIAN_POINT('Ctrl Pts',(0.263159592701876,2.28610223000424,9.42476708997274));
#64344=CARTESIAN_POINT('Ctrl Pts',(0.260036684061468,2.29037369043887,9.42508074119694));
#64345=CARTESIAN_POINT('Ctrl Pts',(0.259913504681772,2.29054183045582,9.42509308798623));
#64346=CARTESIAN_POINT('Ctrl Pts',(0.25932147906525,2.29134830390119,9.42515231092131));
#64347=CARTESIAN_POINT('Ctrl Pts',(0.258850440098123,2.29198503221156,9.42519907565717));
#64348=CARTESIAN_POINT('Ctrl Pts',(0.256999955442098,2.29446723923914,9.42538143701996));
#64349=CARTESIAN_POINT('Ctrl Pts',(0.255603054913416,2.296299676604,9.42551618059549));
#64350=CARTESIAN_POINT('Ctrl Pts',(0.240165254001852,2.31610656686588,9.42697581477699));
#64351=CARTESIAN_POINT('Ctrl Pts',(0.224272862623354,2.33255804960562,9.4282212133178));
#64352=CARTESIAN_POINT('Ctrl Pts',(0.19938621607212,2.35337544520435,9.43005147965133));
#64353=CARTESIAN_POINT('Ctrl Pts',(0.191724027836489,2.35922163952094,9.43060068106986));
#64354=CARTESIAN_POINT('Ctrl Pts',(0.176489233658036,2.36980029911379,9.43168014871905));
#64355=CARTESIAN_POINT('Ctrl Pts',(0.168959322308485,2.37457854332827,9.43220827828904));
#64356=CARTESIAN_POINT('Ctrl Pts',(0.160226663581501,2.37962468730197,9.43281917128163));
#64357=CARTESIAN_POINT('Ctrl Pts',(0.159208622307278,2.38020557453047,9.43289036182301));
#64358=CARTESIAN_POINT('Ctrl Pts',(0.157380071232551,2.38123575084875,9.43301819428699));
#64359=CARTESIAN_POINT('Ctrl Pts',(0.156570745881377,2.38168712409802,9.4330747609426));
#64360=CARTESIAN_POINT('Ctrl Pts',(0.155339561859942,2.38236682920168,9.43316079802449));
#64361=CARTESIAN_POINT('Ctrl Pts',(0.154919116873706,2.38259772280643,9.43319017677444));
#64362=CARTESIAN_POINT('Ctrl Pts',(0.154186809634179,2.38299775480658,9.43324134312015));
#64363=CARTESIAN_POINT('Ctrl Pts',(0.15387517986218,2.38316731893261,9.4332631154851));
#64364=CARTESIAN_POINT('Ctrl Pts',(0.153230812612084,2.38351655452129,9.43330813269705));
#64365=CARTESIAN_POINT('Ctrl Pts',(0.152898037736114,2.38369615555367,9.43333138000991));
#64366=CARTESIAN_POINT('Ctrl Pts',(0.152092765056396,2.38412893868529,9.43338763297719));
#64367=CARTESIAN_POINT('Ctrl Pts',(0.151619951357845,2.38438152775036,9.43342065963198));
#64368=CARTESIAN_POINT('Ctrl Pts',(0.149867663437279,2.38531203218161,9.43354305305116));
#64369=CARTESIAN_POINT('Ctrl Pts',(0.148584269826922,2.38598249404803,9.43363268317355));
#64370=CARTESIAN_POINT('Ctrl Pts',(0.125575466630344,2.39780590928345,9.43523950744023));
#64371=CARTESIAN_POINT('Ctrl Pts',(0.102661022236782,2.40646010635937,9.43684794922477));
#64372=CARTESIAN_POINT('Ctrl Pts',(0.0629198669896975,2.4165077838812,9.43961400874966));
#64373=CARTESIAN_POINT('Ctrl Pts',(0.046555244213754,2.41932542191676,9.44074413869801));
#64374=CARTESIAN_POINT('Ctrl Pts',(0.0237242275602795,2.42146330071826,
9.44226132629087));
#64375=CARTESIAN_POINT('Ctrl Pts',(0.0173857367668061,2.42186835842644,
9.44267607759508));
#64376=CARTESIAN_POINT('Ctrl Pts',(0.00806040830968497,2.42218796979088,
9.44327301086615));
#64377=CARTESIAN_POINT('Ctrl Pts',(0.00508041032992029,2.42224873785607,
9.44346177771094));
#64378=CARTESIAN_POINT('Ctrl Pts',(0.00159514308373494,2.42227144754737,
9.44367989290862));
#64379=CARTESIAN_POINT('Ctrl Pts',(0.00109040439749176,2.42227355059362,
9.44371141530839));
#64380=CARTESIAN_POINT('Ctrl Pts',(0.000319813198342206,2.42227495096366,
9.44375943930489));
#64381=CARTESIAN_POINT('Ctrl Pts',(5.39659598036372E-5,2.42227510513226,
9.44377598869163));
#64382=CARTESIAN_POINT('Ctrl Pts',(-0.000427771212261796,2.42227478841018,
9.4438059437003));
#64383=CARTESIAN_POINT('Ctrl Pts',(-0.000643659632893115,2.42227442954117,
9.44381935556109));
#64384=CARTESIAN_POINT('Ctrl Pts',(-0.00108154367626381,2.42227326164294,
9.44384653363649));
#64385=CARTESIAN_POINT('Ctrl Pts',(-0.00130353786061986,2.4222724401752,
9.44386029909049));
#64386=CARTESIAN_POINT('Ctrl Pts',(-0.00194226324689817,2.42226941664924,
9.44389986827118));
#64387=CARTESIAN_POINT('Ctrl Pts',(-0.00235899321992314,2.42226663564444,
9.44392563945212));
#64388=CARTESIAN_POINT('Ctrl Pts',(-0.00418754460761447,2.42225088594671,
9.44403852534218));
#64389=CARTESIAN_POINT('Ctrl Pts',(-0.00559930503995359,2.42222944771996,
9.44412517217553));
#64390=CARTESIAN_POINT('Ctrl Pts',(-0.0318110010635777,2.42165909221178,
9.44572522627955));
#64391=CARTESIAN_POINT('Ctrl Pts',(-0.0564704156518841,2.41825781489996,
9.44709007386456));
#64392=CARTESIAN_POINT('Ctrl Pts',(-0.0944218169442216,2.40846791367448,
9.44928292744702));
#64393=CARTESIAN_POINT('Ctrl Pts',(-0.108088359660273,2.40394867462966,
9.45009194976089));
#64394=CARTESIAN_POINT('Ctrl Pts',(-0.129318534041725,2.39531481854868,
9.45142260314094));
#64395=CARTESIAN_POINT('Ctrl Pts',(-0.13709873535756,2.39178424076615,9.45192681945133));
#64396=CARTESIAN_POINT('Ctrl Pts',(-0.146221588326327,2.3871989084949,9.45254241476187));
#64397=CARTESIAN_POINT('Ctrl Pts',(-0.14770821413167,2.38643716457588,9.45264351988173));
#64398=CARTESIAN_POINT('Ctrl Pts',(-0.150291767365153,2.3850878961813,9.45282064402546));
#64399=CARTESIAN_POINT('Ctrl Pts',(-0.151391347496616,2.38450550736685,
9.45289648189224));
#64400=CARTESIAN_POINT('Ctrl Pts',(-0.15296634063232,2.38365960175618,9.45300577106128));
#64401=CARTESIAN_POINT('Ctrl Pts',(-0.153444512120132,2.38340122217347,
9.45303903969748));
#64402=CARTESIAN_POINT('Ctrl Pts',(-0.154272963672417,2.38295085767419,
9.45309683311902));
#64403=CARTESIAN_POINT('Ctrl Pts',(-0.154623545695276,2.38275942830104,
9.45312133805));
#64404=CARTESIAN_POINT('Ctrl Pts',(-0.155296788107194,2.38239018919724,
9.45316848911739));
#64405=CARTESIAN_POINT('Ctrl Pts',(-0.155619501475434,2.38221247688586,
9.45319113174278));
#64406=CARTESIAN_POINT('Ctrl Pts',(-0.156378801743565,2.38179264578832,
9.45324450407131));
#64407=CARTESIAN_POINT('Ctrl Pts',(-0.156815131240463,2.38155006564499,
9.45327525027954));
#64408=CARTESIAN_POINT('Ctrl Pts',(-0.158320985185207,2.3807082902142,9.45338162526641));
#64409=CARTESIAN_POINT('Ctrl Pts',(-0.159387642975346,2.38010401236891,
9.45345743657322));
#64410=CARTESIAN_POINT('Ctrl Pts',(-0.175185760898387,2.37103468030694,
9.45458722068634));
#64411=CARTESIAN_POINT('Ctrl Pts',(-0.189226195622882,2.36142518482748,
9.45568369345702));
#64412=CARTESIAN_POINT('Ctrl Pts',(-0.20889186676361,2.34554851778675,9.4573619250163));
#64413=CARTESIAN_POINT('Ctrl Pts',(-0.215137967766779,2.34009483680573,
9.45791877329522));
#64414=CARTESIAN_POINT('Ctrl Pts',(-0.232883932008744,2.32335122024046,
9.45956617884787));
#64415=CARTESIAN_POINT('Ctrl Pts',(-0.243756072219131,2.31143249917826,
9.46066334876295));
#64416=CARTESIAN_POINT('Ctrl Pts',(-0.257575779302565,2.29379257220772,
9.46214546943847));
#64417=CARTESIAN_POINT('Ctrl Pts',(-0.261314064662466,2.28872152455604,
9.46255672074514));
#64418=CARTESIAN_POINT('Ctrl Pts',(-0.266579874975248,2.2811215887171,9.46314808354513));
#64419=CARTESIAN_POINT('Ctrl Pts',(-0.268224961715004,2.2786763304488,9.46333470165444));
#64420=CARTESIAN_POINT('Ctrl Pts',(-0.270111483347827,2.27578741539139,
9.46355062148433));
#64421=CARTESIAN_POINT('Ctrl Pts',(-0.270385636642753,2.275365436594,9.46358204803376));
#64422=CARTESIAN_POINT('Ctrl Pts',(-0.270802937888664,2.27471981844616,
9.46362995624542));
#64423=CARTESIAN_POINT('Ctrl Pts',(-0.270946798110636,2.27449664386975,
9.46364648534541));
#64424=CARTESIAN_POINT('Ctrl Pts',(-0.271207119354334,2.27409170180817,
9.46367641915284));
#64425=CARTESIAN_POINT('Ctrl Pts',(-0.271323673087633,2.27390999583102,
9.4636898300541));
#64426=CARTESIAN_POINT('Ctrl Pts',(-0.271559827030519,2.27354101919044,
9.46371701991688));
#64427=CARTESIAN_POINT('Ctrl Pts',(-0.271679415618944,2.27335374275792,
9.46373079809167));
#64428=CARTESIAN_POINT('Ctrl Pts',(-0.272023285189683,2.27281401119528,
9.46377044337863));
#64429=CARTESIAN_POINT('Ctrl Pts',(-0.272247075716551,2.27246124178854,
9.46379627774612));
#64430=CARTESIAN_POINT('Ctrl Pts',(-0.273228985673921,2.27090674619155,
9.46390978053083));
#64431=CARTESIAN_POINT('Ctrl Pts',(-0.273979853806524,2.26970042542414,
9.46399697477659));
#64432=CARTESIAN_POINT('Ctrl Pts',(-0.28774136849943,2.24726217992771,9.46560325088784));
#64433=CARTESIAN_POINT('Ctrl Pts',(-0.298258316118295,2.22459397480774,
9.46697273787475));
#64434=CARTESIAN_POINT('Ctrl Pts',(-0.310544594283947,2.18733976350732,
9.46916768716732));
#64435=CARTESIAN_POINT('Ctrl Pts',(-0.314117621720231,2.17345921458919,
9.46997349802716));
#64436=CARTESIAN_POINT('Ctrl Pts',(-0.318324573656111,2.15102071091626,
9.47129921116356));
#64437=CARTESIAN_POINT('Ctrl Pts',(-0.319561066207244,2.14259522697368,
9.47180184729937));
#64438=CARTESIAN_POINT('Ctrl Pts',(-0.320729624449961,2.13162346569902,
9.47246714147152));
#64439=CARTESIAN_POINT('Ctrl Pts',(-0.320967260234324,2.12911276150998,
9.47262009726594));
#64440=CARTESIAN_POINT('Ctrl Pts',(-0.321234412885735,2.12588703924306,
9.47281761024139));
#64441=CARTESIAN_POINT('Ctrl Pts',(-0.321291053455397,2.12517430792223,
9.47286131353706));
#64442=CARTESIAN_POINT('Ctrl Pts',(-0.321378388716614,2.12402699912974,
9.47293176656261));
#64443=CARTESIAN_POINT('Ctrl Pts',(-0.321410574994004,2.12359253484346,
9.47295846939065));
#64444=CARTESIAN_POINT('Ctrl Pts',(-0.321470132793487,2.12276585014836,
9.47300932406289));
#64445=CARTESIAN_POINT('Ctrl Pts',(-0.321497667725141,2.1223736420003,9.47303347072777));
#64446=CARTESIAN_POINT('Ctrl Pts',(-0.321558720451101,2.12148061612756,
9.47308849536898));
#64447=CARTESIAN_POINT('Ctrl Pts',(-0.321591786024402,2.12097976940913,
9.47311938748575));
#64448=CARTESIAN_POINT('Ctrl Pts',(-0.321686619014133,2.11949040181011,
9.47321134751648));
#64449=CARTESIAN_POINT('Ctrl Pts',(-0.321744999173261,2.11850167796141,
9.473272521558));
#64450=CARTESIAN_POINT('Ctrl Pts',(-0.322118764873831,2.11163367380052,
9.47369834966237));
#64451=CARTESIAN_POINT('Ctrl Pts',(-0.322277523335093,2.10574731414913,
9.47406788771386));
#64452=CARTESIAN_POINT('Ctrl Pts',(-0.322268664214049,2.08532379795546,
9.47536706946818));
#64453=CARTESIAN_POINT('Ctrl Pts',(-0.321278877098094,2.07080633380078,
9.47632145016023));
#64454=CARTESIAN_POINT('Ctrl Pts',(-0.315359557933376,2.02744830219341,
9.47925015796388));
#64455=CARTESIAN_POINT('Ctrl Pts',(-0.307485361907278,1.99916226809078,
9.48127769601501));
#64456=CARTESIAN_POINT('Ctrl Pts',(-0.295302783577381,1.97092731096894,
9.48322301636947));
#64457=CARTESIAN_POINT('Ctrl Pts',(-0.294689784603897,1.9695338200556,9.48331877406412));
#64458=CARTESIAN_POINT('Ctrl Pts',(-0.293893466352226,1.96775785167776,
9.48344044466888));
#64459=CARTESIAN_POINT('Ctrl Pts',(-0.293719248059145,1.9673713504484,9.48346690112843));
#64460=CARTESIAN_POINT('Ctrl Pts',(-0.293440801682592,1.9667568599397,9.48350892651822));
#64461=CARTESIAN_POINT('Ctrl Pts',(-0.293337070153306,1.96652864824182,
9.48352452587794));
#64462=CARTESIAN_POINT('Ctrl Pts',(-0.293142475352939,1.9661018578994,9.48355368339751));
#64463=CARTESIAN_POINT('Ctrl Pts',(-0.293051677210064,1.96590325209454,
9.4835672453907));
#64464=CARTESIAN_POINT('Ctrl Pts',(-0.292846811189296,1.96545634364368,
9.48359774873974));
#64465=CARTESIAN_POINT('Ctrl Pts',(-0.292732629608321,1.96520809425863,
9.48361468291889));
#64466=CARTESIAN_POINT('Ctrl Pts',(-0.292391785114081,1.96446951849386,
9.48366503589277));
#64467=CARTESIAN_POINT('Ctrl Pts',(-0.292164203564573,1.96397961334793,
9.48369839809519));
#64468=CARTESIAN_POINT('Ctrl Pts',(-0.29027864874859,1.95994722522602,9.48397271058692));
#64469=CARTESIAN_POINT('Ctrl Pts',(-0.288557454015435,1.95643443055387,
9.48420982746064));
#64470=CARTESIAN_POINT('Ctrl Pts',(-0.282738861666761,1.94508689881804,
9.48497251934108));
#64471=CARTESIAN_POINT('Ctrl Pts',(-0.278382745406185,1.93738879035215,
9.48548478703197));
#64472=CARTESIAN_POINT('Ctrl Pts',(-0.263121990917532,1.91283508650598,
9.48713306172484));
#64473=CARTESIAN_POINT('Ctrl Pts',(-0.250959803603303,1.89681752392562,
9.48823403895985));
#64474=CARTESIAN_POINT('Ctrl Pts',(-0.225428417107186,1.86901123125861,
9.49037117181415));
#64475=CARTESIAN_POINT('Ctrl Pts',(-0.212420745365698,1.85699573719498,
9.4913956400729));
#64476=CARTESIAN_POINT('Ctrl Pts',(-0.19748630371246,1.84531985922216,9.49254715982183));
#64477=CARTESIAN_POINT('Ctrl Pts',(-0.196473156370865,1.84453745281758,
9.49262515296697));
#64478=CARTESIAN_POINT('Ctrl Pts',(-0.19505102248142,1.84345266927825,9.49273446645517));
#64479=CARTESIAN_POINT('Ctrl Pts',(-0.194645931477413,1.84314518570579,
9.49276558567021));
#64480=CARTESIAN_POINT('Ctrl Pts',(-0.193944224686769,1.84261516976142,
9.4928194599483));
#64481=CARTESIAN_POINT('Ctrl Pts',(-0.193647948686448,1.84239218743609,
9.49284219731972));
#64482=CARTESIAN_POINT('Ctrl Pts',(-0.193033051858006,1.84193106590439,
9.49288936750593));
#64483=CARTESIAN_POINT('Ctrl Pts',(-0.192714373775032,1.84169300436662,
9.49291380330471));
#64484=CARTESIAN_POINT('Ctrl Pts',(-0.191967022234189,1.84113686447298,
9.49297108452006));
#64485=CARTESIAN_POINT('Ctrl Pts',(-0.191537998598352,1.84081926065425,
9.49300394835082));
#64486=CARTESIAN_POINT('Ctrl Pts',(-0.19014953536488,1.839796719296,9.49311024700899));
#64487=CARTESIAN_POINT('Ctrl Pts',(-0.189186986384869,1.83909603833931,
9.49318384668908));
#64488=CARTESIAN_POINT('Ctrl Pts',(-0.17486368694438,1.82879042979709,9.49427776876171));
#64489=CARTESIAN_POINT('Ctrl Pts',(-0.160792622469784,1.82021880171326,
9.49533787817407));
#64490=CARTESIAN_POINT('Ctrl Pts',(-0.118976140481853,1.7989450772965,9.49844746597816));
#64491=CARTESIAN_POINT('Ctrl Pts',(-0.0900024818253041,1.7890517788638,
9.50056766839039));
#64492=CARTESIAN_POINT('Ctrl Pts',(-0.0564190115584183,1.7826801346126,
9.50276673719013));
#64493=CARTESIAN_POINT('Ctrl Pts',(-0.0527538985608195,1.78205026974294,
9.50300315008199));
#64494=CARTESIAN_POINT('Ctrl Pts',(-0.0485041130863901,1.78139544194962,
9.50327251264313));
#64495=CARTESIAN_POINT('Ctrl Pts',(-0.0479294667994533,1.78130848831257,
9.50330883484219));
#64496=CARTESIAN_POINT('Ctrl Pts',(-0.0470761105143446,1.78118172150566,
9.5033626215749));
#64497=CARTESIAN_POINT('Ctrl Pts',(-0.0467975825365779,1.78114071888459,
9.5033801530505));
#64498=CARTESIAN_POINT('Ctrl Pts',(-0.0463021001400073,1.78106844120686,
9.50341129717223));
#64499=CARTESIAN_POINT('Ctrl Pts',(-0.046085167632363,1.78103702252929,
9.50342491798359));
#64500=CARTESIAN_POINT('Ctrl Pts',(-0.045625302319848,1.78097089845441,
9.50345376077885));
#64501=CARTESIAN_POINT('Ctrl Pts',(-0.0453823625692465,1.78093624929591,
9.50346897950236));
#64502=CARTESIAN_POINT('Ctrl Pts',(-0.044732131235611,1.78084426805622,
9.50350966373129));
#64503=CARTESIAN_POINT('Ctrl Pts',(-0.0443247673666703,1.78078743790415,
9.50353510072));
#64504=CARTESIAN_POINT('Ctrl Pts',(-0.0423933919717215,1.78052176575215,
9.50365546307971));
#64505=CARTESIAN_POINT('Ctrl Pts',(-0.0408679738915177,1.78032305248546,
9.50374982321856));
#64506=CARTESIAN_POINT('Ctrl Pts',(-0.0283770495561705,1.77878675495633,
9.50451717478705));
#64507=CARTESIAN_POINT('Ctrl Pts',(-0.0173495505827463,1.77800270991574,
9.5051612146624));
#64508=CARTESIAN_POINT('Ctrl Pts',(0.021258894589797,1.77724753925847,9.50736621207636));
#64509=CARTESIAN_POINT('Ctrl Pts',(0.0487751108935489,1.78024668439134,
9.50885917040709));
#64510=CARTESIAN_POINT('Ctrl Pts',(0.0776070937649643,1.78720184596617,
9.51057801592824));
#64511=CARTESIAN_POINT('Ctrl Pts',(0.0796345344332012,1.78771185285784,
9.51069966392777));
#64512=CARTESIAN_POINT('Ctrl Pts',(0.0839626336116177,1.78884548339104,
9.51096115963452));
#64513=CARTESIAN_POINT('Ctrl Pts',(0.0862616128379872,1.78947497556769,
9.51110115994581));
#64514=CARTESIAN_POINT('Ctrl Pts',(0.0948214199487309,1.79192116081028,
9.5116268549502));
#64515=CARTESIAN_POINT('Ctrl Pts',(0.101033316806052,1.79390208659309,9.51201729693627));
#64516=CARTESIAN_POINT('Ctrl Pts',(0.108155619489423,1.79641375761126,9.51247693793854));
#64517=CARTESIAN_POINT('Ctrl Pts',(0.109129006680805,1.79676229710562,9.51254001757606));
#64518=CARTESIAN_POINT('Ctrl Pts',(0.110574214667697,1.79728764060791,9.51263406890725));
#64519=CARTESIAN_POINT('Ctrl Pts',(0.111047331850594,1.79746087928598,9.51266492174205));
#64520=CARTESIAN_POINT('Ctrl Pts',(0.11188913772098,1.79777135931316,9.51271993099435));
#64521=CARTESIAN_POINT('Ctrl Pts',(0.112257985831564,1.79790816792534,9.51274407291855));
#64522=CARTESIAN_POINT('Ctrl Pts',(0.113033800919043,1.79819754080995,9.51279493409158));
#64523=CARTESIAN_POINT('Ctrl Pts',(0.113440711338705,1.79835025355325,9.51282165826909));
#64524=CARTESIAN_POINT('Ctrl Pts',(0.114511880722566,1.79875473542803,9.51289213486699));
#64525=CARTESIAN_POINT('Ctrl Pts',(0.115175615597057,1.79900787749082,9.51293593323548));
#64526=CARTESIAN_POINT('Ctrl Pts',(0.118149825392962,1.80015349061443,9.51313277673));
#64527=CARTESIAN_POINT('Ctrl Pts',(0.120450752921286,1.80107036613783,9.51328664025806));
#64528=CARTESIAN_POINT('Ctrl Pts',(0.137280980310969,1.80800275127666,9.51442401013526));
#64529=CARTESIAN_POINT('Ctrl Pts',(0.151361044867126,1.81504708540176,9.51544285665507));
#64530=CARTESIAN_POINT('Ctrl Pts',(0.189802305431232,1.83793456828385,9.51841627303041));
#64531=CARTESIAN_POINT('Ctrl Pts',(0.212614617876141,1.85607759062619,9.520430528713));
#64532=CARTESIAN_POINT('Ctrl Pts',(0.235580777745899,1.88004470970184,9.52257251920456));
#64533=CARTESIAN_POINT('Ctrl Pts',(0.238412745553526,1.88311754461179,9.52283870463431));
#64534=CARTESIAN_POINT('Ctrl Pts',(0.241543513364925,1.88665005258505,9.52313446883139));
#64535=CARTESIAN_POINT('Ctrl Pts',(0.24190169365826,1.88705625267219,9.52316832883036));
#64536=CARTESIAN_POINT('Ctrl Pts',(0.24244188082922,1.88767198237343,9.52321942628094));
#64537=CARTESIAN_POINT('Ctrl Pts',(0.24262464152749,1.88788084486705,9.52323671952709));
#64538=CARTESIAN_POINT('Ctrl Pts',(0.242941862053745,1.88824431703072,9.52326674488746));
#64539=CARTESIAN_POINT('Ctrl Pts',(0.243076444274206,1.88839881888922,9.52327948617231));
#64540=CARTESIAN_POINT('Ctrl Pts',(0.243354850055728,1.88871904787771,9.52330584944662));
#64541=CARTESIAN_POINT('Ctrl Pts',(0.243498651628819,1.88888479346428,9.52331946974435));
#64542=CARTESIAN_POINT('Ctrl Pts',(0.243840898407636,1.88928008172286,9.52335189392682));
#64543=CARTESIAN_POINT('Ctrl Pts',(0.244039189601296,1.88950975881168,9.52337068627775));
#64544=CARTESIAN_POINT('Ctrl Pts',(0.244692432966752,1.89026856261424,9.52343261761529));
#64545=CARTESIAN_POINT('Ctrl Pts',(0.245145994975034,1.89079889161819,9.52347565408988));
#64546=CARTESIAN_POINT('Ctrl Pts',(0.246217765048562,1.89206033450812,9.52357744716268));
#64547=CARTESIAN_POINT('Ctrl Pts',(0.246834448624139,1.8927927430431,9.52363609541454));
#64548=CARTESIAN_POINT('Ctrl Pts',(0.25381349692726,1.90115683009499,9.52430085457905));
#64549=CARTESIAN_POINT('Ctrl Pts',(0.259823622435528,1.90907691296325,9.52488320410247));
#64550=CARTESIAN_POINT('Ctrl Pts',(0.277194578880663,1.93431136866626,9.52664138994009));
#64551=CARTESIAN_POINT('Ctrl Pts',(0.287261287564148,1.95245137868623,9.52777563166682));
#64552=CARTESIAN_POINT('Ctrl Pts',(0.302959451080443,1.98853437346439,9.52999794610384));
#64553=CARTESIAN_POINT('Ctrl Pts',(0.30890014571705,2.00624734981947,9.53107527606678));
#64554=CARTESIAN_POINT('Ctrl Pts',(0.313578157120183,2.02562544018355,9.53228612463053));
#64555=CARTESIAN_POINT('Ctrl Pts',(0.313872999191476,2.02687971503066,9.53236462497757));
#64556=CARTESIAN_POINT('Ctrl Pts',(0.31427403345198,2.02863286735863,9.5324745353521));
#64557=CARTESIAN_POINT('Ctrl Pts',(0.314386577545431,2.02913029153313,9.53250574133487));
#64558=CARTESIAN_POINT('Ctrl Pts',(0.314578991486629,2.02999020413533,9.53255972507368));
#64559=CARTESIAN_POINT('Ctrl Pts',(0.314659416923627,2.03035256830887,9.53258248496662));
#64560=CARTESIAN_POINT('Ctrl Pts',(0.31482468396915,2.03110332348554,9.53262966328984));
#64561=CARTESIAN_POINT('Ctrl Pts',(0.314909433264316,2.03149173400273,9.53265408463713));
#64562=CARTESIAN_POINT('Ctrl Pts',(0.315105995962537,2.03240066290525,9.5327112649062));
#64563=CARTESIAN_POINT('Ctrl Pts',(0.315217238401547,2.03292130236603,9.53274404205147));
#64564=CARTESIAN_POINT('Ctrl Pts',(0.315571499736244,2.03459966691907,9.53284978306714));
#64565=CARTESIAN_POINT('Ctrl Pts',(0.315809432362121,2.03575844503607,9.53292290937718));
#64566=CARTESIAN_POINT('Ctrl Pts',(0.319297336476145,2.0532329903578,9.53402754526642));
#64567=CARTESIAN_POINT('Ctrl Pts',(0.321285037015188,2.06977238603252,9.53509975900824));
#64568=CARTESIAN_POINT('Ctrl Pts',(0.323231592584745,2.11582119407242,9.53815608150583));
#64569=CARTESIAN_POINT('Ctrl Pts',(0.320434628341889,2.14528229190852,9.54020227371234));
#64570=CARTESIAN_POINT('Ctrl Pts',(0.313603712207176,2.17425621027312,9.54212712541004));
#64571=CARTESIAN_POINT('Ctrl Pts',(0.313531637237962,2.17455994585998,9.54214729202866));
#64572=CARTESIAN_POINT('Ctrl Pts',(0.312481985730568,2.1789549113422,9.54243892265675));
#64573=CARTESIAN_POINT('Ctrl Pts',(0.311424783449572,2.18302697085351,9.54270694077793));
#64574=CARTESIAN_POINT('Ctrl Pts',(0.310141489237368,2.18759980985889,9.54300454459229));
#64575=CARTESIAN_POINT('Ctrl Pts',(0.309993562065426,2.18812185609623,9.54303846970813));
#64576=CARTESIAN_POINT('Ctrl Pts',(0.309767905786681,2.18891061433645,9.54308964871059));
#64577=CARTESIAN_POINT('Ctrl Pts',(0.309691150034815,2.18917760026315,9.54310695864112));
#64578=CARTESIAN_POINT('Ctrl Pts',(0.309557162688518,2.18964140038983,9.54313700490263));
#64579=CARTESIAN_POINT('Ctrl Pts',(0.30950008853647,2.18983825928897,9.54314975043534));
#64580=CARTESIAN_POINT('Ctrl Pts',(0.309384964243553,2.19023393165153,9.54317535270668));
#64581=CARTESIAN_POINT('Ctrl Pts',(0.309326910301223,2.1904327434342,9.54318820915659));
#64582=CARTESIAN_POINT('Ctrl Pts',(0.309185640020984,2.19091481060904,9.54321936406198));
#64583=CARTESIAN_POINT('Ctrl Pts',(0.309102225757637,2.19119800884122,9.54323765088659));
#64584=CARTESIAN_POINT('Ctrl Pts',(0.308831880195581,2.19211122222652,9.54329657012141));
#64585=CARTESIAN_POINT('Ctrl Pts',(0.308643409458439,2.19274078553139,9.543337112967));
#64586=CARTESIAN_POINT('Ctrl Pts',(0.30819623401549,2.19421805816325,9.54343207856947));
#64587=CARTESIAN_POINT('Ctrl Pts',(0.307935953978102,2.19506529038031,9.54348641191282));
#64588=CARTESIAN_POINT('Ctrl Pts',(0.305088165925829,2.20420064554312,9.54407096359412));
#64589=CARTESIAN_POINT('Ctrl Pts',(0.302169958604867,2.21238286966036,9.54458296135033));
#64590=CARTESIAN_POINT('Ctrl Pts',(0.293043169543791,2.23503536741487,9.54599360109135));
#64591=CARTESIAN_POINT('Ctrl Pts',(0.286100108734918,2.24918323761678,9.54686730760931));
#64592=CARTESIAN_POINT('Ctrl Pts',(0.265710002651048,2.28402747769003,9.54912528271612));
#64593=CARTESIAN_POINT('Ctrl Pts',(0.250875320436816,2.30378724829836,9.55051749627373));
#64594=CARTESIAN_POINT('Ctrl Pts',(0.232869482148884,2.32279000620268,9.5521047987591));
#64595=CARTESIAN_POINT('Ctrl Pts',(0.231794285951151,2.32390844434582,9.55219921212121));
#64596=CARTESIAN_POINT('Ctrl Pts',(0.230325763386399,2.32541411418644,9.55232768420004));
#64597=CARTESIAN_POINT('Ctrl Pts',(0.22993944413791,2.32580817562161,9.5523614364851));
#64598=CARTESIAN_POINT('Ctrl Pts',(0.229283647535119,2.32647368699355,9.55241865865483));
#64599=CARTESIAN_POINT('Ctrl Pts',(0.229014694614836,2.32674565392945,9.5524421054444));
#64600=CARTESIAN_POINT('Ctrl Pts',(0.228496217131304,2.3272680782101,9.55248726539111));
#64601=CARTESIAN_POINT('Ctrl Pts',(0.228246763204345,2.32751860517724,9.55250897541078));
#64602=CARTESIAN_POINT('Ctrl Pts',(0.227657888815688,2.3281080694983,9.55256018396993));
#64603=CARTESIAN_POINT('Ctrl Pts',(0.227318123576451,2.3284466598574,9.55258969778726));
#64604=CARTESIAN_POINT('Ctrl Pts',(0.226327313114705,2.32942964514087,9.55267567236767));
#64605=CARTESIAN_POINT('Ctrl Pts',(0.225674278834751,2.33007202041072,9.55273222178505));
#64606=CARTESIAN_POINT('Ctrl Pts',(0.221002260832091,2.33462875092592,9.55313598936922));
#64607=CARTESIAN_POINT('Ctrl Pts',(0.216884621938633,2.33844014852408,9.55348765011136));
#64608=CARTESIAN_POINT('Ctrl Pts',(0.203288451437431,2.35038147011633,9.55463661105784));
#64609=CARTESIAN_POINT('Ctrl Pts',(0.193437262798419,2.35806789331508,9.55545130936903));
#64610=CARTESIAN_POINT('Ctrl Pts',(0.163876903271003,2.3784872461229,9.55784086479478));
#64611=CARTESIAN_POINT('Ctrl Pts',(0.143192879968853,2.38966618912064,9.55945293553449));
#64612=CARTESIAN_POINT('Ctrl Pts',(0.112896738166894,2.40199565880107,9.56161953866308));
#64613=CARTESIAN_POINT('Ctrl Pts',(0.104165728386744,2.40511733828523,9.56222222941829));
#64614=CARTESIAN_POINT('Ctrl Pts',(0.0946232931880807,2.40807162624372,
9.56284914231799));
#64615=CARTESIAN_POINT('Ctrl Pts',(0.0939344592572533,2.40828235742213,
9.5628942206823));
#64616=CARTESIAN_POINT('Ctrl Pts',(0.0929724265354901,2.40857314297219,
9.562956926307));
#64617=CARTESIAN_POINT('Ctrl Pts',(0.0926998260241585,2.40865514561766,
9.5629746664034));
#64618=CARTESIAN_POINT('Ctrl Pts',(0.0922290641011621,2.40879607850494,
9.56300525337992));
#64619=CARTESIAN_POINT('Ctrl Pts',(0.0920309545939117,2.4088551792703,9.56301811027563));
#64620=CARTESIAN_POINT('Ctrl Pts',(0.09163316271629,2.40897343330362,9.56304389596315));
#64621=CARTESIAN_POINT('Ctrl Pts',(0.0914334802172228,2.40903258354481,
9.56305682451607));
#64622=CARTESIAN_POINT('Ctrl Pts',(0.090955823126286,2.40917357233683,9.56308771443844));
#64623=CARTESIAN_POINT('Ctrl Pts',(0.0906777943401781,2.40925522987861,
9.5631056651384));
#64624=CARTESIAN_POINT('Ctrl Pts',(0.0898160525804968,2.40950706292818,
9.56316121304228));
#64625=CARTESIAN_POINT('Ctrl Pts',(0.0892319635807685,2.40967596289235,
9.56319873596414));
#64626=CARTESIAN_POINT('Ctrl Pts',(0.0878627563749514,2.41006769860641,
9.56328640551743));
#64627=CARTESIAN_POINT('Ctrl Pts',(0.0870772586301308,2.41028920822259,
9.56333647701758));
#64628=CARTESIAN_POINT('Ctrl Pts',(0.0844105515308456,2.41103029315772,
9.56350573554873));
#64629=CARTESIAN_POINT('Ctrl Pts',(0.082525425212537,2.41153577496495,9.56362415592365));
#64630=CARTESIAN_POINT('Ctrl Pts',(0.0745270477796974,2.41360277975589,
9.56412185688444));
#64631=CARTESIAN_POINT('Ctrl Pts',(0.0683728530071468,2.41500182254504,
9.56449312844384));
#64632=CARTESIAN_POINT('Ctrl Pts',(0.0513576742428597,2.41834767507816,
9.5654975470323));
#64633=CARTESIAN_POINT('Ctrl Pts',(0.0404314161564145,2.41991902349606,
9.56611828907221));
#64634=CARTESIAN_POINT('Ctrl Pts',(0.0064523773799224,2.42303665247454,
9.56802880003962));
#64635=CARTESIAN_POINT('Ctrl Pts',(-0.0166987589237333,2.42266912572022,
9.56930764977649));
#64636=CARTESIAN_POINT('Ctrl Pts',(-0.0470715056288379,2.41890744302973,
9.57110646206526));
#64637=CARTESIAN_POINT('Ctrl Pts',(-0.0544965823404676,2.41772282350899,
9.57155539303144));
#64638=CARTESIAN_POINT('Ctrl Pts',(-0.0628246298547019,2.41609362804777,
9.57207169532607));
#64639=CARTESIAN_POINT('Ctrl Pts',(-0.0637753695140291,2.41590317823654,
9.57213082522459));
#64640=CARTESIAN_POINT('Ctrl Pts',(-0.065213024945841,2.41560843612037,
9.57222052826154));
#64641=CARTESIAN_POINT('Ctrl Pts',(-0.0657005881219724,2.41550729989806,
9.57225100053699));
#64642=CARTESIAN_POINT('Ctrl Pts',(-0.0665481510461026,2.41532943837156,
9.57230406124097));
#64643=CARTESIAN_POINT('Ctrl Pts',(-0.0669082583258361,2.41525322532427,
9.57232663324337));
#64644=CARTESIAN_POINT('Ctrl Pts',(-0.0676591206794027,2.41509296845079,
9.57237375684451));
#64645=CARTESIAN_POINT('Ctrl Pts',(-0.0680498513707639,2.41500881432813,
9.57239831194312));
#64646=CARTESIAN_POINT('Ctrl Pts',(-0.0689729264245647,2.41480820827544,
9.57245640047189));
#64647=CARTESIAN_POINT('Ctrl Pts',(-0.0695051327119088,2.41469113285577,
9.57248995384491));
#64648=CARTESIAN_POINT('Ctrl Pts',(-0.0712593552349693,2.41430056958,9.57260075627762));
#64649=CARTESIAN_POINT('Ctrl Pts',(-0.0724800629376421,2.41402131162136,
9.57267819036309));
#64650=CARTESIAN_POINT('Ctrl Pts',(-0.0753382245780173,2.41334990431894,
9.57286028181588));
#64651=CARTESIAN_POINT('Ctrl Pts',(-0.0769742823434019,2.41295202556255,
9.57296512208139));
#64652=CARTESIAN_POINT('Ctrl Pts',(-0.0869298037493087,2.41044811723346,
9.57360686137637));
#64653=CARTESIAN_POINT('Ctrl Pts',(-0.0951648491774735,2.40802346242178,
9.57415397222917));
#64654=CARTESIAN_POINT('Ctrl Pts',(-0.117424419152896,2.40049167901227,
9.57567884256153));
#64655=CARTESIAN_POINT('Ctrl Pts',(-0.131205561355818,2.39473506651518,
9.57667521699707));
#64656=CARTESIAN_POINT('Ctrl Pts',(-0.156583756946295,2.38200064237059,
9.57859224294938));
#64657=CARTESIAN_POINT('Ctrl Pts',(-0.168239395761824,2.37520601761502,
9.57950883040451));
#64658=CARTESIAN_POINT('Ctrl Pts',(-0.182751116727739,2.36547907146556,
9.58067536921705));
#64659=CARTESIAN_POINT('Ctrl Pts',(-0.186025275815827,2.36319518780022,
9.58094029400329));
#64660=CARTESIAN_POINT('Ctrl Pts',(-0.191152488926826,2.35947522047748,
9.58135698907413));
#64661=CARTESIAN_POINT('Ctrl Pts',(-0.193033706137368,2.35807877267938,
9.58151028002283));
#64662=CARTESIAN_POINT('Ctrl Pts',(-0.195765127100436,2.35600463242039,
9.58173325549735));
#64663=CARTESIAN_POINT('Ctrl Pts',(-0.196627361062241,2.35534298062153,
9.58180370273195));
#64664=CARTESIAN_POINT('Ctrl Pts',(-0.197761355400776,2.35446363813542,
9.58189641586467));
#64665=CARTESIAN_POINT('Ctrl Pts',(-0.198036123619149,2.35424985853898,
9.58191888522254));
#64666=CARTESIAN_POINT('Ctrl Pts',(-0.20149937179276,2.35154630617547,9.58220215049142));
#64667=CARTESIAN_POINT('Ctrl Pts',(-0.204641230168573,2.3489970113427,9.58245972929217));
#64668=CARTESIAN_POINT('Ctrl Pts',(-0.208189879611555,2.34600509048688,
9.58275054800604));
#64669=CARTESIAN_POINT('Ctrl Pts',(-0.208644271420657,2.34561982520748,
9.5827877841282));
#64670=CARTESIAN_POINT('Ctrl Pts',(-0.209311686610368,2.34505075521187,
9.58284247031465));
#64671=CARTESIAN_POINT('Ctrl Pts',(-0.20952553844152,2.34486793077867,9.58285999175023));
#64672=CARTESIAN_POINT('Ctrl Pts',(-0.209906002985302,2.34454180385035,
9.58289116197631));
#64673=CARTESIAN_POINT('Ctrl Pts',(-0.210072708605164,2.34439861092093,
9.58290481885064));
#64674=CARTESIAN_POINT('Ctrl Pts',(-0.210394272972469,2.34412182891296,
9.58293116044853));
#64675=CARTESIAN_POINT('Ctrl Pts',(-0.210549150361129,2.3439882635173,9.58294384684597));
#64676=CARTESIAN_POINT('Ctrl Pts',(-0.210884727460055,2.34369830623031,
9.58297133356393));
#64677=CARTESIAN_POINT('Ctrl Pts',(-0.211065380750687,2.34354186043651,
9.58298612987173));
#64678=CARTESIAN_POINT('Ctrl Pts',(-0.211785288656747,2.34291701736114,
9.58304509117304));
#64679=CARTESIAN_POINT('Ctrl Pts',(-0.212323164792294,2.34244702417345,
9.58308913857432));
#64680=CARTESIAN_POINT('Ctrl Pts',(-0.21956193357634,2.33607926295029,9.58368193039609));
#64681=CARTESIAN_POINT('Ctrl Pts',(-0.226017253251032,2.32990671173682,
9.58421058059388));
#64682=CARTESIAN_POINT('Ctrl Pts',(-0.236605132436258,2.31890497407467,
9.58509501434325));
#64683=CARTESIAN_POINT('Ctrl Pts',(-0.240866136554129,2.31420757980559,
9.58545628349211));
#64684=CARTESIAN_POINT('Ctrl Pts',(-0.264506056783994,2.2865485642281,9.5875119236336));
#64685=CARTESIAN_POINT('Ctrl Pts',(-0.28073531957503,2.26109458618406,9.58914715594871));
#64686=CARTESIAN_POINT('Ctrl Pts',(-0.295462859792642,2.22881175616512,
9.59125345225957));
#64687=CARTESIAN_POINT('Ctrl Pts',(-0.297594985291289,2.2238062574249,9.59158030365337));
#64688=CARTESIAN_POINT('Ctrl Pts',(-0.299923823053417,2.21793070666265,
9.59196512777944));
#64689=CARTESIAN_POINT('Ctrl Pts',(-0.300244966647922,2.21711067922002,
9.59201886148015));
#64690=CARTESIAN_POINT('Ctrl Pts',(-0.300750958895294,2.21580288607428,
9.59210460099196));
#64691=CARTESIAN_POINT('Ctrl Pts',(-0.300937993041113,2.21531596610577,
9.59213653338941));
#64692=CARTESIAN_POINT('Ctrl Pts',(-0.301265398003013,2.21445738694076,
9.59219285725472));
#64693=CARTESIAN_POINT('Ctrl Pts',(-0.301406265576937,2.21408591730771,
9.59221723202037));
#64694=CARTESIAN_POINT('Ctrl Pts',(-0.301695520267472,2.21331887386166,
9.59226757576633));
#64695=CARTESIAN_POINT('Ctrl Pts',(-0.301843817046464,2.21292326700398,
9.59229354771251));
#64696=CARTESIAN_POINT('Ctrl Pts',(-0.30222035125099,2.21191275670874,9.59235990677157));
#64697=CARTESIAN_POINT('Ctrl Pts',(-0.302447489390301,2.2112974481997,9.59240033050724));
#64698=CARTESIAN_POINT('Ctrl Pts',(-0.303358609094866,2.20880587357108,
9.59256409123947));
#64699=CARTESIAN_POINT('Ctrl Pts',(-0.304027010673634,2.20692399322836,
9.59268794572183));
#64700=CARTESIAN_POINT('Ctrl Pts',(-0.308277547784344,2.19459446912556,
9.59350061582068));
#64701=CARTESIAN_POINT('Ctrl Pts',(-0.311337696316926,2.18397589875874,
9.59420655617429));
#64702=CARTESIAN_POINT('Ctrl Pts',(-0.319464805452436,2.14914129510034,
9.59654338974039));
#64703=CARTESIAN_POINT('Ctrl Pts',(-0.322292093734264,2.1244962849695,9.59823599948666));
#64704=CARTESIAN_POINT('Ctrl Pts',(-0.322274922248267,2.09977613648567,
9.59989505973818));
#64705=CARTESIAN_POINT('',(-0.322274904352262,2.10008161445013,9.84943339449977));
#64706=CARTESIAN_POINT('Ctrl Pts',(-0.322274921952289,2.09977571079884,
9.59989508830759));
#64707=CARTESIAN_POINT('Ctrl Pts',(-0.322265671419364,2.08648387703572,
9.60078715195519));
#64708=CARTESIAN_POINT('Ctrl Pts',(-0.321434112451775,2.0732031904389,9.60166524079288));
#64709=CARTESIAN_POINT('Ctrl Pts',(-0.319708691269864,2.05940567424189,
9.60253948376591));
#64710=CARTESIAN_POINT('Ctrl Pts',(-0.319631403647282,2.05880154889031,
9.60257768487487));
#64711=CARTESIAN_POINT('Ctrl Pts',(-0.319507081484653,2.05785118517041,
9.60263765375844));
#64712=CARTESIAN_POINT('Ctrl Pts',(-0.319461196144858,2.05750480179114,
9.60265948449201));
#64713=CARTESIAN_POINT('Ctrl Pts',(-0.319382597378943,2.05691879056035,
9.60269637224838));
#64714=CARTESIAN_POINT('Ctrl Pts',(-0.319350177510797,2.0566791246622,9.60271144566598));
#64715=CARTESIAN_POINT('Ctrl Pts',(-0.319289796358272,2.05623650450128,
9.60273925950681));
#64716=CARTESIAN_POINT('Ctrl Pts',(-0.319261911308225,2.05603354022491,
9.60275200424059));
#64717=CARTESIAN_POINT('Ctrl Pts',(-0.319203803245083,2.05561356484504,
9.60277835619602));
#64718=CARTESIAN_POINT('Ctrl Pts',(-0.319173552697779,2.05539655965656,
9.60279196164848));
#64719=CARTESIAN_POINT('Ctrl Pts',(-0.319104038714989,2.05490158641993,
9.60282297015809));
#64720=CARTESIAN_POINT('Ctrl Pts',(-0.319064633440148,2.05462363918519,
9.60284036503596));
#64721=CARTESIAN_POINT('Ctrl Pts',(-0.318943106250876,2.05377442604973,
9.60289345872754));
#64722=CARTESIAN_POINT('Ctrl Pts',(-0.318859812351775,2.05320332499879,
9.60292909132913));
#64723=CARTESIAN_POINT('Ctrl Pts',(-0.318241105588632,2.04903954156366,
9.60318836732557));
#64724=CARTESIAN_POINT('Ctrl Pts',(-0.317646494603501,2.04545573560968,
9.60340873532879));
#64725=CARTESIAN_POINT('Ctrl Pts',(-0.316854094961741,2.04113373003469,
9.6036719407541));
#64726=CARTESIAN_POINT('Ctrl Pts',(-0.316714147963807,2.04038537314566,
9.6037174218293));
#64727=CARTESIAN_POINT('Ctrl Pts',(-0.316373113190074,2.03859681355242,
9.60382591321105));
#64728=CARTESIAN_POINT('Ctrl Pts',(-0.3161695442495,2.0375570868723,9.60388881331254));
#64729=CARTESIAN_POINT('Ctrl Pts',(-0.314510419600608,2.02929928953474,
9.60438717973276));
#64730=CARTESIAN_POINT('Ctrl Pts',(-0.312812907351446,2.02213156428149,
9.60481246343778));
#64731=CARTESIAN_POINT('Ctrl Pts',(-0.310407601730414,2.01333173463978,
9.60533234307907));
#64732=CARTESIAN_POINT('Ctrl Pts',(-0.309930110064764,2.01163940681742,
9.60543221748913));
#64733=CARTESIAN_POINT('Ctrl Pts',(-0.304111048579226,1.9916431331841,9.60661192046668));
#64734=CARTESIAN_POINT('Ctrl Pts',(-0.297169078320852,1.97384412868202,
9.60766043382897));
#64735=CARTESIAN_POINT('Ctrl Pts',(-0.281881698283323,1.94303241663747,
9.60961232575473));
#64736=CARTESIAN_POINT('Ctrl Pts',(-0.274099228679788,1.92980706379206,
9.61050088783487));
#64737=CARTESIAN_POINT('Ctrl Pts',(-0.264022154742173,1.91517730134154,
9.61157251296456));
#64738=CARTESIAN_POINT('Ctrl Pts',(-0.262615427799732,1.91318387459762,
9.61172052944944));
#64739=CARTESIAN_POINT('Ctrl Pts',(-0.260772342886741,1.91063405802477,
9.61191253060131));
#64740=CARTESIAN_POINT('Ctrl Pts',(-0.260356574365398,1.91006282889596,
9.61195571923108));
#64741=CARTESIAN_POINT('Ctrl Pts',(-0.259682522801638,1.90914311349617,
9.61202554089117));
#64742=CARTESIAN_POINT('Ctrl Pts',(-0.25942540712087,1.90879377125256,9.61205212853279));
#64743=CARTESIAN_POINT('Ctrl Pts',(-0.258933635397163,1.90812842052553,
9.61210289491117));
#64744=CARTESIAN_POINT('Ctrl Pts',(-0.258699103999483,1.90781232053615,
9.61212706875809));
#64745=CARTESIAN_POINT('Ctrl Pts',(-0.258162067194254,1.90709126981355,
9.61218233840468));
#64746=CARTESIAN_POINT('Ctrl Pts',(-0.257859187540174,1.9066866002662,9.61221344881301));
#64747=CARTESIAN_POINT('Ctrl Pts',(-0.256928958667069,1.90544982190382,
9.61230881347616));
#64748=CARTESIAN_POINT('Ctrl Pts',(-0.256298529013032,1.90462004815259,
9.61237318862474));
#64749=CARTESIAN_POINT('Ctrl Pts',(-0.251586643897813,1.89848029776362,
9.61285247640672));
#64750=CARTESIAN_POINT('Ctrl Pts',(-0.247344839087903,1.89329598574655,
9.61327373487159));
#64751=CARTESIAN_POINT('Ctrl Pts',(-0.241631033473346,1.8867404923346,9.61382902560213));
#64752=CARTESIAN_POINT('Ctrl Pts',(-0.240303223799621,1.8852454091279,9.61395725866386));
#64753=CARTESIAN_POINT('Ctrl Pts',(-0.222006648773894,1.86502604300508,
9.6157133478048));
#64754=CARTESIAN_POINT('Ctrl Pts',(-0.202908828305303,1.84835076034038,
9.6174303130816));
#64755=CARTESIAN_POINT('Ctrl Pts',(-0.174981527945144,1.82923012579209,
9.61971458589249));
#64756=CARTESIAN_POINT('Ctrl Pts',(-0.167707311502605,1.82466541746763,
9.62029063096817));
#64757=CARTESIAN_POINT('Ctrl Pts',(-0.156043522334113,1.81798013377205,
9.62117671884305));
#64758=CARTESIAN_POINT('Ctrl Pts',(-0.151773515398532,1.81565937506084,
9.62149357783868));
#64759=CARTESIAN_POINT('Ctrl Pts',(-0.145376582416376,1.81236781300317,
9.62195554228492));
#64760=CARTESIAN_POINT('Ctrl Pts',(-0.143289114450342,1.81132222789547,
9.62210433035351));
#64761=CARTESIAN_POINT('Ctrl Pts',(-0.140353544793918,1.80989152931229,
9.62231064997974));
#64762=CARTESIAN_POINT('Ctrl Pts',(-0.139514912643606,1.80948729545792,
9.62236926126176));
#64763=CARTESIAN_POINT('Ctrl Pts',(-0.138056809206751,1.80879223681351,
9.62247058028614));
#64764=CARTESIAN_POINT('Ctrl Pts',(-0.137438146598455,1.80849974307325,
9.62251338692643));
#64765=CARTESIAN_POINT('Ctrl Pts',(-0.1366045121888,1.80810885803212,9.62257081835119));
#64766=CARTESIAN_POINT('Ctrl Pts',(-0.136390362850642,1.8080087322676,9.62258554959852));
#64767=CARTESIAN_POINT('Ctrl Pts',(-0.135990948615336,1.80782252096879,
9.62261298368893));
#64768=CARTESIAN_POINT('Ctrl Pts',(-0.135805711858567,1.80773637587705,
9.62262569022769));
#64769=CARTESIAN_POINT('Ctrl Pts',(-0.135420355718909,1.80755760993318,
9.62265208950303));
#64770=CARTESIAN_POINT('Ctrl Pts',(-0.135220223738272,1.80746501859875,
9.62266578031125));
#64771=CARTESIAN_POINT('Ctrl Pts',(-0.134759809839212,1.80725258090561,
9.62269723224165));
#64772=CARTESIAN_POINT('Ctrl Pts',(-0.134499462249459,1.80713287587977,
9.62271498455661));
#64773=CARTESIAN_POINT('Ctrl Pts',(-0.133692887145491,1.8067633236822,9.62276988256546));
#64774=CARTESIAN_POINT('Ctrl Pts',(-0.133146116560625,1.80651465442079,
9.62280695577378));
#64775=CARTESIAN_POINT('Ctrl Pts',(-0.128632955691229,1.80447729369562,
9.62311182498411));
#64776=CARTESIAN_POINT('Ctrl Pts',(-0.124631175558136,1.80276746166572,
9.62337489751965));
#64777=CARTESIAN_POINT('Ctrl Pts',(-0.119557146071901,1.80071999931101,
9.62370090705481));
#64778=CARTESIAN_POINT('Ctrl Pts',(-0.118516340536975,1.80030631124409,
9.62376738488982));
#64779=CARTESIAN_POINT('Ctrl Pts',(-0.115374747326695,1.79907655050822,
9.62396691745769));
#64780=CARTESIAN_POINT('Ctrl Pts',(-0.113267499666749,1.79827706622264,
9.62409924544897));
#64781=CARTESIAN_POINT('Ctrl Pts',(-0.107193139454431,1.79604507734008,
9.62447684055135));
#64782=CARTESIAN_POINT('Ctrl Pts',(-0.103205976426813,1.7946682247101,9.62472001124117));
#64783=CARTESIAN_POINT('Ctrl Pts',(-0.0838983303295262,1.78842232724667,
9.62588017845485));
#64784=CARTESIAN_POINT('Ctrl Pts',(-0.0682545337282205,1.78462571766052,
9.62676910178737));
#64785=CARTESIAN_POINT('Ctrl Pts',(-0.0502815599184166,1.78166445983123,
9.62779061851345));
#64786=CARTESIAN_POINT('Ctrl Pts',(-0.0481675119212139,1.78133773035714,
9.62791075662132));
#64787=CARTESIAN_POINT('Ctrl Pts',(-0.0361458714139469,1.77960212916412,
9.62859439336849));
#64788=CARTESIAN_POINT('Ctrl Pts',(-0.0261806462749892,1.77863436023969,
9.62916310060311));
#64789=CARTESIAN_POINT('Ctrl Pts',(-0.0076000591459639,1.77769992674078,
9.63024285808662));
#64790=CARTESIAN_POINT('Ctrl Pts',(0.00100011120099212,1.77761191297262,
9.63075026980546));
#64791=CARTESIAN_POINT('Ctrl Pts',(0.0121569598886418,1.77794416064751,
9.63142311694115));
#64792=CARTESIAN_POINT('Ctrl Pts',(0.014719855418881,1.77805112113135,9.63157867013347));
#64793=CARTESIAN_POINT('Ctrl Pts',(0.0179994393702184,1.77822723353041,
9.63177907620164));
#64794=CARTESIAN_POINT('Ctrl Pts',(0.0187175976236789,1.77826821017325,
9.63182304394822));
#64795=CARTESIAN_POINT('Ctrl Pts',(0.0198714429416238,1.77833792261787,
9.63189382141325));
#64796=CARTESIAN_POINT('Ctrl Pts',(0.0203072220930385,1.77836514026265,
9.63192058344464));
#64797=CARTESIAN_POINT('Ctrl Pts',(0.0211350983192706,1.77841853649556,
9.63197148454883));
#64798=CARTESIAN_POINT('Ctrl Pts',(0.0215272057644241,1.77844454683457,
9.63199561829509));
#64799=CARTESIAN_POINT('Ctrl Pts',(0.0224182961810345,1.77850529426981,
9.63205052208679));
#64800=CARTESIAN_POINT('Ctrl Pts',(0.0229172469440312,1.77854047594726,
9.63208130604097));
#64801=CARTESIAN_POINT('Ctrl Pts',(0.024395816212228,1.77864819170939,9.63217265407773));
#64802=CARTESIAN_POINT('Ctrl Pts',(0.0253751806253729,1.77872404273846,
9.63223332220271));
#64803=CARTESIAN_POINT('Ctrl Pts',(0.0320688451450753,1.77927325943073,
9.63264909427837));
#64804=CARTESIAN_POINT('Ctrl Pts',(0.0377696635335392,1.77989455074883,
9.63300882543525));
#64805=CARTESIAN_POINT('Ctrl Pts',(0.0437967519519885,1.78071463831535,
9.63339546789787));
#64806=CARTESIAN_POINT('Ctrl Pts',(0.0441428303656283,1.78076230142191,
9.63341769119958));
#64807=CARTESIAN_POINT('Ctrl Pts',(0.0677143896289908,1.78404772017893,
9.63493283839322));
#64808=CARTESIAN_POINT('Ctrl Pts',(0.0905134820693072,1.789809683876,9.63650595581321));
#64809=CARTESIAN_POINT('Ctrl Pts',(0.124812493549504,1.80258420156764,9.63898282532728));
#64810=CARTESIAN_POINT('Ctrl Pts',(0.136851079331668,1.80792786370775,9.63987346420303));
#64811=CARTESIAN_POINT('Ctrl Pts',(0.152804503187828,1.81621282385161,9.64105793674554));
#64812=CARTESIAN_POINT('Ctrl Pts',(0.157029198863677,1.81852848583413,9.64137195711746));
#64813=CARTESIAN_POINT('Ctrl Pts',(0.163206786996482,1.82209698088708,9.64182999402412));
#64814=CARTESIAN_POINT('Ctrl Pts',(0.165200474983747,1.82327749076189,9.6419776339886));
#64815=CARTESIAN_POINT('Ctrl Pts',(0.167972782795711,1.82495968130117,9.64218249223668));
#64816=CARTESIAN_POINT('Ctrl Pts',(0.168762181530821,1.82544334135998,9.64224077373028));
#64817=CARTESIAN_POINT('Ctrl Pts',(0.170128254952208,1.82628844443987,9.6423415281116));
#64818=CARTESIAN_POINT('Ctrl Pts',(0.170705884343607,1.8266483220269,9.64238409880506));
#64819=CARTESIAN_POINT('Ctrl Pts',(0.171536094664468,1.82716922173726,9.64244523302585));
#64820=CARTESIAN_POINT('Ctrl Pts',(0.171789592886376,1.82732876734451,9.64246389295051));
#64821=CARTESIAN_POINT('Ctrl Pts',(0.172231289517532,1.8276076209064,9.64249639348975));
#64822=CARTESIAN_POINT('Ctrl Pts',(0.172419587034698,1.82772677089896,9.64251024462435));
#64823=CARTESIAN_POINT('Ctrl Pts',(0.172782171318709,1.8279567322029,9.64253690832689));
#64824=CARTESIAN_POINT('Ctrl Pts',(0.172956474762788,1.82806751551614,9.64254972272716));
#64825=CARTESIAN_POINT('Ctrl Pts',(0.173370103738522,1.82833096728078,9.6425801237524));
#64826=CARTESIAN_POINT('Ctrl Pts',(0.173609334766229,1.8284837848445,9.64259770041354));
#64827=CARTESIAN_POINT('Ctrl Pts',(0.174451010046514,1.82902300289317,9.6426595181164));
#64828=CARTESIAN_POINT('Ctrl Pts',(0.175052374439053,1.82941109761541,9.64270364720757));
#64829=CARTESIAN_POINT('Ctrl Pts',(0.183194095914158,1.83470391641883,9.6433006448549));
#64830=CARTESIAN_POINT('Ctrl Pts',(0.190527998055029,1.83992077136793,9.64383312506809));
#64831=CARTESIAN_POINT('Ctrl Pts',(0.216893752261523,1.8603904120473,9.64576569496135));
#64832=CARTESIAN_POINT('Ctrl Pts',(0.234394833718438,1.87748059127205,9.64709132827387));
#64833=CARTESIAN_POINT('Ctrl Pts',(0.259513590099184,1.90829672842963,9.64934713552132));
#64834=CARTESIAN_POINT('Ctrl Pts',(0.268359252205346,1.92088923103108,9.65023808329113));
#64835=CARTESIAN_POINT('Ctrl Pts',(0.277530494507211,1.93615869645021,9.65131255051548));
#64836=CARTESIAN_POINT('Ctrl Pts',(0.278764921540662,1.93826791864038,9.65146081333302));
#64837=CARTESIAN_POINT('Ctrl Pts',(0.280325336210399,1.94100509040068,9.65165308969602));
#64838=CARTESIAN_POINT('Ctrl Pts',(0.280673433229465,1.94162039504213,9.65169630436787));
#64839=CARTESIAN_POINT('Ctrl Pts',(0.28123188701732,1.94261515453396,9.65176615797292));
#64840=CARTESIAN_POINT('Ctrl Pts',(0.281443508322857,1.94299389987107,9.65179275144132));
#64841=CARTESIAN_POINT('Ctrl Pts',(0.281845645913678,1.94371704375871,9.65184352221876));
#64842=CARTESIAN_POINT('Ctrl Pts',(0.282036297505233,1.94406136649512,9.65186769462323));
#64843=CARTESIAN_POINT('Ctrl Pts',(0.282470267050254,1.94484852830807,9.65192295155037));
#64844=CARTESIAN_POINT('Ctrl Pts',(0.282713174801769,1.94529159129355,9.65195405065742));
#64845=CARTESIAN_POINT('Ctrl Pts',(0.283453424575645,1.94664936981929,9.65204934708391));
#64846=CARTESIAN_POINT('Ctrl Pts',(0.283947372955939,1.94756591906286,9.65211366504469));
#64847=CARTESIAN_POINT('Ctrl Pts',(0.287576036548408,1.95437794819383,9.65259163766534));
#64848=CARTESIAN_POINT('Ctrl Pts',(0.290531097615571,1.96036680430612,9.65301159912822));
#64849=CARTESIAN_POINT('Ctrl Pts',(0.294156953708207,1.96832935245155,9.65357023009964));
#64850=CARTESIAN_POINT('Ctrl Pts',(0.29499779666557,1.97022414518271,9.65370317838104));
#64851=CARTESIAN_POINT('Ctrl Pts',(0.305847921418465,1.99532470676818,9.65546456822883));
#64852=CARTESIAN_POINT('Ctrl Pts',(0.313110758852136,2.01961877240534,9.65718200063609));
#64853=CARTESIAN_POINT('Ctrl Pts',(0.320268831644503,2.06056772313276,9.65998738362136));
#64854=CARTESIAN_POINT('Ctrl Pts',(0.321853887246089,2.07682140030427,9.66107582920751));
#64855=CARTESIAN_POINT('Ctrl Pts',(0.322215262751302,2.09376267499009,9.66214167892647));
#64856=CARTESIAN_POINT('Ctrl Pts',(0.322226939854633,2.09439830194317,9.6621815673453));
#64857=CARTESIAN_POINT('Ctrl Pts',(0.322244471416836,2.09553589239932,9.6622527692901));
#64858=CARTESIAN_POINT('Ctrl Pts',(0.322251034004431,2.0960378406693,9.6622841211853));
#64859=CARTESIAN_POINT('Ctrl Pts',(0.322259260764259,2.0968040192095,9.66233187551054));
#64860=CARTESIAN_POINT('Ctrl Pts',(0.322261772797697,2.09706823670336,9.66234832521787));
#64861=CARTESIAN_POINT('Ctrl Pts',(0.322265765375423,2.09755057736286,9.66237832088129));
#64862=CARTESIAN_POINT('Ctrl Pts',(0.322267349413251,2.09776869829432,9.66239187260473));
#64863=CARTESIAN_POINT('Ctrl Pts',(0.322270087853262,2.09820706682223,9.66241908258498));
#64864=CARTESIAN_POINT('Ctrl Pts',(0.322271237920267,2.09842731300957,9.66243274054373));
#64865=CARTESIAN_POINT('Ctrl Pts',(0.322273874681947,2.09905562592237,9.66247166713947));
#64866=CARTESIAN_POINT('Ctrl Pts',(0.32227481212114,2.09946369639774,9.66249690488908));
#64867=CARTESIAN_POINT('Ctrl Pts',(0.322275506782068,2.10120956097637,9.66260469689603));
#64868=CARTESIAN_POINT('Ctrl Pts',(0.322267709156086,2.10254736943902,9.66268683354602));
#64869=CARTESIAN_POINT('Ctrl Pts',(0.321951589917165,2.12876791924119,9.66428831208858));
#64870=CARTESIAN_POINT('Ctrl Pts',(0.318770551402111,2.15353685246092,9.66565743017571));
#64871=CARTESIAN_POINT('Ctrl Pts',(0.306800021331985,2.20172479472154,9.6684354142871));
#64872=CARTESIAN_POINT('Ctrl Pts',(0.298083129666597,2.22498148203089,9.66983795219054));
#64873=CARTESIAN_POINT('Ctrl Pts',(0.286265095832769,2.24803648785005,9.67141335290156));
#64874=CARTESIAN_POINT('Ctrl Pts',(0.285733281451517,2.24906038589736,9.67148370389835));
#64875=CARTESIAN_POINT('Ctrl Pts',(0.28495057673139,2.25054774042919,9.67158647004403));
#64876=CARTESIAN_POINT('Ctrl Pts',(0.284704025456033,2.25101348023208,9.67161873158768));
#64877=CARTESIAN_POINT('Ctrl Pts',(0.284269884461784,2.2518287382732,9.67167534896254));
#64878=CARTESIAN_POINT('Ctrl Pts',(0.284082789190552,2.25217851970955,9.6716996872001));
#64879=CARTESIAN_POINT('Ctrl Pts',(0.283718663239946,2.25285625485431,9.67174693631743));
#64880=CARTESIAN_POINT('Ctrl Pts',(0.283541708444874,2.25318424882833,9.67176984446861));
#64881=CARTESIAN_POINT('Ctrl Pts',(0.283118528240819,2.25396538753692,9.67182450147889));
#64882=CARTESIAN_POINT('Ctrl Pts',(0.28287178384129,2.25441824857883,9.67185626882006));
#64883=CARTESIAN_POINT('Ctrl Pts',(0.282124383929233,2.2557821823214,9.67195218965671));
#64884=CARTESIAN_POINT('Ctrl Pts',(0.281620409717601,2.2566914200783,9.67201646177737));
#64885=CARTESIAN_POINT('Ctrl Pts',(0.276344230003707,2.26610268074635,9.67268517407986));
#64886=CARTESIAN_POINT('Ctrl Pts',(0.271193412625119,2.27438558959964,9.67330326804845));
#64887=CARTESIAN_POINT('Ctrl Pts',(0.261509293112508,2.28848936287505,9.67441054044638));
#64888=CARTESIAN_POINT('Ctrl Pts',(0.257136625599697,2.29441217568341,9.67489382549423));
#64889=CARTESIAN_POINT('Ctrl Pts',(0.238615214911081,2.31778049432349,9.67687366376702));
#64890=CARTESIAN_POINT('Ctrl Pts',(0.222864766559749,2.33387339158329,9.67841484158103));
#64891=CARTESIAN_POINT('Ctrl Pts',(0.197911726851365,2.35454078085146,9.68057325155991));
#64892=CARTESIAN_POINT('Ctrl Pts',(0.189963004524117,2.3605266976066,9.6812247720704));
#64893=CARTESIAN_POINT('Ctrl Pts',(0.180958338940764,2.36667615704189,9.68191393890143));
#64894=CARTESIAN_POINT('Ctrl Pts',(0.180164898438415,2.36721284136648,9.68197426281579));
#64895=CARTESIAN_POINT('Ctrl Pts',(0.178787591654736,2.36813553018986,9.68207826765918));
#64896=CARTESIAN_POINT('Ctrl Pts',(0.178204844040433,2.3685231816104,9.68212205462098));
#64897=CARTESIAN_POINT('Ctrl Pts',(0.177368225348745,2.36907578841551,9.6821845999154));
#64898=CARTESIAN_POINT('Ctrl Pts',(0.177115382723512,2.36924228583061,9.68220346099222));
#64899=CARTESIAN_POINT('Ctrl Pts',(0.176678980784834,2.36952877669255,9.6822359431325));
#64900=CARTESIAN_POINT('Ctrl Pts',(0.176495533225426,2.36964893930644,9.68224957563233));
#64901=CARTESIAN_POINT('Ctrl Pts',(0.176140324807471,2.36988109167672,9.68227592976769));
#64902=CARTESIAN_POINT('Ctrl Pts',(0.175968579954325,2.36999310461074,9.68228865298913));
#64903=CARTESIAN_POINT('Ctrl Pts',(0.17556363916719,2.37025665870057,9.68231860712343));
#64904=CARTESIAN_POINT('Ctrl Pts',(0.175330353299151,2.37040806234831,9.68233582875854));
#64905=CARTESIAN_POINT('Ctrl Pts',(0.174640333455753,2.37085462018545,9.68238666526919));
#64906=CARTESIAN_POINT('Ctrl Pts',(0.174183045180023,2.37114892241593,9.68242022347555));
#64907=CARTESIAN_POINT('Ctrl Pts',(0.170154189514572,2.37372742101109,9.68271474276128));
#64908=CARTESIAN_POINT('Ctrl Pts',(0.166538410301764,2.37594222461734,9.68297120683739));
#64909=CARTESIAN_POINT('Ctrl Pts',(0.162356524760671,2.37839163458479,9.68326020257542));
#64910=CARTESIAN_POINT('Ctrl Pts',(0.161832410481271,2.37869663483361,9.68329628750687));
#64911=CARTESIAN_POINT('Ctrl Pts',(0.15904979780779,2.38030543720248,9.68348717209885));
#64912=CARTESIAN_POINT('Ctrl Pts',(0.15677633734971,2.38158330403717,9.68364070339821));
#64913=CARTESIAN_POINT('Ctrl Pts',(0.149981342156572,2.3852948244332,9.68409317572655));
#64914=CARTESIAN_POINT('Ctrl Pts',(0.145416761874995,2.38764823919489,9.68438882259132));
#64915=CARTESIAN_POINT('Ctrl Pts',(0.121561678236722,2.39923443416423,9.68590119894104));
#64916=CARTESIAN_POINT('Ctrl Pts',(0.101443229204911,2.406639562047,9.68707168908333));
#64917=CARTESIAN_POINT('Ctrl Pts',(0.0695304733343461,2.41489797057564,
9.6889442843749));
#64918=CARTESIAN_POINT('Ctrl Pts',(0.0581748171368487,2.41719216728342,
9.68961281322766));
#64919=CARTESIAN_POINT('Ctrl Pts',(0.0413260937403642,2.41966085187465,
9.69062409246578));
#64920=CARTESIAN_POINT('Ctrl Pts',(0.0359121933148562,2.42031424441174,
9.69095186100929));
#64921=CARTESIAN_POINT('Ctrl Pts',(0.0295793738233886,2.42091597502776,
9.69133939689434));
#64922=CARTESIAN_POINT('Ctrl Pts',(0.0286738354842033,2.42099815188848,
9.69139490884812));
#64923=CARTESIAN_POINT('Ctrl Pts',(0.0272915038827543,2.42111770140799,
9.69147980256366));
#64924=CARTESIAN_POINT('Ctrl Pts',(0.0268149499466486,2.42115784716734,
9.69150909710441));
#64925=CARTESIAN_POINT('Ctrl Pts',(0.0259861122009029,2.42122581228064,
9.69156009594456));
#64926=CARTESIAN_POINT('Ctrl Pts',(0.0256338678025295,2.42125411331618,
9.69158178506865));
#64927=CARTESIAN_POINT('Ctrl Pts',(0.0248995719417467,2.42131189485429,
9.69162703090765));
#64928=CARTESIAN_POINT('Ctrl Pts',(0.0245175132111387,2.42134127341768,
9.69165059079047));
#64929=CARTESIAN_POINT('Ctrl Pts',(0.0235826274313552,2.42141148485099,
9.69170828600677));
#64930=CARTESIAN_POINT('Ctrl Pts',(0.0230297471775385,2.42145157279051,
9.69174244468525));
#64931=CARTESIAN_POINT('Ctrl Pts',(0.0209124089596778,2.42159960503841,
9.69187340946448));
#64932=CARTESIAN_POINT('Ctrl Pts',(0.0193472941819304,2.42169755497616,
9.69197052875342));
#64933=CARTESIAN_POINT('Ctrl Pts',(-0.00686478916152614,2.42314601520544,
9.69360243189247));
#64934=CARTESIAN_POINT('Ctrl Pts',(-0.0315806032064484,2.42167164901584,
9.69523050539107));
#64935=CARTESIAN_POINT('Ctrl Pts',(-0.0716019339014607,2.41462541349623,
9.6979739930568));
#64936=CARTESIAN_POINT('Ctrl Pts',(-0.0870959446429602,2.41069327699743,
9.69906119939571));
#64937=CARTESIAN_POINT('Ctrl Pts',(-0.110216104805449,2.40295941855171,
9.70067542809187));
#64938=CARTESIAN_POINT('Ctrl Pts',(-0.118090272894714,2.39997785619139,
9.70122338454239));
#64939=CARTESIAN_POINT('Ctrl Pts',(-0.127048357691948,2.39617835001626,
9.70183762162377));
#64940=CARTESIAN_POINT('Ctrl Pts',(-0.128254220233477,2.39565817313808,
9.70192010783991));
#64941=CARTESIAN_POINT('Ctrl Pts',(-0.129812836578354,2.39497449746875,
9.70202643575861));
#64942=CARTESIAN_POINT('Ctrl Pts',(-0.130168498951857,2.39481772094273,
9.70205067931136));
#64943=CARTESIAN_POINT('Ctrl Pts',(-0.130743614574762,2.39456296547718,
9.70208984911431));
#64944=CARTESIAN_POINT('Ctrl Pts',(-0.130963242017428,2.39446538442401,
9.70210479970951));
#64945=CARTESIAN_POINT('Ctrl Pts',(-0.131384167197612,2.39427780217893,
9.70213343803841));
#64946=CARTESIAN_POINT('Ctrl Pts',(-0.131585481074299,2.39418784036079,
9.70214712808035));
#64947=CARTESIAN_POINT('Ctrl Pts',(-0.132048121301452,2.39398052885806,
9.70217857413504));
#64948=CARTESIAN_POINT('Ctrl Pts',(-0.132309384380341,2.39386303696335,
9.7021963213514));
#64949=CARTESIAN_POINT('Ctrl Pts',(-0.133117600435273,2.39349828002055,
9.7022511890696));
#64950=CARTESIAN_POINT('Ctrl Pts',(-0.133664023498712,2.39324983334435,
9.70228823720047));
#64951=CARTESIAN_POINT('Ctrl Pts',(-0.138156680864627,2.39119195371399,
9.70259248181589));
#64952=CARTESIAN_POINT('Ctrl Pts',(-0.142066911009777,2.38930437203179,
9.70285497621379));
#64953=CARTESIAN_POINT('Ctrl Pts',(-0.14689292630858,2.38685325666065,9.70317750791687));
#64954=CARTESIAN_POINT('Ctrl Pts',(-0.14784540715445,2.38636350727143,9.7032410929945));
#64955=CARTESIAN_POINT('Ctrl Pts',(-0.149430478977077,2.38553847395275,
9.70334681858821));
#64956=CARTESIAN_POINT('Ctrl Pts',(-0.150064419122236,2.38520581740939,
9.70338907886743));
#64957=CARTESIAN_POINT('Ctrl Pts',(-0.152724417639674,2.38379867384474,
9.70356632267326));
#64958=CARTESIAN_POINT('Ctrl Pts',(-0.154740126592792,2.38270466695156,
9.70370044158105));
#64959=CARTESIAN_POINT('Ctrl Pts',(-0.161481743353048,2.37895200834256,
9.7041489224728));
#64960=CARTESIAN_POINT('Ctrl Pts',(-0.166152336016913,2.37619555069267,
9.70445949578441));
#64961=CARTESIAN_POINT('Ctrl Pts',(-0.179231155407598,2.36802488752522,
9.70533497675114));
#64962=CARTESIAN_POINT('Ctrl Pts',(-0.187460092760589,2.36233541870357,
9.70589297686367));
#64963=CARTESIAN_POINT('Ctrl Pts',(-0.203056072827663,2.3504432621868,9.70698924188116));
#64964=CARTESIAN_POINT('Ctrl Pts',(-0.210435944569906,2.34427505366086,
9.70752688782505));
#64965=CARTESIAN_POINT('Ctrl Pts',(-0.228924020742574,2.32736201188725,
9.70894832220236));
#64966=CARTESIAN_POINT('Ctrl Pts',(-0.239553668861767,2.3161333811544,9.70984326695604));
#64967=CARTESIAN_POINT('Ctrl Pts',(-0.250889476024387,2.30229100929007,
9.71092249646669));
#64968=CARTESIAN_POINT('Ctrl Pts',(-0.252420486900822,2.30037734128407,
9.71107117090017));
#64969=CARTESIAN_POINT('Ctrl Pts',(-0.25436524669452,2.29788885184356,9.71126390705666));
#64970=CARTESIAN_POINT('Ctrl Pts',(-0.254799161135035,2.29732983525618,
9.71130716515514));
#64971=CARTESIAN_POINT('Ctrl Pts',(-0.255496223572909,2.29642566974901,
9.71137707203077));
#64972=CARTESIAN_POINT('Ctrl Pts',(-0.255760523333499,2.29608140834261,
9.71140367521613));
#64973=CARTESIAN_POINT('Ctrl Pts',(-0.256263148569348,2.29542397290897,
9.71145445334595));
#64974=CARTESIAN_POINT('Ctrl Pts',(-0.25650159757932,2.29511089395335,9.71147862336127));
#64975=CARTESIAN_POINT('Ctrl Pts',(-0.25704470366133,2.2943950898266,9.71153385915595));
#64976=CARTESIAN_POINT('Ctrl Pts',(-0.257348988279848,2.29399208451827,
9.71156493947937));
#64977=CARTESIAN_POINT('Ctrl Pts',(-0.258276833755342,2.29275718830385,
9.71166012255043));
#64978=CARTESIAN_POINT('Ctrl Pts',(-0.258897312791394,2.2919229998888,9.71172434552073));
#64979=CARTESIAN_POINT('Ctrl Pts',(-0.263452869759912,2.28573609627654,
9.71220014117438));
#64980=CARTESIAN_POINT('Ctrl Pts',(-0.267225378558869,2.28026618793135,
9.71261795633226));
#64981=CARTESIAN_POINT('Ctrl Pts',(-0.271829750123041,2.27312767567176,
9.7131602462047));
#64982=CARTESIAN_POINT('Ctrl Pts',(-0.272820089718979,2.27156282685928,
9.71327894152324));
#64983=CARTESIAN_POINT('Ctrl Pts',(-0.281416262211291,2.25771724002261,
9.71432756605408));
#64984=CARTESIAN_POINT('Ctrl Pts',(-0.288201062742526,2.24494792928204,
9.71528495834222));
#64985=CARTESIAN_POINT('Ctrl Pts',(-0.300859456614982,2.21669440842931,
9.7173676534232));
#64986=CARTESIAN_POINT('Ctrl Pts',(-0.306444003449681,2.20112404943818,
9.71849456135099));
#64987=CARTESIAN_POINT('Ctrl Pts',(-0.312946266858358,2.17740212115723,
9.72013459231386));
#64988=CARTESIAN_POINT('Ctrl Pts',(-0.314788507213134,2.16953179872205,
9.72066632354187));
#64989=CARTESIAN_POINT('Ctrl Pts',(-0.316979362341212,2.15828114388953,
9.72140167119534));
#64990=CARTESIAN_POINT('Ctrl Pts',(-0.31757340398167,2.15495219027247,9.72161621065504));
#64991=CARTESIAN_POINT('Ctrl Pts',(-0.31819849644698,2.15109955449355,9.72186051960799));
#64992=CARTESIAN_POINT('Ctrl Pts',(-0.318280772477322,2.15058455783018,
9.72189309549596));
#64993=CARTESIAN_POINT('Ctrl Pts',(-0.318403650038842,2.14980325121976,
9.72194239029906));
#64994=CARTESIAN_POINT('Ctrl Pts',(-0.318445167899288,2.14953708946823,
9.72195916095425));
#64995=CARTESIAN_POINT('Ctrl Pts',(-0.318516492815986,2.14907604605006,
9.72198817209834));
#64996=CARTESIAN_POINT('Ctrl Pts',(-0.318546454713478,2.14888118944879,
9.72200042141288));
#64997=CARTESIAN_POINT('Ctrl Pts',(-0.318608694726064,2.14847392523885,
9.72202599815512));
#64998=CARTESIAN_POINT('Ctrl Pts',(-0.318640939144057,2.14826151349862,
9.72203932361471));
#64999=CARTESIAN_POINT('Ctrl Pts',(-0.318719844368782,2.14773819508709,
9.72207211869405));
#65000=CARTESIAN_POINT('Ctrl Pts',(-0.318766262804444,2.14742725128325,
9.72209157450558));
#65001=CARTESIAN_POINT('Ctrl Pts',(-0.318945597953094,2.14621377924434,
9.72216738532989));
#65002=CARTESIAN_POINT('Ctrl Pts',(-0.319075138935293,2.1453107449331,9.7222235507548));
#65003=CARTESIAN_POINT('Ctrl Pts',(-0.321235572864455,2.12978143980146,
9.7231852928539));
#65004=CARTESIAN_POINT('Ctrl Pts',(-0.322262972831485,2.11503094359889,
9.7240362840308));
#65005=CARTESIAN_POINT('Ctrl Pts',(-0.322300767273116,2.06820607996235,
9.72668330494058));
#65006=CARTESIAN_POINT('Ctrl Pts',(-0.317544968751828,2.03633060995106,
9.72842447962931));
#65007=CARTESIAN_POINT('Ctrl Pts',(-0.307477373763807,2.00343735682915,
9.7304832467373));
#65008=CARTESIAN_POINT('Ctrl Pts',(-0.306766309896965,2.00120166950783,
9.73062441121389));
#65009=CARTESIAN_POINT('Ctrl Pts',(-0.305444310734931,1.99719703144561,
9.73087960000979));
#65010=CARTESIAN_POINT('Ctrl Pts',(-0.304842251356212,1.99542524748887,
9.730993331519));
#65011=CARTESIAN_POINT('Ctrl Pts',(-0.304006080716402,1.99303309904718,
9.73114804232437));
#65012=CARTESIAN_POINT('Ctrl Pts',(-0.303785427008262,1.9924080424053,9.73118857507883));
#65013=CARTESIAN_POINT('Ctrl Pts',(-0.303434701125111,1.99142420426905,
9.7312525448391));
#65014=CARTESIAN_POINT('Ctrl Pts',(-0.303305916509385,1.99106496305656,
9.7312759389906));
#65015=CARTESIAN_POINT('Ctrl Pts',(-0.303056524254529,1.99037316079052,
9.73132105974718));
#65016=CARTESIAN_POINT('Ctrl Pts',(-0.302936006472565,1.99004056771163,
9.73134278333345));
#65017=CARTESIAN_POINT('Ctrl Pts',(-0.302650155580088,1.9892557414458,9.73139411890376));
#65018=CARTESIAN_POINT('Ctrl Pts',(-0.302484356422846,1.98880367995816,
9.73142374640063));
#65019=CARTESIAN_POINT('Ctrl Pts',(-0.301997176602442,1.9874845072084,9.73151037401496));
#65020=CARTESIAN_POINT('Ctrl Pts',(-0.301673078094324,1.98661841102477,
9.73156746486838));
#65021=CARTESIAN_POINT('Ctrl Pts',(-0.299281311234648,1.98030969217412,
9.73198491353995));
#65022=CARTESIAN_POINT('Ctrl Pts',(-0.297070335008483,1.97492289594797,
9.73235006275498));
#65023=CARTESIAN_POINT('Ctrl Pts',(-0.289269990753396,1.95729357993644,
9.73357532485345));
#65024=CARTESIAN_POINT('Ctrl Pts',(-0.283060489148429,1.94534253341921,
9.73445601783751));
#65025=CARTESIAN_POINT('Ctrl Pts',(-0.261621058323524,1.90971991670575,
9.73723009563142));
#65026=CARTESIAN_POINT('Ctrl Pts',(-0.244028179681372,1.88762691483951,
9.73917902711662));
#65027=CARTESIAN_POINT('Ctrl Pts',(-0.221170331638683,1.8655684991073,9.74122155877672));
#65028=CARTESIAN_POINT('Ctrl Pts',(-0.218506355108674,1.86308351732256,
9.74145307689391));
#65029=CARTESIAN_POINT('Ctrl Pts',(-0.215371676566136,1.86025732501612,
9.74171745831677));
#65030=CARTESIAN_POINT('Ctrl Pts',(-0.214941627583548,1.85987168842602,
9.74175355710316));
#65031=CARTESIAN_POINT('Ctrl Pts',(-0.214300963401061,1.85930028755412,
9.74180707716083));
#65032=CARTESIAN_POINT('Ctrl Pts',(-0.214091141458655,1.8591136416554,9.74182456441686));
#65033=CARTESIAN_POINT('Ctrl Pts',(-0.213717169702861,1.85878185182211,
9.74185565924366));
#65034=CARTESIAN_POINT('Ctrl Pts',(-0.213553115917034,1.85863660111901,
9.74186927488278));
#65035=CARTESIAN_POINT('Ctrl Pts',(-0.213204708513569,1.85832875985435,
9.74189813777571));
#65036=CARTESIAN_POINT('Ctrl Pts',(-0.213020317505783,1.85816621332701,
9.74191338170609));
#65037=CARTESIAN_POINT('Ctrl Pts',(-0.212525516932343,1.85773103591591,
9.74195420407385));
#65038=CARTESIAN_POINT('Ctrl Pts',(-0.212214767481759,1.85745878953687,
9.74197975365453));
#65039=CARTESIAN_POINT('Ctrl Pts',(-0.210729671253993,1.85616274171573,
9.74210144243915));
#65040=CARTESIAN_POINT('Ctrl Pts',(-0.209548408523966,1.85514684484544,
9.74219700117327));
#65041=CARTESIAN_POINT('Ctrl Pts',(-0.199734165937715,1.84682955171127,
9.74298125232645));
#65042=CARTESIAN_POINT('Ctrl Pts',(-0.19072877516724,1.83997768036777,9.74363963203563));
#65043=CARTESIAN_POINT('Ctrl Pts',(-0.15892139623462,1.81832030671233,9.74583449180678));
#65044=CARTESIAN_POINT('Ctrl Pts',(-0.134618638082729,1.80592964816968,
9.74730762375319));
#65045=CARTESIAN_POINT('Ctrl Pts',(-0.106281484435177,1.79574013115965,
9.74905205083636));
#65046=CARTESIAN_POINT('Ctrl Pts',(-0.103501078798846,1.79478311366284,
9.74922335098398));
#65047=CARTESIAN_POINT('Ctrl Pts',(-0.0990619497888775,1.79332279428349,
9.74949733525782));
#65048=CARTESIAN_POINT('Ctrl Pts',(-0.0974115587450161,1.79279458587281,
9.74959930415271));
#65049=CARTESIAN_POINT('Ctrl Pts',(-0.0896109569113862,1.79036717906932,
9.75008190877611));
#65050=CARTESIAN_POINT('Ctrl Pts',(-0.0834093462170028,1.78863930956249,
9.75046751725774));
#65051=CARTESIAN_POINT('Ctrl Pts',(-0.076160367902026,1.78685173636693,
9.75092193315365));
#65052=CARTESIAN_POINT('Ctrl Pts',(-0.0751590965736733,1.78660991269828,
9.75098477934524));
#65053=CARTESIAN_POINT('Ctrl Pts',(-0.073667119580352,1.78625713681564,
9.75107854952184));
#65054=CARTESIAN_POINT('Ctrl Pts',(-0.0731772788433954,1.78614252508037,
9.75110935569268));
#65055=CARTESIAN_POINT('Ctrl Pts',(-0.0723039980370705,1.78594035250311,
9.75116431261855));
#65056=CARTESIAN_POINT('Ctrl Pts',(-0.0719206614173105,1.78585234558072,
9.75118844898208));
#65057=CARTESIAN_POINT('Ctrl Pts',(-0.0711129818411954,1.7856684732704,
9.75123933012168));
#65058=CARTESIAN_POINT('Ctrl Pts',(-0.0706886042531613,1.78557276500231,
9.75126607988946));
#65059=CARTESIAN_POINT('Ctrl Pts',(-0.0695689524903573,1.78532263550188,
9.75133669605044));
#65060=CARTESIAN_POINT('Ctrl Pts',(-0.0688733608220415,1.78516965992118,
9.75138060872165));
#65061=CARTESIAN_POINT('Ctrl Pts',(-0.0657389434237606,1.78449121892634,
9.75157867745487));
#65062=CARTESIAN_POINT('Ctrl Pts',(-0.0632946256190451,1.78399178899606,
9.75173366448414));
#65063=CARTESIAN_POINT('Ctrl Pts',(-0.0452105093404361,1.78051502144944,
9.75288447522972));
#65064=CARTESIAN_POINT('Ctrl Pts',(-0.0293774122755313,1.77867232730593,
9.75391655261541));
#65065=CARTESIAN_POINT('Ctrl Pts',(0.0182164670955005,1.7766805863597,9.75708440028588));
#65066=CARTESIAN_POINT('Ctrl Pts',(0.0499282451455137,1.78003998795388,
9.75929698971051));
#65067=CARTESIAN_POINT('Ctrl Pts',(0.0821433670759884,1.78836550093969,
9.76140249415399));
#65068=CARTESIAN_POINT('Ctrl Pts',(0.0836461376065765,1.78876549411481,
9.7615003284772));
#65069=CARTESIAN_POINT('Ctrl Pts',(0.0855581871992815,1.78928927458937,
9.76162426648897));
#65070=CARTESIAN_POINT('Ctrl Pts',(0.0859701627662228,1.78940301128151,
9.76165093837499));
#65071=CARTESIAN_POINT('Ctrl Pts',(0.0866241935255073,1.78958497464807,
9.76169322881389));
#65072=CARTESIAN_POINT('Ctrl Pts',(0.086866395380693,1.78965266519142,9.7617088784478));
#65073=CARTESIAN_POINT('Ctrl Pts',(0.0873186854715271,1.78977964211888,
9.7617380810263));
#65074=CARTESIAN_POINT('Ctrl Pts',(0.0875287911310894,1.78983885801099,
9.76175163792258));
#65075=CARTESIAN_POINT('Ctrl Pts',(0.0880006895482849,1.78997237491008,
9.76178206715779));
#65076=CARTESIAN_POINT('Ctrl Pts',(0.0882624478338104,1.79004679388081,
9.76179893247027));
#65077=CARTESIAN_POINT('Ctrl Pts',(0.0890383013993388,1.79026843480901,
9.76184888207946));
#65078=CARTESIAN_POINT('Ctrl Pts',(0.0895521280628243,1.79041660580567,
9.76188191113579));
#65079=CARTESIAN_POINT('Ctrl Pts',(0.0936629554860278,1.79161312640784,
9.76214576469217));
#65080=CARTESIAN_POINT('Ctrl Pts',(0.0972419811627356,1.79272290501854,
9.76237307565771));
#65081=CARTESIAN_POINT('Ctrl Pts',(0.11156924178437,1.79744090082164,9.76327632329368));
#65082=CARTESIAN_POINT('Ctrl Pts',(0.122143946869559,1.80155300183936,9.76392779428118));
#65083=CARTESIAN_POINT('Ctrl Pts',(0.163961068408712,1.82041017204418,9.76652284785366));
#65084=CARTESIAN_POINT('Ctrl Pts',(0.192951955020495,1.83957111075647,9.76839450543246));
#65085=CARTESIAN_POINT('Ctrl Pts',(0.218703677811659,1.86329320329376,9.77051183125216));
#65086=CARTESIAN_POINT('Ctrl Pts',(0.219056193903442,1.86361939545728,9.77054090819852));
#65087=CARTESIAN_POINT('Ctrl Pts',(0.22058720489933,1.86504244508946,9.77066759887071));
#65088=CARTESIAN_POINT('Ctrl Pts',(0.221758184847625,1.86614732226996,9.7707655495504));
#65089=CARTESIAN_POINT('Ctrl Pts',(0.223370552162238,1.86769167069714,9.77090191309662));
#65090=CARTESIAN_POINT('Ctrl Pts',(0.223819031526821,1.86812373007451,9.77094000462172));
#65091=CARTESIAN_POINT('Ctrl Pts',(0.224534650771843,1.86881715914905,9.77100104697609));
#65092=CARTESIAN_POINT('Ctrl Pts',(0.224802594727857,1.86907769985801,9.77102396159791));
#65093=CARTESIAN_POINT('Ctrl Pts',(0.225347931006958,1.86960981723044,9.77107071967927));
#65094=CARTESIAN_POINT('Ctrl Pts',(0.225625286996249,1.86988143014629,9.7710945647096));
#65095=CARTESIAN_POINT('Ctrl Pts',(0.226264064954431,1.87050924628127,9.77114963059154));
#65096=CARTESIAN_POINT('Ctrl Pts',(0.22662513699759,1.87086580262165,9.77118086696125));
#65097=CARTESIAN_POINT('Ctrl Pts',(0.227382268672478,1.87161700560702,9.77124659932501));
#65098=CARTESIAN_POINT('Ctrl Pts',(0.227778146090162,1.8720118327808,9.77128110326399));
#65099=CARTESIAN_POINT('Ctrl Pts',(0.228825916945846,1.87306227691534,9.77137278497359));
#65100=CARTESIAN_POINT('Ctrl Pts',(0.22947601639894,1.87371966878665,9.77143004166578));
#65101=CARTESIAN_POINT('Ctrl Pts',(0.243259384165461,1.88777813655942,9.7726519915521));
#65102=CARTESIAN_POINT('Ctrl Pts',(0.255197887340063,1.90229551906481,9.77386903115211));
#65103=CARTESIAN_POINT('Ctrl Pts',(0.281626223112089,1.94084367876889,9.77698851182424));
#65104=CARTESIAN_POINT('Ctrl Pts',(0.294374741620874,1.9658822423925,9.77892701233516));
#65105=CARTESIAN_POINT('Ctrl Pts',(0.304950197733185,1.99569331770424,9.78096102740234));
#65106=CARTESIAN_POINT('Ctrl Pts',(0.3061124275919,1.99915511147793,9.78119310223587));
#65107=CARTESIAN_POINT('Ctrl Pts',(0.307390263170965,2.00318710904358,9.78145805059677));
#65108=CARTESIAN_POINT('Ctrl Pts',(0.307563414212104,2.00373860587871,9.78149417505562));
#65109=CARTESIAN_POINT('Ctrl Pts',(0.307818505013988,2.00455880081039,9.78154772576481));
#65110=CARTESIAN_POINT('Ctrl Pts',(0.307901577571977,2.00482714114871,9.78156521810957));
#65111=CARTESIAN_POINT('Ctrl Pts',(0.308048827702213,2.00530499806484,9.78159631860327));
#65112=CARTESIAN_POINT('Ctrl Pts',(0.308113142402317,2.00551447137122,9.78160993483173));
#65113=CARTESIAN_POINT('Ctrl Pts',(0.308249136583684,2.00595902053908,9.78163879538399));
#65114=CARTESIAN_POINT('Ctrl Pts',(0.30832076062506,2.00619411217248,9.78165403639164));
#65115=CARTESIAN_POINT('Ctrl Pts',(0.30851200583889,2.00682442174181,9.78169484274036));
#65116=CARTESIAN_POINT('Ctrl Pts',(0.308631136977836,2.00721978970296,9.78172037926421));
#65117=CARTESIAN_POINT('Ctrl Pts',(0.309195461631544,2.00910576352573,9.78184191345836));
#65118=CARTESIAN_POINT('Ctrl Pts',(0.309630627898888,2.01059938359611,9.7819373324459));
#65119=CARTESIAN_POINT('Ctrl Pts',(0.313130584089651,2.02294444683579,9.78271959206433));
#65120=CARTESIAN_POINT('Ctrl Pts',(0.315635098361298,2.03394801525893,9.78337628213403));
#65121=CARTESIAN_POINT('Ctrl Pts',(0.322155219336695,2.07163582938955,9.78555813824877));
#65122=CARTESIAN_POINT('Ctrl Pts',(0.323398923842031,2.09868184702976,9.78702067276346));
#65123=CARTESIAN_POINT('Ctrl Pts',(0.320378619023862,2.13663214696955,9.78922402044224));
#65124=CARTESIAN_POINT('Ctrl Pts',(0.318927124970838,2.14764264086941,9.7898800679227));
#65125=CARTESIAN_POINT('Ctrl Pts',(0.316694071962356,2.15972823985174,9.7906272109261));
#65126=CARTESIAN_POINT('Ctrl Pts',(0.316470883100705,2.16089973679362,9.79069991398587));
#65127=CARTESIAN_POINT('Ctrl Pts',(0.316148607372668,2.16254170449757,9.79080221637746));
#65128=CARTESIAN_POINT('Ctrl Pts',(0.31605496024707,2.16301324340491,9.79083164208852));
#65129=CARTESIAN_POINT('Ctrl Pts',(0.315881412704016,2.16387698285339,9.79088562862509));
#65130=CARTESIAN_POINT('Ctrl Pts',(0.315801835935989,2.16426924807016,9.79091017906894));
#65131=CARTESIAN_POINT('Ctrl Pts',(0.315640920104777,2.16505495053901,9.79095941904348));
#65132=CARTESIAN_POINT('Ctrl Pts',(0.315559575688438,2.16544838594824,9.79098410870578));
#65133=CARTESIAN_POINT('Ctrl Pts',(0.315359149252482,2.16640872053921,9.79104445484282));
#65134=CARTESIAN_POINT('Ctrl Pts',(0.315239274383579,2.16697545117448,9.79108013664686));
#65135=CARTESIAN_POINT('Ctrl Pts',(0.314979858368417,2.16818576181493,9.79115648794718));
#65136=CARTESIAN_POINT('Ctrl Pts',(0.314839871428315,2.16882924262811,9.79119717161536));
#65137=CARTESIAN_POINT('Ctrl Pts',(0.314446231074637,2.1706123680326,9.79131016129677));
#65138=CARTESIAN_POINT('Ctrl Pts',(0.314188357284911,2.17175106163078,9.79138260254216));
#65139=CARTESIAN_POINT('Ctrl Pts',(0.313346532433743,2.17537673570273,9.79161418765129));
#65140=CARTESIAN_POINT('Ctrl Pts',(0.312739206997953,2.17785813685601,9.79177407938707));
#65141=CARTESIAN_POINT('Ctrl Pts',(0.310268245600061,2.18745821073826,9.79239822090368));
#65142=CARTESIAN_POINT('Ctrl Pts',(0.308190632893165,2.19451900712157,9.79286924683453));
#65143=CARTESIAN_POINT('Ctrl Pts',(0.301226618323582,2.21550484502384,9.79430584212117));
#65144=CARTESIAN_POINT('Ctrl Pts',(0.29562429095259,2.22917059562471,9.7952918092807));
#65145=CARTESIAN_POINT('Ctrl Pts',(0.278418297757441,2.26410209784424,9.79792124053179));
#65146=CARTESIAN_POINT('Ctrl Pts',(0.265320475326925,2.28453050723108,9.79957735230041));
#65147=CARTESIAN_POINT('Ctrl Pts',(0.249241907795073,2.30430693640791,9.80118637676125));
#65148=CARTESIAN_POINT('Ctrl Pts',(0.248418858778753,2.30530690101256,9.80126773464385));
#65149=CARTESIAN_POINT('Ctrl Pts',(0.247331879236521,2.30661142141867,9.80137384056511));
#65150=CARTESIAN_POINT('Ctrl Pts',(0.247073388823163,2.30692046415704,9.80139897491786));
#65151=CARTESIAN_POINT('Ctrl Pts',(0.246673365335428,2.30739690091608,9.80143771872869));
#65152=CARTESIAN_POINT('Ctrl Pts',(0.246532241046418,2.30756463523639,9.80145135798197));
#65153=CARTESIAN_POINT('Ctrl Pts',(0.246250265723156,2.30789908583057,9.80147855169367));
#65154=CARTESIAN_POINT('Ctrl Pts',(0.246109417455107,2.30806580184707,9.80149210610182));
#65155=CARTESIAN_POINT('Ctrl Pts',(0.245792941783322,2.30843962946974,9.80152249697373));
#65156=CARTESIAN_POINT('Ctrl Pts',(0.245617222328977,2.30864666175303,9.80153932648921));
#65157=CARTESIAN_POINT('Ctrl Pts',(0.245096504855787,2.30925860054939,9.80158906704795));
#65158=CARTESIAN_POINT('Ctrl Pts',(0.244750763626019,2.30966287775965,9.80162192354511));
#65159=CARTESIAN_POINT('Ctrl Pts',(0.242015102189969,2.31284571408807,9.80188058045424));
#65160=CARTESIAN_POINT('Ctrl Pts',(0.239578821676315,2.31558431919263,9.8021030208893));
#65161=CARTESIAN_POINT('Ctrl Pts',(0.230729078116558,2.32519689068969,9.8028858984349));
#65162=CARTESIAN_POINT('Ctrl Pts',(0.224061794823854,2.33183159833205,9.80343025197276));
#65163=CARTESIAN_POINT('Ctrl Pts',(0.205783185856824,2.34849449029425,9.80483885472536));
#65164=CARTESIAN_POINT('Ctrl Pts',(0.193730038034315,2.35800181279671,9.80568719428609));
#65165=CARTESIAN_POINT('Ctrl Pts',(0.162787017217855,2.37901372553495,9.80778553300111));
#65166=CARTESIAN_POINT('Ctrl Pts',(0.143306339627397,2.38950189517053,9.80904601614843));
#65167=CARTESIAN_POINT('Ctrl Pts',(0.121694501942709,2.39841807773674,9.81046581508964));
#65168=CARTESIAN_POINT('Ctrl Pts',(0.120477235076516,2.3989115867137,9.81054583182497));
#65169=CARTESIAN_POINT('Ctrl Pts',(0.118779274795616,2.3995879235457,9.81065752485154));
#65170=CARTESIAN_POINT('Ctrl Pts',(0.118301097827358,2.39977706767429,9.81068898823407));
#65171=CARTESIAN_POINT('Ctrl Pts',(0.117475953634054,2.40010117384551,9.81074329712354));
#65172=CARTESIAN_POINT('Ctrl Pts',(0.117129200448578,2.40023668101362,9.81076612425621));
#65173=CARTESIAN_POINT('Ctrl Pts',(0.116419688903491,2.40051253376765,9.81081284214876));
#65174=CARTESIAN_POINT('Ctrl Pts',(0.116056909790656,2.40065282404065,9.81083673472225));
#65175=CARTESIAN_POINT('Ctrl Pts',(0.115225767745568,2.40097250641598,9.8108914862161));
#65176=CARTESIAN_POINT('Ctrl Pts',(0.114757239124534,2.40115146228244,9.81092235970036));
#65177=CARTESIAN_POINT('Ctrl Pts',(0.113764403587105,2.40152802531138,9.8109878023171));
#65178=CARTESIAN_POINT('Ctrl Pts',(0.113239995765255,2.40172536009499,9.81102238046181));
#65179=CARTESIAN_POINT('Ctrl Pts',(0.11184622637586,2.40224569043652,9.8111143149589));
#65180=CARTESIAN_POINT('Ctrl Pts',(0.110975985405429,2.40256630079437,9.81117175081183));
#65181=CARTESIAN_POINT('Ctrl Pts',(0.108346120928033,2.40352231171719,9.81134542986833));
#65182=CARTESIAN_POINT('Ctrl Pts',(0.106582360375462,2.40414614225624,9.81146205638334));
#65183=CARTESIAN_POINT('Ctrl Pts',(0.10025131831194,2.40632355799008,9.8118812592682));
#65184=CARTESIAN_POINT('Ctrl Pts',(0.0956548951231364,2.40778984065767,
9.81218667542687));
#65185=CARTESIAN_POINT('Ctrl Pts',(0.080153260606281,2.41235417541674,9.81322065839277));
#65186=CARTESIAN_POINT('Ctrl Pts',(0.0691187538204526,2.41497972720595,
9.81396350932832));
#65187=CARTESIAN_POINT('Ctrl Pts',(0.0305340384473812,2.42203530744081,
9.81657670303438));
#65188=CARTESIAN_POINT('Ctrl Pts',(0.00256458125903367,2.42346938800602,
9.81850897116996));
#65189=CARTESIAN_POINT('Ctrl Pts',(-0.0262775840383949,2.42120359299221,
9.82037856688336));
#65190=CARTESIAN_POINT('Ctrl Pts',(-0.0273151276336311,2.42111702451621,
9.82044563888817));
#65191=CARTESIAN_POINT('Ctrl Pts',(-0.0317707886967957,2.42072351050581,
9.82073283700814));
#65192=CARTESIAN_POINT('Ctrl Pts',(-0.0351844622785023,2.4203669913696,
9.82095075277452));
#65193=CARTESIAN_POINT('Ctrl Pts',(-0.0391551363605281,2.41988806278194,
9.8212012476538));
#65194=CARTESIAN_POINT('Ctrl Pts',(-0.0397181435593944,2.41981864626323,
9.82123669569291));
#65195=CARTESIAN_POINT('Ctrl Pts',(-0.0405575357942016,2.41971290186362,
9.82128943812064));
#65196=CARTESIAN_POINT('Ctrl Pts',(-0.0408340579087389,2.41967770182461,
9.82130679574245));
#65197=CARTESIAN_POINT('Ctrl Pts',(-0.0413276357228092,2.41961422068304,
9.82133774673884));
#65198=CARTESIAN_POINT('Ctrl Pts',(-0.0415447080740114,2.4195860772458,
9.82135134789764));
#65199=CARTESIAN_POINT('Ctrl Pts',(-0.0420067188432984,2.41952569885671,
9.82138027294159));
#65200=CARTESIAN_POINT('Ctrl Pts',(-0.0422516482006496,2.41949340350492,
9.82139559331395));
#65201=CARTESIAN_POINT('Ctrl Pts',(-0.0429115727820625,2.41940561649061,
9.82143683486676));
#65202=CARTESIAN_POINT('Ctrl Pts',(-0.0433264991968739,2.41934959745774,
9.82146272614848));
#65203=CARTESIAN_POINT('Ctrl Pts',(-0.0453456446989847,2.41907298585237,
9.82158853414293));
#65204=CARTESIAN_POINT('Ctrl Pts',(-0.0469483314443001,2.41884110811782,
9.82168782168162));
#65205=CARTESIAN_POINT('Ctrl Pts',(-0.0561712425098101,2.4174356801978,
9.82225624082922));
#65206=CARTESIAN_POINT('Ctrl Pts',(-0.0637497986412662,2.41600095528132,
9.82271172595628));
#65207=CARTESIAN_POINT('Ctrl Pts',(-0.0876204508400575,2.41058800460521,
9.82413005955618));
#65208=CARTESIAN_POINT('Ctrl Pts',(-0.103657548743789,2.40560994981487,
9.82505945897578));
#65209=CARTESIAN_POINT('Ctrl Pts',(-0.127451694350232,2.3961341862218,9.82649228668662));
#65210=CARTESIAN_POINT('Ctrl Pts',(-0.135529663329763,2.39252537164029,
9.82698860603385));
#65211=CARTESIAN_POINT('Ctrl Pts',(-0.157593381427512,2.38155817281449,
9.82839101693977));
#65212=CARTESIAN_POINT('Ctrl Pts',(-0.171200041977602,2.37349793258629,
9.82931164810513));
#65213=CARTESIAN_POINT('Ctrl Pts',(-0.184664880412759,2.364122009939,9.83030846627022));
#65214=CARTESIAN_POINT('Ctrl Pts',(-0.185168795053712,2.36376897376731,
9.83034590089087));
#65215=CARTESIAN_POINT('Ctrl Pts',(-0.186323926310053,2.36295476203241,
9.83043201224257));
#65216=CARTESIAN_POINT('Ctrl Pts',(-0.186974445283326,2.36249260786568,
9.83048072605661));
#65217=CARTESIAN_POINT('Ctrl Pts',(-0.188031682064817,2.36173558131828,
9.83056025861495));
#65218=CARTESIAN_POINT('Ctrl Pts',(-0.188439441338247,2.36144216364572,
9.83059102129112));
#65219=CARTESIAN_POINT('Ctrl Pts',(-0.189152804213951,2.36092630215752,
9.83064499532782));
#65220=CARTESIAN_POINT('Ctrl Pts',(-0.189458706395216,2.36070427128975,
9.83066819068289));
#65221=CARTESIAN_POINT('Ctrl Pts',(-0.190105498825275,2.36023307482224,
9.83071734153009));
#65222=CARTESIAN_POINT('Ctrl Pts',(-0.190446291167721,2.35998377659539,
9.83074330214249));
#65223=CARTESIAN_POINT('Ctrl Pts',(-0.191326213007467,2.359337432986,9.8308104964579));
#65224=CARTESIAN_POINT('Ctrl Pts',(-0.191864594848648,2.35893937739228,
9.83085176945416));
#65225=CARTESIAN_POINT('Ctrl Pts',(-0.193033805870256,2.35806926627845,
9.83094175359172));
#65226=CARTESIAN_POINT('Ctrl Pts',(-0.193664150981611,2.35759657026664,
9.83099048967102));
#65227=CARTESIAN_POINT('Ctrl Pts',(-0.195487387279479,2.3562188500057,9.83113211065772));
#65228=CARTESIAN_POINT('Ctrl Pts',(-0.196675700259383,2.3553078269252,9.83122523124823));
#65229=CARTESIAN_POINT('Ctrl Pts',(-0.200677259442015,2.35219550578571,
9.83154161715574));
#65230=CARTESIAN_POINT('Ctrl Pts',(-0.203460160790687,2.349955789927,9.83176640025358));
#65231=CARTESIAN_POINT('Ctrl Pts',(-0.215004127988372,2.34034452341427,
9.83271936626098));
#65232=CARTESIAN_POINT('Ctrl Pts',(-0.22340551048689,2.33255578609056,9.83346416268097));
#65233=CARTESIAN_POINT('Ctrl Pts',(-0.25249579373195,2.30255304101051,9.83623390624631));
#65234=CARTESIAN_POINT('Ctrl Pts',(-0.270433535774029,2.27789720867154,
9.83834498563828));
#65235=CARTESIAN_POINT('Ctrl Pts',(-0.286458392377609,2.24770748579684,
9.84054561332755));
#65236=CARTESIAN_POINT('Ctrl Pts',(-0.28819757730976,2.24428468938073,9.84078981356777));
#65237=CARTESIAN_POINT('Ctrl Pts',(-0.2901316535362,2.24030375416991,9.84106708524926));
#65238=CARTESIAN_POINT('Ctrl Pts',(-0.290386588485125,2.23977535211428,
9.84110375283607));
#65239=CARTESIAN_POINT('Ctrl Pts',(-0.290762191932402,2.23899137829089,
9.84115795153868));
#65240=CARTESIAN_POINT('Ctrl Pts',(-0.290883967651328,2.23873634297265,
9.84117555108893));
#65241=CARTESIAN_POINT('Ctrl Pts',(-0.291099651241241,2.23828310372187,
9.84120677131972));
#65242=CARTESIAN_POINT('Ctrl Pts',(-0.291193692243867,2.23808496415691,
9.84122040031466));
#65243=CARTESIAN_POINT('Ctrl Pts',(-0.291392261997477,2.23766548292999,
9.8412492132196));
#65244=CARTESIAN_POINT('Ctrl Pts',(-0.291496740571661,2.23744411875162,
9.84126439396475));
#65245=CARTESIAN_POINT('Ctrl Pts',(-0.291774925424906,2.236852970124,9.84130487012847));
#65246=CARTESIAN_POINT('Ctrl Pts',(-0.291948181635381,2.23648297250073,
9.84133013753929));
#65247=CARTESIAN_POINT('Ctrl Pts',(-0.292758067308076,2.23474482098909,
9.84144853012219));
#65248=CARTESIAN_POINT('Ctrl Pts',(-0.293385799449378,2.23337250709149,
9.84154111229115));
#65249=CARTESIAN_POINT('Ctrl Pts',(-0.298375254537974,2.22225912972098,
9.8422840919691));
#65250=CARTESIAN_POINT('Ctrl Pts',(-0.302260753147022,2.21231017605921,
9.84290744226122));
#65251=CARTESIAN_POINT('Ctrl Pts',(-0.3166513036255,2.16926687404924,9.84550322046113));
#65252=CARTESIAN_POINT('Ctrl Pts',(-0.322266174513031,2.1347901479798,9.84736301833545));
#65253=CARTESIAN_POINT('Ctrl Pts',(-0.322274989605974,2.10008185028294,
9.84943323242055));
#65254=CARTESIAN_POINT('',(-0.322761847823037,2.10004974457569,10.0997435871451));
#65255=CARTESIAN_POINT('Ctrl Pts',(-0.322274989668007,2.10008160567334,
9.84943324701056));
#65256=CARTESIAN_POINT('Ctrl Pts',(-0.322276075480573,2.09579354310276,
9.84968901325225));
#65257=CARTESIAN_POINT('Ctrl Pts',(-0.322191578554922,2.09150600937965,
9.84994727655726));
#65258=CARTESIAN_POINT('Ctrl Pts',(-0.321992795503579,2.08649660667005,
9.85025238532329));
#65259=CARTESIAN_POINT('Ctrl Pts',(-0.321961580811205,2.08577177257329,
9.85029661511192));
#65260=CARTESIAN_POINT('Ctrl Pts',(-0.321905854955554,2.08457202841941,
9.85036996250775));
#65261=CARTESIAN_POINT('Ctrl Pts',(-0.321882739602497,2.08409705360839,
9.85039903640613));
#65262=CARTESIAN_POINT('Ctrl Pts',(-0.321839399303173,2.08324532807595,
9.85045123682059));
#65263=CARTESIAN_POINT('Ctrl Pts',(-0.321819563820713,2.08286855769527,
9.85047435109949));
#65264=CARTESIAN_POINT('Ctrl Pts',(-0.32177812602574,2.08210693387075,9.85052112207276));
#65265=CARTESIAN_POINT('Ctrl Pts',(-0.321756494791382,2.08172208267726,
9.85054477963659));
#65266=CARTESIAN_POINT('Ctrl Pts',(-0.321708563443494,2.08089577512828,
9.85059562638415));
#65267=CARTESIAN_POINT('Ctrl Pts',(-0.321682045016571,2.08045433266224,
9.85062282237284));
#65268=CARTESIAN_POINT('Ctrl Pts',(-0.321608451333084,2.07926997850794,
9.8506958732354));
#65269=CARTESIAN_POINT('Ctrl Pts',(-0.321559710766366,2.0785271763172,9.85074178029472));
#65270=CARTESIAN_POINT('Ctrl Pts',(-0.32133604818166,2.07529026623484,9.85094223178424));
#65271=CARTESIAN_POINT('Ctrl Pts',(-0.321134682523868,2.07279812658345,
9.8510976042842));
#65272=CARTESIAN_POINT('Ctrl Pts',(-0.320836937763716,2.06958010023945,
9.85129962789211));
#65273=CARTESIAN_POINT('Ctrl Pts',(-0.320767050268643,2.06885179968644,
9.85134544216127));
#65274=CARTESIAN_POINT('Ctrl Pts',(-0.320468730706367,2.06585052154357,
9.85153462404034));
#65275=CARTESIAN_POINT('Ctrl Pts',(-0.320218618402679,2.06357981003516,
9.85167866540678));
#65276=CARTESIAN_POINT('Ctrl Pts',(-0.315533855977145,2.02483747949882,
9.85415209806566));
#65277=CARTESIAN_POINT('Ctrl Pts',(-0.304917763229506,1.98938860429618,
9.85670064504704));
#65278=CARTESIAN_POINT('Ctrl Pts',(-0.285754470621778,1.95085087955732,
9.85954762836783));
#65279=CARTESIAN_POINT('Ctrl Pts',(-0.28277602106689,1.94527827982151,9.85996014309698));
#65280=CARTESIAN_POINT('Ctrl Pts',(-0.278165236209072,1.93723014821545,
9.86055343052394));
#65281=CARTESIAN_POINT('Ctrl Pts',(-0.276659661824865,1.93468407115852,
9.86074074043838));
#65282=CARTESIAN_POINT('Ctrl Pts',(-0.274856854593043,1.93172897211034,
9.86095736729327));
#65283=CARTESIAN_POINT('Ctrl Pts',(-0.274593514779189,1.93129958211901,
9.86098882484963));
#65284=CARTESIAN_POINT('Ctrl Pts',(-0.274189766800146,1.93064469903557,
9.86103677051984));
#65285=CARTESIAN_POINT('Ctrl Pts',(-0.274050086284967,1.9304187616772,9.86105330618524));
#65286=CARTESIAN_POINT('Ctrl Pts',(-0.273806455055637,1.93002576810647,
9.86108205774386));
#65287=CARTESIAN_POINT('Ctrl Pts',(-0.273702630986612,1.92985863486613,
9.86109428196359));
#65288=CARTESIAN_POINT('Ctrl Pts',(-0.273467238821166,1.92948047983886,
9.86112193289518));
#65289=CARTESIAN_POINT('Ctrl Pts',(-0.273335579777427,1.92926951563005,
9.86113735345064));
#65290=CARTESIAN_POINT('Ctrl Pts',(-0.272977728863717,1.92869758721397,
9.86117914516922));
#65291=CARTESIAN_POINT('Ctrl Pts',(-0.272751064283301,1.92833691713364,
9.86120548504222));
#65292=CARTESIAN_POINT('Ctrl Pts',(-0.271725910058636,1.92671284180386,
9.86132402980173));
#65293=CARTESIAN_POINT('Ctrl Pts',(-0.270919336085076,1.92545452474796,
9.86141570736903));
#65294=CARTESIAN_POINT('Ctrl Pts',(-0.254033039025549,1.89950967639892,
9.86330344367826));
#65295=CARTESIAN_POINT('Ctrl Pts',(-0.234649100297479,1.87713319544882,
9.86489286782279));
#65296=CARTESIAN_POINT('Ctrl Pts',(-0.203010029153907,1.84938654639059,
9.8672636296581));
#65297=CARTESIAN_POINT('Ctrl Pts',(-0.193050708013449,1.84163677184903,
9.86798330521246));
#65298=CARTESIAN_POINT('Ctrl Pts',(-0.178484854515807,1.83161583639994,
9.86902257548378));
#65299=CARTESIAN_POINT('Ctrl Pts',(-0.174238991980849,1.82884013555731,
9.869323965932));
#65300=CARTESIAN_POINT('Ctrl Pts',(-0.168279932652965,1.8251422020362,9.86974581259091));
#65301=CARTESIAN_POINT('Ctrl Pts',(-0.16662111599647,1.8241334592818,9.86986311894782));
#65302=CARTESIAN_POINT('Ctrl Pts',(-0.164134544812902,1.82265196020739,
9.87003882571773));
#65303=CARTESIAN_POINT('Ctrl Pts',(-0.163313623156456,1.82216777645696,
9.87009681200351));
#65304=CARTESIAN_POINT('Ctrl Pts',(-0.161997496540433,1.82139936694686,
9.8701897476582));
#65305=CARTESIAN_POINT('Ctrl Pts',(-0.161503658796771,1.82111280091829,
9.87022461236561));
#65306=CARTESIAN_POINT('Ctrl Pts',(-0.160561846611432,1.82056962303987,
9.87029109244038));
#65307=CARTESIAN_POINT('Ctrl Pts',(-0.160114011548544,1.82031277208945,
9.8703226990605));
#65308=CARTESIAN_POINT('Ctrl Pts',(-0.159327204175501,1.81986401629918,
9.87037822138686));
#65309=CARTESIAN_POINT('Ctrl Pts',(-0.158988496644061,1.81967164737203,
9.87040212031164));
#65310=CARTESIAN_POINT('Ctrl Pts',(-0.158326312022943,1.81929714579968,
9.87044883897443));
#65311=CARTESIAN_POINT('Ctrl Pts',(-0.158002867224354,1.81911495699827,
9.87047165664716));
#65312=CARTESIAN_POINT('Ctrl Pts',(-0.157234172910046,1.81868371755589,
9.87052588017673));
#65313=CARTESIAN_POINT('Ctrl Pts',(-0.156788646388517,1.81843516509024,
9.87055730384404));
#65314=CARTESIAN_POINT('Ctrl Pts',(-0.155214953969575,1.81756211932166,
9.87066828720677));
#65315=CARTESIAN_POINT('Ctrl Pts',(-0.154083643474161,1.81694334645859,
9.87074805108102));
#65316=CARTESIAN_POINT('Ctrl Pts',(-0.136406860190665,1.80741236473101,
9.87199413054736));
#65317=CARTESIAN_POINT('Ctrl Pts',(-0.119119718695546,1.79995896382205,
9.8732128517394));
#65318=CARTESIAN_POINT('Ctrl Pts',(-0.0929608241397392,1.79129894940395,
9.8750518601239));
#65319=CARTESIAN_POINT('Ctrl Pts',(-0.0845283854181895,1.78888427311213,
9.87564335847589));
#65320=CARTESIAN_POINT('Ctrl Pts',(-0.0735270853278912,1.78621430509336,
9.87640915894608));
#65321=CARTESIAN_POINT('Ctrl Pts',(-0.0710388166221223,1.78564163583795,
9.87658197292038));
#65322=CARTESIAN_POINT('Ctrl Pts',(-0.0605914599342707,1.78336757895998,
9.87730545787967));
#65323=CARTESIAN_POINT('Ctrl Pts',(-0.0525759843857189,1.7819383900288,
9.87785553570679));
#65324=CARTESIAN_POINT('Ctrl Pts',(-0.0358680333711405,1.77960823825756,
9.87898304808197));
#65325=CARTESIAN_POINT('Ctrl Pts',(-0.0271750550664454,1.77875408388538,
9.87955912624351));
#65326=CARTESIAN_POINT('Ctrl Pts',(-0.0149468507266521,1.77805259405645,
9.88034564956765));
#65327=CARTESIAN_POINT('Ctrl Pts',(-0.0114330013516283,1.77790866273691,
9.88056890195889));
#65328=CARTESIAN_POINT('Ctrl Pts',(-0.00739085921732094,1.77780932949561,
9.88082201302364));
#65329=CARTESIAN_POINT('Ctrl Pts',(-0.00686435670550724,1.77779768222994,
9.8808549093006));
#65330=CARTESIAN_POINT('Ctrl Pts',(-0.00606743225273874,1.77778200697258,
9.88090458992848));
#65331=CARTESIAN_POINT('Ctrl Pts',(-0.00579703313422386,1.77777702879389,
9.88092142724901));
#65332=CARTESIAN_POINT('Ctrl Pts',(-0.00532938696109524,1.77776900804757,
9.88095051276104));
#65333=CARTESIAN_POINT('Ctrl Pts',(-0.00513214369712841,1.77776580621873,
9.8809627699194));
#65334=CARTESIAN_POINT('Ctrl Pts',(-0.00472059483463152,1.77775950356115,
9.88098832256555));
#65335=CARTESIAN_POINT('Ctrl Pts',(-0.00450628973259388,1.77775643541844,
9.88100161615761));
#65336=CARTESIAN_POINT('Ctrl Pts',(-0.00391332761659985,1.7777485377911,
9.88103836438608));
#65337=CARTESIAN_POINT('Ctrl Pts',(-0.0035346633455427,1.77774416190341,
9.88106179348087));
#65338=CARTESIAN_POINT('Ctrl Pts',(-0.00204854543050816,1.77772960787937,
9.88115359704473));
#65339=CARTESIAN_POINT('Ctrl Pts',(-0.000941033447506969,1.77772447080819,
9.88122169219538));
#65340=CARTESIAN_POINT('Ctrl Pts',(0.0194687415531727,1.77773501542436,
9.88247103936936));
#65341=CARTESIAN_POINT('Ctrl Pts',(0.0387343882509863,1.77947911042484,
9.88356014564101));
#65342=CARTESIAN_POINT('Ctrl Pts',(0.0739802413587024,1.78589666372575,
9.88556630697484));
#65343=CARTESIAN_POINT('Ctrl Pts',(0.0899781765223071,1.7901002019261,9.88648275333677));
#65344=CARTESIAN_POINT('Ctrl Pts',(0.111817456346848,1.79767306215114,9.88780643457743));
#65345=CARTESIAN_POINT('Ctrl Pts',(0.117983986742064,1.80002584716446,9.88818847242845));
#65346=CARTESIAN_POINT('Ctrl Pts',(0.128819480882107,1.80454584366554,9.88887828701004));
#65347=CARTESIAN_POINT('Ctrl Pts',(0.133516984408784,1.80663874198001,9.8891837318254));
#65348=CARTESIAN_POINT('Ctrl Pts',(0.13993405414394,1.80968382338513,9.8896109025952));
#65349=CARTESIAN_POINT('Ctrl Pts',(0.141698139353985,1.8105407473271,9.88972938775935));
#65350=CARTESIAN_POINT('Ctrl Pts',(0.144314100417334,1.81184112359528,9.88990671319791));
#65351=CARTESIAN_POINT('Ctrl Pts',(0.145172014790615,1.81227237928788,9.88996513019462));
#65352=CARTESIAN_POINT('Ctrl Pts',(0.14653960323938,1.81296751108813,9.89005867740894));
#65353=CARTESIAN_POINT('Ctrl Pts',(0.147050526379472,1.81322892807446,9.89009372147586));
#65354=CARTESIAN_POINT('Ctrl Pts',(0.148021778848039,1.81372915352097,9.89016052244851));
#65355=CARTESIAN_POINT('Ctrl Pts',(0.148482235835225,1.81396771127447,9.89019227046276));
#65356=CARTESIAN_POINT('Ctrl Pts',(0.149287847022244,1.81438755917555,9.89024795520635));
#65357=CARTESIAN_POINT('Ctrl Pts',(0.149633252687581,1.81456836666163,9.89027187484308));
#65358=CARTESIAN_POINT('Ctrl Pts',(0.150306412628952,1.81492229946361,9.89031857961225));
#65359=CARTESIAN_POINT('Ctrl Pts',(0.150634198124144,1.81509536442133,9.89034136257993));
#65360=CARTESIAN_POINT('Ctrl Pts',(0.151410524137539,1.81550696512249,9.89039541875431));
#65361=CARTESIAN_POINT('Ctrl Pts',(0.151858799630959,1.81574599618765,9.89042670951346));
#65362=CARTESIAN_POINT('Ctrl Pts',(0.15343178422973,1.81658953157698,9.89053678000544));
#65363=CARTESIAN_POINT('Ctrl Pts',(0.154553452938725,1.81719965323017,9.89061575952742));
#65364=CARTESIAN_POINT('Ctrl Pts',(0.170842968429254,1.82618604616891,9.89176998977606));
#65365=CARTESIAN_POINT('Ctrl Pts',(0.185312173956877,1.83576408018195,9.89288948426452));
#65366=CARTESIAN_POINT('Ctrl Pts',(0.21179508236492,1.8565435983744,9.89512724377984));
#65367=CARTESIAN_POINT('Ctrl Pts',(0.223864112527872,1.86759306457073,9.89623844810752));
#65368=CARTESIAN_POINT('Ctrl Pts',(0.237721011914614,1.8823644708832,9.89760519421292));
#65369=CARTESIAN_POINT('Ctrl Pts',(0.240347348290867,1.88526840880596,9.89786869226733));
#65370=CARTESIAN_POINT('Ctrl Pts',(0.250516385788705,1.89693267694138,9.89890494401018));
#65371=CARTESIAN_POINT('Ctrl Pts',(0.257639237428898,1.90604927942632,9.89966704432621));
#65372=CARTESIAN_POINT('Ctrl Pts',(0.265159879357793,1.91682276380576,9.90049838079363));
#65373=CARTESIAN_POINT('Ctrl Pts',(0.266052881237803,1.91812222206426,9.90059755897435));
#65374=CARTESIAN_POINT('Ctrl Pts',(0.267168773655424,1.91977182764946,9.90072203198418));
#65375=CARTESIAN_POINT('Ctrl Pts',(0.267400553280895,1.92011589332288,9.90074791593235));
#65376=CARTESIAN_POINT('Ctrl Pts',(0.267768822149501,1.92066485531472,9.9007890888712));
#65377=CARTESIAN_POINT('Ctrl Pts',(0.267905741099022,1.92086946066687,9.90080440691191));
#65378=CARTESIAN_POINT('Ctrl Pts',(0.268164037732097,1.9212564057875,9.90083332352173));
#65379=CARTESIAN_POINT('Ctrl Pts',(0.268285462971969,1.92143871090572,9.90084692525057));
#65380=CARTESIAN_POINT('Ctrl Pts',(0.268561777972551,1.9218544821409,9.90087789584407));
#65381=CARTESIAN_POINT('Ctrl Pts',(0.268716548942019,1.92208802612757,9.90089525660364));
#65382=CARTESIAN_POINT('Ctrl Pts',(0.269177175995301,1.92278506856004,9.90094696627878));
#65383=CARTESIAN_POINT('Ctrl Pts',(0.269482140843537,1.92324915904211,9.90098125533155));
#65384=CARTESIAN_POINT('Ctrl Pts',(0.271609373003768,1.92650464947872,9.90122082926981));
#65385=CARTESIAN_POINT('Ctrl Pts',(0.273389517539276,1.92932351666184,9.90142336071257));
#65386=CARTESIAN_POINT('Ctrl Pts',(0.282846026764444,1.94482564885782,9.90251358000512));
#65387=CARTESIAN_POINT('Ctrl Pts',(0.289684835359071,1.95800086894476,9.90335578426171));
#65388=CARTESIAN_POINT('Ctrl Pts',(0.307616996932311,1.99928342431079,9.90588331071758));
#65389=CARTESIAN_POINT('Ctrl Pts',(0.315692156896018,2.02851332731368,9.90754137125232));
#65390=CARTESIAN_POINT('Ctrl Pts',(0.319839763281418,2.0604065994335,9.9094752219177));
#65391=CARTESIAN_POINT('Ctrl Pts',(0.320077433658286,2.06237623438598,9.90959506280617));
#65392=CARTESIAN_POINT('Ctrl Pts',(0.320404029791101,2.06531036012148,9.90977424880363));
#65393=CARTESIAN_POINT('Ctrl Pts',(0.32050682061774,2.06627328467042,9.90983315998312));
#65394=CARTESIAN_POINT('Ctrl Pts',(0.32066395980513,2.06781096781645,9.90992740869623));
#65395=CARTESIAN_POINT('Ctrl Pts',(0.320721106995287,2.06838543956142,9.9099626583548));
#65396=CARTESIAN_POINT('Ctrl Pts',(0.320826887074585,2.06947860483655,9.91002981009851));
#65397=CARTESIAN_POINT('Ctrl Pts',(0.320875806472424,2.0699972693188,9.91006170308344));
#65398=CARTESIAN_POINT('Ctrl Pts',(0.320959176359397,2.07090472409303,9.91011755995921));
#65399=CARTESIAN_POINT('Ctrl Pts',(0.320994178664902,2.07129346362793,9.91014150644712));
#65400=CARTESIAN_POINT('Ctrl Pts',(0.321060986415239,2.07205084022368,9.91018819705763));
#65401=CARTESIAN_POINT('Ctrl Pts',(0.321092863393407,2.07241947052397,9.91021093889342));
#65402=CARTESIAN_POINT('Ctrl Pts',(0.321166785292379,2.07329181499574,9.9102647958708));
#65403=CARTESIAN_POINT('Ctrl Pts',(0.321208280027281,2.07379557368435,9.91029592825864));
#65404=CARTESIAN_POINT('Ctrl Pts',(0.321349224621394,2.07555733400026,9.91040491591632));
#65405=CARTESIAN_POINT('Ctrl Pts',(0.321442469587056,2.07681580799171,9.91048296583224));
#65406=CARTESIAN_POINT('Ctrl Pts',(0.32262236244452,2.09411866833812,9.91155886056253));
#65407=CARTESIAN_POINT('Ctrl Pts',(0.322513876835275,2.11021932538932,9.91259461139189));
#65408=CARTESIAN_POINT('Ctrl Pts',(0.319449043936508,2.14773230764201,9.91508747392847));
#65409=CARTESIAN_POINT('Ctrl Pts',(0.31554110726248,2.1689910424194,9.91656371437978));
#65410=CARTESIAN_POINT('Ctrl Pts',(0.306331142177803,2.20077393989518,9.91877942206794));
#65411=CARTESIAN_POINT('Ctrl Pts',(0.302528988629397,2.21167106943813,9.91953961106161));
#65412=CARTESIAN_POINT('Ctrl Pts',(0.297552562134759,2.2237987392997,9.92036904579229));
#65413=CARTESIAN_POINT('Ctrl Pts',(0.296944118203446,2.2252511316899,9.9204680952189));
#65414=CARTESIAN_POINT('Ctrl Pts',(0.2961620178131,2.22708031624389,9.92059242944381));
#65415=CARTESIAN_POINT('Ctrl Pts',(0.295998259941087,2.2274612791722,9.92061830178424));
#65416=CARTESIAN_POINT('Ctrl Pts',(0.295736122410401,2.22806788089092,9.92065946055417));
#65417=CARTESIAN_POINT('Ctrl Pts',(0.295638219438636,2.22829372323835,9.92067477599926));
#65418=CARTESIAN_POINT('Ctrl Pts',(0.295452702632546,2.22872033295208,9.92070369048485));
#65419=CARTESIAN_POINT('Ctrl Pts',(0.295365143574476,2.22892112150346,9.9207172926788));
#65420=CARTESIAN_POINT('Ctrl Pts',(0.295165098370304,2.2293785873482,9.92074826804565));
#65421=CARTESIAN_POINT('Ctrl Pts',(0.295052482293247,2.22963520684671,9.92076563310412));
#65422=CARTESIAN_POINT('Ctrl Pts',(0.2947078976741,2.23041764053126,9.92081854708047));
#65423=CARTESIAN_POINT('Ctrl Pts',(0.294474855631371,2.23094298502076,9.9208540304404));
#65424=CARTESIAN_POINT('Ctrl Pts',(0.292779812831057,2.23473669293124,9.92110996780169));
#65425=CARTESIAN_POINT('Ctrl Pts',(0.291264768321077,2.23798127608504,9.9213272407064));
#65426=CARTESIAN_POINT('Ctrl Pts',(0.278666561604475,2.2638286286931,9.92305030691874));
#65427=CARTESIAN_POINT('Ctrl Pts',(0.265022357965995,2.28509021679271,9.92442435825353));
#65428=CARTESIAN_POINT('Ctrl Pts',(0.235344627055456,2.32122316266972,9.92704919348635));
#65429=CARTESIAN_POINT('Ctrl Pts',(0.220011460893924,2.33647733566107,9.92828313599592));
#65430=CARTESIAN_POINT('Ctrl Pts',(0.202532675550062,2.35068425519987,9.92965049157533));
#65431=CARTESIAN_POINT('Ctrl Pts',(0.201791875006027,2.35128095753941,9.9297083666877));
#65432=CARTESIAN_POINT('Ctrl Pts',(0.200602810351679,2.35223007994785,9.92980114446508));
#65433=CARTESIAN_POINT('Ctrl Pts',(0.200156230012903,2.35258460826414,9.92983596285092));
#65434=CARTESIAN_POINT('Ctrl Pts',(0.199303744449869,2.35325769348716,9.92990237933494));
#65435=CARTESIAN_POINT('Ctrl Pts',(0.198898010065265,2.35357646469923,9.92993396877016));
#65436=CARTESIAN_POINT('Ctrl Pts',(0.198184731015751,2.35413409778234,9.92998946684694));
#65437=CARTESIAN_POINT('Ctrl Pts',(0.197877514914445,2.35437337980331,9.93001335873649));
#65438=CARTESIAN_POINT('Ctrl Pts',(0.197276422359329,2.35483980608267,9.93006008272068));
#65439=CARTESIAN_POINT('Ctrl Pts',(0.196982585302058,2.35506700035299,9.93008291278487));
#65440=CARTESIAN_POINT('Ctrl Pts',(0.19628361481496,2.35560551487419,9.93013719591712));
#65441=CARTESIAN_POINT('Ctrl Pts',(0.195878133424185,2.35591637993763,9.93016866688768));
#65442=CARTESIAN_POINT('Ctrl Pts',(0.194443131470358,2.35701112550417,9.93027997609215));
#65443=CARTESIAN_POINT('Ctrl Pts',(0.193409641273601,2.35778976045026,9.93036002008375));
#65444=CARTESIAN_POINT('Ctrl Pts',(0.176726594643034,2.37020202900604,9.93165028138012));
#65445=CARTESIAN_POINT('Ctrl Pts',(0.16006056982947,2.38039577286334,9.93291711967311));
#65446=CARTESIAN_POINT('Ctrl Pts',(0.127597832294581,2.39641019621713,9.93533714572109));
#65447=CARTESIAN_POINT('Ctrl Pts',(0.112065407743267,2.40262439505264,9.93647616678091));
#65448=CARTESIAN_POINT('Ctrl Pts',(0.0860523836713744,2.41075306387351,
9.93830713282158));
#65449=CARTESIAN_POINT('Ctrl Pts',(0.0758331156550389,2.41340366642323,
9.93900768035754));
#65450=CARTESIAN_POINT('Ctrl Pts',(0.0618442749261837,2.41630746455329,
9.93992647390684));
#65451=CARTESIAN_POINT('Ctrl Pts',(0.0581740305197722,2.41700301519994,
9.94016383877853));
#65452=CARTESIAN_POINT('Ctrl Pts',(0.0539656603337894,2.4177249890654,9.94043115520065));
#65453=CARTESIAN_POINT('Ctrl Pts',(0.0534387602673929,2.41781403380391,
9.94046453738085));
#65454=CARTESIAN_POINT('Ctrl Pts',(0.0526432792788163,2.41794643382568,
9.94051480256152));
#65455=CARTESIAN_POINT('Ctrl Pts',(0.0523748642389889,2.417990759666,9.94053174042147));
#65456=CARTESIAN_POINT('Ctrl Pts',(0.0519115275516,2.41806667213618,9.94056093864365));
#65457=CARTESIAN_POINT('Ctrl Pts',(0.0517166332464374,2.41809841946003,
9.94057320818576));
#65458=CARTESIAN_POINT('Ctrl Pts',(0.0513108815777127,2.41816413165286,
9.94059872682051));
#65459=CARTESIAN_POINT('Ctrl Pts',(0.0511000202553528,2.418198065942,9.94061197412402));
#65460=CARTESIAN_POINT('Ctrl Pts',(0.0505188924337464,2.41829099533184,
9.94064844447225));
#65461=CARTESIAN_POINT('Ctrl Pts',(0.050148554969326,2.41834955416954,9.94067164262755));
#65462=CARTESIAN_POINT('Ctrl Pts',(0.0487080625215991,2.41857475302515,
9.94076170999835));
#65463=CARTESIAN_POINT('Ctrl Pts',(0.0476371567331209,2.41873664677367,
9.94082831289414));
#65464=CARTESIAN_POINT('Ctrl Pts',(0.0281230779108912,2.42158613299846,
9.94203580996059));
#65465=CARTESIAN_POINT('Ctrl Pts',(0.00947872784101369,2.42267464108025,
9.9430906431631));
#65466=CARTESIAN_POINT('Ctrl Pts',(-0.0258971944186755,2.421669007309,9.94507415722131));
#65467=CARTESIAN_POINT('Ctrl Pts',(-0.0425735994511782,2.41988917303906,
9.94600210184314));
#65468=CARTESIAN_POINT('Ctrl Pts',(-0.0732644266709059,2.41417030179155,
9.94778708822536));
#65469=CARTESIAN_POINT('Ctrl Pts',(-0.0872963369329439,2.41056387395722,
9.94863438715372));
#65470=CARTESIAN_POINT('Ctrl Pts',(-0.102181929484982,2.40564927937652,
9.94958726974118));
#65471=CARTESIAN_POINT('Ctrl Pts',(-0.103324448849124,2.40526494542432,
9.94966075252034));
#65472=CARTESIAN_POINT('Ctrl Pts',(-0.104972315384738,2.40470030599128,
9.94976724728498));
#65473=CARTESIAN_POINT('Ctrl Pts',(-0.105479420156125,2.40452513096039,
9.94980008937827));
#65474=CARTESIAN_POINT('Ctrl Pts',(-0.10636216686101,2.40421772413405,9.94985738251494));
#65475=CARTESIAN_POINT('Ctrl Pts',(-0.106738006570783,2.40408606046261,
9.94988181466686));
#65476=CARTESIAN_POINT('Ctrl Pts',(-0.107462669458365,2.40383068850838,
9.94992899826131));
#65477=CARTESIAN_POINT('Ctrl Pts',(-0.107811525671363,2.4037070752176,9.94995174651599));
#65478=CARTESIAN_POINT('Ctrl Pts',(-0.108636693031225,2.40341308550093,
9.95000563464235));
#65479=CARTESIAN_POINT('Ctrl Pts',(-0.10911281643243,2.40324218837669,9.95003679180811));
#65480=CARTESIAN_POINT('Ctrl Pts',(-0.110777452670948,2.40264026492484,
9.95014594843901));
#65481=CARTESIAN_POINT('Ctrl Pts',(-0.11196381814408,2.4022033708078,9.95022414334812));
#65482=CARTESIAN_POINT('Ctrl Pts',(-0.128368697873202,2.39605220677752,
9.95131104490252));
#65483=CARTESIAN_POINT('Ctrl Pts',(-0.143133699455842,2.38920239935996,
9.952358514376));
#65484=CARTESIAN_POINT('Ctrl Pts',(-0.161735498329928,2.37879819084325,
9.95377093461385));
#65485=CARTESIAN_POINT('Ctrl Pts',(-0.166094720906318,2.37622335781735,
9.95410890814488));
#65486=CARTESIAN_POINT('Ctrl Pts',(-0.1773944440358,2.36918480387902,9.95500239195419));
#65487=CARTESIAN_POINT('Ctrl Pts',(-0.184227280524771,2.36455538343687,
9.95556058283267));
#65488=CARTESIAN_POINT('Ctrl Pts',(-0.196980720924983,2.35518071683819,
9.95663172144273));
#65489=CARTESIAN_POINT('Ctrl Pts',(-0.2029265615126,2.35047837784963,9.9571443138424));
#65490=CARTESIAN_POINT('Ctrl Pts',(-0.217822841365875,2.33781859729511,
9.95845490429192));
#65491=CARTESIAN_POINT('Ctrl Pts',(-0.226506590135773,2.32956329579587,
9.95924533382984));
#65492=CARTESIAN_POINT('Ctrl Pts',(-0.23581215421961,2.31967335462556,9.96010477741338));
#65493=CARTESIAN_POINT('Ctrl Pts',(-0.236903944096473,2.31849548355999,
9.96020581620743));
#65494=CARTESIAN_POINT('Ctrl Pts',(-0.238268428881213,2.31700116527138,
9.96033229292212));
#65495=CARTESIAN_POINT('Ctrl Pts',(-0.238549350450033,2.31669231028167,
9.96035834297832));
#65496=CARTESIAN_POINT('Ctrl Pts',(-0.238995368527162,2.31620002393444,
9.96039971865969));
#65497=CARTESIAN_POINT('Ctrl Pts',(-0.239160854681028,2.31601694867743,
9.96041507382979));
#65498=CARTESIAN_POINT('Ctrl Pts',(-0.239472756486994,2.3156710978745,9.96044402103891));
#65499=CARTESIAN_POINT('Ctrl Pts',(-0.239619215357413,2.31550836454692,
9.96045761632779));
#65500=CARTESIAN_POINT('Ctrl Pts',(-0.239952063011153,2.31513777219875,
9.96048851964247));
#65501=CARTESIAN_POINT('Ctrl Pts',(-0.240138347255088,2.31492982052045,
9.96050581969523));
#65502=CARTESIAN_POINT('Ctrl Pts',(-0.240703754211891,2.31429699620476,
9.96055834303852));
#65503=CARTESIAN_POINT('Ctrl Pts',(-0.241082023882774,2.31387135770453,
9.96059350218161));
#65504=CARTESIAN_POINT('Ctrl Pts',(-0.243760405447751,2.31084144065498,
9.96084261094786));
#65505=CARTESIAN_POINT('Ctrl Pts',(-0.246019506756295,2.30820099191381,
9.96105356744091));
#65506=CARTESIAN_POINT('Ctrl Pts',(-0.267991281892727,2.28166313904493,
9.96311981497746));
#65507=CARTESIAN_POINT('Ctrl Pts',(-0.284206343142693,2.25507481408311,
9.96477620875413));
#65508=CARTESIAN_POINT('Ctrl Pts',(-0.302128827212125,2.21310964691832,
9.96737142239807));
#65509=CARTESIAN_POINT('Ctrl Pts',(-0.306955121896611,2.19926777803044,
9.9682223365515));
#65510=CARTESIAN_POINT('Ctrl Pts',(-0.311237435956427,2.18363545863939,
9.96920044902112));
#65511=CARTESIAN_POINT('Ctrl Pts',(-0.311640441698801,2.18212104752749,
9.96929536633618));
#65512=CARTESIAN_POINT('Ctrl Pts',(-0.312328031226317,2.17945925916442,
9.96946250560583));
#65513=CARTESIAN_POINT('Ctrl Pts',(-0.312617379242658,2.17831313487435,
9.96953457310703));
#65514=CARTESIAN_POINT('Ctrl Pts',(-0.313027849879069,2.1766487057733,9.96963938468727));
#65515=CARTESIAN_POINT('Ctrl Pts',(-0.31315400664538,2.17613164265411,9.96967196633314));
#65516=CARTESIAN_POINT('Ctrl Pts',(-0.313372151010175,2.17522784472116,
9.96972895552328));
#65517=CARTESIAN_POINT('Ctrl Pts',(-0.313464705242304,2.17484124675072,
9.96975334476004));
#65518=CARTESIAN_POINT('Ctrl Pts',(-0.313642307090249,2.17409329684037,
9.96980055453524));
#65519=CARTESIAN_POINT('Ctrl Pts',(-0.31372744614752,2.17373196705319,9.96982337208892));
#65520=CARTESIAN_POINT('Ctrl Pts',(-0.313928106322365,2.17287372607629,
9.96987759504555));
#65521=CARTESIAN_POINT('Ctrl Pts',(-0.314043071939718,2.17237668722231,
9.96990901825806));
#65522=CARTESIAN_POINT('Ctrl Pts',(-0.314383795249423,2.17088751794692,
9.97000322793127));
#65523=CARTESIAN_POINT('Ctrl Pts',(-0.314606033473852,2.1698945962138,9.97006612723546));
#65524=CARTESIAN_POINT('Ctrl Pts',(-0.316740867253675,2.16014002929923,
9.970684906583));
#65525=CARTESIAN_POINT('Ctrl Pts',(-0.318291493428664,2.15130399091243,
9.97125231117246));
#65526=CARTESIAN_POINT('Ctrl Pts',(-0.320070783976515,2.13790244324655,
9.97212438986133));
#65527=CARTESIAN_POINT('Ctrl Pts',(-0.320574246079929,2.13337741258019,
9.97242076883965));
#65528=CARTESIAN_POINT('Ctrl Pts',(-0.321852373819689,2.11915385970834,
9.97335807673244));
#65529=CARTESIAN_POINT('Ctrl Pts',(-0.322283826669288,2.10943047574389,
9.97400729087377));
#65530=CARTESIAN_POINT('Ctrl Pts',(-0.322250579164992,2.0733493113159,9.97643634402248));
#65531=CARTESIAN_POINT('Ctrl Pts',(-0.318993923940641,2.04709668394773,
9.97825145316637));
#65532=CARTESIAN_POINT('Ctrl Pts',(-0.31223920016274,2.02018912324031,9.98000427312217));
#65533=CARTESIAN_POINT('Ctrl Pts',(-0.311893288057679,2.01884785156172,
9.98009133286119));
#65534=CARTESIAN_POINT('Ctrl Pts',(-0.311432852017357,2.01710895455509,
9.9802037562032));
#65535=CARTESIAN_POINT('Ctrl Pts',(-0.311326201769074,2.01670928726914,
9.98022956487852));
#65536=CARTESIAN_POINT('Ctrl Pts',(-0.311161294179648,2.01609604517341,
9.98026911696058));
#65537=CARTESIAN_POINT('Ctrl Pts',(-0.311103586287571,2.01588232509867,
9.98028289218651));
#65538=CARTESIAN_POINT('Ctrl Pts',(-0.310988606913736,2.01545823796048,
9.98031020839601));
#65539=CARTESIAN_POINT('Ctrl Pts',(-0.310931342532343,2.01524787087951,
9.98032374961862));
#65540=CARTESIAN_POINT('Ctrl Pts',(-0.310803261417333,2.01477922766307,
9.98035389621517));
#65541=CARTESIAN_POINT('Ctrl Pts',(-0.310732336388528,2.01452098228729,
9.98037049514583));
#65542=CARTESIAN_POINT('Ctrl Pts',(-0.310524339961979,2.01376732559113,
9.98041889894385));
#65543=CARTESIAN_POINT('Ctrl Pts',(-0.310386404303334,2.01327215051197,
9.9804506536021));
#65544=CARTESIAN_POINT('Ctrl Pts',(-0.309382772373545,2.00970227601466,
9.98067924995945));
#65545=CARTESIAN_POINT('Ctrl Pts',(-0.30847255199729,2.00664012995879,9.98087355011733));
#65546=CARTESIAN_POINT('Ctrl Pts',(-0.305795756082405,1.99810184441902,
9.98141161832246));
#65547=CARTESIAN_POINT('Ctrl Pts',(-0.303927780068221,1.99265852929653,
9.98175034146277));
#65548=CARTESIAN_POINT('Ctrl Pts',(-0.298970432652464,1.97938195352247,
9.98257245907948));
#65549=CARTESIAN_POINT('Ctrl Pts',(-0.295717932675965,1.97161405236998,
9.98304995743626));
#65550=CARTESIAN_POINT('Ctrl Pts',(-0.281756877286434,1.94162587728681,
9.98491068472604));
#65551=CARTESIAN_POINT('Ctrl Pts',(-0.268818199870231,1.92053962821151,
9.9862646134698));
#65552=CARTESIAN_POINT('Ctrl Pts',(-0.252089269540585,1.89920611414663,
9.98784895971462));
#65553=CARTESIAN_POINT('Ctrl Pts',(-0.250554736038744,1.89729452837739,
9.98799294140806));
#65554=CARTESIAN_POINT('Ctrl Pts',(-0.244885185310744,1.89039465229281,
9.98852038512737));
#65555=CARTESIAN_POINT('Ctrl Pts',(-0.240622011560437,1.88551411621042,
9.9889084893278));
#65556=CARTESIAN_POINT('Ctrl Pts',(-0.235512787001667,1.8800091640062,9.98936560320263));
#65557=CARTESIAN_POINT('Ctrl Pts',(-0.234807086604242,1.87925609226046,
9.9894285702673));
#65558=CARTESIAN_POINT('Ctrl Pts',(-0.233751762674211,1.87814071452223,
9.98952248603017));
#65559=CARTESIAN_POINT('Ctrl Pts',(-0.233404882920069,1.8777758120039,9.98955331637382));
#65560=CARTESIAN_POINT('Ctrl Pts',(-0.232785466982795,1.87712726340465,
9.98960830039701));
#65561=CARTESIAN_POINT('Ctrl Pts',(-0.232513263285326,1.87684330001067,
9.98963243963232));
#65562=CARTESIAN_POINT('Ctrl Pts',(-0.231939069307073,1.87624649092155,
9.9896833103864));
#65563=CARTESIAN_POINT('Ctrl Pts',(-0.231636964606391,1.87593375684647,
9.98971004686416));
#65564=CARTESIAN_POINT('Ctrl Pts',(-0.23083902742191,1.87511108312504,9.98978059054528));
#65565=CARTESIAN_POINT('Ctrl Pts',(-0.230342140133861,1.87460217396817,
9.98982444385522));
#65566=CARTESIAN_POINT('Ctrl Pts',(-0.228101341536908,1.87232230866073,
9.99002187534543));
#65567=CARTESIAN_POINT('Ctrl Pts',(-0.22633870052059,1.87056995568458,9.99017627794503));
#65568=CARTESIAN_POINT('Ctrl Pts',(-0.213209513221816,1.85781595430748,
9.99132007996892));
#65569=CARTESIAN_POINT('Ctrl Pts',(-0.201068667300165,1.84764575309584,
9.9923452550347));
#65570=CARTESIAN_POINT('Ctrl Pts',(-0.162384402036427,1.81980987897678,
9.99551361721086));
#65571=CARTESIAN_POINT('Ctrl Pts',(-0.133924730622777,1.8051452683665,9.99773546654406));
#65572=CARTESIAN_POINT('Ctrl Pts',(-0.102314385090887,1.7943935011591,9.99984809662761));
#65573=CARTESIAN_POINT('Ctrl Pts',(-0.100847200872162,1.79390621072366,
9.99994535328652));
#65574=CARTESIAN_POINT('Ctrl Pts',(-0.0989708781197706,1.79329799029727,
10.0000686610128));
#65575=CARTESIAN_POINT('Ctrl Pts',(-0.0985649603050398,1.7931672995319,
10.000095273368));
#65576=CARTESIAN_POINT('Ctrl Pts',(-0.0979194594167723,1.79296088486271,
10.000137490571));
#65577=CARTESIAN_POINT('Ctrl Pts',(-0.0976800469248476,1.79288463537205,
10.0001531263191));
#65578=CARTESIAN_POINT('Ctrl Pts',(-0.097232447600714,1.79274265766306,
10.0001823163973));
#65579=CARTESIAN_POINT('Ctrl Pts',(-0.0970242847209387,1.79267686149397,
10.0001958746464));
#65580=CARTESIAN_POINT('Ctrl Pts',(-0.0965562015934771,1.79252943266054,
10.0002263240949));
#65581=CARTESIAN_POINT('Ctrl Pts',(-0.0962962452092579,1.79244791822177,
10.0002432082268));
#65582=CARTESIAN_POINT('Ctrl Pts',(-0.0955243096152806,1.79220693729672,
10.0002932679086));
#65583=CARTESIAN_POINT('Ctrl Pts',(-0.0950120322138111,1.79204841789635,
10.0003263878507));
#65584=CARTESIAN_POINT('Ctrl Pts',(-0.0908753458001397,1.79077966420559,
10.000593037779));
#65585=CARTESIAN_POINT('Ctrl Pts',(-0.08723181153509,1.78973211789303,10.0008229701226));
#65586=CARTESIAN_POINT('Ctrl Pts',(-0.0739276427774553,1.78615996693607,
10.0016475816422));
#65587=CARTESIAN_POINT('Ctrl Pts',(-0.0641688221698824,1.78402015758211,
10.0022240770525));
#65588=CARTESIAN_POINT('Ctrl Pts',(-0.0231551310390569,1.7770061473479,
10.0045877304807));
#65589=CARTESIAN_POINT('Ctrl Pts',(0.00862809475382032,1.77629211274213,
10.006297304328));
#65590=CARTESIAN_POINT('Ctrl Pts',(0.0455835936598826,1.7809155383611,10.0085061184341));
#65591=CARTESIAN_POINT('Ctrl Pts',(0.0511404263871118,1.78175888303605,
10.0088435882033));
#65592=CARTESIAN_POINT('Ctrl Pts',(0.0576333180037274,1.78291873335546,
10.0092451504272));
#65593=CARTESIAN_POINT('Ctrl Pts',(0.0585937186121705,1.78309480107246,
10.0093047342403));
#65594=CARTESIAN_POINT('Ctrl Pts',(0.0600436272590493,1.78336742527747,
10.0093949743796));
#65595=CARTESIAN_POINT('Ctrl Pts',(0.0605337415108948,1.78346075964565,
10.0094255279822));
#65596=CARTESIAN_POINT('Ctrl Pts',(0.0614093543027511,1.78362961399434,
10.0094802029463));
#65597=CARTESIAN_POINT('Ctrl Pts',(0.061794936038622,1.78370470156029,10.0095043104668));
#65598=CARTESIAN_POINT('Ctrl Pts',(0.0626095111423033,1.78386487696688,
10.0095553057556));
#65599=CARTESIAN_POINT('Ctrl Pts',(0.0630384701982962,1.78395013340819,
10.0095821988651));
#65600=CARTESIAN_POINT('Ctrl Pts',(0.0641756528600635,1.78417855791006,
10.0096535967567));
#65601=CARTESIAN_POINT('Ctrl Pts',(0.0648835678082039,1.78432323443327,
10.0096981496821));
#65602=CARTESIAN_POINT('Ctrl Pts',(0.0681341695864665,1.78499895582335,
10.0099032226238));
#65603=CARTESIAN_POINT('Ctrl Pts',(0.0706708067876858,1.78555833715908,
10.0100646474071));
#65604=CARTESIAN_POINT('Ctrl Pts',(0.0898402821141142,1.79002927764957,
10.0112954443779));
#65605=CARTESIAN_POINT('Ctrl Pts',(0.106142484036681,1.79522675361664,10.0124067915338));
#65606=CARTESIAN_POINT('Ctrl Pts',(0.150179965491559,1.81323002052585,10.0155814421998));
#65607=CARTESIAN_POINT('Ctrl Pts',(0.176624734051185,1.82871641425103,10.0177028746455));
#65608=CARTESIAN_POINT('Ctrl Pts',(0.201671789353781,1.84861999108225,10.0197262758824));
#65609=CARTESIAN_POINT('Ctrl Pts',(0.202838069695964,1.84956011261482,10.0198204890985));
#65610=CARTESIAN_POINT('Ctrl Pts',(0.204327838149167,1.85077822736923,10.0199407825683));
#65611=CARTESIAN_POINT('Ctrl Pts',(0.204657363582775,1.85104875792182,10.0199673873037));
#65612=CARTESIAN_POINT('Ctrl Pts',(0.205178304540571,1.85147816826047,10.0200094397432));
#65613=CARTESIAN_POINT('Ctrl Pts',(0.205370073154367,1.85163661590547,10.0200249186697));
#65614=CARTESIAN_POINT('Ctrl Pts',(0.205726712068326,1.85193198211999,10.0200537024504));
#65615=CARTESIAN_POINT('Ctrl Pts',(0.205891627962975,1.85206884203781,10.0200670113537));
#65616=CARTESIAN_POINT('Ctrl Pts',(0.206262723577866,1.85237743138563,10.0200969566319));
#65617=CARTESIAN_POINT('Ctrl Pts',(0.206468824965786,1.85254925349993,10.0201135860709));
#65618=CARTESIAN_POINT('Ctrl Pts',(0.206898908070391,1.85290871557259,10.0201482845458));
#65619=CARTESIAN_POINT('Ctrl Pts',(0.207122849832648,1.85309640326738,10.0201663500833));
#65620=CARTESIAN_POINT('Ctrl Pts',(0.207706270799739,1.85358672619504,10.0202134114093));
#65621=CARTESIAN_POINT('Ctrl Pts',(0.20806534550537,1.8538898449006,10.0202423723477));
#65622=CARTESIAN_POINT('Ctrl Pts',(0.209125658827076,1.85478890457828,10.0203278849192));
#65623=CARTESIAN_POINT('Ctrl Pts',(0.209825016394904,1.85538707098831,10.0203842787865));
#65624=CARTESIAN_POINT('Ctrl Pts',(0.21753954073014,1.8620427977235,10.0210063854916));
#65625=CARTESIAN_POINT('Ctrl Pts',(0.224293554856847,1.86839793062974,10.0215513762008));
#65626=CARTESIAN_POINT('Ctrl Pts',(0.250570037705361,1.89535197081546,10.023718920552));
#65627=CARTESIAN_POINT('Ctrl Pts',(0.267606251569835,1.91819448574496,10.0252490948596));
#65628=CARTESIAN_POINT('Ctrl Pts',(0.287218367823149,1.95334456810785,10.027571557539));
#65629=CARTESIAN_POINT('Ctrl Pts',(0.292426433353957,1.96402596669467,10.0282718903007));
#65630=CARTESIAN_POINT('Ctrl Pts',(0.297456134115654,1.97597494648757,10.0290599145351));
#65631=CARTESIAN_POINT('Ctrl Pts',(0.297874238444646,1.97698250674355,10.0291263925352));
#65632=CARTESIAN_POINT('Ctrl Pts',(0.298487274332091,1.97848126919075,10.0292253316143));
#65633=CARTESIAN_POINT('Ctrl Pts',(0.298686129149449,1.97897086663054,10.0292576600168));
#65634=CARTESIAN_POINT('Ctrl Pts',(0.299024442254204,1.97980973418222,10.0293130657912));
#65635=CARTESIAN_POINT('Ctrl Pts',(0.299164495439643,1.9801587644874,10.0293361230424));
#65636=CARTESIAN_POINT('Ctrl Pts',(0.299435754494424,1.98083821523551,10.0293810170383));
#65637=CARTESIAN_POINT('Ctrl Pts',(0.29956702524685,1.98116860936139,10.0294028515589));
#65638=CARTESIAN_POINT('Ctrl Pts',(0.299879677716944,1.9819593319255,10.0294551175539));
#65639=CARTESIAN_POINT('Ctrl Pts',(0.300060546166007,1.98241986112747,10.0294855662441));
#65640=CARTESIAN_POINT('Ctrl Pts',(0.300599729566863,1.98380208213375,10.0295769797203));
#65641=CARTESIAN_POINT('Ctrl Pts',(0.300954861026685,1.98472500218336,10.0296380512263));
#65642=CARTESIAN_POINT('Ctrl Pts',(0.304058379934767,1.99290256438331,10.030179501053));
#65643=CARTESIAN_POINT('Ctrl Pts',(0.306548023346412,2.00025205919967,10.030668467506));
#65644=CARTESIAN_POINT('Ctrl Pts',(0.310662501093312,2.01401374049299,10.0315895083546));
#65645=CARTESIAN_POINT('Ctrl Pts',(0.312359840783128,2.02040008244564,10.0320190321001));
#65646=CARTESIAN_POINT('Ctrl Pts',(0.31761456941973,2.04294117313595,10.0335414190866));
#65647=CARTESIAN_POINT('Ctrl Pts',(0.320123685651727,2.05931257776974,10.0346599663261));
#65648=CARTESIAN_POINT('Ctrl Pts',(0.322808464585944,2.09496919208831,10.0370793280725));
#65649=CARTESIAN_POINT('Ctrl Pts',(0.322534243252063,2.11422892232142,10.0383756988085));
#65650=CARTESIAN_POINT('Ctrl Pts',(0.32042751547386,2.13447700439629,10.0396588409609));
#65651=CARTESIAN_POINT('Ctrl Pts',(0.320304461898369,2.13560208256892,10.0397298679327));
#65652=CARTESIAN_POINT('Ctrl Pts',(0.320131972249648,2.13710581810401,10.0398244168798));
#65653=CARTESIAN_POINT('Ctrl Pts',(0.320087788372978,2.1374850521102,10.039848229011));
#65654=CARTESIAN_POINT('Ctrl Pts',(0.320017675697562,2.13807767154349,10.0398853877054));
#65655=CARTESIAN_POINT('Ctrl Pts',(0.31999220734791,2.13829110949441,10.0398987602574));
#65656=CARTESIAN_POINT('Ctrl Pts',(0.319940871747783,2.13871770025601,10.039925466224));
#65657=CARTESIAN_POINT('Ctrl Pts',(0.319915005221037,2.13893085103824,10.039938799498));
#65658=CARTESIAN_POINT('Ctrl Pts',(0.31985584637584,2.13941430367954,10.0399690170347));
#65659=CARTESIAN_POINT('Ctrl Pts',(0.319822424494001,2.13968458879009,10.0399858938383));
#65660=CARTESIAN_POINT('Ctrl Pts',(0.319751749917167,2.1402502507352,10.0400211792267));
#65661=CARTESIAN_POINT('Ctrl Pts',(0.319714430431215,2.14054561918466,10.0400395840306));
#65662=CARTESIAN_POINT('Ctrl Pts',(0.319615473795863,2.14132018835923,10.040087797096));
#65663=CARTESIAN_POINT('Ctrl Pts',(0.319553167957908,2.14179930514878,10.0401175681276));
#65664=CARTESIAN_POINT('Ctrl Pts',(0.319364365143869,2.14322605583921,10.0402060736799));
#65665=CARTESIAN_POINT('Ctrl Pts',(0.319234727294358,2.14417327890292,10.0402646369325));
#65666=CARTESIAN_POINT('Ctrl Pts',(0.317713408985149,2.1549324724664,10.0409277538621));
#65667=CARTESIAN_POINT('Ctrl Pts',(0.315873912944015,2.16467689009704,10.0415086670916));
#65668=CARTESIAN_POINT('Ctrl Pts',(0.306566166799982,2.20394921670598,10.0438252563361));
#65669=CARTESIAN_POINT('Ctrl Pts',(0.295381578901694,2.23243173423859,10.0454630598711));
#65670=CARTESIAN_POINT('Ctrl Pts',(0.275823699545849,2.26693496690597,10.0477766090386));
#65671=CARTESIAN_POINT('Ctrl Pts',(0.270941100815863,2.27474808060135,10.0483239516167));
#65672=CARTESIAN_POINT('Ctrl Pts',(0.265086969010754,2.28327948655966,10.0489531946683));
#65673=CARTESIAN_POINT('Ctrl Pts',(0.264437970117213,2.28421463362371,10.0490226066098));
#65674=CARTESIAN_POINT('Ctrl Pts',(0.263486216019777,2.28557062896258,10.0491239055313));
#65675=CARTESIAN_POINT('Ctrl Pts',(0.263187372965285,2.28599422322389,10.0491556427783));
#65676=CARTESIAN_POINT('Ctrl Pts',(0.262658014215155,2.28674073097179,10.0492117389238));
#65677=CARTESIAN_POINT('Ctrl Pts',(0.262427921269005,2.28706394407133,10.0492360815443));
#65678=CARTESIAN_POINT('Ctrl Pts',(0.261950830653486,2.28773150382335,10.049286472444));
#65679=CARTESIAN_POINT('Ctrl Pts',(0.261703749579431,2.28807578967311,10.0493125239089));
#65680=CARTESIAN_POINT('Ctrl Pts',(0.261069126621931,2.28895640924114,10.0493793208585));
#65681=CARTESIAN_POINT('Ctrl Pts',(0.260680612075579,2.28949203662928,10.0494201039213));
#65682=CARTESIAN_POINT('Ctrl Pts',(0.259085279263435,2.2916772580937,10.0495871250029));
#65683=CARTESIAN_POINT('Ctrl Pts',(0.257864451417593,2.2933165217645,10.0497139069075));
#65684=CARTESIAN_POINT('Ctrl Pts',(0.249691029458126,2.30407617424146,10.0505561218514));
#65685=CARTESIAN_POINT('Ctrl Pts',(0.242272222905628,2.31283047775968,10.0512900464087));
#65686=CARTESIAN_POINT('Ctrl Pts',(0.230993583310355,2.32478395707709,10.0523655881955));
#65687=CARTESIAN_POINT('Ctrl Pts',(0.227500733080137,2.32831836522635,10.0526936302465));
#65688=CARTESIAN_POINT('Ctrl Pts',(0.221149700209213,2.334454487639,10.0532808609856));
#65689=CARTESIAN_POINT('Ctrl Pts',(0.218323735815392,2.33708825744754,10.0535390780551));
#65690=CARTESIAN_POINT('Ctrl Pts',(0.194683860401407,2.35833925820666,10.0556724792574));
#65691=CARTESIAN_POINT('Ctrl Pts',(0.171577836929273,2.37423013679064,10.0576037036079));
#65692=CARTESIAN_POINT('Ctrl Pts',(0.145370249745591,2.38762986132018,10.0594654836716));
#65693=CARTESIAN_POINT('Ctrl Pts',(0.144023647930538,2.38830649607923,10.0595602695413));
#65694=CARTESIAN_POINT('Ctrl Pts',(0.142293638560569,2.38916063771463,10.0596808774873));
#65695=CARTESIAN_POINT('Ctrl Pts',(0.141914588918462,2.38934685661899,10.0597072317602));
#65696=CARTESIAN_POINT('Ctrl Pts',(0.141310303128175,2.38964225607499,10.0597491313995));
#65697=CARTESIAN_POINT('Ctrl Pts',(0.14108530559608,2.38975191944191,10.0597647068882));
#65698=CARTESIAN_POINT('Ctrl Pts',(0.140667597538195,2.3899549076566,10.0597935756167));
#65699=CARTESIAN_POINT('Ctrl Pts',(0.140474923219946,2.39004830187067,10.0598068731337));
#65700=CARTESIAN_POINT('Ctrl Pts',(0.140042562181576,2.39025734654998,10.0598366711179));
#65701=CARTESIAN_POINT('Ctrl Pts',(0.139802825765173,2.39037289191299,10.0598531649365));
#65702=CARTESIAN_POINT('Ctrl Pts',(0.139302312836595,2.39061335976269,10.0598875409973));
#65703=CARTESIAN_POINT('Ctrl Pts',(0.139041510597097,2.39073822859509,10.059905419894));
#65704=CARTESIAN_POINT('Ctrl Pts',(0.138362997413867,2.39106197038264,10.059951848352));
#65705=CARTESIAN_POINT('Ctrl Pts',(0.137945023846851,2.39126029605574,10.0599803643388));
#65706=CARTESIAN_POINT('Ctrl Pts',(0.136712012319527,2.39184210225519,10.0600642409506));
#65707=CARTESIAN_POINT('Ctrl Pts',(0.135895784014709,2.39222307043142,10.060119450942));
#65708=CARTESIAN_POINT('Ctrl Pts',(0.133051519628272,2.39353611423178,10.0603107826097));
#65709=CARTESIAN_POINT('Ctrl Pts',(0.131015354820701,2.39445056401582,10.0604458944035));
#65710=CARTESIAN_POINT('Ctrl Pts',(0.121643065576511,2.39854322530255,10.0610600536024));
#65711=CARTESIAN_POINT('Ctrl Pts',(0.114199220759256,2.40146915449024,10.0615262725987));
#65712=CARTESIAN_POINT('Ctrl Pts',(0.0785255281206204,2.41397996879105,
10.0636941082193));
#65713=CARTESIAN_POINT('Ctrl Pts',(0.0491651148219065,2.41989473106437,
10.0652998090308));
#65714=CARTESIAN_POINT('Ctrl Pts',(0.00981194732096487,2.42226903786307,
10.0675955972732));
#65715=CARTESIAN_POINT('Ctrl Pts',(0.000195004456875578,2.42241827066467,
10.0681663027694));
#65716=CARTESIAN_POINT('Ctrl Pts',(-0.0105491199298504,2.42210430337797,
10.0688199306789));
#65717=CARTESIAN_POINT('Ctrl Pts',(-0.0116844687873054,2.42206511658875,
10.0688891979826));
#65718=CARTESIAN_POINT('Ctrl Pts',(-0.0132980408704505,2.4220008804739,
10.0689879297154));
#65719=CARTESIAN_POINT('Ctrl Pts',(-0.0137764611758626,2.42198076655372,
10.0690172394603));
#65720=CARTESIAN_POINT('Ctrl Pts',(-0.0146542047701276,2.42194190425937,
10.0690710799557));
#65721=CARTESIAN_POINT('Ctrl Pts',(-0.0150535420119537,2.42192347896077,
10.0690956005338));
#65722=CARTESIAN_POINT('Ctrl Pts',(-0.0158629427642707,2.42188462411497,
10.0691453521569));
#65723=CARTESIAN_POINT('Ctrl Pts',(-0.0162730034983033,2.42186415387464,
10.0691705844336));
#65724=CARTESIAN_POINT('Ctrl Pts',(-0.0172828762691735,2.42181180619153,
10.0692327919395));
#65725=CARTESIAN_POINT('Ctrl Pts',(-0.0178826386742273,2.42177903543059,
10.069269795128));
#65726=CARTESIAN_POINT('Ctrl Pts',(-0.0200732184320803,2.42165319972201,
10.069405161047));
#65727=CARTESIAN_POINT('Ctrl Pts',(-0.0216634109427543,2.42155001394733,
10.0695038407802));
#65728=CARTESIAN_POINT('Ctrl Pts',(-0.0308585546252037,2.42088483326614,
10.0700769067982));
#65729=CARTESIAN_POINT('Ctrl Pts',(-0.0384418589597235,2.42006489058921,
10.0705593454794));
#65730=CARTESIAN_POINT('Ctrl Pts',(-0.0572952377763669,2.41734670606582,
10.0717846142746));
#65731=CARTESIAN_POINT('Ctrl Pts',(-0.0685062651080066,2.41511668192953,
10.0725367942953));
#65732=CARTESIAN_POINT('Ctrl Pts',(-0.0827250179006591,2.41149368892836,
10.0735176224775));
#65733=CARTESIAN_POINT('Ctrl Pts',(-0.0858633084840799,2.41064326558604,
10.0737357880406));
#65734=CARTESIAN_POINT('Ctrl Pts',(-0.0915917984008716,2.40899750260009,
10.0741368471783));
#65735=CARTESIAN_POINT('Ctrl Pts',(-0.0941858918084206,2.40821669598797,
10.074319538732));
#65736=CARTESIAN_POINT('Ctrl Pts',(-0.0989884622834605,2.40670485841018,
10.0746595819456));
#65737=CARTESIAN_POINT('Ctrl Pts',(-0.101199478592809,2.40598243623779,
10.074816855182));
#65738=CARTESIAN_POINT('Ctrl Pts',(-0.107818674728302,2.40374010271626,
10.0752896496324));
#65739=CARTESIAN_POINT('Ctrl Pts',(-0.11220189867558,2.40214839191601,10.0756053726803));
#65740=CARTESIAN_POINT('Ctrl Pts',(-0.129177695927073,2.39556349220256,
10.0768358176508));
#65741=CARTESIAN_POINT('Ctrl Pts',(-0.141486106149191,2.38987307802758,
10.0777452325721));
#65742=CARTESIAN_POINT('Ctrl Pts',(-0.157296139880944,2.38131604874326,
10.0789071394773));
#65743=CARTESIAN_POINT('Ctrl Pts',(-0.161147908016124,2.37912748255708,
10.0791896371829));
#65744=CARTESIAN_POINT('Ctrl Pts',(-0.165478887266146,2.37654707994299,
10.079505567464));
#65745=CARTESIAN_POINT('Ctrl Pts',(-0.16600332705698,2.37623259216902,10.0795437944543));
#65746=CARTESIAN_POINT('Ctrl Pts',(-0.166770336862275,2.37576967061939,
10.0795996562494));
#65747=CARTESIAN_POINT('Ctrl Pts',(-0.167013606618918,2.37562240782694,
10.0796173668758));
#65748=CARTESIAN_POINT('Ctrl Pts',(-0.167440375738403,2.37536329163493,
10.0796484242046));
#65749=CARTESIAN_POINT('Ctrl Pts',(-0.167623958324693,2.37525157656968,
10.0796617800078));
#65750=CARTESIAN_POINT('Ctrl Pts',(-0.168007895648443,2.37501741355672,
10.0796897031084));
#65751=CARTESIAN_POINT('Ctrl Pts',(-0.168208227897725,2.37489493052437,
10.0797042680053));
#65752=CARTESIAN_POINT('Ctrl Pts',(-0.168617436603636,2.37464412572187,
10.0797340093067));
#65753=CARTESIAN_POINT('Ctrl Pts',(-0.168826300927369,2.37451578431203,
10.0797491844028));
#65754=CARTESIAN_POINT('Ctrl Pts',(-0.169339320966691,2.37419974059354,
10.0797864458234));
#65755=CARTESIAN_POINT('Ctrl Pts',(-0.169643312154016,2.37401176984087,
10.0798085146099));
#65756=CARTESIAN_POINT('Ctrl Pts',(-0.170481351914948,2.37349164485476,
10.0798693262738));
#65757=CARTESIAN_POINT('Ctrl Pts',(-0.171014745343242,2.37315843030494,
10.0799080008233));
#65758=CARTESIAN_POINT('Ctrl Pts',(-0.172706811089052,2.37209448633088,
10.080030600397));
#65759=CARTESIAN_POINT('Ctrl Pts',(-0.17386181949199,2.37135791855282,10.0801141580076));
#65760=CARTESIAN_POINT('Ctrl Pts',(-0.178340812662885,2.36846125354458,
10.080437824106));
#65761=CARTESIAN_POINT('Ctrl Pts',(-0.181629668934853,2.36624717197366,
10.0806747085568));
#65762=CARTESIAN_POINT('Ctrl Pts',(-0.190121772504208,2.36029961146984,
10.0812866340461));
#65763=CARTESIAN_POINT('Ctrl Pts',(-0.195256212302711,2.35647065480835,
10.0816568964678));
#65764=CARTESIAN_POINT('Ctrl Pts',(-0.223204838544721,2.33430207943499,
10.083694306211));
#65765=CARTESIAN_POINT('Ctrl Pts',(-0.243551203222896,2.31307461682332,
10.0852752850844));
#65766=CARTESIAN_POINT('Ctrl Pts',(-0.266156278462439,2.28195204779663,
10.0875192617124));
#65767=CARTESIAN_POINT('Ctrl Pts',(-0.271238260151538,2.27428566776057,
10.0880657110223));
#65768=CARTESIAN_POINT('Ctrl Pts',(-0.276572796725634,2.26543868447924,
10.0886939876289));
#65769=CARTESIAN_POINT('Ctrl Pts',(-0.277155151356056,2.26446121802928,
10.0887633696755));
#65770=CARTESIAN_POINT('Ctrl Pts',(-0.277995235659732,2.26303402473525,
10.0888646329674));
#65771=CARTESIAN_POINT('Ctrl Pts',(-0.278257080324322,2.26258671998448,
10.0888963646294));
#65772=CARTESIAN_POINT('Ctrl Pts',(-0.278717443517387,2.26179591991917,
10.0889524542699));
#65773=CARTESIAN_POINT('Ctrl Pts',(-0.278916409446151,2.26145268521394,
10.0889767959825));
#65774=CARTESIAN_POINT('Ctrl Pts',(-0.279326607812478,2.26074203372973,
10.0890271882922));
#65775=CARTESIAN_POINT('Ctrl Pts',(-0.279537750199431,2.26037456609545,
10.0890532420813));
#65776=CARTESIAN_POINT('Ctrl Pts',(-0.280076777295388,2.25943215645658,
10.0891200518152));
#65777=CARTESIAN_POINT('Ctrl Pts',(-0.280403615619079,2.25885662098217,
10.0891608453661));
#65778=CARTESIAN_POINT('Ctrl Pts',(-0.28173318929537,2.25649846293582,10.0893279624801));
#65779=CARTESIAN_POINT('Ctrl Pts',(-0.282720699522567,2.25470735148448,
10.0894548307171));
#65780=CARTESIAN_POINT('Ctrl Pts',(-0.289138256698171,2.24280074309152,
10.0902979225703));
#65781=CARTESIAN_POINT('Ctrl Pts',(-0.294040889921586,2.23241180373817,
10.0910326791248));
#65782=CARTESIAN_POINT('Ctrl Pts',(-0.311442017544307,2.18977810527554,
10.0940464125566));
#65783=CARTESIAN_POINT('Ctrl Pts',(-0.319268929465149,2.15588456150291,
10.0964678626981));
#65784=CARTESIAN_POINT('Ctrl Pts',(-0.321696806114809,2.11939981487197,
10.0988163687835));
#65785=CARTESIAN_POINT('Ctrl Pts',(-0.321811173040243,2.11739992055465,
10.0989441957669));
#65786=CARTESIAN_POINT('Ctrl Pts',(-0.321987311309268,2.11371786375243,
10.0991777192447));
#65787=CARTESIAN_POINT('Ctrl Pts',(-0.322054564250783,2.11203604448895,
10.0992836849202));
#65788=CARTESIAN_POINT('Ctrl Pts',(-0.322122783971838,2.10991370253467,
10.0994164600543));
#65789=CARTESIAN_POINT('Ctrl Pts',(-0.322136026533639,2.10947364060515,
10.0994439393119));
#65790=CARTESIAN_POINT('Ctrl Pts',(-0.322155500553171,2.10877917124101,
10.0994872223651));
#65791=CARTESIAN_POINT('Ctrl Pts',(-0.322162332459915,2.10852478324684,
10.0995030597352));
#65792=CARTESIAN_POINT('Ctrl Pts',(-0.322173911592672,2.10807372378392,
10.0995311099667));
#65793=CARTESIAN_POINT('Ctrl Pts',(-0.322178780022493,2.10787705721271,
10.0995433295934));
#65794=CARTESIAN_POINT('Ctrl Pts',(-0.32218840795021,2.1074731765057,10.0995684025574));
#65795=CARTESIAN_POINT('Ctrl Pts',(-0.322193147609165,2.10726596303698,
10.0995812547188));
#65796=CARTESIAN_POINT('Ctrl Pts',(-0.322203252332036,2.10680473110434,
10.0996098363601));
#65797=CARTESIAN_POINT('Ctrl Pts',(-0.322208516919066,2.10655071023746,
10.0996255601846));
#65798=CARTESIAN_POINT('Ctrl Pts',(-0.322220884430889,2.10591784060842,
10.0996646920056));
#65799=CARTESIAN_POINT('Ctrl Pts',(-0.32222761964591,2.10553898381157,10.0996880795481));
#65800=CARTESIAN_POINT('Ctrl Pts',(-0.322260867011647,2.10346278515451,
10.0998160428866));
#65801=CARTESIAN_POINT('Ctrl Pts',(-0.322274636765795,2.10176523081878,
10.0999199208158));
#65802=CARTESIAN_POINT('Ctrl Pts',(-0.322274992908106,2.10006760976513,
10.1000231250268));
#65803=CARTESIAN_POINT('',(-0.322021890547819,2.10026805526597,10.2247225257975));
#65804=CARTESIAN_POINT('Ctrl Pts',(-0.32279818296466,2.10004841125406,10.0997227245674));
#65805=CARTESIAN_POINT('Ctrl Pts',(-0.32257517298749,1.99588884229921,10.1061816902479));
#65806=CARTESIAN_POINT('Ctrl Pts',(-0.21115554484217,1.78450861019514,10.1192641037693));
#65807=CARTESIAN_POINT('Ctrl Pts',(0.14909372275915,1.74930620373942,10.1389699651317));
#65808=CARTESIAN_POINT('Ctrl Pts',(0.375576748934469,2.03552378297651,10.1588403086545));
#65809=CARTESIAN_POINT('Ctrl Pts',(0.25751923811976,2.38088951368832,10.1787106521773));
#65810=CARTESIAN_POINT('Ctrl Pts',(-0.0967771155912757,2.46857735524538,
10.1985809957001));
#65811=CARTESIAN_POINT('Ctrl Pts',(-0.301720943666828,2.27527702420129,
10.2139182869069));
#65812=CARTESIAN_POINT('Ctrl Pts',(-0.322284932565275,2.13418886036719,
10.2226321302726));
#65813=CARTESIAN_POINT('Ctrl Pts',(-0.322021890547819,2.10026805526597,
10.2247225257975));
#65814=CARTESIAN_POINT('',(-0.32227501893165,2.09982663045473,10.4749490325485));
#65815=CARTESIAN_POINT('Ctrl Pts',(-0.322274896795217,2.10025791594028,
10.2245769286166));
#65816=CARTESIAN_POINT('Ctrl Pts',(-0.322289186763215,2.08240210618882,
10.2255878655148));
#65817=CARTESIAN_POINT('Ctrl Pts',(-0.320819566308015,2.06457809785206,
10.2266228926931));
#65818=CARTESIAN_POINT('Ctrl Pts',(-0.317749005383167,2.04617253167104,
10.2277574470772));
#65819=CARTESIAN_POINT('Ctrl Pts',(-0.317613233356406,2.04537710418631,
10.2278066036694));
#65820=CARTESIAN_POINT('Ctrl Pts',(-0.317386802593762,2.04407993994302,
10.2278869741934));
#65821=CARTESIAN_POINT('Ctrl Pts',(-0.317297937453292,2.04357789032069,
10.2279181312054));
#65822=CARTESIAN_POINT('Ctrl Pts',(-0.317139251707659,2.04269361622364,
10.2279730991149));
#65823=CARTESIAN_POINT('Ctrl Pts',(-0.317069930372312,2.04231130226097,
10.2279968941079));
#65824=CARTESIAN_POINT('Ctrl Pts',(-0.316928446102455,2.04153896165246,
10.2280450246363));
#65825=CARTESIAN_POINT('Ctrl Pts',(-0.316856254180393,2.04114894106235,
10.2280693610562));
#65826=CARTESIAN_POINT('Ctrl Pts',(-0.316714825281104,2.04039266817819,
10.2281166117624));
#65827=CARTESIAN_POINT('Ctrl Pts',(-0.316645672528919,2.04002640058617,
10.2281395233296));
#65828=CARTESIAN_POINT('Ctrl Pts',(-0.316479287063874,2.03915344983397,
10.228194196631));
#65829=CARTESIAN_POINT('Ctrl Pts',(-0.316381472969988,2.03864687975364,
10.2282259768727));
#65830=CARTESIAN_POINT('Ctrl Pts',(-0.316082741725912,2.03711949070694,
10.2283219620967));
#65831=CARTESIAN_POINT('Ctrl Pts',(-0.315878098760873,2.0360994151166,10.2283862859247));
#65832=CARTESIAN_POINT('Ctrl Pts',(-0.313698295684725,2.02550023138706,
10.2290569653176));
#65833=CARTESIAN_POINT('Ctrl Pts',(-0.311293176051704,2.01601570756492,
10.2296770624348));
#65834=CARTESIAN_POINT('Ctrl Pts',(-0.306633324098645,2.00061695603321,
10.2307184494957));
#65835=CARTESIAN_POINT('Ctrl Pts',(-0.304628990680189,1.9946332347348,10.2311319335632));
#65836=CARTESIAN_POINT('Ctrl Pts',(-0.301630268935016,1.98648349238708,
10.2317067818988));
#65837=CARTESIAN_POINT('Ctrl Pts',(-0.300785506333512,1.98426368122619,
10.2318645692362));
#65838=CARTESIAN_POINT('Ctrl Pts',(-0.291491246625091,1.96063009646229,
10.2335570552045));
#65839=CARTESIAN_POINT('Ctrl Pts',(-0.280795620286707,1.94017235607578,
10.2351395371016));
#65840=CARTESIAN_POINT('Ctrl Pts',(-0.264497698000053,1.91576592051357,
10.2370810044563));
#65841=CARTESIAN_POINT('Ctrl Pts',(-0.260828605663076,1.9106070804191,10.237494330679));
#65842=CARTESIAN_POINT('Ctrl Pts',(-0.255220716385519,1.90319462967187,
10.2380888941103));
#65843=CARTESIAN_POINT('Ctrl Pts',(-0.253399087442226,1.9008546463468,10.2382766871127));
#65844=CARTESIAN_POINT('Ctrl Pts',(-0.251230253392885,1.8981466139241,10.2384938075672));
#65845=CARTESIAN_POINT('Ctrl Pts',(-0.250914238234083,1.89775392525496,
10.2385252866926));
#65846=CARTESIAN_POINT('Ctrl Pts',(-0.250430235487796,1.89715537134316,
10.2385732584181));
#65847=CARTESIAN_POINT('Ctrl Pts',(-0.250262914271691,1.89694897202214,
10.238589798649));
#65848=CARTESIAN_POINT('Ctrl Pts',(-0.249971239873216,1.89659008486088,
10.2386185552105));
#65849=CARTESIAN_POINT('Ctrl Pts',(-0.249847002642167,1.89643750440697,
10.2386307798773));
#65850=CARTESIAN_POINT('Ctrl Pts',(-0.249565467325961,1.89609238622371,
10.2386584279182));
#65851=CARTESIAN_POINT('Ctrl Pts',(-0.2494080864596,1.89589991708202,10.2386738451439));
#65852=CARTESIAN_POINT('Ctrl Pts',(-0.248980605991111,1.89537836205425,
10.2387156185595));
#65853=CARTESIAN_POINT('Ctrl Pts',(-0.248710075562783,1.89504962748558,
10.238741943506));
#65854=CARTESIAN_POINT('Ctrl Pts',(-0.247488309677663,1.89357098234382,
10.2388603366209));
#65855=CARTESIAN_POINT('Ctrl Pts',(-0.24652972554941,1.89242712754289,10.2389518791127));
#65856=CARTESIAN_POINT('Ctrl Pts',(-0.2270735993675,1.86953551928615,10.2407839546233));
#65857=CARTESIAN_POINT('Ctrl Pts',(-0.205771740181726,1.85033042717011,
10.2423300020338));
#65858=CARTESIAN_POINT('Ctrl Pts',(-0.174358043342163,1.8287968143773,10.2444717581156));
#65859=CARTESIAN_POINT('Ctrl Pts',(-0.166267415039652,1.82376273558261,
10.2450120249765));
#65860=CARTESIAN_POINT('Ctrl Pts',(-0.152254961981358,1.8158828869014,10.2459416839309));
#65861=CARTESIAN_POINT('Ctrl Pts',(-0.146447500848813,1.81284633238072,
10.2463252832646));
#65862=CARTESIAN_POINT('Ctrl Pts',(-0.135862035555112,1.80771616098096,
10.2470246592357));
#65863=CARTESIAN_POINT('Ctrl Pts',(-0.131118066165703,1.80555750440072,
10.2473381415954));
#65864=CARTESIAN_POINT('Ctrl Pts',(-0.125500300067949,1.80316393068865,
10.2477101674222));
#65865=CARTESIAN_POINT('Ctrl Pts',(-0.124675103988472,1.80281639382124,
10.2477648339227));
#65866=CARTESIAN_POINT('Ctrl Pts',(-0.123489723870174,1.80232296909608,
10.2478433929205));
#65867=CARTESIAN_POINT('Ctrl Pts',(-0.123130702395561,1.80217428459787,
10.2478671905697));
#65868=CARTESIAN_POINT('Ctrl Pts',(-0.122404655649986,1.80187513816042,
10.2479153251275));
#65869=CARTESIAN_POINT('Ctrl Pts',(-0.12203761980767,1.80172470380358,10.2479396629184));
#65870=CARTESIAN_POINT('Ctrl Pts',(-0.121325191944509,1.80143424119896,
10.2479869124249));
#65871=CARTESIAN_POINT('Ctrl Pts',(-0.120979832739626,1.80129413364098,
10.2480098214143));
#65872=CARTESIAN_POINT('Ctrl Pts',(-0.120155957729404,1.80096156188959,
10.2480644824227));
#65873=CARTESIAN_POINT('Ctrl Pts',(-0.119677222516891,1.80076964717615,
10.24809625293));
#65874=CARTESIAN_POINT('Ctrl Pts',(-0.118231989138262,1.80019430708374,
10.2481921895673));
#65875=CARTESIAN_POINT('Ctrl Pts',(-0.117264101098603,1.79981441188242,
10.2482564743766));
#65876=CARTESIAN_POINT('Ctrl Pts',(-0.10719448462534,1.79591822830214,10.2489256687463));
#65877=CARTESIAN_POINT('Ctrl Pts',(-0.0979402591169397,1.79281267297462,
10.2495442535744));
#65878=CARTESIAN_POINT('Ctrl Pts',(-0.0825642552487831,1.78841821766854,
10.2505792789928));
#65879=CARTESIAN_POINT('Ctrl Pts',(-0.0765201606717785,1.78687906346459,
10.250987854762));
#65880=CARTESIAN_POINT('Ctrl Pts',(-0.0516971704430958,1.7813194123793,
10.2526712626576));
#65881=CARTESIAN_POINT('Ctrl Pts',(-0.0326220444416347,1.77880594115431,
10.2539802864642));
#65882=CARTESIAN_POINT('Ctrl Pts',(-0.0107480220564935,1.77789301861101,
10.2554546940015));
#65883=CARTESIAN_POINT('Ctrl Pts',(-0.00805610718413378,1.77781445259254,
10.2556356211309));
#65884=CARTESIAN_POINT('Ctrl Pts',(0.00385066369330159,1.77761626566589,
10.2564328642348));
#65885=CARTESIAN_POINT('Ctrl Pts',(0.013067981666414,1.77785817320986,10.2570421222263));
#65886=CARTESIAN_POINT('Ctrl Pts',(0.0258782267889083,1.77874523224125,
10.257867300995));
#65887=CARTESIAN_POINT('Ctrl Pts',(0.0294892036004231,1.77905655007578,
10.2580974898134));
#65888=CARTESIAN_POINT('Ctrl Pts',(0.0336220472947169,1.77948320636909,
10.2583575906857));
#65889=CARTESIAN_POINT('Ctrl Pts',(0.0341496198844267,1.7795389874961,10.2583907306631));
#65890=CARTESIAN_POINT('Ctrl Pts',(0.0349467321499745,1.7796252583088,10.2584407045574));
#65891=CARTESIAN_POINT('Ctrl Pts',(0.0352163717474638,1.77965478563913,
10.2584575923881));
#65892=CARTESIAN_POINT('Ctrl Pts',(0.0357028758430757,1.77970868275124,
10.2584880318516));
#65893=CARTESIAN_POINT('Ctrl Pts',(0.0359197522951721,1.7797329323137,10.2585015902357));
#65894=CARTESIAN_POINT('Ctrl Pts',(0.0363545920404164,1.77978200021622,
10.2585287526718));
#65895=CARTESIAN_POINT('Ctrl Pts',(0.0365725536536326,1.77980682070367,
10.2585423565409));
#65896=CARTESIAN_POINT('Ctrl Pts',(0.0371915625517916,1.77987795095816,
10.2585809600463));
#65897=CARTESIAN_POINT('Ctrl Pts',(0.0375925502096143,1.77992479199297,
10.2586059296149));
#65898=CARTESIAN_POINT('Ctrl Pts',(0.0392861385887283,1.78012585360475,
10.2587112356613));
#65899=CARTESIAN_POINT('Ctrl Pts',(0.0405779098421487,1.78028715448827,
10.2587911779562));
#65900=CARTESIAN_POINT('Ctrl Pts',(0.0658722427759269,1.78360138231084,
10.2603497261576));
#65901=CARTESIAN_POINT('Ctrl Pts',(0.0894494086236765,1.78944170706587,
10.2616856986518));
#65902=CARTESIAN_POINT('Ctrl Pts',(0.125252625922606,1.80273210048699,10.2638213674105));
#65903=CARTESIAN_POINT('Ctrl Pts',(0.138021612273087,1.80844138989162,10.2646057966907));
#65904=CARTESIAN_POINT('Ctrl Pts',(0.157349493077741,1.81863827322671,10.2658689643433));
#65905=CARTESIAN_POINT('Ctrl Pts',(0.164182145611151,1.82256984103195,10.2663312666692));
#65906=CARTESIAN_POINT('Ctrl Pts',(0.1731426001874,1.82817277370093,10.2669631005404));
#65907=CARTESIAN_POINT('Ctrl Pts',(0.175403742118743,1.8296263186784,10.267124799998));
#65908=CARTESIAN_POINT('Ctrl Pts',(0.179153710418547,1.83210377500325,10.2673969205519));
#65909=CARTESIAN_POINT('Ctrl Pts',(0.18065260914817,1.83311224470635,10.2675067658514));
#65910=CARTESIAN_POINT('Ctrl Pts',(0.182662229796387,1.83448901778054,10.2676555281578));
#65911=CARTESIAN_POINT('Ctrl Pts',(0.183180486756208,1.8348463065763,10.2676940270045));
#65912=CARTESIAN_POINT('Ctrl Pts',(0.183998891571361,1.8354140632816,10.2677550375467));
#65913=CARTESIAN_POINT('Ctrl Pts',(0.184299734682345,1.83562353016409,10.2677775110391));
#65914=CARTESIAN_POINT('Ctrl Pts',(0.184922829725932,1.83605895057268,10.2678241535532));
#65915=CARTESIAN_POINT('Ctrl Pts',(0.185245026296541,1.83628498192774,10.2678483255271));
#65916=CARTESIAN_POINT('Ctrl Pts',(0.185979875680278,1.83680251383722,10.2679035786525));
#65917=CARTESIAN_POINT('Ctrl Pts',(0.186392257934494,1.83709439515692,10.267934674381));
#65918=CARTESIAN_POINT('Ctrl Pts',(0.18765215391923,1.83799059513652,10.2680299504132));
#65919=CARTESIAN_POINT('Ctrl Pts',(0.18849742138888,1.83859804668583,10.2680942512828));
#65920=CARTESIAN_POINT('Ctrl Pts',(0.194738023071094,1.84312886412046,10.2685718315196));
#65921=CARTESIAN_POINT('Ctrl Pts',(0.200012973693616,1.84721456190441,10.2689914060697));
#65922=CARTESIAN_POINT('Ctrl Pts',(0.206600154996923,1.85265195961018,10.2695367547646));
#65923=CARTESIAN_POINT('Ctrl Pts',(0.208032826312183,1.85385569257473,10.2696567094761));
#65924=CARTESIAN_POINT('Ctrl Pts',(0.210842751077901,1.8562586521992,10.2698946569848));
#65925=CARTESIAN_POINT('Ctrl Pts',(0.212220457098058,1.85745724563736,10.2700126231219));
#65926=CARTESIAN_POINT('Ctrl Pts',(0.215518019065318,1.86037570532157,10.2702981294229));
#65927=CARTESIAN_POINT('Ctrl Pts',(0.217427552842903,1.86210700333985,10.2704660834801));
#65928=CARTESIAN_POINT('Ctrl Pts',(0.237790579035869,1.88101933340853,10.2722855149302));
#65929=CARTESIAN_POINT('Ctrl Pts',(0.254186611715538,1.90028570784347,10.2740151155493));
#65930=CARTESIAN_POINT('Ctrl Pts',(0.273084475597025,1.92863884876591,10.2762957974566));
#65931=CARTESIAN_POINT('Ctrl Pts',(0.27769539110461,1.93621639172546,10.2768820103732));
#65932=CARTESIAN_POINT('Ctrl Pts',(0.283866325917067,1.94736929244823,10.2777025005035));
#65933=CARTESIAN_POINT('Ctrl Pts',(0.285683058870289,1.95079739580824,10.2779491786113));
#65934=CARTESIAN_POINT('Ctrl Pts',(0.287681366006325,1.95473851866833,10.2782258366814));
#65935=CARTESIAN_POINT('Ctrl Pts',(0.287923979962347,1.95522000110996,10.2782595191284));
#65936=CARTESIAN_POINT('Ctrl Pts',(0.28828763770042,1.95594623183476,10.2783101451791));
#65937=CARTESIAN_POINT('Ctrl Pts',(0.288409579060359,1.95619052576048,10.2783271448254));
#65938=CARTESIAN_POINT('Ctrl Pts',(0.288628484209064,1.95663047252122,10.2783577045202));
#65939=CARTESIAN_POINT('Ctrl Pts',(0.288725559394213,1.9568260685049,10.2783712715666));
#65940=CARTESIAN_POINT('Ctrl Pts',(0.28893371816455,1.95724655854101,10.2784003959263));
#65941=CARTESIAN_POINT('Ctrl Pts',(0.28904473767325,1.95747148297549,10.2784159491646));
#65942=CARTESIAN_POINT('Ctrl Pts',(0.28934297783424,1.95807749620927,10.2784577857074));
#65943=CARTESIAN_POINT('Ctrl Pts',(0.289529708970822,1.95845882743037,10.278484038322));
#65944=CARTESIAN_POINT('Ctrl Pts',(0.290385141304568,1.96021451668704,10.278604578435));
#65945=CARTESIAN_POINT('Ctrl Pts',(0.291044828172861,1.9615932810663,10.2786983121904));
#65946=CARTESIAN_POINT('Ctrl Pts',(0.304007117161189,1.98918735780193,10.2805568443567));
#65947=CARTESIAN_POINT('Ctrl Pts',(0.312732948275626,2.01694278963421,10.2821222149668));
#65948=CARTESIAN_POINT('Ctrl Pts',(0.31958088425493,2.05684955171536,10.2844011476943));
#65949=CARTESIAN_POINT('Ctrl Pts',(0.320918958240834,2.06829992143884,10.2850568632171));
#65950=CARTESIAN_POINT('Ctrl Pts',(0.32215558256936,2.08798724773891,10.2862088087062));
#65951=CARTESIAN_POINT('Ctrl Pts',(0.322356978497306,2.09619387131056,10.2866961407268));
#65952=CARTESIAN_POINT('Ctrl Pts',(0.322229719012095,2.1055166859955,10.2872611755887));
#65953=CARTESIAN_POINT('Ctrl Pts',(0.322208641537457,2.10663452399926,10.2873291097527));
#65954=CARTESIAN_POINT('Ctrl Pts',(0.322160317794637,2.10864285582931,10.287451502947));
#65955=CARTESIAN_POINT('Ctrl Pts',(0.322135194773617,2.10953339297213,10.287505895282));
#65956=CARTESIAN_POINT('Ctrl Pts',(0.322091101520321,2.11089591987457,10.2875893042163));
#65957=CARTESIAN_POINT('Ctrl Pts',(0.322074785431026,2.11136799605421,10.2876182376057));
#65958=CARTESIAN_POINT('Ctrl Pts',(0.32204305676644,2.11223103862364,10.287671197105));
#65959=CARTESIAN_POINT('Ctrl Pts',(0.32202796991844,2.11262201668986,10.287695212959));
#65960=CARTESIAN_POINT('Ctrl Pts',(0.321996399459953,2.11340324310042,10.2877432481592));
#65961=CARTESIAN_POINT('Ctrl Pts',(0.321979918313899,2.1137934909015,10.2877672673893));
#65962=CARTESIAN_POINT('Ctrl Pts',(0.321931587402049,2.11489057735698,10.2878348598585));
#65963=CARTESIAN_POINT('Ctrl Pts',(0.321898119373994,2.11559733925875,10.2878784837748));
#65964=CARTESIAN_POINT('Ctrl Pts',(0.321751176765813,2.11849818232091,10.2880578657236));
#65965=CARTESIAN_POINT('Ctrl Pts',(0.32161759690553,2.12069114486311,10.2881942528057));
#65966=CARTESIAN_POINT('Ctrl Pts',(0.321317544338146,2.12490638643325,10.2884579600083));
#65967=CARTESIAN_POINT('Ctrl Pts',(0.321154373679745,2.12692880145859,10.2885851701079));
#65968=CARTESIAN_POINT('Ctrl Pts',(0.318270792049573,2.15889996398606,10.2906072660428));
#65969=CARTESIAN_POINT('Ctrl Pts',(0.311391022411776,2.18831958361098,10.2926433544757));
#65970=CARTESIAN_POINT('Ctrl Pts',(0.294416785485336,2.2321645713901,10.295817557353));
#65971=CARTESIAN_POINT('Ctrl Pts',(0.287055325469245,2.24747242954231,10.2969505211211));
#65972=CARTESIAN_POINT('Ctrl Pts',(0.278167041848874,2.26274142260704,10.2980589376631));
#65973=CARTESIAN_POINT('Ctrl Pts',(0.277809949407753,2.26335025508241,10.2981030946836));
#65974=CARTESIAN_POINT('Ctrl Pts',(0.277295758445557,2.26422037301077,10.2981661395487));
#65975=CARTESIAN_POINT('Ctrl Pts',(0.277140288112532,2.26448261084514,10.2981851319739));
#65976=CARTESIAN_POINT('Ctrl Pts',(0.276870611608382,2.26493601680645,10.2982179549739));
#65977=CARTESIAN_POINT('Ctrl Pts',(0.276756579164224,2.26512728757804,10.2982317969315));
#65978=CARTESIAN_POINT('Ctrl Pts',(0.27653629923257,2.26549590197447,10.2982584640149));
#65979=CARTESIAN_POINT('Ctrl Pts',(0.27643007958993,2.26567326115612,10.2982712909328));
#65980=CARTESIAN_POINT('Ctrl Pts',(0.276177199620714,2.26609458468611,10.2983017526148));
#65981=CARTESIAN_POINT('Ctrl Pts',(0.276030386288819,2.26633845766714,10.2983193773212));
#65982=CARTESIAN_POINT('Ctrl Pts',(0.275588863886564,2.26706968033769,10.2983722018605));
#65983=CARTESIAN_POINT('Ctrl Pts',(0.275293183875609,2.26755644693569,10.2984073385962));
#65984=CARTESIAN_POINT('Ctrl Pts',(0.272389903116128,2.27230757559489,10.2987500460582));
#65985=CARTESIAN_POINT('Ctrl Pts',(0.269684541971895,2.27651179699531,10.299051350106));
#65986=CARTESIAN_POINT('Ctrl Pts',(0.266574439471851,2.28110644785504,10.2993804241255));
#65987=CARTESIAN_POINT('Ctrl Pts',(0.266265426526621,2.28156045791568,10.2994129384818));
#65988=CARTESIAN_POINT('Ctrl Pts',(0.265374717851849,2.28286194609129,10.299506145785));
#65989=CARTESIAN_POINT('Ctrl Pts',(0.264790121657977,2.28370744057338,10.2995666966828));
#65990=CARTESIAN_POINT('Ctrl Pts',(0.263806564645909,2.28511549820027,10.2996675618232));
#65991=CARTESIAN_POINT('Ctrl Pts',(0.263409828921515,2.28567959840798,10.2997079776702));
#65992=CARTESIAN_POINT('Ctrl Pts',(0.260709261774106,2.28949333542838,10.299981297453));
#65993=CARTESIAN_POINT('Ctrl Pts',(0.258347086209562,2.2927013973038,10.3002116002105));
#65994=CARTESIAN_POINT('Ctrl Pts',(0.242452856737662,2.31346951408991,10.3017108681893));
#65995=CARTESIAN_POINT('Ctrl Pts',(0.22719890564693,2.32963747778471,10.302922037766));
#65996=CARTESIAN_POINT('Ctrl Pts',(0.204405324288364,2.34928374436306,10.3046290045851));
#65997=CARTESIAN_POINT('Ctrl Pts',(0.198216914756707,2.35423210914159,10.3050831683033));
#65998=CARTESIAN_POINT('Ctrl Pts',(0.185041992381582,2.36399334526722,10.3060394604555));
#65999=CARTESIAN_POINT('Ctrl Pts',(0.178035295499419,2.36876837572816,10.3065423531545));
#66000=CARTESIAN_POINT('Ctrl Pts',(0.16988337951624,2.37386513074081,10.3071248670226));
#66001=CARTESIAN_POINT('Ctrl Pts',(0.168914598959794,2.37446371468405,10.3071940511584));
#66002=CARTESIAN_POINT('Ctrl Pts',(0.167169924400801,2.37552896719064,10.3073185792449));
#66003=CARTESIAN_POINT('Ctrl Pts',(0.166395194463173,2.37599752647189,10.3073738534692));
#66004=CARTESIAN_POINT('Ctrl Pts',(0.16521104767199,2.37670690442477,10.307458307176));
#66005=CARTESIAN_POINT('Ctrl Pts',(0.164803051474384,2.37695009559504,10.3074874000111));
#66006=CARTESIAN_POINT('Ctrl Pts',(0.164089914202477,2.37737303600528,10.3075382423271));
#66007=CARTESIAN_POINT('Ctrl Pts',(0.163785010927808,2.37755318632567,10.3075599771664));
#66008=CARTESIAN_POINT('Ctrl Pts',(0.163152176645483,2.37792568686343,10.3076050826588));
#66009=CARTESIAN_POINT('Ctrl Pts',(0.162824201111661,2.37811796003331,10.3076284560666));
#66010=CARTESIAN_POINT('Ctrl Pts',(0.162026556817637,2.3785836784028,10.307685293474));
#66011=CARTESIAN_POINT('Ctrl Pts',(0.161556536328935,2.378856516062,10.3077187794156));
#66012=CARTESIAN_POINT('Ctrl Pts',(0.159790137367185,2.3798759110276,10.3078446028563));
#66013=CARTESIAN_POINT('Ctrl Pts',(0.15848927163179,2.38061461870304,10.3079372231037));
#66014=CARTESIAN_POINT('Ctrl Pts',(0.135182726994371,2.39363567905473,10.3095960238398));
#66015=CARTESIAN_POINT('Ctrl Pts',(0.111821227939386,2.40330145987106,10.3112598357882));
#66016=CARTESIAN_POINT('Ctrl Pts',(0.0723803038835808,2.41443864390435,
10.314027925672));
#66017=CARTESIAN_POINT('Ctrl Pts',(0.0568871147793168,2.4176073937109,10.3151029889319));
#66018=CARTESIAN_POINT('Ctrl Pts',(0.0349587514689426,2.42043558379176,
10.316565528261));
#66019=CARTESIAN_POINT('Ctrl Pts',(0.0286709789840776,2.42105928394083,
10.3169780432867));
#66020=CARTESIAN_POINT('Ctrl Pts',(0.0194180102140337,2.42170306834132,
10.3175713311735));
#66021=CARTESIAN_POINT('Ctrl Pts',(0.0164646793796068,2.42186773550386,
10.3177586412581));
#66022=CARTESIAN_POINT('Ctrl Pts',(0.0130061121029357,2.42201284196738,
10.3179752682868));
#66023=CARTESIAN_POINT('Ctrl Pts',(0.0125027967532464,2.42203277694278,
10.3180067258508));
#66024=CARTESIAN_POINT('Ctrl Pts',(0.011733989911379,2.42206142219062,10.3180546715302));
#66025=CARTESIAN_POINT('Ctrl Pts',(0.0114685338580242,2.42207098427995,
10.3180712071972));
#66026=CARTESIAN_POINT('Ctrl Pts',(0.010987316294063,2.42208772269296,10.318101147863));
#66027=CARTESIAN_POINT('Ctrl Pts',(0.0107715602575569,2.42209501039176,
10.3181145590702));
#66028=CARTESIAN_POINT('Ctrl Pts',(0.0103337797621303,2.42210935715143,
10.3181417450994));
#66029=CARTESIAN_POINT('Ctrl Pts',(0.010111756290258,2.42211640342295,10.3181555191432));
#66030=CARTESIAN_POINT('Ctrl Pts',(0.00947249210757115,2.42213602990904,
10.3181951397135));
#66031=CARTESIAN_POINT('Ctrl Pts',(0.00905523204150777,2.42214802909473,
10.3182209535599));
#66032=CARTESIAN_POINT('Ctrl Pts',(0.00722050985474629,2.42219722288538,
10.3183342556767));
#66033=CARTESIAN_POINT('Ctrl Pts',(0.00580280664003967,2.42222587389353,
10.3184212718284));
#66034=CARTESIAN_POINT('Ctrl Pts',(-0.0204808567483181,2.42258352712238,
10.3200253944839));
#66035=CARTESIAN_POINT('Ctrl Pts',(-0.0453068091482655,2.42004269421073,
10.3213932681915));
#66036=CARTESIAN_POINT('Ctrl Pts',(-0.0835976613275468,2.41157378620364,
10.3235874985344));
#66037=CARTESIAN_POINT('Ctrl Pts',(-0.0973756250825092,2.40754631841912,
10.3243944364557));
#66038=CARTESIAN_POINT('Ctrl Pts',(-0.118841462392824,2.39968402662316,
10.3257218652746));
#66039=CARTESIAN_POINT('Ctrl Pts',(-0.126724072873708,2.39643683906635,
10.3262250370146));
#66040=CARTESIAN_POINT('Ctrl Pts',(-0.135980944302133,2.39218680479038,
10.3268391887076));
#66041=CARTESIAN_POINT('Ctrl Pts',(-0.137488183678816,2.39148060878248,
10.3269399379096));
#66042=CARTESIAN_POINT('Ctrl Pts',(-0.14010928043266,2.39022767715955,10.3271164891046));
#66043=CARTESIAN_POINT('Ctrl Pts',(-0.141225585360997,2.38968612156072,
10.3271921115397));
#66044=CARTESIAN_POINT('Ctrl Pts',(-0.142825784352268,2.3888983656394,10.3273011454233));
#66045=CARTESIAN_POINT('Ctrl Pts',(-0.143312236546422,2.38865736296745,
10.3273343753931));
#66046=CARTESIAN_POINT('Ctrl Pts',(-0.144155450027245,2.38823695342095,
10.3273921233431));
#66047=CARTESIAN_POINT('Ctrl Pts',(-0.144512492158249,2.38805810993242,
10.3274166215567));
#66048=CARTESIAN_POINT('Ctrl Pts',(-0.145198421853844,2.38771292941303,
10.3274637750717));
#66049=CARTESIAN_POINT('Ctrl Pts',(-0.145527358498768,2.38754669079455,
10.327486426891));
#66050=CARTESIAN_POINT('Ctrl Pts',(-0.146301701700489,2.3871536827492,10.3275398443999));
#66051=CARTESIAN_POINT('Ctrl Pts',(-0.146746866352384,2.38692644117988,
10.3275706266635));
#66052=CARTESIAN_POINT('Ctrl Pts',(-0.148060545011294,2.3862519955314,10.3276616816947));
#66053=CARTESIAN_POINT('Ctrl Pts',(-0.148927550505155,2.38580187998264,
10.3277220570389));
#66054=CARTESIAN_POINT('Ctrl Pts',(-0.156622937781367,2.38176220953369,
10.3282604625113));
#66055=CARTESIAN_POINT('Ctrl Pts',(-0.163321915227626,2.37793276676771,
10.3287469856543));
#66056=CARTESIAN_POINT('Ctrl Pts',(-0.18264423861435,2.36594734366647,10.3302056700982));
#66057=CARTESIAN_POINT('Ctrl Pts',(-0.194840867457226,2.35714557268727,
10.3312002394182));
#66058=CARTESIAN_POINT('Ctrl Pts',(-0.214612880909925,2.34066042891563,
10.3329315992068));
#66059=CARTESIAN_POINT('Ctrl Pts',(-0.222499947271515,2.33338787014627,
10.3336592954323));
#66060=CARTESIAN_POINT('Ctrl Pts',(-0.241942571303382,2.31357714498271,
10.3355336234373));
#66061=CARTESIAN_POINT('Ctrl Pts',(-0.25289427796135,2.30048952352188,10.3366724815783));
#66062=CARTESIAN_POINT('Ctrl Pts',(-0.263197843587707,2.28598021525638,
10.3377895501186));
#66063=CARTESIAN_POINT('Ctrl Pts',(-0.263632706327043,2.28536326906358,
10.3378367887308));
#66064=CARTESIAN_POINT('Ctrl Pts',(-0.264245010490872,2.28448807067453,
10.337903427729));
#66065=CARTESIAN_POINT('Ctrl Pts',(-0.264424244695574,2.28423108480846,
10.3379229496669));
#66066=CARTESIAN_POINT('Ctrl Pts',(-0.264731105215501,2.2837897381052,10.3379563982328));
#66067=CARTESIAN_POINT('Ctrl Pts',(-0.264858914170717,2.28360550505589,
10.3379703374296));
#66068=CARTESIAN_POINT('Ctrl Pts',(-0.265103093514358,2.28325274180215,
10.3379969828344));
#66069=CARTESIAN_POINT('Ctrl Pts',(-0.26521949537384,2.28308423428333,10.3380096912342));
#66070=CARTESIAN_POINT('Ctrl Pts',(-0.265493044182715,2.28268742685574,
10.3380395717475));
#66071=CARTESIAN_POINT('Ctrl Pts',(-0.265650057713977,2.28245903452138,
10.3380567346961));
#66072=CARTESIAN_POINT('Ctrl Pts',(-0.266112174803341,2.28178497669168,
10.3381072842279));
#66073=CARTESIAN_POINT('Ctrl Pts',(-0.2664164548113,2.28133874364045,10.3381406150405));
#66074=CARTESIAN_POINT('Ctrl Pts',(-0.26904252835157,2.27746667459992,10.33842869963));
#66075=CARTESIAN_POINT('Ctrl Pts',(-0.27129938664848,2.27399698097526,10.338679170051));
#66076=CARTESIAN_POINT('Ctrl Pts',(-0.281104644147349,2.25826752817198,
10.3397852614992));
#66077=CARTESIAN_POINT('Ctrl Pts',(-0.28789405549644,2.24555251049751,10.3406013622875));
#66078=CARTESIAN_POINT('Ctrl Pts',(-0.306530683079391,2.20420343675961,
10.3431464018821));
#66079=CARTESIAN_POINT('Ctrl Pts',(-0.315116785478717,2.17430091953921,
10.3448499312024));
#66080=CARTESIAN_POINT('Ctrl Pts',(-0.319580938659845,2.14163265865075,
10.3468437847235));
#66081=CARTESIAN_POINT('Ctrl Pts',(-0.319835563553847,2.13962911327923,
10.3469664948881));
#66082=CARTESIAN_POINT('Ctrl Pts',(-0.320148235054558,2.13696913730879,
10.3471300167791));
#66083=CARTESIAN_POINT('Ctrl Pts',(-0.320223128285117,2.1363147025741,10.3471702967699));
#66084=CARTESIAN_POINT('Ctrl Pts',(-0.320342831839338,2.13523953372498,
10.3472365541192));
#66085=CARTESIAN_POINT('Ctrl Pts',(-0.320388821146545,2.13481893062148,
10.3472624942729));
#66086=CARTESIAN_POINT('Ctrl Pts',(-0.320476358109924,2.13400348721692,
10.3473128258209));
#66087=CARTESIAN_POINT('Ctrl Pts',(-0.320518004716193,2.13360865812287,
10.3473372140497));
#66088=CARTESIAN_POINT('Ctrl Pts',(-0.320612516783115,2.13269648523803,
10.3473936006653));
#66089=CARTESIAN_POINT('Ctrl Pts',(-0.320664859722767,2.13217908946577,
10.3474256154448));
#66090=CARTESIAN_POINT('Ctrl Pts',(-0.320828646004199,2.1305200160197,10.3475283761459));
#66091=CARTESIAN_POINT('Ctrl Pts',(-0.320935245268407,2.1293778788327,10.3475992742476));
#66092=CARTESIAN_POINT('Ctrl Pts',(-0.32186721319046,2.11878135662402,10.3482585339651));
#66093=CARTESIAN_POINT('Ctrl Pts',(-0.322280608452412,2.10929629717948,
10.3488597856719));
#66094=CARTESIAN_POINT('Ctrl Pts',(-0.322270166261914,2.09180868584661,
10.3499903677247));
#66095=CARTESIAN_POINT('Ctrl Pts',(-0.321967595462726,2.08381328509359,
10.3505157288825));
#66096=CARTESIAN_POINT('Ctrl Pts',(-0.318973647345409,2.04399231676612,
10.3531699568388));
#66097=CARTESIAN_POINT('Ctrl Pts',(-0.311859686864174,2.01268146281999,
10.3553986265746));
#66098=CARTESIAN_POINT('Ctrl Pts',(-0.299701487269705,1.98149873776168,
10.3575161254572));
#66099=CARTESIAN_POINT('Ctrl Pts',(-0.29913380087351,1.98007293874681,10.3576126631307));
#66100=CARTESIAN_POINT('Ctrl Pts',(-0.298395816820164,1.97825726730662,
10.357735185896));
#66101=CARTESIAN_POINT('Ctrl Pts',(-0.29823491475411,1.97786363323736,10.3577617237329));
#66102=CARTESIAN_POINT('Ctrl Pts',(-0.297977808701813,1.97723818126699,
10.3578038492537));
#66103=CARTESIAN_POINT('Ctrl Pts',(-0.297882112935714,1.9770061570185,10.3578194676126));
#66104=CARTESIAN_POINT('Ctrl Pts',(-0.297702659138811,1.97657249074447,
10.3578486420955));
#66105=CARTESIAN_POINT('Ctrl Pts',(-0.297618967871208,1.97637082357697,
10.3578622020975));
#66106=CARTESIAN_POINT('Ctrl Pts',(-0.297430242059429,1.9759173615482,10.3578926771343));
#66107=CARTESIAN_POINT('Ctrl Pts',(-0.297325092936461,1.97566561550265,
10.3579095850496));
#66108=CARTESIAN_POINT('Ctrl Pts',(-0.297011599905573,1.97491772824144,
10.3579597840054));
#66109=CARTESIAN_POINT('Ctrl Pts',(-0.296802331604503,1.97442197186298,
10.3579930189716));
#66110=CARTESIAN_POINT('Ctrl Pts',(-0.295086771549548,1.97038605598993,
10.3582632685398));
#66111=CARTESIAN_POINT('Ctrl Pts',(-0.293518358746154,1.96687241643497,
10.3584965757081));
#66112=CARTESIAN_POINT('Ctrl Pts',(-0.288118582297884,1.95533521092282,
10.359258787464));
#66113=CARTESIAN_POINT('Ctrl Pts',(-0.284017927955936,1.94744161309117,
10.3597740438604));
#66114=CARTESIAN_POINT('Ctrl Pts',(-0.267022939846461,1.91779388855637,
10.3617225464507));
#66115=CARTESIAN_POINT('Ctrl Pts',(-0.251913169269096,1.8974163128423,10.3630973811836));
#66116=CARTESIAN_POINT('Ctrl Pts',(-0.230792491949408,1.87499676659573,
10.3648696769891));
#66117=CARTESIAN_POINT('Ctrl Pts',(-0.226906024345914,1.87107800239181,
10.3651903363216));
#66118=CARTESIAN_POINT('Ctrl Pts',(-0.222333881607314,1.86669873196306,
10.3655627832236));
#66119=CARTESIAN_POINT('Ctrl Pts',(-0.221744638254826,1.8661386052228,10.3656106942259));
#66120=CARTESIAN_POINT('Ctrl Pts',(-0.216380868404734,1.86107837591119,
10.3660460453336));
#66121=CARTESIAN_POINT('Ctrl Pts',(-0.211472359255203,1.85672309064134,
10.3664389571224));
#66122=CARTESIAN_POINT('Ctrl Pts',(-0.205639159019191,1.85185732953281,
10.3669012678651));
#66123=CARTESIAN_POINT('Ctrl Pts',(-0.204840522495499,1.8511976508688,10.3669644657762));
#66124=CARTESIAN_POINT('Ctrl Pts',(-0.203648428635293,1.8502226043387,10.3670586595194));
#66125=CARTESIAN_POINT('Ctrl Pts',(-0.203257383641885,1.8499042866032,10.3670895359617));
#66126=CARTESIAN_POINT('Ctrl Pts',(-0.202559876788322,1.8493392197724,10.3671445717128));
#66127=CARTESIAN_POINT('Ctrl Pts',(-0.202253706391801,1.84909211116944,
10.3671687164767));
#66128=CARTESIAN_POINT('Ctrl Pts',(-0.20160853659243,1.84857334605037,10.3672195676775));
#66129=CARTESIAN_POINT('Ctrl Pts',(-0.201269439127227,1.84830181324905,
10.3672462790114));
#66130=CARTESIAN_POINT('Ctrl Pts',(-0.200375118144687,1.84758864730866,
10.3673166855608));
#66131=CARTESIAN_POINT('Ctrl Pts',(-0.199818985819162,1.84714816229201,
10.3673604265592));
#66132=CARTESIAN_POINT('Ctrl Pts',(-0.197321776417721,1.84518362947927,
10.3675566579049));
#66133=CARTESIAN_POINT('Ctrl Pts',(-0.19536472741941,1.84368010442129,10.3677099604148));
#66134=CARTESIAN_POINT('Ctrl Pts',(-0.180888730686399,1.83282085663207,
10.3688406686116));
#66135=CARTESIAN_POINT('Ctrl Pts',(-0.167723113800082,1.82436572137034,
10.3698529667051));
#66136=CARTESIAN_POINT('Ctrl Pts',(-0.12580003502154,1.80156084868131,10.3730238363504));
#66137=CARTESIAN_POINT('Ctrl Pts',(-0.0954707291611789,1.7905216495933,
10.3752647326888));
#66138=CARTESIAN_POINT('Ctrl Pts',(-0.0625320003943831,1.7838462348125,
10.3773905632051));
#66139=CARTESIAN_POINT('Ctrl Pts',(-0.0610504204559197,1.78355679705627,
10.3774855106009));
#66140=CARTESIAN_POINT('Ctrl Pts',(-0.0591515178741482,1.78319966518136,
10.3776062952398));
#66141=CARTESIAN_POINT('Ctrl Pts',(-0.058736052186312,1.78312237316838,
10.3776326665586));
#66142=CARTESIAN_POINT('Ctrl Pts',(-0.0580742042754473,1.78300059131918,
10.3776745871755));
#66143=CARTESIAN_POINT('Ctrl Pts',(-0.05782792197665,1.78295557133565,10.3776901666471));
#66144=CARTESIAN_POINT('Ctrl Pts',(-0.0573687337082872,1.78287218536047,
10.3777191771398));
#66145=CARTESIAN_POINT('Ctrl Pts',(-0.0571558431921249,1.78283374704308,
10.3777326121902));
#66146=CARTESIAN_POINT('Ctrl Pts',(-0.0566745345987861,1.78274734500622,
10.3777629529841));
#66147=CARTESIAN_POINT('Ctrl Pts',(-0.0564060948498825,1.78269950766238,
10.3777798514007));
#66148=CARTESIAN_POINT('Ctrl Pts',(-0.0556084473500054,1.7825584070011,
10.3778299947104));
#66149=CARTESIAN_POINT('Ctrl Pts',(-0.0550790633735103,1.78246612594857,
10.3778631837158));
#66150=CARTESIAN_POINT('Ctrl Pts',(-0.0507801159260038,1.78172781716147,
10.3781319867265));
#66151=CARTESIAN_POINT('Ctrl Pts',(-0.046999356795059,1.78114757935618,
10.3783639376251));
#66152=CARTESIAN_POINT('Ctrl Pts',(-0.0346098940189089,1.77947132978813,
10.3791121556485));
#66153=CARTESIAN_POINT('Ctrl Pts',(-0.0259666172483175,1.77865558582802,
10.379615516642));
#66154=CARTESIAN_POINT('Ctrl Pts',(0.0112969168478374,1.77665232392053,
10.3817452230985));
#66155=CARTESIAN_POINT('Ctrl Pts',(0.039970835702141,1.7789333776358,10.383294139838));
#66156=CARTESIAN_POINT('Ctrl Pts',(0.0773610490664642,1.78700031958462,
10.3855215895428));
#66157=CARTESIAN_POINT('Ctrl Pts',(0.086658937365287,1.78944608733933,10.3860920692034));
#66158=CARTESIAN_POINT('Ctrl Pts',(0.096917573850852,1.79264117094517,10.386745452651));
#66159=CARTESIAN_POINT('Ctrl Pts',(0.0980002965777421,1.79298467833339,
10.3868147128344));
#66160=CARTESIAN_POINT('Ctrl Pts',(0.0995368021366322,1.79348111001578,
10.3869134361264));
#66161=CARTESIAN_POINT('Ctrl Pts',(0.0999921037531905,1.79362933547767,
10.3869427445868));
#66162=CARTESIAN_POINT('Ctrl Pts',(0.100826915903225,1.79390317142987,10.3869965834661));
#66163=CARTESIAN_POINT('Ctrl Pts',(0.101206526870368,1.79402847461275,10.3870211037148));
#66164=CARTESIAN_POINT('Ctrl Pts',(0.101975550583113,1.79428390411406,10.3870708554381));
#66165=CARTESIAN_POINT('Ctrl Pts',(0.102364949679723,1.79441406891832,10.3870960881458));
#66166=CARTESIAN_POINT('Ctrl Pts',(0.103323438938877,1.79473650165447,10.3871582981351));
#66167=CARTESIAN_POINT('Ctrl Pts',(0.103892240639572,1.79492961667281,10.387195303381));
#66168=CARTESIAN_POINT('Ctrl Pts',(0.105968210452394,1.79564091262227,10.3873306850688));
#66169=CARTESIAN_POINT('Ctrl Pts',(0.107472049770653,1.79616867497327,10.3874293786102));
#66170=CARTESIAN_POINT('Ctrl Pts',(0.116150065628597,1.79928665512679,10.3880025688954));
#66171=CARTESIAN_POINT('Ctrl Pts',(0.123233874051823,1.80211957113634,10.3884851218318));
#66172=CARTESIAN_POINT('Ctrl Pts',(0.136852446194015,1.80813477037234,10.3894427799752));
#66173=CARTESIAN_POINT('Ctrl Pts',(0.143393343232581,1.81129211774023,10.3899168529905));
#66174=CARTESIAN_POINT('Ctrl Pts',(0.167065995390002,1.82372209393221,10.3916835908986));
#66175=CARTESIAN_POINT('Ctrl Pts',(0.183453123415775,1.83432091460619,10.3930109872827));
#66176=CARTESIAN_POINT('Ctrl Pts',(0.210712546858192,1.85568226252787,10.3953441616867));
#66177=CARTESIAN_POINT('Ctrl Pts',(0.221970678282373,1.86586312692097,10.3963521235913));
#66178=CARTESIAN_POINT('Ctrl Pts',(0.233109304943099,1.8774644390391,10.3973636821887));
#66179=CARTESIAN_POINT('Ctrl Pts',(0.233744354697579,1.87813156907901,10.3974214049744));
#66180=CARTESIAN_POINT('Ctrl Pts',(0.234593198227199,1.87903098269818,10.3974986172242));
#66181=CARTESIAN_POINT('Ctrl Pts',(0.234809515413488,1.87926086270181,10.3975182987843));
#66182=CARTESIAN_POINT('Ctrl Pts',(0.235172740797678,1.87964799996004,10.3975513545586));
#66183=CARTESIAN_POINT('Ctrl Pts',(0.235319829251599,1.87980508657664,10.3975647426871));
#66184=CARTESIAN_POINT('Ctrl Pts',(0.235613315132623,1.88011915174055,10.3975914601518));
#66185=CARTESIAN_POINT('Ctrl Pts',(0.235759711938809,1.88027612800174,10.3976047893837));
#66186=CARTESIAN_POINT('Ctrl Pts',(0.236091131045357,1.88063220988054,10.3976349693831));
#66187=CARTESIAN_POINT('Ctrl Pts',(0.236276058013356,1.88083140299955,10.3976518127614));
#66188=CARTESIAN_POINT('Ctrl Pts',(0.236662503945287,1.88124871877441,10.3976870184341));
#66189=CARTESIAN_POINT('Ctrl Pts',(0.236863974012249,1.88146688665493,10.3977053769873));
#66190=CARTESIAN_POINT('Ctrl Pts',(0.237391211102245,1.8820394067626,10.397753432931));
#66191=CARTESIAN_POINT('Ctrl Pts',(0.237716487809621,1.88239421252312,10.3977830934207));
#66192=CARTESIAN_POINT('Ctrl Pts',(0.238682143848504,1.88345228126765,10.3978711894635));
#66193=CARTESIAN_POINT('Ctrl Pts',(0.239320212813764,1.88415765922584,10.3979294556308));
#66194=CARTESIAN_POINT('Ctrl Pts',(0.246510880413049,1.89217794740038,10.3985868551063));
#66195=CARTESIAN_POINT('Ctrl Pts',(0.252729669881703,1.89978667654771,10.3991627665697));
#66196=CARTESIAN_POINT('Ctrl Pts',(0.276855734981084,1.93222440850118,10.4014841485089));
#66197=CARTESIAN_POINT('Ctrl Pts',(0.291529037378584,1.95925639656827,10.4031295816653));
#66198=CARTESIAN_POINT('Ctrl Pts',(0.305353509151775,1.99653867211054,10.405449618392));
#66199=CARTESIAN_POINT('Ctrl Pts',(0.308169308093801,2.00525473494782,10.4059938592449));
#66200=CARTESIAN_POINT('Ctrl Pts',(0.31091311697873,2.01517370029135,10.4066197466409));
#66201=CARTESIAN_POINT('Ctrl Pts',(0.311210339524429,2.01627072224747,10.4066890545838));
#66202=CARTESIAN_POINT('Ctrl Pts',(0.311634585424211,2.01787004686112,10.406790229551));
#66203=CARTESIAN_POINT('Ctrl Pts',(0.311766212643437,2.01837112836667,10.4068219473626));
#66204=CARTESIAN_POINT('Ctrl Pts',(0.311996492487229,2.01925644502881,10.4068780208743));
#66205=CARTESIAN_POINT('Ctrl Pts',(0.312095645243799,2.01964054995619,10.4069023603386));
#66206=CARTESIAN_POINT('Ctrl Pts',(0.312299283119881,2.02043547850106,10.4069527561596));
#66207=CARTESIAN_POINT('Ctrl Pts',(0.312403667329038,2.02084632696341,10.4069788157244));
#66208=CARTESIAN_POINT('Ctrl Pts',(0.312669059344056,2.02189959296783,10.407045657224));
#66209=CARTESIAN_POINT('Ctrl Pts',(0.31282889742508,2.02254230073753,10.4070864768347));
#66210=CARTESIAN_POINT('Ctrl Pts',(0.313475068905385,2.02517517726691,10.4072538327746));
#66211=CARTESIAN_POINT('Ctrl Pts',(0.313944392191883,2.0271694348365,10.4073809157409));
#66212=CARTESIAN_POINT('Ctrl Pts',(0.316924870372072,2.04039857370554,10.408226190087));
#66213=CARTESIAN_POINT('Ctrl Pts',(0.318851226726684,2.05175536018906,10.408963017709));
#66214=CARTESIAN_POINT('Ctrl Pts',(0.323918924248395,2.09583290568706,10.4118671565514));
#66215=CARTESIAN_POINT('Ctrl Pts',(0.322657621397719,2.12885198904343,10.4141594439876));
#66216=CARTESIAN_POINT('Ctrl Pts',(0.3154722993399,2.16605938354124,10.4166179188866));
#66217=CARTESIAN_POINT('Ctrl Pts',(0.314399777879935,2.17098873523387,10.4169404385053));
#66218=CARTESIAN_POINT('Ctrl Pts',(0.313062595447996,2.17650744409736,10.41729638456));
#66219=CARTESIAN_POINT('Ctrl Pts',(0.312911460864029,2.17712324777334,10.4173360301406));
#66220=CARTESIAN_POINT('Ctrl Pts',(0.312688888666618,2.17801870179066,10.4173935699488));
#66221=CARTESIAN_POINT('Ctrl Pts',(0.312618892470348,2.17829870367279,10.4174115465898));
#66222=CARTESIAN_POINT('Ctrl Pts',(0.312494675248389,2.17879278097519,10.4174432392002));
#66223=CARTESIAN_POINT('Ctrl Pts',(0.312440610255716,2.1790068949942,10.4174569642303));
#66224=CARTESIAN_POINT('Ctrl Pts',(0.312328686608581,2.17944823550562,10.4174852354168));
#66225=CARTESIAN_POINT('Ctrl Pts',(0.312270800180339,2.17967545393137,10.4174997798989));
#66226=CARTESIAN_POINT('Ctrl Pts',(0.312120730378924,2.18026183894202,10.417537288182));
#66227=CARTESIAN_POINT('Ctrl Pts',(0.31202817468496,2.18062091123695,10.4175602303556));
#66228=CARTESIAN_POINT('Ctrl Pts',(0.311824977726453,2.18140362770902,10.4176101852892));
#66229=CARTESIAN_POINT('Ctrl Pts',(0.311714092212591,2.18182720855345,10.4176371840414));
#66230=CARTESIAN_POINT('Ctrl Pts',(0.311389253565988,2.18305784427461,10.4177155249283));
#66231=CARTESIAN_POINT('Ctrl Pts',(0.311173025036667,2.18386430263709,10.4177667392737));
#66232=CARTESIAN_POINT('Ctrl Pts',(0.30889618123039,2.19222610225664,10.4182965572304));
#66233=CARTESIAN_POINT('Ctrl Pts',(0.306563766631296,2.19970548765169,10.4187602954756));
#66234=CARTESIAN_POINT('Ctrl Pts',(0.298665152302906,2.22212401915989,10.4201398569616));
#66235=CARTESIAN_POINT('Ctrl Pts',(0.292261379047564,2.23674248361303,10.4210258221697));
#66236=CARTESIAN_POINT('Ctrl Pts',(0.277245670525367,2.26509599250208,10.4228195801948));
#66237=CARTESIAN_POINT('Ctrl Pts',(0.26862836638918,2.27877526057871,10.4237253341536));
#66238=CARTESIAN_POINT('Ctrl Pts',(0.25318096909016,2.2996421329099,10.4252358722444));
#66239=CARTESIAN_POINT('Ctrl Pts',(0.246981805578643,2.30726201430168,10.4258183828522));
#66240=CARTESIAN_POINT('Ctrl Pts',(0.239751532301661,2.31536355997245,10.4264786716171));
#66241=CARTESIAN_POINT('Ctrl Pts',(0.239054340033127,2.31613718485374,10.4265421541153));
#66242=CARTESIAN_POINT('Ctrl Pts',(0.238005997112949,2.3172891792323,10.4266373383659));
#66243=CARTESIAN_POINT('Ctrl Pts',(0.237657662538449,2.31767011164844,10.426668920926));
#66244=CARTESIAN_POINT('Ctrl Pts',(0.237056175502255,2.3183247220695,10.4267233805703));
#66245=CARTESIAN_POINT('Ctrl Pts',(0.236803459823008,2.31859880151647,10.4267462390423));
#66246=CARTESIAN_POINT('Ctrl Pts',(0.236280913422218,2.31916355280118,10.4267934573859));
#66247=CARTESIAN_POINT('Ctrl Pts',(0.236011020653077,2.3194541661764,10.4268178198894));
#66248=CARTESIAN_POINT('Ctrl Pts',(0.235381564498682,2.32012944367354,10.4268745803274));
#66249=CARTESIAN_POINT('Ctrl Pts',(0.235021594251671,2.32051372544135,10.4269069956926));
#66250=CARTESIAN_POINT('Ctrl Pts',(0.23387141535911,2.32173556919203,10.4270104293539));
#66251=CARTESIAN_POINT('Ctrl Pts',(0.23307766549747,2.32256977188756,10.4270816003023));
#66252=CARTESIAN_POINT('Ctrl Pts',(0.215871308497118,2.34046005370663,10.4286199904444));
#66253=CARTESIAN_POINT('Ctrl Pts',(0.197637211132556,2.355657101423,10.4301727128665));
#66254=CARTESIAN_POINT('Ctrl Pts',(0.158220874573533,2.38175310302006,10.4333572861666));
#66255=CARTESIAN_POINT('Ctrl Pts',(0.137160007867019,2.39258487758418,10.4349779958288));
#66256=CARTESIAN_POINT('Ctrl Pts',(0.111902726607968,2.40224278500013,10.4367141485652));
#66257=CARTESIAN_POINT('Ctrl Pts',(0.108682093079082,2.40341576472092,10.4369317644403));
#66258=CARTESIAN_POINT('Ctrl Pts',(0.104907386525659,2.40472272215475,10.437181952391));
#66259=CARTESIAN_POINT('Ctrl Pts',(0.104371074400361,2.40490683164731,10.4372173855491));
#66260=CARTESIAN_POINT('Ctrl Pts',(0.103570431817143,2.40517932261941,10.4372701101793));
#66261=CARTESIAN_POINT('Ctrl Pts',(0.103306471742261,2.40526877697991,10.4372874648222));
#66262=CARTESIAN_POINT('Ctrl Pts',(0.102835000865762,2.40542787386226,10.4373184125258));
#66263=CARTESIAN_POINT('Ctrl Pts',(0.102627535356699,2.40549764732767,10.4373320133643));
#66264=CARTESIAN_POINT('Ctrl Pts',(0.102190452345232,2.40564414878222,10.4373606306271));
#66265=CARTESIAN_POINT('Ctrl Pts',(0.101960820147184,2.40572082917454,10.4373756441786));
#66266=CARTESIAN_POINT('Ctrl Pts',(0.101346897423774,2.40592506591728,10.4374157268217));
#66267=CARTESIAN_POINT('Ctrl Pts',(0.100962450961458,2.40605215744057,10.437440768345));
#66268=CARTESIAN_POINT('Ctrl Pts',(0.100115069881432,2.40633051691694,10.4374958366018));
#66269=CARTESIAN_POINT('Ctrl Pts',(0.0996520287937277,2.40648146106491,
10.4375258444693));
#66270=CARTESIAN_POINT('Ctrl Pts',(0.0982690068269478,2.40692883890308,
10.4376152285617));
#66271=CARTESIAN_POINT('Ctrl Pts',(0.0973480228500361,2.40722218727596,
10.4376744294435));
#66272=CARTESIAN_POINT('Ctrl Pts',(0.0940811866091533,2.40824656245011,
10.4378833292304));
#66273=CARTESIAN_POINT('Ctrl Pts',(0.0917282437612715,2.4089549207262,10.4380317992542));
#66274=CARTESIAN_POINT('Ctrl Pts',(0.084505548079991,2.4110395378678,10.4384821330487));
#66275=CARTESIAN_POINT('Ctrl Pts',(0.0796111009683528,2.41232812863234,
10.4387798217001));
#66276=CARTESIAN_POINT('Ctrl Pts',(0.0641925383506842,2.41600142768055,
10.4397000778383));
#66277=CARTESIAN_POINT('Ctrl Pts',(0.0535773906457115,2.41797338797259,
10.4403085006574));
#66278=CARTESIAN_POINT('Ctrl Pts',(0.0191642312316019,2.42259357846918,
10.4422542619353));
#66279=CARTESIAN_POINT('Ctrl Pts',(-0.00483297969329889,2.42312602856722,
10.443576694952));
#66280=CARTESIAN_POINT('Ctrl Pts',(-0.030440004569496,2.42083913226407,
10.4450886510365));
#66281=CARTESIAN_POINT('Ctrl Pts',(-0.0322112026507477,2.42066615181653,
10.4451937127245));
#66282=CARTESIAN_POINT('Ctrl Pts',(-0.0396785979762269,2.41987437185192,
10.445638826916));
#66283=CARTESIAN_POINT('Ctrl Pts',(-0.0453589210570994,2.41911842144803,
10.4459827853222));
#66284=CARTESIAN_POINT('Ctrl Pts',(-0.0519855170223322,2.4180560424297,
10.4463913642048));
#66285=CARTESIAN_POINT('Ctrl Pts',(-0.0529544899626497,2.41789614981222,
10.4464512921979));
#66286=CARTESIAN_POINT('Ctrl Pts',(-0.0544158016741092,2.41764814858091,
10.4465419522384));
#66287=CARTESIAN_POINT('Ctrl Pts',(-0.054908697067118,2.41756331770318,
10.4465725801213));
#66288=CARTESIAN_POINT('Ctrl Pts',(-0.0557885055890453,2.41740978669611,
10.4466273377849));
#66289=CARTESIAN_POINT('Ctrl Pts',(-0.0561754951234036,2.41734152547657,
10.4466514535628));
#66290=CARTESIAN_POINT('Ctrl Pts',(-0.0569922359181447,2.41719591948637,
10.4467024141892));
#66291=CARTESIAN_POINT('Ctrl Pts',(-0.0574219564553425,2.41711840881224,
10.4467292642746));
#66292=CARTESIAN_POINT('Ctrl Pts',(-0.0585592784539783,2.41691087727973,
10.4468004275212));
#66293=CARTESIAN_POINT('Ctrl Pts',(-0.0592666013618192,2.41677936040857,
10.4468447882625));
#66294=CARTESIAN_POINT('Ctrl Pts',(-0.0624949398894309,2.41616790473061,
10.4470477332154));
#66295=CARTESIAN_POINT('Ctrl Pts',(-0.0650105511544492,2.41566024317196,
10.4472071994173));
#66296=CARTESIAN_POINT('Ctrl Pts',(-0.075929102684722,2.41332077871046,
10.4479052882282));
#66297=CARTESIAN_POINT('Ctrl Pts',(-0.0842622238161775,2.41118321637384,
10.4484536176869));
#66298=CARTESIAN_POINT('Ctrl Pts',(-0.108203743666885,2.40400969737504,
10.4500756115429));
#66299=CARTESIAN_POINT('Ctrl Pts',(-0.123524558398253,2.39811326873441,
10.4511738834494));
#66300=CARTESIAN_POINT('Ctrl Pts',(-0.144863899821745,2.38797218474657,
10.4527712166224));
#66301=CARTESIAN_POINT('Ctrl Pts',(-0.151292590798713,2.38464729286863,
10.4532615940045));
#66302=CARTESIAN_POINT('Ctrl Pts',(-0.166601572640246,2.37606429770608,
10.454445646444));
#66303=CARTESIAN_POINT('Ctrl Pts',(-0.175352472452942,2.37059031752537,
10.4551364626226));
#66304=CARTESIAN_POINT('Ctrl Pts',(-0.184092010063403,2.36452109963622,
10.4558310234848));
#66305=CARTESIAN_POINT('Ctrl Pts',(-0.184357501475641,2.36433613444458,
10.4558521273706));
#66306=CARTESIAN_POINT('Ctrl Pts',(-0.189391370235722,2.36081781602418,
10.4562523457996));
#66307=CARTESIAN_POINT('Ctrl Pts',(-0.194069280840105,2.35735607447334,
10.4566255851434));
#66308=CARTESIAN_POINT('Ctrl Pts',(-0.199169778810791,2.35336339216137,
10.4570317344039));
#66309=CARTESIAN_POINT('Ctrl Pts',(-0.199687081178477,2.35295588332282,
10.4570729172066));
#66310=CARTESIAN_POINT('Ctrl Pts',(-0.200412175015025,2.35238107474349,
10.4571306244766));
#66311=CARTESIAN_POINT('Ctrl Pts',(-0.200621008910719,2.35221510178386,
10.4571472426149));
#66312=CARTESIAN_POINT('Ctrl Pts',(-0.201003625326346,2.35191023742833,
10.4571776854075));
#66313=CARTESIAN_POINT('Ctrl Pts',(-0.201177470485556,2.35177142507748,
10.4571915157491));
#66314=CARTESIAN_POINT('Ctrl Pts',(-0.201510824402877,2.35150468202842,
10.4572180325739));
#66315=CARTESIAN_POINT('Ctrl Pts',(-0.201670355025856,2.35137677963179,
10.4572307210795));
#66316=CARTESIAN_POINT('Ctrl Pts',(-0.202078550105742,2.35104887382148,
10.4572631840884));
#66317=CARTESIAN_POINT('Ctrl Pts',(-0.202327040168917,2.35084865213602,
10.4572829428178));
#66318=CARTESIAN_POINT('Ctrl Pts',(-0.203188037817808,2.3501527887829,10.457351395591));
#66319=CARTESIAN_POINT('Ctrl Pts',(-0.203799031112506,2.34965526510846,
10.4573999551223));
#66320=CARTESIAN_POINT('Ctrl Pts',(-0.205270308511925,2.34844822305168,
10.4575168630094));
#66321=CARTESIAN_POINT('Ctrl Pts',(-0.206128753494383,2.34773646513873,
10.4575850552738));
#66322=CARTESIAN_POINT('Ctrl Pts',(-0.209273320324868,2.34510156601223,
10.4578348501145));
#66323=CARTESIAN_POINT('Ctrl Pts',(-0.211536441011745,2.34315105550405,
10.4580146257314));
#66324=CARTESIAN_POINT('Ctrl Pts',(-0.219839210484209,2.33579148931068,
10.4586755949131));
#66325=CARTESIAN_POINT('Ctrl Pts',(-0.225701593183277,2.33018626187017,
10.4591451741325));
#66326=CARTESIAN_POINT('Ctrl Pts',(-0.25075357951981,2.30435477352191,10.4611980795352));
#66327=CARTESIAN_POINT('Ctrl Pts',(-0.267482002121666,2.28191125638656,
10.4627076759838));
#66328=CARTESIAN_POINT('Ctrl Pts',(-0.28205751679078,2.25591168619819,10.464438727284));
#66329=CARTESIAN_POINT('Ctrl Pts',(-0.28298567018958,2.25422064368605,10.4645511841005));
#66330=CARTESIAN_POINT('Ctrl Pts',(-0.284778784891755,2.2508829957844,10.4647729768903));
#66331=CARTESIAN_POINT('Ctrl Pts',(-0.285644783813262,2.2492370330387,10.4648822760457));
#66332=CARTESIAN_POINT('Ctrl Pts',(-0.289545410307402,2.24166495139706,
10.465384918935));
#66333=CARTESIAN_POINT('Ctrl Pts',(-0.29241001677758,2.23565351250714,10.4657835195678));
#66334=CARTESIAN_POINT('Ctrl Pts',(-0.295504479684383,2.22860544448502,
10.4662519794118));
#66335=CARTESIAN_POINT('Ctrl Pts',(-0.295918075819724,2.22765089199882,
10.4663154472849));
#66336=CARTESIAN_POINT('Ctrl Pts',(-0.296525610459625,2.22622992158104,
10.4664099660043));
#66337=CARTESIAN_POINT('Ctrl Pts',(-0.296723088645769,2.22576501668084,
10.4664408962446));
#66338=CARTESIAN_POINT('Ctrl Pts',(-0.297072487496587,2.22493705490202,
10.4664959924483));
#66339=CARTESIAN_POINT('Ctrl Pts',(-0.297224837952698,2.22457417957511,
10.4665201437492));
#66340=CARTESIAN_POINT('Ctrl Pts',(-0.297543775112242,2.2238106046695,10.4665709725445));
#66341=CARTESIAN_POINT('Ctrl Pts',(-0.297710217843865,2.22340984614323,
10.4665976548638));
#66342=CARTESIAN_POINT('Ctrl Pts',(-0.298145839210858,2.22235495305218,
10.466667903162));
#66343=CARTESIAN_POINT('Ctrl Pts',(-0.29841367343731,2.22170026897278,10.4667115145513));
#66344=CARTESIAN_POINT('Ctrl Pts',(-0.29959871652637,2.21877616026796,10.4669063698174));
#66345=CARTESIAN_POINT('Ctrl Pts',(-0.300492188249824,2.21649725945899,
10.4670584119241));
#66346=CARTESIAN_POINT('Ctrl Pts',(-0.306821695442285,2.1997957133266,10.4681742695162));
#66347=CARTESIAN_POINT('Ctrl Pts',(-0.311242013049874,2.18501189589775,
10.4691719910449));
#66348=CARTESIAN_POINT('Ctrl Pts',(-0.319710188476083,2.14693893366483,
10.4717616584561));
#66349=CARTESIAN_POINT('Ctrl Pts',(-0.322287609168167,2.12341734939115,
10.4733837697346));
#66350=CARTESIAN_POINT('Ctrl Pts',(-0.322274953623987,2.09982710796216,
10.4749491144816));
#66351=CARTESIAN_POINT('',(-0.322274999420556,2.10001932564221,10.7244193016094));
#66352=CARTESIAN_POINT('Ctrl Pts',(-0.322274953371521,2.09982663799766,
10.4749491456664));
#66353=CARTESIAN_POINT('Ctrl Pts',(-0.322269664666157,2.08999508753374,
10.4756015237701));
#66354=CARTESIAN_POINT('Ctrl Pts',(-0.321814482242808,2.08016755982393,
10.4762419206767));
#66355=CARTESIAN_POINT('Ctrl Pts',(-0.320868210385068,2.0699171372135,10.4768874415527));
#66356=CARTESIAN_POINT('Ctrl Pts',(-0.320824960434261,2.0694593412374,10.4769162240009));
#66357=CARTESIAN_POINT('Ctrl Pts',(-0.320753030884765,2.06871499184235,
10.4769629439478));
#66358=CARTESIAN_POINT('Ctrl Pts',(-0.320724946944098,2.06842838353156,
10.4769809142826));
#66359=CARTESIAN_POINT('Ctrl Pts',(-0.320674946744877,2.06792506275924,
10.4770124387095));
#66360=CARTESIAN_POINT('Ctrl Pts',(-0.320653194935537,2.06770833471107,
10.477026002008));
#66361=CARTESIAN_POINT('Ctrl Pts',(-0.320610240716335,2.06728467572564,
10.4770524937478));
#66362=CARTESIAN_POINT('Ctrl Pts',(-0.320589057628016,2.0670777427154,10.4770654232931));
#66363=CARTESIAN_POINT('Ctrl Pts',(-0.320546460293919,2.06666555828951,
10.4770911569344));
#66364=CARTESIAN_POINT('Ctrl Pts',(-0.320525049291612,2.06646030727147,
10.4771039611912));
#66365=CARTESIAN_POINT('Ctrl Pts',(-0.320473783551785,2.06597339415416,
10.4771343129506));
#66366=CARTESIAN_POINT('Ctrl Pts',(-0.320443754554873,2.06569175000694,
10.4771518505655));
#66367=CARTESIAN_POINT('Ctrl Pts',(-0.320336934899071,2.06470225630211,
10.477213400517));
#66368=CARTESIAN_POINT('Ctrl Pts',(-0.320258169087202,2.06399461531421,
10.4772573021753));
#66369=CARTESIAN_POINT('Ctrl Pts',(-0.319176293521734,2.05455943060468,
10.477841176338));
#66370=CARTESIAN_POINT('Ctrl Pts',(-0.317818968337538,2.04587526089332,
10.4783617059311));
#66371=CARTESIAN_POINT('Ctrl Pts',(-0.315809565456272,2.03575166984567,
10.4789599322486));
#66372=CARTESIAN_POINT('Ctrl Pts',(-0.315500116371917,2.03424890687167,
10.4790485086148));
#66373=CARTESIAN_POINT('Ctrl Pts',(-0.310390827631978,2.01030382358679,
10.480457083047));
#66374=CARTESIAN_POINT('Ctrl Pts',(-0.303217832213464,1.98843417167246,
10.4817088251937));
#66375=CARTESIAN_POINT('Ctrl Pts',(-0.287422327018391,1.95340910052672,
10.4838882489798));
#66376=CARTESIAN_POINT('Ctrl Pts',(-0.280056399379121,1.93978512656579,
10.4847846032852));
#66377=CARTESIAN_POINT('Ctrl Pts',(-0.270422667165388,1.924675231332,10.4858655124247));
#66378=CARTESIAN_POINT('Ctrl Pts',(-0.269080314765277,1.92262193732711,
10.4860143316882));
#66379=CARTESIAN_POINT('Ctrl Pts',(-0.267320574075358,1.91999614603866,
10.4862072296032));
#66380=CARTESIAN_POINT('Ctrl Pts',(-0.26692453357615,1.91940938527299,10.4862505029552));
#66381=CARTESIAN_POINT('Ctrl Pts',(-0.26628253854229,1.9184649518342,10.4863204285422));
#66382=CARTESIAN_POINT('Ctrl Pts',(-0.266037787509282,1.91810646064433,
10.4863470351407));
#66383=CARTESIAN_POINT('Ctrl Pts',(-0.265569765885311,1.9174239064406,10.486397815858));
#66384=CARTESIAN_POINT('Ctrl Pts',(-0.26534662436447,1.91709975552781,10.4864219850389));
#66385=CARTESIAN_POINT('Ctrl Pts',(-0.264835853514157,1.91636067628332,
10.4864772134339));
#66386=CARTESIAN_POINT('Ctrl Pts',(-0.264547842273797,1.9159460142639,10.4865082871779));
#66387=CARTESIAN_POINT('Ctrl Pts',(-0.263664077137738,1.91467998000386,
10.4866034305609));
#66388=CARTESIAN_POINT('Ctrl Pts',(-0.263065183361337,1.91383081713983,
10.4866676202762));
#66389=CARTESIAN_POINT('Ctrl Pts',(-0.258613769537593,1.90758358993761,
10.4871426560152));
#66390=CARTESIAN_POINT('Ctrl Pts',(-0.254599797432523,1.90230303676831,
10.4875597221389));
#66391=CARTESIAN_POINT('Ctrl Pts',(-0.246932825620288,1.89283785243854,
10.4883372930651));
#66392=CARTESIAN_POINT('Ctrl Pts',(-0.243328985047084,1.88861652141776,
10.4886957894891));
#66393=CARTESIAN_POINT('Ctrl Pts',(-0.224499516469823,1.86768063502768,
10.4905340921578));
#66394=CARTESIAN_POINT('Ctrl Pts',(-0.207655182980231,1.85250974497609,
10.4920742201139));
#66395=CARTESIAN_POINT('Ctrl Pts',(-0.184401597531442,1.83562364735243,
10.4940114888477));
#66396=CARTESIAN_POINT('Ctrl Pts',(-0.179335906894013,1.83216153611763,
10.4944230000212));
#66397=CARTESIAN_POINT('Ctrl Pts',(-0.168464327424338,1.82517823468396,
10.4952802265356));
#66398=CARTESIAN_POINT('Ctrl Pts',(-0.162639472269889,1.82169145236355,
10.4957247331461));
#66399=CARTESIAN_POINT('Ctrl Pts',(-0.154840600597502,1.81735157296715,
10.4962967116169));
#66400=CARTESIAN_POINT('Ctrl Pts',(-0.152962391732179,1.81633073453648,
10.496432742654));
#66401=CARTESIAN_POINT('Ctrl Pts',(-0.150303320436226,1.81491957462676,
10.4966227739306));
#66402=CARTESIAN_POINT('Ctrl Pts',(-0.149530863688142,1.8145136467174,10.496677677098));
#66403=CARTESIAN_POINT('Ctrl Pts',(-0.148181292869036,1.81381142425413,
10.496773063602));
#66404=CARTESIAN_POINT('Ctrl Pts',(-0.147604919549748,1.81351372775322,
10.4968136317398));
#66405=CARTESIAN_POINT('Ctrl Pts',(-0.146766192832983,1.81308372895409,
10.496872415544));
#66406=CARTESIAN_POINT('Ctrl Pts',(-0.146504555871096,1.81295004431243,
10.4968907176244));
#66407=CARTESIAN_POINT('Ctrl Pts',(-0.146057926309308,1.81272260653101,
10.4969218997645));
#66408=CARTESIAN_POINT('Ctrl Pts',(-0.145873025719352,1.81262867400431,
10.4969347912038));
#66409=CARTESIAN_POINT('Ctrl Pts',(-0.14550481741615,1.81244206510033,10.4969604276663));
#66410=CARTESIAN_POINT('Ctrl Pts',(-0.145321511995711,1.81234938559609,
10.4969731728897));
#66411=CARTESIAN_POINT('Ctrl Pts',(-0.144888553296427,1.81213100049349,
10.4970032357463));
#66412=CARTESIAN_POINT('Ctrl Pts',(-0.144638824354234,1.81200544407228,
10.4970205439356));
#66413=CARTESIAN_POINT('Ctrl Pts',(-0.143771658359252,1.81157087075749,
10.4970805356722));
#66414=CARTESIAN_POINT('Ctrl Pts',(-0.143153386215205,1.81126351048257,
10.4971231157937));
#66415=CARTESIAN_POINT('Ctrl Pts',(-0.135662536049415,1.80756957578739,
10.4976367360521));
#66416=CARTESIAN_POINT('Ctrl Pts',(-0.128671631440922,1.80442681077598,
10.4980930063276));
#66417=CARTESIAN_POINT('Ctrl Pts',(-0.106573022092281,1.7954252840235,10.4994846545273));
#66418=CARTESIAN_POINT('Ctrl Pts',(-0.0911307722786908,1.79045382964229,
10.5003863743916));
#66419=CARTESIAN_POINT('Ctrl Pts',(-0.0735248795059124,1.78621838016865,
10.501398571833));
#66420=CARTESIAN_POINT('Ctrl Pts',(-0.0716667096891907,1.78578877239762,
10.5015051947685));
#66421=CARTESIAN_POINT('Ctrl Pts',(-0.0676339574842302,1.78489403666191,
10.5017363156833));
#66422=CARTESIAN_POINT('Ctrl Pts',(-0.0654581575823177,1.7844348722277,
10.5018608370571));
#66423=CARTESIAN_POINT('Ctrl Pts',(-0.0413701404003216,1.77961136561737,
10.5032387443593));
#66424=CARTESIAN_POINT('Ctrl Pts',(-0.0190694523605319,1.77751512097902,
10.5045143456594));
#66425=CARTESIAN_POINT('Ctrl Pts',(0.00451678436843235,1.77775422956733,
10.505947698763));
#66426=CARTESIAN_POINT('Ctrl Pts',(0.00576653294046906,1.77777417091147,
10.5060238771631));
#66427=CARTESIAN_POINT('Ctrl Pts',(0.00756050901915792,1.77781323610676,
10.5061335697268));
#66428=CARTESIAN_POINT('Ctrl Pts',(0.00810486417989138,1.77782647021286,
10.50616689934));
#66429=CARTESIAN_POINT('Ctrl Pts',(0.00904865474546904,1.7778518086859,
10.5062247645166));
#66430=CARTESIAN_POINT('Ctrl Pts',(0.00944810719990214,1.77786327656155,
10.5062492800873));
#66431=CARTESIAN_POINT('Ctrl Pts',(0.0102155435385683,1.77788673754187,
10.5062964274895));
#66432=CARTESIAN_POINT('Ctrl Pts',(0.0105835304636266,1.77789861834759,
10.5063190557647));
#66433=CARTESIAN_POINT('Ctrl Pts',(0.0114495260047386,1.77792806346895,
10.5063723574571));
#66434=CARTESIAN_POINT('Ctrl Pts',(0.0119475147749535,1.77794615227753,
10.5064030472718));
#66435=CARTESIAN_POINT('Ctrl Pts',(0.0134158190744853,1.77800289685818,
10.5064936507183));
#66436=CARTESIAN_POINT('Ctrl Pts',(0.0143859976958136,1.77804478312911,
10.5065536654983));
#66437=CARTESIAN_POINT('Ctrl Pts',(0.0229042000524346,1.77845112538205,
10.5070819258858));
#66438=CARTESIAN_POINT('Ctrl Pts',(0.0304368681016007,1.77907654702705,
10.5075583165908));
#66439=CARTESIAN_POINT('Ctrl Pts',(0.0409692202001078,1.78032516045509,
10.5082382436887));
#66440=CARTESIAN_POINT('Ctrl Pts',(0.0439929903616167,1.78072723905905,
10.5084350461257));
#66441=CARTESIAN_POINT('Ctrl Pts',(0.0750860518564352,1.78531184831656,
10.5104751526767));
#66442=CARTESIAN_POINT('Ctrl Pts',(0.102490002526301,1.79314187201147,10.5124272195866));
#66443=CARTESIAN_POINT('Ctrl Pts',(0.136250253933023,1.80782143212454,10.5148851567934));
#66444=CARTESIAN_POINT('Ctrl Pts',(0.143857689417009,1.81149101253808,10.5154415694871));
#66445=CARTESIAN_POINT('Ctrl Pts',(0.15333709739228,1.81653189453997,10.5161307112324));
#66446=CARTESIAN_POINT('Ctrl Pts',(0.155349929378248,1.81762997260444,10.5162767887091));
#66447=CARTESIAN_POINT('Ctrl Pts',(0.158152677303352,1.81919802302192,10.5164796567165));
#66448=CARTESIAN_POINT('Ctrl Pts',(0.15895250940828,1.81965000550513,10.5165374881731));
#66449=CARTESIAN_POINT('Ctrl Pts',(0.160158014229074,1.82033804983997,10.5166245452301));
#66450=CARTESIAN_POINT('Ctrl Pts',(0.160565113825703,1.82057158319565,10.5166539260257));
#66451=CARTESIAN_POINT('Ctrl Pts',(0.161311633573284,1.82100199559477,10.5167077671956));
#66452=CARTESIAN_POINT('Ctrl Pts',(0.161651206251521,1.82119860633508,10.516732244468));
#66453=CARTESIAN_POINT('Ctrl Pts',(0.162197430194848,1.82151620046571,10.5167715945562));
#66454=CARTESIAN_POINT('Ctrl Pts',(0.162404305844222,1.82163679408186,10.5167864925645));
#66455=CARTESIAN_POINT('Ctrl Pts',(0.162800479435068,1.82186832675622,10.5168150121731));
#66456=CARTESIAN_POINT('Ctrl Pts',(0.162989796923876,1.82197922763819,10.5168286360262));
#66457=CARTESIAN_POINT('Ctrl Pts',(0.163423320083916,1.82223377752504,10.5168598231647));
#66458=CARTESIAN_POINT('Ctrl Pts',(0.163667449323333,1.82237755507033,10.516877377923));
#66459=CARTESIAN_POINT('Ctrl Pts',(0.164419600876964,1.82282186436041,10.5169314409022));
#66460=CARTESIAN_POINT('Ctrl Pts',(0.164926991014534,1.82312347214489,10.5169678793259));
#66461=CARTESIAN_POINT('Ctrl Pts',(0.168797030039666,1.82543835138596,10.5172455881328));
#66462=CARTESIAN_POINT('Ctrl Pts',(0.172123710437412,1.82751152702084,10.517483037393));
#66463=CARTESIAN_POINT('Ctrl Pts',(0.176237549213364,1.8301806706476,10.5177761492502));
#66464=CARTESIAN_POINT('Ctrl Pts',(0.17706072897645,1.83072014084796,10.5178347743073));
#66465=CARTESIAN_POINT('Ctrl Pts',(0.201711597453075,1.84703697863535,10.5195899606402));
#66466=CARTESIAN_POINT('Ctrl Pts',(0.223340684507864,1.86591190641704,10.5211285623242));
#66467=CARTESIAN_POINT('Ctrl Pts',(0.252408971761341,1.89902627697551,10.5236278863721));
#66468=CARTESIAN_POINT('Ctrl Pts',(0.261767007933318,1.91137691964034,10.5245246670195));
#66469=CARTESIAN_POINT('Ctrl Pts',(0.271538418164638,1.92640828229311,10.52560608421));
#66470=CARTESIAN_POINT('Ctrl Pts',(0.27285226477248,1.92848079381511,10.5257549472457));
#66471=CARTESIAN_POINT('Ctrl Pts',(0.274514504462495,1.93117031152111,10.525947894047));
#66472=CARTESIAN_POINT('Ctrl Pts',(0.274884732165576,1.93177378063503,10.5259911720064));
#66473=CARTESIAN_POINT('Ctrl Pts',(0.275478745136297,1.93274921513507,10.5260611032453));
#66474=CARTESIAN_POINT('Ctrl Pts',(0.275703774055899,1.93312042357371,10.5260877108749));
#66475=CARTESIAN_POINT('Ctrl Pts',(0.276131372795722,1.93382901743504,10.5261384923742));
#66476=CARTESIAN_POINT('Ctrl Pts',(0.276334076130049,1.9341663217081,10.5261626613036));
#66477=CARTESIAN_POINT('Ctrl Pts',(0.276795408427319,1.93493718661414,10.5262178874658));
#66478=CARTESIAN_POINT('Ctrl Pts',(0.27705363699152,1.93537098459127,10.5262489592243));
#66479=CARTESIAN_POINT('Ctrl Pts',(0.277840176126017,1.93669938279737,10.5263440906324));
#66480=CARTESIAN_POINT('Ctrl Pts',(0.278365176968788,1.93759592597739,10.5264082703141));
#66481=CARTESIAN_POINT('Ctrl Pts',(0.282207533088732,1.94423088193846,10.5268830769975));
#66482=CARTESIAN_POINT('Ctrl Pts',(0.285351273774903,1.95006751548306,10.5272999173633));
#66483=CARTESIAN_POINT('Ctrl Pts',(0.289290629753467,1.95795459399824,10.527862693549));
#66484=CARTESIAN_POINT('Ctrl Pts',(0.290248603942787,1.95992247370025,10.5280030644539));
#66485=CARTESIAN_POINT('Ctrl Pts',(0.301821281773637,1.98432366824271,10.5297430823078));
#66486=CARTESIAN_POINT('Ctrl Pts',(0.309828958062536,2.00789811863785,10.5314280909666));
#66487=CARTESIAN_POINT('Ctrl Pts',(0.318347059231642,2.04745229743454,10.5341599592961));
#66488=CARTESIAN_POINT('Ctrl Pts',(0.32052344195725,2.06297361398135,10.5352066821043));
#66489=CARTESIAN_POINT('Ctrl Pts',(0.32164225185983,2.07977991494844,10.5362745133951));
#66490=CARTESIAN_POINT('Ctrl Pts',(0.321714680829075,2.08096702174728,10.5363495845125));
#66491=CARTESIAN_POINT('Ctrl Pts',(0.32181192666296,2.08272050904744,10.5364599223271));
#66492=CARTESIAN_POINT('Ctrl Pts',(0.321841822342641,2.08328658165731,10.5364954576631));
#66493=CARTESIAN_POINT('Ctrl Pts',(0.321886872663395,2.08418458866005,10.5365516928382));
#66494=CARTESIAN_POINT('Ctrl Pts',(0.32190300761598,2.08451646942695,10.5365724461804));
#66495=CARTESIAN_POINT('Ctrl Pts',(0.32193259837074,2.08514516872753,10.5366117032035));
#66496=CARTESIAN_POINT('Ctrl Pts',(0.321946157007971,2.08544198174986,10.536630212584));
#66497=CARTESIAN_POINT('Ctrl Pts',(0.321968970378172,2.08595701444704,10.5366622878935));
#66498=CARTESIAN_POINT('Ctrl Pts',(0.321978413769105,2.08617522522909,10.5366758644792));
#66499=CARTESIAN_POINT('Ctrl Pts',(0.321996350456338,2.08659968184639,10.5367022473699));
#66500=CARTESIAN_POINT('Ctrl Pts',(0.322004867418532,2.08680592583026,10.5367150550038));
#66501=CARTESIAN_POINT('Ctrl Pts',(0.322024609421249,2.08729539862132,10.5367454231772));
#66502=CARTESIAN_POINT('Ctrl Pts',(0.322035658987624,2.08757863490053,10.5367629738036));
#66503=CARTESIAN_POINT('Ctrl Pts',(0.322073198118167,2.08857461665292,10.536824612895));
#66504=CARTESIAN_POINT('Ctrl Pts',(0.322097695508164,2.08928744185935,10.5368685902591));
#66505=CARTESIAN_POINT('Ctrl Pts',(0.322394574180558,2.0988508277221,10.5374568198488));
#66506=CARTESIAN_POINT('Ctrl Pts',(0.322304473587786,2.1077098242799,10.5379813178887));
#66507=CARTESIAN_POINT('Ctrl Pts',(0.320543344624518,2.14194887734258,10.5399677603813));
#66508=CARTESIAN_POINT('Ctrl Pts',(0.316236397413458,2.16710050031738,10.5413468143285));
#66509=CARTESIAN_POINT('Ctrl Pts',(0.304438959983997,2.20694942041212,10.5437109711794));
#66510=CARTESIAN_POINT('Ctrl Pts',(0.298707296777487,2.2220454769318,10.5446506404175));
#66511=CARTESIAN_POINT('Ctrl Pts',(0.291369965154471,2.23771751407591,10.5457027066269));
#66512=CARTESIAN_POINT('Ctrl Pts',(0.290863358505971,2.23878428188328,10.545774705388));
#66513=CARTESIAN_POINT('Ctrl Pts',(0.290120038527578,2.24032755224431,10.54587943514));
#66514=CARTESIAN_POINT('Ctrl Pts',(0.289887986375206,2.24080629966053,10.5459120040562));
#66515=CARTESIAN_POINT('Ctrl Pts',(0.289480492622174,2.24164172412853,10.5459689784225));
#66516=CARTESIAN_POINT('Ctrl Pts',(0.289305574159119,2.24199865626495,10.5459933655934));
#66517=CARTESIAN_POINT('Ctrl Pts',(0.288965993843291,2.24268835929184,10.5460405767786));
#66518=CARTESIAN_POINT('Ctrl Pts',(0.288801416301194,2.24302117121557,10.5460633978182));
#66519=CARTESIAN_POINT('Ctrl Pts',(0.288409239192875,2.24381080230298,10.5461176375502));
#66520=CARTESIAN_POINT('Ctrl Pts',(0.288181129362104,2.24426736562937,10.546149074078));
#66521=CARTESIAN_POINT('Ctrl Pts',(0.287372324604835,2.24587662110384,10.5462601459671));
#66522=CARTESIAN_POINT('Ctrl Pts',(0.286785796323622,2.24702635302132,10.5463399859354));
#66523=CARTESIAN_POINT('Ctrl Pts',(0.277473990296513,2.26501192831503,10.5475966630482));
#66524=CARTESIAN_POINT('Ctrl Pts',(0.267288070416979,2.28104587333796,10.5488268991088));
#66525=CARTESIAN_POINT('Ctrl Pts',(0.242114820432351,2.31387863424393,10.5515892470896));
#66526=CARTESIAN_POINT('Ctrl Pts',(0.226657609926543,2.33019544606607,10.5531291554941));
#66527=CARTESIAN_POINT('Ctrl Pts',(0.20347539793629,2.35004931177874,10.5551473341641));
#66528=CARTESIAN_POINT('Ctrl Pts',(0.197120678219569,2.3550889241483,10.555674495576));
#66529=CARTESIAN_POINT('Ctrl Pts',(0.189895166827062,2.36038764720717,10.5562399506711));
#66530=CARTESIAN_POINT('Ctrl Pts',(0.18920626158819,2.360888657891,10.5562935330643));
#66531=CARTESIAN_POINT('Ctrl Pts',(0.188155054648464,2.36164680084135,10.5563747839907));
#66532=CARTESIAN_POINT('Ctrl Pts',(0.187794200757419,2.36190592041364,10.5564025843925));
#66533=CARTESIAN_POINT('Ctrl Pts',(0.187127349168036,2.36238268200749,10.5564537894692));
#66534=CARTESIAN_POINT('Ctrl Pts',(0.186821505342916,2.36260053649778,10.5564772085336));
#66535=CARTESIAN_POINT('Ctrl Pts',(0.186323273899272,2.36295411892931,10.5565152516241));
#66536=CARTESIAN_POINT('Ctrl Pts',(0.186131118183713,2.36309017066962,10.5565298979796));
#66537=CARTESIAN_POINT('Ctrl Pts',(0.185758703992458,2.36335323833534,10.5565582334004));
#66538=CARTESIAN_POINT('Ctrl Pts',(0.185578464815048,2.36348027942862,10.5565719241584));
#66539=CARTESIAN_POINT('Ctrl Pts',(0.185163715864568,2.3637719773942,10.5566033757038));
#66540=CARTESIAN_POINT('Ctrl Pts',(0.184929116103176,2.36393650704296,10.5566211276847));
#66541=CARTESIAN_POINT('Ctrl Pts',(0.184202088224695,2.36444494147689,10.5566760237087));
#66542=CARTESIAN_POINT('Ctrl Pts',(0.183708914321381,2.36478778520095,10.5567130952737));
#66543=CARTESIAN_POINT('Ctrl Pts',(0.179637343743088,2.36760140121782,10.5570178070266));
#66544=CARTESIAN_POINT('Ctrl Pts',(0.176010022518462,2.37000104018423,10.5572807293496));
#66545=CARTESIAN_POINT('Ctrl Pts',(0.172160430631532,2.37243715686939,10.5575521722855));
#66546=CARTESIAN_POINT('Ctrl Pts',(0.171985724289401,2.37254748019269,10.5575644750564));
#66547=CARTESIAN_POINT('Ctrl Pts',(0.16118216205862,2.37935517464807,10.5583242693841));
#66548=CARTESIAN_POINT('Ctrl Pts',(0.150169800502539,2.38542616349531,10.5590398337862));
#66549=CARTESIAN_POINT('Ctrl Pts',(0.117976353414167,2.40079349279074,10.5610469234844));
#66550=CARTESIAN_POINT('Ctrl Pts',(0.096113673907244,2.40847572411003,10.5623166835501));
#66551=CARTESIAN_POINT('Ctrl Pts',(0.065274844612407,2.41571158265307,10.5641554768292));
#66552=CARTESIAN_POINT('Ctrl Pts',(0.0568579670839611,2.4173354081519,10.564661284396));
#66553=CARTESIAN_POINT('Ctrl Pts',(0.0458654961957418,2.41900475848226,
10.5653315777093));
#66554=CARTESIAN_POINT('Ctrl Pts',(0.0433397028400127,2.419357713633,10.5654862416734));
#66555=CARTESIAN_POINT('Ctrl Pts',(0.0400979718247462,2.41977154905724,
10.5656856576872));
#66556=CARTESIAN_POINT('Ctrl Pts',(0.0393856053207816,2.41986007098623,
10.5657295353681));
#66557=CARTESIAN_POINT('Ctrl Pts',(0.0382398082148054,2.41999856726033,
10.5658002023354));
#66558=CARTESIAN_POINT('Ctrl Pts',(0.0378065587415218,2.42005004310909,
10.5658269442029));
#66559=CARTESIAN_POINT('Ctrl Pts',(0.0369828209617547,2.42014621824729,
10.5658778294155));
#66560=CARTESIAN_POINT('Ctrl Pts',(0.0365923524976448,2.42019108332501,
10.5659019674842));
#66561=CARTESIAN_POINT('Ctrl Pts',(0.035704192363729,2.42029148764023,10.5659569120619));
#66562=CARTESIAN_POINT('Ctrl Pts',(0.0352064522332342,2.42034658125813,
10.565987732558));
#66563=CARTESIAN_POINT('Ctrl Pts',(0.0337292669033049,2.42050660290181,
10.5660792871369));
#66564=CARTESIAN_POINT('Ctrl Pts',(0.0327494734469116,2.42060819999485,
10.5661401259636));
#66565=CARTESIAN_POINT('Ctrl Pts',(0.0260113855047616,2.42127567857826,
10.5665593061371));
#66566=CARTESIAN_POINT('Ctrl Pts',(0.0202395431237707,2.42169085735756,
10.5669223609759));
#66567=CARTESIAN_POINT('Ctrl Pts',(-0.0172178028731702,2.42337320013905,
10.5693063371594));
#66568=CARTESIAN_POINT('Ctrl Pts',(-0.0489280897835026,2.4201123125505,
10.5714783113904));
#66569=CARTESIAN_POINT('Ctrl Pts',(-0.0880236101749342,2.41014165716153,
10.5741841571817));
#66570=CARTESIAN_POINT('Ctrl Pts',(-0.0963168031990844,2.40766718858197,
10.5747580994913));
#66571=CARTESIAN_POINT('Ctrl Pts',(-0.109057063921883,2.40330006584989,
10.5756301787366));
#66572=CARTESIAN_POINT('Ctrl Pts',(-0.113577934620847,2.40163625797509,
10.5759376712134));
#66573=CARTESIAN_POINT('Ctrl Pts',(-0.118586076441395,2.39966454183678,
10.5762747683519));
#66574=CARTESIAN_POINT('Ctrl Pts',(-0.119111513942201,2.39945607761063,
10.5763100914047));
#66575=CARTESIAN_POINT('Ctrl Pts',(-0.119894867027678,2.39914289890518,
10.5763626843279));
#66576=CARTESIAN_POINT('Ctrl Pts',(-0.120153196292357,2.39903923242129,
10.5763800169092));
#66577=CARTESIAN_POINT('Ctrl Pts',(-0.120595346399146,2.39886113394254,
10.5764096633702));
#66578=CARTESIAN_POINT('Ctrl Pts',(-0.120779232835042,2.3987868669657,10.5764219872662));
#66579=CARTESIAN_POINT('Ctrl Pts',(-0.12115854960684,2.3986332633328,10.576447396615));
#66580=CARTESIAN_POINT('Ctrl Pts',(-0.121353970099612,2.3985539047698,10.5764604806711));
#66581=CARTESIAN_POINT('Ctrl Pts',(-0.121884230864947,2.39833796383233,
10.5764959658328));
#66582=CARTESIAN_POINT('Ctrl Pts',(-0.122218920670413,2.39820100910352,
10.5765183443094));
#66583=CARTESIAN_POINT('Ctrl Pts',(-0.123470866648126,2.3976862522899,10.5766019848372));
#66584=CARTESIAN_POINT('Ctrl Pts',(-0.124386619531889,2.39730477402026,
10.5766630265201));
#66585=CARTESIAN_POINT('Ctrl Pts',(-0.141116613272475,2.39024467361929,
10.5777759245174));
#66586=CARTESIAN_POINT('Ctrl Pts',(-0.156376640253126,2.38231613100658,
10.5787543278887));
#66587=CARTESIAN_POINT('Ctrl Pts',(-0.179136967381346,2.36807601148445,
10.5802630195009));
#66588=CARTESIAN_POINT('Ctrl Pts',(-0.187104549930598,2.36257701927363,
10.5808015566657));
#66589=CARTESIAN_POINT('Ctrl Pts',(-0.203188372799222,2.35037213921557,
10.5819329174542));
#66590=CARTESIAN_POINT('Ctrl Pts',(-0.211247659363526,2.34361061522045,
10.5825257741194));
#66591=CARTESIAN_POINT('Ctrl Pts',(-0.227386279839951,2.32866674752519,
10.5837914802736));
#66592=CARTESIAN_POINT('Ctrl Pts',(-0.235387082588142,2.320422047849,10.5844658289547));
#66593=CARTESIAN_POINT('Ctrl Pts',(-0.244274463793905,2.31022689081575,
10.5852835815859));
#66594=CARTESIAN_POINT('Ctrl Pts',(-0.245603773718876,2.30867233961381,
10.5854078444174));
#66595=CARTESIAN_POINT('Ctrl Pts',(-0.247343519735688,2.30659815331847,
10.5855731266076));
#66596=CARTESIAN_POINT('Ctrl Pts',(-0.247767301216633,2.30608973324105,
10.585613599555));
#66597=CARTESIAN_POINT('Ctrl Pts',(-0.248459862033337,2.30525362895798,
10.5856800930083));
#66598=CARTESIAN_POINT('Ctrl Pts',(-0.248729567957947,2.30492671193083,
10.5857060757857));
#66599=CARTESIAN_POINT('Ctrl Pts',(-0.249250497121747,2.30429273777351,
10.5857564321111));
#66600=CARTESIAN_POINT('Ctrl Pts',(-0.249501799890435,2.30398574673646,
10.5857808023739));
#66601=CARTESIAN_POINT('Ctrl Pts',(-0.250080102888337,2.30327662532351,
10.5858370638657));
#66602=CARTESIAN_POINT('Ctrl Pts',(-0.250406700518736,2.30287416936089,
10.5858689712581));
#66603=CARTESIAN_POINT('Ctrl Pts',(-0.251447128460819,2.30158574283301,
10.5859710467707));
#66604=CARTESIAN_POINT('Ctrl Pts',(-0.252157232493726,2.30069678665248,
10.586041364226));
#66605=CARTESIAN_POINT('Ctrl Pts',(-0.258562226195379,2.29259092985175,
10.5866815882502));
#66606=CARTESIAN_POINT('Ctrl Pts',(-0.263950066744734,2.28513785547657,
10.5872635778829));
#66607=CARTESIAN_POINT('Ctrl Pts',(-0.28512229784868,2.25304382565872,10.5897461654487));
#66608=CARTESIAN_POINT('Ctrl Pts',(-0.297830858428574,2.22654401784866,
10.5917569510796));
#66609=CARTESIAN_POINT('Ctrl Pts',(-0.310491968264639,2.18719026581581,
10.5945207747618));
#66610=CARTESIAN_POINT('Ctrl Pts',(-0.313545147746194,2.17547794401441,
10.5953150983829));
#66611=CARTESIAN_POINT('Ctrl Pts',(-0.31606938711927,2.16294279820265,10.5961171699345));
#66612=CARTESIAN_POINT('Ctrl Pts',(-0.316203649537132,2.16226480032803,
10.596160404658));
#66613=CARTESIAN_POINT('Ctrl Pts',(-0.316393491237794,2.16128968660102,
10.5962223688447));
#66614=CARTESIAN_POINT('Ctrl Pts',(-0.316450834122996,2.16099292226107,
10.5962411980469));
#66615=CARTESIAN_POINT('Ctrl Pts',(-0.316549613774467,2.16047782263469,
10.5962738296575));
#66616=CARTESIAN_POINT('Ctrl Pts',(-0.316591242288312,2.16025952471552,
10.596287643086));
#66617=CARTESIAN_POINT('Ctrl Pts',(-0.316671285119646,2.15983741155213,
10.5963143228405));
#66618=CARTESIAN_POINT('Ctrl Pts',(-0.31670972839222,2.15963360280017,10.59632719083));
#66619=CARTESIAN_POINT('Ctrl Pts',(-0.316800935970401,2.15914748578624,
10.5963578505104));
#66620=CARTESIAN_POINT('Ctrl Pts',(-0.31685351981461,2.15886514324398,10.5963756318366));
#66621=CARTESIAN_POINT('Ctrl Pts',(-0.31703935137816,2.15785987962582,10.5964388492212));
#66622=CARTESIAN_POINT('Ctrl Pts',(-0.317170504314376,2.15713656632056,
10.5964841665712));
#66623=CARTESIAN_POINT('Ctrl Pts',(-0.319092072746676,2.14632852151334,
10.5971588772194));
#66624=CARTESIAN_POINT('Ctrl Pts',(-0.320403414841058,2.13616328860763,
10.5977618094621));
#66625=CARTESIAN_POINT('Ctrl Pts',(-0.321918157653852,2.11741394208228,
10.5988441931149));
#66626=CARTESIAN_POINT('Ctrl Pts',(-0.322267290657169,2.10885164379212,
10.5993272535047));
#66627=CARTESIAN_POINT('Ctrl Pts',(-0.322296636588479,2.07570046651955,
10.601186051383));
#66628=CARTESIAN_POINT('Ctrl Pts',(-0.319505367940961,2.0511961850701,10.602542691801));
#66629=CARTESIAN_POINT('Ctrl Pts',(-0.312340037700187,2.02027477169855,
10.6044113735494));
#66630=CARTESIAN_POINT('Ctrl Pts',(-0.31049241481586,2.01335786510524,10.6048392905674));
#66631=CARTESIAN_POINT('Ctrl Pts',(-0.308107975234007,2.00549190605433,
10.605339434162));
#66632=CARTESIAN_POINT('Ctrl Pts',(-0.307794765507169,2.00447677503312,
10.6054042398864));
#66633=CARTESIAN_POINT('Ctrl Pts',(-0.307325575837745,2.00298237238634,
10.6055000329622));
#66634=CARTESIAN_POINT('Ctrl Pts',(-0.307173479392267,2.00250188111931,
10.6055308927902));
#66635=CARTESIAN_POINT('Ctrl Pts',(-0.306900312063915,2.00164589620389,
10.6055859762537));
#66636=CARTESIAN_POINT('Ctrl Pts',(-0.306779677323799,2.00127026356069,
10.6056101855034));
#66637=CARTESIAN_POINT('Ctrl Pts',(-0.306526043773771,2.0004854521705,10.6056608436686));
#66638=CARTESIAN_POINT('Ctrl Pts',(-0.306392914790433,2.00007631659774,
10.6056872968324));
#66639=CARTESIAN_POINT('Ctrl Pts',(-0.306043897466262,1.99901096257498,
10.605756294479));
#66640=CARTESIAN_POINT('Ctrl Pts',(-0.305826718586659,1.99835517207938,
10.6057988814705));
#66641=CARTESIAN_POINT('Ctrl Pts',(-0.304879275481652,1.99552481129498,
10.6059831852163));
#66642=CARTESIAN_POINT('Ctrl Pts',(-0.304127928140794,1.99335741675813,
10.6061255976407));
#66643=CARTESIAN_POINT('Ctrl Pts',(-0.298682269830024,1.9781742054304,10.6071324663503));
#66644=CARTESIAN_POINT('Ctrl Pts',(-0.293177774983284,1.96546627276261,
10.6080240757013));
#66645=CARTESIAN_POINT('Ctrl Pts',(-0.271213723579515,1.92255826332494,
10.6112075045243));
#66646=CARTESIAN_POINT('Ctrl Pts',(-0.25076190532429,1.8946693392804,10.6136178430061));
#66647=CARTESIAN_POINT('Ctrl Pts',(-0.225367068715988,1.86962519463814,
10.6158695597912));
#66648=CARTESIAN_POINT('Ctrl Pts',(-0.22443565534175,1.86871769770558,10.615951252841));
#66649=CARTESIAN_POINT('Ctrl Pts',(-0.223208023036623,1.86753598789736,
10.6160577312765));
#66650=CARTESIAN_POINT('Ctrl Pts',(-0.222916762839665,1.8672566750257,10.6160829063184));
#66651=CARTESIAN_POINT('Ctrl Pts',(-0.222466385788397,1.86682639315913,
10.6161216989087));
#66652=CARTESIAN_POINT('Ctrl Pts',(-0.222307639481643,1.86667503956559,
10.6161353463728));
#66653=CARTESIAN_POINT('Ctrl Pts',(-0.221990636653397,1.86637341656219,
10.6161625472941));
#66654=CARTESIAN_POINT('Ctrl Pts',(-0.22183238311201,1.86622314688169,10.6161761007187));
#66655=CARTESIAN_POINT('Ctrl Pts',(-0.221477040660004,1.86588641710555,
10.6162064759576));
#66656=CARTESIAN_POINT('Ctrl Pts',(-0.221279869335252,1.86570004553253,
10.6162232908556));
#66657=CARTESIAN_POINT('Ctrl Pts',(-0.220696249650655,1.86514978652333,
10.6162729461702));
#66658=CARTESIAN_POINT('Ctrl Pts',(-0.220309134979495,1.86478660235013,
10.6163057323226));
#66659=CARTESIAN_POINT('Ctrl Pts',(-0.217265954467987,1.86194564770577,
10.6165623119707));
#66660=CARTESIAN_POINT('Ctrl Pts',(-0.214568933619921,1.85951186088423,
10.6167828058736));
#66661=CARTESIAN_POINT('Ctrl Pts',(-0.204857607450188,1.85104184937922,
10.6175550935828));
#66662=CARTESIAN_POINT('Ctrl Pts',(-0.197624665123048,1.845262249667,10.6180913142792));
#66663=CARTESIAN_POINT('Ctrl Pts',(-0.174733631410519,1.8285335379895,10.619707080129));
#66664=CARTESIAN_POINT('Ctrl Pts',(-0.158343497741734,1.81865809511967,
10.6207566475133));
#66665=CARTESIAN_POINT('Ctrl Pts',(-0.133136484103511,1.80637470779252,
10.6223407512847));
#66666=CARTESIAN_POINT('Ctrl Pts',(-0.124938929559806,1.80279403674246,
10.6228512335219));
#66667=CARTESIAN_POINT('Ctrl Pts',(-0.107467592621994,1.79601327518428,
10.623941705396));
#66668=CARTESIAN_POINT('Ctrl Pts',(-0.0981755345735269,1.79288642586867,
10.6245231228728));
#66669=CARTESIAN_POINT('Ctrl Pts',(-0.0877554484144572,1.78990124086157,
10.6251822306309));
#66670=CARTESIAN_POINT('Ctrl Pts',(-0.0867534059837163,1.78961941804284,
10.6252456822977));
#66671=CARTESIAN_POINT('Ctrl Pts',(-0.0852525691471043,1.78920514580274,
10.6253408278287));
#66672=CARTESIAN_POINT('Ctrl Pts',(-0.0847547865849184,1.78906903002799,
10.6253724026358));
#66673=CARTESIAN_POINT('Ctrl Pts',(-0.0838968731253664,1.78883665179657,
10.625426852469));
#66674=CARTESIAN_POINT('Ctrl Pts',(-0.0835368971228926,1.78873981719055,
10.6254497088985));
#66675=CARTESIAN_POINT('Ctrl Pts',(-0.0827935649358112,1.7885412410224,
10.625496926344));
#66676=CARTESIAN_POINT('Ctrl Pts',(-0.0824101874477816,1.78843958219748,
10.6255212899976));
#66677=CARTESIAN_POINT('Ctrl Pts',(-0.0815173047724491,1.78820458306228,
10.6255780587906));
#66678=CARTESIAN_POINT('Ctrl Pts',(-0.0810076595440639,1.78807178375359,
10.6256104813763));
#66679=CARTESIAN_POINT('Ctrl Pts',(-0.0793820940251987,1.78765245934999,
10.6257139607775));
#66680=CARTESIAN_POINT('Ctrl Pts',(-0.0782649712204857,1.78737067119903,
10.6257851704363));
#66681=CARTESIAN_POINT('Ctrl Pts',(-0.0539025035305845,1.78136413467667,
10.6273403146344));
#66682=CARTESIAN_POINT('Ctrl Pts',(-0.0300976181337822,1.77824236614711,
10.6289118564704));
#66683=CARTESIAN_POINT('Ctrl Pts',(0.0194202162551432,1.77729392558828,
10.6322496605817));
#66684=CARTESIAN_POINT('Ctrl Pts',(0.0449808675715732,1.77985429211685,
10.634009325584));
#66685=CARTESIAN_POINT('Ctrl Pts',(0.0713675412905889,1.78572321458893,
10.635717942723));
#66686=CARTESIAN_POINT('Ctrl Pts',(0.0727624928167553,1.78604324562439,
10.6358079194757));
#66687=CARTESIAN_POINT('Ctrl Pts',(0.074562984093129,1.78646896082003,10.6359235592042));
#66688=CARTESIAN_POINT('Ctrl Pts',(0.074970486011003,1.78656615154366,10.6359496988704));
#66689=CARTESIAN_POINT('Ctrl Pts',(0.0755940662386094,1.78671616343589,
10.6359896475533));
#66690=CARTESIAN_POINT('Ctrl Pts',(0.0758102793292276,1.78676841370714,
10.6360034894033));
#66691=CARTESIAN_POINT('Ctrl Pts',(0.0762362066212751,1.78687181056222,
10.6360307380852));
#66692=CARTESIAN_POINT('Ctrl Pts',(0.0764459223098293,1.786922943697,10.6360441455386));
#66693=CARTESIAN_POINT('Ctrl Pts',(0.0769131365888853,1.78703735789413,
10.636073995078));
#66694=CARTESIAN_POINT('Ctrl Pts',(0.0771706078483092,1.78710074589516,
10.6360904308459));
#66695=CARTESIAN_POINT('Ctrl Pts',(0.0779148099409177,1.78728493877614,
10.6361378985708));
#66696=CARTESIAN_POINT('Ctrl Pts',(0.0784013401768999,1.78740656278343,
10.6361688832511));
#66697=CARTESIAN_POINT('Ctrl Pts',(0.0817089081797216,1.78824160454065,
10.6363792123137));
#66698=CARTESIAN_POINT('Ctrl Pts',(0.0845205709420133,1.78899209442381,
10.6365564546037));
#66699=CARTESIAN_POINT('Ctrl Pts',(0.0933128253739693,1.79146697340311,
10.6371069265859));
#66700=CARTESIAN_POINT('Ctrl Pts',(0.0992541580732603,1.79332666479782,
10.6374733897348));
#66701=CARTESIAN_POINT('Ctrl Pts',(0.119215023012988,1.80021556029978,10.6386973012408));
#66702=CARTESIAN_POINT('Ctrl Pts',(0.132939064138795,1.80604388748199,10.639527016108));
#66703=CARTESIAN_POINT('Ctrl Pts',(0.169542697212373,1.82467860025403,10.641822881413));
#66704=CARTESIAN_POINT('Ctrl Pts',(0.191335748512181,1.83935279048595,10.6432943581486));
#66705=CARTESIAN_POINT('Ctrl Pts',(0.212279481607717,1.8575108658658,10.6449751645429));
#66706=CARTESIAN_POINT('Ctrl Pts',(0.213438517119665,1.85853042062116,10.6450691072026));
#66707=CARTESIAN_POINT('Ctrl Pts',(0.215001014936618,1.85992492331234,10.6451970344123));
#66708=CARTESIAN_POINT('Ctrl Pts',(0.21541091963552,1.86029264807644,10.6452307158567));
#66709=CARTESIAN_POINT('Ctrl Pts',(0.216103699136472,1.86091735131971,10.6452878474066));
#66710=CARTESIAN_POINT('Ctrl Pts',(0.216387063987401,1.86117378657834,10.645311274568));
#66711=CARTESIAN_POINT('Ctrl Pts',(0.216954906414712,1.86168950429582,10.6453583396015));
#66712=CARTESIAN_POINT('Ctrl Pts',(0.217239376954549,1.8619487935788,10.6453819777428));
#66713=CARTESIAN_POINT('Ctrl Pts',(0.217881641035293,1.86253631461306,10.6454354833417));
#66714=CARTESIAN_POINT('Ctrl Pts',(0.21823915807105,1.86286484600949,10.645465363519));
#66715=CARTESIAN_POINT('Ctrl Pts',(0.218983914879014,1.8635523325278,10.6455278100063));
#66716=CARTESIAN_POINT('Ctrl Pts',(0.219371017367135,1.86391143364668,10.6455603825151));
#66717=CARTESIAN_POINT('Ctrl Pts',(0.22037907645848,1.8648511938419,10.6456455061342));
#66718=CARTESIAN_POINT('Ctrl Pts',(0.22099861800348,1.86543335873016,10.6456981218718));
#66719=CARTESIAN_POINT('Ctrl Pts',(0.222822318519872,1.86716067479155,10.6458538967324));
#66720=CARTESIAN_POINT('Ctrl Pts',(0.224019918100671,1.86831268243233,10.6459573520598));
#66721=CARTESIAN_POINT('Ctrl Pts',(0.231298667419133,1.87542353177667,10.6465933494701));
#66722=CARTESIAN_POINT('Ctrl Pts',(0.237150126908992,1.88161167821181,10.6471359483214));
#66723=CARTESIAN_POINT('Ctrl Pts',(0.252169280378877,1.89881119941972,10.6486170249649));
#66724=CARTESIAN_POINT('Ctrl Pts',(0.260858721349144,1.91021346007024,10.6495720562922));
#66725=CARTESIAN_POINT('Ctrl Pts',(0.282501343320614,1.94291984497887,10.6522176987259));
#66726=CARTESIAN_POINT('Ctrl Pts',(0.293790414935612,1.96520912059328,10.6539263126378));
#66727=CARTESIAN_POINT('Ctrl Pts',(0.302891766995221,1.98991017059744,10.6555900763948));
#66728=CARTESIAN_POINT('Ctrl Pts',(0.303374033980378,1.99124620128637,10.6556793697068));
#66729=CARTESIAN_POINT('Ctrl Pts',(0.303986684019226,1.99297922612357,10.6557942567575));
#66730=CARTESIAN_POINT('Ctrl Pts',(0.304125140544139,1.99337331949361,10.6558203196843));
#66731=CARTESIAN_POINT('Ctrl Pts',(0.30433607238275,1.99397745503928,10.6558601764265));
#66732=CARTESIAN_POINT('Ctrl Pts',(0.304409096665997,1.99418730293108,10.6558740028388));
#66733=CARTESIAN_POINT('Ctrl Pts',(0.304552642169033,1.99460118418463,10.6559012370012));
#66734=CARTESIAN_POINT('Ctrl Pts',(0.30462317498462,1.99480521167726,10.6559146453406));
#66735=CARTESIAN_POINT('Ctrl Pts',(0.304780011128814,1.99526036589225,10.6559445193687));
#66736=CARTESIAN_POINT('Ctrl Pts',(0.304866208885128,1.99551152782277,10.6559609786875));
#66737=CARTESIAN_POINT('Ctrl Pts',(0.305114883856299,1.9962390411451,10.6560085810441));
#66738=CARTESIAN_POINT('Ctrl Pts',(0.305276556676943,1.99671566970388,10.6560396763884));
#66739=CARTESIAN_POINT('Ctrl Pts',(0.30637777793519,1.99998736124088,10.6562525096066));
#66740=CARTESIAN_POINT('Ctrl Pts',(0.307280082143515,2.00279494187017,10.6564320877241));
#66741=CARTESIAN_POINT('Ctrl Pts',(0.309989318788065,2.011639897083,10.6569894177268));
#66742=CARTESIAN_POINT('Ctrl Pts',(0.311657886227521,2.01771842015475,10.6573602506798));
#66743=CARTESIAN_POINT('Ctrl Pts',(0.316814249258722,2.0389205061916,10.6586241857859));
#66744=CARTESIAN_POINT('Ctrl Pts',(0.319387696355035,2.0542448223527,10.6594871295216));
#66745=CARTESIAN_POINT('Ctrl Pts',(0.323242548071882,2.09505818281226,10.6617790406768));
#66746=CARTESIAN_POINT('Ctrl Pts',(0.322622227332921,2.1206108252254,10.6632148622806));
#66747=CARTESIAN_POINT('Ctrl Pts',(0.318785689652102,2.14731963711145,10.6648513518471));
#66748=CARTESIAN_POINT('Ctrl Pts',(0.318560066550367,2.14881544695234,10.6649434247268));
#66749=CARTESIAN_POINT('Ctrl Pts',(0.318238675818512,2.1508489827476,10.6650691896555));
#66750=CARTESIAN_POINT('Ctrl Pts',(0.318152057451664,2.15138815200677,10.6651025916431));
#66751=CARTESIAN_POINT('Ctrl Pts',(0.318002696188449,2.15230302025392,10.6651593659371));
#66752=CARTESIAN_POINT('Ctrl Pts',(0.317940656624139,2.15267883421451,10.6651827158922));
#66753=CARTESIAN_POINT('Ctrl Pts',(0.317814554358334,2.15343437997761,10.6652297157877));
#66754=CARTESIAN_POINT('Ctrl Pts',(0.317750476992271,2.15381410869614,10.6652533661601));
#66755=CARTESIAN_POINT('Ctrl Pts',(0.317603577694458,2.15467523815503,10.6653070649342));
#66756=CARTESIAN_POINT('Ctrl Pts',(0.317520341721644,2.15515656643058,10.6653371264502));
#66757=CARTESIAN_POINT('Ctrl Pts',(0.317344161921807,2.15616174478203,10.6654000032942));
#66758=CARTESIAN_POINT('Ctrl Pts',(0.317251014614405,2.15668555727431,10.6654328250236));
#66759=CARTESIAN_POINT('Ctrl Pts',(0.317003956941087,2.15805519807774,10.6655187927285));
#66760=CARTESIAN_POINT('Ctrl Pts',(0.316847959092205,2.15890064122136,10.6655720050934));
#66761=CARTESIAN_POINT('Ctrl Pts',(0.316375773450556,2.16140352331891,10.6657299770651));
#66762=CARTESIAN_POINT('Ctrl Pts',(0.316049953459208,2.16305909487507,10.6658350429276));
#66763=CARTESIAN_POINT('Ctrl Pts',(0.313985769809988,2.17312964953418,10.6664776997566));
#66764=CARTESIAN_POINT('Ctrl Pts',(0.311924574635606,2.18147420811947,10.6670255271976));
#66765=CARTESIAN_POINT('Ctrl Pts',(0.305501076672879,2.20363372966154,10.6685227574027));
#66766=CARTESIAN_POINT('Ctrl Pts',(0.3005371700682,2.21725267244046,10.6694890652514));
#66767=CARTESIAN_POINT('Ctrl Pts',(0.284694823309773,2.25302803402335,10.6721293955553));
#66768=CARTESIAN_POINT('Ctrl Pts',(0.272161205444852,2.27434795152359,10.673819509377));
#66769=CARTESIAN_POINT('Ctrl Pts',(0.256480566732366,2.29514310635147,10.6754651586792));
#66770=CARTESIAN_POINT('Ctrl Pts',(0.255635325303682,2.29624906035773,10.6755526496523));
#66771=CARTESIAN_POINT('Ctrl Pts',(0.254529139669122,2.29767717228812,10.675665549127));
#66772=CARTESIAN_POINT('Ctrl Pts',(0.254274718886656,2.29800433006433,10.6756914073089));
#66773=CARTESIAN_POINT('Ctrl Pts',(0.253883333029285,2.29850561178841,10.6757310187178));
#66774=CARTESIAN_POINT('Ctrl Pts',(0.253746819537513,2.29868008525477,10.6757448039148));
#66775=CARTESIAN_POINT('Ctrl Pts',(0.253475606289268,2.29902597863009,10.6757721293538));
#66776=CARTESIAN_POINT('Ctrl Pts',(0.25334091333697,2.29919740154807,10.6757856698557));
#66777=CARTESIAN_POINT('Ctrl Pts',(0.25304053294945,2.29957889640688,10.6758157996974));
#66778=CARTESIAN_POINT('Ctrl Pts',(0.252874758251384,2.29978889820728,10.6758323826292));
#66779=CARTESIAN_POINT('Ctrl Pts',(0.252390492903354,2.30040079258708,10.6758806942903));
#66780=CARTESIAN_POINT('Ctrl Pts',(0.252071302452214,2.30080213411753,10.6759123731031));
#66781=CARTESIAN_POINT('Ctrl Pts',(0.249775341585834,2.30367491241943,10.6761390787685));
#66782=CARTESIAN_POINT('Ctrl Pts',(0.247763131919493,2.30611798440837,10.6763316115882));
#66783=CARTESIAN_POINT('Ctrl Pts',(0.242982958190087,2.31175053055,10.6767759438701));
#66784=CARTESIAN_POINT('Ctrl Pts',(0.240187605164842,2.31491608346832,10.6770260078519));
#66785=CARTESIAN_POINT('Ctrl Pts',(0.236070163782979,2.31939809758182,10.6773821157901));
#66786=CARTESIAN_POINT('Ctrl Pts',(0.234797714351001,2.32075932828418,10.6774905507741));
#66787=CARTESIAN_POINT('Ctrl Pts',(0.221179417581971,2.33507684602119,10.6786350476556));
#66788=CARTESIAN_POINT('Ctrl Pts',(0.207785796953426,2.34699515946784,10.6796240725259));
#66789=CARTESIAN_POINT('Ctrl Pts',(0.174864977644883,2.37170695202786,10.6819295707037));
#66790=CARTESIAN_POINT('Ctrl Pts',(0.154804513776457,2.3836155056448,10.6832522843232));
#66791=CARTESIAN_POINT('Ctrl Pts',(0.132384573503583,2.39383226526825,10.6847478978134));
#66792=CARTESIAN_POINT('Ctrl Pts',(0.131126697112627,2.39439576190327,10.6848318390195));
#66793=CARTESIAN_POINT('Ctrl Pts',(0.129384850896691,2.39516268652608,10.6849481306165));
#66794=CARTESIAN_POINT('Ctrl Pts',(0.128903928264723,2.39537303267501,10.6849802442848));
#66795=CARTESIAN_POINT('Ctrl Pts',(0.128078434539242,2.39573168743855,10.6850353772197));
#66796=CARTESIAN_POINT('Ctrl Pts',(0.127734113380773,2.39588057155916,10.6850583768034));
#66797=CARTESIAN_POINT('Ctrl Pts',(0.12703355943618,2.39618203960731,10.6851051783191));
#66798=CARTESIAN_POINT('Ctrl Pts',(0.126677309862307,2.39633458281642,10.6851289815937));
#66799=CARTESIAN_POINT('Ctrl Pts',(0.125857034529815,2.39668406865077,10.685183797833));
#66800=CARTESIAN_POINT('Ctrl Pts',(0.125392821014815,2.39688056548915,10.6852148258958));
#66801=CARTESIAN_POINT('Ctrl Pts',(0.124417825513626,2.39729057638326,10.6852800085365));
#66802=CARTESIAN_POINT('Ctrl Pts',(0.123906950977858,2.39750386485739,10.6853141706643));
#66803=CARTESIAN_POINT('Ctrl Pts',(0.122553639292316,2.39806477763315,10.6854046888093));
#66804=CARTESIAN_POINT('Ctrl Pts',(0.121710277337476,2.39841014482141,10.6854611211099));
#66805=CARTESIAN_POINT('Ctrl Pts',(0.104502349013638,2.40537192190849,10.6866130685066));
#66806=CARTESIAN_POINT('Ctrl Pts',(0.0876259173606703,2.41063525641142,
10.6877546825072));
#66807=CARTESIAN_POINT('Ctrl Pts',(0.0396795872400225,2.42136915630836,
10.6910242769546));
#66808=CARTESIAN_POINT('Ctrl Pts',(0.00811265859031779,2.42370783364828,
10.6932195853288));
#66809=CARTESIAN_POINT('Ctrl Pts',(-0.0248352673564854,2.42132037092403,
10.6953098178013));
#66810=CARTESIAN_POINT('Ctrl Pts',(-0.0263782197607249,2.42119738639265,
10.6954071922975));
#66811=CARTESIAN_POINT('Ctrl Pts',(-0.0283452870637515,2.42102632655017,
10.695530628623));
#66812=CARTESIAN_POINT('Ctrl Pts',(-0.0287702407712169,2.42098852142714,
10.6955572531464));
#66813=CARTESIAN_POINT('Ctrl Pts',(-0.0294453934027655,2.42092710634487,
10.6955994853193));
#66814=CARTESIAN_POINT('Ctrl Pts',(-0.0296956400592102,2.42090404756258,
10.6956151239062));
#66815=CARTESIAN_POINT('Ctrl Pts',(-0.0301632261325376,2.4208604105738,
10.6956443165365));
#66816=CARTESIAN_POINT('Ctrl Pts',(-0.0303805699767417,2.42083990439567,
10.6956578745056));
#66817=CARTESIAN_POINT('Ctrl Pts',(-0.0308690375485982,2.42079331715749,
10.6956883198061));
#66818=CARTESIAN_POINT('Ctrl Pts',(-0.0311401485078071,2.42076711328361,
10.6957052000784));
#66819=CARTESIAN_POINT('Ctrl Pts',(-0.0319446094951967,2.42068832965132,
10.6957552371758));
#66820=CARTESIAN_POINT('Ctrl Pts',(-0.0324778652822323,2.42063476281721,
10.6957883384688));
#66821=CARTESIAN_POINT('Ctrl Pts',(-0.0367726541316475,2.42019251661014,
10.6960544111927));
#66822=CARTESIAN_POINT('Ctrl Pts',(-0.0405274109805555,2.41973896820824,
10.6962838024268));
#66823=CARTESIAN_POINT('Ctrl Pts',(-0.0541199133891425,2.41785378269916,
10.697105310293));
#66824=CARTESIAN_POINT('Ctrl Pts',(-0.0638987778620044,2.41603318470171,
10.6976794049073));
#66825=CARTESIAN_POINT('Ctrl Pts',(-0.0883490186137163,2.41029951428344,
10.6991062673484));
#66826=CARTESIAN_POINT('Ctrl Pts',(-0.102856753168576,2.4057970769823,10.699945623268));
#66827=CARTESIAN_POINT('Ctrl Pts',(-0.137106292330893,2.39245334591317,
10.7020093375182));
#66828=CARTESIAN_POINT('Ctrl Pts',(-0.156377485599329,2.38261805928396,
10.7032442401006));
#66829=CARTESIAN_POINT('Ctrl Pts',(-0.17561307943088,2.37022752149179,10.7046339209849));
#66830=CARTESIAN_POINT('Ctrl Pts',(-0.176702141183835,2.36951664190246,
10.7047131527609));
#66831=CARTESIAN_POINT('Ctrl Pts',(-0.178213932620552,2.36851672578854,
10.7048239229565));
#66832=CARTESIAN_POINT('Ctrl Pts',(-0.178640331559171,2.3682332375824,10.7048552530785));
#66833=CARTESIAN_POINT('Ctrl Pts',(-0.179375106664404,2.36774219859225,
10.7049093935526));
#66834=CARTESIAN_POINT('Ctrl Pts',(-0.179683803582517,2.36753512764891,
10.7049321857958));
#66835=CARTESIAN_POINT('Ctrl Pts',(-0.18031505475115,2.36711010501215,10.7049788890919));
#66836=CARTESIAN_POINT('Ctrl Pts',(-0.180637573651193,2.36689210208032,
10.7050028020579));
#66837=CARTESIAN_POINT('Ctrl Pts',(-0.181385962907543,2.36638425902912,
10.7050584107111));
#66838=CARTESIAN_POINT('Ctrl Pts',(-0.181811533996101,2.3660939817047,10.7050901229393));
#66839=CARTESIAN_POINT('Ctrl Pts',(-0.182705622995961,2.36548098727846,
10.7051569390628));
#66840=CARTESIAN_POINT('Ctrl Pts',(-0.183173985591036,2.36515804773142,
10.7051920513624));
#66841=CARTESIAN_POINT('Ctrl Pts',(-0.184420619600864,2.3642936049633,10.7052858074805));
#66842=CARTESIAN_POINT('Ctrl Pts',(-0.185197356223901,2.36374990763086,
10.705344535034));
#66843=CARTESIAN_POINT('Ctrl Pts',(-0.203196940280945,2.35103190892641,
10.706712755718));
#66844=CARTESIAN_POINT('Ctrl Pts',(-0.219182381455994,2.33720199514564,
10.7080891514079));
#66845=CARTESIAN_POINT('Ctrl Pts',(-0.248567640916915,2.30625586813309,
10.7109528096696));
#66846=CARTESIAN_POINT('Ctrl Pts',(-0.261823764726807,2.28914461730038,
10.7124343056609));
#66847=CARTESIAN_POINT('Ctrl Pts',(-0.274078660937576,2.26954171839249,
10.7139536215175));
#66848=CARTESIAN_POINT('Ctrl Pts',(-0.274878797931887,2.2682413541729,10.7140536067864));
#66849=CARTESIAN_POINT('Ctrl Pts',(-0.276346327984832,2.26581793949615,
10.7142384018279));
#66850=CARTESIAN_POINT('Ctrl Pts',(-0.277016190000943,2.26469642567655,
10.7143233161256));
#66851=CARTESIAN_POINT('Ctrl Pts',(-0.277825243331271,2.26332297009478,
10.7144265419354));
#66852=CARTESIAN_POINT('Ctrl Pts',(-0.2779709307249,2.26307489097193,10.714445156741));
#66853=CARTESIAN_POINT('Ctrl Pts',(-0.278331126464863,2.26245965800917,
10.7144912456802));
#66854=CARTESIAN_POINT('Ctrl Pts',(-0.27854524135384,2.26209227298867,10.7145187010535));
#66855=CARTESIAN_POINT('Ctrl Pts',(-0.280800362596487,2.25820520176694,
10.7148084784105));
#66856=CARTESIAN_POINT('Ctrl Pts',(-0.282775387957434,2.25464738370695,
10.7150675629167));
#66857=CARTESIAN_POINT('Ctrl Pts',(-0.284934457358211,2.25057828308921,
10.7153561810135));
#66858=CARTESIAN_POINT('Ctrl Pts',(-0.285185114169217,2.25010301460757,
10.715389774017));
#66859=CARTESIAN_POINT('Ctrl Pts',(-0.28556292910928,2.24938227994497,10.7154405369427));
#66860=CARTESIAN_POINT('Ctrl Pts',(-0.285690960411689,2.24913727630437,
10.7154577616426));
#66861=CARTESIAN_POINT('Ctrl Pts',(-0.285913212403205,2.24871063333872,
10.7154877011998));
#66862=CARTESIAN_POINT('Ctrl Pts',(-0.286007575378837,2.24852906894342,
10.7155004251011));
#66863=CARTESIAN_POINT('Ctrl Pts',(-0.286205055633203,2.24814820993236,
10.715527078906));
#66864=CARTESIAN_POINT('Ctrl Pts',(-0.286308137666018,2.24794889753811,
10.7155410065065));
#66865=CARTESIAN_POINT('Ctrl Pts',(-0.286555054845509,2.24747025084163,
10.7155744035995));
#66866=CARTESIAN_POINT('Ctrl Pts',(-0.286698690340707,2.24719081255205,
10.7155938603938));
#66867=CARTESIAN_POINT('Ctrl Pts',(-0.287188368144886,2.24623472373415,
10.7156602935379));
#66868=CARTESIAN_POINT('Ctrl Pts',(-0.287532428853326,2.24555705276143,
10.7157071456582));
#66869=CARTESIAN_POINT('Ctrl Pts',(-0.297370732583404,2.22600826288821,
10.7170521064542));
#66870=CARTESIAN_POINT('Ctrl Pts',(-0.304990758557198,2.20624680751465,
10.7182370965088));
#66871=CARTESIAN_POINT('Ctrl Pts',(-0.317150367442741,2.16226567269911,
10.7207893142002));
#66872=CARTESIAN_POINT('Ctrl Pts',(-0.320964350568361,2.13798819359144,
10.7221516127689));
#66873=CARTESIAN_POINT('Ctrl Pts',(-0.322180229001526,2.10901803356642,
10.7238757771092));
#66874=CARTESIAN_POINT('Ctrl Pts',(-0.322274729601769,2.10451883197574,
10.7241460642757));
#66875=CARTESIAN_POINT('Ctrl Pts',(-0.322274999420556,2.10001932564221,
10.7244193016094));
#66876=CARTESIAN_POINT('',(-0.322274972444447,2.10013327014249,10.9749989620444));
#66877=CARTESIAN_POINT('Ctrl Pts',(-0.322274999426371,2.10001922843493,
10.7244193075124));
#66878=CARTESIAN_POINT('Ctrl Pts',(-0.322275071231016,2.09881575857202,
10.724492389518));
#66879=CARTESIAN_POINT('Ctrl Pts',(-0.322268401869339,2.09761230732818,
10.7245656794142));
#66880=CARTESIAN_POINT('Ctrl Pts',(-0.322249745832144,2.09593815378055,
10.724667934721));
#66881=CARTESIAN_POINT('Ctrl Pts',(-0.322243468099963,2.09546739072966,
10.7246967213388));
#66882=CARTESIAN_POINT('Ctrl Pts',(-0.32223032281347,2.09462078146521,10.7247485504602));
#66883=CARTESIAN_POINT('Ctrl Pts',(-0.322223829186279,2.09424492961336,
10.7247715812266));
#66884=CARTESIAN_POINT('Ctrl Pts',(-0.322209296423054,2.09348114419906,
10.7248184266186));
#66885=CARTESIAN_POINT('Ctrl Pts',(-0.322201214246663,2.09309321216156,
10.7248422425534));
#66886=CARTESIAN_POINT('Ctrl Pts',(-0.322183613877894,2.09231583909616,
10.7248900131817));
#66887=CARTESIAN_POINT('Ctrl Pts',(-0.322174090116559,2.0919263988397,10.7249139680112));
#66888=CARTESIAN_POINT('Ctrl Pts',(-0.322145415167206,2.09083482274152,
10.7249811773983));
#66889=CARTESIAN_POINT('Ctrl Pts',(-0.322124674678532,2.09013273400593,
10.7250244816914));
#66890=CARTESIAN_POINT('Ctrl Pts',(-0.322030837631842,2.08727302403359,
10.7252011801512));
#66891=CARTESIAN_POINT('Ctrl Pts',(-0.321938358205441,2.08511613442245,
10.7253351802876));
#66892=CARTESIAN_POINT('Ctrl Pts',(-0.319893129560837,2.04648827570738,
10.7277484858106));
#66893=CARTESIAN_POINT('Ctrl Pts',(-0.311775686476974,2.01061565133469,
10.7302506036039));
#66894=CARTESIAN_POINT('Ctrl Pts',(-0.293430908289663,1.9662386319519,10.7334657931135));
#66895=CARTESIAN_POINT('Ctrl Pts',(-0.288463479569405,1.95583799611667,
10.7342249254026));
#66896=CARTESIAN_POINT('Ctrl Pts',(-0.282196014634781,1.94434313099519,
10.7350533084369));
#66897=CARTESIAN_POINT('Ctrl Pts',(-0.281432640259525,1.94296713471299,
10.7351522865069));
#66898=CARTESIAN_POINT('Ctrl Pts',(-0.280455436392794,1.94123572289609,
10.7352765438088));
#66899=CARTESIAN_POINT('Ctrl Pts',(-0.280250974865409,1.94087508498612,
10.7353024097097));
#66900=CARTESIAN_POINT('Ctrl Pts',(-0.279924015668816,1.94030096539189,
10.7353435606193));
#66901=CARTESIAN_POINT('Ctrl Pts',(-0.279801969214595,1.94008722931695,
10.7353588746244));
#66902=CARTESIAN_POINT('Ctrl Pts',(-0.279570837359988,1.9396835301415,10.7353877879324));
#66903=CARTESIAN_POINT('Ctrl Pts',(-0.279461804032013,1.93949354001307,
10.7354013903852));
#66904=CARTESIAN_POINT('Ctrl Pts',(-0.279212819747438,1.93906070874216,
10.7354323684042));
#66905=CARTESIAN_POINT('Ctrl Pts',(-0.279072745893889,1.93881793932771,
10.7354497358507));
#66906=CARTESIAN_POINT('Ctrl Pts',(-0.278653946759488,1.93809427890708,
10.7355014835879));
#66907=CARTESIAN_POINT('Ctrl Pts',(-0.278374292100854,1.93761392277815,
10.7355358038853));
#66908=CARTESIAN_POINT('Ctrl Pts',(-0.27640369126366,1.93424911953815,10.7357760234984));
#66909=CARTESIAN_POINT('Ctrl Pts',(-0.274669110858645,1.93139028324105,
10.7359791525689));
#66910=CARTESIAN_POINT('Ctrl Pts',(-0.264994806037818,1.9159912772424,10.7370709058047));
#66911=CARTESIAN_POINT('Ctrl Pts',(-0.256239619859653,1.90398260881372,
10.7379139780569));
#66912=CARTESIAN_POINT('Ctrl Pts',(-0.227230156318473,1.86947483551174,
10.7404454445568));
#66913=CARTESIAN_POINT('Ctrl Pts',(-0.204616214479551,1.84918645442211,
10.7421067196102));
#66914=CARTESIAN_POINT('Ctrl Pts',(-0.177897636787063,1.83126711826859,
10.744041884923));
#66915=CARTESIAN_POINT('Ctrl Pts',(-0.176278550159977,1.83020229170451,
10.7441589768219));
#66916=CARTESIAN_POINT('Ctrl Pts',(-0.173850089544586,1.82863635492723,
10.7443343890193));
#66917=CARTESIAN_POINT('Ctrl Pts',(-0.173047919611941,1.82812411105513,
10.7443922968442));
#66918=CARTESIAN_POINT('Ctrl Pts',(-0.171761381140242,1.82731056317374,
10.7444851210777));
#66919=CARTESIAN_POINT('Ctrl Pts',(-0.171278457192703,1.82700697609108,
10.7445199530947));
#66920=CARTESIAN_POINT('Ctrl Pts',(-0.170357014085049,1.82643112420485,
10.7445863944146));
#66921=CARTESIAN_POINT('Ctrl Pts',(-0.169918641423097,1.82615862740662,
10.7446179950448));
#66922=CARTESIAN_POINT('Ctrl Pts',(-0.169148383254385,1.82568238896164,
10.7446735058839));
#66923=CARTESIAN_POINT('Ctrl Pts',(-0.168816778715979,1.82547819302436,
10.7446973993161));
#66924=CARTESIAN_POINT('Ctrl Pts',(-0.168168216441499,1.8250804398906,10.7447441222339));
#66925=CARTESIAN_POINT('Ctrl Pts',(-0.167851292509247,1.82488682846319,
10.7447669496817));
#66926=CARTESIAN_POINT('Ctrl Pts',(-0.167097703197015,1.82442824146782,
10.7448212202359));
#66927=CARTESIAN_POINT('Ctrl Pts',(-0.166660742142921,1.82416375593876,
10.7448526812252));
#66928=CARTESIAN_POINT('Ctrl Pts',(-0.165115391301949,1.82323339236031,
10.7449639216238));
#66929=CARTESIAN_POINT('Ctrl Pts',(-0.16400363594759,1.82257315402616,10.7450439064569));
#66930=CARTESIAN_POINT('Ctrl Pts',(-0.146216114275567,1.81215396132018,
10.7463230212281));
#66931=CARTESIAN_POINT('Ctrl Pts',(-0.128703039825372,1.80390917296598,
10.7475776898895));
#66932=CARTESIAN_POINT('Ctrl Pts',(-0.10122452635352,1.7938733127751,10.7495326277874));
#66933=CARTESIAN_POINT('Ctrl Pts',(-0.0917365454891338,1.79089751362767,
10.7502046010085));
#66934=CARTESIAN_POINT('Ctrl Pts',(-0.0792810318761317,1.78761505619139,
10.751076284176));
#66935=CARTESIAN_POINT('Ctrl Pts',(-0.0764253359104456,1.78690416281836,
10.7512754185548));
#66936=CARTESIAN_POINT('Ctrl Pts',(-0.0645557636823324,1.78412143610218,
10.7520994078017));
#66937=CARTESIAN_POINT('Ctrl Pts',(-0.0554640918823204,1.78239889135977,
10.7527218807366));
#66938=CARTESIAN_POINT('Ctrl Pts',(-0.0404041775757072,1.78021210346509,
10.7537277357974));
#66939=CARTESIAN_POINT('Ctrl Pts',(-0.0344747202440961,1.77951864414725,
10.7541173818149));
#66940=CARTESIAN_POINT('Ctrl Pts',(-0.0254375787758044,1.77871548758478,
10.7546983185686));
#66941=CARTESIAN_POINT('Ctrl Pts',(-0.0223421527856966,1.77848539956211,
10.7548950059402));
#66942=CARTESIAN_POINT('Ctrl Pts',(-0.0187344709486156,1.7782695918707,
10.755121197609));
#66943=CARTESIAN_POINT('Ctrl Pts',(-0.0182251175399177,1.77824033656169,
10.7551530620477));
#66944=CARTESIAN_POINT('Ctrl Pts',(-0.0174490977715468,1.77819761358838,
10.7552014989999));
#66945=CARTESIAN_POINT('Ctrl Pts',(-0.017182483583713,1.77818326772464,
10.7552181205703));
#66946=CARTESIAN_POINT('Ctrl Pts',(-0.0167192312684698,1.7781589185688,
10.7552469665411));
#66947=CARTESIAN_POINT('Ctrl Pts',(-0.0165226022818038,1.77814876416959,
10.7552591994507));
#66948=CARTESIAN_POINT('Ctrl Pts',(-0.0161101781189644,1.77812784452729,
10.7552848348399));
#66949=CARTESIAN_POINT('Ctrl Pts',(-0.015894382099532,1.77811711613384,
10.7552982351843));
#66950=CARTESIAN_POINT('Ctrl Pts',(-0.015291720758094,1.77808776209614,
10.7553356227266));
#66951=CARTESIAN_POINT('Ctrl Pts',(-0.0149048307575997,1.77806961674947,
10.7553595828572));
#66952=CARTESIAN_POINT('Ctrl Pts',(-0.0133463366482733,1.77799933805927,
10.7554559366748));
#66953=CARTESIAN_POINT('Ctrl Pts',(-0.0121744659209222,1.7779529017814,
10.755528014592));
#66954=CARTESIAN_POINT('Ctrl Pts',(0.00903217720685857,1.77722849271919,
10.756826039568));
#66955=CARTESIAN_POINT('Ctrl Pts',(0.0290903524390058,1.7784148001388,10.7579530513595));
#66956=CARTESIAN_POINT('Ctrl Pts',(0.0649687280313703,1.78392378279875,
10.7599840783063));
#66957=CARTESIAN_POINT('Ctrl Pts',(0.0808168358435746,1.78760006349287,
10.760886989693));
#66958=CARTESIAN_POINT('Ctrl Pts',(0.101692487984703,1.79413807960347,10.7621420781163));
#66959=CARTESIAN_POINT('Ctrl Pts',(0.107020254088062,1.79596129022122,10.7624682339063));
#66960=CARTESIAN_POINT('Ctrl Pts',(0.117375475337941,1.79981085195418,10.7631161872089));
#66961=CARTESIAN_POINT('Ctrl Pts',(0.122404960042232,1.80182631309415,10.7634375768791));
#66962=CARTESIAN_POINT('Ctrl Pts',(0.129253350831111,1.80477313558491,10.7638856613695));
#66963=CARTESIAN_POINT('Ctrl Pts',(0.131117928720049,1.80559650367018,10.7640087444872));
#66964=CARTESIAN_POINT('Ctrl Pts',(0.133874424361935,1.80684510907278,10.7641923755897));
#66965=CARTESIAN_POINT('Ctrl Pts',(0.134772422951401,1.80725686079639,10.7642524636148));
#66966=CARTESIAN_POINT('Ctrl Pts',(0.136199478095798,1.8079191542628,10.7643483820709));
#66967=CARTESIAN_POINT('Ctrl Pts',(0.13672977459112,1.80816702206007,10.7643841204526));
#66968=CARTESIAN_POINT('Ctrl Pts',(0.137736167825031,1.80864076917502,10.7644521264135));
#66969=CARTESIAN_POINT('Ctrl Pts',(0.138212392101161,1.80886637435961,10.7644843844402));
#66970=CARTESIAN_POINT('Ctrl Pts',(0.139041197517942,1.80926150225879,10.7645406616215));
#66971=CARTESIAN_POINT('Ctrl Pts',(0.139394028259233,1.80943050132624,10.7645646625604));
#66972=CARTESIAN_POINT('Ctrl Pts',(0.140078642529937,1.80975995218214,10.764611317028));
#66973=CARTESIAN_POINT('Ctrl Pts',(0.140410460431428,1.80992033154662,10.7646339680096));
#66974=CARTESIAN_POINT('Ctrl Pts',(0.141191584680361,1.81029953089555,10.7646873814043));
#66975=CARTESIAN_POINT('Ctrl Pts',(0.1416406576133,1.81051882705386,10.7647181603851));
#66976=CARTESIAN_POINT('Ctrl Pts',(0.143192286539123,1.81128101022069,10.764824755585));
#66977=CARTESIAN_POINT('Ctrl Pts',(0.144292235541167,1.81182915366252,10.7649007553378));
#66978=CARTESIAN_POINT('Ctrl Pts',(0.15783027375413,1.81867258041363,10.765841590102));
#66979=CARTESIAN_POINT('Ctrl Pts',(0.1698486129835,1.82576129681626,10.7667346747713));
#66980=CARTESIAN_POINT('Ctrl Pts',(0.197570455402011,1.84463508076959,10.7689403637104));
#66981=CARTESIAN_POINT('Ctrl Pts',(0.212730673774667,1.85711965645391,10.770273185989));
#66982=CARTESIAN_POINT('Ctrl Pts',(0.229498787228987,1.87370944920864,10.7718653456669));
#66983=CARTESIAN_POINT('Ctrl Pts',(0.232283817602781,1.87656916981761,10.772134070984));
#66984=CARTESIAN_POINT('Ctrl Pts',(0.243001812815436,1.88799166851324,10.7731833122818));
#66985=CARTESIAN_POINT('Ctrl Pts',(0.250521232929412,1.89693205973604,10.7739531628135));
#66986=CARTESIAN_POINT('Ctrl Pts',(0.258492362605685,1.90752822086026,10.774792203657));
#66987=CARTESIAN_POINT('Ctrl Pts',(0.259435760607198,1.90880174254579,10.7748918997785));
#66988=CARTESIAN_POINT('Ctrl Pts',(0.260614658193905,1.91041796425722,10.7750169309105));
#66989=CARTESIAN_POINT('Ctrl Pts',(0.260858920101935,1.91075420176454,10.7750428614043));
#66990=CARTESIAN_POINT('Ctrl Pts',(0.26124694007584,1.91129050734682,10.7750840911573));
#66991=CARTESIAN_POINT('Ctrl Pts',(0.261391119279807,1.91149026794609,10.7750994196049));
#66992=CARTESIAN_POINT('Ctrl Pts',(0.261663041772791,1.91186792893938,10.7751283447513));
#66993=CARTESIAN_POINT('Ctrl Pts',(0.261790831721598,1.91204579276277,10.7751419446351));
#66994=CARTESIAN_POINT('Ctrl Pts',(0.26208152337631,1.91245126214818,10.7751728961832));
#66995=CARTESIAN_POINT('Ctrl Pts',(0.262244309660165,1.91267894934807,10.7751902397797));
#66996=CARTESIAN_POINT('Ctrl Pts',(0.262739426309118,1.91337337335538,10.7752430246139));
#66997=CARTESIAN_POINT('Ctrl Pts',(0.263070811067957,1.91384078780257,10.7752784007617));
#66998=CARTESIAN_POINT('Ctrl Pts',(0.265443659316382,1.91720665248914,10.7755320661917));
#66999=CARTESIAN_POINT('Ctrl Pts',(0.267438519436596,1.92013787222983,10.7757472375644));
#67000=CARTESIAN_POINT('Ctrl Pts',(0.284868547498301,1.9466806888883,10.7776505903795));
#67001=CARTESIAN_POINT('Ctrl Pts',(0.297191888038881,1.9721940208487,10.7791735754917));
#67002=CARTESIAN_POINT('Ctrl Pts',(0.311383905834111,2.01519216786424,10.781730448985));
#67003=CARTESIAN_POINT('Ctrl Pts',(0.315435945604865,2.03179184338841,10.7827136778393));
#67004=CARTESIAN_POINT('Ctrl Pts',(0.318427311624856,2.05031960030041,10.7838448242673));
#67005=CARTESIAN_POINT('Ctrl Pts',(0.318686220057063,2.05200846036615,10.7839482138366));
#67006=CARTESIAN_POINT('Ctrl Pts',(0.319056336079188,2.05455791775516,10.7841047438543));
#67007=CARTESIAN_POINT('Ctrl Pts',(0.319177520085052,2.05541705392875,10.784157570415));
#67008=CARTESIAN_POINT('Ctrl Pts',(0.319367864126841,2.05680706549928,10.7842431691628));
#67009=CARTESIAN_POINT('Ctrl Pts',(0.319439173841702,2.0573376461311,10.7842758735413));
#67010=CARTESIAN_POINT('Ctrl Pts',(0.319573262441995,2.05835452029766,10.7843386119768));
#67011=CARTESIAN_POINT('Ctrl Pts',(0.319636254253694,2.05884078462938,10.7843686392312));
#67012=CARTESIAN_POINT('Ctrl Pts',(0.319746816419192,2.05970982999606,10.7844223507599));
#67013=CARTESIAN_POINT('Ctrl Pts',(0.319794809844953,2.06009255704398,10.7844460216299));
#67014=CARTESIAN_POINT('Ctrl Pts',(0.319888703606981,2.06085236625626,10.7844930470443));
#67015=CARTESIAN_POINT('Ctrl Pts',(0.319934624587577,2.0612294453074,10.7845164008981));
#67016=CARTESIAN_POINT('Ctrl Pts',(0.32004448721629,2.06214506709988,10.7845731479283));
#67017=CARTESIAN_POINT('Ctrl Pts',(0.320107736194813,2.06268369036332,10.7846065629006));
#67018=CARTESIAN_POINT('Ctrl Pts',(0.320339488150029,2.06470122478588,10.7847318514268));
#67019=CARTESIAN_POINT('Ctrl Pts',(0.320499102103547,2.06618112019379,10.7848240046562));
#67020=CARTESIAN_POINT('Ctrl Pts',(0.323161621160324,2.09258145131041,10.7864725971496));
#67021=CARTESIAN_POINT('Ctrl Pts',(0.322760823560495,2.11770335857479,10.7881253734787));
#67022=CARTESIAN_POINT('Ctrl Pts',(0.317370000806845,2.1582051174682,10.7908846012924));
#67023=CARTESIAN_POINT('Ctrl Pts',(0.314129935263931,2.1737154431584,10.7919619721888));
#67024=CARTESIAN_POINT('Ctrl Pts',(0.308007233188501,2.19504332688944,10.7934305446403));
#67025=CARTESIAN_POINT('Ctrl Pts',(0.306069928919368,2.20110835592257,10.7938464622694));
#67026=CARTESIAN_POINT('Ctrl Pts',(0.302944530816949,2.20997733351943,10.7944482968885));
#67027=CARTESIAN_POINT('Ctrl Pts',(0.301894443458182,2.21282796327431,10.7946407403734));
#67028=CARTESIAN_POINT('Ctrl Pts',(0.300622092144337,2.21613694802083,10.7948626076759));
#67029=CARTESIAN_POINT('Ctrl Pts',(0.30043890366985,2.21661002594482,10.7948942910111));
#67030=CARTESIAN_POINT('Ctrl Pts',(0.300157818160025,2.21733086032883,10.7949425093532));
#67031=CARTESIAN_POINT('Ctrl Pts',(0.300060730798659,2.21757892847742,10.7949590927445));
#67032=CARTESIAN_POINT('Ctrl Pts',(0.299891372668915,2.21801007993265,10.7949878966836));
#67033=CARTESIAN_POINT('Ctrl Pts',(0.299819241944028,2.21819321692788,10.7950001256592));
#67034=CARTESIAN_POINT('Ctrl Pts',(0.299655806368628,2.21860706090262,10.7950277468018));
#67035=CARTESIAN_POINT('Ctrl Pts',(0.299564403033707,2.21883772811042,10.7950431328937));
#67036=CARTESIAN_POINT('Ctrl Pts',(0.299316277833658,2.21946179629435,10.7950847352356));
#67037=CARTESIAN_POINT('Ctrl Pts',(0.299159046126975,2.21985499603826,10.7951109206773));
#67038=CARTESIAN_POINT('Ctrl Pts',(0.298451903872994,2.22161333269684,10.7952279047314));
#67039=CARTESIAN_POINT('Ctrl Pts',(0.297893409748926,2.22297503094965,10.7953181927988));
#67040=CARTESIAN_POINT('Ctrl Pts',(0.285909481187194,2.25163300556032,10.7972128404567));
#67041=CARTESIAN_POINT('Ctrl Pts',(0.270785710903568,2.27723590320793,10.7988084950194));
#67042=CARTESIAN_POINT('Ctrl Pts',(0.24122658197557,2.31445832677159,10.8014868305058));
#67043=CARTESIAN_POINT('Ctrl Pts',(0.228925952603847,2.32754211943909,10.8025169019109));
#67044=CARTESIAN_POINT('Ctrl Pts',(0.214298546585514,2.34070809314253,10.8037025636924));
#67045=CARTESIAN_POINT('Ctrl Pts',(0.212985107102912,2.34187103410509,10.8038086875691));
#67046=CARTESIAN_POINT('Ctrl Pts',(0.210995186752885,2.34360416524386,10.8039689954851));
#67047=CARTESIAN_POINT('Ctrl Pts',(0.2103257315894,2.34418240060269,10.8040228470717));
#67048=CARTESIAN_POINT('Ctrl Pts',(0.20924193374412,2.34511075668446,10.8041099048132));
#67049=CARTESIAN_POINT('Ctrl Pts',(0.208829069788589,2.34546260302739,10.8041430399556));
#67050=CARTESIAN_POINT('Ctrl Pts',(0.208037002557996,2.34613416504979,10.8042065548076));
#67051=CARTESIAN_POINT('Ctrl Pts',(0.20765794534745,2.34645405123024,10.8042369274126));
#67052=CARTESIAN_POINT('Ctrl Pts',(0.206982296850754,2.34702156525532,10.8042910238912));
#67053=CARTESIAN_POINT('Ctrl Pts',(0.206685995220396,2.34726953772846,10.8043147336184));
#67054=CARTESIAN_POINT('Ctrl Pts',(0.206098948599138,2.34775903995795,10.8043616812232));
#67055=CARTESIAN_POINT('Ctrl Pts',(0.205808223139834,2.34800059229907,10.8043849181289));
#67056=CARTESIAN_POINT('Ctrl Pts',(0.205104635561037,2.34858308629771,10.8044411226769));
#67057=CARTESIAN_POINT('Ctrl Pts',(0.204691348444434,2.34892351071844,10.804474111242));
#67058=CARTESIAN_POINT('Ctrl Pts',(0.203160106725728,2.35017840181598,10.8045962407549));
#67059=CARTESIAN_POINT('Ctrl Pts',(0.202036869694835,2.35108636935311,10.8046856436219));
#67060=CARTESIAN_POINT('Ctrl Pts',(0.183212918503481,2.36609459736832,10.8061809839103));
#67061=CARTESIAN_POINT('Ctrl Pts',(0.164085273225239,2.37829651302239,10.8076644148569));
#67062=CARTESIAN_POINT('Ctrl Pts',(0.13053103940573,2.39503232310662,10.8101881365517));
#67063=CARTESIAN_POINT('Ctrl Pts',(0.116776874677528,2.40074172530887,10.8112014203117));
#67064=CARTESIAN_POINT('Ctrl Pts',(0.0943347948087751,2.40828491315693,
10.8127862245283));
#67065=CARTESIAN_POINT('Ctrl Pts',(0.0858799204869176,2.41074636828859,
10.8133683030458));
#67066=CARTESIAN_POINT('Ctrl Pts',(0.0734880712214339,2.41380945811665,
10.8141904316879));
#67067=CARTESIAN_POINT('Ctrl Pts',(0.0696244618758618,2.41468922841304,
10.8144424608387));
#67068=CARTESIAN_POINT('Ctrl Pts',(0.065215004831091,2.41560809923774,10.8147244750418));
#67069=CARTESIAN_POINT('Ctrl Pts',(0.0646843278196683,2.41571728952382,
10.8147583232459));
#67070=CARTESIAN_POINT('Ctrl Pts',(0.0638852701128547,2.41587960164093,
10.8148091483914));
#67071=CARTESIAN_POINT('Ctrl Pts',(0.0636170963927311,2.41593372013465,
10.8148261820332));
#67072=CARTESIAN_POINT('Ctrl Pts',(0.0631366636616038,2.41603003680119,
10.814856654556));
#67073=CARTESIAN_POINT('Ctrl Pts',(0.0629244314745457,2.41607236257451,
10.8148701007417));
#67074=CARTESIAN_POINT('Ctrl Pts',(0.0624672025695226,2.41616306961944,
10.8148990363215));
#67075=CARTESIAN_POINT('Ctrl Pts',(0.0622221929196218,2.41621137977204,
10.8149145215638));
#67076=CARTESIAN_POINT('Ctrl Pts',(0.0615650924013758,2.41634015128421,
10.8149559986977));
#67077=CARTESIAN_POINT('Ctrl Pts',(0.0611528982619297,2.4164200925286,10.8149819607921));
#67078=CARTESIAN_POINT('Ctrl Pts',(0.0592829254556997,2.41677896597784,
10.8150994913233));
#67079=CARTESIAN_POINT('Ctrl Pts',(0.0578233566397278,2.41704863690329,
10.8151905390028));
#67080=CARTESIAN_POINT('Ctrl Pts',(0.0265580188201806,2.42260214956994,
10.8171271643803));
#67081=CARTESIAN_POINT('Ctrl Pts',(-0.00384872525162251,2.4236716980109,
10.8187548963342));
#67082=CARTESIAN_POINT('Ctrl Pts',(-0.0530840573723664,2.41845409433168,
10.8215490266969));
#67083=CARTESIAN_POINT('Ctrl Pts',(-0.0719831599756393,2.41472080240122,
10.822659071048));
#67084=CARTESIAN_POINT('Ctrl Pts',(-0.091524759306847,2.40900757677434,
10.8238972788867));
#67085=CARTESIAN_POINT('Ctrl Pts',(-0.0926125469361866,2.40868330076067,
10.8239664970896));
#67086=CARTESIAN_POINT('Ctrl Pts',(-0.0941994387379478,2.40820109568343,
10.8240679109315));
#67087=CARTESIAN_POINT('Ctrl Pts',(-0.094699915616857,2.40804768399724,
10.8240999586601));
#67088=CARTESIAN_POINT('Ctrl Pts',(-0.0955784662769301,2.40777603761185,
10.8241563288398));
#67089=CARTESIAN_POINT('Ctrl Pts',(-0.09595670094703,2.40765832360753,10.824180634172));
#67090=CARTESIAN_POINT('Ctrl Pts',(-0.0966913457913917,2.40742820127332,
10.8242279142929));
#67091=CARTESIAN_POINT('Ctrl Pts',(-0.0970477795345313,2.4073158697085,
10.8242508865286));
#67092=CARTESIAN_POINT('Ctrl Pts',(-0.0979975577110319,2.40701472605729,
10.8243121882635));
#67093=CARTESIAN_POINT('Ctrl Pts',(-0.0985905494928701,2.40682481463428,
10.8243505538678));
#67094=CARTESIAN_POINT('Ctrl Pts',(-0.100714310377563,2.40613786700255,
10.8244882904055));
#67095=CARTESIAN_POINT('Ctrl Pts',(-0.102241882122486,2.40563109023276,
10.8245879818237));
#67096=CARTESIAN_POINT('Ctrl Pts',(-0.127946706426711,2.39688915963633,
10.8262761910808));
#67097=CARTESIAN_POINT('Ctrl Pts',(-0.151059162560088,2.38582184079047,
10.8279651261308));
#67098=CARTESIAN_POINT('Ctrl Pts',(-0.184131832636683,2.36484433623847,
10.8306116114405));
#67099=CARTESIAN_POINT('Ctrl Pts',(-0.195170152865896,2.35681838654928,
10.8315382837865));
#67100=CARTESIAN_POINT('Ctrl Pts',(-0.210789316526204,2.34387148828902,
10.8328885251643));
#67101=CARTESIAN_POINT('Ctrl Pts',(-0.215779104269205,2.33946780280964,
10.8333263034291));
#67102=CARTESIAN_POINT('Ctrl Pts',(-0.223697172863672,2.332031171653,10.8340270430967));
#67103=CARTESIAN_POINT('Ctrl Pts',(-0.226708509838199,2.32908981985936,
10.8342950598146));
#67104=CARTESIAN_POINT('Ctrl Pts',(-0.230046852423466,2.32569874386905,
10.8345930303718));
#67105=CARTESIAN_POINT('Ctrl Pts',(-0.230431173545317,2.32530635047225,
10.834627346729));
#67106=CARTESIAN_POINT('Ctrl Pts',(-0.23100648633209,2.3247159419805,10.8346787337311));
#67107=CARTESIAN_POINT('Ctrl Pts',(-0.231198228158653,2.32451866426945,
10.8346958629541));
#67108=CARTESIAN_POINT('Ctrl Pts',(-0.23152743898233,2.3241790796921,10.8347252774116));
#67109=CARTESIAN_POINT('Ctrl Pts',(-0.231665029448718,2.32403689183852,
10.8347375722316));
#67110=CARTESIAN_POINT('Ctrl Pts',(-0.231949932871431,2.32374192568121,
10.8347630333303));
#67111=CARTESIAN_POINT('Ctrl Pts',(-0.232097225443932,2.32358912900327,
10.834776198015));
#67112=CARTESIAN_POINT('Ctrl Pts',(-0.232499656477737,2.32317083354989,
10.8348121709493));
#67113=CARTESIAN_POINT('Ctrl Pts',(-0.232754492031633,2.3229050417822,10.8348349554606));
#67114=CARTESIAN_POINT('Ctrl Pts',(-0.23372454376118,2.3218898070262,10.8349217083476));
#67115=CARTESIAN_POINT('Ctrl Pts',(-0.23443661033113,2.32113734334974,10.8349854347236));
#67116=CARTESIAN_POINT('Ctrl Pts',(-0.247795835104529,2.30688316912171,
10.8361821808254));
#67117=CARTESIAN_POINT('Ctrl Pts',(-0.259262987732564,2.29231833894362,
10.8372301352378));
#67118=CARTESIAN_POINT('Ctrl Pts',(-0.278643658436492,2.26279292648151,
10.8392101534994));
#67119=CARTESIAN_POINT('Ctrl Pts',(-0.286755077178749,2.24803827813328,
10.8401414151025));
#67120=CARTESIAN_POINT('Ctrl Pts',(-0.299756742200531,2.21926828385461,
10.8419457599582));
#67121=CARTESIAN_POINT('Ctrl Pts',(-0.304903156312032,2.20541823329652,
10.8428097187293));
#67122=CARTESIAN_POINT('Ctrl Pts',(-0.309394616577889,2.19020734037224,
10.8437745034147));
#67123=CARTESIAN_POINT('Ctrl Pts',(-0.309701638749541,2.18914756268587,
10.8438417966249));
#67124=CARTESIAN_POINT('Ctrl Pts',(-0.310144633697823,2.18758852399087,
10.8439409079549));
#67125=CARTESIAN_POINT('Ctrl Pts',(-0.310284858175825,2.18709047093874,
10.8439725876028));
#67126=CARTESIAN_POINT('Ctrl Pts',(-0.310530075467895,2.18621139170129,
10.8440285346253));
#67127=CARTESIAN_POINT('Ctrl Pts',(-0.310635568186558,2.18583050509191,
10.8440527856941));
#67128=CARTESIAN_POINT('Ctrl Pts',(-0.310839950692917,2.18508725969011,
10.8441001288166));
#67129=CARTESIAN_POINT('Ctrl Pts',(-0.310938908203602,2.18472492001555,
10.844123218628));
#67130=CARTESIAN_POINT('Ctrl Pts',(-0.311202776233992,2.18375206039317,
10.844185239422));
#67131=CARTESIAN_POINT('Ctrl Pts',(-0.311366522910841,2.18314122898511,
10.8442242080835));
#67132=CARTESIAN_POINT('Ctrl Pts',(-0.311956201487708,2.18091534947454,
10.8443663133828));
#67133=CARTESIAN_POINT('Ctrl Pts',(-0.312371368305348,2.17929750009675,
10.8444697977315));
#67134=CARTESIAN_POINT('Ctrl Pts',(-0.319109652835105,2.15216497995407,
10.8462087973236));
#67135=CARTESIAN_POINT('Ctrl Pts',(-0.322298967491384,2.12597977636967,
10.8479511623769));
#67136=CARTESIAN_POINT('Ctrl Pts',(-0.322261340588192,2.08496170084742,
10.8507246764572));
#67137=CARTESIAN_POINT('Ctrl Pts',(-0.321236218004765,2.07023679775949,
10.8517263176096));
#67138=CARTESIAN_POINT('Ctrl Pts',(-0.318013606332761,2.04705094368035,
10.8532730678785));
#67139=CARTESIAN_POINT('Ctrl Pts',(-0.316474955975911,2.03851918886136,
10.8538353008064));
#67140=CARTESIAN_POINT('Ctrl Pts',(-0.31444002312565,2.02936607487704,10.8544236901166));
#67141=CARTESIAN_POINT('Ctrl Pts',(-0.314283677364257,2.02867363960958,
10.8544681089694));
#67142=CARTESIAN_POINT('Ctrl Pts',(-0.314061830390749,2.02770600071265,
10.8545300462583));
#67143=CARTESIAN_POINT('Ctrl Pts',(-0.313998254241525,2.02743036464106,
10.8545476739591));
#67144=CARTESIAN_POINT('Ctrl Pts',(-0.313887691233006,2.02695388125218,
10.8545781193426));
#67145=CARTESIAN_POINT('Ctrl Pts',(-0.313840874447394,2.02675299529436,
10.8545909468267));
#67146=CARTESIAN_POINT('Ctrl Pts',(-0.313743037445857,2.02633500276789,
10.854617620023));
#67147=CARTESIAN_POINT('Ctrl Pts',(-0.313691984790493,2.0261179044596,10.8546314637561));
#67148=CARTESIAN_POINT('Ctrl Pts',(-0.313570175067326,2.02560231835343,
10.8546643180725));
#67149=CARTESIAN_POINT('Ctrl Pts',(-0.313499216860585,2.02530387723714,
10.854683317005));
#67150=CARTESIAN_POINT('Ctrl Pts',(-0.313261068712301,2.02430857365992,
10.8547466185388));
#67151=CARTESIAN_POINT('Ctrl Pts',(-0.313091978983786,2.02361216123397,
10.8547908122397));
#67152=CARTESIAN_POINT('Ctrl Pts',(-0.310092295551753,2.01143497243676,
10.8555619368634));
#67153=CARTESIAN_POINT('Ctrl Pts',(-0.306633895325478,2.00011645781304,
10.856253425238));
#67154=CARTESIAN_POINT('Ctrl Pts',(-0.292518746355445,1.96163749784622,
10.8585962757962));
#67155=CARTESIAN_POINT('Ctrl Pts',(-0.27880864834607,1.93575243663756,10.8601708704603));
#67156=CARTESIAN_POINT('Ctrl Pts',(-0.256261597751206,1.90434346911651,
10.8624234177236));
#67157=CARTESIAN_POINT('Ctrl Pts',(-0.250381539066271,1.8968730875613,10.8629877131863));
#67158=CARTESIAN_POINT('Ctrl Pts',(-0.243431566881132,1.88880443984327,
10.8636353048508));
#67159=CARTESIAN_POINT('Ctrl Pts',(-0.242678043332475,1.88793901911214,
10.8637052752765));
#67160=CARTESIAN_POINT('Ctrl Pts',(-0.241576291273093,1.88668722111408,
10.8638072395696));
#67161=CARTESIAN_POINT('Ctrl Pts',(-0.241231718005775,1.8862976266761,10.8638390808942));
#67162=CARTESIAN_POINT('Ctrl Pts',(-0.240622451104511,1.88561210555517,
10.8638952983856));
#67163=CARTESIAN_POINT('Ctrl Pts',(-0.240358150248578,1.88531582995742,
10.8639196580485));
#67164=CARTESIAN_POINT('Ctrl Pts',(-0.239811078399718,1.88470485072827,
10.863970023294));
#67165=CARTESIAN_POINT('Ctrl Pts',(-0.239528233964862,1.88439021415036,
10.8639960319446));
#67166=CARTESIAN_POINT('Ctrl Pts',(-0.238803526882096,1.88358723490584,
10.8640625932487));
#67167=CARTESIAN_POINT('Ctrl Pts',(-0.238360786972351,1.88309968978662,
10.8641031829652));
#67168=CARTESIAN_POINT('Ctrl Pts',(-0.23655494989471,1.88112330874004,10.8642684425734));
#67169=CARTESIAN_POINT('Ctrl Pts',(-0.235179396245872,1.87964596309556,
10.8643936420003));
#67170=CARTESIAN_POINT('Ctrl Pts',(-0.212496239219926,1.85573857485373,
10.8664474989823));
#67171=CARTESIAN_POINT('Ctrl Pts',(-0.188086092579508,1.83648340023354,
10.8685289412811));
#67172=CARTESIAN_POINT('Ctrl Pts',(-0.145843842433668,1.81205871572784,
10.8718279115494));
#67173=CARTESIAN_POINT('Ctrl Pts',(-0.129651809717556,1.80441382868556,
10.8730280100167));
#67174=CARTESIAN_POINT('Ctrl Pts',(-0.111895017570926,1.79777185905241,
10.8742223714685));
#67175=CARTESIAN_POINT('Ctrl Pts',(-0.110880635296253,1.79739823375761,
10.8742901895303));
#67176=CARTESIAN_POINT('Ctrl Pts',(-0.109512171682685,1.79690199565565,
10.8743811085517));
#67177=CARTESIAN_POINT('Ctrl Pts',(-0.109159743472639,1.79677489155321,
10.8744044725445));
#67178=CARTESIAN_POINT('Ctrl Pts',(-0.108606114174695,1.79657631407934,
10.8744410942665));
#67179=CARTESIAN_POINT('Ctrl Pts',(-0.108405063751985,1.79650442611567,
10.8744543767429));
#67180=CARTESIAN_POINT('Ctrl Pts',(-0.108017925339663,1.79636643395622,
10.8744799208599));
#67181=CARTESIAN_POINT('Ctrl Pts',(-0.107831849433781,1.79630030149659,
10.8744921841024));
#67182=CARTESIAN_POINT('Ctrl Pts',(-0.107389166940257,1.79614342770171,
10.8745213248039));
#67183=CARTESIAN_POINT('Ctrl Pts',(-0.107132506356514,1.79605284046718,
10.8745381929596));
#67184=CARTESIAN_POINT('Ctrl Pts',(-0.106371022967843,1.79578516258503,
10.874588159191));
#67185=CARTESIAN_POINT('Ctrl Pts',(-0.105865870471747,1.79560900258117,
10.874621201971));
#67186=CARTESIAN_POINT('Ctrl Pts',(-0.101813268529822,1.79420706210006,
10.8748854751099));
#67187=CARTESIAN_POINT('Ctrl Pts',(-0.0982449064654422,1.79304201614351,
10.8751131793803));
#67188=CARTESIAN_POINT('Ctrl Pts',(-0.0852828923600123,1.78905921700752,
10.8759251296168));
#67189=CARTESIAN_POINT('Ctrl Pts',(-0.0757815139115759,1.78660801116049,
10.8764918455314));
#67190=CARTESIAN_POINT('Ctrl Pts',(-0.0352192502788053,1.77809674492801,
10.8788479777394));
#67191=CARTESIAN_POINT('Ctrl Pts',(-0.00347017465484709,1.77619431317332,
10.8805571999396));
#67192=CARTESIAN_POINT('Ctrl Pts',(0.0288798137658721,1.77902051645085,
10.8824813382952));
#67193=CARTESIAN_POINT('Ctrl Pts',(0.0297111471255038,1.77909640042432,
10.8825308945931));
#67194=CARTESIAN_POINT('Ctrl Pts',(0.0355616695097354,1.77965336431316,
10.882880441744));
#67195=CARTESIAN_POINT('Ctrl Pts',(0.040569032653257,1.78024892712483,10.8831837450786));
#67196=CARTESIAN_POINT('Ctrl Pts',(0.0464111151192779,1.78108320378603,
10.8835431284651));
#67197=CARTESIAN_POINT('Ctrl Pts',(0.0472615724770881,1.78120812705068,
10.8835955825203));
#67198=CARTESIAN_POINT('Ctrl Pts',(0.0486211417301354,1.78141339349703,
10.8836796602766));
#67199=CARTESIAN_POINT('Ctrl Pts',(0.0491305823272808,1.78149155875938,
10.8837112149715));
#67200=CARTESIAN_POINT('Ctrl Pts',(0.0500313645639767,1.78163198149173,
10.8837670988584));
#67201=CARTESIAN_POINT('Ctrl Pts',(0.0504227839274482,1.78169373944612,
10.8837914121679));
#67202=CARTESIAN_POINT('Ctrl Pts',(0.0512337911253736,1.78182323322659,
10.8838418509587));
#67203=CARTESIAN_POINT('Ctrl Pts',(0.0516533606498985,1.78189107746202,
10.8838679798364));
#67204=CARTESIAN_POINT('Ctrl Pts',(0.0527313552383046,1.78206757773024,
10.8839352021998));
#67205=CARTESIAN_POINT('Ctrl Pts',(0.0533895768346469,1.782177448833,10.8839763341998));
#67206=CARTESIAN_POINT('Ctrl Pts',(0.0561081615480556,1.78263992175687,
10.8841465771644));
#67207=CARTESIAN_POINT('Ctrl Pts',(0.058165374948528,1.78301051455767,10.8842762587965));
#67208=CARTESIAN_POINT('Ctrl Pts',(0.0719027439351294,1.78562343530252,
10.8851481079116));
#67209=CARTESIAN_POINT('Ctrl Pts',(0.0834533185927601,1.78849058779111,
10.8859101941257));
#67210=CARTESIAN_POINT('Ctrl Pts',(0.128326777924193,1.80230441663914,10.888988199625));
#67211=CARTESIAN_POINT('Ctrl Pts',(0.159922118083132,1.8180161936087,10.8914480006426));
#67212=CARTESIAN_POINT('Ctrl Pts',(0.190235096140064,1.8398517811264,10.8938322911741));
#67213=CARTESIAN_POINT('Ctrl Pts',(0.192090755508233,1.84121895363696,10.8939782256543));
#67214=CARTESIAN_POINT('Ctrl Pts',(0.194489892606779,1.84302656588351,10.894166698071));
#67215=CARTESIAN_POINT('Ctrl Pts',(0.195046771873976,1.84344898953423,10.8942104311826));
#67216=CARTESIAN_POINT('Ctrl Pts',(0.195825597072403,1.8440437730517,10.8942715687392));
#67217=CARTESIAN_POINT('Ctrl Pts',(0.196048693471399,1.84421461266912,10.8942890787938));
#67218=CARTESIAN_POINT('Ctrl Pts',(0.196434784587293,1.84451106995502,10.8943193761975));
#67219=CARTESIAN_POINT('Ctrl Pts',(0.196597882464655,1.84463655198454,10.8943321731249));
#67220=CARTESIAN_POINT('Ctrl Pts',(0.196934062000048,1.84489571019799,10.8943585465853));
#67221=CARTESIAN_POINT('Ctrl Pts',(0.19710712760593,1.84502940620839,10.8943721215994));
#67222=CARTESIAN_POINT('Ctrl Pts',(0.197516812198245,1.84534656065699,10.8944042520772));
#67223=CARTESIAN_POINT('Ctrl Pts',(0.197753312654186,1.84553017348571,10.8944227965578));
#67224=CARTESIAN_POINT('Ctrl Pts',(0.198254369210672,1.84592030118297,10.8944620785442));
#67225=CARTESIAN_POINT('Ctrl Pts',(0.198518859564754,1.84612690047666,10.8944828100633));
#67226=CARTESIAN_POINT('Ctrl Pts',(0.199235655516072,1.84668861084085,10.8945389850039));
#67227=CARTESIAN_POINT('Ctrl Pts',(0.199687336793267,1.84704452201451,10.8945743726409));
#67228=CARTESIAN_POINT('Ctrl Pts',(0.212941385742961,1.85754593529842,10.8956125547702));
#67229=CARTESIAN_POINT('Ctrl Pts',(0.224956979001012,1.86865063590422,10.8965480141698));
#67230=CARTESIAN_POINT('Ctrl Pts',(0.253256335860199,1.89910428734379,10.8988893224661));
#67231=CARTESIAN_POINT('Ctrl Pts',(0.268201510462072,1.91954012300735,10.9002722466885));
#67232=CARTESIAN_POINT('Ctrl Pts',(0.281774268365464,1.94357097186685,10.9018853522377));
#67233=CARTESIAN_POINT('Ctrl Pts',(0.282915646310602,1.94564483865028,10.9020243886057));
#67234=CARTESIAN_POINT('Ctrl Pts',(0.287118611846333,1.95348481774788,10.9025496488998));
#67235=CARTESIAN_POINT('Ctrl Pts',(0.290027441447156,1.95933063614475,10.9029406451016));
#67236=CARTESIAN_POINT('Ctrl Pts',(0.29318905587905,1.96620006347498,10.9034008851928));
#67237=CARTESIAN_POINT('Ctrl Pts',(0.293616975175867,1.96714173962145,10.9034639914284));
#67238=CARTESIAN_POINT('Ctrl Pts',(0.294246618215615,1.96854522741762,10.903558074788));
#67239=CARTESIAN_POINT('Ctrl Pts',(0.294451806911116,1.9690054849689,10.9035889329338));
#67240=CARTESIAN_POINT('Ctrl Pts',(0.294815262256672,1.96982591832359,10.903643948146));
#67241=CARTESIAN_POINT('Ctrl Pts',(0.2949739508228,1.97018590703018,10.9036680907075));
#67242=CARTESIAN_POINT('Ctrl Pts',(0.295306543653845,1.97094416031045,10.9037189496296));
#67243=CARTESIAN_POINT('Ctrl Pts',(0.295480302190845,1.97134248759977,10.9037456709116));
#67244=CARTESIAN_POINT('Ctrl Pts',(0.295935884318789,1.97239266349623,10.9038161317182));
#67245=CARTESIAN_POINT('Ctrl Pts',(0.296216358738336,1.97304509162687,10.9038599171535));
#67246=CARTESIAN_POINT('Ctrl Pts',(0.297464574525642,1.97597529552459,10.9040566224848));
#67247=CARTESIAN_POINT('Ctrl Pts',(0.298408194869985,1.97826319741798,10.9042103593725));
#67248=CARTESIAN_POINT('Ctrl Pts',(0.305145194551675,1.99514684885435,10.9053462226367));
#67249=CARTESIAN_POINT('Ctrl Pts',(0.309890359206995,2.01013561618187,10.9063635876285));
#67250=CARTESIAN_POINT('Ctrl Pts',(0.319342784572609,2.04986621749384,10.9090776630549));
#67251=CARTESIAN_POINT('Ctrl Pts',(0.322279455761842,2.07491881408578,10.9108109894218));
#67252=CARTESIAN_POINT('Ctrl Pts',(0.322273592482529,2.10796044840965,10.9129869508134));
#67253=CARTESIAN_POINT('Ctrl Pts',(0.321981467241188,2.11586179408585,10.9134982412682));
#67254=CARTESIAN_POINT('Ctrl Pts',(0.321347810561823,2.12443857123039,10.9140378168913));
#67255=CARTESIAN_POINT('Ctrl Pts',(0.321294333757685,2.12513185693778,10.91408132207));
#67256=CARTESIAN_POINT('Ctrl Pts',(0.321216146366285,2.12610443531726,10.9141421935344));
#67257=CARTESIAN_POINT('Ctrl Pts',(0.321193314990505,2.12638387076451,10.9141596642279));
#67258=CARTESIAN_POINT('Ctrl Pts',(0.321153106963466,2.12686819295285,10.9141899121766));
#67259=CARTESIAN_POINT('Ctrl Pts',(0.321135898874397,2.12707309290631,10.9142026989355));
#67260=CARTESIAN_POINT('Ctrl Pts',(0.321099968102112,2.12749607278979,10.9142290738959));
#67261=CARTESIAN_POINT('Ctrl Pts',(0.321081219364787,2.12771414991567,10.9142426605403));
#67262=CARTESIAN_POINT('Ctrl Pts',(0.321036260027539,2.12823092774375,10.9142748297268));
#67263=CARTESIAN_POINT('Ctrl Pts',(0.321009854612441,2.12852961228594,10.9142934012386));
#67264=CARTESIAN_POINT('Ctrl Pts',(0.320952934379791,2.12916338027077,10.9143327627248));
#67265=CARTESIAN_POINT('Ctrl Pts',(0.320922311548323,2.12949845400558,10.9143535466324));
#67266=CARTESIAN_POINT('Ctrl Pts',(0.320837736757134,2.13040814681732,10.9144099023265));
#67267=CARTESIAN_POINT('Ctrl Pts',(0.320782765574531,2.13098267326406,10.9144454178637));
#67268=CARTESIAN_POINT('Ctrl Pts',(0.320606908573613,2.13276997433638,10.91455567401));
#67269=CARTESIAN_POINT('Ctrl Pts',(0.320480684622271,2.13398222968042,10.9146301273247));
#67270=CARTESIAN_POINT('Ctrl Pts',(0.319454339014239,2.14332443472775,10.9152015612954));
#67271=CARTESIAN_POINT('Ctrl Pts',(0.318251788945937,2.15141891176627,10.9156830338338));
#67272=CARTESIAN_POINT('Ctrl Pts',(0.313730137988612,2.17550585337633,10.9170979416891));
#67273=CARTESIAN_POINT('Ctrl Pts',(0.309502699192559,2.19130102853537,10.9180028538564));
#67274=CARTESIAN_POINT('Ctrl Pts',(0.299047824853666,2.22109514109726,10.9197697354791));
#67275=CARTESIAN_POINT('Ctrl Pts',(0.292985262477462,2.23510446761896,10.9206284530444));
#67276=CARTESIAN_POINT('Ctrl Pts',(0.281663860477681,2.25688592850269,10.9220598444195));
#67277=CARTESIAN_POINT('Ctrl Pts',(0.27701823389186,2.26495028832841,10.9226125870655));
#67278=CARTESIAN_POINT('Ctrl Pts',(0.271418718418372,2.27376523640135,10.923247673354));
#67279=CARTESIAN_POINT('Ctrl Pts',(0.270801677535746,2.27472529719778,10.9233172650414));
#67280=CARTESIAN_POINT('Ctrl Pts',(0.26989665885054,2.27611711580354,10.9234187781613));
#67281=CARTESIAN_POINT('Ctrl Pts',(0.269612712191117,2.27655149491753,10.9234505489591));
#67282=CARTESIAN_POINT('Ctrl Pts',(0.269109784217348,2.27731682702414,10.9235066841963));
#67283=CARTESIAN_POINT('Ctrl Pts',(0.268891237945403,2.27764806574058,10.923531032285));
#67284=CARTESIAN_POINT('Ctrl Pts',(0.268438173528964,2.27833199940078,10.9235814147865));
#67285=CARTESIAN_POINT('Ctrl Pts',(0.268203570893212,2.27868463721106,10.9236074523469));
#67286=CARTESIAN_POINT('Ctrl Pts',(0.267601237897133,2.27958616206266,10.923674172798));
#67287=CARTESIAN_POINT('Ctrl Pts',(0.267232514896873,2.28013438067171,10.9237148930991));
#67288=CARTESIAN_POINT('Ctrl Pts',(0.265720830930905,2.28236710105095,10.9238813405545));
#67289=CARTESIAN_POINT('Ctrl Pts',(0.264563627137085,2.28404186052861,10.9240076068985));
#67290=CARTESIAN_POINT('Ctrl Pts',(0.256825522724552,2.29501700255983,10.924844591866));
#67291=CARTESIAN_POINT('Ctrl Pts',(0.249771992862943,2.30397274367543,10.9255735559959));
#67292=CARTESIAN_POINT('Ctrl Pts',(0.239105141218199,2.31613141821105,10.9266317562559));
#67293=CARTESIAN_POINT('Ctrl Pts',(0.235870867762312,2.31965652538539,10.9269473918592));
#67294=CARTESIAN_POINT('Ctrl Pts',(0.21283791635488,2.34366518889734,10.9291580803373));
#67295=CARTESIAN_POINT('Ctrl Pts',(0.190479444856319,2.36151517768232,10.9311336135066));
#67296=CARTESIAN_POINT('Ctrl Pts',(0.165772275101214,2.37637084979726,10.9330007166504));
#67297=CARTESIAN_POINT('Ctrl Pts',(0.165477366585806,2.37654752748797,10.9330229590571));
#67298=CARTESIAN_POINT('Ctrl Pts',(0.16465254870239,2.37703987850495,10.9330850450253));
#67299=CARTESIAN_POINT('Ctrl Pts',(0.164122012053392,2.37735450464635,10.9331248382677));
#67300=CARTESIAN_POINT('Ctrl Pts',(0.160271490278829,2.37962307699123,10.9334126080442));
#67301=CARTESIAN_POINT('Ctrl Pts',(0.156917427912352,2.3815189866872,10.933657681958));
#67302=CARTESIAN_POINT('Ctrl Pts',(0.153013637944836,2.38363417835583,10.9339358398401));
#67303=CARTESIAN_POINT('Ctrl Pts',(0.152496509678359,2.38391254829179,10.9339725454677));
#67304=CARTESIAN_POINT('Ctrl Pts',(0.151731962159788,2.38432141235384,10.9340266010447));
#67305=CARTESIAN_POINT('Ctrl Pts',(0.151485133033698,2.38445299846359,10.9340440200348));
#67306=CARTESIAN_POINT('Ctrl Pts',(0.15105061491398,2.38468391674351,10.9340746268837));
#67307=CARTESIAN_POINT('Ctrl Pts',(0.150862998977748,2.38478338480114,10.934087823434));
#67308=CARTESIAN_POINT('Ctrl Pts',(0.150466061533849,2.3849933261858,10.9341157032804));
#67309=CARTESIAN_POINT('Ctrl Pts',(0.150256717099342,2.38510375411654,10.9341303836514));
#67310=CARTESIAN_POINT('Ctrl Pts',(0.149710045158083,2.38539135092291,10.9341686586376));
#67311=CARTESIAN_POINT('Ctrl Pts',(0.149372523518038,2.38556815302874,10.9341922298953));
#67312=CARTESIAN_POINT('Ctrl Pts',(0.148633746319999,2.38595347447336,10.9342436936415));
#67313=CARTESIAN_POINT('Ctrl Pts',(0.148232363050393,2.38616174911893,10.9342715708207));
#67314=CARTESIAN_POINT('Ctrl Pts',(0.147054897629151,2.3867695846028,10.9343531086353));
#67315=CARTESIAN_POINT('Ctrl Pts',(0.146277621545877,2.38716684182743,10.934406628531));
#67316=CARTESIAN_POINT('Ctrl Pts',(0.143590535186885,2.388526441128,10.9345906314389));
#67317=CARTESIAN_POINT('Ctrl Pts',(0.141672719740869,2.38947295219074,10.9347201892511));
#67318=CARTESIAN_POINT('Ctrl Pts',(0.133607087817728,2.39335427117415,10.935258287291));
#67319=CARTESIAN_POINT('Ctrl Pts',(0.127376041355683,2.39611305215611,10.935657659415));
#67320=CARTESIAN_POINT('Ctrl Pts',(0.105820504938987,2.4048502236292,10.9369995364899));
#67321=CARTESIAN_POINT('Ctrl Pts',(0.0901277915379695,2.40985268145701,
10.9379105683123));
#67322=CARTESIAN_POINT('Ctrl Pts',(0.0585939231336889,2.41730503161373,
10.939724164058));
#67323=CARTESIAN_POINT('Ctrl Pts',(0.0428168215292512,2.41981617630719,
10.9406238840494));
#67324=CARTESIAN_POINT('Ctrl Pts',(0.0250778754289856,2.42130311589696,
10.9416660801061));
#67325=CARTESIAN_POINT('Ctrl Pts',(0.0232346903394261,2.42144166048897,
10.9417747160147));
#67326=CARTESIAN_POINT('Ctrl Pts',(0.0147657889760138,2.42200501129435,
10.9422756274501));
#67327=CARTESIAN_POINT('Ctrl Pts',(0.00812950234340606,2.4222408375359,
10.9426731362181));
#67328=CARTESIAN_POINT('Ctrl Pts',(0.000451560457815039,2.42227635996316,
10.9431404158847));
#67329=CARTESIAN_POINT('Ctrl Pts',(-0.000587893916345153,2.42227614003989,
10.9432038322062));
#67330=CARTESIAN_POINT('Ctrl Pts',(-0.00213225426868554,2.42226834173135,
10.9432982888775));
#67331=CARTESIAN_POINT('Ctrl Pts',(-0.0026371799767455,2.42226460535982,
10.9433292088539));
#67332=CARTESIAN_POINT('Ctrl Pts',(-0.00353561351639392,2.42225584546371,
10.9433842935171));
#67333=CARTESIAN_POINT('Ctrl Pts',(-0.00392912572336737,2.42225128776676,
10.9434084435639));
#67334=CARTESIAN_POINT('Ctrl Pts',(-0.0047566259865352,2.42224018762881,
10.9434592765997));
#67335=CARTESIAN_POINT('Ctrl Pts',(-0.00519061085343672,2.42223348921219,
10.9434859644275));
#67336=CARTESIAN_POINT('Ctrl Pts',(-0.0063322228811744,2.42221356192837,
10.9435562427709));
#67337=CARTESIAN_POINT('Ctrl Pts',(-0.00703981941321461,2.42219887874889,
10.9435998787676));
#67338=CARTESIAN_POINT('Ctrl Pts',(-0.0101982263588391,2.42212293000704,
10.9437949945642));
#67339=CARTESIAN_POINT('Ctrl Pts',(-0.012648286661351,2.4220360324057,10.9439472752221));
#67340=CARTESIAN_POINT('Ctrl Pts',(-0.0305337345986822,2.42119726268091,
10.9450659315417));
#67341=CARTESIAN_POINT('Ctrl Pts',(-0.0458959992238623,2.41936409121903,
10.946066397893));
#67342=CARTESIAN_POINT('Ctrl Pts',(-0.0645551773513158,2.41576325716946,
10.9473283150609));
#67343=CARTESIAN_POINT('Ctrl Pts',(-0.0680331992839133,2.41503220198344,
10.9475654933345));
#67344=CARTESIAN_POINT('Ctrl Pts',(-0.074307969169397,2.41360453432287,
10.9479966685379));
#67345=CARTESIAN_POINT('Ctrl Pts',(-0.0771088526425831,2.41292763168831,
10.9481903264274));
#67346=CARTESIAN_POINT('Ctrl Pts',(-0.08225352289581,2.41161103027343,10.9485480461931));
#67347=CARTESIAN_POINT('Ctrl Pts',(-0.0845998964871797,2.41098220780366,
10.9487119712565));
#67348=CARTESIAN_POINT('Ctrl Pts',(-0.088958974454173,2.40976100041126,
10.9490178211939));
#67349=CARTESIAN_POINT('Ctrl Pts',(-0.0909734478491825,2.40917536810437,
10.9491596906761));
#67350=CARTESIAN_POINT('Ctrl Pts',(-0.0947473084584657,2.40803818308583,
10.9494263536089));
#67351=CARTESIAN_POINT('Ctrl Pts',(-0.0965079658691028,2.40749111729511,
10.9495511287727));
#67352=CARTESIAN_POINT('Ctrl Pts',(-0.116662664991957,2.40103855624245,
10.9509832100453));
#67353=CARTESIAN_POINT('Ctrl Pts',(-0.134496813281154,2.39350497703906,
10.9522889214736));
#67354=CARTESIAN_POINT('Ctrl Pts',(-0.152971177015249,2.38366104242875,
10.9536141979254));
#67355=CARTESIAN_POINT('Ctrl Pts',(-0.154386468234403,2.38289324253364,
10.9537155263969));
#67356=CARTESIAN_POINT('Ctrl Pts',(-0.156175044295363,2.38190551373694,
10.9538432696754));
#67357=CARTESIAN_POINT('Ctrl Pts',(-0.156553688728325,2.38169541296712,
10.9538702953475));
#67358=CARTESIAN_POINT('Ctrl Pts',(-0.157152711796571,2.38136144850785,
10.9539130208945));
#67359=CARTESIAN_POINT('Ctrl Pts',(-0.157373368413679,2.38123808854179,
10.9539287529331));
#67360=CARTESIAN_POINT('Ctrl Pts',(-0.157783734795642,2.38100803552845,
10.9539579984019));
#67361=CARTESIAN_POINT('Ctrl Pts',(-0.157973480259551,2.38090141069915,
10.953971516037));
#67362=CARTESIAN_POINT('Ctrl Pts',(-0.158393747014589,2.38066468712013,
10.9540014454602));
#67363=CARTESIAN_POINT('Ctrl Pts',(-0.158624215498863,2.38053449689501,
10.9540178512001));
#67364=CARTESIAN_POINT('Ctrl Pts',(-0.159294454143511,2.38015479320819,
10.9540655416513));
#67365=CARTESIAN_POINT('Ctrl Pts',(-0.159733800374228,2.37990452712422,
10.9540967779604));
#67366=CARTESIAN_POINT('Ctrl Pts',(-0.160728233209435,2.37933496154287,
10.9541674266003));
#67367=CARTESIAN_POINT('Ctrl Pts',(-0.161282962752072,2.37901503836335,
10.9542067994757));
#67368=CARTESIAN_POINT('Ctrl Pts',(-0.163050744685599,2.37798849089676,
10.9543321632354));
#67369=CARTESIAN_POINT('Ctrl Pts',(-0.164260154428481,2.37727558176294,
10.9544177673243));
#67370=CARTESIAN_POINT('Ctrl Pts',(-0.16898370950396,2.37444944173226,10.9547516262125));
#67371=CARTESIAN_POINT('Ctrl Pts',(-0.172462205319981,2.37227703041422,
10.954996432063));
#67372=CARTESIAN_POINT('Ctrl Pts',(-0.181939370062623,2.36610377217654,
10.9556631878612));
#67373=CARTESIAN_POINT('Ctrl Pts',(-0.187846909062409,2.36196698860046,
10.9560785793407));
#67374=CARTESIAN_POINT('Ctrl Pts',(-0.219072103021601,2.33850148411132,
10.9583009966784));
#67375=CARTESIAN_POINT('Ctrl Pts',(-0.241555082508471,2.31570063702235,
10.960020041645));
#67376=CARTESIAN_POINT('Ctrl Pts',(-0.263772148334165,2.28525530336174,
10.9622529216656));
#67377=CARTESIAN_POINT('Ctrl Pts',(-0.267085267268975,2.28044591165535,
10.9626033508674));
#67378=CARTESIAN_POINT('Ctrl Pts',(-0.270803857736533,2.27472098350322,
10.9630189369418));
#67379=CARTESIAN_POINT('Ctrl Pts',(-0.271338133537857,2.27389010522579,
10.9630792141947));
#67380=CARTESIAN_POINT('Ctrl Pts',(-0.272137808888918,2.27263383207967,
10.9631703001465));
#67381=CARTESIAN_POINT('Ctrl Pts',(-0.272406052927599,2.27221024745726,
10.9632010032093));
#67382=CARTESIAN_POINT('Ctrl Pts',(-0.272882849420923,2.27145343581024,
10.9632558447674));
#67383=CARTESIAN_POINT('Ctrl Pts',(-0.273091783146859,2.27112044920089,
10.9632799690961));
#67384=CARTESIAN_POINT('Ctrl Pts',(-0.273531142866867,2.27041736875368,
10.9633308955763));
#67385=CARTESIAN_POINT('Ctrl Pts',(-0.273761428011194,2.27004718821927,
10.9633577028604));
#67386=CARTESIAN_POINT('Ctrl Pts',(-0.274368122860366,2.26906750710678,
10.9634286326884));
#67387=CARTESIAN_POINT('Ctrl Pts',(-0.274743251130419,2.26845721933555,
10.9634728022551));
#67388=CARTESIAN_POINT('Ctrl Pts',(-0.276436894559954,2.26568116365865,
10.9636736522902));
#67389=CARTESIAN_POINT('Ctrl Pts',(-0.277731827901016,2.26350117994996,
10.9638311926291));
#67390=CARTESIAN_POINT('Ctrl Pts',(-0.283275559870006,2.25391254579048,
10.9645235048124));
#67391=CARTESIAN_POINT('Ctrl Pts',(-0.287254297008239,2.24635252434112,
10.9650678601259));
#67392=CARTESIAN_POINT('Ctrl Pts',(-0.294913678652514,2.23028022388178,
10.9662228655744));
#67393=CARTESIAN_POINT('Ctrl Pts',(-0.298536681400055,2.2217490934837,10.9668347079274));
#67394=CARTESIAN_POINT('Ctrl Pts',(-0.310613646588465,2.1895165660611,10.969135254109));
#67395=CARTESIAN_POINT('Ctrl Pts',(-0.316651403064107,2.16500717140273,
10.9708704080542));
#67396=CARTESIAN_POINT('Ctrl Pts',(-0.319949542429548,2.13867022547181,
10.9725997397257));
#67397=CARTESIAN_POINT('Ctrl Pts',(-0.320112869977615,2.13729405635418,
10.9726896947713));
#67398=CARTESIAN_POINT('Ctrl Pts',(-0.320317146764235,2.13547253885684,
10.9728081870754));
#67399=CARTESIAN_POINT('Ctrl Pts',(-0.320366050795247,2.13502811765518,
10.9728370522035));
#67400=CARTESIAN_POINT('Ctrl Pts',(-0.320847886025833,2.13056395555407,
10.9731265370863));
#67401=CARTESIAN_POINT('Ctrl Pts',(-0.321206088488374,2.12653627360764,
10.9733839585624));
#67402=CARTESIAN_POINT('Ctrl Pts',(-0.321530009532216,2.12190852265042,
10.9736746182531));
#67403=CARTESIAN_POINT('Ctrl Pts',(-0.321569951881506,2.12131423127655,
10.973711847856));
#67404=CARTESIAN_POINT('Ctrl Pts',(-0.321626334010426,2.12043908122525,
10.9737665262981));
#67405=CARTESIAN_POINT('Ctrl Pts',(-0.321644053705415,2.12015831063642,
10.9737840464796));
#67406=CARTESIAN_POINT('Ctrl Pts',(-0.321674558231837,2.11966468110594,
10.9738148099156));
#67407=CARTESIAN_POINT('Ctrl Pts',(-0.321687499459502,2.11945183254085,
10.9738280620025));
#67408=CARTESIAN_POINT('Ctrl Pts',(-0.321712427713363,2.11903500018582,
10.973853989));
#67409=CARTESIAN_POINT('Ctrl Pts',(-0.321724431955575,2.11883101857893,
10.9738666648614));
#67410=CARTESIAN_POINT('Ctrl Pts',(-0.321749941839371,2.11839039780635,
10.97389402076));
#67411=CARTESIAN_POINT('Ctrl Pts',(-0.321763380448994,2.11815375465339,
10.9739086970079));
#67412=CARTESIAN_POINT('Ctrl Pts',(-0.321795326792112,2.11758002415924,
10.9739442412565));
#67413=CARTESIAN_POINT('Ctrl Pts',(-0.32181356600365,2.11724292124719,10.9739650942513));
#67414=CARTESIAN_POINT('Ctrl Pts',(-0.3218616962146,2.11632667843549,10.974021688422));
#67415=CARTESIAN_POINT('Ctrl Pts',(-0.321890553974519,2.11574748211461,
10.9740573727328));
#67416=CARTESIAN_POINT('Ctrl Pts',(-0.322153811874418,2.11016030736698,
10.9744007455043));
#67417=CARTESIAN_POINT('Ctrl Pts',(-0.322272898997973,2.10514729573573,
10.9747022220165));
#67418=CARTESIAN_POINT('Ctrl Pts',(-0.322274972444447,2.10013327014249,
10.9749989620444));
#67419=CARTESIAN_POINT('',(-0.322274851933155,2.09976304472565,11.2245150602744));
#67420=CARTESIAN_POINT('Ctrl Pts',(-0.322274972285662,2.10013365356628,
10.9749989393526));
#67421=CARTESIAN_POINT('Ctrl Pts',(-0.322286505590925,2.07232372871807,
10.9766447874895));
#67422=CARTESIAN_POINT('Ctrl Pts',(-0.318698447630823,2.0446243611031,10.9781452314249));
#67423=CARTESIAN_POINT('Ctrl Pts',(-0.307582929054177,2.00252678812056,
10.980613112068));
#67424=CARTESIAN_POINT('Ctrl Pts',(-0.30246370257334,1.98764388337767,10.9815231732153));
#67425=CARTESIAN_POINT('Ctrl Pts',(-0.295305324641373,1.97091834625809,
10.9826204205879));
#67426=CARTESIAN_POINT('Ctrl Pts',(-0.294304759986646,1.96865307078078,
10.98277063913));
#67427=CARTESIAN_POINT('Ctrl Pts',(-0.292983742380287,1.96575318668376,
10.9829650992664));
#67428=CARTESIAN_POINT('Ctrl Pts',(-0.292687140388391,1.96510775402837,
10.9830085192869));
#67429=CARTESIAN_POINT('Ctrl Pts',(-0.292205626817879,1.96406900217425,
10.9830786247952));
#67430=CARTESIAN_POINT('Ctrl Pts',(-0.292022048046513,1.96367506476905,
10.9831052642163));
#67431=CARTESIAN_POINT('Ctrl Pts',(-0.291670779306314,1.96292525071276,
10.9831560699419));
#67432=CARTESIAN_POINT('Ctrl Pts',(-0.291503233346953,1.9625693071421,10.9831802312259));
#67433=CARTESIAN_POINT('Ctrl Pts',(-0.291119615562072,1.96175818673965,
10.9832353890754));
#67434=CARTESIAN_POINT('Ctrl Pts',(-0.290903127566555,1.96130320888384,
10.9832664000362));
#67435=CARTESIAN_POINT('Ctrl Pts',(-0.29023911087759,1.95991608471161,10.9833611651593));
#67436=CARTESIAN_POINT('Ctrl Pts',(-0.28978816549436,1.95898558972559,10.983425038007));
#67437=CARTESIAN_POINT('Ctrl Pts',(-0.286460554789652,1.95220266464841,
10.9838928902086));
#67438=CARTESIAN_POINT('Ctrl Pts',(-0.283411501660716,1.94643694292837,
10.9843028802144));
#67439=CARTESIAN_POINT('Ctrl Pts',(-0.279294527895826,1.9391925816273,10.9848345157245));
#67440=CARTESIAN_POINT('Ctrl Pts',(-0.278385964976796,1.93762477586695,
10.9849505817826));
#67441=CARTESIAN_POINT('Ctrl Pts',(-0.276190157854215,1.9339083212073,10.9852281369164));
#67442=CARTESIAN_POINT('Ctrl Pts',(-0.274891004631814,1.93176687572201,
10.9853900192953));
#67443=CARTESIAN_POINT('Ctrl Pts',(-0.258638755590362,1.90566860378542,
10.9873869655372));
#67444=CARTESIAN_POINT('Ctrl Pts',(-0.240624897632953,1.8837641769449,10.9893295095311));
#67445=CARTESIAN_POINT('Ctrl Pts',(-0.216796979188666,1.86150602677445,
10.9915064069956));
#67446=CARTESIAN_POINT('Ctrl Pts',(-0.213540201652061,1.85858564558906,
10.9917964689506));
#67447=CARTESIAN_POINT('Ctrl Pts',(-0.206372239800927,1.85241665856006,
10.9924173105733));
#67448=CARTESIAN_POINT('Ctrl Pts',(-0.202441458342558,1.84919235544017,
10.9927469917213));
#67449=CARTESIAN_POINT('Ctrl Pts',(-0.197142943171452,1.84505191155942,
10.9931756268706));
#67450=CARTESIAN_POINT('Ctrl Pts',(-0.195842342519386,1.84405147983064,
10.9932796230344));
#67451=CARTESIAN_POINT('Ctrl Pts',(-0.193961465477244,1.84262742674652,
10.9934282078485));
#67452=CARTESIAN_POINT('Ctrl Pts',(-0.193387349586159,1.84219576303671,
10.9934733217587));
#67453=CARTESIAN_POINT('Ctrl Pts',(-0.192367766777382,1.84143448606023,
10.9935530093519));
#67454=CARTESIAN_POINT('Ctrl Pts',(-0.191922886322869,1.84110409734757,
10.9935876354554));
#67455=CARTESIAN_POINT('Ctrl Pts',(-0.191255678264736,1.8406112628323,10.9936393472546));
#67456=CARTESIAN_POINT('Ctrl Pts',(-0.191033993975276,1.84044795399541,
10.993656492858));
#67457=CARTESIAN_POINT('Ctrl Pts',(-0.19064074625559,1.8401590357485,10.9936868434776));
#67458=CARTESIAN_POINT('Ctrl Pts',(-0.19046926782256,1.84003331203363,10.9937000565092));
#67459=CARTESIAN_POINT('Ctrl Pts',(-0.190125726777528,1.83978195867729,
10.9937264843247));
#67460=CARTESIAN_POINT('Ctrl Pts',(-0.189953664640784,1.83965633039631,
10.993739699024));
#67461=CARTESIAN_POINT('Ctrl Pts',(-0.18953259415636,1.83934953250683,10.9937719854924));
#67462=CARTESIAN_POINT('Ctrl Pts',(-0.18928344986884,1.83916854856127,10.9937910442971));
#67463=CARTESIAN_POINT('Ctrl Pts',(-0.188330687951089,1.838478525171,10.9938637581903));
#67464=CARTESIAN_POINT('Ctrl Pts',(-0.187625264868729,1.83797196744496,
10.9939172427132));
#67465=CARTESIAN_POINT('Ctrl Pts',(-0.171601045978219,1.82656301689355,
10.9951244317931));
#67466=CARTESIAN_POINT('Ctrl Pts',(-0.155356641582743,1.81701723021737,
10.9961892365301));
#67467=CARTESIAN_POINT('Ctrl Pts',(-0.127038638249114,1.80355476045963,
10.9979468928977));
#67468=CARTESIAN_POINT('Ctrl Pts',(-0.1154023415154,1.79883411312044,10.9986438678778));
#67469=CARTESIAN_POINT('Ctrl Pts',(-0.0908192867085159,1.79049568797157,
11.0001099554788));
#67470=CARTESIAN_POINT('Ctrl Pts',(-0.0778625531357536,1.78698493563875,
11.0008794379299));
#67471=CARTESIAN_POINT('Ctrl Pts',(-0.0590317109278613,1.78312428875382,
11.0020190229934));
#67472=CARTESIAN_POINT('Ctrl Pts',(-0.0533075363000413,1.78211124699869,
11.0023680606024));
#67473=CARTESIAN_POINT('Ctrl Pts',(-0.0466451239344354,1.7811171649638,
11.0027783817122));
#67474=CARTESIAN_POINT('Ctrl Pts',(-0.0457303090077639,1.78098468864694,
11.0028348106505));
#67475=CARTESIAN_POINT('Ctrl Pts',(-0.0443381956867634,1.78078920475774,
11.0029208186924));
#67476=CARTESIAN_POINT('Ctrl Pts',(-0.0438612997994791,1.78072332723506,
11.0029503069855));
#67477=CARTESIAN_POINT('Ctrl Pts',(-0.0430337339081151,1.78061089795157,
11.003001521745));
#67478=CARTESIAN_POINT('Ctrl Pts',(-0.0426831306197502,1.78056385439297,
11.0030232326285));
#67479=CARTESIAN_POINT('Ctrl Pts',(-0.0419540916280925,1.78046725443173,
11.0030684061299));
#67480=CARTESIAN_POINT('Ctrl Pts',(-0.0415756440955298,1.7804177928751,
11.0030918717088));
#67481=CARTESIAN_POINT('Ctrl Pts',(-0.0406527590303697,1.78029884258931,
11.0031491339876));
#67482=CARTESIAN_POINT('Ctrl Pts',(-0.0401082315710116,1.78023007236325,
11.0031829533213));
#67483=CARTESIAN_POINT('Ctrl Pts',(-0.038043606937609,1.77997468049737,
11.0033113093046));
#67484=CARTESIAN_POINT('Ctrl Pts',(-0.0365223807408191,1.77979750668268,
11.0034061434928));
#67485=CARTESIAN_POINT('Ctrl Pts',(-0.0344065489643755,1.77956635419292,
11.0035384208527));
#67486=CARTESIAN_POINT('Ctrl Pts',(-0.0338129519234283,1.7795031727905,
11.0035755722486));
#67487=CARTESIAN_POINT('Ctrl Pts',(0.00112730891194376,1.7758823437247,
11.0057648121165));
#67488=CARTESIAN_POINT('Ctrl Pts',(0.0358162906273977,1.77786733165216,
11.0081134930966));
#67489=CARTESIAN_POINT('Ctrl Pts',(0.0791987263826779,1.78745069442327,
11.0111031474422));
#67490=CARTESIAN_POINT('Ctrl Pts',(0.0887783865065095,1.79003559102699,
11.011764032059));
#67491=CARTESIAN_POINT('Ctrl Pts',(0.10150815450842,1.79410923732769,11.012630987656));
#67492=CARTESIAN_POINT('Ctrl Pts',(0.104775151156336,1.79521280541231,11.0128524443016));
#67493=CARTESIAN_POINT('Ctrl Pts',(0.10919022981537,1.79678357282061,11.0131497184835));
#67494=CARTESIAN_POINT('Ctrl Pts',(0.110354129889588,1.79720522770592,11.0132278941916));
#67495=CARTESIAN_POINT('Ctrl Pts',(0.112063308930015,1.79783558909977,11.0133423821373));
#67496=CARTESIAN_POINT('Ctrl Pts',(0.112610480119193,1.79803908166318,11.0133789866153));
#67497=CARTESIAN_POINT('Ctrl Pts',(0.113474674488532,1.7983631506095,11.0134367208747));
#67498=CARTESIAN_POINT('Ctrl Pts',(0.113792062177418,1.79848274137554,11.0134579078631));
#67499=CARTESIAN_POINT('Ctrl Pts',(0.114391741679551,1.79870978062201,11.013497906566));
#67500=CARTESIAN_POINT('Ctrl Pts',(0.114674072055389,1.79881712522565,11.0135167244092));
#67501=CARTESIAN_POINT('Ctrl Pts',(0.115161179424897,1.7990031121493,11.0135491669555));
#67502=CARTESIAN_POINT('Ctrl Pts',(0.115366027466735,1.7990815667827,11.0135628029791));
#67503=CARTESIAN_POINT('Ctrl Pts',(0.115762385097162,1.7992338317814,11.0135891726748));
#67504=CARTESIAN_POINT('Ctrl Pts',(0.115953904001306,1.79930761583351,11.0136019079176));
#67505=CARTESIAN_POINT('Ctrl Pts',(0.116405490607794,1.79948208846341,11.0136319215314));
#67506=CARTESIAN_POINT('Ctrl Pts',(0.116665498857491,1.79958293195018,11.0136491905337));
#67507=CARTESIAN_POINT('Ctrl Pts',(0.117434918962496,1.79988249897222,11.013700259126));
#67508=CARTESIAN_POINT('Ctrl Pts',(0.117943959583554,1.80008218288509,11.0137340013147));
#67509=CARTESIAN_POINT('Ctrl Pts',(0.122473263983379,1.80187223047611,11.0140338562746));
#67510=CARTESIAN_POINT('Ctrl Pts',(0.126461891364466,1.80354214154966,11.0142952907844));
#67511=CARTESIAN_POINT('Ctrl Pts',(0.144029989661839,1.81131647862155,11.0154401865152));
#67512=CARTESIAN_POINT('Ctrl Pts',(0.157211761980527,1.81827784859222,11.0162819372703));
#67513=CARTESIAN_POINT('Ctrl Pts',(0.182288593846631,1.83383139104344,11.0179360459235));
#67514=CARTESIAN_POINT('Ctrl Pts',(0.194172430617465,1.84237252236545,11.0187469857272));
#67515=CARTESIAN_POINT('Ctrl Pts',(0.218344214336702,1.86237068973899,11.0205284698258));
#67516=CARTESIAN_POINT('Ctrl Pts',(0.230398962818633,1.87403964793668,11.0215028961044));
#67517=CARTESIAN_POINT('Ctrl Pts',(0.242267860162846,1.8874703898857,11.0225926581617));
#67518=CARTESIAN_POINT('Ctrl Pts',(0.243039713951109,1.88835348188817,11.0226641666582));
#67519=CARTESIAN_POINT('Ctrl Pts',(0.244153673844902,1.8896421129742,11.0227683125976));
#67520=CARTESIAN_POINT('Ctrl Pts',(0.24449963233475,1.89004432165627,11.0228007905086));
#67521=CARTESIAN_POINT('Ctrl Pts',(0.245102895285899,1.89074918362958,11.0228576589865));
#67522=CARTESIAN_POINT('Ctrl Pts',(0.24536063694186,1.89105146263633,11.0228820314777));
#67523=CARTESIAN_POINT('Ctrl Pts',(0.245858454383012,1.89163749333182,11.022929253109));
#67524=CARTESIAN_POINT('Ctrl Pts',(0.246098599593246,1.89192118547748,11.0229520993466));
#67525=CARTESIAN_POINT('Ctrl Pts',(0.246668331848672,1.89259659655669,11.0230064601568));
#67526=CARTESIAN_POINT('Ctrl Pts',(0.246997476611873,1.89298868572125,11.0230379927519));
#67527=CARTESIAN_POINT('Ctrl Pts',(0.248159056598995,1.89437911611605,11.0231497273836));
#67528=CARTESIAN_POINT('Ctrl Pts',(0.248986376023775,1.89538169745484,11.0232301372489));
#67529=CARTESIAN_POINT('Ctrl Pts',(0.263090155004585,1.91268545502951,11.0246153598456));
#67530=CARTESIAN_POINT('Ctrl Pts',(0.274743587065271,1.93023893518118,11.0259865192235));
#67531=CARTESIAN_POINT('Ctrl Pts',(0.297624392304764,1.97330706051475,11.0292580007473));
#67532=CARTESIAN_POINT('Ctrl Pts',(0.307425042725117,1.99939509541718,11.0311773524713));
#67533=CARTESIAN_POINT('Ctrl Pts',(0.314047052837155,2.0276316273834,11.0330174070865));
#67534=CARTESIAN_POINT('Ctrl Pts',(0.314324914044205,2.02884818148198,11.0330962190931));
#67535=CARTESIAN_POINT('Ctrl Pts',(0.314723135176345,2.03063957436843,11.0332115561625));
#67536=CARTESIAN_POINT('Ctrl Pts',(0.314848997305213,2.03121315992428,11.0332483784213));
#67537=CARTESIAN_POINT('Ctrl Pts',(0.315045377313401,2.03211994515133,11.0333064177723));
#67538=CARTESIAN_POINT('Ctrl Pts',(0.31511693523804,2.03245291463347,11.0333276928405));
#67539=CARTESIAN_POINT('Ctrl Pts',(0.31525112495666,2.03308217317511,11.0333678288733));
#67540=CARTESIAN_POINT('Ctrl Pts',(0.315313867131693,2.03337843795238,11.0333866960886));
#67541=CARTESIAN_POINT('Ctrl Pts',(0.315421382194234,2.03388967179714,11.0334192019865));
#67542=CARTESIAN_POINT('Ctrl Pts',(0.315466353070964,2.03410459863101,11.033432852088));
#67543=CARTESIAN_POINT('Ctrl Pts',(0.31555288081542,2.03452025463806,11.0334592201462));
#67544=CARTESIAN_POINT('Ctrl Pts',(0.31559446577971,2.03472097723323,11.0334719397283));
#67545=CARTESIAN_POINT('Ctrl Pts',(0.315691971851304,2.03519389111773,11.0335018758161));
#67546=CARTESIAN_POINT('Ctrl Pts',(0.315747732592164,2.0354661158454,11.0335190830717));
#67547=CARTESIAN_POINT('Ctrl Pts',(0.315911394195508,2.036270404244,11.0335698492085));
#67548=CARTESIAN_POINT('Ctrl Pts',(0.316018303468171,2.03680267220058,11.0336033516415));
#67549=CARTESIAN_POINT('Ctrl Pts',(0.316943371249401,2.04146934412526,11.0338962822342));
#67550=CARTESIAN_POINT('Ctrl Pts',(0.317681746909734,2.04561939614342,11.0341512666328));
#67551=CARTESIAN_POINT('Ctrl Pts',(0.318487897271585,2.0507297891205,11.0344598276248));
#67552=CARTESIAN_POINT('Ctrl Pts',(0.318633031377166,2.05167727506182,11.0345168080056));
#67553=CARTESIAN_POINT('Ctrl Pts',(0.318790664114814,2.05273795343883,11.0345803547889));
#67554=CARTESIAN_POINT('Ctrl Pts',(0.318807330912431,2.05285051083551,11.0345870952348));
#67555=CARTESIAN_POINT('Ctrl Pts',(0.323594825879833,2.08530093292347,11.0365295054938));
#67556=CARTESIAN_POINT('Ctrl Pts',(0.323418871791408,2.1181796131024,11.0382671601089));
#67557=CARTESIAN_POINT('Ctrl Pts',(0.316499908032065,2.16181264824939,11.040809420811));
#67558=CARTESIAN_POINT('Ctrl Pts',(0.314097276321906,2.17304691931913,11.0414837537174));
#67559=CARTESIAN_POINT('Ctrl Pts',(0.310566713491625,2.18610270396061,11.0423014877548));
#67560=CARTESIAN_POINT('Ctrl Pts',(0.310014005571546,2.18807198878652,11.0424257487357));
#67561=CARTESIAN_POINT('Ctrl Pts',(0.309257687246741,2.19067136584204,11.0425910288291));
#67562=CARTESIAN_POINT('Ctrl Pts',(0.309070818809496,2.19130631224068,11.0426315015477));
#67563=CARTESIAN_POINT('Ctrl Pts',(0.308761089093054,2.19234687381505,11.0426979947211));
#67564=CARTESIAN_POINT('Ctrl Pts',(0.308639380696337,2.19275283242039,11.0427239774479));
#67565=CARTESIAN_POINT('Ctrl Pts',(0.308402190327191,2.19353834520715,11.0427743337435));
#67566=CARTESIAN_POINT('Ctrl Pts',(0.308286807508776,2.19391792872775,11.0427987040273));
#67567=CARTESIAN_POINT('Ctrl Pts',(0.308019068861919,2.19479291895021,11.0428549656657));
#67568=CARTESIAN_POINT('Ctrl Pts',(0.307866218534672,2.19528817211921,11.0428868731841));
#67569=CARTESIAN_POINT('Ctrl Pts',(0.307374018766481,2.19686941073919,11.042988949499));
#67570=CARTESIAN_POINT('Ctrl Pts',(0.307030115601695,2.19795395964441,11.0430592676338));
#67571=CARTESIAN_POINT('Ctrl Pts',(0.303855251642027,2.20778535809125,11.043699513596));
#67572=CARTESIAN_POINT('Ctrl Pts',(0.300657221435879,2.21640835345211,11.0442815254013));
#67573=CARTESIAN_POINT('Ctrl Pts',(0.285742114969969,2.25189144740712,11.0467668190956));
#67574=CARTESIAN_POINT('Ctrl Pts',(0.270759418599727,2.27722408076043,11.0487806693746));
#67575=CARTESIAN_POINT('Ctrl Pts',(0.248599651072349,2.3051832800998,11.0511655147813));
#67576=CARTESIAN_POINT('Ctrl Pts',(0.244484503756594,2.31006975374366,11.0515885027043));
#67577=CARTESIAN_POINT('Ctrl Pts',(0.23672517478167,2.31874633191602,11.0523466005296));
#67578=CARTESIAN_POINT('Ctrl Pts',(0.233128257590068,2.32257580577685,11.0526838601655));
#67579=CARTESIAN_POINT('Ctrl Pts',(0.228972287035158,2.32678912949382,11.0530562838448));
#67580=CARTESIAN_POINT('Ctrl Pts',(0.228504018334942,2.32726093177172,11.0530980069804));
#67581=CARTESIAN_POINT('Ctrl Pts',(0.227771615230126,2.32799430935568,11.0531628878784));
#67582=CARTESIAN_POINT('Ctrl Pts',(0.227508485623431,2.32825687892315,11.0531861222213));
#67583=CARTESIAN_POINT('Ctrl Pts',(0.2270668660611,2.32869603626308,11.0532249902718));
#67584=CARTESIAN_POINT('Ctrl Pts',(0.226888623818351,2.32887287093074,11.0532406433113));
#67585=CARTESIAN_POINT('Ctrl Pts',(0.226540279482203,2.32921765756393,11.0532711669051));
#67586=CARTESIAN_POINT('Ctrl Pts',(0.226370196877471,2.32938562887312,11.0532860389899));
#67587=CARTESIAN_POINT('Ctrl Pts',(0.22604755403463,2.32970355831272,11.0533141913446));
#67588=CARTESIAN_POINT('Ctrl Pts',(0.225895032625989,2.32985355255407,11.0533274744534));
#67589=CARTESIAN_POINT('Ctrl Pts',(0.225541776537568,2.33020026423165,11.053358181479));
#67590=CARTESIAN_POINT('Ctrl Pts',(0.225340934053014,2.33039687076347,11.0533755965801));
#67591=CARTESIAN_POINT('Ctrl Pts',(0.224725701221314,2.33099755373371,11.0534288123423));
#67592=CARTESIAN_POINT('Ctrl Pts',(0.224310476424354,2.33140077959882,11.053464546345));
#67593=CARTESIAN_POINT('Ctrl Pts',(0.221256457636975,2.33435060040325,11.0537260645824));
#67594=CARTESIAN_POINT('Ctrl Pts',(0.218575320882135,2.33685323690722,11.0539485093795));
#67595=CARTESIAN_POINT('Ctrl Pts',(0.198326479432866,2.35511723274437,11.0555814939783));
#67596=CARTESIAN_POINT('Ctrl Pts',(0.179115160409457,2.36895402044413,11.0568769247291));
#67597=CARTESIAN_POINT('Ctrl Pts',(0.147215452101506,2.38698198964458,11.0589296486043));
#67598=CARTESIAN_POINT('Ctrl Pts',(0.135490552676234,2.39270006243359,11.059665335046));
#67599=CARTESIAN_POINT('Ctrl Pts',(0.115554219353248,2.40096761646637,11.0609183459603));
#67600=CARTESIAN_POINT('Ctrl Pts',(0.107529464692874,2.40392709493348,11.0614230845691));
#67601=CARTESIAN_POINT('Ctrl Pts',(0.0978051816322179,2.40707999350992,
11.062039403416));
#67602=CARTESIAN_POINT('Ctrl Pts',(0.0962093673241007,2.4075837015274,11.0621406881873));
#67603=CARTESIAN_POINT('Ctrl Pts',(0.0934185450418449,2.40844076221392,
11.0623181014675));
#67604=CARTESIAN_POINT('Ctrl Pts',(0.0922252666255146,2.40879965751356,
11.0623940480093));
#67605=CARTESIAN_POINT('Ctrl Pts',(0.0905082591785677,2.4093052317748,11.0625034659324));
#67606=CARTESIAN_POINT('Ctrl Pts',(0.08998618313039,2.40945752248523,11.0625367540473));
#67607=CARTESIAN_POINT('Ctrl Pts',(0.0890799301691933,2.40971939116687,
11.0625945703844));
#67608=CARTESIAN_POINT('Ctrl Pts',(0.0886959292143868,2.4098295779331,11.062619078708));
#67609=CARTESIAN_POINT('Ctrl Pts',(0.0879574884210784,2.41003998375589,
11.0626662285788));
#67610=CARTESIAN_POINT('Ctrl Pts',(0.0876030794755914,2.41014030979758,
11.0626888666004));
#67611=CARTESIAN_POINT('Ctrl Pts',(0.0867681950696272,2.4103751035249,11.0627422162835));
#67612=CARTESIAN_POINT('Ctrl Pts',(0.0862875788253872,2.4105090631523,11.0627729444155));
#67613=CARTESIAN_POINT('Ctrl Pts',(0.0848683063736579,2.41090109983592,
11.0628637349262));
#67614=CARTESIAN_POINT('Ctrl Pts',(0.0839287959360401,2.4111560388058,11.0629238990436));
#67615=CARTESIAN_POINT('Ctrl Pts',(0.0756229958424341,2.41336948821514,
11.0634563689979));
#67616=CARTESIAN_POINT('Ctrl Pts',(0.0681910842962278,2.41507020443631,
11.0639369634235));
#67617=CARTESIAN_POINT('Ctrl Pts',(0.0556381306158246,2.41747788255345,
11.0647566078587));
#67618=CARTESIAN_POINT('Ctrl Pts',(0.050547519747401,2.41832805591596,11.0650911187698));
#67619=CARTESIAN_POINT('Ctrl Pts',(0.0203676535977019,2.4226261780475,11.0670861740336));
#67620=CARTESIAN_POINT('Ctrl Pts',(-0.0050358085002599,2.42322881557018,
11.0688234755355));
#67621=CARTESIAN_POINT('Ctrl Pts',(-0.0390981100356025,2.42001815879886,
11.0711134265003));
#67622=CARTESIAN_POINT('Ctrl Pts',(-0.0479155718867667,2.41881720162864,
11.0717014867406));
#67623=CARTESIAN_POINT('Ctrl Pts',(-0.0604554131837114,2.41657713777353,
11.0725212685571));
#67624=CARTESIAN_POINT('Ctrl Pts',(-0.0642259500314016,2.41583377232668,
11.0727655796292));
#67625=CARTESIAN_POINT('Ctrl Pts',(-0.0685083407886799,2.41490962554986,
11.0730398658279));
#67626=CARTESIAN_POINT('Ctrl Pts',(-0.0690339110882322,2.41479482866049,
11.0730734734072));
#67627=CARTESIAN_POINT('Ctrl Pts',(-0.0698255561840318,2.41461983685557,
11.0731240095053));
#67628=CARTESIAN_POINT('Ctrl Pts',(-0.0700918427085674,2.414560619955,11.0731409937705));
#67629=CARTESIAN_POINT('Ctrl Pts',(-0.0705711293419392,2.41445339718521,
11.073171536866));
#67630=CARTESIAN_POINT('Ctrl Pts',(-0.0707841553714158,2.41440551306747,
11.0731851026602));
#67631=CARTESIAN_POINT('Ctrl Pts',(-0.0712419734018721,2.4143021155744,
11.0732142365868));
#67632=CARTESIAN_POINT('Ctrl Pts',(-0.0714867485126919,2.41424653286369,
11.0732298006185));
#67633=CARTESIAN_POINT('Ctrl Pts',(-0.0721461328219506,2.41409599179341,
11.0732716942551));
#67634=CARTESIAN_POINT('Ctrl Pts',(-0.0725606211979494,2.41400049808581,
11.0732979930275));
#67635=CARTESIAN_POINT('Ctrl Pts',(-0.0744705605062103,2.41355648465866,
11.073419017539));
#67636=CARTESIAN_POINT('Ctrl Pts',(-0.0759637296475638,2.41319809298793,
11.073513184125));
#67637=CARTESIAN_POINT('Ctrl Pts',(-0.107942151474649,2.40528045594786,
11.0755213688631));
#67638=CARTESIAN_POINT('Ctrl Pts',(-0.137168483565152,2.39331424067264,
11.0772023830586));
#67639=CARTESIAN_POINT('Ctrl Pts',(-0.170823547680819,2.37338555260755,
11.0794161170358));
#67640=CARTESIAN_POINT('Ctrl Pts',(-0.177299603940018,2.36923072925723,
11.0798557117326));
#67641=CARTESIAN_POINT('Ctrl Pts',(-0.190568968560996,2.36003101958675,
11.0807933381482));
#67642=CARTESIAN_POINT('Ctrl Pts',(-0.197324598403303,2.35494243947079,
11.0812924888056));
#67643=CARTESIAN_POINT('Ctrl Pts',(-0.20586390398981,2.3479674246868,11.0819571186211));
#67644=CARTESIAN_POINT('Ctrl Pts',(-0.207836242385954,2.34631663855998,
11.0821130853541));
#67645=CARTESIAN_POINT('Ctrl Pts',(-0.210335139219411,2.34417375628028,
11.0823139517104));
#67646=CARTESIAN_POINT('Ctrl Pts',(-0.210880134570738,2.34370322705424,
11.0823579611775));
#67647=CARTESIAN_POINT('Ctrl Pts',(-0.21175319877268,2.34294433357055,11.082428789828));
#67648=CARTESIAN_POINT('Ctrl Pts',(-0.212082268297347,2.34265711997669,
11.0824555611999));
#67649=CARTESIAN_POINT('Ctrl Pts',(-0.212706264277336,2.34211025414729,
11.0825064696922));
#67650=CARTESIAN_POINT('Ctrl Pts',(-0.213001301961375,2.34185072955579,
11.082530601463));
#67651=CARTESIAN_POINT('Ctrl Pts',(-0.213670623451771,2.34125979818048,
11.0825854864903));
#67652=CARTESIAN_POINT('Ctrl Pts',(-0.214044611588771,2.3409280593656,11.0826162536195));
#67653=CARTESIAN_POINT('Ctrl Pts',(-0.215150220485708,2.33994274459153,
11.0827075066318));
#67654=CARTESIAN_POINT('Ctrl Pts',(-0.215879625557522,2.33928670103503,
11.0827680962354));
#67655=CARTESIAN_POINT('Ctrl Pts',(-0.220834003862298,2.33478952925394,
11.0831823111476));
#67656=CARTESIAN_POINT('Ctrl Pts',(-0.22495901039486,2.33084024175663,11.0835405245172));
#67657=CARTESIAN_POINT('Ctrl Pts',(-0.251185289099338,2.30436034631158,
11.0859092796138));
#67658=CARTESIAN_POINT('Ctrl Pts',(-0.269976449189104,2.2787990379345,11.0880695269971));
#67659=CARTESIAN_POINT('Ctrl Pts',(-0.289414584760995,2.24212520419406,
11.0908546960212));
#67660=CARTESIAN_POINT('Ctrl Pts',(-0.293668901525981,2.2331126833806,11.0915150774641));
#67661=CARTESIAN_POINT('Ctrl Pts',(-0.298954795570931,2.22042232468121,
11.0923994514248));
#67662=CARTESIAN_POINT('Ctrl Pts',(-0.300348763214145,2.2169022225204,11.0926400767577));
#67663=CARTESIAN_POINT('Ctrl Pts',(-0.301869012781538,2.21285637827059,
11.0929106664692));
#67664=CARTESIAN_POINT('Ctrl Pts',(-0.302056320621364,2.21235409283417,
11.0929441555249));
#67665=CARTESIAN_POINT('Ctrl Pts',(-0.302336917480526,2.21159586979602,
11.0929945491833));
#67666=CARTESIAN_POINT('Ctrl Pts',(-0.302431135537317,2.21134028060896,
11.0930115090652));
#67667=CARTESIAN_POINT('Ctrl Pts',(-0.302593108131419,2.21089916837023,
11.0930407320606));
#67668=CARTESIAN_POINT('Ctrl Pts',(-0.302661016100332,2.21071370270996,
11.0930530044007));
#67669=CARTESIAN_POINT('Ctrl Pts',(-0.302801946771057,2.2103277036916,11.0930785159454));
#67670=CARTESIAN_POINT('Ctrl Pts',(-0.302874940562762,2.21012716081844,
11.0930917533838));
#67671=CARTESIAN_POINT('Ctrl Pts',(-0.303075351311409,2.20957484670271,
11.0931281644425));
#67672=CARTESIAN_POINT('Ctrl Pts',(-0.30320235550609,2.20922292443155,11.0931513133117));
#67673=CARTESIAN_POINT('Ctrl Pts',(-0.303692695285387,2.20785677135116,
11.0932409800713));
#67674=CARTESIAN_POINT('Ctrl Pts',(-0.304051562363496,2.20684092753995,
11.0933072346486));
#67675=CARTESIAN_POINT('Ctrl Pts',(-0.310770061875346,2.18751486839519,
11.0945600868534));
#67676=CARTESIAN_POINT('Ctrl Pts',(-0.315471163088868,2.16866639143661,
11.0956535704891));
#67677=CARTESIAN_POINT('Ctrl Pts',(-0.320984911269382,2.1331996890645,11.0976634125365));
#67678=CARTESIAN_POINT('Ctrl Pts',(-0.322263687232037,2.11672194114262,
11.0985791771401));
#67679=CARTESIAN_POINT('Ctrl Pts',(-0.322279119157057,2.09406097418821,
11.0998769815226));
#67680=CARTESIAN_POINT('Ctrl Pts',(-0.322106784972583,2.08790389574324,
11.1002333037848));
#67681=CARTESIAN_POINT('Ctrl Pts',(-0.321662121054868,2.08006173344352,
11.100693995383));
#67682=CARTESIAN_POINT('Ctrl Pts',(-0.321552690927278,2.07836850894687,
11.1007938705203));
#67683=CARTESIAN_POINT('Ctrl Pts',(-0.320967512822546,2.07030403697101,
11.1012716286859));
#67684=CARTESIAN_POINT('Ctrl Pts',(-0.320315770191979,2.06394735442926,
11.1016544275016));
#67685=CARTESIAN_POINT('Ctrl Pts',(-0.319340408853926,2.05659567667398,
11.1021058058224));
#67686=CARTESIAN_POINT('Ctrl Pts',(-0.319200360194628,2.05557746040996,
11.1021685150284));
#67687=CARTESIAN_POINT('Ctrl Pts',(-0.318984575929597,2.05406234036855,
11.1022621201842));
#67688=CARTESIAN_POINT('Ctrl Pts',(-0.318912543737527,2.05356490878941,
11.1022928989308));
#67689=CARTESIAN_POINT('Ctrl Pts',(-0.318782079289554,2.05267858625138,
11.1023478251374));
#67690=CARTESIAN_POINT('Ctrl Pts',(-0.318724098206761,2.05228962905771,
11.1023719582658));
#67691=CARTESIAN_POINT('Ctrl Pts',(-0.31860044012786,2.05147037352446,11.1024228512993));
#67692=CARTESIAN_POINT('Ctrl Pts',(-0.318534603035533,2.0510401004744,11.1024496162334));
#67693=CARTESIAN_POINT('Ctrl Pts',(-0.318358576800999,2.04990507995941,
11.1025203151052));
#67694=CARTESIAN_POINT('Ctrl Pts',(-0.318246919680029,2.04920056557668,
11.1025642955169));
#67695=CARTESIAN_POINT('Ctrl Pts',(-0.317732518027707,2.0460231526446,11.1027630939253));
#67696=CARTESIAN_POINT('Ctrl Pts',(-0.317303291637972,2.04355468479851,
11.1029187504209));
#67697=CARTESIAN_POINT('Ctrl Pts',(-0.313913752637339,2.02532369735203,
11.1040776362655));
#67698=CARTESIAN_POINT('Ctrl Pts',(-0.309809723394746,2.00979916520171,
11.1051176746206));
#67699=CARTESIAN_POINT('Ctrl Pts',(-0.294241904758251,1.96479393743857,
11.108285739829));
#67700=CARTESIAN_POINT('Ctrl Pts',(-0.279583656067169,1.9366233733669,11.110488570131));
#67701=CARTESIAN_POINT('Ctrl Pts',(-0.260150544648588,1.9097756882248,11.112585806053));
#67702=CARTESIAN_POINT('Ctrl Pts',(-0.259229454663409,1.90852236491617,
11.1126836589867));
#67703=CARTESIAN_POINT('Ctrl Pts',(-0.258043706543295,1.90693316229477,
11.1128076172985));
#67704=CARTESIAN_POINT('Ctrl Pts',(-0.257787424646087,1.90659110152979,
11.1128342910974));
#67705=CARTESIAN_POINT('Ctrl Pts',(-0.257379267004166,1.90604858394906,
11.1128765838894));
#67706=CARTESIAN_POINT('Ctrl Pts',(-0.257227836950572,1.90584779483474,
11.1128922339694));
#67707=CARTESIAN_POINT('Ctrl Pts',(-0.256944527580794,1.90547305322312,
11.1129214369502));
#67708=CARTESIAN_POINT('Ctrl Pts',(-0.256812707547586,1.90529905876304,
11.1129349938037));
#67709=CARTESIAN_POINT('Ctrl Pts',(-0.256516162449057,1.9049084623133,11.1129654223928));
#67710=CARTESIAN_POINT('Ctrl Pts',(-0.256351340160191,1.90469193546109,
11.1129822871032));
#67711=CARTESIAN_POINT('Ctrl Pts',(-0.255861833515929,1.90405055832936,
11.1130322331928));
#67712=CARTESIAN_POINT('Ctrl Pts',(-0.255536363815494,1.90362630441212,
11.1130652593433));
#67713=CARTESIAN_POINT('Ctrl Pts',(-0.252922796162288,1.9002369859955,11.1133290241799));
#67714=CARTESIAN_POINT('Ctrl Pts',(-0.250584106784911,1.89731104871572,
11.1135562519831));
#67715=CARTESIAN_POINT('Ctrl Pts',(-0.241048559871339,1.88579851360797,
11.1144514044096));
#67716=CARTESIAN_POINT('Ctrl Pts',(-0.233456541942335,1.877548259749,11.115095504736));
#67717=CARTESIAN_POINT('Ctrl Pts',(-0.200685871950773,1.84546646406922,
11.117690914745));
#67718=CARTESIAN_POINT('Ctrl Pts',(-0.172177353774156,1.82537831924969,
11.1195680576262));
#67719=CARTESIAN_POINT('Ctrl Pts',(-0.140584914647754,1.81000467626274,
11.1216926054115));
#67720=CARTESIAN_POINT('Ctrl Pts',(-0.140152846737291,1.80979561415512,
11.1217216627831));
#67721=CARTESIAN_POINT('Ctrl Pts',(-0.138259922433071,1.80888490956204,
11.1218489735811));
#67722=CARTESIAN_POINT('Ctrl Pts',(-0.13679427193258,1.80819333618129,11.1219475688659));
#67723=CARTESIAN_POINT('Ctrl Pts',(-0.134756737461304,1.80725064082534,
11.1220846867209));
#67724=CARTESIAN_POINT('Ctrl Pts',(-0.13418922897129,1.8069900745575,11.1221228832378));
#67725=CARTESIAN_POINT('Ctrl Pts',(-0.133280570599592,1.80657606598691,
11.122184051147));
#67726=CARTESIAN_POINT('Ctrl Pts',(-0.132939902700795,1.80642156445158,
11.1222069860545));
#67727=CARTESIAN_POINT('Ctrl Pts',(-0.132238082429994,1.80610474321743,
11.12225423995));
#67728=CARTESIAN_POINT('Ctrl Pts',(-0.131876898473017,1.80594249533295,
11.1222785613567));
#67729=CARTESIAN_POINT('Ctrl Pts',(-0.131038579711416,1.80556776831032,
11.1223350188168));
#67730=CARTESIAN_POINT('Ctrl Pts',(-0.130561226541323,1.80535578310536,
11.1223671717287));
#67731=CARTESIAN_POINT('Ctrl Pts',(-0.129050429952884,1.80468925388385,
11.1224689512538));
#67732=CARTESIAN_POINT('Ctrl Pts',(-0.128015120729468,1.80423898320546,
11.1225387236975));
#67733=CARTESIAN_POINT('Ctrl Pts',(-0.110311589729551,1.79664983588963,
11.1237323178894));
#67734=CARTESIAN_POINT('Ctrl Pts',(-0.0930755304292735,1.79092604324175,
11.1249048460923));
#67735=CARTESIAN_POINT('Ctrl Pts',(-0.0449721212638717,1.7793419217712,
11.1281989993795));
#67736=CARTESIAN_POINT('Ctrl Pts',(-0.0135855239974599,1.77648877419941,
11.1303842054922));
#67737=CARTESIAN_POINT('Ctrl Pts',(0.0192291216163404,1.77829562354102,
11.1324630413769));
#67738=CARTESIAN_POINT('Ctrl Pts',(0.0207393158627849,1.77838944989073,
11.1325582119755));
#67739=CARTESIAN_POINT('Ctrl Pts',(0.0226707846860111,1.77852311117779,
11.1326792407297));
#67740=CARTESIAN_POINT('Ctrl Pts',(0.0230926863436832,1.77855314223438,
11.1327056355626));
#67741=CARTESIAN_POINT('Ctrl Pts',(0.0237643128038553,1.77860227787508,
11.1327475851168));
#67742=CARTESIAN_POINT('Ctrl Pts',(0.0240140747259697,1.77862084298106,
11.1327631700821));
#67743=CARTESIAN_POINT('Ctrl Pts',(0.0244816004614455,1.77865614279342,
11.1327923148035));
#67744=CARTESIAN_POINT('Ctrl Pts',(0.0246993672333281,1.77867280758666,
11.1328058783589));
#67745=CARTESIAN_POINT('Ctrl Pts',(0.0251898742010052,1.77871084564593,
11.1328364034087));
#67746=CARTESIAN_POINT('Ctrl Pts',(0.0254626036031507,1.7787323447857,11.1328533576827));
#67747=CARTESIAN_POINT('Ctrl Pts',(0.026275343225585,1.77879745412792,11.1329038286545));
#67748=CARTESIAN_POINT('Ctrl Pts',(0.0268152746379742,1.7788420790444,11.1329372883614));
#67749=CARTESIAN_POINT('Ctrl Pts',(0.0313020651314989,1.779224302717,11.133214773746));
#67750=CARTESIAN_POINT('Ctrl Pts',(0.0352427199463631,1.77963330163458,
11.1334548661034));
#67751=CARTESIAN_POINT('Ctrl Pts',(0.047911748249203,1.78118482665181,11.1342179552807));
#67752=CARTESIAN_POINT('Ctrl Pts',(0.0566016863271637,1.78261234316721,
11.1347279086689));
#67753=CARTESIAN_POINT('Ctrl Pts',(0.0895115152696047,1.78941346595069,
11.1366437919211));
#67754=CARTESIAN_POINT('Ctrl Pts',(0.113139435671579,1.79721980039706,11.1379936325884));
#67755=CARTESIAN_POINT('Ctrl Pts',(0.1407353486564,1.81002361846842,11.1397412842303));
#67756=CARTESIAN_POINT('Ctrl Pts',(0.145768833303795,1.81252098725543,11.1400672070263));
#67757=CARTESIAN_POINT('Ctrl Pts',(0.157494543444109,1.8187258588255,11.1408464662675));
#67758=CARTESIAN_POINT('Ctrl Pts',(0.164124831897628,1.82254243790705,11.14130306007));
#67759=CARTESIAN_POINT('Ctrl Pts',(0.171439417038848,1.82710688635928,11.1418276163898));
#67760=CARTESIAN_POINT('Ctrl Pts',(0.17226376568294,1.82762650608545,11.1418870388028));
#67761=CARTESIAN_POINT('Ctrl Pts',(0.173506818849672,1.82841795231551,11.1419771111624));
#67762=CARTESIAN_POINT('Ctrl Pts',(0.173927274350962,1.82868702934756,11.1420076590608));
#67763=CARTESIAN_POINT('Ctrl Pts',(0.174656936134254,1.82915638090702,11.1420608146164));
#67764=CARTESIAN_POINT('Ctrl Pts',(0.17496642814806,1.82935621129893,11.1420834057006));
#67765=CARTESIAN_POINT('Ctrl Pts',(0.17560395929017,1.82976939803651,11.1421300343566));
#67766=CARTESIAN_POINT('Ctrl Pts',(0.17593195371403,1.82998282199794,11.1421540744307));
#67767=CARTESIAN_POINT('Ctrl Pts',(0.176700603101929,1.83048497253621,11.1422105315963));
#67768=CARTESIAN_POINT('Ctrl Pts',(0.177140939442664,1.83077418263936,11.1422429667704));
#67769=CARTESIAN_POINT('Ctrl Pts',(0.178069410538245,1.83138726049994,11.1423115546311));
#67770=CARTESIAN_POINT('Ctrl Pts',(0.178557374861144,1.8317113817796,11.1423477167863));
#67771=CARTESIAN_POINT('Ctrl Pts',(0.179866742980831,1.8325862598275,11.1424450638094));
#67772=CARTESIAN_POINT('Ctrl Pts',(0.180686494911895,1.83313946679022,11.1425063410808));
#67773=CARTESIAN_POINT('Ctrl Pts',(0.195021465764697,1.84290970756538,11.143583771011));
#67774=CARTESIAN_POINT('Ctrl Pts',(0.207815921021083,1.85313731898319,11.1446392699356));
#67775=CARTESIAN_POINT('Ctrl Pts',(0.237178893393102,1.88051555649975,11.1473024126867));
#67776=CARTESIAN_POINT('Ctrl Pts',(0.252728699838661,1.89861643817499,11.1489383549451));
#67777=CARTESIAN_POINT('Ctrl Pts',(0.271690434451924,1.92638487766024,11.1511705096389));
#67778=CARTESIAN_POINT('Ctrl Pts',(0.276862542093809,1.93475751247217,11.1518115320709));
#67779=CARTESIAN_POINT('Ctrl Pts',(0.281998506430586,1.94399182776937,11.152474737774));
#67780=CARTESIAN_POINT('Ctrl Pts',(0.28235080702904,1.94463034650834,11.1525203771726));
#67781=CARTESIAN_POINT('Ctrl Pts',(0.282838351275772,1.94552111929646,11.1525837369018));
#67782=CARTESIAN_POINT('Ctrl Pts',(0.282975427445434,1.94577235980716,11.1526015731464));
#67783=CARTESIAN_POINT('Ctrl Pts',(0.283211136270214,1.94620575165398,11.1526322814067));
#67784=CARTESIAN_POINT('Ctrl Pts',(0.283309928013786,1.94638781551856,11.1526451636222));
#67785=CARTESIAN_POINT('Ctrl Pts',(0.283514427702919,1.94676555748459,11.1526718537622));
#67786=CARTESIAN_POINT('Ctrl Pts',(0.283620108458385,1.94696124945941,11.1526856598679));
#67787=CARTESIAN_POINT('Ctrl Pts',(0.283869410557732,1.94742403419987,11.1527182603433));
#67788=CARTESIAN_POINT('Ctrl Pts',(0.284012858109618,1.94769122145967,11.1527370435491));
#67789=CARTESIAN_POINT('Ctrl Pts',(0.284484656637369,1.94857298366152,11.1527989054581));
#67790=CARTESIAN_POINT('Ctrl Pts',(0.284811394511033,1.94918842644795,11.1528418819509));
#67791=CARTESIAN_POINT('Ctrl Pts',(0.29165395039516,1.96217859959539,11.153744858478));
#67792=CARTESIAN_POINT('Ctrl Pts',(0.297360377069753,1.97496527303764,11.1545550935495));
#67793=CARTESIAN_POINT('Ctrl Pts',(0.313884725756788,2.01958768505058,11.1572540602539));
#67794=CARTESIAN_POINT('Ctrl Pts',(0.320553073793347,2.05271880752622,11.1590699414324));
#67795=CARTESIAN_POINT('Ctrl Pts',(0.322085127160976,2.08868147677592,11.1612285137931));
#67796=CARTESIAN_POINT('Ctrl Pts',(0.32216049744579,2.09108083412663,11.1613732673326));
#67797=CARTESIAN_POINT('Ctrl Pts',(0.322239605059702,2.09499067569081,11.1616104480026));
#67798=CARTESIAN_POINT('Ctrl Pts',(0.322259540798553,2.09650076545826,11.1617023692229));
#67799=CARTESIAN_POINT('Ctrl Pts',(0.32227222932597,2.09855654849124,11.1618279543588));
#67800=CARTESIAN_POINT('Ctrl Pts',(0.322274211292739,2.099102182169,11.1618613292478));
#67801=CARTESIAN_POINT('Ctrl Pts',(0.322275223682472,2.10002859379283,11.1619180689192));
#67802=CARTESIAN_POINT('Ctrl Pts',(0.322274964945271,2.10040937110595,11.1619414114075));
#67803=CARTESIAN_POINT('Ctrl Pts',(0.322273095781549,2.10117174049117,11.1619881889911));
#67804=CARTESIAN_POINT('Ctrl Pts',(0.322271482446517,2.10155333196045,11.1620116241413));
#67805=CARTESIAN_POINT('Ctrl Pts',(0.322266267738438,2.10242186458755,11.162065013517));
#67806=CARTESIAN_POINT('Ctrl Pts',(0.322262240451007,2.10290880138403,11.1620949810332));
#67807=CARTESIAN_POINT('Ctrl Pts',(0.322246977394136,2.10435727807169,11.1621842300725));
#67808=CARTESIAN_POINT('Ctrl Pts',(0.3222325417138,2.10531877245459,11.1622436116892));
#67809=CARTESIAN_POINT('Ctrl Pts',(0.322189905118657,2.10750630536493,11.1623790335668));
#67810=CARTESIAN_POINT('Ctrl Pts',(0.32215900881206,2.10873227089407,11.1624551575809));
#67811=CARTESIAN_POINT('Ctrl Pts',(0.321503220180181,2.12994566825458,11.1637764065909));
#67812=CARTESIAN_POINT('Ctrl Pts',(0.319026501717544,2.14982859651757,11.1650811496727));
#67813=CARTESIAN_POINT('Ctrl Pts',(0.308585551081056,2.19721124704738,11.1683336249915));
#67814=CARTESIAN_POINT('Ctrl Pts',(0.298774269560823,2.22413351992096,11.1703094168567));
#67815=CARTESIAN_POINT('Ctrl Pts',(0.284856885159457,2.25073136570968,11.1722078420144));
#67816=CARTESIAN_POINT('Ctrl Pts',(0.284157902583248,2.25204498095543,11.1723014206999));
#67817=CARTESIAN_POINT('Ctrl Pts',(0.283247475481208,2.25372775968843,11.1724210184171));
#67818=CARTESIAN_POINT('Ctrl Pts',(0.283044378329125,2.25410138340238,11.1724475546315));
#67819=CARTESIAN_POINT('Ctrl Pts',(0.282721421815863,2.25469271162721,11.1724895234929));
#67820=CARTESIAN_POINT('Ctrl Pts',(0.282602050054987,2.25491067971539,11.1725049871528));
#67821=CARTESIAN_POINT('Ctrl Pts',(0.282387706101224,2.25530099094743,11.1725326658846));
#67822=CARTESIAN_POINT('Ctrl Pts',(0.282292828877308,2.25547338393156,11.1725448869095));
#67823=CARTESIAN_POINT('Ctrl Pts',(0.282069400650137,2.2558784767551,11.172573594508));
#67824=CARTESIAN_POINT('Ctrl Pts',(0.28194071975812,2.25611110416018,11.1725900725981));
#67825=CARTESIAN_POINT('Ctrl Pts',(0.28156689170883,2.25678493510139,11.1726377823765));
#67826=CARTESIAN_POINT('Ctrl Pts',(0.281320994312782,2.25722572483017,11.172668966038));
#67827=CARTESIAN_POINT('Ctrl Pts',(0.279616040169678,2.26026517893233,11.172883825757));
#67828=CARTESIAN_POINT('Ctrl Pts',(0.278121972265919,2.26284418187908,11.1730652947945));
#67829=CARTESIAN_POINT('Ctrl Pts',(0.273333523543109,2.27085162051902,11.1736272681463));
#67830=CARTESIAN_POINT('Ctrl Pts',(0.269914203680284,2.27620393033147,11.174000771798));
#67831=CARTESIAN_POINT('Ctrl Pts',(0.257752745426355,2.29405474722714,11.1752514271106));
#67832=CARTESIAN_POINT('Ctrl Pts',(0.248282504099237,2.30603296205102,11.1760999098117));
#67833=CARTESIAN_POINT('Ctrl Pts',(0.221156571177228,2.33574332645426,11.1783489491363));
#67834=CARTESIAN_POINT('Ctrl Pts',(0.202229380756787,2.35216697703358,11.1797551868193));
#67835=CARTESIAN_POINT('Ctrl Pts',(0.179922596490352,2.36738201859145,11.1813875425534));
#67836=CARTESIAN_POINT('Ctrl Pts',(0.178237281197064,2.36850839073381,11.1815106690491));
#67837=CARTESIAN_POINT('Ctrl Pts',(0.175968427178553,2.36999399520502,11.1816762042101));
#67838=CARTESIAN_POINT('Ctrl Pts',(0.175394181580329,2.37036739053891,11.1817180820357));
#67839=CARTESIAN_POINT('Ctrl Pts',(0.174494435259594,2.37094836542319,11.1817836695924));
#67840=CARTESIAN_POINT('Ctrl Pts',(0.174169742201446,2.37115719714116,11.1818073326218));
#67841=CARTESIAN_POINT('Ctrl Pts',(0.173520135129708,2.3715733545157,11.1818546638438));
#67842=CARTESIAN_POINT('Ctrl Pts',(0.173195222840069,2.37178068173016,11.1818783319284));
#67843=CARTESIAN_POINT('Ctrl Pts',(0.172466555108044,2.37224380883074,11.1819313995992));
#67844=CARTESIAN_POINT('Ctrl Pts',(0.172062601591138,2.37249929395738,11.1819608107834));
#67845=CARTESIAN_POINT('Ctrl Pts',(0.170880352858381,2.37324334405928,11.1820468657141));
#67846=CARTESIAN_POINT('Ctrl Pts',(0.17010053937595,2.37372947693246,11.1821035991339));
#67847=CARTESIAN_POINT('Ctrl Pts',(0.168331705417179,2.37482168410834,11.1822322267473));
#67848=CARTESIAN_POINT('Ctrl Pts',(0.167341474578119,2.37542576483375,11.1823041933915));
#67849=CARTESIAN_POINT('Ctrl Pts',(0.164179170187885,2.37733154889983,11.1825338985548));
#67850=CARTESIAN_POINT('Ctrl Pts',(0.161995047655948,2.37861297867182,11.1826923710873));
#67851=CARTESIAN_POINT('Ctrl Pts',(0.153481426301801,2.38347398822047,11.1833095203347));
#67852=CARTESIAN_POINT('Ctrl Pts',(0.147046978135979,2.38686446794562,11.1837748103081));
#67853=CARTESIAN_POINT('Ctrl Pts',(0.128654760880419,2.3957743667495,11.185101971699));
#67854=CARTESIAN_POINT('Ctrl Pts',(0.116466245112043,2.40078244236685,11.1859787824058));
#67855=CARTESIAN_POINT('Ctrl Pts',(0.0796325709258978,2.41334166493395,
11.1886009359856));
#67856=CARTESIAN_POINT('Ctrl Pts',(0.0543486863065345,2.41870168158942,
11.1903719732322));
#67857=CARTESIAN_POINT('Ctrl Pts',(0.0272812749704597,2.42112135170366,
11.1920895017625));
#67858=CARTESIAN_POINT('Ctrl Pts',(0.0258666048432852,2.42123839965724,
11.192178737775));
#67859=CARTESIAN_POINT('Ctrl Pts',(0.02403477896752,2.42137778301569,11.1922935616967));
#67860=CARTESIAN_POINT('Ctrl Pts',(0.023618317034262,2.42140865750825,11.1923196181675));
#67861=CARTESIAN_POINT('Ctrl Pts',(0.0229802009126081,2.42145471741773,
11.1923594671744));
#67862=CARTESIAN_POINT('Ctrl Pts',(0.0227585910815346,2.42147048311903,
11.1923732922878));
#67863=CARTESIAN_POINT('Ctrl Pts',(0.0223216154817358,2.42150111618827,
11.1924005252316));
#67864=CARTESIAN_POINT('Ctrl Pts',(0.0221062523520976,2.42151599623583,
11.1924139336489));
#67865=CARTESIAN_POINT('Ctrl Pts',(0.0216259129545834,2.42154869933305,
11.1924438097529));
#67866=CARTESIAN_POINT('Ctrl Pts',(0.0213609302254168,2.42156641120462,
11.1924602710655));
#67867=CARTESIAN_POINT('Ctrl Pts',(0.0205935547748246,2.42161675110045,
11.1925078848268));
#67868=CARTESIAN_POINT('Ctrl Pts',(0.0200911042269686,2.42164852964958,
11.1925389895467));
#67869=CARTESIAN_POINT('Ctrl Pts',(0.0166419652946308,2.42185856417759,
11.1927520367056));
#67870=CARTESIAN_POINT('Ctrl Pts',(0.0136929007994413,2.42199750977293,
11.1929318144236));
#67871=CARTESIAN_POINT('Ctrl Pts',(0.0044383185330517,2.4223061592897,11.193489681011));
#67872=CARTESIAN_POINT('Ctrl Pts',(-0.00187083683493692,2.42233130450191,
11.1938608401677));
#67873=CARTESIAN_POINT('Ctrl Pts',(-0.0163995557725327,2.4219625489532,
11.1947026508984));
#67874=CARTESIAN_POINT('Ctrl Pts',(-0.0246114516756555,2.42143913584733,
11.1951689748867));
#67875=CARTESIAN_POINT('Ctrl Pts',(-0.0351547796587503,2.42036064899454,
11.1957650207563));
#67876=CARTESIAN_POINT('Ctrl Pts',(-0.0375121522217631,2.42009317789086,
11.195898112615));
#67877=CARTESIAN_POINT('Ctrl Pts',(-0.0418937100685406,2.41954697097701,
11.1961454641326));
#67878=CARTESIAN_POINT('Ctrl Pts',(-0.0439186067174756,2.41927496869533,
11.1962597668203));
#67879=CARTESIAN_POINT('Ctrl Pts',(-0.0638294318043176,2.41640736494172,
11.1973846302653));
#67880=CARTESIAN_POINT('Ctrl Pts',(-0.0814690164902492,2.41233085379869,
11.1983907870723));
#67881=CARTESIAN_POINT('Ctrl Pts',(-0.100618705595673,2.40617189574131,
11.1995566211787));
#67882=CARTESIAN_POINT('Ctrl Pts',(-0.102558538860407,2.40552757572936,
11.1996755550277));
#67883=CARTESIAN_POINT('Ctrl Pts',(-0.106836055389708,2.40406146176682,
11.199939800347));
#67884=CARTESIAN_POINT('Ctrl Pts',(-0.109170637815719,2.40323107797723,
11.2000853432664));
#67885=CARTESIAN_POINT('Ctrl Pts',(-0.11755954849835,2.40013780571722,11.2006134550837));
#67886=CARTESIAN_POINT('Ctrl Pts',(-0.123554730358445,2.39771995155523,
11.2010006241662));
#67887=CARTESIAN_POINT('Ctrl Pts',(-0.130417294100534,2.39470929511149,
11.2014567271557));
#67888=CARTESIAN_POINT('Ctrl Pts',(-0.131359714293648,2.39429044267108,
11.2015196490164));
#67889=CARTESIAN_POINT('Ctrl Pts',(-0.132759053095792,2.39366045490954,
11.2016135103359));
#67890=CARTESIAN_POINT('Ctrl Pts',(-0.133217520149066,2.39345275816962,
11.2016443316423));
#67891=CARTESIAN_POINT('Ctrl Pts',(-0.134033404477511,2.39308083667459,
11.2016993055327));
#67892=CARTESIAN_POINT('Ctrl Pts',(-0.134391011972061,2.39291702961872,
11.2017234436921));
#67893=CARTESIAN_POINT('Ctrl Pts',(-0.135081400093194,2.39259925738513,
11.2017701272468));
#67894=CARTESIAN_POINT('Ctrl Pts',(-0.135414219765039,2.39244537807448,
11.2017926696489));
#67895=CARTESIAN_POINT('Ctrl Pts',(-0.13632040550142,2.39202452413079,11.2018541493673));
#67896=CARTESIAN_POINT('Ctrl Pts',(-0.136893247206196,2.3917564301093,11.2018931253493));
#67897=CARTESIAN_POINT('Ctrl Pts',(-0.1391180957658,2.39070719009987,11.2020449417559));
#67898=CARTESIAN_POINT('Ctrl Pts',(-0.140764211166632,2.38991369677706,
11.20215820977));
#67899=CARTESIAN_POINT('Ctrl Pts',(-0.144850628005584,2.3879008731621,11.2024417902872));
#67900=CARTESIAN_POINT('Ctrl Pts',(-0.147282327270247,2.38666449472945,
11.202612693031));
#67901=CARTESIAN_POINT('Ctrl Pts',(-0.156816333497679,2.38166367362775,
11.2032914477006));
#67902=CARTESIAN_POINT('Ctrl Pts',(-0.16379195800011,2.37766520122641,11.2038074154449));
#67903=CARTESIAN_POINT('Ctrl Pts',(-0.176650172920616,2.36964156864037,
11.2047957960116));
#67904=CARTESIAN_POINT('Ctrl Pts',(-0.182563094925284,2.36567379508756,
11.2052661636137));
#67905=CARTESIAN_POINT('Ctrl Pts',(-0.210308784578101,2.34569163092447,
11.2075470149174));
#67906=CARTESIAN_POINT('Ctrl Pts',(-0.230195878789479,2.32716512388663,
11.2094200873821));
#67907=CARTESIAN_POINT('Ctrl Pts',(-0.247662065263262,2.30621522266743,
11.2111860568691));
#67908=CARTESIAN_POINT('Ctrl Pts',(-0.247791589476958,2.30605956618204,
11.2111991598836));
#67909=CARTESIAN_POINT('Ctrl Pts',(-0.248089630244186,2.30570070656009,
11.2112293266428));
#67910=CARTESIAN_POINT('Ctrl Pts',(-0.248258044236419,2.30549741795663,
11.2112463849195));
#67911=CARTESIAN_POINT('Ctrl Pts',(-0.251145595213711,2.30200319204345,
11.2115390605021));
#67912=CARTESIAN_POINT('Ctrl Pts',(-0.253799495321363,2.29865855167063,
11.2118111382571));
#67913=CARTESIAN_POINT('Ctrl Pts',(-0.256716433460838,2.29482850226574,
11.2121128142802));
#67914=CARTESIAN_POINT('Ctrl Pts',(-0.257045463295528,2.29439419310629,
11.2121468821952));
#67915=CARTESIAN_POINT('Ctrl Pts',(-0.257540935355721,2.29373672790081,
11.212198239991));
#67916=CARTESIAN_POINT('Ctrl Pts',(-0.257708190424643,2.29351418994768,
11.2122155864644));
#67917=CARTESIAN_POINT('Ctrl Pts',(-0.257998178775376,2.29312730890536,
11.2122456785265));
#67918=CARTESIAN_POINT('Ctrl Pts',(-0.258121043541063,2.29296306532144,
11.2122584333852));
#67919=CARTESIAN_POINT('Ctrl Pts',(-0.258377728025089,2.29261924991804,
11.2122850910418));
#67920=CARTESIAN_POINT('Ctrl Pts',(-0.258511517298682,2.2924396560033,11.2122989916365));
#67921=CARTESIAN_POINT('Ctrl Pts',(-0.258831157502417,2.29200964761838,
11.2123322169018));
#67922=CARTESIAN_POINT('Ctrl Pts',(-0.259016833025361,2.29175910169806,
11.2123515292061));
#67923=CARTESIAN_POINT('Ctrl Pts',(-0.259645523864615,2.29090818282496,
11.2124169626358));
#67924=CARTESIAN_POINT('Ctrl Pts',(-0.260086822032264,2.29030653526275,
11.2124629645414));
#67925=CARTESIAN_POINT('Ctrl Pts',(-0.268088613375624,2.27931740455733,
11.213298517819));
#67926=CARTESIAN_POINT('Ctrl Pts',(-0.275024432899713,2.26848705185273,
11.2140462713635));
#67927=CARTESIAN_POINT('Ctrl Pts',(-0.292880680164075,2.23654908737248,
11.2161293400547));
#67928=CARTESIAN_POINT('Ctrl Pts',(-0.302140674970359,2.21461159974322,
11.2174241064268));
#67929=CARTESIAN_POINT('Ctrl Pts',(-0.309548391236215,2.18969965145635,
11.2189136991572));
#67930=CARTESIAN_POINT('Ctrl Pts',(-0.310166834987415,2.18753723888272,
11.2190430949091));
#67931=CARTESIAN_POINT('Ctrl Pts',(-0.313810715440795,2.1742726163118,11.2198379475692));
#67932=CARTESIAN_POINT('Ctrl Pts',(-0.316262076377164,2.16302253524376,
11.2205172739084));
#67933=CARTESIAN_POINT('Ctrl Pts',(-0.318299394224182,2.15047889144871,
11.2212897620399));
#67934=CARTESIAN_POINT('Ctrl Pts',(-0.318485604562547,2.14929038922978,
11.2213630975516));
#67935=CARTESIAN_POINT('Ctrl Pts',(-0.318737164351746,2.14762382239962,
11.2214661403069));
#67936=CARTESIAN_POINT('Ctrl Pts',(-0.318808102795438,2.1471466010113,11.221495670528));
#67937=CARTESIAN_POINT('Ctrl Pts',(-0.318935995832331,2.14627274307627,
11.2215497889005));
#67938=CARTESIAN_POINT('Ctrl Pts',(-0.318993282907696,2.14587615553678,
11.2215743664815));
#67939=CARTESIAN_POINT('Ctrl Pts',(-0.319101766146809,2.14511511843883,
11.2216215625014));
#67940=CARTESIAN_POINT('Ctrl Pts',(-0.319153077988528,2.14475068578719,
11.2216441772396));
#67941=CARTESIAN_POINT('Ctrl Pts',(-0.319258908054122,2.14398960733594,
11.221691435867));
#67942=CARTESIAN_POINT('Ctrl Pts',(-0.319313311565178,2.14359294645298,
11.2217160833448));
#67943=CARTESIAN_POINT('Ctrl Pts',(-0.319439626120075,2.14265905157697,
11.2217741538407));
#67944=CARTESIAN_POINT('Ctrl Pts',(-0.319510921106644,2.14212173672847,
11.221807596281));
#67945=CARTESIAN_POINT('Ctrl Pts',(-0.319694872427188,2.1407080446414,11.2218956688574));
#67946=CARTESIAN_POINT('Ctrl Pts',(-0.319805280096866,2.13983138400767,
11.2219503698759));
#67947=CARTESIAN_POINT('Ctrl Pts',(-0.321495713817078,2.12594869728428,
11.222817986632));
#67948=CARTESIAN_POINT('Ctrl Pts',(-0.32228455980763,2.11286066814297,11.2236558602518));
#67949=CARTESIAN_POINT('Ctrl Pts',(-0.322274912584447,2.09976263174766,
11.2245149816093));
#67950=CARTESIAN_POINT('',(-0.322274869595754,2.100295846535,11.4747410785928));
#67951=CARTESIAN_POINT('Ctrl Pts',(-0.322274912883247,2.0997630377757,11.2245149549773));
#67952=CARTESIAN_POINT('Ctrl Pts',(-0.322257167869846,2.07562934868397,
11.2260979218609));
#67953=CARTESIAN_POINT('Ctrl Pts',(-0.319528452590636,2.05157412299925,
11.2277513364805));
#67954=CARTESIAN_POINT('Ctrl Pts',(-0.311483480343985,2.01644805456151,
11.2301667567537));
#67955=CARTESIAN_POINT('Ctrl Pts',(-0.308184629440469,2.00499902034208,
11.2309525967105));
#67956=CARTESIAN_POINT('Ctrl Pts',(-0.303911148762247,1.99276052604722,
11.2317729952443));
#67957=CARTESIAN_POINT('Ctrl Pts',(-0.303558063396941,1.99176510112813,
11.2318395761317));
#67958=CARTESIAN_POINT('Ctrl Pts',(-0.302942032987554,1.99005510487359,
11.2319536776715));
#67959=CARTESIAN_POINT('Ctrl Pts',(-0.302681440042532,1.98933970361187,
11.2320013305429));
#67960=CARTESIAN_POINT('Ctrl Pts',(-0.302309650396511,1.98833017523488,
11.2320684508034));
#67961=CARTESIAN_POINT('Ctrl Pts',(-0.302200557391591,1.98803528412861,
11.2320880421188));
#67962=CARTESIAN_POINT('Ctrl Pts',(-0.302012854502684,1.98753017422174,
11.2321215731145));
#67963=CARTESIAN_POINT('Ctrl Pts',(-0.301934456415664,1.98731987741595,
11.2321355255213));
#67964=CARTESIAN_POINT('Ctrl Pts',(-0.301784177725824,1.9869180494076,11.2321621700806));
#67965=CARTESIAN_POINT('Ctrl Pts',(-0.301712334521615,1.98672650498237,
11.2321748644755));
#67966=CARTESIAN_POINT('Ctrl Pts',(-0.301543047730908,1.98627646547573,
11.2322046751093));
#67967=CARTESIAN_POINT('Ctrl Pts',(-0.301445453870973,1.98601802650689,
11.2322217822912));
#67968=CARTESIAN_POINT('Ctrl Pts',(-0.301157318252216,1.98525797103119,
11.2322720596991));
#67969=CARTESIAN_POINT('Ctrl Pts',(-0.300965854689481,1.98475670141155,
11.2323051749995));
#67970=CARTESIAN_POINT('Ctrl Pts',(-0.299318688184017,1.98047636682896,
11.2325875928504));
#67971=CARTESIAN_POINT('Ctrl Pts',(-0.29779304371687,1.97672436254925,11.2328327953071));
#67972=CARTESIAN_POINT('Ctrl Pts',(-0.296023082510531,1.97259629120257,
11.2331010007329));
#67973=CARTESIAN_POINT('Ctrl Pts',(-0.295848336032624,1.97219103135824,
11.2331273139276));
#67974=CARTESIAN_POINT('Ctrl Pts',(-0.283624759562947,1.94400236081858,
11.2349564830699));
#67975=CARTESIAN_POINT('Ctrl Pts',(-0.267719471077407,1.91805198310139,
11.2365783853178));
#67976=CARTESIAN_POINT('Ctrl Pts',(-0.243934627392196,1.88927101815344,
11.2387041703094));
#67977=CARTESIAN_POINT('Ctrl Pts',(-0.239270176327684,1.88398939690268,
11.2391094837015));
#67978=CARTESIAN_POINT('Ctrl Pts',(-0.228471273512003,1.8725409209569,11.2400288599434));
#67979=CARTESIAN_POINT('Ctrl Pts',(-0.22225296988535,1.86646124084567,11.2405458271256));
#67980=CARTESIAN_POINT('Ctrl Pts',(-0.214875712963193,1.85981019588915,
11.2411494126321));
#67981=CARTESIAN_POINT('Ctrl Pts',(-0.213949728487726,1.85898500537721,
11.2412250040009));
#67982=CARTESIAN_POINT('Ctrl Pts',(-0.212699250071877,1.85788352756138,
11.2413268671389));
#67983=CARTESIAN_POINT('Ctrl Pts',(-0.212378929457911,1.85760250098894,
11.2413529411975));
#67984=CARTESIAN_POINT('Ctrl Pts',(-0.211781971716141,1.85708086427266,
11.2414014986026));
#67985=CARTESIAN_POINT('Ctrl Pts',(-0.211505479232515,1.85684008903736,
11.2414239750444));
#67986=CARTESIAN_POINT('Ctrl Pts',(-0.210931433715147,1.85634191848747,
11.2414706116191));
#67987=CARTESIAN_POINT('Ctrl Pts',(-0.21063381914024,1.85608459530462,11.2414947746824));
#67988=CARTESIAN_POINT('Ctrl Pts',(-0.209953811668142,1.85549882066492,
11.2415499485096));
#67989=CARTESIAN_POINT('Ctrl Pts',(-0.209571118545734,1.85517072071112,
11.2415809736993));
#67990=CARTESIAN_POINT('Ctrl Pts',(-0.2084002012148,1.85417159779695,11.241675824477));
#67991=CARTESIAN_POINT('Ctrl Pts',(-0.207609518140649,1.85350347845571,
11.2417397690647));
#67992=CARTESIAN_POINT('Ctrl Pts',(-0.201795264100384,1.84863831137625,
11.2422092385638));
#67993=CARTESIAN_POINT('Ctrl Pts',(-0.196648388665452,1.84459164417501,
11.2426208209571));
#67994=CARTESIAN_POINT('Ctrl Pts',(-0.189495550032751,1.83931223572083,
11.2431881050269));
#67995=CARTESIAN_POINT('Ctrl Pts',(-0.187593837865329,1.83794041617636,
11.2433384873584));
#67996=CARTESIAN_POINT('Ctrl Pts',(-0.184035739725214,1.83543232224418,
11.2436190439595));
#67997=CARTESIAN_POINT('Ctrl Pts',(-0.182383362731027,1.83429053773368,
11.243749016994));
#67998=CARTESIAN_POINT('Ctrl Pts',(-0.168332390862551,1.82477420293039,
11.2448515396291));
#67999=CARTESIAN_POINT('Ctrl Pts',(-0.155376344667364,1.81725781901964,
11.2458517930096));
#68000=CARTESIAN_POINT('Ctrl Pts',(-0.13079968673523,1.80520045178729,11.2477007096753));
#68001=CARTESIAN_POINT('Ctrl Pts',(-0.119346105964983,1.8003804960653,11.2485444080226));
#68002=CARTESIAN_POINT('Ctrl Pts',(-0.0970106230450789,1.79246568542562,
11.2501299296301));
#68003=CARTESIAN_POINT('Ctrl Pts',(-0.086186609550036,1.7892584001102,11.2508728244769));
#68004=CARTESIAN_POINT('Ctrl Pts',(-0.0737025519997631,1.78626200338303,
11.2516850210315));
#68005=CARTESIAN_POINT('Ctrl Pts',(-0.0721868982699399,1.78590980810848,
11.2517828872688));
#68006=CARTESIAN_POINT('Ctrl Pts',(-0.0702658157767175,1.78547804323444,
11.2519059453327));
#68007=CARTESIAN_POINT('Ctrl Pts',(-0.0698627378677819,1.78538826465537,
11.2519317103064));
#68008=CARTESIAN_POINT('Ctrl Pts',(-0.0692194963123179,1.7852462909575,
11.2519727380133));
#68009=CARTESIAN_POINT('Ctrl Pts',(-0.0689794453095743,1.78519359575845,
11.2519880294441));
#68010=CARTESIAN_POINT('Ctrl Pts',(-0.0685252521055096,1.78509443722911,
11.2520169243712));
#68011=CARTESIAN_POINT('Ctrl Pts',(-0.0683111245664494,1.78504791808762,
11.2520305309624));
#68012=CARTESIAN_POINT('Ctrl Pts',(-0.0678223976239946,1.78494226417037,
11.2520615509351));
#68013=CARTESIAN_POINT('Ctrl Pts',(-0.0675477687064621,1.78488327008905,
11.2520789561148));
#68014=CARTESIAN_POINT('Ctrl Pts',(-0.0667078168726211,1.78470398535475,
11.2521321119707));
#68015=CARTESIAN_POINT('Ctrl Pts',(-0.06614224326597,1.78458485554578,11.2521677962077));
#68016=CARTESIAN_POINT('Ctrl Pts',(-0.0620026591585345,1.78372453660465,
11.2524282111753));
#68017=CARTESIAN_POINT('Ctrl Pts',(-0.0584164268455472,1.78304255442916,
11.2526496340625));
#68018=CARTESIAN_POINT('Ctrl Pts',(-0.03055591582342,1.77823337656398,11.2543429452643));
#68019=CARTESIAN_POINT('Ctrl Pts',(-0.00588914584610395,1.7768389150058,
11.2556894071172));
#68020=CARTESIAN_POINT('Ctrl Pts',(0.0300302398492489,1.77892648370263,
11.2577077226902));
#68021=CARTESIAN_POINT('Ctrl Pts',(0.0413187149275944,1.78018324381883,
11.2583496134809));
#68022=CARTESIAN_POINT('Ctrl Pts',(0.0586195670072356,1.78304072566145,
11.2593649253089));
#68023=CARTESIAN_POINT('Ctrl Pts',(0.0646917388519135,1.78422411853641,
11.259727309717));
#68024=CARTESIAN_POINT('Ctrl Pts',(0.0740938039734348,1.78633903505189,
11.2603001699505));
#68025=CARTESIAN_POINT('Ctrl Pts',(0.077449270889123,1.7871506723797,11.260506972013));
#68026=CARTESIAN_POINT('Ctrl Pts',(0.0829176465982549,1.78856675578361,
11.2608481862337));
#68027=CARTESIAN_POINT('Ctrl Pts',(0.0850386049789374,1.78913919993995,
11.2609815698259));
#68028=CARTESIAN_POINT('Ctrl Pts',(0.0877992221061013,1.78991465356809,
11.2611565962173));
#68029=CARTESIAN_POINT('Ctrl Pts',(0.0884443672169454,1.79009804877814,
11.2611976005212));
#68030=CARTESIAN_POINT('Ctrl Pts',(0.0894979249321199,1.79040110114194,
11.2612647303043));
#68031=CARTESIAN_POINT('Ctrl Pts',(0.0899066835533084,1.79051955636749,
11.261290816564));
#68032=CARTESIAN_POINT('Ctrl Pts',(0.0906929159306681,1.79074908981536,
11.2613410725349));
#68033=CARTESIAN_POINT('Ctrl Pts',(0.0910704234621937,1.79086005043303,
11.2613652383682));
#68034=CARTESIAN_POINT('Ctrl Pts',(0.0919314357614094,1.7911148413918,11.261420436972));
#68035=CARTESIAN_POINT('Ctrl Pts',(0.0924148070601843,1.79125911589007,
11.2614514842156));
#68036=CARTESIAN_POINT('Ctrl Pts',(0.0938907790914673,1.79170343415643,
11.2615464678369));
#68037=CARTESIAN_POINT('Ctrl Pts',(0.0948822648417215,1.79200713208325,
11.2616105237025));
#68038=CARTESIAN_POINT('Ctrl Pts',(0.102159028085886,1.79427451951713,11.262082512362));
#68039=CARTESIAN_POINT('Ctrl Pts',(0.10838387406563,1.79642552484246,11.2624965759582));
#68040=CARTESIAN_POINT('Ctrl Pts',(0.116248919051294,1.79941604432397,11.2630335978392));
#68041=CARTESIAN_POINT('Ctrl Pts',(0.117954114325009,1.80008109047539,11.263150871693));
#68042=CARTESIAN_POINT('Ctrl Pts',(0.146771383088917,1.81160393129525,11.2651471377833));
#68043=CARTESIAN_POINT('Ctrl Pts',(0.172286652735094,1.82608235507904,11.2671494677046));
#68044=CARTESIAN_POINT('Ctrl Pts',(0.204971970430768,1.85102267464569,11.2699053832089));
#68045=CARTESIAN_POINT('Ctrl Pts',(0.214039640544268,1.85877331096139,11.2706921812367));
#68046=CARTESIAN_POINT('Ctrl Pts',(0.223816313852621,1.86811640709246,11.271548030196));
#68047=CARTESIAN_POINT('Ctrl Pts',(0.224966466390309,1.86923208139158,11.2716488355227));
#68048=CARTESIAN_POINT('Ctrl Pts',(0.226405540697228,1.87064900088079,11.2717750610047));
#68049=CARTESIAN_POINT('Ctrl Pts',(0.226702236821778,1.87094226605491,11.271801090384));
#68050=CARTESIAN_POINT('Ctrl Pts',(0.227173488688738,1.87140988095001,11.2718424408301));
#68051=CARTESIAN_POINT('Ctrl Pts',(0.227348413830684,1.87158385516791,11.2718577913799));
#68052=CARTESIAN_POINT('Ctrl Pts',(0.227678203862228,1.87191260655261,11.2718867347598));
#68053=CARTESIAN_POINT('Ctrl Pts',(0.227833109527904,1.87206733940324,11.2719003308286));
#68054=CARTESIAN_POINT('Ctrl Pts',(0.22818526800376,1.87241982269153,11.2719312424145));
#68055=CARTESIAN_POINT('Ctrl Pts',(0.22838242114157,1.87261767141523,11.2719485499423));
#68056=CARTESIAN_POINT('Ctrl Pts',(0.228981157206632,1.8732200842038,11.2720011181253));
#68057=CARTESIAN_POINT('Ctrl Pts',(0.229381926927629,1.87362546040922,11.272036314472));
#68058=CARTESIAN_POINT('Ctrl Pts',(0.232226322258109,1.87651785884341,11.2722862001482));
#68059=CARTESIAN_POINT('Ctrl Pts',(0.234630639580509,1.879043448759,11.2724978752574));
#68060=CARTESIAN_POINT('Ctrl Pts',(0.257991289299909,1.90439381299478,11.2745651011999));
#68061=CARTESIAN_POINT('Ctrl Pts',(0.275596164965768,1.9300922031378,11.2762218342607));
#68062=CARTESIAN_POINT('Ctrl Pts',(0.295710064412846,1.97104014851827,11.2788165890518));
#68063=CARTESIAN_POINT('Ctrl Pts',(0.301256481100086,1.9845897037151,11.2796664942681));
#68064=CARTESIAN_POINT('Ctrl Pts',(0.306356744928255,1.99995414673547,11.2806434453885));
#68065=CARTESIAN_POINT('Ctrl Pts',(0.306839257642292,2.00144393598077,11.2807382945257));
#68066=CARTESIAN_POINT('Ctrl Pts',(0.307664227776886,2.00405587594661,11.2809048243429));
#68067=CARTESIAN_POINT('Ctrl Pts',(0.308011453500283,2.00517649843207,11.2809763480761));
#68068=CARTESIAN_POINT('Ctrl Pts',(0.308506226462004,2.00680470380926,11.2810803869012));
#68069=CARTESIAN_POINT('Ctrl Pts',(0.308658658701833,2.00731080213404,11.2811127420596));
#68070=CARTESIAN_POINT('Ctrl Pts',(0.30892184219017,2.00819246025817,11.2811691366466));
#68071=CARTESIAN_POINT('Ctrl Pts',(0.309033155635182,2.00856785219853,11.2811931576518));
#68072=CARTESIAN_POINT('Ctrl Pts',(0.309247806959349,2.00929660942484,11.2812398086958));
#68073=CARTESIAN_POINT('Ctrl Pts',(0.309351224022832,2.00964995094177,11.2812624361087));
#68074=CARTESIAN_POINT('Ctrl Pts',(0.309593177179976,2.01048190945071,11.2813157335523));
#68075=CARTESIAN_POINT('Ctrl Pts',(0.309731208926827,2.01096067102533,11.2813464199739));
#68076=CARTESIAN_POINT('Ctrl Pts',(0.31020349724187,2.01261318549312,11.2814523939515));
#68077=CARTESIAN_POINT('Ctrl Pts',(0.310532193280485,2.01378850470286,11.2815278622122));
#68078=CARTESIAN_POINT('Ctrl Pts',(0.314402545366612,2.02793708354436,11.2824375688188));
#68079=CARTESIAN_POINT('Ctrl Pts',(0.317135030240786,2.04111611572456,11.2832980494071));
#68080=CARTESIAN_POINT('Ctrl Pts',(0.322742264988997,2.0803688734147,11.2859013645669));
#68081=CARTESIAN_POINT('Ctrl Pts',(0.323269632531096,2.10666646822778,11.2877051827109));
#68082=CARTESIAN_POINT('Ctrl Pts',(0.319617273894639,2.14244057510283,11.29009909489));
#68083=CARTESIAN_POINT('Ctrl Pts',(0.318185586963727,2.15209968310979,11.2907379834616));
#68084=CARTESIAN_POINT('Ctrl Pts',(0.316043172614847,2.16308679297468,11.2914453740954));
#68085=CARTESIAN_POINT('Ctrl Pts',(0.315759436189301,2.16449193006609,11.2915354728));
#68086=CARTESIAN_POINT('Ctrl Pts',(0.31538429782932,2.16628786658685,11.2916501158366));
#68087=CARTESIAN_POINT('Ctrl Pts',(0.315301534410007,2.16668042423969,11.2916751431238));
#68088=CARTESIAN_POINT('Ctrl Pts',(0.315167436732576,2.16731063482504,11.2917152700823));
#68089=CARTESIAN_POINT('Ctrl Pts',(0.315116566530907,2.16754838440588,11.2917303963055));
#68090=CARTESIAN_POINT('Ctrl Pts',(0.315019214972943,2.16800086833013,11.2917591616201));
#68091=CARTESIAN_POINT('Ctrl Pts',(0.314972783464189,2.16821561091787,11.2917728033984));
#68092=CARTESIAN_POINT('Ctrl Pts',(0.314866479012346,2.16870483931604,11.2918038600185));
#68093=CARTESIAN_POINT('Ctrl Pts',(0.31480646681093,2.16897929404199,11.291821266724));
#68094=CARTESIAN_POINT('Ctrl Pts',(0.314618535360809,2.16983341035285,11.2918753886939));
#68095=CARTESIAN_POINT('Ctrl Pts',(0.31448937248105,2.17041280142002,11.2919120327856));
#68096=CARTESIAN_POINT('Ctrl Pts',(0.313478347910406,2.17488971435916,11.2921946636391));
#68097=CARTESIAN_POINT('Ctrl Pts',(0.312525617069997,2.17877109973992,11.2924366761619));
#68098=CARTESIAN_POINT('Ctrl Pts',(0.30799726752279,2.19584137804758,11.2934916812047));
#68099=CARTESIAN_POINT('Ctrl Pts',(0.303656822016394,2.20881406188279,11.294268873093));
#68100=CARTESIAN_POINT('Ctrl Pts',(0.290351415807177,2.24151046574074,11.2962528514013));
#68101=CARTESIAN_POINT('Ctrl Pts',(0.280201191802749,2.2606748753388,11.2974441550979));
#68102=CARTESIAN_POINT('Ctrl Pts',(0.262493935972236,2.28725469291956,11.2992912576973));
#68103=CARTESIAN_POINT('Ctrl Pts',(0.256372492668453,2.29555178005256,11.2998989495893));
#68104=CARTESIAN_POINT('Ctrl Pts',(0.249059496054933,2.3045291371305,11.3005995906683));
#68105=CARTESIAN_POINT('Ctrl Pts',(0.248248573686606,2.30551264219229,11.3006769543108));
#68106=CARTESIAN_POINT('Ctrl Pts',(0.246982526573189,2.30702970550629,11.3007972441958));
#68107=CARTESIAN_POINT('Ctrl Pts',(0.246531453051886,2.30756663999412,11.3008400059698));
#68108=CARTESIAN_POINT('Ctrl Pts',(0.245700304824471,2.30854946441163,11.3009186261479));
#68109=CARTESIAN_POINT('Ctrl Pts',(0.24532075895096,2.30899579928265,11.3009544628246));
#68110=CARTESIAN_POINT('Ctrl Pts',(0.244671769330094,2.30975478843058,11.3010156303718));
#68111=CARTESIAN_POINT('Ctrl Pts',(0.244402937250365,2.31006796575765,11.3010409359902));
#68112=CARTESIAN_POINT('Ctrl Pts',(0.243873813643848,2.31068198047981,11.3010906811962));
#68113=CARTESIAN_POINT('Ctrl Pts',(0.243613565174485,2.31098285413941,11.3011151189757));
#68114=CARTESIAN_POINT('Ctrl Pts',(0.24300875987902,2.31167945949151,11.3011718438711));
#68115=CARTESIAN_POINT('Ctrl Pts',(0.242663793045512,2.31207483228363,11.3012041479994));
#68116=CARTESIAN_POINT('Ctrl Pts',(0.241544851271979,2.31335096725937,11.3013087690935));
#68117=CARTESIAN_POINT('Ctrl Pts',(0.240767041588981,2.31422834087198,11.3013812461048));
#68118=CARTESIAN_POINT('Ctrl Pts',(0.23307386710797,2.32281146512357,11.3020957210278));
#68119=CARTESIAN_POINT('Ctrl Pts',(0.225796459080732,2.33018317935379,11.3027531061938));
#68120=CARTESIAN_POINT('Ctrl Pts',(0.197347848397992,2.35635129128395,11.3052610380192));
#68121=CARTESIAN_POINT('Ctrl Pts',(0.174086138107179,2.37268248188999,11.3072069488528));
#68122=CARTESIAN_POINT('Ctrl Pts',(0.138576019735989,2.39119753100971,11.3098822932387));
#68123=CARTESIAN_POINT('Ctrl Pts',(0.127863449913641,2.39605797217822,11.3106536980132));
#68124=CARTESIAN_POINT('Ctrl Pts',(0.116213653022638,2.40059294347934,11.3114383495289));
#68125=CARTESIAN_POINT('Ctrl Pts',(0.115518351187812,2.40086083391411,11.311484978988));
#68126=CARTESIAN_POINT('Ctrl Pts',(0.114530898660844,2.40123735826879,11.3115509095041));
#68127=CARTESIAN_POINT('Ctrl Pts',(0.114239516564171,2.40134798094888,11.3115703286612));
#68128=CARTESIAN_POINT('Ctrl Pts',(0.11373852004471,2.40153735228262,11.3116036552946));
#68129=CARTESIAN_POINT('Ctrl Pts',(0.113528983575527,2.40161630535005,11.3116175751078));
#68130=CARTESIAN_POINT('Ctrl Pts',(0.113127313881231,2.40176717609063,11.3116442225777));
#68131=CARTESIAN_POINT('Ctrl Pts',(0.112935194565043,2.40183912857819,11.3116569523507));
#68132=CARTESIAN_POINT('Ctrl Pts',(0.112482077369429,2.40200833676204,11.3116869389236));
#68133=CARTESIAN_POINT('Ctrl Pts',(0.112221021355397,2.40210543783657,11.3117041863963));
#68134=CARTESIAN_POINT('Ctrl Pts',(0.111448374755254,2.40239168786539,11.3117551494511));
#68135=CARTESIAN_POINT('Ctrl Pts',(0.110936426235142,2.4025798778341,11.3117888079655));
#68136=CARTESIAN_POINT('Ctrl Pts',(0.106398522394149,2.40423492566739,11.3120862116029));
#68137=CARTESIAN_POINT('Ctrl Pts',(0.102343927612831,2.40562274192891,11.3123453622156));
#68138=CARTESIAN_POINT('Ctrl Pts',(0.0980224894931366,2.40700623894997,
11.3126158478163));
#68139=CARTESIAN_POINT('Ctrl Pts',(0.0977822626798492,2.40708283622927,
11.3126308654065));
#68140=CARTESIAN_POINT('Ctrl Pts',(0.0966090843650532,2.40745539258839,
11.3127041161562));
#68141=CARTESIAN_POINT('Ctrl Pts',(0.0956748679776952,2.40774738551964,
11.3127621702724));
#68142=CARTESIAN_POINT('Ctrl Pts',(0.0703085130019445,2.41554906524073,
11.3143313667764));
#68143=CARTESIAN_POINT('Ctrl Pts',(0.0450678822283201,2.42013075071515,
11.3157200024032));
#68144=CARTESIAN_POINT('Ctrl Pts',(0.00560066933125505,2.42252918148792,
11.3179496253073));
#68145=CARTESIAN_POINT('Ctrl Pts',(-0.00838631442558622,2.42246868166866,
11.3187497060787));
#68146=CARTESIAN_POINT('Ctrl Pts',(-0.0282407562157118,2.42109003106072,
11.3199289193568));
#68147=CARTESIAN_POINT('Ctrl Pts',(-0.0341443830088618,2.42051599415301,
11.3202849405618));
#68148=CARTESIAN_POINT('Ctrl Pts',(-0.0409504086324087,2.41966404680808,
11.3207027368468));
#68149=CARTESIAN_POINT('Ctrl Pts',(-0.0418717694873003,2.41954466617439,
11.3207594515585));
#68150=CARTESIAN_POINT('Ctrl Pts',(-0.0432707353759901,2.41935724793347,
11.3208458066171));
#68151=CARTESIAN_POINT('Ctrl Pts',(-0.0437487305075147,2.41929211847863,
11.3208753550211));
#68152=CARTESIAN_POINT('Ctrl Pts',(-0.0445770921586413,2.41917735461621,
11.3209266370696));
#68153=CARTESIAN_POINT('Ctrl Pts',(-0.0449275274405052,2.419128215803,11.3209483550046));
#68154=CARTESIAN_POINT('Ctrl Pts',(-0.0456553103582945,2.41902494194536,
11.3209935073609));
#68155=CARTESIAN_POINT('Ctrl Pts',(-0.0460326441284862,2.41897071436066,
11.3210169446802));
#68156=CARTESIAN_POINT('Ctrl Pts',(-0.046951383250179,2.41883701584333,
11.3210740768854));
#68157=CARTESIAN_POINT('Ctrl Pts',(-0.0474926826939706,2.41875683544925,
11.3211077941926));
#68158=CARTESIAN_POINT('Ctrl Pts',(-0.0495373726868952,2.41844864030113,
11.3212353718955));
#68159=CARTESIAN_POINT('Ctrl Pts',(-0.0510393287386378,2.41821136779986,
11.3213295252425));
#68160=CARTESIAN_POINT('Ctrl Pts',(-0.0770921258318028,2.41390646556157,
11.3229704965056));
#68161=CARTESIAN_POINT('Ctrl Pts',(-0.101086797606177,2.40702023379844,
11.3246122974463));
#68162=CARTESIAN_POINT('Ctrl Pts',(-0.138710738571104,2.39132966209393,
11.327364818185));
#68163=CARTESIAN_POINT('Ctrl Pts',(-0.152903697696493,2.38413751822651,
11.328446828231));
#68164=CARTESIAN_POINT('Ctrl Pts',(-0.173666221616018,2.37160837115654,
11.3300520978402));
#68165=CARTESIAN_POINT('Ctrl Pts',(-0.180653825076045,2.3670117722686,11.330596297387));
#68166=CARTESIAN_POINT('Ctrl Pts',(-0.188519344907763,2.36138734314269,
11.3312066561789));
#68167=CARTESIAN_POINT('Ctrl Pts',(-0.189578713243375,2.36062002644359,
11.3312888128107));
#68168=CARTESIAN_POINT('Ctrl Pts',(-0.190946334140453,2.35961668616787,
11.3313947790735));
#68169=CARTESIAN_POINT('Ctrl Pts',(-0.191258853566124,2.3593865401188,11.3314189872067));
#68170=CARTESIAN_POINT('Ctrl Pts',(-0.191764115654627,2.35901304459273,
11.3314581137563));
#68171=CARTESIAN_POINT('Ctrl Pts',(-0.191957113952789,2.35887004408742,
11.3314730564196));
#68172=CARTESIAN_POINT('Ctrl Pts',(-0.192327006519708,2.35859533411609,
11.3315016893146));
#68173=CARTESIAN_POINT('Ctrl Pts',(-0.192503924903201,2.35846365926477,
11.3315153818342));
#68174=CARTESIAN_POINT('Ctrl Pts',(-0.192910549194887,2.35816037234505,
11.3315468468583));
#68175=CARTESIAN_POINT('Ctrl Pts',(-0.193140162007362,2.3579886347522,11.3315646105313));
#68176=CARTESIAN_POINT('Ctrl Pts',(-0.193850792248245,2.35745564249114,
11.3316195760497));
#68177=CARTESIAN_POINT('Ctrl Pts',(-0.194331031122767,2.35709334464808,
11.3316567051538));
#68178=CARTESIAN_POINT('Ctrl Pts',(-0.198295633680705,2.35408494615743,
11.3319631153394));
#68179=CARTESIAN_POINT('Ctrl Pts',(-0.201727001701122,2.35136932905977,
11.332227619736));
#68180=CARTESIAN_POINT('Ctrl Pts',(-0.20587752965679,2.34794480990606,11.3325481729399));
#68181=CARTESIAN_POINT('Ctrl Pts',(-0.206649866688878,2.34730147314956,
11.3326078487002));
#68182=CARTESIAN_POINT('Ctrl Pts',(-0.20837924623776,2.3458471860078,11.3327415645579));
#68183=CARTESIAN_POINT('Ctrl Pts',(-0.209334593514034,2.34503423673766,
11.3328154966818));
#68184=CARTESIAN_POINT('Ctrl Pts',(-0.210800206431039,2.34377225130663,
11.3329290602555));
#68185=CARTESIAN_POINT('Ctrl Pts',(-0.211313829647995,2.34332715210315,
11.3329688859367));
#68186=CARTESIAN_POINT('Ctrl Pts',(-0.212446244318525,2.34233952653793,
11.3330567624215));
#68187=CARTESIAN_POINT('Ctrl Pts',(-0.213064374936227,2.34179624687297,
11.3331047768513));
#68188=CARTESIAN_POINT('Ctrl Pts',(-0.236477748626727,2.32105855934872,
11.3349255390429));
#68189=CARTESIAN_POINT('Ctrl Pts',(-0.256299221631263,2.29773633896801,
11.3365569851879));
#68190=CARTESIAN_POINT('Ctrl Pts',(-0.278381798287223,2.26273919428442,
11.338943891826));
#68191=CARTESIAN_POINT('Ctrl Pts',(-0.283736358910085,2.25321263410087,
11.33958659776));
#68192=CARTESIAN_POINT('Ctrl Pts',(-0.2894794297308,2.24165722459343,11.3403670821373));
#68193=CARTESIAN_POINT('Ctrl Pts',(-0.290345742613333,2.23987301022815,
11.3404876059498));
#68194=CARTESIAN_POINT('Ctrl Pts',(-0.291475806249693,2.23748984672977,
11.3406486459071));
#68195=CARTESIAN_POINT('Ctrl Pts',(-0.29175429411947,2.23689790150177,11.3406886506411));
#68196=CARTESIAN_POINT('Ctrl Pts',(-0.292209507155768,2.23592261670422,
11.3407545713113));
#68197=CARTESIAN_POINT('Ctrl Pts',(-0.292387285852208,2.23553976860403,
11.3407804507856));
#68198=CARTESIAN_POINT('Ctrl Pts',(-0.292730993831924,2.2347957671431,11.3408307481886));
#68199=CARTESIAN_POINT('Ctrl Pts',(-0.292897008268704,2.23443465377095,
11.3408551631245));
#68200=CARTESIAN_POINT('Ctrl Pts',(-0.293279756734901,2.23359802768407,
11.3409117332416));
#68201=CARTESIAN_POINT('Ctrl Pts',(-0.2934960025927,2.23312229403271,11.3409439051514));
#68202=CARTESIAN_POINT('Ctrl Pts',(-0.294074930190123,2.23184040535424,
11.3410306065643));
#68203=CARTESIAN_POINT('Ctrl Pts',(-0.29443545179984,2.23103328488892,11.3410852100494));
#68204=CARTESIAN_POINT('Ctrl Pts',(-0.297016792335192,2.22518984491185,
11.3414806416937));
#68205=CARTESIAN_POINT('Ctrl Pts',(-0.299111467723363,2.22009910922912,
11.3418257499965));
#68206=CARTESIAN_POINT('Ctrl Pts',(-0.312392693735311,2.18531545867443,
11.3441898417103));
#68207=CARTESIAN_POINT('Ctrl Pts',(-0.319269283773583,2.15416829051745,
11.3463611927753));
#68208=CARTESIAN_POINT('Ctrl Pts',(-0.322014613897808,2.11499428314519,
11.348996619342));
#68209=CARTESIAN_POINT('Ctrl Pts',(-0.322277630461605,2.10744195239842,
11.3494990518891));
#68210=CARTESIAN_POINT('Ctrl Pts',(-0.322274760262603,2.09926006986015,
11.3500329025093));
#68211=CARTESIAN_POINT('Ctrl Pts',(-0.322272711291937,2.0986331910827,11.3500737381608));
#68212=CARTESIAN_POINT('Ctrl Pts',(-0.322262647519997,2.09700643224205,
11.3501795272261));
#68213=CARTESIAN_POINT('Ctrl Pts',(-0.322251808357313,2.09600656880701,
11.3502443724598));
#68214=CARTESIAN_POINT('Ctrl Pts',(-0.322231286061559,2.0946821723725,11.3503300176523));
#68215=CARTESIAN_POINT('Ctrl Pts',(-0.322225765931273,2.09435759100465,
11.3503509877838));
#68216=CARTESIAN_POINT('Ctrl Pts',(-0.322142162270717,2.08984295570853,
11.3506423847816));
#68217=CARTESIAN_POINT('Ctrl Pts',(-0.321982842034037,2.08565455274893,
11.3509093892228));
#68218=CARTESIAN_POINT('Ctrl Pts',(-0.321710696427258,2.08092915467588,
11.3512059711591));
#68219=CARTESIAN_POINT('Ctrl Pts',(-0.321678170886067,2.08038817390923,
11.3512398558992));
#68220=CARTESIAN_POINT('Ctrl Pts',(-0.321626919389701,2.07957018283672,
11.3512909843371));
#68221=CARTESIAN_POINT('Ctrl Pts',(-0.32160920007326,2.0792931138242,11.351308283924));
#68222=CARTESIAN_POINT('Ctrl Pts',(-0.321577779737462,2.07881157869098,
11.3513383172269));
#68223=CARTESIAN_POINT('Ctrl Pts',(-0.321564241736346,2.0786071026854,11.3513510601254));
#68224=CARTESIAN_POINT('Ctrl Pts',(-0.321535489433735,2.07817902642415,
11.3513777160785));
#68225=CARTESIAN_POINT('Ctrl Pts',(-0.32152023692546,2.07795542921854,11.3513916268917));
#68226=CARTESIAN_POINT('Ctrl Pts',(-0.321483142001477,2.07741985742535,
11.3514249174701));
#68227=CARTESIAN_POINT('Ctrl Pts',(-0.321461078615877,2.07710789728034,
11.3514442847425));
#68228=CARTESIAN_POINT('Ctrl Pts',(-0.321384460829354,2.07604653384006,
11.3515100972263));
#68229=CARTESIAN_POINT('Ctrl Pts',(-0.321327739172489,2.0752972821618,11.3515564213311));
#68230=CARTESIAN_POINT('Ctrl Pts',(-0.321186363489505,2.07351274876815,
11.3516664465324));
#68231=CARTESIAN_POINT('Ctrl Pts',(-0.321099323082241,2.07247765721126,
11.3517300183183));
#68232=CARTESIAN_POINT('Ctrl Pts',(-0.319985740555356,2.05995995741967,
11.3524960223014));
#68233=CARTESIAN_POINT('Ctrl Pts',(-0.318348655376113,2.04853860388575,
11.3531666224636));
#68234=CARTESIAN_POINT('Ctrl Pts',(-0.312585255584749,2.01951552768629,
11.3548528312258));
#68235=CARTESIAN_POINT('Ctrl Pts',(-0.307585194892534,2.00212924602347,
11.3558471779224));
#68236=CARTESIAN_POINT('Ctrl Pts',(-0.294198592816751,1.96699598748604,
11.3579662293857));
#68237=CARTESIAN_POINT('Ctrl Pts',(-0.285597735543596,1.94941234818879,
11.3590915593017));
#68238=CARTESIAN_POINT('Ctrl Pts',(-0.27478706982546,1.93161081744876,11.3603565552511));
#68239=CARTESIAN_POINT('Ctrl Pts',(-0.274108648226786,1.93050870395655,
11.3604354020208));
#68240=CARTESIAN_POINT('Ctrl Pts',(-0.273153143741806,1.92897720392091,
11.3605457199085));
#68241=CARTESIAN_POINT('Ctrl Pts',(-0.272881643774218,1.92854433459032,
11.3605769849733));
#68242=CARTESIAN_POINT('Ctrl Pts',(-0.272411008231611,1.9277979204997,11.360631043289));
#68243=CARTESIAN_POINT('Ctrl Pts',(-0.272212357359613,1.92748407004326,
11.3606538185599));
#68244=CARTESIAN_POINT('Ctrl Pts',(-0.27180004984217,1.92683514659664,11.3607010026624));
#68245=CARTESIAN_POINT('Ctrl Pts',(-0.271586315203881,1.92650012409172,
11.3607254143657));
#68246=CARTESIAN_POINT('Ctrl Pts',(-0.271085298505831,1.92571799002968,
11.360782526825));
#68247=CARTESIAN_POINT('Ctrl Pts',(-0.270797529683122,1.92527119305217,
11.3608152456765));
#68248=CARTESIAN_POINT('Ctrl Pts',(-0.269868427986225,1.92383645513704,
11.3609206127401));
#68249=CARTESIAN_POINT('Ctrl Pts',(-0.26922278931383,1.92285132623277,11.3609934217841));
#68250=CARTESIAN_POINT('Ctrl Pts',(-0.267709438798386,1.92056960668969,
11.3611631456716));
#68251=CARTESIAN_POINT('Ctrl Pts',(-0.26683768871196,1.91927574205359,11.3612602116797));
#68252=CARTESIAN_POINT('Ctrl Pts',(-0.257749077940783,1.90599541108135,
11.3622651230337));
#68253=CARTESIAN_POINT('Ctrl Pts',(-0.248740970689,1.8945731459135,11.3632034653423));
#68254=CARTESIAN_POINT('Ctrl Pts',(-0.218226273014972,1.86084144644508,
11.3662147778078));
#68255=CARTESIAN_POINT('Ctrl Pts',(-0.19426128068826,1.84099825800115,11.3683709608921));
#68256=CARTESIAN_POINT('Ctrl Pts',(-0.164748890010322,1.82299448536771,
11.370593445208));
#68257=CARTESIAN_POINT('Ctrl Pts',(-0.161630216819241,1.821163259902,11.3708232524154));
#68258=CARTESIAN_POINT('Ctrl Pts',(-0.157979280602623,1.81910134419536,
11.371085897172));
#68259=CARTESIAN_POINT('Ctrl Pts',(-0.157476572978896,1.8188192095686,11.3711219228752));
#68260=CARTESIAN_POINT('Ctrl Pts',(-0.156728050133536,1.81840175309935,
11.3711753556645));
#68261=CARTESIAN_POINT('Ctrl Pts',(-0.156482814323158,1.81826540294255,
11.3711928284236));
#68262=CARTESIAN_POINT('Ctrl Pts',(-0.156045778826928,1.81802315957682,
11.3712239071148));
#68263=CARTESIAN_POINT('Ctrl Pts',(-0.155854049346688,1.81791714173303,
11.3712375210835));
#68264=CARTESIAN_POINT('Ctrl Pts',(-0.155446859434647,1.81769252577277,
11.3712663906848));
#68265=CARTESIAN_POINT('Ctrl Pts',(-0.155231371927921,1.81757397909718,
11.3712816429731));
#68266=CARTESIAN_POINT('Ctrl Pts',(-0.154653012969298,1.81725666694516,
11.3713225111528));
#68267=CARTESIAN_POINT('Ctrl Pts',(-0.154289892564901,1.81705835254545,
11.3713480980743));
#68268=CARTESIAN_POINT('Ctrl Pts',(-0.152551827026258,1.81611346716004,
11.3714702300917));
#68269=CARTESIAN_POINT('Ctrl Pts',(-0.151171809089077,1.81537619947339,
11.3715661895778));
#68270=CARTESIAN_POINT('Ctrl Pts',(-0.139697066005331,1.80935287758154,
11.3723561844237));
#68271=CARTESIAN_POINT('Ctrl Pts',(-0.12933267025224,1.80459495419969,11.3730194368098));
#68272=CARTESIAN_POINT('Ctrl Pts',(-0.0849952756713622,1.78702350160199,
11.3757387256628));
#68273=CARTESIAN_POINT('Ctrl Pts',(-0.0492400728219842,1.7794472788211,
11.3776858655186));
#68274=CARTESIAN_POINT('Ctrl Pts',(-0.0105334510163253,1.77788793613816,
11.3800220205265));
#68275=CARTESIAN_POINT('Ctrl Pts',(-0.00809320590537355,1.77781738906632,
11.3801700830293));
#68276=CARTESIAN_POINT('Ctrl Pts',(-0.00491502393441853,1.77776163772369,
11.3803640108235));
#68277=CARTESIAN_POINT('Ctrl Pts',(-0.004177565082357,1.77775123348794,
11.380409085805));
#68278=CARTESIAN_POINT('Ctrl Pts',(-0.00299940278673548,1.77773865663401,
11.3804812216926));
#68279=CARTESIAN_POINT('Ctrl Pts',(-0.00255871632707988,1.77773485634833,
11.3805082315666));
#68280=CARTESIAN_POINT('Ctrl Pts',(-0.00176502681447951,1.77772964002475,
11.380556927659));
#68281=CARTESIAN_POINT('Ctrl Pts',(-0.00141202599249764,1.77772790002978,
11.3805786036913));
#68282=CARTESIAN_POINT('Ctrl Pts',(-0.000584296812591893,1.77772518002378,
11.3806294729498));
#68283=CARTESIAN_POINT('Ctrl Pts',(-0.000109568635152322,1.77772466897949,
11.3806586808236));
#68284=CARTESIAN_POINT('Ctrl Pts',(0.00125787086624673,1.77772621837162,
11.380742908553));
#68285=CARTESIAN_POINT('Ctrl Pts',(0.00215056945188629,1.77773093913696,
11.3807980116101));
#68286=CARTESIAN_POINT('Ctrl Pts',(0.0081326857779983,1.77778743053788,
11.3811680640883));
#68287=CARTESIAN_POINT('Ctrl Pts',(0.0132200369947419,1.77795604905191,
11.381486655182));
#68288=CARTESIAN_POINT('Ctrl Pts',(0.0278436129398111,1.77878782063104,
11.3824143393393));
#68289=CARTESIAN_POINT('Ctrl Pts',(0.0373564599011915,1.77975478698624,
11.3830325667887));
#68290=CARTESIAN_POINT('Ctrl Pts',(0.0766474732230871,1.78552312003411,
11.3856457197092));
#68291=CARTESIAN_POINT('Ctrl Pts',(0.105716704378513,1.79406826305974,11.387740093877));
#68292=CARTESIAN_POINT('Ctrl Pts',(0.133983641781497,1.80689532244629,11.3897667565093));
#68293=CARTESIAN_POINT('Ctrl Pts',(0.134792858967848,1.80726658292542,11.3898247507822));
#68294=CARTESIAN_POINT('Ctrl Pts',(0.136146108144932,1.80789424082443,11.3899216813483));
#68295=CARTESIAN_POINT('Ctrl Pts',(0.136690975470414,1.8081488143903,11.3899606946782));
#68296=CARTESIAN_POINT('Ctrl Pts',(0.137494730866613,1.80852709057561,11.3900182201424));
#68297=CARTESIAN_POINT('Ctrl Pts',(0.137754168508875,1.80864961471797,11.3900367845145));
#68298=CARTESIAN_POINT('Ctrl Pts',(0.13839585018029,1.80895370925731,11.3900826907974));
#68299=CARTESIAN_POINT('Ctrl Pts',(0.138777901985562,1.80913568691488,11.3901100141952));
#68300=CARTESIAN_POINT('Ctrl Pts',(0.142831562103555,1.81107631796754,11.3903998199027));
#68301=CARTESIAN_POINT('Ctrl Pts',(0.146470105386644,1.81290374222548,11.3906590610497));
#68302=CARTESIAN_POINT('Ctrl Pts',(0.150548826194132,1.81504997743624,11.3909478367668));
#68303=CARTESIAN_POINT('Ctrl Pts',(0.151023783824546,1.81530142052213,11.3909814355843));
#68304=CARTESIAN_POINT('Ctrl Pts',(0.15174212484499,1.81568401451245,11.391032205797));
#68305=CARTESIAN_POINT('Ctrl Pts',(0.151985969156564,1.8158142909343,11.3910494319919));
#68306=CARTESIAN_POINT('Ctrl Pts',(0.152410005983539,1.81604153900037,11.3910793734193));
#68307=CARTESIAN_POINT('Ctrl Pts',(0.152590273849286,1.81613836852379,11.3910920976985));
#68308=CARTESIAN_POINT('Ctrl Pts',(0.15296802205246,1.81634173693857,11.3911187515392));
#68309=CARTESIAN_POINT('Ctrl Pts',(0.15316548329971,1.81644831035666,11.3911326787989));
#68310=CARTESIAN_POINT('Ctrl Pts',(0.15363914237129,1.8167045918943,11.3911660737386));
#68311=CARTESIAN_POINT('Ctrl Pts',(0.153915233883513,1.81685449835297,11.3911855287245));
#68312=CARTESIAN_POINT('Ctrl Pts',(0.154842833757168,1.81735990500328,11.3912508584859));
#68313=CARTESIAN_POINT('Ctrl Pts',(0.155493339355823,1.81771725538503,11.3912966159694));
#68314=CARTESIAN_POINT('Ctrl Pts',(0.157045116931194,1.81857670452074,11.3914056481177));
#68315=CARTESIAN_POINT('Ctrl Pts',(0.157945230156048,1.81908089362418,11.3914687936616));
#68316=CARTESIAN_POINT('Ctrl Pts',(0.168745359740301,1.82519879412834,11.3922254513136));
#68317=CARTESIAN_POINT('Ctrl Pts',(0.178344914343773,1.83132947468025,11.3928879275854));
#68318=CARTESIAN_POINT('Ctrl Pts',(0.20869985926452,1.85306099628176,11.3950166235831));
#68319=CARTESIAN_POINT('Ctrl Pts',(0.227897196189615,1.87065865649994,11.3964262556818));
#68320=CARTESIAN_POINT('Ctrl Pts',(0.248366278791247,1.89455946420404,11.3982412623956));
#68321=CARTESIAN_POINT('Ctrl Pts',(0.251847116713623,1.89884173553397,11.3985627468047));
#68322=CARTESIAN_POINT('Ctrl Pts',(0.259313591127547,1.90852503108503,11.3992841385145));
#68323=CARTESIAN_POINT('Ctrl Pts',(0.26324378173639,1.91396531586363,11.3996858096092));
#68324=CARTESIAN_POINT('Ctrl Pts',(0.267585024537801,1.92038786939276,11.400157588205));
#68325=CARTESIAN_POINT('Ctrl Pts',(0.26816473361342,1.92125454292723,11.4002212003856));
#68326=CARTESIAN_POINT('Ctrl Pts',(0.269019271110226,1.92254560301677,11.4003158927731));
#68327=CARTESIAN_POINT('Ctrl Pts',(0.269297327119056,1.92296785365566,11.4003468517216));
#68328=CARTESIAN_POINT('Ctrl Pts',(0.269790093827069,1.92372000727747,11.4004019802214));
#68329=CARTESIAN_POINT('Ctrl Pts',(0.27000519637855,1.9240496533454,11.4004261350477));
#68330=CARTESIAN_POINT('Ctrl Pts',(0.27045603463757,1.92474333949884,11.4004769520664));
#68331=CARTESIAN_POINT('Ctrl Pts',(0.27069164032874,1.92510746278041,11.400503619046));
#68332=CARTESIAN_POINT('Ctrl Pts',(0.271301335856536,1.92605391685708,11.4005729150985));
#68333=CARTESIAN_POINT('Ctrl Pts',(0.271674284558492,1.92663697690686,11.4006155865113));
#68334=CARTESIAN_POINT('Ctrl Pts',(0.273285967541569,1.92917462005297,11.4008012298959));
#68335=CARTESIAN_POINT('Ctrl Pts',(0.274505483292307,1.93114127300455,11.4009449107577));
#68336=CARTESIAN_POINT('Ctrl Pts',(0.283023197408598,1.94521352336701,11.4019718709127));
#68337=CARTESIAN_POINT('Ctrl Pts',(0.289538172460316,1.95777295085765,11.4028835285566));
#68338=CARTESIAN_POINT('Ctrl Pts',(0.30440342555142,1.99171679812595,11.4053333954308));
#68339=CARTESIAN_POINT('Ctrl Pts',(0.311332480722723,2.01363654946929,11.4069056397352));
#68340=CARTESIAN_POINT('Ctrl Pts',(0.316736882305902,2.04035329504781,11.4087269090854));
#68341=CARTESIAN_POINT('Ctrl Pts',(0.317510852410453,2.04462091306966,11.4090148190689));
#68342=CARTESIAN_POINT('Ctrl Pts',(0.319393179477519,2.05634280540895,11.4097953207747));
#68343=CARTESIAN_POINT('Ctrl Pts',(0.320326704382693,2.06382296571582,11.4102820877981));
#68344=CARTESIAN_POINT('Ctrl Pts',(0.321058357966574,2.07201465751626,11.4107980363229));
#68345=CARTESIAN_POINT('Ctrl Pts',(0.321117348903699,2.07269987421677,11.4108410637669));
#68346=CARTESIAN_POINT('Ctrl Pts',(0.321197190871934,2.07366337027746,11.4109013770768));
#68347=CARTESIAN_POINT('Ctrl Pts',(0.321219874124523,2.07394148971953,11.4109187648537));
#68348=CARTESIAN_POINT('Ctrl Pts',(0.321258617694233,2.07442426300877,11.4109489087156));
#68349=CARTESIAN_POINT('Ctrl Pts',(0.321274843696754,2.07462890279038,11.4109616741484));
#68350=CARTESIAN_POINT('Ctrl Pts',(0.321308351169368,2.07505668060003,11.4109883335251));
#68351=CARTESIAN_POINT('Ctrl Pts',(0.321325595718477,2.07527982098841,11.4110022252993));
#68352=CARTESIAN_POINT('Ctrl Pts',(0.321366253171583,2.07581315001459,11.4110353938813));
#68353=CARTESIAN_POINT('Ctrl Pts',(0.321389449521425,2.0761233560143,11.4110546584326));
#68354=CARTESIAN_POINT('Ctrl Pts',(0.321464784825603,2.07715082233046,11.4111183764601));
#68355=CARTESIAN_POINT('Ctrl Pts',(0.321514972572268,2.07786823011169,11.411162720841));
#68356=CARTESIAN_POINT('Ctrl Pts',(0.32162883875125,2.07957808321426,11.4112680764456));
#68357=CARTESIAN_POINT('Ctrl Pts',(0.321690326159174,2.08057067380755,11.4113289688813));
#68358=CARTESIAN_POINT('Ctrl Pts',(0.322355582655625,2.09218052293047,11.4120382332205));
#68359=CARTESIAN_POINT('Ctrl Pts',(0.322438135198141,2.10282233956264,11.4126594456948));
#68360=CARTESIAN_POINT('Ctrl Pts',(0.321142405703716,2.13384257073631,11.41443548328));
#68361=CARTESIAN_POINT('Ctrl Pts',(0.318355255251917,2.15410883659745,11.4155545094065));
#68362=CARTESIAN_POINT('Ctrl Pts',(0.309497782562498,2.19166588644357,11.4177362954637));
#68363=CARTESIAN_POINT('Ctrl Pts',(0.303837524600769,2.20896845452589,11.4187877654759));
#68364=CARTESIAN_POINT('Ctrl Pts',(0.296248992178024,2.22688325539048,11.4199695504907));
#68365=CARTESIAN_POINT('Ctrl Pts',(0.295740877035584,2.22806310725788,11.4200478176743));
#68366=CARTESIAN_POINT('Ctrl Pts',(0.295021468249988,2.22970646987592,11.4201574536801));
#68367=CARTESIAN_POINT('Ctrl Pts',(0.294816104463046,2.2301725762232,11.420188619804));
#68368=CARTESIAN_POINT('Ctrl Pts',(0.294459243057607,2.23097735473361,11.4202425532499));
#68369=CARTESIAN_POINT('Ctrl Pts',(0.294308263554812,2.23131625671087,11.4202653027877));
#68370=CARTESIAN_POINT('Ctrl Pts',(0.293994250533588,2.23201785639865,11.4203124773208));
#68371=CARTESIAN_POINT('Ctrl Pts',(0.293831130325233,2.23238051444411,11.4203369052638));
#68372=CARTESIAN_POINT('Ctrl Pts',(0.293447786975302,2.23322858578083,11.4203941317023));
#68373=CARTESIAN_POINT('Ctrl Pts',(0.293227030418377,2.23371375537482,11.4204269485085));
#68374=CARTESIAN_POINT('Ctrl Pts',(0.292523891044995,2.23524897073322,11.4205310402435));
#68375=CARTESIAN_POINT('Ctrl Pts',(0.292037067877216,2.23629696198534,11.4206024681837));
#68376=CARTESIAN_POINT('Ctrl Pts',(0.288152271303356,2.24454344936577,11.4211674933057));
#68377=CARTESIAN_POINT('Ctrl Pts',(0.284494553420535,2.25161586709843,11.421670086572));
#68378=CARTESIAN_POINT('Ctrl Pts',(0.277531053500126,2.26393924564599,11.4225795579248));
#68379=CARTESIAN_POINT('Ctrl Pts',(0.274328306406912,2.26924400883745,11.4229827547632));
#68380=CARTESIAN_POINT('Ctrl Pts',(0.260528830244049,2.29067850604845,11.4246598769326));
#68381=CARTESIAN_POINT('Ctrl Pts',(0.248647277148233,2.30593196769664,11.4259716245397));
#68382=CARTESIAN_POINT('Ctrl Pts',(0.232954964968058,2.32272578851382,11.4275234458375));
#68383=CARTESIAN_POINT('Ctrl Pts',(0.230389420628076,2.32537858867961,11.4277720321297));
#68384=CARTESIAN_POINT('Ctrl Pts',(0.220784360342617,2.33497488884179,11.4286826959563));
#68385=CARTESIAN_POINT('Ctrl Pts',(0.213471340959871,2.34163806224665,11.4293378125982));
#68386=CARTESIAN_POINT('Ctrl Pts',(0.203086352975509,2.35026012890085,11.4302055166265));
#68387=CARTESIAN_POINT('Ctrl Pts',(0.200271129216339,2.35251866542901,11.4304348499554));
#68388=CARTESIAN_POINT('Ctrl Pts',(0.196963062473938,2.35508245635267,11.4306970112674));
#68389=CARTESIAN_POINT('Ctrl Pts',(0.196506756064167,2.35543414484239,11.4307330143777));
#68390=CARTESIAN_POINT('Ctrl Pts',(0.19582686122584,2.35595525925136,11.4307864201857));
#68391=CARTESIAN_POINT('Ctrl Pts',(0.195603993844891,2.35612561744066,11.4308038884601));
#68392=CARTESIAN_POINT('Ctrl Pts',(0.195206675191319,2.3564285038407,11.4308349621622));
#68393=CARTESIAN_POINT('Ctrl Pts',(0.195032311319071,2.35656114507822,11.4308485756167));
#68394=CARTESIAN_POINT('Ctrl Pts',(0.194661882860758,2.35684233976215,11.4308774473053));
#68395=CARTESIAN_POINT('Ctrl Pts',(0.194465783973343,2.35699084613658,11.4308927021888));
#68396=CARTESIAN_POINT('Ctrl Pts',(0.194065529267228,2.35729323997252,11.4309237794022));
#68397=CARTESIAN_POINT('Ctrl Pts',(0.193861359922479,2.35744710935531,11.4309396004527));
#68398=CARTESIAN_POINT('Ctrl Pts',(0.192953573085077,2.35812955803287,11.431009806456));
#68399=CARTESIAN_POINT('Ctrl Pts',(0.192247966515316,2.35865550353666,11.4310640078875));
#68400=CARTESIAN_POINT('Ctrl Pts',(0.190511285100771,2.35993895967821,11.431196534431));
#68401=CARTESIAN_POINT('Ctrl Pts',(0.189477827138661,2.36069324052468,11.4312746445315));
#68402=CARTESIAN_POINT('Ctrl Pts',(0.185512878239694,2.36355106880785,11.4315715704013));
#68403=CARTESIAN_POINT('Ctrl Pts',(0.182550512776564,2.36561157079062,11.4317877151375));
#68404=CARTESIAN_POINT('Ctrl Pts',(0.175001473048611,2.37067640342882,11.4323260228765));
#68405=CARTESIAN_POINT('Ctrl Pts',(0.170371475048728,2.37361432270027,11.4326448646238));
#68406=CARTESIAN_POINT('Ctrl Pts',(0.151255883351461,2.38507045976688,11.4339253876778));
#68407=CARTESIAN_POINT('Ctrl Pts',(0.136189064409516,2.39256812394989,11.4348542788846));
#68408=CARTESIAN_POINT('Ctrl Pts',(0.108011185590584,2.40393948673635,11.4365572958474));
#68409=CARTESIAN_POINT('Ctrl Pts',(0.0951088359956848,2.40822053020989,
11.4373250345767));
#68410=CARTESIAN_POINT('Ctrl Pts',(0.0728200079417232,2.41408286838521,
11.4386679479792));
#68411=CARTESIAN_POINT('Ctrl Pts',(0.0635634144105625,2.41608617101461,
11.4392301645112));
#68412=CARTESIAN_POINT('Ctrl Pts',(0.0531026622613474,2.41787198223381,
11.4398755053916));
#68413=CARTESIAN_POINT('Ctrl Pts',(0.0519716139524046,2.41805886423508,
11.4399454082582));
#68414=CARTESIAN_POINT('Ctrl Pts',(0.0503262083653341,2.41832172197047,
11.4400472920871));
#68415=CARTESIAN_POINT('Ctrl Pts',(0.0498126174761309,2.41840249537629,
11.4400791208478));
#68416=CARTESIAN_POINT('Ctrl Pts',(0.0489065097601256,2.41854275464342,
11.4401353236783));
#68417=CARTESIAN_POINT('Ctrl Pts',(0.0485140732948712,2.41860275881235,
11.4401596812714));
#68418=CARTESIAN_POINT('Ctrl Pts',(0.0477031080657034,2.41872522362356,
11.4402100495519));
#68419=CARTESIAN_POINT('Ctrl Pts',(0.0472845653396324,2.41878758534633,
11.4402360633213));
#68420=CARTESIAN_POINT('Ctrl Pts',(0.0462139581986469,2.41894494808144,
11.4403026528132));
#68421=CARTESIAN_POINT('Ctrl Pts',(0.0455617253508072,2.41903877352418,
11.4403432656603));
#68422=CARTESIAN_POINT('Ctrl Pts',(0.0429493223209359,2.41940640033758,
11.4405061180151));
#68423=CARTESIAN_POINT('Ctrl Pts',(0.0409869685045067,2.41966413780157,
11.4406288641107));
#68424=CARTESIAN_POINT('Ctrl Pts',(0.0279561741863934,2.42125365595445,
11.4414468333331));
#68425=CARTESIAN_POINT('Ctrl Pts',(0.0168285981275828,2.42202827323941,
11.4421595293942));
#68426=CARTESIAN_POINT('Ctrl Pts',(-0.0118298918335914,2.42253382824022,
11.444032691079));
#68427=CARTESIAN_POINT('Ctrl Pts',(-0.0293384821624809,2.42141430629471,
11.4452145718946));
#68428=CARTESIAN_POINT('Ctrl Pts',(-0.0665240705506868,2.415972231577,11.4477578117019));
#68429=CARTESIAN_POINT('Ctrl Pts',(-0.0860683125025795,2.4112175228195,
11.449114888552));
#68430=CARTESIAN_POINT('Ctrl Pts',(-0.106121627391803,2.40430358617244,
11.4504519737043));
#68431=CARTESIAN_POINT('Ctrl Pts',(-0.10719622394402,2.40392670501595,11.4505234420489));
#68432=CARTESIAN_POINT('Ctrl Pts',(-0.108629373528265,2.40341552592135,
11.4506184916307));
#68433=CARTESIAN_POINT('Ctrl Pts',(-0.108989700695743,2.40328627946075,
11.4506423668456));
#68434=CARTESIAN_POINT('Ctrl Pts',(-0.109552188931617,2.40308338756261,
11.4506796011478));
#68435=CARTESIAN_POINT('Ctrl Pts',(-0.109754506487611,2.40301018171417,
11.450692986401));
#68436=CARTESIAN_POINT('Ctrl Pts',(-0.110142003605072,2.40286953215308,
11.4507186088649));
#68437=CARTESIAN_POINT('Ctrl Pts',(-0.110327193273273,2.40280212167267,
11.4507308479087));
#68438=CARTESIAN_POINT('Ctrl Pts',(-0.110764785458685,2.40264237997746,
11.4507597533917));
#68439=CARTESIAN_POINT('Ctrl Pts',(-0.111017134075308,2.40254990298973,
11.45077641097));
#68440=CARTESIAN_POINT('Ctrl Pts',(-0.1115392958736,2.4023578076107,11.4508108557249));
#68441=CARTESIAN_POINT('Ctrl Pts',(-0.111809092120167,2.40225814342697,
11.4508286401532));
#68442=CARTESIAN_POINT('Ctrl Pts',(-0.113289902190313,2.40170887024669,
11.4509261833984));
#68443=CARTESIAN_POINT('Ctrl Pts',(-0.114498360508774,2.40125233591932,
11.4510055335957));
#68444=CARTESIAN_POINT('Ctrl Pts',(-0.117660610527874,2.40003591596145,
11.4512125911184));
#68445=CARTESIAN_POINT('Ctrl Pts',(-0.119609823440329,2.39926419897227,
11.4513396346509));
#68446=CARTESIAN_POINT('Ctrl Pts',(-0.122305406930449,2.39816643981833,
11.4515146902266));
#68447=CARTESIAN_POINT('Ctrl Pts',(-0.123058231790622,2.39785652588867,
11.4515635107545));
#68448=CARTESIAN_POINT('Ctrl Pts',(-0.133771613180375,2.39339861862727,
11.4522573943448));
#68449=CARTESIAN_POINT('Ctrl Pts',(-0.143519862387249,2.38875540943751,
11.4528780562243));
#68450=CARTESIAN_POINT('Ctrl Pts',(-0.162018124310045,2.37877570012278,
11.4540683483744));
#68451=CARTESIAN_POINT('Ctrl Pts',(-0.170782634744406,2.3734941770556,11.4546382976379));
#68452=CARTESIAN_POINT('Ctrl Pts',(-0.191790201953743,2.35943070424253,
11.4560518017516));
#68453=CARTESIAN_POINT('Ctrl Pts',(-0.2036963572905,2.35019096949125,11.4568964773903));
#68454=CARTESIAN_POINT('Ctrl Pts',(-0.216439868090448,2.3387868502637,11.4578879684261));
#68455=CARTESIAN_POINT('Ctrl Pts',(-0.217954075312678,2.33740555422382,
11.4580072722552));
#68456=CARTESIAN_POINT('Ctrl Pts',(-0.221083807544876,2.33449535743689,
11.4582571241224));
#68457=CARTESIAN_POINT('Ctrl Pts',(-0.22269688148436,2.33296399135776,11.458387757009));
#68458=CARTESIAN_POINT('Ctrl Pts',(-0.229037555234947,2.3268184599815,11.4589089661364));
#68459=CARTESIAN_POINT('Ctrl Pts',(-0.233638391883418,2.3220763558671,11.4593045225998));
#68460=CARTESIAN_POINT('Ctrl Pts',(-0.238789550991669,2.31642967280185,
11.4597696920269));
#68461=CARTESIAN_POINT('Ctrl Pts',(-0.239485349140365,2.31565950115755,
11.4598330158626));
#68462=CARTESIAN_POINT('Ctrl Pts',(-0.240513890358391,2.31450990380329,
11.4599273612062));
#68463=CARTESIAN_POINT('Ctrl Pts',(-0.240849487050015,2.31413303077337,
11.4599582627578));
#68464=CARTESIAN_POINT('Ctrl Pts',(-0.241445193846402,2.31346088362359,
11.4600133267127));
#68465=CARTESIAN_POINT('Ctrl Pts',(-0.241705651510153,2.31316591776071,
11.4600374745164));
#68466=CARTESIAN_POINT('Ctrl Pts',(-0.242252365654404,2.3125444788454,11.4600883152048));
#68467=CARTESIAN_POINT('Ctrl Pts',(-0.242538503691286,2.31221790305502,
11.4601150129529));
#68468=CARTESIAN_POINT('Ctrl Pts',(-0.243117828666712,2.31155400434653,
11.4601692473874));
#68469=CARTESIAN_POINT('Ctrl Pts',(-0.243410975560251,2.31121664788614,
11.4601967856532));
#68470=CARTESIAN_POINT('Ctrl Pts',(-0.244133539122185,2.3103816122781,11.4602648989441));
#68471=CARTESIAN_POINT('Ctrl Pts',(-0.244562135298083,2.30988322867072,
11.4603055077896));
#68472=CARTESIAN_POINT('Ctrl Pts',(-0.248500652182109,2.30527496717996,
11.4606805967958));
#68473=CARTESIAN_POINT('Ctrl Pts',(-0.251908008977126,2.30107892873676,
11.461019251086));
#68474=CARTESIAN_POINT('Ctrl Pts',(-0.26349469955704,2.28605338878381,11.4622230154228));
#68475=CARTESIAN_POINT('Ctrl Pts',(-0.271093300244179,2.27479606001237,
11.4631099453408));
#68476=CARTESIAN_POINT('Ctrl Pts',(-0.280346600429231,2.25902582795637,
11.4643290027014));
#68477=CARTESIAN_POINT('Ctrl Pts',(-0.28264431077338,2.2549052030052,11.4646454138578));
#68478=CARTESIAN_POINT('Ctrl Pts',(-0.287116581784,2.24645379221042,11.4652892583565));
#68479=CARTESIAN_POINT('Ctrl Pts',(-0.289285605294081,2.24212136470088,
11.4656166806061));
#68480=CARTESIAN_POINT('Ctrl Pts',(-0.299422882711818,2.22067864346843,
11.467221393532));
#68481=CARTESIAN_POINT('Ctrl Pts',(-0.305975819114873,2.20293842151257,
11.4685028272173));
#68482=CARTESIAN_POINT('Ctrl Pts',(-0.311884705337857,2.18125305061516,
11.4699476056887));
#68483=CARTESIAN_POINT('Ctrl Pts',(-0.312772665988365,2.17776496481335,
11.4701763008842));
#68484=CARTESIAN_POINT('Ctrl Pts',(-0.313734693619783,2.17370243536213,
11.4704378110769));
#68485=CARTESIAN_POINT('Ctrl Pts',(-0.31386583448979,2.17314195041977,11.4704737836992));
#68486=CARTESIAN_POINT('Ctrl Pts',(-0.314058629481986,2.17230789382675,
11.4705271530946));
#68487=CARTESIAN_POINT('Ctrl Pts',(-0.314121428440611,2.17203459209038,
11.4705446153147));
#68488=CARTESIAN_POINT('Ctrl Pts',(-0.314232651272593,2.17154763791132,
11.4705756822835));
#68489=CARTESIAN_POINT('Ctrl Pts',(-0.314281213988249,2.17133401819357,
11.4705892950457));
#68490=CARTESIAN_POINT('Ctrl Pts',(-0.314383856272639,2.17088037158899,
11.4706181695613));
#68491=CARTESIAN_POINT('Ctrl Pts',(-0.314437878643613,2.17064033293045,
11.4706334279553));
#68492=CARTESIAN_POINT('Ctrl Pts',(-0.314547491622685,2.1701506702798,11.4706645136694));
#68493=CARTESIAN_POINT('Ctrl Pts',(-0.314603060113425,2.16990104144555,
11.4706803397064));
#68494=CARTESIAN_POINT('Ctrl Pts',(-0.314741085308612,2.16927749602512,
11.4707198186209));
#68495=CARTESIAN_POINT('Ctrl Pts',(-0.314823173155208,2.16890349689813,
11.4707434504841));
#68496=CARTESIAN_POINT('Ctrl Pts',(-0.315051943684686,2.16785225548443,
11.4708097444342));
#68497=CARTESIAN_POINT('Ctrl Pts',(-0.315197110005239,2.16717468018985,
11.4708523216657));
#68498=CARTESIAN_POINT('Ctrl Pts',(-0.315662529000211,2.16496757198191,
11.4709905310224));
#68499=CARTESIAN_POINT('Ctrl Pts',(-0.315973848210064,2.16343614972098,
11.4710856792933));
#68500=CARTESIAN_POINT('Ctrl Pts',(-0.320245880130619,2.1416093583186,11.4724319212824));
#68501=CARTESIAN_POINT('Ctrl Pts',(-0.322255880839034,2.12097861176568,
11.4735849954418));
#68502=CARTESIAN_POINT('Ctrl Pts',(-0.322274864254423,2.10029579518797,
11.4747410908026));
#68503=CARTESIAN_POINT('',(-0.322274879003935,2.09972073668561,11.7247944044677));
#68504=CARTESIAN_POINT('Ctrl Pts',(-0.322274864206818,2.10029584705048,
11.4747410879037));
#68505=CARTESIAN_POINT('Ctrl Pts',(-0.322300036387824,2.07287505241094,
11.4762738121076));
#68506=CARTESIAN_POINT('Ctrl Pts',(-0.318825877456706,2.04556637550985,
11.4778092777199));
#68507=CARTESIAN_POINT('Ctrl Pts',(-0.311694069518997,2.01809202581767,
11.4795321329028));
#68508=CARTESIAN_POINT('Ctrl Pts',(-0.311447100466804,2.01715790449816,
11.4795909126418));
#68509=CARTESIAN_POINT('Ctrl Pts',(-0.311046099801683,2.01566832345317,
11.4796849747927));
#68510=CARTESIAN_POINT('Ctrl Pts',(-0.310894770908584,2.01511213699265,
11.4797201697899));
#68511=CARTESIAN_POINT('Ctrl Pts',(-0.310602184302145,2.01404805620748,
11.4797876462982));
#68512=CARTESIAN_POINT('Ctrl Pts',(-0.310461170783618,2.01354009619816,
11.479819919803));
#68513=CARTESIAN_POINT('Ctrl Pts',(-0.310211858606244,2.01265049638237,
11.4798765510346));
#68514=CARTESIAN_POINT('Ctrl Pts',(-0.310104100144894,2.01226870528007,
11.4799008911412));
#68515=CARTESIAN_POINT('Ctrl Pts',(-0.309893757497413,2.01152868520873,
11.4799481386391));
#68516=CARTESIAN_POINT('Ctrl Pts',(-0.309791256362075,2.01117043309485,
11.479971043292));
#68517=CARTESIAN_POINT('Ctrl Pts',(-0.309517377810665,2.01021943878283,
11.4800319289907));
#68518=CARTESIAN_POINT('Ctrl Pts',(-0.309344919677988,2.00962701177772,
11.4800699452409));
#68519=CARTESIAN_POINT('Ctrl Pts',(-0.308726236192182,2.00752423567982,
11.4802051935106));
#68520=CARTESIAN_POINT('Ctrl Pts',(-0.308270647798801,2.00601668518114,
11.4803027310344));
#68521=CARTESIAN_POINT('Ctrl Pts',(-0.300012608945608,1.97939687465801,
11.4820353647899));
#68522=CARTESIAN_POINT('Ctrl Pts',(-0.289178276617797,1.95533480414639,
11.4837774849787));
#68523=CARTESIAN_POINT('Ctrl Pts',(-0.273220773402468,1.92902723115153,
11.4858578169994));
#68524=CARTESIAN_POINT('Ctrl Pts',(-0.27081570574098,1.92524264784903,11.4861614143527));
#68525=CARTESIAN_POINT('Ctrl Pts',(-0.266047539806185,1.91807445896218,
11.4867437230064));
#68526=CARTESIAN_POINT('Ctrl Pts',(-0.263696839886045,1.91468358601546,
11.4870224336136));
#68527=CARTESIAN_POINT('Ctrl Pts',(-0.255164453629505,1.90286687206271,
11.48800344053));
#68528=CARTESIAN_POINT('Ctrl Pts',(-0.248638295625961,1.89469680465762,
11.4886998085046));
#68529=CARTESIAN_POINT('Ctrl Pts',(-0.239451881133808,1.88427842600382,
11.4895986227768));
#68530=CARTESIAN_POINT('Ctrl Pts',(-0.23713633480027,1.88173556913315,11.4898188986773));
#68531=CARTESIAN_POINT('Ctrl Pts',(-0.233735433919225,1.87811883907701,
11.4901328964604));
#68532=CARTESIAN_POINT('Ctrl Pts',(-0.232682540074257,1.8770149368117,11.4902288313966));
#68533=CARTESIAN_POINT('Ctrl Pts',(-0.231411835578182,1.87570147306234,
11.4903430482569));
#68534=CARTESIAN_POINT('Ctrl Pts',(-0.231201541992224,1.87548471362899,
11.4903618996373));
#68535=CARTESIAN_POINT('Ctrl Pts',(-0.230835446840317,1.87510842205462,
11.4903946288729));
#68536=CARTESIAN_POINT('Ctrl Pts',(-0.230679784274552,1.87494875588769,
11.4904085174729));
#68537=CARTESIAN_POINT('Ctrl Pts',(-0.230367275548818,1.87462887440837,
11.4904363443925));
#68538=CARTESIAN_POINT('Ctrl Pts',(-0.230210427414233,1.874468660703,11.4904502825807));
#68539=CARTESIAN_POINT('Ctrl Pts',(-0.229909974599999,1.87416240092585,
11.4904769280684));
#68540=CARTESIAN_POINT('Ctrl Pts',(-0.229766398081505,1.87401632826821,
11.4904896375556));
#68541=CARTESIAN_POINT('Ctrl Pts',(-0.22942816148061,1.87367286685185,11.4905195234819));
#68542=CARTESIAN_POINT('Ctrl Pts',(-0.229233385390726,1.87347559181608,
11.4905366907478));
#68543=CARTESIAN_POINT('Ctrl Pts',(-0.22865820303797,1.87289453153451,11.4905872613698));
#68544=CARTESIAN_POINT('Ctrl Pts',(-0.228277083400759,1.87251144901886,
11.4906206088896));
#68545=CARTESIAN_POINT('Ctrl Pts',(-0.224963595263786,1.86919760720726,
11.4909091629549));
#68546=CARTESIAN_POINT('Ctrl Pts',(-0.221975723413425,1.86632256018818,
11.4911600707356));
#68547=CARTESIAN_POINT('Ctrl Pts',(-0.218668300037411,1.86326073344151,
11.4914290154668));
#68548=CARTESIAN_POINT('Ctrl Pts',(-0.218403152916785,1.86301610060982,
11.4914505158638));
#68549=CARTESIAN_POINT('Ctrl Pts',(-0.217945850173143,1.86259559846163,
11.4914874955826));
#68550=CARTESIAN_POINT('Ctrl Pts',(-0.217753891632086,1.86241951646358,
11.4915029873584));
#68551=CARTESIAN_POINT('Ctrl Pts',(-0.205505824868496,1.85121177942031,
11.492489499747));
#68552=CARTESIAN_POINT('Ctrl Pts',(-0.192626928169415,1.84111159791732,
11.4934071571877));
#68553=CARTESIAN_POINT('Ctrl Pts',(-0.168119893824159,1.82473788067897,
11.4950559483026));
#68554=CARTESIAN_POINT('Ctrl Pts',(-0.156768373938024,1.81811847014041,
11.4957866415096));
#68555=CARTESIAN_POINT('Ctrl Pts',(-0.134914282452979,1.80710408576295,
11.4971779421657));
#68556=CARTESIAN_POINT('Ctrl Pts',(-0.124521756421104,1.8025371014388,11.4978335105095));
#68557=CARTESIAN_POINT('Ctrl Pts',(-0.110577280362001,1.79726820581965,
11.4987189037373));
#68558=CARTESIAN_POINT('Ctrl Pts',(-0.107223247718585,1.79606407288629,
11.4989322532449));
#68559=CARTESIAN_POINT('Ctrl Pts',(-0.101718662701923,1.79419032324544,
11.4992833833423));
#68560=CARTESIAN_POINT('Ctrl Pts',(-0.0995797905910993,1.79348717865874,
11.499420057571));
#68561=CARTESIAN_POINT('Ctrl Pts',(-0.0969471876172316,1.79265218560044,
11.4995886273974));
#68562=CARTESIAN_POINT('Ctrl Pts',(-0.0964602437650322,1.792499012081,11.4996198216239));
#68563=CARTESIAN_POINT('Ctrl Pts',(-0.0955151720130558,1.79220419514818,
11.4996803929389));
#68564=CARTESIAN_POINT('Ctrl Pts',(-0.0950570876118069,1.79206241596736,
11.4997097654923));
#68565=CARTESIAN_POINT('Ctrl Pts',(-0.0942607389623816,1.79181788874921,
11.4997608510882));
#68566=CARTESIAN_POINT('Ctrl Pts',(-0.0939226180269496,1.79171467367697,
11.4997825487915));
#68567=CARTESIAN_POINT('Ctrl Pts',(-0.0932182483540775,1.79150092357473,
11.49982776472));
#68568=CARTESIAN_POINT('Ctrl Pts',(-0.0928519714335364,1.7913904839763,
11.499851286029));
#68569=CARTESIAN_POINT('Ctrl Pts',(-0.0919566267182979,1.79112225843007,
11.499908804359));
#68570=CARTESIAN_POINT('Ctrl Pts',(-0.0914273498627072,1.7909651797519,
11.4999428244338));
#68571=CARTESIAN_POINT('Ctrl Pts',(-0.0894075920349929,1.79037139932322,
11.5000727198406));
#68572=CARTESIAN_POINT('Ctrl Pts',(-0.0879143836163184,1.78994411973268,
11.5001689018952));
#68573=CARTESIAN_POINT('Ctrl Pts',(-0.0626760899065705,1.78291918791218,
11.5017972692741));
#68574=CARTESIAN_POINT('Ctrl Pts',(-0.0382595575110669,1.77905724232482,
11.5034224355678));
#68575=CARTESIAN_POINT('Ctrl Pts',(0.00195367112345285,1.77735286556368,
11.5061395770682));
#68576=CARTESIAN_POINT('Ctrl Pts',(0.017581956956381,1.77782630548259,11.5072028867821));
#68577=CARTESIAN_POINT('Ctrl Pts',(0.0424096820951024,1.78039099817006,
11.5088581357477));
#68578=CARTESIAN_POINT('Ctrl Pts',(0.0516596151429787,1.78175509859245,
11.5094668303981));
#68579=CARTESIAN_POINT('Ctrl Pts',(0.0617159469430251,1.78368826036074,
11.5101106670232));
#68580=CARTESIAN_POINT('Ctrl Pts',(0.0625931131909332,1.78386066842813,
11.5101666741714));
#68581=CARTESIAN_POINT('Ctrl Pts',(0.0637222040510651,1.7840874761284,11.5102385611435));
#68582=CARTESIAN_POINT('Ctrl Pts',(0.0639747852367891,1.78413852896711,
11.5102546292145));
#68583=CARTESIAN_POINT('Ctrl Pts',(0.0644697565418142,1.78423919285321,
11.5102860906599));
#68584=CARTESIAN_POINT('Ctrl Pts',(0.0647121512356568,1.7842887801772,11.5103014853775));
#68585=CARTESIAN_POINT('Ctrl Pts',(0.0651688274105437,1.78438275166764,
11.5103304656057));
#68586=CARTESIAN_POINT('Ctrl Pts',(0.0653831190488537,1.7844270745854,11.5103440544618));
#68587=CARTESIAN_POINT('Ctrl Pts',(0.0658697065494724,1.78452823460986,
11.5103748881207));
#68588=CARTESIAN_POINT('Ctrl Pts',(0.0661419735546816,1.78458520590344,
11.5103921250876));
#68589=CARTESIAN_POINT('Ctrl Pts',(0.0669663848953701,1.78475882662979,
11.510444270816));
#68590=CARTESIAN_POINT('Ctrl Pts',(0.0675183006269034,1.78487657467964,
11.5104791167787));
#68591=CARTESIAN_POINT('Ctrl Pts',(0.0713664729464188,1.78570813412444,
11.5107216487909));
#68592=CARTESIAN_POINT('Ctrl Pts',(0.0746518098132963,1.78647223426109,
11.5109265173873));
#68593=CARTESIAN_POINT('Ctrl Pts',(0.0923436990885821,1.79088087327393,
11.5120208548015));
#68594=CARTESIAN_POINT('Ctrl Pts',(0.106498699583136,1.79546736880027,11.5128647754025));
#68595=CARTESIAN_POINT('Ctrl Pts',(0.136216340816891,1.80742340489367,11.5146633473693));
#68596=CARTESIAN_POINT('Ctrl Pts',(0.151606717232641,1.81509414483439,11.5156128191301));
#68597=CARTESIAN_POINT('Ctrl Pts',(0.17245749060505,1.82765636836675,11.5170013797609));
#68598=CARTESIAN_POINT('Ctrl Pts',(0.17847664634258,1.8315624515842,11.5174151494616));
#68599=CARTESIAN_POINT('Ctrl Pts',(0.191008502118423,1.84030281480634,11.5183104835166));
#68600=CARTESIAN_POINT('Ctrl Pts',(0.197479005921777,1.84518849907411,11.5187935646229));
#68601=CARTESIAN_POINT('Ctrl Pts',(0.204638500756096,1.85103102420079,11.5193555072261));
#68602=CARTESIAN_POINT('Ctrl Pts',(0.205515085251483,1.85175412070992,11.5194247946692));
#68603=CARTESIAN_POINT('Ctrl Pts',(0.206795589068756,1.85282184188117,11.5195267314757));
#68604=CARTESIAN_POINT('Ctrl Pts',(0.207202516891855,1.85316285835057,11.5195592336723));
#68605=CARTESIAN_POINT('Ctrl Pts',(0.207912485053595,1.85376082350786,11.519616130392));
#68606=CARTESIAN_POINT('Ctrl Pts',(0.208215897196949,1.85401733062496,11.5196405067851));
#68607=CARTESIAN_POINT('Ctrl Pts',(0.208802151316757,1.85451481653447,11.5196877255656));
#68608=CARTESIAN_POINT('Ctrl Pts',(0.209085052539872,1.8547557248411,11.5197105650311));
#68609=CARTESIAN_POINT('Ctrl Pts',(0.209756402796594,1.85532942809465,11.5197648933318));
#68610=CARTESIAN_POINT('Ctrl Pts',(0.210144476511901,1.85566265889679,11.5197964001392));
#68611=CARTESIAN_POINT('Ctrl Pts',(0.211514048391049,1.85684435807869,11.519907956616));
#68612=CARTESIAN_POINT('Ctrl Pts',(0.212491204601813,1.85769781933947,11.5199882132454));
#68613=CARTESIAN_POINT('Ctrl Pts',(0.228594145571592,1.87193466580153,11.5213219443861));
#68614=CARTESIAN_POINT('Ctrl Pts',(0.24243115815712,1.88670223451989,11.5226363767671));
#68615=CARTESIAN_POINT('Ctrl Pts',(0.265174715581445,1.91606804183148,11.5251235949813));
#68616=CARTESIAN_POINT('Ctrl Pts',(0.274481470815994,1.93026934932985,11.5262803806405));
#68617=CARTESIAN_POINT('Ctrl Pts',(0.287252231163573,1.95357615037385,11.5280619158883));
#68618=CARTESIAN_POINT('Ctrl Pts',(0.291496720035063,1.9622194415589,11.5286991731304));
#68619=CARTESIAN_POINT('Ctrl Pts',(0.296337184543605,1.97330526426592,11.5294769840491));
#68620=CARTESIAN_POINT('Ctrl Pts',(0.297300039901078,1.97558147194635,11.5296346488267));
#68621=CARTESIAN_POINT('Ctrl Pts',(0.298786006309718,1.97921010199178,11.5298825157586));
#68622=CARTESIAN_POINT('Ctrl Pts',(0.299326318979447,1.98055531832086,11.5299736556224));
#68623=CARTESIAN_POINT('Ctrl Pts',(0.300008135942414,1.98228652215027,11.5300899439757));
#68624=CARTESIAN_POINT('Ctrl Pts',(0.300157993173823,1.98266917013226,11.530115584587));
#68625=CARTESIAN_POINT('Ctrl Pts',(0.300396822814261,1.98328245386878,11.5301565783158));
#68626=CARTESIAN_POINT('Ctrl Pts',(0.300486261856708,1.98351290557249,11.5301719595071));
#68627=CARTESIAN_POINT('Ctrl Pts',(0.300654388543525,1.98394758866713,11.5302009283933));
#68628=CARTESIAN_POINT('Ctrl Pts',(0.300733132652277,1.98415179564563,11.5302145194011));
#68629=CARTESIAN_POINT('Ctrl Pts',(0.300911608721305,1.98461604561564,11.5302453766564));
#68630=CARTESIAN_POINT('Ctrl Pts',(0.301011211464575,1.98487613728402,11.5302626350216));
#68631=CARTESIAN_POINT('Ctrl Pts',(0.301312228593085,1.98566524174221,11.5303149086718));
#68632=CARTESIAN_POINT('Ctrl Pts',(0.301512587849395,1.9861946599431,11.5303498607029));
#68633=CARTESIAN_POINT('Ctrl Pts',(0.302909493931732,1.98991535069655,11.5305946840036));
#68634=CARTESIAN_POINT('Ctrl Pts',(0.304056802264673,1.9931250507782,11.5308016771025));
#68635=CARTESIAN_POINT('Ctrl Pts',(0.30835246401238,2.0057720920444,11.531603122784));
#68636=CARTESIAN_POINT('Ctrl Pts',(0.311114334807051,2.01533567591138,11.5321786276792));
#68637=CARTESIAN_POINT('Ctrl Pts',(0.318089201093232,2.04448893066623,11.5338836486623));
#68638=CARTESIAN_POINT('Ctrl Pts',(0.320923469273321,2.06435747231275,11.5349826079845));
#68639=CARTESIAN_POINT('Ctrl Pts',(0.322651337208529,2.09992202811594,11.5370016500021));
#68640=CARTESIAN_POINT('Ctrl Pts',(0.322277938761377,2.11551537065162,11.5379040195773));
#68641=CARTESIAN_POINT('Ctrl Pts',(0.320542517469727,2.13346179084894,11.5389915232467));
#68642=CARTESIAN_POINT('Ctrl Pts',(0.320278449922763,2.13590140601419,11.5391403776386));
#68643=CARTESIAN_POINT('Ctrl Pts',(0.319901635130056,2.13904649854756,11.5393336711109));
#68644=CARTESIAN_POINT('Ctrl Pts',(0.319814361532946,2.13975499153655,11.5393773056542));
#68645=CARTESIAN_POINT('Ctrl Pts',(0.319670068310917,2.14089514185,11.5394476743335));
#68646=CARTESIAN_POINT('Ctrl Pts',(0.319614526238513,2.14132698652482,11.5394743617711));
#68647=CARTESIAN_POINT('Ctrl Pts',(0.31950715678073,2.14214863011245,11.5395252044871));
#68648=CARTESIAN_POINT('Ctrl Pts',(0.31945549072856,2.14253844961513,11.5395493546247));
#68649=CARTESIAN_POINT('Ctrl Pts',(0.319336190075152,2.14342609513884,11.5396044112339));
#68650=CARTESIAN_POINT('Ctrl Pts',(0.319268104684871,2.14392385863166,11.539635331907));
#68651=CARTESIAN_POINT('Ctrl Pts',(0.319057339008716,2.14543835556062,11.5397295545003));
#68652=CARTESIAN_POINT('Ctrl Pts',(0.318910964799818,2.1464545608391,11.5397929731253));
#68653=CARTESIAN_POINT('Ctrl Pts',(0.317822100641731,2.15376624741762,11.5402507139636));
#68654=CARTESIAN_POINT('Ctrl Pts',(0.316698182763316,2.16003289707887,11.5406507583335));
#68655=CARTESIAN_POINT('Ctrl Pts',(0.315175392709095,2.16728099301359,11.5411229586531));
#68656=CARTESIAN_POINT('Ctrl Pts',(0.314956332180802,2.16829911397336,11.5411895062166));
#68657=CARTESIAN_POINT('Ctrl Pts',(0.314119814477821,2.17209735134805,11.5414385905456));
#68658=CARTESIAN_POINT('Ctrl Pts',(0.31347046354994,2.17487024517658,11.541622078546));
#68659=CARTESIAN_POINT('Ctrl Pts',(0.311389630989868,2.18325383010857,11.5421818236745));
#68660=CARTESIAN_POINT('Ctrl Pts',(0.309843664500307,2.1888346787487,11.5425612800199));
#68661=CARTESIAN_POINT('Ctrl Pts',(0.301398072630265,2.21641206096363,11.5444690840411));
#68662=CARTESIAN_POINT('Ctrl Pts',(0.292302442066179,2.2376652227163,11.5460507612595));
#68663=CARTESIAN_POINT('Ctrl Pts',(0.275853287058625,2.26696557423439,11.5482939167655));
#68664=CARTESIAN_POINT('Ctrl Pts',(0.270237857399356,2.27590931943745,11.548986980369));
#68665=CARTESIAN_POINT('Ctrl Pts',(0.263625931597988,2.28537401226372,11.5497170074157));
#68666=CARTESIAN_POINT('Ctrl Pts',(0.263055078675454,2.28618319439693,11.5497793911423));
#68667=CARTESIAN_POINT('Ctrl Pts',(0.26206333046707,2.28757532722642,11.5498866475975));
#68668=CARTESIAN_POINT('Ctrl Pts',(0.261644201190781,2.28815951893643,11.549931635104));
#68669=CARTESIAN_POINT('Ctrl Pts',(0.261043913400579,2.28899032919334,11.5499955779287));
#68670=CARTESIAN_POINT('Ctrl Pts',(0.260864357140167,2.28923809454706,11.5500146424192));
#68671=CARTESIAN_POINT('Ctrl Pts',(0.260552727305522,2.28966681867745,11.5500476223554));
#68672=CARTESIAN_POINT('Ctrl Pts',(0.260420817620313,2.28984789586578,11.5500615492034));
#68673=CARTESIAN_POINT('Ctrl Pts',(0.26016782755644,2.29019442463864,11.5500881958069));
#68674=CARTESIAN_POINT('Ctrl Pts',(0.260046778287583,2.29035989798773,11.5501009177061));
#68675=CARTESIAN_POINT('Ctrl Pts',(0.259761206078221,2.29074949210748,11.5501308652863));
#68676=CARTESIAN_POINT('Ctrl Pts',(0.259596550546737,2.2909735161431,11.5501480816996));
#68677=CARTESIAN_POINT('Ctrl Pts',(0.259109177083391,2.29163482287312,11.5501988926499));
#68678=CARTESIAN_POINT('Ctrl Pts',(0.258785640650641,2.29207150540782,11.5502324305982));
#68679=CARTESIAN_POINT('Ctrl Pts',(0.255933988083595,2.29590014305912,11.5505263717919));
#68680=CARTESIAN_POINT('Ctrl Pts',(0.253340269676402,2.29924302811231,11.5507822974457));
#68681=CARTESIAN_POINT('Ctrl Pts',(0.250496953269214,2.30276226991565,11.5510521042505));
#68682=CARTESIAN_POINT('Ctrl Pts',(0.250312264312243,2.30299022645092,11.551069582536));
#68683=CARTESIAN_POINT('Ctrl Pts',(0.250049060513017,2.30331418627907,11.5510944247329));
#68684=CARTESIAN_POINT('Ctrl Pts',(0.249970801676966,2.3034103962801,11.5511018027744));
#68685=CARTESIAN_POINT('Ctrl Pts',(0.248304773843184,2.30545616736796,11.551258695054));
#68686=CARTESIAN_POINT('Ctrl Pts',(0.246694255513354,2.30738717995559,11.5514069518324));
#68687=CARTESIAN_POINT('Ctrl Pts',(0.228128425389095,2.32912527432822,11.5530803943711));
#68688=CARTESIAN_POINT('Ctrl Pts',(0.208850918622891,2.34682490214154,11.5544926725794));
#68689=CARTESIAN_POINT('Ctrl Pts',(0.174907822703956,2.37113475499553,11.5568594392085));
#68690=CARTESIAN_POINT('Ctrl Pts',(0.161519081643916,2.37931754651797,11.5577669120608));
#68691=CARTESIAN_POINT('Ctrl Pts',(0.145399318262787,2.38762177142336,11.5588605686963));
#68692=CARTESIAN_POINT('Ctrl Pts',(0.143196393845611,2.38872484724655,11.5590100136225));
#68693=CARTESIAN_POINT('Ctrl Pts',(0.140338885087336,2.39011494787469,11.5592039233685));
#68694=CARTESIAN_POINT('Ctrl Pts',(0.139695652374363,2.39042522332378,11.5592475766606));
#68695=CARTESIAN_POINT('Ctrl Pts',(0.138658546069605,2.39092124855844,11.559317968341));
#68696=CARTESIAN_POINT('Ctrl Pts',(0.13826531554256,2.39110834370712,11.5593446599755));
#68697=CARTESIAN_POINT('Ctrl Pts',(0.137516293855436,2.39146286069906,11.5593955059471));
#68698=CARTESIAN_POINT('Ctrl Pts',(0.137160572858918,2.39163042964247,11.559419655133));
#68699=CARTESIAN_POINT('Ctrl Pts',(0.136349773670778,2.39201055995282,11.5594747030017));
#68700=CARTESIAN_POINT('Ctrl Pts',(0.135894504258505,2.39222270892559,11.5595056158694));
#68701=CARTESIAN_POINT('Ctrl Pts',(0.134507686132918,2.39286500440821,11.5595997916401));
#68702=CARTESIAN_POINT('Ctrl Pts',(0.13357458417131,2.39329176405129,11.5596631710777));
#68703=CARTESIAN_POINT('Ctrl Pts',(0.126850040042698,2.39632852698699,11.5601200505271));
#68704=CARTESIAN_POINT('Ctrl Pts',(0.12098493897138,2.39877108937195,11.5605192484609));
#68705=CARTESIAN_POINT('Ctrl Pts',(0.112561613054045,2.40199034050775,11.5610941373801));
#68706=CARTESIAN_POINT('Ctrl Pts',(0.110059756970473,2.40291109542363,11.5612650743948));
#68707=CARTESIAN_POINT('Ctrl Pts',(0.0790684922863867,2.41388214388985,
11.5633848410861));
#68708=CARTESIAN_POINT('Ctrl Pts',(0.0493160837766237,2.41990805106609,
11.5654644547761));
#68709=CARTESIAN_POINT('Ctrl Pts',(0.00779220350546494,2.4223823083516,
11.5682405252315));
#68710=CARTESIAN_POINT('Ctrl Pts',(-0.00361422939399656,2.4224563113289,
11.5689876574152));
#68711=CARTESIAN_POINT('Ctrl Pts',(-0.0157565970924718,2.42189047226933,
11.5697506937988));
#68712=CARTESIAN_POINT('Ctrl Pts',(-0.0165112169790477,2.42185264676695,
11.569797980487));
#68713=CARTESIAN_POINT('Ctrl Pts',(-0.0175786983845659,2.42179537478719,
11.5698646753597));
#68714=CARTESIAN_POINT('Ctrl Pts',(-0.0178916678621757,2.42177812556858,
11.5698842053705));
#68715=CARTESIAN_POINT('Ctrl Pts',(-0.0184285035061297,2.42174775239437,
11.5699176635231));
#68716=CARTESIAN_POINT('Ctrl Pts',(-0.0186523816238351,2.42173485134996,
11.5699316042519));
#68717=CARTESIAN_POINT('Ctrl Pts',(-0.0190806710450227,2.42170972249897,
11.5699582495359));
#68718=CARTESIAN_POINT('Ctrl Pts',(-0.0192850838892537,2.42169753355886,
11.5699709562888));
#68719=CARTESIAN_POINT('Ctrl Pts',(-0.0197660285946986,2.4216683952385,
11.5700008286008));
#68720=CARTESIAN_POINT('Ctrl Pts',(-0.0200425510249569,2.4216512840507,
11.5700179850077));
#68721=CARTESIAN_POINT('Ctrl Pts',(-0.0208576627637052,2.42159978978246,
11.5700685025891));
#68722=CARTESIAN_POINT('Ctrl Pts',(-0.0213961915499814,2.42156441015942,
11.5701018080924));
#68723=CARTESIAN_POINT('Ctrl Pts',(-0.0260523959849527,2.42124676367071,
11.5703891825053));
#68724=CARTESIAN_POINT('Ctrl Pts',(-0.0301646190358144,2.42088675597886,
11.5706389913146));
#68725=CARTESIAN_POINT('Ctrl Pts',(-0.063066890822936,2.4173681530483,11.5726137822695));
#68726=CARTESIAN_POINT('Ctrl Pts',(-0.0913219801422467,2.41042029982934,
11.5741721611729));
#68727=CARTESIAN_POINT('Ctrl Pts',(-0.132986146390127,2.39398315379957,
11.5767100861028));
#68728=CARTESIAN_POINT('Ctrl Pts',(-0.147251921351612,2.38710308795363,
11.5776255706286));
#68729=CARTESIAN_POINT('Ctrl Pts',(-0.163107234313584,2.37796291748983,
11.5787292850434));
#68730=CARTESIAN_POINT('Ctrl Pts',(-0.165246085137236,2.37669673687579,
11.5788800525975));
#68731=CARTESIAN_POINT('Ctrl Pts',(-0.1679778548328,2.37503658267105,11.5790751253761));
#68732=CARTESIAN_POINT('Ctrl Pts',(-0.16858445010462,2.37466518653035,11.5791186025966));
#68733=CARTESIAN_POINT('Ctrl Pts',(-0.169559890647617,2.37406351121688,
11.5791887782749));
#68734=CARTESIAN_POINT('Ctrl Pts',(-0.169929510345819,2.37383448688515,
11.5792154304981));
#68735=CARTESIAN_POINT('Ctrl Pts',(-0.170632616863394,2.37339685517219,
11.5792662460395));
#68736=CARTESIAN_POINT('Ctrl Pts',(-0.170966187720178,2.37318838373902,
11.5792904043049));
#68737=CARTESIAN_POINT('Ctrl Pts',(-0.171725830636405,2.37271169427819,
11.5793455349365));
#68738=CARTESIAN_POINT('Ctrl Pts',(-0.172151656749483,2.3724430879609,11.5793765216458));
#68739=CARTESIAN_POINT('Ctrl Pts',(-0.173448450451586,2.37162083089572,
11.5794711408778));
#68740=CARTESIAN_POINT('Ctrl Pts',(-0.174317383146928,2.37106399730259,
11.5795348915516));
#68741=CARTESIAN_POINT('Ctrl Pts',(-0.180621804251176,2.36698111733284,
11.5800000019099));
#68742=CARTESIAN_POINT('Ctrl Pts',(-0.185952200698111,2.36329626357821,
11.5804072932857));
#68743=CARTESIAN_POINT('Ctrl Pts',(-0.192610371048218,2.35839046437724,
11.5809348582146));
#68744=CARTESIAN_POINT('Ctrl Pts',(-0.194044190173149,2.35731544682622,
11.5810496175182));
#68745=CARTESIAN_POINT('Ctrl Pts',(-0.200437187080528,2.35243842432353,
11.5815664929444));
#68746=CARTESIAN_POINT('Ctrl Pts',(-0.205293871926056,2.34850481347523,
11.581973364511));
#68747=CARTESIAN_POINT('Ctrl Pts',(-0.218592929113318,2.33707737508756,
11.5831275501657));
#68748=CARTESIAN_POINT('Ctrl Pts',(-0.226760106438218,2.32927793946239,
11.58388435836));
#68749=CARTESIAN_POINT('Ctrl Pts',(-0.245321299615967,2.30958878761414,
11.5857118133949));
#68750=CARTESIAN_POINT('Ctrl Pts',(-0.255284670277783,2.29733161726445,
11.5867857237935));
#68751=CARTESIAN_POINT('Ctrl Pts',(-0.267955254158262,2.27916956648074,
11.5882511730193));
#68752=CARTESIAN_POINT('Ctrl Pts',(-0.271444472905799,2.27383803183175,
11.588667332731));
#68753=CARTESIAN_POINT('Ctrl Pts',(-0.276342307012434,2.26584666768287,
11.5892670505577));
#68754=CARTESIAN_POINT('Ctrl Pts',(-0.277875262406565,2.26326520744194,
11.5894572100316));
#68755=CARTESIAN_POINT('Ctrl Pts',(-0.27962410035098,2.26022419878823,11.5896767470799));
#68756=CARTESIAN_POINT('Ctrl Pts',(-0.279875183294306,2.25978520944908,
11.5897083308891));
#68757=CARTESIAN_POINT('Ctrl Pts',(-0.280256781289631,2.25911437066009,
11.5897564290526));
#68758=CARTESIAN_POINT('Ctrl Pts',(-0.280388042836235,2.25888295013964,
11.5897729914233));
#68759=CARTESIAN_POINT('Ctrl Pts',(-0.280615898526883,2.25848006766776,
11.5898017722693));
#68760=CARTESIAN_POINT('Ctrl Pts',(-0.280712621932126,2.25830868025067,
11.5898139991277));
#68761=CARTESIAN_POINT('Ctrl Pts',(-0.280931057294658,2.25792079772892,
11.5898416332746));
#68762=CARTESIAN_POINT('Ctrl Pts',(-0.281052675761352,2.25770425091423,
11.5898570344523));
#68763=CARTESIAN_POINT('Ctrl Pts',(-0.281381518936521,2.25711714318444,
11.5898987196739));
#68764=CARTESIAN_POINT('Ctrl Pts',(-0.281588262819436,2.2567463113719,11.5899249726992));
#68765=CARTESIAN_POINT('Ctrl Pts',(-0.282513225566171,2.25507949065013,
11.5900426375257));
#68766=CARTESIAN_POINT('Ctrl Pts',(-0.283223249255329,2.25377893977755,
11.5901335315008));
#68767=CARTESIAN_POINT('Ctrl Pts',(-0.297898443549344,2.22645193587756,
11.5920252812356));
#68768=CARTESIAN_POINT('Ctrl Pts',(-0.30823167155431,2.19862796003161,11.593618310384));
#68769=CARTESIAN_POINT('Ctrl Pts',(-0.318520117292683,2.15223947607352,
11.5962955128742));
#68770=CARTESIAN_POINT('Ctrl Pts',(-0.320936382997456,2.13440545864712,
11.5973276698267));
#68771=CARTESIAN_POINT('Ctrl Pts',(-0.321990560442423,2.11379795139737,
11.5985708108872));
#68772=CARTESIAN_POINT('Ctrl Pts',(-0.322093819741655,2.11112991915533,
11.5987326684898));
#68773=CARTESIAN_POINT('Ctrl Pts',(-0.322183069083759,2.10773161967271,
11.5989400820847));
#68774=CARTESIAN_POINT('Ctrl Pts',(-0.322199747055235,2.10700220899107,
11.5989846747466));
#68775=CARTESIAN_POINT('Ctrl Pts',(-0.32222249118166,2.10583390614677,11.5990562189057));
#68776=CARTESIAN_POINT('Ctrl Pts',(-0.322230137909884,2.1053950443746,11.5990831208393));
#68777=CARTESIAN_POINT('Ctrl Pts',(-0.322242924628796,2.10456368619702,
11.5991341343135));
#68778=CARTESIAN_POINT('Ctrl Pts',(-0.322248244140542,2.10417119301832,
11.5991582401835));
#68779=CARTESIAN_POINT('Ctrl Pts',(-0.322258664822077,2.1032825008821,11.5992128711703));
#68780=CARTESIAN_POINT('Ctrl Pts',(-0.322263337039576,2.10278629874118,
11.5992434096704));
#68781=CARTESIAN_POINT('Ctrl Pts',(-0.32227239197695,2.1015120666034,11.5993219230351));
#68782=CARTESIAN_POINT('Ctrl Pts',(-0.322275103222484,2.10073403126868,
11.5993699501528));
#68783=CARTESIAN_POINT('Ctrl Pts',(-0.322274377752403,2.09542047604823,
11.599698555776));
#68784=CARTESIAN_POINT('Ctrl Pts',(-0.322178013225252,2.09088567023784,
11.5999820311716));
#68785=CARTESIAN_POINT('Ctrl Pts',(-0.321605378908561,2.07737342051489,
11.6008362740597));
#68786=CARTESIAN_POINT('Ctrl Pts',(-0.320849202675792,2.06841288027864,
11.6014155175924));
#68787=CARTESIAN_POINT('Ctrl Pts',(-0.315383956854345,2.02527246823403,
11.6042653785859));
#68788=CARTESIAN_POINT('Ctrl Pts',(-0.305582855616318,1.99197271155528,
11.606682232021));
#68789=CARTESIAN_POINT('Ctrl Pts',(-0.289313275863257,1.95798168310811,
11.6090977647223));
#68790=CARTESIAN_POINT('Ctrl Pts',(-0.287891731459744,1.95512168285173,
11.6093003244147));
#68791=CARTESIAN_POINT('Ctrl Pts',(-0.286176650735651,1.95179608461336,
11.6095346450617));
#68792=CARTESIAN_POINT('Ctrl Pts',(-0.285924213285312,1.95130964984272,
11.6095688883125));
#68793=CARTESIAN_POINT('Ctrl Pts',(-0.285541569005008,1.95057689061059,
11.6096204226893));
#68794=CARTESIAN_POINT('Ctrl Pts',(-0.285412283173555,1.95033009031703,
11.6096377715127));
#68795=CARTESIAN_POINT('Ctrl Pts',(-0.285180860618937,1.94988970632409,
11.6096687127855));
#68796=CARTESIAN_POINT('Ctrl Pts',(-0.285078846836794,1.94969605920642,
11.6096823129997));
#68797=CARTESIAN_POINT('Ctrl Pts',(-0.284861226729738,1.94928398158569,
11.6097112424425));
#68798=CARTESIAN_POINT('Ctrl Pts',(-0.284745566745866,1.9490655807306,11.6097265681452));
#68799=CARTESIAN_POINT('Ctrl Pts',(-0.284433101514647,1.94847718979725,
11.6097678389454));
#68800=CARTESIAN_POINT('Ctrl Pts',(-0.284235824768456,1.94810744859642,
11.609793754071));
#68801=CARTESIAN_POINT('Ctrl Pts',(-0.283270702998693,1.94630705681918,
11.609919854892));
#68802=CARTESIAN_POINT('Ctrl Pts',(-0.282492757320223,1.94488180544531,
11.6100194078714));
#68803=CARTESIAN_POINT('Ctrl Pts',(-0.277953886764267,1.93671368019125,
11.6105887253818));
#68804=CARTESIAN_POINT('Ctrl Pts',(-0.273962069616423,1.93010123335591,
11.6110448102347));
#68805=CARTESIAN_POINT('Ctrl Pts',(-0.261347311798038,1.91080763514703,
11.6123804553721));
#68806=CARTESIAN_POINT('Ctrl Pts',(-0.252053084280766,1.89859127761922,
11.6132334581119));
#68807=CARTESIAN_POINT('Ctrl Pts',(-0.232263507153112,1.8761057188586,11.6149079425629));
#68808=CARTESIAN_POINT('Ctrl Pts',(-0.221867601011758,1.86579983858226,
11.6157272450068));
#68809=CARTESIAN_POINT('Ctrl Pts',(-0.202071096458281,1.84867971434771,
11.617239284847));
#68810=CARTESIAN_POINT('Ctrl Pts',(-0.192934642654253,1.8415995521945,11.6179211527213));
#68811=CARTESIAN_POINT('Ctrl Pts',(-0.182461551238716,1.8343491575479,11.6186954510481));
#68812=CARTESIAN_POINT('Ctrl Pts',(-0.181480775372377,1.83367817234211,
11.6187678895224));
#68813=CARTESIAN_POINT('Ctrl Pts',(-0.180091934526216,1.83273924902574,
11.6188703738423));
#68814=CARTESIAN_POINT('Ctrl Pts',(-0.17968692915405,1.8324667845299,11.6189002485926));
#68815=CARTESIAN_POINT('Ctrl Pts',(-0.17897746753938,1.83199183700675,11.6189525624917));
#68816=CARTESIAN_POINT('Ctrl Pts',(-0.178673282048293,1.83178894952271,
11.6189749863637));
#68817=CARTESIAN_POINT('Ctrl Pts',(-0.178034119153083,1.83136420664323,
11.619022091784));
#68818=CARTESIAN_POINT('Ctrl Pts',(-0.177699071003547,1.83114245925169,
11.619046777338));
#68819=CARTESIAN_POINT('Ctrl Pts',(-0.176899006707475,1.83061509564786,
11.6191057079155));
#68820=CARTESIAN_POINT('Ctrl Pts',(-0.176433613140975,1.83031005688991,
11.619139974486));
#68821=CARTESIAN_POINT('Ctrl Pts',(-0.1748631052955,1.82928648426307,11.6192555675552));
#68822=CARTESIAN_POINT('Ctrl Pts',(-0.173754384360246,1.82857353292461,
11.6193371018863));
#68823=CARTESIAN_POINT('Ctrl Pts',(-0.158515211917701,1.8189057784121,11.6204569039393));
#68824=CARTESIAN_POINT('Ctrl Pts',(-0.143715155243382,1.81105912853269,
11.6215362852948));
#68825=CARTESIAN_POINT('Ctrl Pts',(-0.100861560692302,1.79244856020525,
11.6246370316621));
#68826=CARTESIAN_POINT('Ctrl Pts',(-0.0718168907659464,1.78440031422148,
11.6267228143369));
#68827=CARTESIAN_POINT('Ctrl Pts',(-0.0383846183829855,1.77999736653987,
11.6288923096056));
#68828=CARTESIAN_POINT('Ctrl Pts',(-0.0346814010707901,1.77957486406645,
11.6291292652265));
#68829=CARTESIAN_POINT('Ctrl Pts',(-0.0303926174221089,1.7791607837939,
11.6293991796128));
#68830=CARTESIAN_POINT('Ctrl Pts',(-0.029813582926488,1.77910645981082,
11.6294355262708));
#68831=CARTESIAN_POINT('Ctrl Pts',(-0.0289539546364591,1.77902815787421,
11.6294893421895));
#68832=CARTESIAN_POINT('Ctrl Pts',(-0.0286734754234494,1.77900298017691,
11.6295068784974));
#68833=CARTESIAN_POINT('Ctrl Pts',(-0.0281746103864681,1.77895885776884,
11.6295380280129));
#68834=CARTESIAN_POINT('Ctrl Pts',(-0.0279562383214456,1.77893976824352,
11.6295516493964));
#68835=CARTESIAN_POINT('Ctrl Pts',(-0.0274934026084197,1.77889978412336,
11.6295804900284));
#68836=CARTESIAN_POINT('Ctrl Pts',(-0.0272489352186839,1.77887894595118,
11.6295957060232));
#68837=CARTESIAN_POINT('Ctrl Pts',(-0.0265947813079852,1.77882393887186,
11.6296363753008));
#68838=CARTESIAN_POINT('Ctrl Pts',(-0.0261850510851788,1.77879027452655,
11.6296618001036));
#68839=CARTESIAN_POINT('Ctrl Pts',(-0.0242440437561171,1.77863453566225,
11.629782019799));
#68840=CARTESIAN_POINT('Ctrl Pts',(-0.0227119380452166,1.77852262378633,
11.6298762510855));
#68841=CARTESIAN_POINT('Ctrl Pts',(-0.0101836873572701,1.7776975168496,
11.6306418095175));
#68842=CARTESIAN_POINT('Ctrl Pts',(0.000842895172138619,1.77753768701612,
11.6312843275724));
#68843=CARTESIAN_POINT('Ctrl Pts',(0.0404173256039185,1.77899469635037,
11.6335458604291));
#68844=CARTESIAN_POINT('Ctrl Pts',(0.0687102306005357,1.78384026189208,
11.6350912251872));
#68845=CARTESIAN_POINT('Ctrl Pts',(0.105375118861746,1.79528074083744,11.6373258087251));
#68846=CARTESIAN_POINT('Ctrl Pts',(0.114616287970004,1.79863507244393,11.6379087836228));
#68847=CARTESIAN_POINT('Ctrl Pts',(0.12465104495111,1.80280582501161,11.63856957402));
#68848=CARTESIAN_POINT('Ctrl Pts',(0.12561096622351,1.80321026672242,11.6386330695936));
#68849=CARTESIAN_POINT('Ctrl Pts',(0.12704366217022,1.80382209732776,11.6387282702642));
#68850=CARTESIAN_POINT('Ctrl Pts',(0.127517933146498,1.80402598281251,11.6387598561118));
#68851=CARTESIAN_POINT('Ctrl Pts',(0.128333868553212,1.80437907245378,11.6388143199164));
#68852=CARTESIAN_POINT('Ctrl Pts',(0.128675768744317,1.80452773199962,11.6388371792547));
#68853=CARTESIAN_POINT('Ctrl Pts',(0.129380842810447,1.80483575685466,11.6388843979801));
#68854=CARTESIAN_POINT('Ctrl Pts',(0.129743981882299,1.8049951999017,11.6389087599966));
#68855=CARTESIAN_POINT('Ctrl Pts',(0.130588510369989,1.80536786701859,11.6389655168954));
#68856=CARTESIAN_POINT('Ctrl Pts',(0.131069672395004,1.80558160078071,11.6389979292017));
#68857=CARTESIAN_POINT('Ctrl Pts',(0.132601260817074,1.80626643605271,11.6391013434893));
#68858=CARTESIAN_POINT('Ctrl Pts',(0.133649678736999,1.80674198343807,11.6391724980422));
#68859=CARTESIAN_POINT('Ctrl Pts',(0.140013600139703,1.80966978194355,11.6396066556019));
#68860=CARTESIAN_POINT('Ctrl Pts',(0.1452637304307,1.8122607341547,11.6399744335374));
#68861=CARTESIAN_POINT('Ctrl Pts',(0.155182720155349,1.81749644611086,11.6406885216269));
#68862=CARTESIAN_POINT('Ctrl Pts',(0.15986185199902,1.82011767187691,11.641033930799));
#68863=CARTESIAN_POINT('Ctrl Pts',(0.177432588813707,1.83054509460032,11.6423638753915));
#68864=CARTESIAN_POINT('Ctrl Pts',(0.189835326956287,1.83913464139733,11.643372984266));
#68865=CARTESIAN_POINT('Ctrl Pts',(0.217442502888987,1.86126847913411,11.6457642146428));
#68866=CARTESIAN_POINT('Ctrl Pts',(0.232058102594201,1.8754490358269,11.6471497636331));
#68867=CARTESIAN_POINT('Ctrl Pts',(0.247857831656728,1.89398075368579,11.6487197220496));
#68868=CARTESIAN_POINT('Ctrl Pts',(0.250416228320391,1.89709817427318,11.6489764471714));
#68869=CARTESIAN_POINT('Ctrl Pts',(0.253284449496401,1.90073003866605,11.649266402911));
#68870=CARTESIAN_POINT('Ctrl Pts',(0.253652025246222,1.90119813897083,11.6493036036124));
#68871=CARTESIAN_POINT('Ctrl Pts',(0.254191384182196,1.90188893284851,11.6493582477198));
#68872=CARTESIAN_POINT('Ctrl Pts',(0.254364173301848,1.90211083389363,11.6493757623403));
#68873=CARTESIAN_POINT('Ctrl Pts',(0.25467145326886,1.90250651959351,11.6494069248232));
#68874=CARTESIAN_POINT('Ctrl Pts',(0.254806056900456,1.90268021568752,11.6494205807547));
#68875=CARTESIAN_POINT('Ctrl Pts',(0.255089115037092,1.9030462540395,11.6494493087416));
#68876=CARTESIAN_POINT('Ctrl Pts',(0.255237529325224,1.90323862603861,11.6494643779174));
#68877=CARTESIAN_POINT('Ctrl Pts',(0.255625086304347,1.90374214696252,11.649503745614));
#68878=CARTESIAN_POINT('Ctrl Pts',(0.255863879390579,1.90405356636553,11.6495280192667));
#68879=CARTESIAN_POINT('Ctrl Pts',(0.25692093544817,1.90543734159228,11.6496355511383));
#68880=CARTESIAN_POINT('Ctrl Pts',(0.257733045384272,1.90651441246081,11.6497183804235));
#68881=CARTESIAN_POINT('Ctrl Pts',(0.263834334288215,1.91471290146194,11.6503425793381));
#68882=CARTESIAN_POINT('Ctrl Pts',(0.268834751355689,1.92204558785675,11.6508651865999));
#68883=CARTESIAN_POINT('Ctrl Pts',(0.285445062684285,1.94870475716014,11.6526776442871));
#68884=CARTESIAN_POINT('Ctrl Pts',(0.29532459810369,1.96903189587887,11.6539081582701));
#68885=CARTESIAN_POINT('Ctrl Pts',(0.309133039964591,2.00714606197448,11.6562012862632));
#68886=CARTESIAN_POINT('Ctrl Pts',(0.313834413111732,2.02454863896376,11.6572430729892));
#68887=CARTESIAN_POINT('Ctrl Pts',(0.317288633751638,2.04351332247817,11.6584139948067));
#68888=CARTESIAN_POINT('Ctrl Pts',(0.317511002865627,2.04477695380665,11.6584921671831));
#68889=CARTESIAN_POINT('Ctrl Pts',(0.317811052036545,2.04654375632469,11.6586016916113));
#68890=CARTESIAN_POINT('Ctrl Pts',(0.317895096510152,2.04704584629552,11.6586328415039));
#68891=CARTESIAN_POINT('Ctrl Pts',(0.318038323393932,2.04791412786243,11.6586867544743));
#68892=CARTESIAN_POINT('Ctrl Pts',(0.318098064042576,2.04828022743618,11.6587094997998));
#68893=CARTESIAN_POINT('Ctrl Pts',(0.318220544424159,2.04903904538053,11.6587566728148));
#68894=CARTESIAN_POINT('Ctrl Pts',(0.318283189524069,2.04943177822474,11.6587811034646));
#68895=CARTESIAN_POINT('Ctrl Pts',(0.318428136743616,2.05035141734731,11.6588383488025));
#68896=CARTESIAN_POINT('Ctrl Pts',(0.318509858077849,2.05087841277801,11.6588711818371));
#68897=CARTESIAN_POINT('Ctrl Pts',(0.318769383208879,2.05257988850592,11.6589772821713));
#68898=CARTESIAN_POINT('Ctrl Pts',(0.318942000137274,2.05375513938439,11.6590507134631));
#68899=CARTESIAN_POINT('Ctrl Pts',(0.319328600653571,2.05649245765527,11.6592220930409));
#68900=CARTESIAN_POINT('Ctrl Pts',(0.319537624892319,2.05805518420373,11.6593201965411));
#68901=CARTESIAN_POINT('Ctrl Pts',(0.32158934226764,2.07430074640087,11.6603428715395));
#68902=CARTESIAN_POINT('Ctrl Pts',(0.322429874233752,2.08909025726703,11.6612990911777));
#68903=CARTESIAN_POINT('Ctrl Pts',(0.321975591097415,2.12678690609023,11.6637971479464));
#68904=CARTESIAN_POINT('Ctrl Pts',(0.319258802395855,2.14959353172216,11.6653691607795));
#68905=CARTESIAN_POINT('Ctrl Pts',(0.313256289760883,2.17581316446439,11.6671624285807));
#68906=CARTESIAN_POINT('Ctrl Pts',(0.312292296682133,2.1796910446217,11.6674270968607));
#68907=CARTESIAN_POINT('Ctrl Pts',(0.311072082449083,2.1842368130202,11.6677359799147));
#68908=CARTESIAN_POINT('Ctrl Pts',(0.310885481460665,2.18492289784849,11.6677825619809));
#68909=CARTESIAN_POINT('Ctrl Pts',(0.31029683662742,2.18705925397643,11.6679274840545));
#68910=CARTESIAN_POINT('Ctrl Pts',(0.309886898089565,2.18850735038045,11.6680255347787));
#68911=CARTESIAN_POINT('Ctrl Pts',(0.30806018014137,2.19479187066617,11.6684501151593));
#68912=CARTESIAN_POINT('Ctrl Pts',(0.306540116345514,2.19959787870943,11.6687723726319));
#68913=CARTESIAN_POINT('Ctrl Pts',(0.304702551508788,2.20496634030109,11.6691280575734));
#68914=CARTESIAN_POINT('Ctrl Pts',(0.304495486311521,2.20556550726584,11.6691676942922));
#68915=CARTESIAN_POINT('Ctrl Pts',(0.304191584724653,2.2064365477278,11.6692252236362));
#68916=CARTESIAN_POINT('Ctrl Pts',(0.304096150606751,2.2067089035518,11.6692431986329));
#68917=CARTESIAN_POINT('Ctrl Pts',(0.303927044721102,2.20718943920772,11.6692748893394));
#68918=CARTESIAN_POINT('Ctrl Pts',(0.303853524718333,2.20739767179972,11.6692886141064));
#68919=CARTESIAN_POINT('Ctrl Pts',(0.30369987500955,2.20783143710921,11.6693171872511));
#68920=CARTESIAN_POINT('Ctrl Pts',(0.303619708251891,2.20805695568442,11.6693320333437));
#68921=CARTESIAN_POINT('Ctrl Pts',(0.303412767844019,2.20863705506181,11.669370198254));
#68922=CARTESIAN_POINT('Ctrl Pts',(0.30328562337729,2.20899150462009,11.669393494926));
#68923=CARTESIAN_POINT('Ctrl Pts',(0.302747497313431,2.2104834434498,11.6694914622987));
#68924=CARTESIAN_POINT('Ctrl Pts',(0.302330728541014,2.21161885635859,11.669565792367));
#68925=CARTESIAN_POINT('Ctrl Pts',(0.301234494287541,2.21455416271915,11.6697574315919));
#68926=CARTESIAN_POINT('Ctrl Pts',(0.300545275993852,2.21635039417139,11.6698741931758));
#68927=CARTESIAN_POINT('Ctrl Pts',(0.297556638115072,2.22393554887978,11.6703655206203));
#68928=CARTESIAN_POINT('Ctrl Pts',(0.295105593015899,2.22966369072847,11.6707322610364));
#68929=CARTESIAN_POINT('Ctrl Pts',(0.284879350479015,2.25176778895219,11.6721438452319));
#68930=CARTESIAN_POINT('Ctrl Pts',(0.275894079011462,2.26754777038506,11.6731451304909));
#68931=CARTESIAN_POINT('Ctrl Pts',(0.252564213523024,2.30150640374914,11.675452940969));
#68932=CARTESIAN_POINT('Ctrl Pts',(0.237497327138924,2.31906232258689,11.6767650541417));
#68933=CARTESIAN_POINT('Ctrl Pts',(0.219635087677082,2.33584674485049,11.6782522888263));
#68934=CARTESIAN_POINT('Ctrl Pts',(0.218576652532869,2.33682800859974,11.6783401630285));
#68935=CARTESIAN_POINT('Ctrl Pts',(0.217116698444672,2.33816339224909,11.678461043699));
#68936=CARTESIAN_POINT('Ctrl Pts',(0.216720824415134,2.33852368102661,11.6784937883162));
#68937=CARTESIAN_POINT('Ctrl Pts',(0.216043914286319,2.33913666712065,11.678549723828));
#68938=CARTESIAN_POINT('Ctrl Pts',(0.215763326998765,2.33938986023259,11.6785728937459));
#68939=CARTESIAN_POINT('Ctrl Pts',(0.215218433398933,2.33987981879738,11.6786178584926));
#68940=CARTESIAN_POINT('Ctrl Pts',(0.2149541800147,2.34011664255857,11.678639650824));
#68941=CARTESIAN_POINT('Ctrl Pts',(0.214324081043995,2.34067946324338,11.6786915807907));
#68942=CARTESIAN_POINT('Ctrl Pts',(0.213957882815853,2.34100506243483,11.6787217350297));
#68943=CARTESIAN_POINT('Ctrl Pts',(0.212867825331273,2.34196982677535,11.6788114181472));
#68944=CARTESIAN_POINT('Ctrl Pts',(0.21214183913221,2.34260657078502,11.6788710478177));
#68945=CARTESIAN_POINT('Ctrl Pts',(0.206255398754909,2.34772279295457,11.6793537533184));
#68946=CARTESIAN_POINT('Ctrl Pts',(0.200956867167417,2.35204007158081,11.6797834652237));
#68947=CARTESIAN_POINT('Ctrl Pts',(0.187643444634022,2.36220112035548,11.6808529751251));
#68948=CARTESIAN_POINT('Ctrl Pts',(0.179488730895552,2.36784931207831,11.6814996458115));
#68949=CARTESIAN_POINT('Ctrl Pts',(0.155240465916205,2.38303929248595,11.6833958241118));
#68950=CARTESIAN_POINT('Ctrl Pts',(0.138560330615208,2.3915678244327,11.6846703045923));
#68951=CARTESIAN_POINT('Ctrl Pts',(0.107339552280378,2.40424391470092,11.6869397568061));
#68952=CARTESIAN_POINT('Ctrl Pts',(0.0930636111457863,2.40891005785235,
11.6879365643188));
#68953=CARTESIAN_POINT('Ctrl Pts',(0.0776272905968485,2.41278748864775,
11.6889375328384));
#68954=CARTESIAN_POINT('Ctrl Pts',(0.0767407883785567,2.41300616726648,
11.6889947521092));
#68955=CARTESIAN_POINT('Ctrl Pts',(0.0755476888938698,2.41329510248296,
11.6890713923113));
#68956=CARTESIAN_POINT('Ctrl Pts',(0.075241911878687,2.41336867941118,11.6890910017969));
#68957=CARTESIAN_POINT('Ctrl Pts',(0.0747270389134289,2.41349177254316,
11.6891239653934));
#68958=CARTESIAN_POINT('Ctrl Pts',(0.0745180011093741,2.41354152724687,
11.6891373332667));
#68959=CARTESIAN_POINT('Ctrl Pts',(0.0741170851783154,2.41363652876188,
11.689162942107));
#68960=CARTESIAN_POINT('Ctrl Pts',(0.0739252166960136,2.41368180824816,
11.6891751848684));
#68961=CARTESIAN_POINT('Ctrl Pts',(0.0735290342556281,2.41377492056864,
11.6892004377969));
#68962=CARTESIAN_POINT('Ctrl Pts',(0.0733247158077496,2.41382272975159,
11.6892134465479));
#68963=CARTESIAN_POINT('Ctrl Pts',(0.0727010144003571,2.41396802944874,
11.6892531127247));
#68964=CARTESIAN_POINT('Ctrl Pts',(0.072281480449289,2.41406487960281,11.6892797332001));
#68965=CARTESIAN_POINT('Ctrl Pts',(0.0701513391982144,2.41455213210589,
11.6894145920859));
#68966=CARTESIAN_POINT('Ctrl Pts',(0.0684377157826533,2.41492941048388,
11.6895220874162));
#68967=CARTESIAN_POINT('Ctrl Pts',(0.0636351078458215,2.41594572030417,
11.6898207961471));
#68968=CARTESIAN_POINT('Ctrl Pts',(0.0605396151090193,2.41655344220464,
11.6900103777501));
#68969=CARTESIAN_POINT('Ctrl Pts',(0.0493213918298268,2.418585272238,11.6906884293629));
#68970=CARTESIAN_POINT('Ctrl Pts',(0.0411531768135743,2.41974303959515,
11.691165193645));
#68971=CARTESIAN_POINT('Ctrl Pts',(0.0219252772709739,2.42171923116479,
11.6922663191834));
#68972=CARTESIAN_POINT('Ctrl Pts',(0.0108500919752149,2.42228290911793,
11.6928844785792));
#68973=CARTESIAN_POINT('Ctrl Pts',(-0.026349379231974,2.42225608012335,
11.6949638055561));
#68974=CARTESIAN_POINT('Ctrl Pts',(-0.0523627545378986,2.41906292409022,
11.696432267091));
#68975=CARTESIAN_POINT('Ctrl Pts',(-0.0791787362356968,2.41240072264719,
11.6981080005207));
#68976=CARTESIAN_POINT('Ctrl Pts',(-0.080650547254897,2.41202399408809,
11.6982004683781));
#68977=CARTESIAN_POINT('Ctrl Pts',(-0.08264857140053,2.41149749354986,11.6983266872025));
#68978=CARTESIAN_POINT('Ctrl Pts',(-0.0831771643241079,2.41135676349097,
11.6983601453683));
#68979=CARTESIAN_POINT('Ctrl Pts',(-0.0840734690315348,2.41111569023454,
11.6984169914503));
#68980=CARTESIAN_POINT('Ctrl Pts',(-0.0844413670449397,2.41101603887046,
11.6984403568963));
#68981=CARTESIAN_POINT('Ctrl Pts',(-0.085150492101369,2.41082260945812,
11.6984854566663));
#68982=CARTESIAN_POINT('Ctrl Pts',(-0.0854917433633932,2.41072892152256,
11.6985071880369));
#68983=CARTESIAN_POINT('Ctrl Pts',(-0.0862979438368308,2.41050615670808,
11.6985585947473));
#68984=CARTESIAN_POINT('Ctrl Pts',(-0.086762757867981,2.41037659755082,
11.6985882857314));
#68985=CARTESIAN_POINT('Ctrl Pts',(-0.0881222202801561,2.40999437761453,
11.6986752790105));
#68986=CARTESIAN_POINT('Ctrl Pts',(-0.0890160628457078,2.40973889065822,
11.6987326732174));
#68987=CARTESIAN_POINT('Ctrl Pts',(-0.0955137384121603,2.4078512114935,
11.6991513405159));
#68988=CARTESIAN_POINT('Ctrl Pts',(-0.101073105861682,2.40607100927709,
11.6995174282468));
#68989=CARTESIAN_POINT('Ctrl Pts',(-0.119370659259948,2.39965895631597,
11.7007498438901));
#68990=CARTESIAN_POINT('Ctrl Pts',(-0.131863520340114,2.39437523243346,
11.7016370915332));
#68991=CARTESIAN_POINT('Ctrl Pts',(-0.156027163894041,2.38230809878514,
11.7034397379492));
#68992=CARTESIAN_POINT('Ctrl Pts',(-0.16767985280604,2.37554632807435,11.7043531213799));
#68993=CARTESIAN_POINT('Ctrl Pts',(-0.191221103348493,2.35983831857301,
11.7062658056417));
#68994=CARTESIAN_POINT('Ctrl Pts',(-0.202984559992781,2.35075649383721,
11.7072620933955));
#68995=CARTESIAN_POINT('Ctrl Pts',(-0.216576113052761,2.33867782766144,
11.708428811427));
#68996=CARTESIAN_POINT('Ctrl Pts',(-0.219036767035541,2.33642168895417,
11.7086406807862));
#68997=CARTESIAN_POINT('Ctrl Pts',(-0.221865632774627,2.3337458561133,11.7088845507742));
#68998=CARTESIAN_POINT('Ctrl Pts',(-0.222268243982232,2.33336304759886,
11.7089192660681));
#68999=CARTESIAN_POINT('Ctrl Pts',(-0.222872443920402,2.33278558350855,
11.7089713713294));
#69000=CARTESIAN_POINT('Ctrl Pts',(-0.223074769299489,2.33259170546664,
11.7089888208954));
#69001=CARTESIAN_POINT('Ctrl Pts',(-0.223434800798351,2.33224580383475,
11.709019873798));
#69002=CARTESIAN_POINT('Ctrl Pts',(-0.223592604692754,2.33209388344898,
11.7090334851205));
#69003=CARTESIAN_POINT('Ctrl Pts',(-0.223927417576696,2.3317708952344,11.7090623655788));
#69004=CARTESIAN_POINT('Ctrl Pts',(-0.224104384985417,2.33159978594896,
11.7090776313369));
#69005=CARTESIAN_POINT('Ctrl Pts',(-0.224464926652284,2.33125037906326,
11.7091087348809));
#69006=CARTESIAN_POINT('Ctrl Pts',(-0.224648484985861,2.33107206518433,
11.7091245713763));
#69007=CARTESIAN_POINT('Ctrl Pts',(-0.225106451055752,2.33062612220227,
11.7091640857884));
#69008=CARTESIAN_POINT('Ctrl Pts',(-0.225380594993654,2.33035822093609,
11.7091877426331));
#69009=CARTESIAN_POINT('Ctrl Pts',(-0.228482204711251,2.32731640264702,
11.7094554352374));
#69010=CARTESIAN_POINT('Ctrl Pts',(-0.231258934104973,2.32449092110601,
11.7096955018236));
#69011=CARTESIAN_POINT('Ctrl Pts',(-0.240431501661529,2.31480643737695,
11.7104929587089));
#69012=CARTESIAN_POINT('Ctrl Pts',(-0.246580321137079,2.30771925200631,
11.7110351008034));
#69013=CARTESIAN_POINT('Ctrl Pts',(-0.256877153641243,2.29474826262257,
11.7119772671885));
#69014=CARTESIAN_POINT('Ctrl Pts',(-0.261153422113637,2.28897527214057,
11.7123805541285));
#69015=CARTESIAN_POINT('Ctrl Pts',(-0.278346260679777,2.26406534111136,
11.7140747231586));
#69016=CARTESIAN_POINT('Ctrl Pts',(-0.289378786448976,2.24371461358229,
11.7153544460444));
#69017=CARTESIAN_POINT('Ctrl Pts',(-0.298348076118668,2.22186014041684,
11.7167446716449));
#69018=CARTESIAN_POINT('Ctrl Pts',(-0.298552234293598,2.22135910241772,
11.7167765487307));
#69019=CARTESIAN_POINT('Ctrl Pts',(-0.299422126779447,2.21920876235513,
11.7169133816852));
#69020=CARTESIAN_POINT('Ctrl Pts',(-0.300075454400406,2.21755450020109,
11.7170187078431));
#69021=CARTESIAN_POINT('Ctrl Pts',(-0.302547578480107,2.21114002754951,
11.7174274673825));
#69022=CARTESIAN_POINT('Ctrl Pts',(-0.304266991499749,2.20634254274059,
11.7177339474231));
#69023=CARTESIAN_POINT('Ctrl Pts',(-0.306143539801097,2.20068789692954,
11.7180967647819));
#69024=CARTESIAN_POINT('Ctrl Pts',(-0.306411914166872,2.19986820507022,
11.7181493963221));
#69025=CARTESIAN_POINT('Ctrl Pts',(-0.306835661514563,2.19855617169906,
11.7182337047387));
#69026=CARTESIAN_POINT('Ctrl Pts',(-0.306993148798102,2.19806451316955,
11.7182653120054));
#69027=CARTESIAN_POINT('Ctrl Pts',(-0.307269468453475,2.19719468357653,
11.718321256941));
#69028=CARTESIAN_POINT('Ctrl Pts',(-0.307388786045428,2.1968166668013,11.7183455786138));
#69029=CARTESIAN_POINT('Ctrl Pts',(-0.307634480680699,2.19603323515355,
11.7183960032265));
#69030=CARTESIAN_POINT('Ctrl Pts',(-0.307760754392193,2.19562778890543,
11.7184221095017));
#69031=CARTESIAN_POINT('Ctrl Pts',(-0.3080829155303,2.19458612965494,11.7184892077374));
#69032=CARTESIAN_POINT('Ctrl Pts',(-0.308277633036435,2.19394955946454,
11.7185302379382));
#69033=CARTESIAN_POINT('Ctrl Pts',(-0.30869366980271,2.19257423286936,11.71861894199));
#69034=CARTESIAN_POINT('Ctrl Pts',(-0.308914312006688,2.19183527747259,
11.7186666377402));
#69035=CARTESIAN_POINT('Ctrl Pts',(-0.310021486365612,2.18807808644813,
11.718909331594));
#69036=CARTESIAN_POINT('Ctrl Pts',(-0.310866420089562,2.18504786329901,
11.7191056804272));
#69037=CARTESIAN_POINT('Ctrl Pts',(-0.318735136329981,2.15514245817528,
11.7210500832756));
#69038=CARTESIAN_POINT('Ctrl Pts',(-0.322298937199578,2.12748432642362,
11.7229160354673));
#69039=CARTESIAN_POINT('Ctrl Pts',(-0.322274879003935,2.09972073668561,
11.7247944044677));
#69040=CARTESIAN_POINT('',(-0.322274882473144,2.10017262650289,11.9744806947813));
#69041=CARTESIAN_POINT('Ctrl Pts',(-0.322274878830663,2.09972053679725,
11.7247944179913));
#69042=CARTESIAN_POINT('Ctrl Pts',(-0.322258357831344,2.08066864373516,
11.7260833897981));
#69043=CARTESIAN_POINT('Ctrl Pts',(-0.320552428193726,2.0616526188374,11.7273676966839));
#69044=CARTESIAN_POINT('Ctrl Pts',(-0.317040312090144,2.04214501967275,
11.7286169371805));
#69045=CARTESIAN_POINT('Ctrl Pts',(-0.31690239481546,2.04139427991564,11.7286649034451));
#69046=CARTESIAN_POINT('Ctrl Pts',(-0.316686225496915,2.04024066078012,
11.7287384336421));
#69047=CARTESIAN_POINT('Ctrl Pts',(-0.316609870106264,2.03983743523448,
11.7287641014531));
#69048=CARTESIAN_POINT('Ctrl Pts',(-0.316482519396665,2.03917186535682,
11.7288064129159));
#69049=CARTESIAN_POINT('Ctrl Pts',(-0.316431967886135,2.03890943813674,
11.7288230814444));
#69050=CARTESIAN_POINT('Ctrl Pts',(-0.316340940502728,2.03844003359228,
11.7288528702927));
#69051=CARTESIAN_POINT('Ctrl Pts',(-0.316300587867842,2.03823303295985,
11.7288659976201));
#69052=CARTESIAN_POINT('Ctrl Pts',(-0.316222029871392,2.03783214253678,
11.7288914029485));
#69053=CARTESIAN_POINT('Ctrl Pts',(-0.316183849369666,2.03763824829164,
11.7289036823447));
#69054=CARTESIAN_POINT('Ctrl Pts',(-0.316104141202829,2.03723541669019,
11.7289291768685));
#69055=CARTESIAN_POINT('Ctrl Pts',(-0.316062584844273,2.0370264859976,11.7289423902863));
#69056=CARTESIAN_POINT('Ctrl Pts',(-0.315947853945584,2.036452633936,11.7289786568704));
#69057=CARTESIAN_POINT('Ctrl Pts',(-0.315874254068038,2.03608779641753,
11.7290016856212));
#69058=CARTESIAN_POINT('Ctrl Pts',(-0.315588033875181,2.03468156304085,
11.7290903410722));
#69059=CARTESIAN_POINT('Ctrl Pts',(-0.315370891194541,2.0336410790217,11.7291557120302));
#69060=CARTESIAN_POINT('Ctrl Pts',(-0.311263355965539,2.01443460896736,
11.730358545139));
#69061=CARTESIAN_POINT('Ctrl Pts',(-0.30581382126515,1.9966344346182,11.7314103826875));
#69062=CARTESIAN_POINT('Ctrl Pts',(-0.297707451480833,1.97654584893946,
11.7326246449452));
#69063=CARTESIAN_POINT('Ctrl Pts',(-0.296514504510577,1.97370747109345,
11.7327968396689));
#69064=CARTESIAN_POINT('Ctrl Pts',(-0.294235888609452,1.96849629863782,
11.7331147972916));
#69065=CARTESIAN_POINT('Ctrl Pts',(-0.293161724471731,1.96611876563191,
11.733260570526));
#69066=CARTESIAN_POINT('Ctrl Pts',(-0.289843927380256,1.95900666174207,
11.733699385616));
#69067=CARTESIAN_POINT('Ctrl Pts',(-0.287513617992391,1.95431354882682,
11.7339926716667));
#69068=CARTESIAN_POINT('Ctrl Pts',(-0.278203408493568,1.93665754731237,
11.735116110529));
#69069=CARTESIAN_POINT('Ctrl Pts',(-0.270453392731345,1.92412280084275,
11.7359567844403));
#69070=CARTESIAN_POINT('Ctrl Pts',(-0.258376519481509,1.90728579213341,
11.7371836552982));
#69071=CARTESIAN_POINT('Ctrl Pts',(-0.254743302284678,1.90250814072322,
11.7375437221857));
#69072=CARTESIAN_POINT('Ctrl Pts',(-0.250366235949369,1.89707420643385,
11.7379685736147));
#69073=CARTESIAN_POINT('Ctrl Pts',(-0.249750022135621,1.89631628389044,
11.738028187837));
#69074=CARTESIAN_POINT('Ctrl Pts',(-0.24881807558594,1.89518060820616,11.738118056729));
#69075=CARTESIAN_POINT('Ctrl Pts',(-0.24850490354374,1.89480075316036,11.7381482075975));
#69076=CARTESIAN_POINT('Ctrl Pts',(-0.247964305069852,1.89414809892012,
11.7382001711221));
#69077=CARTESIAN_POINT('Ctrl Pts',(-0.247737295154548,1.89387495456681,
11.738221966796));
#69078=CARTESIAN_POINT('Ctrl Pts',(-0.247268371999136,1.89331262742267,
11.7382669378538));
#69079=CARTESIAN_POINT('Ctrl Pts',(-0.247026401956639,1.89302349285848,
11.7382901155404));
#69080=CARTESIAN_POINT('Ctrl Pts',(-0.246372562586775,1.89224498766539,
11.7383526704311));
#69081=CARTESIAN_POINT('Ctrl Pts',(-0.245959744420385,1.89175641940034,
11.7383920864978));
#69082=CARTESIAN_POINT('Ctrl Pts',(-0.244433787483275,1.88996132438122,
11.7385374963559));
#69083=CARTESIAN_POINT('Ctrl Pts',(-0.243311685935253,1.88866248552757,
11.7386438592414));
#69084=CARTESIAN_POINT('Ctrl Pts',(-0.224173958965546,1.866864904691,11.7404486931334));
#69085=CARTESIAN_POINT('Ctrl Pts',(-0.203640703875255,1.84873171117412,
11.742263101875));
#69086=CARTESIAN_POINT('Ctrl Pts',(-0.174853944328719,1.82917933412451,
11.7446174232807));
#69087=CARTESIAN_POINT('Ctrl Pts',(-0.168486629653042,1.82517279446666,
11.7451268872452));
#69088=CARTESIAN_POINT('Ctrl Pts',(-0.154874298789226,1.81725845766967,
11.7461865073697));
#69089=CARTESIAN_POINT('Ctrl Pts',(-0.147607568234485,1.81339774973521,
11.7467356447559));
#69090=CARTESIAN_POINT('Ctrl Pts',(-0.13600980730416,1.80779429961115,11.7475787927971));
#69091=CARTESIAN_POINT('Ctrl Pts',(-0.131775305159434,1.80586038529376,
11.7478799431085));
#69092=CARTESIAN_POINT('Ctrl Pts',(-0.126086839063073,1.80340995838733,
11.748274292824));
#69093=CARTESIAN_POINT('Ctrl Pts',(-0.124669140740509,1.80281125638688,
11.7483717432364));
#69094=CARTESIAN_POINT('Ctrl Pts',(-0.122307174138058,1.80183366093716,
11.7485326603685));
#69095=CARTESIAN_POINT('Ctrl Pts',(-0.121365319681414,1.80144904984179,
11.748596449517));
#69096=CARTESIAN_POINT('Ctrl Pts',(-0.120173618139414,1.80096898383512,
11.7486766692601));
#69097=CARTESIAN_POINT('Ctrl Pts',(-0.119925466091536,1.8008693768447,11.7486933468897));
#69098=CARTESIAN_POINT('Ctrl Pts',(-0.119481332684988,1.8006917454184,11.7487231476064));
#69099=CARTESIAN_POINT('Ctrl Pts',(-0.119285398542744,1.80061360449083,
11.7487362777163));
#69100=CARTESIAN_POINT('Ctrl Pts',(-0.118905737971855,1.80046262309496,
11.7487616871518));
#69101=CARTESIAN_POINT('Ctrl Pts',(-0.118722021266612,1.80038975926554,
11.7487739678759));
#69102=CARTESIAN_POINT('Ctrl Pts',(-0.118340213229229,1.80023873681532,
11.7487994593262));
#69103=CARTESIAN_POINT('Ctrl Pts',(-0.118142112032152,1.80016060575966,
11.7488126683528));
#69104=CARTESIAN_POINT('Ctrl Pts',(-0.117597900401303,1.79994659191713,
11.7488489085078));
#69105=CARTESIAN_POINT('Ctrl Pts',(-0.117251630629727,1.79981111113348,
11.748871915282));
#69106=CARTESIAN_POINT('Ctrl Pts',(-0.115917086858522,1.79929162176353,
11.7489603873084));
#69107=CARTESIAN_POINT('Ctrl Pts',(-0.114927140457945,1.79891188627372,
11.7490255981782));
#69108=CARTESIAN_POINT('Ctrl Pts',(-0.0975638905877046,1.79234959602426,
11.7501623926708));
#69109=CARTESIAN_POINT('Ctrl Pts',(-0.0807129274239811,1.78750504435862,
11.7511579841937));
#69110=CARTESIAN_POINT('Ctrl Pts',(-0.0449280728360833,1.78030728269999,
11.7532075353054));
#69111=CARTESIAN_POINT('Ctrl Pts',(-0.0260126232552263,1.77821546568542,
11.7542565112898));
#69112=CARTESIAN_POINT('Ctrl Pts',(0.00478950206968854,1.77754404360837,
11.7560245429554));
#69113=CARTESIAN_POINT('Ctrl Pts',(0.0166062876633351,1.77793639184922,
11.7567164723318));
#69114=CARTESIAN_POINT('Ctrl Pts',(0.0307648249340058,1.77918780903631,
11.7575740533033));
#69115=CARTESIAN_POINT('Ctrl Pts',(0.033153163073487,1.77942582196759,11.7577196781388));
#69116=CARTESIAN_POINT('Ctrl Pts',(0.0362418092435508,1.77976850948186,
11.7579093222204));
#69117=CARTESIAN_POINT('Ctrl Pts',(0.0369447840398306,1.7798488494845,11.757952573734));
#69118=CARTESIAN_POINT('Ctrl Pts',(0.0380785062502868,1.77998220153079,
11.7580224725321));
#69119=CARTESIAN_POINT('Ctrl Pts',(0.0385094237913649,1.78003377013867,
11.758049074244));
#69120=CARTESIAN_POINT('Ctrl Pts',(0.039330900900313,1.7801337611734,11.7580998512577));
#69121=CARTESIAN_POINT('Ctrl Pts',(0.0397214787946563,1.78018202891819,
11.758124021634));
#69122=CARTESIAN_POINT('Ctrl Pts',(0.0406130640235536,1.78029386977093,
11.7581792606267));
#69123=CARTESIAN_POINT('Ctrl Pts',(0.0411140113856175,1.78035790524622,
11.7582103437934));
#69124=CARTESIAN_POINT('Ctrl Pts',(0.0426459795508157,1.78055739575476,
11.758305544018));
#69125=CARTESIAN_POINT('Ctrl Pts',(0.0436764894256331,1.78069666270193,
11.758369781362));
#69126=CARTESIAN_POINT('Ctrl Pts',(0.0512906053982372,1.78176321211027,
11.7588459058248));
#69127=CARTESIAN_POINT('Ctrl Pts',(0.0578443630311506,1.78288898091934,
11.7592640451124));
#69128=CARTESIAN_POINT('Ctrl Pts',(0.0661755824306511,1.78458692513058,
11.7598068497073));
#69129=CARTESIAN_POINT('Ctrl Pts',(0.067989654627021,1.78497298187326,11.7599257278585));
#69130=CARTESIAN_POINT('Ctrl Pts',(0.0722858348494677,1.78592609812625,
11.7602088936562));
#69131=CARTESIAN_POINT('Ctrl Pts',(0.0747647285274502,1.78650694971935,
11.7603735796461));
#69132=CARTESIAN_POINT('Ctrl Pts',(0.0916792670192907,1.79068237296024,
11.7615061557513));
#69133=CARTESIAN_POINT('Ctrl Pts',(0.105856486095041,1.79524303949041,11.7625009824833));
#69134=CARTESIAN_POINT('Ctrl Pts',(0.134850615103314,1.80683808428629,11.7646101919796));
#69135=CARTESIAN_POINT('Ctrl Pts',(0.149550754543677,1.81405733675741,11.7657237341072));
#69136=CARTESIAN_POINT('Ctrl Pts',(0.167951729265524,1.82490284665707,11.7671330871891));
#69137=CARTESIAN_POINT('Ctrl Pts',(0.172204100899809,1.82754453513131,11.7674598126102));
#69138=CARTESIAN_POINT('Ctrl Pts',(0.178407147214478,1.83160131354508,11.7679360941594));
#69139=CARTESIAN_POINT('Ctrl Pts',(0.180406118597845,1.83294083385767,11.7680895264074));
#69140=CARTESIAN_POINT('Ctrl Pts',(0.183572549349485,1.83511445440992,11.768332246967));
#69141=CARTESIAN_POINT('Ctrl Pts',(0.184749726214653,1.83593415218344,11.7684224106087));
#69142=CARTESIAN_POINT('Ctrl Pts',(0.186248715108876,1.83699286643263,11.7685370892849));
#69143=CARTESIAN_POINT('Ctrl Pts',(0.186575584211952,1.83722464429261,11.7685620878989));
#69144=CARTESIAN_POINT('Ctrl Pts',(0.187101497838295,1.8375990375636,11.7686022948937));
#69145=CARTESIAN_POINT('Ctrl Pts',(0.187300812286686,1.83774127031004,11.7686175294956));
#69146=CARTESIAN_POINT('Ctrl Pts',(0.187678335107111,1.83801132419063,11.7686463788368));
#69147=CARTESIAN_POINT('Ctrl Pts',(0.187856573624218,1.83813909900984,11.7686599965318));
#69148=CARTESIAN_POINT('Ctrl Pts',(0.188264093107926,1.83843186993913,11.7686911253479));
#69149=CARTESIAN_POINT('Ctrl Pts',(0.188493287310915,1.83859698537034,11.7687086280551));
#69150=CARTESIAN_POINT('Ctrl Pts',(0.189197254081118,1.83910554235006,11.7687623744014));
#69151=CARTESIAN_POINT('Ctrl Pts',(0.189671310653218,1.83944998001894,11.7687985494251));
#69152=CARTESIAN_POINT('Ctrl Pts',(0.193231114661388,1.84205130879584,11.7690700810946));
#69153=CARTESIAN_POINT('Ctrl Pts',(0.196277585772294,1.84436177238076,11.7693018043733));
#69154=CARTESIAN_POINT('Ctrl Pts',(0.205983871660226,1.85199892397352,11.7700405502315));
#69155=CARTESIAN_POINT('Ctrl Pts',(0.212473999017151,1.85753616329091,11.7705352656361));
#69156=CARTESIAN_POINT('Ctrl Pts',(0.230085147851148,1.87381253880505,11.7719042433702));
#69157=CARTESIAN_POINT('Ctrl Pts',(0.240664423655455,1.88510324536843,11.7727594998356));
#69158=CARTESIAN_POINT('Ctrl Pts',(0.264782072222983,1.91486758388619,11.7749071415005));
#69159=CARTESIAN_POINT('Ctrl Pts',(0.277238784185174,1.93410250623397,11.7762105954028));
#69160=CARTESIAN_POINT('Ctrl Pts',(0.288071407502033,1.95551005780231,11.7776695524184));
#69161=CARTESIAN_POINT('Ctrl Pts',(0.288581490011106,1.95653152685366,11.7777391689828));
#69162=CARTESIAN_POINT('Ctrl Pts',(0.289320578544577,1.95803148301144,11.7778414067238));
#69163=CARTESIAN_POINT('Ctrl Pts',(0.289553852210817,1.95850786718032,11.7778738788605));
#69164=CARTESIAN_POINT('Ctrl Pts',(0.289959760409528,1.95934200783372,11.777930740625));
#69165=CARTESIAN_POINT('Ctrl Pts',(0.290132912040883,1.95969951259745,11.77795511219));
#69166=CARTESIAN_POINT('Ctrl Pts',(0.290466812210881,1.96039217500428,11.778002334506));
#69167=CARTESIAN_POINT('Ctrl Pts',(0.290627642816581,1.96072729260524,11.7780251823591));
#69168=CARTESIAN_POINT('Ctrl Pts',(0.291008635641253,1.96152468891259,11.7780795509204));
#69169=CARTESIAN_POINT('Ctrl Pts',(0.291228276144563,1.96198721447788,11.7781110896634));
#69170=CARTESIAN_POINT('Ctrl Pts',(0.292001854695574,1.9636263088293,11.7782228667951));
#69171=CARTESIAN_POINT('Ctrl Pts',(0.292549766802917,1.96480569297037,11.7783033132202));
#69172=CARTESIAN_POINT('Ctrl Pts',(0.302002168028159,1.9854785906559,11.7797138555546));
#69173=CARTESIAN_POINT('Ctrl Pts',(0.308945720199433,2.00580511466784,11.7811130502327));
#69174=CARTESIAN_POINT('Ctrl Pts',(0.318545781976656,2.04688721452165,11.7839454490837));
#69175=CARTESIAN_POINT('Ctrl Pts',(0.321305555521644,2.0675171414673,11.7853688126219));
#69176=CARTESIAN_POINT('Ctrl Pts',(0.322329488724655,2.09562862630801,11.7872223375088));
#69177=CARTESIAN_POINT('Ctrl Pts',(0.322345239189801,2.1029957365363,11.7876996961705));
#69178=CARTESIAN_POINT('Ctrl Pts',(0.322069741459443,2.11156343222941,11.7882402996076));
#69179=CARTESIAN_POINT('Ctrl Pts',(0.32202419281672,2.11276912991203,11.788316039976));
#69180=CARTESIAN_POINT('Ctrl Pts',(0.321955555706071,2.11435051851738,11.788414914027));
#69181=CARTESIAN_POINT('Ctrl Pts',(0.321938579642829,2.1147264446734,11.7884383836547));
#69182=CARTESIAN_POINT('Ctrl Pts',(0.32190973176689,2.11534136487403,11.7884767164492));
#69183=CARTESIAN_POINT('Ctrl Pts',(0.321898252215036,2.11558037561262,11.7884916016271));
#69184=CARTESIAN_POINT('Ctrl Pts',(0.321875665641876,2.11603995846333,11.788520195994));
#69185=CARTESIAN_POINT('Ctrl Pts',(0.321864598119062,2.11626053128858,11.7885339073225));
#69186=CARTESIAN_POINT('Ctrl Pts',(0.321838538878732,2.11676943275992,11.7885655137618));
#69187=CARTESIAN_POINT('Ctrl Pts',(0.321823386384843,2.1170577536633,11.7885833997797));
#69188=CARTESIAN_POINT('Ctrl Pts',(0.3217736892413,2.11797974604633,11.788640530314));
#69189=CARTESIAN_POINT('Ctrl Pts',(0.321737660071789,2.11861334100938,11.78867969178));
#69190=CARTESIAN_POINT('Ctrl Pts',(0.32139742612532,2.12430015637966,11.7890303309067));
#69191=CARTESIAN_POINT('Ctrl Pts',(0.320976046170345,2.12934600283102,11.7893353986273));
#69192=CARTESIAN_POINT('Ctrl Pts',(0.320313048749553,2.13552538623077,11.78970384451));
#69193=CARTESIAN_POINT('Ctrl Pts',(0.320184035140333,2.1366699601125,11.789771871841));
#69194=CARTESIAN_POINT('Ctrl Pts',(0.319931153549727,2.13881030048345,11.7898987147928));
#69195=CARTESIAN_POINT('Ctrl Pts',(0.319808766330212,2.13980622381987,11.7899575870811));
#69196=CARTESIAN_POINT('Ctrl Pts',(0.316843118895036,2.16304217557256,11.7913279905411));
#69197=CARTESIAN_POINT('Ctrl Pts',(0.311691099760403,2.18492775296392,11.7925550281665));
#69198=CARTESIAN_POINT('Ctrl Pts',(0.297747301946518,2.22491927571672,11.7949365619973));
#69199=CARTESIAN_POINT('Ctrl Pts',(0.289456582201734,2.24308388088151,11.7960789470654));
#69200=CARTESIAN_POINT('Ctrl Pts',(0.278615209895248,2.26198214311942,11.7973974035842));
#69201=CARTESIAN_POINT('Ctrl Pts',(0.277673715326556,2.26359082329075,11.7975106943063));
#69202=CARTESIAN_POINT('Ctrl Pts',(0.276380174828903,2.26575768404406,11.79766476984));
#69203=CARTESIAN_POINT('Ctrl Pts',(0.276040278957232,2.26632310495274,11.7977051114966));
#69204=CARTESIAN_POINT('Ctrl Pts',(0.27547943067571,2.26724962813779,11.7977714442932));
#69205=CARTESIAN_POINT('Ctrl Pts',(0.275259497501414,2.2676113476773,11.7977973980613));
#69206=CARTESIAN_POINT('Ctrl Pts',(0.274831970781404,2.26831138111555,11.7978477374538));
#69207=CARTESIAN_POINT('Ctrl Pts',(0.274624463568972,2.26864974706126,11.7978721198744));
#69208=CARTESIAN_POINT('Ctrl Pts',(0.274143938595106,2.26943006349542,11.7979284661934));
#69209=CARTESIAN_POINT('Ctrl Pts',(0.273870476845853,2.26987173806047,11.7979604464106));
#69210=CARTESIAN_POINT('Ctrl Pts',(0.272991330782801,2.27128402695609,11.7980629862771));
#69211=CARTESIAN_POINT('Ctrl Pts',(0.272381550396838,2.27225206971811,11.7981336971865));
#69212=CARTESIAN_POINT('Ctrl Pts',(0.266717805087173,2.28113814017874,11.7987867538698));
#69213=CARTESIAN_POINT('Ctrl Pts',(0.261325544388627,2.28883416953473,11.7993817237438));
#69214=CARTESIAN_POINT('Ctrl Pts',(0.251872262981872,2.30114449346192,11.8003847679703));
#69215=CARTESIAN_POINT('Ctrl Pts',(0.248001440858772,2.30589808711745,11.8007857119392));
#69216=CARTESIAN_POINT('Ctrl Pts',(0.227662105725203,2.32946981486172,11.8028429286825));
#69217=CARTESIAN_POINT('Ctrl Pts',(0.209180734789248,2.34643393556545,11.8045639601435));
#69218=CARTESIAN_POINT('Ctrl Pts',(0.181555619120013,2.36642351475296,11.8068281901526));
#69219=CARTESIAN_POINT('Ctrl Pts',(0.173962360821164,2.37144255925349,11.8074221833282));
#69220=CARTESIAN_POINT('Ctrl Pts',(0.164991719543398,2.37684072475377,11.8080834490993));
#69221=CARTESIAN_POINT('Ctrl Pts',(0.163812758172484,2.37753996976898,11.8081695761182));
#69222=CARTESIAN_POINT('Ctrl Pts',(0.162289313951313,2.37843043893781,11.8082798330742));
#69223=CARTESIAN_POINT('Ctrl Pts',(0.161948915003612,2.37862856939478,11.8083044027569));
#69224=CARTESIAN_POINT('Ctrl Pts',(0.161397657919383,2.37894807910312,11.8083440839672));
#69225=CARTESIAN_POINT('Ctrl Pts',(0.161187025374068,2.37906984371154,11.8083592205061));
#69226=CARTESIAN_POINT('Ctrl Pts',(0.160785955008397,2.37930109299815,11.8083879936448));
#69227=CARTESIAN_POINT('Ctrl Pts',(0.160595544725543,2.37941062057926,11.8084016329572));
#69228=CARTESIAN_POINT('Ctrl Pts',(0.160161617150881,2.37965963379146,11.8084326683852));
#69229=CARTESIAN_POINT('Ctrl Pts',(0.15991802990074,2.37979899587893,11.8084500564044));
#69230=CARTESIAN_POINT('Ctrl Pts',(0.159159996015875,2.38023137191248,11.8085040629998));
#69231=CARTESIAN_POINT('Ctrl Pts',(0.158644920066477,2.38052328866954,11.8085406108402));
#69232=CARTESIAN_POINT('Ctrl Pts',(0.154678558884764,2.38275678611862,11.8088209274459));
#69233=CARTESIAN_POINT('Ctrl Pts',(0.151192369877625,2.3846361316279,11.8090607943519));
#69234=CARTESIAN_POINT('Ctrl Pts',(0.146594411267985,2.38700648888283,11.8093698981345));
#69235=CARTESIAN_POINT('Ctrl Pts',(0.145513441970028,2.38755605430353,11.8094420517271));
#69236=CARTESIAN_POINT('Ctrl Pts',(0.144323493189536,2.38815259667175,11.8095209427483));
#69237=CARTESIAN_POINT('Ctrl Pts',(0.144217575896015,2.38820562183606,11.809527960182));
#69238=CARTESIAN_POINT('Ctrl Pts',(0.143194695477665,2.38871699936055,11.8095956853169));
#69239=CARTESIAN_POINT('Ctrl Pts',(0.142275569439957,2.38917103748531,11.8096561943016));
#69240=CARTESIAN_POINT('Ctrl Pts',(0.126043049663522,2.39709359372834,11.8107190102569));
#69241=CARTESIAN_POINT('Ctrl Pts',(0.110161823517475,2.40334128709682,11.811668806838));
#69242=CARTESIAN_POINT('Ctrl Pts',(0.0777240397127478,2.41321660566566,
11.8135640327894));
#69243=CARTESIAN_POINT('Ctrl Pts',(0.061228309141513,2.41685439574087,11.8145069310016));
#69244=CARTESIAN_POINT('Ctrl Pts',(0.0360242051667638,2.42037025066754,
11.8159840525524));
#69245=CARTESIAN_POINT('Ctrl Pts',(0.0274803215562856,2.42121589880442,
11.8164906218053));
#69246=CARTESIAN_POINT('Ctrl Pts',(0.0163604997795346,2.42186961553835,
11.8171621255569));
#69247=CARTESIAN_POINT('Ctrl Pts',(0.0138059799212023,2.42198930059415,
11.8173172095709));
#69248=CARTESIAN_POINT('Ctrl Pts',(0.0105322509925847,2.42210365354363,
11.8175170933146));
#69249=CARTESIAN_POINT('Ctrl Pts',(0.00981406307787783,2.42212633560431,
11.8175610136008));
#69250=CARTESIAN_POINT('Ctrl Pts',(0.00865952887527339,2.42215893387814,
11.8176317328388));
#69251=CARTESIAN_POINT('Ctrl Pts',(0.00822322502517501,2.42217036593247,
11.8176584842447));
#69252=CARTESIAN_POINT('Ctrl Pts',(0.00739400962481082,2.42219040752398,
11.8177093769649));
#69253=CARTESIAN_POINT('Ctrl Pts',(0.00700110260858537,2.42219918472722,
11.817733512979));
#69254=CARTESIAN_POINT('Ctrl Pts',(0.00610778547895219,2.42221750586125,
11.8177884382155));
#69255=CARTESIAN_POINT('Ctrl Pts',(0.00560736809805012,2.42222660278972,
11.8178192413877));
#69256=CARTESIAN_POINT('Ctrl Pts',(0.00412331072681669,2.42225012287198,
11.8179106980219));
#69257=CARTESIAN_POINT('Ctrl Pts',(0.0031396302956104,2.4222612078262,11.8179714558947));
#69258=CARTESIAN_POINT('Ctrl Pts',(-0.00360499709869908,2.42230632837212,
11.8183890043709));
#69259=CARTESIAN_POINT('Ctrl Pts',(-0.00936558974634618,2.42219038490161,
11.8187504670316));
#69260=CARTESIAN_POINT('Ctrl Pts',(-0.0162913166439642,2.42186510272379,
11.819191244171));
#69261=CARTESIAN_POINT('Ctrl Pts',(-0.0174626163683917,2.42180367978286,
11.8192660025406));
#69262=CARTESIAN_POINT('Ctrl Pts',(-0.0513626445563393,2.4198403375196,
11.8214358662419));
#69263=CARTESIAN_POINT('Ctrl Pts',(-0.083607918300789,2.41296138676534,
11.8236957992876));
#69264=CARTESIAN_POINT('Ctrl Pts',(-0.124568318091742,2.39743179102914,
11.8266152975117));
#69265=CARTESIAN_POINT('Ctrl Pts',(-0.134679767225662,2.39299207485365,
11.827337462497));
#69266=CARTESIAN_POINT('Ctrl Pts',(-0.145179240796961,2.38772324883421,
11.8280744936241));
#69267=CARTESIAN_POINT('Ctrl Pts',(-0.14581287106627,2.38740265575012,11.8281189205441));
#69268=CARTESIAN_POINT('Ctrl Pts',(-0.146717682533934,2.3869410926603,11.8281822812153));
#69269=CARTESIAN_POINT('Ctrl Pts',(-0.146989725126854,2.38680183007471,
11.8282013209847));
#69270=CARTESIAN_POINT('Ctrl Pts',(-0.147459763948895,2.38656036587058,
11.8282341996362));
#69271=CARTESIAN_POINT('Ctrl Pts',(-0.147657852710915,2.38645834567303,
11.8282480500063));
#69272=CARTESIAN_POINT('Ctrl Pts',(-0.148039362459526,2.38626135863725,
11.8282747139783));
#69273=CARTESIAN_POINT('Ctrl Pts',(-0.148222797553566,2.38616642111238,
11.8282875294092));
#69274=CARTESIAN_POINT('Ctrl Pts',(-0.14865818230571,2.38594055514912,11.8283179354342));
#69275=CARTESIAN_POINT('Ctrl Pts',(-0.148910050957868,2.38580946970068,
11.8283355160567));
#69276=CARTESIAN_POINT('Ctrl Pts',(-0.149664084723506,2.38541576429168,
11.8283881217005));
#69277=CARTESIAN_POINT('Ctrl Pts',(-0.1501657340924,2.38515215075168,11.8284230843498));
#69278=CARTESIAN_POINT('Ctrl Pts',(-0.155006881105659,2.38259184069591,
11.8287601743047));
#69279=CARTESIAN_POINT('Ctrl Pts',(-0.159294341576421,2.3801974317452,11.8290562566643));
#69280=CARTESIAN_POINT('Ctrl Pts',(-0.165386879340408,2.37660987133092,
11.8294758619985));
#69281=CARTESIAN_POINT('Ctrl Pts',(-0.167237050380818,2.37549520901356,
11.8296031327435));
#69282=CARTESIAN_POINT('Ctrl Pts',(-0.16965739164014,2.3740036707823,11.8297696084987));
#69283=CARTESIAN_POINT('Ctrl Pts',(-0.170237728877009,2.37364348671123,
11.8298095239649));
#69284=CARTESIAN_POINT('Ctrl Pts',(-0.182206386362924,2.36616237464167,
11.8306327922391));
#69285=CARTESIAN_POINT('Ctrl Pts',(-0.193140532014059,2.35833769497382,
11.8313865547347));
#69286=CARTESIAN_POINT('Ctrl Pts',(-0.212647012642128,2.34244577287646,
11.8327939443665));
#69287=CARTESIAN_POINT('Ctrl Pts',(-0.221327718684909,2.33454794245605,
11.8334470657655));
#69288=CARTESIAN_POINT('Ctrl Pts',(-0.236672016406793,2.31897546261698,
11.834685523274));
#69289=CARTESIAN_POINT('Ctrl Pts',(-0.243440550226437,2.3114250962219,11.8352672648673));
#69290=CARTESIAN_POINT('Ctrl Pts',(-0.254753569990906,2.29754052727777,
11.836319382539));
#69291=CARTESIAN_POINT('Ctrl Pts',(-0.259445219213881,2.29133688695115,
11.8367837582573));
#69292=CARTESIAN_POINT('Ctrl Pts',(-0.26447554142552,2.2841598286851,11.8373173544009));
#69293=CARTESIAN_POINT('Ctrl Pts',(-0.265039662540447,2.28334702550041,
11.8373777317379));
#69294=CARTESIAN_POINT('Ctrl Pts',(-0.265880317129291,2.28212379715537,
11.8374685232586));
#69295=CARTESIAN_POINT('Ctrl Pts',(-0.266159666204504,2.28171530647875,
11.8374988304081));
#69296=CARTESIAN_POINT('Ctrl Pts',(-0.266638088351222,2.28101224231749,
11.8375509726073));
#69297=CARTESIAN_POINT('Ctrl Pts',(-0.266837617456695,2.28071797900809,
11.8375727903431));
#69298=CARTESIAN_POINT('Ctrl Pts',(-0.26724718425741,2.28011179733906,11.8376177226416));
#69299=CARTESIAN_POINT('Ctrl Pts',(-0.267457163715863,2.27979984040434,
11.8376408393615));
#69300=CARTESIAN_POINT('Ctrl Pts',(-0.268020039298423,2.27896043389243,
11.8377030239784));
#69301=CARTESIAN_POINT('Ctrl Pts',(-0.268371922898259,2.27843231028932,
11.837742129916));
#69302=CARTESIAN_POINT('Ctrl Pts',(-0.269652033914422,2.276498705992,11.8378852432835));
#69303=CARTESIAN_POINT('Ctrl Pts',(-0.270570786436317,2.27508701255458,
11.8379896048751));
#69304=CARTESIAN_POINT('Ctrl Pts',(-0.285988659492705,2.25098576838733,
11.8397694514625));
#69305=CARTESIAN_POINT('Ctrl Pts',(-0.297595819282992,2.2265793046525,11.8415575433361));
#69306=CARTESIAN_POINT('Ctrl Pts',(-0.306993897314332,2.19810874971128,
11.8435855798235));
#69307=CARTESIAN_POINT('Ctrl Pts',(-0.307913549237319,2.19518311788768,
11.8437931629675));
#69308=CARTESIAN_POINT('Ctrl Pts',(-0.311247655873619,2.18402213070639,
11.8445812641169));
#69309=CARTESIAN_POINT('Ctrl Pts',(-0.313374665135546,2.17570435945351,
11.8451608812378));
#69310=CARTESIAN_POINT('Ctrl Pts',(-0.3174896470563,2.1564370796737,11.8464743064071));
#69311=CARTESIAN_POINT('Ctrl Pts',(-0.319248051768745,2.14544845427597,
11.8472022648895));
#69312=CARTESIAN_POINT('Ctrl Pts',(-0.320510752778471,2.13368290768133,
11.8479446849101));
#69313=CARTESIAN_POINT('Ctrl Pts',(-0.320584267995804,2.13297587076742,
11.8479891578022));
#69314=CARTESIAN_POINT('Ctrl Pts',(-0.320686057364261,2.13196438198879,
11.8480525722451));
#69315=CARTESIAN_POINT('Ctrl Pts',(-0.320716237875869,2.13166013058033,
11.8480716200598));
#69316=CARTESIAN_POINT('Ctrl Pts',(-0.320767666625017,2.13113405418223,
11.848104508174));
#69317=CARTESIAN_POINT('Ctrl Pts',(-0.320789117811177,2.1309122496268,11.8481183599797));
#69318=CARTESIAN_POINT('Ctrl Pts',(-0.32083000555721,2.13048484553704,11.8481450234474));
#69319=CARTESIAN_POINT('Ctrl Pts',(-0.320849474508391,2.13027925001634,
11.8481578369448));
#69320=CARTESIAN_POINT('Ctrl Pts',(-0.320895230721912,2.12979105699431,
11.8481882335886));
#69321=CARTESIAN_POINT('Ctrl Pts',(-0.320921342374644,2.12950844263593,
11.8482058067782));
#69322=CARTESIAN_POINT('Ctrl Pts',(-0.321011955699495,2.12851335989533,
11.8482676006445));
#69323=CARTESIAN_POINT('Ctrl Pts',(-0.321074459008251,2.12780070485117,
11.8483117094844));
#69324=CARTESIAN_POINT('Ctrl Pts',(-0.321889070701451,2.11814323507957,
11.8489075331983));
#69325=CARTESIAN_POINT('Ctrl Pts',(-0.322269600647659,2.10917003746095,
11.8494389452187));
#69326=CARTESIAN_POINT('Ctrl Pts',(-0.322284274189371,2.08450966955439,
11.8508668647107));
#69327=CARTESIAN_POINT('Ctrl Pts',(-0.321148945012806,2.06884677325038,
11.851738443188));
#69328=CARTESIAN_POINT('Ctrl Pts',(-0.315240713484417,2.02847994117197,
11.8540195117517));
#69329=CARTESIAN_POINT('Ctrl Pts',(-0.308712891507352,2.00414633866884,
11.8554360006477));
#69330=CARTESIAN_POINT('Ctrl Pts',(-0.298835027863087,1.97932949640279,
11.8570550188287));
#69331=CARTESIAN_POINT('Ctrl Pts',(-0.298231232476188,1.97784486851709,
11.8571525319499));
#69332=CARTESIAN_POINT('Ctrl Pts',(-0.297377942157259,1.9757908155867,11.8572883832299));
#69333=CARTESIAN_POINT('Ctrl Pts',(-0.297137828864432,1.97521749872879,
11.8573264032261));
#69334=CARTESIAN_POINT('Ctrl Pts',(-0.296750777633431,1.97430079115112,
11.8573873600653));
#69335=CARTESIAN_POINT('Ctrl Pts',(-0.296604897871146,1.973956953035,11.8574102608891));
#69336=CARTESIAN_POINT('Ctrl Pts',(-0.296303028280497,1.97324887352863,
11.8574574984729));
#69337=CARTESIAN_POINT('Ctrl Pts',(-0.296146963822613,1.97288466478659,
11.8574818377459));
#69338=CARTESIAN_POINT('Ctrl Pts',(-0.295782888023978,1.9720393281884,11.8575384280255));
#69339=CARTESIAN_POINT('Ctrl Pts',(-0.295574374208098,1.9715584191759,11.8575706961416));
#69340=CARTESIAN_POINT('Ctrl Pts',(-0.294909112237652,1.97003428108864,
11.8576731997394));
#69341=CARTESIAN_POINT('Ctrl Pts',(-0.29444801092008,1.96899297200225,11.8577435840178));
#69342=CARTESIAN_POINT('Ctrl Pts',(-0.285787813666087,1.94971226951271,
11.8590534412962));
#69343=CARTESIAN_POINT('Ctrl Pts',(-0.27591580065792,1.93227618811299,11.8603526939427));
#69344=CARTESIAN_POINT('Ctrl Pts',(-0.247643213747223,1.89166402675304,
11.8636627652313));
#69345=CARTESIAN_POINT('Ctrl Pts',(-0.227549557780284,1.86988627721789,
11.8657099719235));
#69346=CARTESIAN_POINT('Ctrl Pts',(-0.203623533619788,1.85019837393665,
11.8676695236398));
#69347=CARTESIAN_POINT('Ctrl Pts',(-0.202466377476437,1.84925957242019,
11.8677632342839));
#69348=CARTESIAN_POINT('Ctrl Pts',(-0.200970458605046,1.84806304076782,
11.8678829767281));
#69349=CARTESIAN_POINT('Ctrl Pts',(-0.200637663452224,1.84779792889735,
11.8679095272247));
#69350=CARTESIAN_POINT('Ctrl Pts',(-0.200109619252282,1.84737898406483,
11.8679515135071));
#69351=CARTESIAN_POINT('Ctrl Pts',(-0.199914717071086,1.84722471776537,
11.8679669803497));
#69352=CARTESIAN_POINT('Ctrl Pts',(-0.199565205221356,1.84694873403057,
11.867994661863));
#69353=CARTESIAN_POINT('Ctrl Pts',(-0.19941066367725,1.84682693358912,11.8680068824943));
#69354=CARTESIAN_POINT('Ctrl Pts',(-0.199047120205912,1.84654094965893,
11.8680355854545));
#69355=CARTESIAN_POINT('Ctrl Pts',(-0.198838026974118,1.84637688336367,
11.8680520593087));
#69356=CARTESIAN_POINT('Ctrl Pts',(-0.19823151483918,1.84590219092132,11.8680997448379));
#69357=CARTESIAN_POINT('Ctrl Pts',(-0.197833567044267,1.84559223712172,
11.8681309085613));
#69358=CARTESIAN_POINT('Ctrl Pts',(-0.195085038511268,1.84346181045368,
11.8683453085849));
#69359=CARTESIAN_POINT('Ctrl Pts',(-0.192709993592025,1.84167293050021,
11.8685263486336));
#69360=CARTESIAN_POINT('Ctrl Pts',(-0.185193755521249,1.83617307446806,
11.8690873647851));
#69361=CARTESIAN_POINT('Ctrl Pts',(-0.179967348573326,1.83258059491871,
11.8694603542844));
#69362=CARTESIAN_POINT('Ctrl Pts',(-0.161472693599664,1.8206559015049,11.8707346192801));
#69363=CARTESIAN_POINT('Ctrl Pts',(-0.147705132802424,1.81313798701479,
11.871605283269));
#69364=CARTESIAN_POINT('Ctrl Pts',(-0.110494886851804,1.79621103429578,
11.8738909348181));
#69365=CARTESIAN_POINT('Ctrl Pts',(-0.0864033617983778,1.78850191072719,
11.875313000937));
#69366=CARTESIAN_POINT('Ctrl Pts',(-0.0601407595611295,1.78338246264711,
11.8769353967941));
#69367=CARTESIAN_POINT('Ctrl Pts',(-0.0586179968316454,1.78309700816043,
11.8770296802902));
#69368=CARTESIAN_POINT('Ctrl Pts',(-0.0565504585056609,1.78272484269528,
11.8771580020592));
#69369=CARTESIAN_POINT('Ctrl Pts',(-0.0560074143208578,1.78262853100025,
11.8771917348199));
#69370=CARTESIAN_POINT('Ctrl Pts',(-0.0550874280701067,1.78246780143117,
11.8772489320117));
#69371=CARTESIAN_POINT('Ctrl Pts',(-0.0547106123608324,1.78240265940597,
11.8772723733894));
#69372=CARTESIAN_POINT('Ctrl Pts',(-0.0539851810074332,1.78227857978515,
11.8773175292657));
#69373=CARTESIAN_POINT('Ctrl Pts',(-0.0536365823558393,1.78221954486885,
11.8773392406389));
#69374=CARTESIAN_POINT('Ctrl Pts',(-0.0528146352802478,1.78208173976765,
11.8773904620561));
#69375=CARTESIAN_POINT('Ctrl Pts',(-0.0523412076390352,1.78200345305664,
11.8774199874018));
#69376=CARTESIAN_POINT('Ctrl Pts',(-0.0509626512087354,1.78177865481395,
11.8775060281071));
#69377=CARTESIAN_POINT('Ctrl Pts',(-0.0500570754135329,1.78163494927446,
11.8775626323308));
#69378=CARTESIAN_POINT('Ctrl Pts',(-0.0435855719649405,1.78063628247278,
11.8779677568109));
#69379=CARTESIAN_POINT('Ctrl Pts',(-0.0379989908904124,1.77992351479139,
11.8783207536229));
#69380=CARTESIAN_POINT('Ctrl Pts',(-0.0198728252425622,1.77809209464067,
11.8794776300977));
#69381=CARTESIAN_POINT('Ctrl Pts',(-0.00728683287487953,1.77756168578663,
11.8802992322672));
#69382=CARTESIAN_POINT('Ctrl Pts',(0.0368384164631355,1.77828700113255,
11.883235446806));
#69383=CARTESIAN_POINT('Ctrl Pts',(0.0681313773255557,1.78343340978731,
11.8854351470669));
#69384=CARTESIAN_POINT('Ctrl Pts',(0.0996567720394734,1.79351653253819,
11.8875295500734));
#69385=CARTESIAN_POINT('Ctrl Pts',(0.101132736536379,1.79400039563498,11.8876272676468));
#69386=CARTESIAN_POINT('Ctrl Pts',(0.103010142977465,1.7946309305739,11.8877510783012));
#69387=CARTESIAN_POINT('Ctrl Pts',(0.10341483798138,1.79476774513709,11.88777773818));
#69388=CARTESIAN_POINT('Ctrl Pts',(0.104057295772176,1.79498636416991,11.8878200138478));
#69389=CARTESIAN_POINT('Ctrl Pts',(0.104295235127536,1.79506764229351,11.8878356606814));
#69390=CARTESIAN_POINT('Ctrl Pts',(0.104739574125223,1.79522000575755,11.8878648607357));
#69391=CARTESIAN_POINT('Ctrl Pts',(0.104945995115022,1.79529102181243,11.8878784179014));
#69392=CARTESIAN_POINT('Ctrl Pts',(0.105409641091001,1.79545105930514,11.8879088511974));
#69393=CARTESIAN_POINT('Ctrl Pts',(0.105666824935934,1.79554019670479,11.8879257202929));
#69394=CARTESIAN_POINT('Ctrl Pts',(0.106429226274875,1.79580551993146,11.8879756920193));
#69395=CARTESIAN_POINT('Ctrl Pts',(0.106934121427034,1.79598263932137,11.8880087393361));
#69396=CARTESIAN_POINT('Ctrl Pts',(0.110979180094051,1.79741298688306,11.8882731513907));
#69397=CARTESIAN_POINT('Ctrl Pts',(0.114497816973326,1.79872681530517,11.8885009858784));
#69398=CARTESIAN_POINT('Ctrl Pts',(0.127127971983891,1.8036960641637,11.8893136682817));
#69399=CARTESIAN_POINT('Ctrl Pts',(0.136094933320498,1.80770606039616,11.8898809487722));
#69400=CARTESIAN_POINT('Ctrl Pts',(0.17334106174489,1.82644884197759,11.8922512176522));
#69401=CARTESIAN_POINT('Ctrl Pts',(0.199531473828622,1.84492233697124,11.8939730704327));
#69402=CARTESIAN_POINT('Ctrl Pts',(0.22661699792488,1.87079050115555,11.8961948397034));
#69403=CARTESIAN_POINT('Ctrl Pts',(0.23054799738413,1.87474487083542,11.8965296739284));
#69404=CARTESIAN_POINT('Ctrl Pts',(0.235042760660081,1.87950731347566,11.8969283760793));
#69405=CARTESIAN_POINT('Ctrl Pts',(0.235708014946101,1.88021861815218,11.8969878088939));
#69406=CARTESIAN_POINT('Ctrl Pts',(0.236708808978657,1.88129845961459,11.8970778647568));
#69407=CARTESIAN_POINT('Ctrl Pts',(0.237046738934835,1.88166478165217,11.8971083857105));
#69408=CARTESIAN_POINT('Ctrl Pts',(0.237649460408076,1.88232119106848,11.8971630243864));
#69409=CARTESIAN_POINT('Ctrl Pts',(0.237914574477576,1.88261098201822,11.8971871283389));
#69410=CARTESIAN_POINT('Ctrl Pts',(0.238467999778197,1.88321814523423,11.8972375934571));
#69411=CARTESIAN_POINT('Ctrl Pts',(0.238756208534521,1.88353560949364,11.8972639588897));
#69412=CARTESIAN_POINT('Ctrl Pts',(0.23951118487641,1.88437056413067,11.8973332475421));
#69413=CARTESIAN_POINT('Ctrl Pts',(0.23997690708086,1.88488899295959,11.8973762146872));
#69414=CARTESIAN_POINT('Ctrl Pts',(0.240992621419867,1.88602706131453,11.8974704201715));
#69415=CARTESIAN_POINT('Ctrl Pts',(0.241541911743713,1.88664731799404,11.897521687546));
#69416=CARTESIAN_POINT('Ctrl Pts',(0.243147718865144,1.8884747393112,11.8976725170221));
#69417=CARTESIAN_POINT('Ctrl Pts',(0.244197609384204,1.88968766912045,11.8977723533518));
#69418=CARTESIAN_POINT('Ctrl Pts',(0.255131809680098,1.90251212134189,11.8988251624081));
#69419=CARTESIAN_POINT('Ctrl Pts',(0.264187728835675,1.91480165729399,11.8998117902089));
#69420=CARTESIAN_POINT('Ctrl Pts',(0.289755626950704,1.95521084335876,11.9029850798514));
#69421=CARTESIAN_POINT('Ctrl Pts',(0.302897445200297,1.98521645232034,11.9052612673115));
#69422=CARTESIAN_POINT('Ctrl Pts',(0.311698195297557,2.01810025438366,11.9074136872392));
#69423=CARTESIAN_POINT('Ctrl Pts',(0.312068256596787,2.01952182467518,11.9075060574541));
#69424=CARTESIAN_POINT('Ctrl Pts',(0.312532393362588,2.02135613320944,11.9076243288732));
#69425=CARTESIAN_POINT('Ctrl Pts',(0.312635385857129,2.02176656597363,11.9076507334961));
#69426=CARTESIAN_POINT('Ctrl Pts',(0.312797468325896,2.02241790824809,11.9076925418296));
#69427=CARTESIAN_POINT('Ctrl Pts',(0.312857088609165,2.0226586833595,11.9077079761529));
#69428=CARTESIAN_POINT('Ctrl Pts',(0.312963522720707,2.02309065195168,11.9077356293546));
#69429=CARTESIAN_POINT('Ctrl Pts',(0.313010439018017,2.02328181808054,11.9077478541171));
#69430=CARTESIAN_POINT('Ctrl Pts',(0.313120459793668,2.02373189199893,11.9077766049823));
#69431=CARTESIAN_POINT('Ctrl Pts',(0.313183418214199,2.02399083478711,11.9077931225183));
#69432=CARTESIAN_POINT('Ctrl Pts',(0.313365403317879,2.02474338934705,11.9078410583693));
#69433=CARTESIAN_POINT('Ctrl Pts',(0.313483585405194,2.02523720756027,11.9078724279517));
#69434=CARTESIAN_POINT('Ctrl Pts',(0.314302998613926,2.02869719136046,11.9080916373238));
#69435=CARTESIAN_POINT('Ctrl Pts',(0.314963317101599,2.03167302164196,11.9082771668378));
#69436=CARTESIAN_POINT('Ctrl Pts',(0.316868720677611,2.0408755088131,11.9088429173463));
#69437=CARTESIAN_POINT('Ctrl Pts',(0.317972154470192,2.04713023912698,11.9092162532531));
#69438=CARTESIAN_POINT('Ctrl Pts',(0.321175562452994,2.06905813338983,11.910498907868));
#69439=CARTESIAN_POINT('Ctrl Pts',(0.322306833356607,2.08485036634992,11.9113771759143));
#69440=CARTESIAN_POINT('Ctrl Pts',(0.32222273102675,2.1257504314663,11.9136642529783));
#69441=CARTESIAN_POINT('Ctrl Pts',(0.319242167848216,2.15074204212297,11.9150806065274));
#69442=CARTESIAN_POINT('Ctrl Pts',(0.313052036700598,2.17656210544553,11.9166914055921));
#69443=CARTESIAN_POINT('Ctrl Pts',(0.312699795496268,2.17798827769494,11.9167808351785));
#69444=CARTESIAN_POINT('Ctrl Pts',(0.312204923070445,2.1799346765526,11.9169035280593));
#69445=CARTESIAN_POINT('Ctrl Pts',(0.312070714450355,2.1804570424628,11.9169365192217));
#69446=CARTESIAN_POINT('Ctrl Pts',(0.311839952112226,2.18134594990796,11.9169927690346));
#69447=CARTESIAN_POINT('Ctrl Pts',(0.311744061507356,2.18171266372291,11.9170160061959));
#69448=CARTESIAN_POINT('Ctrl Pts',(0.311549303120863,2.18245214418087,11.9170629282279));
#69449=CARTESIAN_POINT('Ctrl Pts',(0.311450412739822,2.18282490420944,11.9170866137991));
#69450=CARTESIAN_POINT('Ctrl Pts',(0.311231151082831,2.18364544949951,11.9171388251013));
#69451=CARTESIAN_POINT('Ctrl Pts',(0.311110482187376,2.18409315368016,11.9171673604459));
#69452=CARTESIAN_POINT('Ctrl Pts',(0.310851205469512,2.18504692232507,11.9172282536997));
#69453=CARTESIAN_POINT('Ctrl Pts',(0.310712327242414,2.18555291130754,11.9172606203346));
#69454=CARTESIAN_POINT('Ctrl Pts',(0.310347304674683,2.18687022212318,11.9173450470936));
#69455=CARTESIAN_POINT('Ctrl Pts',(0.31011921547614,2.18768099669506,11.9173971704074));
#69456=CARTESIAN_POINT('Ctrl Pts',(0.309437452251883,2.19006847722662,11.9175511359824));
#69457=CARTESIAN_POINT('Ctrl Pts',(0.308974918309365,2.19164260549263,11.9176532663039));
#69458=CARTESIAN_POINT('Ctrl Pts',(0.30391269167118,2.20839667470287,11.9187469789045));
#69459=CARTESIAN_POINT('Ctrl Pts',(0.298211056544918,2.22321848218613,11.919775051054));
#69460=CARTESIAN_POINT('Ctrl Pts',(0.27787342459795,2.2663073864259,11.9229431098404));
#69461=CARTESIAN_POINT('Ctrl Pts',(0.260126349595312,2.29288862247379,11.9251609732479));
#69462=CARTESIAN_POINT('Ctrl Pts',(0.237734888667022,2.31759067874664,11.9272706180569));
#69463=CARTESIAN_POINT('Ctrl Pts',(0.236685022506325,2.31873221325915,11.9273681869276));
#69464=CARTESIAN_POINT('Ctrl Pts',(0.235335654474263,2.32017830874775,11.9274918353485));
#69465=CARTESIAN_POINT('Ctrl Pts',(0.235043754869597,2.32048988913702,11.927518479916));
#69466=CARTESIAN_POINT('Ctrl Pts',(0.234579006285329,2.32098400083996,11.9275607367477));
#69467=CARTESIAN_POINT('Ctrl Pts',(0.234406562734848,2.32116691019436,11.9275763800102));
#69468=CARTESIAN_POINT('Ctrl Pts',(0.234083967020305,2.3215082835132,11.9276055768478));
#69469=CARTESIAN_POINT('Ctrl Pts',(0.233933868985738,2.3216667954898,11.9276191343596));
#69470=CARTESIAN_POINT('Ctrl Pts',(0.233596202296759,2.32202266557389,11.9276495728457));
#69471=CARTESIAN_POINT('Ctrl Pts',(0.233408544976355,2.32221993810038,11.9276664467746));
#69472=CARTESIAN_POINT('Ctrl Pts',(0.232851108099107,2.32280445187023,11.9277164467658));
#69473=CARTESIAN_POINT('Ctrl Pts',(0.232480610926652,2.32319101207061,11.9277495174197));
#69474=CARTESIAN_POINT('Ctrl Pts',(0.229496020341915,2.32628950549246,11.9280146456769));
#69475=CARTESIAN_POINT('Ctrl Pts',(0.226835392082965,2.32895648398696,11.9282431515341));
#69476=CARTESIAN_POINT('Ctrl Pts',(0.217036305224036,2.33844041663441,11.92905962284));
#69477=CARTESIAN_POINT('Ctrl Pts',(0.209631890823145,2.34497570336214,11.9296298266413));
#69478=CARTESIAN_POINT('Ctrl Pts',(0.191237395366663,2.35976523321532,11.9309712492244));
#69479=CARTESIAN_POINT('Ctrl Pts',(0.179997022229583,2.36767669349779,11.9317328745752));
#69480=CARTESIAN_POINT('Ctrl Pts',(0.148640230057736,2.38687611980003,11.9337927806612));
#69481=CARTESIAN_POINT('Ctrl Pts',(0.127764831403284,2.39676209536793,11.9351037140861));
#69482=CARTESIAN_POINT('Ctrl Pts',(0.104736435116182,2.40478400597705,11.9365842368593));
#69483=CARTESIAN_POINT('Ctrl Pts',(0.103454245097934,2.4052216083831,11.936666754527));
#69484=CARTESIAN_POINT('Ctrl Pts',(0.101675156603859,2.40581630052915,11.9367813799651));
#69485=CARTESIAN_POINT('Ctrl Pts',(0.101180566586012,2.40598029361391,11.9368132597954));
#69486=CARTESIAN_POINT('Ctrl Pts',(0.100330205310402,2.40625996388917,11.9368680960105));
#69487=CARTESIAN_POINT('Ctrl Pts',(0.0999746252684269,2.4063762227712,11.9368910331859));
#69488=CARTESIAN_POINT('Ctrl Pts',(0.0992603919978063,2.40660836953332,
11.9369371207987));
#69489=CARTESIAN_POINT('Ctrl Pts',(0.0989017362848541,2.4067242478928,11.9369602715091));
#69490=CARTESIAN_POINT('Ctrl Pts',(0.0980657832762865,2.4069927179476,11.9370142491381));
#69491=CARTESIAN_POINT('Ctrl Pts',(0.0975883327136098,2.40714482583319,
11.9370450919026));
#69492=CARTESIAN_POINT('Ctrl Pts',(0.0961293001700396,2.4076059041071,11.9371393867013));
#69493=CARTESIAN_POINT('Ctrl Pts',(0.0951465985366241,2.40791128485376,
11.9372029563425));
#69494=CARTESIAN_POINT('Ctrl Pts',(0.0928870560330176,2.40860160228108,
11.9373492659192));
#69495=CARTESIAN_POINT('Ctrl Pts',(0.0916092612740967,2.40898332846891,
11.9374321098634));
#69496=CARTESIAN_POINT('Ctrl Pts',(0.0873955585469937,2.41021368708271,
11.9377056604697));
#69497=CARTESIAN_POINT('Ctrl Pts',(0.0844500168335711,2.41102846964457,
11.9378974603774));
#69498=CARTESIAN_POINT('Ctrl Pts',(0.0724967516520152,2.41415261514852,
11.9386783188074));
#69499=CARTESIAN_POINT('Ctrl Pts',(0.0634033320567419,2.41611332574865,
11.9392782776601));
#69500=CARTESIAN_POINT('Ctrl Pts',(0.0382237152840651,2.42041235076216,
11.9409549749743));
#69501=CARTESIAN_POINT('Ctrl Pts',(0.0220263157463984,2.42193148861396,
11.9420517138141));
#69502=CARTESIAN_POINT('Ctrl Pts',(-0.0142620859097455,2.4225829854974,
11.9445078361993));
#69503=CARTESIAN_POINT('Ctrl Pts',(-0.0343015208324877,2.421071318454,11.9458638563658));
#69504=CARTESIAN_POINT('Ctrl Pts',(-0.055237241858519,2.41750813990561,
11.9472030730987));
#69505=CARTESIAN_POINT('Ctrl Pts',(-0.0564010099644147,2.41730347929402,
11.9472772506192));
#69506=CARTESIAN_POINT('Ctrl Pts',(-0.0579458128205222,2.41702304216756,
11.9473753367658));
#69507=CARTESIAN_POINT('Ctrl Pts',(-0.058327854988515,2.41695297415362,
11.9473995634741));
#69508=CARTESIAN_POINT('Ctrl Pts',(-0.0589224359550742,2.41684281425423,
11.947437219113));
#69509=CARTESIAN_POINT('Ctrl Pts',(-0.0591350610163383,2.41680319910424,
11.9474506752031));
#69510=CARTESIAN_POINT('Ctrl Pts',(-0.0595411298601977,2.41672711950472,
11.9474763546452));
#69511=CARTESIAN_POINT('Ctrl Pts',(-0.0597345787697421,2.41669069211817,
11.9474885799867));
#69512=CARTESIAN_POINT('Ctrl Pts',(-0.0601899289174849,2.41660451536295,
11.9475173374345));
#69513=CARTESIAN_POINT('Ctrl Pts',(-0.0604518015141238,2.41655461833028,
11.9475338609617));
#69514=CARTESIAN_POINT('Ctrl Pts',(-0.0612127313247458,2.41640865259135,
11.9475818311893));
#69515=CARTESIAN_POINT('Ctrl Pts',(-0.0617116264791871,2.41631172769368,
11.9476132290494));
#69516=CARTESIAN_POINT('Ctrl Pts',(-0.0652111528068321,2.41562324830059,
11.9478331101284));
#69517=CARTESIAN_POINT('Ctrl Pts',(-0.0682035880346649,2.41499016103255,
11.9480192669058));
#69518=CARTESIAN_POINT('Ctrl Pts',(-0.0773541649728065,2.41291771711632,
11.9485840471005));
#69519=CARTESIAN_POINT('Ctrl Pts',(-0.0834796232035285,2.41133957013502,
11.9489558759193));
#69520=CARTESIAN_POINT('Ctrl Pts',(-0.104267788750449,2.4053260257712,11.9502085157357));
#69521=CARTESIAN_POINT('Ctrl Pts',(-0.118659356281344,2.40002628499509,
11.9510604433797));
#69522=CARTESIAN_POINT('Ctrl Pts',(-0.139700753455025,2.39052578260807,
11.9523511284678));
#69523=CARTESIAN_POINT('Ctrl Pts',(-0.146663289992089,2.38707386884959,
11.9527860036273));
#69524=CARTESIAN_POINT('Ctrl Pts',(-0.165004478480103,2.3771390577625,11.9539657056869));
#69525=CARTESIAN_POINT('Ctrl Pts',(-0.176123148351679,2.37020940025921,
11.9547181227331));
#69526=CARTESIAN_POINT('Ctrl Pts',(-0.191249313945377,2.35945102414004,
11.9558197711838));
#69527=CARTESIAN_POINT('Ctrl Pts',(-0.195627870514173,2.35616569793313,
11.9561485939121));
#69528=CARTESIAN_POINT('Ctrl Pts',(-0.20061255038541,2.35222323222255,11.9565355474609));
#69529=CARTESIAN_POINT('Ctrl Pts',(-0.201302384122906,2.35167301080386,
11.9565893856552));
#69530=CARTESIAN_POINT('Ctrl Pts',(-0.202396779152602,2.35079272719641,
11.9566752607316));
#69531=CARTESIAN_POINT('Ctrl Pts',(-0.202802816422597,2.35046450022299,
11.9567072238346));
#69532=CARTESIAN_POINT('Ctrl Pts',(-0.203516472054414,2.34988473168529,
11.9567635836033));
#69533=CARTESIAN_POINT('Ctrl Pts',(-0.203824426925171,2.3496336045353,11.9567879634999));
#69534=CARTESIAN_POINT('Ctrl Pts',(-0.20441530110516,2.34914994363757,11.9568348565242));
#69535=CARTESIAN_POINT('Ctrl Pts',(-0.204698290214955,2.34891749581303,
11.9568573661455));
#69536=CARTESIAN_POINT('Ctrl Pts',(-0.205439747869139,2.3483063415082,11.9569164778506));
#69537=CARTESIAN_POINT('Ctrl Pts',(-0.20589756396956,2.34792684885174,11.9569531118843));
#69538=CARTESIAN_POINT('Ctrl Pts',(-0.207552874278974,2.34654698283765,
11.9570860618835));
#69539=CARTESIAN_POINT('Ctrl Pts',(-0.208744134628662,2.345539195422,11.9571826806891));
#69540=CARTESIAN_POINT('Ctrl Pts',(-0.211624607772102,2.34306624821065,
11.9574186303411));
#69541=CARTESIAN_POINT('Ctrl Pts',(-0.213305961844113,2.34159209811111,
11.9575583309558));
#69542=CARTESIAN_POINT('Ctrl Pts',(-0.21954818525648,2.33600318229971,11.9580845359022));
#69543=CARTESIAN_POINT('Ctrl Pts',(-0.224006212412139,2.33177600454659,
11.9584757180441));
#69544=CARTESIAN_POINT('Ctrl Pts',(-0.232800997142482,2.32294578708031,
11.9592797713753));
#69545=CARTESIAN_POINT('Ctrl Pts',(-0.237128531158594,2.31833730790587,
11.9596927696632));
#69546=CARTESIAN_POINT('Ctrl Pts',(-0.264136268315157,2.28782562682128,
11.9623833732619));
#69547=CARTESIAN_POINT('Ctrl Pts',(-0.282674580828835,2.25855998744229,
11.9647980413033));
#69548=CARTESIAN_POINT('Ctrl Pts',(-0.296742751309248,2.22572430624604,
11.9670532449211));
#69549=CARTESIAN_POINT('Ctrl Pts',(-0.297246903106023,2.22452766907421,
11.9671348168656));
#69550=CARTESIAN_POINT('Ctrl Pts',(-0.297898156102656,2.22295538569893,
11.9672411607182));
#69551=CARTESIAN_POINT('Ctrl Pts',(-0.298051794890168,2.2225824858971,11.9672663210735));
#69552=CARTESIAN_POINT('Ctrl Pts',(-0.298287890024066,2.22200638662459,
11.9673050960571));
#69553=CARTESIAN_POINT('Ctrl Pts',(-0.298370838962983,2.22180339145282,
11.9673187405576));
#69554=CARTESIAN_POINT('Ctrl Pts',(-0.298535926514821,2.22139820358291,
11.9673459388737));
#69555=CARTESIAN_POINT('Ctrl Pts',(-0.298618066365931,2.22119601352165,
11.9673594926504));
#69556=CARTESIAN_POINT('Ctrl Pts',(-0.2988018940132,2.22074219401556,11.9673898735181));
#69557=CARTESIAN_POINT('Ctrl Pts',(-0.298903469124256,2.22049052007669,
11.9674066936813));
#69558=CARTESIAN_POINT('Ctrl Pts',(-0.299202920669377,2.21974585621456,
11.9674563796927));
#69559=CARTESIAN_POINT('Ctrl Pts',(-0.299399897464345,2.21925250196752,
11.9674891911753));
#69560=CARTESIAN_POINT('Ctrl Pts',(-0.300938493977236,2.21537104325906,
11.9677465161175));
#69561=CARTESIAN_POINT('Ctrl Pts',(-0.302223848577097,2.21196072020821,
11.9679677083848));
#69562=CARTESIAN_POINT('Ctrl Pts',(-0.306585057431664,2.19976663452508,
11.968743790018));
#69563=CARTESIAN_POINT('Ctrl Pts',(-0.309338236253323,2.19087169219695,
11.9692829243192));
#69564=CARTESIAN_POINT('Ctrl Pts',(-0.318707330195921,2.15520055744231,
11.9713842265054));
#69565=CARTESIAN_POINT('Ctrl Pts',(-0.322260151683405,2.12774507942207,
11.9728789771032));
#69566=CARTESIAN_POINT('Ctrl Pts',(-0.322274953560087,2.10017301110915,
11.9744805487749));
#69567=CARTESIAN_POINT('',(-0.322759928630395,2.09993784294859,12.2247412594466));
#69568=CARTESIAN_POINT('Ctrl Pts',(-0.322274953770146,2.10017261938011,
11.9744805715291));
#69569=CARTESIAN_POINT('Ctrl Pts',(-0.322280140850064,2.09048850430689,
11.9750430905345));
#69570=CARTESIAN_POINT('Ctrl Pts',(-0.321848831765366,2.08080970305467,
11.9756163851485));
#69571=CARTESIAN_POINT('Ctrl Pts',(-0.320889619698775,2.07013188223727,
11.9762666160024));
#69572=CARTESIAN_POINT('Ctrl Pts',(-0.320791782188379,2.06909878755829,
11.9763297091459));
#69573=CARTESIAN_POINT('Ctrl Pts',(-0.320628924429427,2.06746332065255,
11.9764298860425));
#69574=CARTESIAN_POINT('Ctrl Pts',(-0.320567191588716,2.06686062232353,
11.9764668666521));
#69575=CARTESIAN_POINT('Ctrl Pts',(-0.320459192676731,2.06583477427253,
11.9765299208147));
#69576=CARTESIAN_POINT('Ctrl Pts',(-0.320413786902972,2.06541153400647,
11.97655596728));
#69577=CARTESIAN_POINT('Ctrl Pts',(-0.320327716372621,2.06462396092436,
11.9766044947544));
#69578=CARTESIAN_POINT('Ctrl Pts',(-0.320287268185173,2.06425960473219,
11.9766269689109));
#69579=CARTESIAN_POINT('Ctrl Pts',(-0.320202109701468,2.06350425444715,
11.9766736100176));
#69580=CARTESIAN_POINT('Ctrl Pts',(-0.320157304747916,2.06311327182989,
11.9766977799149));
#69581=CARTESIAN_POINT('Ctrl Pts',(-0.320053374576734,2.06222079889792,
11.976753014664));
#69582=CARTESIAN_POINT('Ctrl Pts',(-0.319993786735539,2.06171936442678,
11.9767840940578));
#69583=CARTESIAN_POINT('Ctrl Pts',(-0.319807920601414,2.06018605444385,
11.9768792715208));
#69584=CARTESIAN_POINT('Ctrl Pts',(-0.319677828682961,2.05915465573492,
11.9769434897918));
#69585=CARTESIAN_POINT('Ctrl Pts',(-0.318679712191136,2.05153835440923,
11.9774191779939));
#69586=CARTESIAN_POINT('Ctrl Pts',(-0.317613353017002,2.04498148074331,
11.9778368872331));
#69587=CARTESIAN_POINT('Ctrl Pts',(-0.315932899967771,2.03634277701505,
11.9783987082447));
#69588=CARTESIAN_POINT('Ctrl Pts',(-0.315499250006797,2.03422719243243,
11.9785372131014));
#69589=CARTESIAN_POINT('Ctrl Pts',(-0.314578913072934,2.02995596973158,
11.9788187064767));
#69590=CARTESIAN_POINT('Ctrl Pts',(-0.314091250581152,2.02780066014975,
11.978961716818));
#69591=CARTESIAN_POINT('Ctrl Pts',(-0.307367604592412,1.99944252826692,
11.9808560295979));
#69592=CARTESIAN_POINT('Ctrl Pts',(-0.29789291162276,1.97411874585603,11.9827037981042));
#69593=CARTESIAN_POINT('Ctrl Pts',(-0.281047570084969,1.94201107663383,
11.9851321291597));
#69594=CARTESIAN_POINT('Ctrl Pts',(-0.276355449123813,1.93393997442173,
11.9857492851136));
#69595=CARTESIAN_POINT('Ctrl Pts',(-0.269349813934889,1.92301081340079,
11.9865836565265));
#69596=CARTESIAN_POINT('Ctrl Pts',(-0.267328199079778,1.91997185991686,
11.9868154957117));
#69597=CARTESIAN_POINT('Ctrl Pts',(-0.264953485993235,1.91653036141997,
11.9870772574279));
#69598=CARTESIAN_POINT('Ctrl Pts',(-0.264650594565342,1.916093717273,11.9871104539786));
#69599=CARTESIAN_POINT('Ctrl Pts',(-0.264191359206747,1.91543517392646,
11.9871604959271));
#69600=CARTESIAN_POINT('Ctrl Pts',(-0.264035814569343,1.91521272249132,
11.9871773954587));
#69601=CARTESIAN_POINT('Ctrl Pts',(-0.263754702030048,1.91481177032229,
11.9872078474552));
#69602=CARTESIAN_POINT('Ctrl Pts',(-0.263629234181853,1.9146332010857,11.987221406697));
#69603=CARTESIAN_POINT('Ctrl Pts',(-0.263377344520193,1.91427547793548,
11.9872485636152));
#69604=CARTESIAN_POINT('Ctrl Pts',(-0.263250921824196,1.91409632638916,
11.9872621611223));
#69605=CARTESIAN_POINT('Ctrl Pts',(-0.262891507522944,1.91358810803321,
11.9873007266314));
#69606=CARTESIAN_POINT('Ctrl Pts',(-0.262658080023907,1.91325934776626,
11.9873256646614));
#69607=CARTESIAN_POINT('Ctrl Pts',(-0.261670835978958,1.9118744224225,11.9874306815702));
#69608=CARTESIAN_POINT('Ctrl Pts',(-0.260911247895749,1.91082235809651,
11.9875103689434));
#69609=CARTESIAN_POINT('Ctrl Pts',(-0.239813944938682,1.88197041301535,
11.9896941254943));
#69610=CARTESIAN_POINT('Ctrl Pts',(-0.215152759056864,1.85759965938156,
11.9915162503771));
#69611=CARTESIAN_POINT('Ctrl Pts',(-0.178630626541909,1.83155943299207,
11.9940749490111));
#69612=CARTESIAN_POINT('Ctrl Pts',(-0.169880079880557,1.82593802132801,
11.9946775529013));
#69613=CARTESIAN_POINT('Ctrl Pts',(-0.157875553349675,1.81902231789463,
11.9955010447022));
#69614=CARTESIAN_POINT('Ctrl Pts',(-0.154849820146373,1.81734353003614,
11.9957083186952));
#69615=CARTESIAN_POINT('Ctrl Pts',(-0.150507733696608,1.81502502520281,
11.9960056453086));
#69616=CARTESIAN_POINT('Ctrl Pts',(-0.149213083247758,1.81434501607311,
11.9960942813772));
#69617=CARTESIAN_POINT('Ctrl Pts',(-0.146928124361533,1.81316462405401,
11.9962507116368));
#69618=CARTESIAN_POINT('Ctrl Pts',(-0.145939769705516,1.81266049663759,
11.9963183733908));
#69619=CARTESIAN_POINT('Ctrl Pts',(-0.144487299898654,1.8119290663169,11.9964178124959));
#69620=CARTESIAN_POINT('Ctrl Pts',(-0.144025202468255,1.81169775631445,
11.9964494493051));
#69621=CARTESIAN_POINT('Ctrl Pts',(-0.143228510114815,1.81130135309551,
11.9965039955819));
#69622=CARTESIAN_POINT('Ctrl Pts',(-0.142894180152883,1.81113572718191,
11.9965268863734));
#69623=CARTESIAN_POINT('Ctrl Pts',(-0.142229191429349,1.81080773103358,
11.9965724180849));
#69624=CARTESIAN_POINT('Ctrl Pts',(-0.141898540346243,1.8106453463819,11.9965950584603));
#69625=CARTESIAN_POINT('Ctrl Pts',(-0.14111925679983,1.81026429272008,11.9966484197235));
#69626=CARTESIAN_POINT('Ctrl Pts',(-0.140670394317473,1.81004609871425,
11.9966791570994));
#69627=CARTESIAN_POINT('Ctrl Pts',(-0.139343993182991,1.80940513425141,
11.9967699927608));
#69628=CARTESIAN_POINT('Ctrl Pts',(-0.138465048435954,1.80898530146423,
11.9968301929278));
#69629=CARTESIAN_POINT('Ctrl Pts',(-0.130677267381999,1.80530869362934,
11.9973636780659));
#69630=CARTESIAN_POINT('Ctrl Pts',(-0.123657102274845,1.80229474429172,
11.9978452864166));
#69631=CARTESIAN_POINT('Ctrl Pts',(-0.0973871452182989,1.792105861998,11.9996522730904));
#69632=CARTESIAN_POINT('Ctrl Pts',(-0.077573843073094,1.78652731697814,
12.0010283370725));
#69633=CARTESIAN_POINT('Ctrl Pts',(-0.0552039993273162,1.78248066367391,
12.0025663110488));
#69634=CARTESIAN_POINT('Ctrl Pts',(-0.0530363378706432,1.78211140734768,
12.0027151318981));
#69635=CARTESIAN_POINT('Ctrl Pts',(-0.0483532023407551,1.78136288020533,
12.003036050105));
#69636=CARTESIAN_POINT('Ctrl Pts',(-0.0458366618553275,1.78099114933279,
12.0032081263859));
#69637=CARTESIAN_POINT('Ctrl Pts',(-0.0258175782646707,1.77827580842671,
12.0045730993834));
#69638=CARTESIAN_POINT('Ctrl Pts',(-0.00815113662796364,1.77734424781082,
12.0057557076176));
#69639=CARTESIAN_POINT('Ctrl Pts',(0.0102113679736316,1.77788603971825,
12.0069082379681));
#69640=CARTESIAN_POINT('Ctrl Pts',(0.0109179768508587,1.77790921582853,
12.0069524680628));
#69641=CARTESIAN_POINT('Ctrl Pts',(0.0119293765709213,1.77794572093613,
12.0070155984508));
#69642=CARTESIAN_POINT('Ctrl Pts',(0.012234227252519,1.77795715754873,12.007034603713));
#69643=CARTESIAN_POINT('Ctrl Pts',(0.0127616123662588,1.77797769257668,
12.0070674417965));
#69644=CARTESIAN_POINT('Ctrl Pts',(0.0129841540810078,1.77798658883144,
12.0070812860292));
#69645=CARTESIAN_POINT('Ctrl Pts',(0.013413196383939,1.77800418557804,12.0071079522445));
#69646=CARTESIAN_POINT('Ctrl Pts',(0.0136196973612327,1.77801285400363,
12.0071207760293));
#69647=CARTESIAN_POINT('Ctrl Pts',(0.0141103867407583,1.77803392488116,
12.0071512225435));
#69648=CARTESIAN_POINT('Ctrl Pts',(0.0143945679148747,1.7780465049772,12.0071688352387));
#69649=CARTESIAN_POINT('Ctrl Pts',(0.0152468967022026,1.77808536652297,
12.0072216001003));
#69650=CARTESIAN_POINT('Ctrl Pts',(0.0158149956011329,1.77811277591143,
12.0072566893676));
#69651=CARTESIAN_POINT('Ctrl Pts',(0.0213507606199708,1.77839455385049,
12.0075978595259));
#69652=CARTESIAN_POINT('Ctrl Pts',(0.0263123131510297,1.77876241380163,
12.0078977348205));
#69653=CARTESIAN_POINT('Ctrl Pts',(0.0316003009612357,1.77927782896817,
12.0082129091073));
#69654=CARTESIAN_POINT('Ctrl Pts',(0.0319368670015658,1.77931116866954,
12.0082329498713));
#69655=CARTESIAN_POINT('Ctrl Pts',(0.0326193524279296,1.77937985967693,
12.0082735504688));
#69656=CARTESIAN_POINT('Ctrl Pts',(0.0329652683854436,1.77941524113622,
12.0082941090338));
#69657=CARTESIAN_POINT('Ctrl Pts',(0.0337575093247992,1.7794975700599,12.0083411498375));
#69658=CARTESIAN_POINT('Ctrl Pts',(0.0342037957024968,1.77954489020023,
12.008367617034));
#69659=CARTESIAN_POINT('Ctrl Pts',(0.0360959270022173,1.77974951228507,
12.0084797007805));
#69660=CARTESIAN_POINT('Ctrl Pts',(0.0375408164208962,1.7799156704009,12.0085649696864));
#69661=CARTESIAN_POINT('Ctrl Pts',(0.0696308772562227,1.7838262169437,12.0104525461949));
#69662=CARTESIAN_POINT('Ctrl Pts',(0.0995833500407337,1.79194504281586,
12.0121040237752));
#69663=CARTESIAN_POINT('Ctrl Pts',(0.135602593779702,1.80752252732983,12.014366563192));
#69664=CARTESIAN_POINT('Ctrl Pts',(0.143146923892467,1.81114003921337,12.0148561730258));
#69665=CARTESIAN_POINT('Ctrl Pts',(0.153026876241346,1.81635964457534,12.0155236012933));
#69666=CARTESIAN_POINT('Ctrl Pts',(0.155494798840177,1.81770504279601,12.0156925699906));
#69667=CARTESIAN_POINT('Ctrl Pts',(0.159037209010758,1.81969674900383,12.0159385279017));
#69668=CARTESIAN_POINT('Ctrl Pts',(0.160126062786958,1.82031733997859,12.0160146035594));
#69669=CARTESIAN_POINT('Ctrl Pts',(0.162059132023687,1.82143407931396,12.0161505233134));
#69670=CARTESIAN_POINT('Ctrl Pts',(0.162904762613146,1.82192775628501,12.0162102780267));
#69671=CARTESIAN_POINT('Ctrl Pts',(0.164170518899697,1.82267445689397,12.0163001703966));
#69672=CARTESIAN_POINT('Ctrl Pts',(0.164592343648889,1.82292460133961,12.0163302033129));
#69673=CARTESIAN_POINT('Ctrl Pts',(0.165340284638635,1.82337044526916,12.0163835898017));
#69674=CARTESIAN_POINT('Ctrl Pts',(0.165666629225812,1.82356576146592,12.0164069293558));
#69675=CARTESIAN_POINT('Ctrl Pts',(0.166317488049061,1.82395686489884,12.016453569345));
#69676=CARTESIAN_POINT('Ctrl Pts',(0.166642004204567,1.82415264782818,12.0164768695978));
#69677=CARTESIAN_POINT('Ctrl Pts',(0.167521828158983,1.82468557112558,12.0165401655595));
#69678=CARTESIAN_POINT('Ctrl Pts',(0.168076460918846,1.82502381751995,12.0165802017942));
#69679=CARTESIAN_POINT('Ctrl Pts',(0.170148333428435,1.82629597287729,12.0167302695134));
#69680=CARTESIAN_POINT('Ctrl Pts',(0.171658821171498,1.82724076781729,12.0168407013711));
#69681=CARTESIAN_POINT('Ctrl Pts',(0.175211939345334,1.82950441148556,12.0171029417462));
#69682=CARTESIAN_POINT('Ctrl Pts',(0.177247609027421,1.83083393291993,12.017255143187));
#69683=CARTESIAN_POINT('Ctrl Pts',(0.20798603168023,1.85140949010392,12.0195837696654));
#69684=CARTESIAN_POINT('Ctrl Pts',(0.233420781080795,1.87512447848566,12.0219535093765));
#69685=CARTESIAN_POINT('Ctrl Pts',(0.261660880641864,1.91151269188097,12.0250376035386));
#69686=CARTESIAN_POINT('Ctrl Pts',(0.268231536649158,1.92098663329777,12.0257969754443));
#69687=CARTESIAN_POINT('Ctrl Pts',(0.275107559463095,1.93213254313696,12.0266255969777));
#69688=CARTESIAN_POINT('Ctrl Pts',(0.275924042788517,1.93347800386039,12.0267245912393));
#69689=CARTESIAN_POINT('Ctrl Pts',(0.276943137679035,1.93518541933912,12.0268488659962));
#69690=CARTESIAN_POINT('Ctrl Pts',(0.277154932863702,1.93554182689864,12.0268747333587));
#69691=CARTESIAN_POINT('Ctrl Pts',(0.277491370211385,1.93611047726076,12.0269158860523));
#69692=CARTESIAN_POINT('Ctrl Pts',(0.277616457102722,1.93632245434332,12.0269312003843));
#69693=CARTESIAN_POINT('Ctrl Pts',(0.277852410815398,1.93672335925277,12.0269601139595));
#69694=CARTESIAN_POINT('Ctrl Pts',(0.277963326941763,1.93691225525686,12.0269737163535));
#69695=CARTESIAN_POINT('Ctrl Pts',(0.27821571869168,1.93734309713439,12.0270046937703));
#69696=CARTESIAN_POINT('Ctrl Pts',(0.278357071102478,1.9375851141501,12.0270220606746));
#69697=CARTESIAN_POINT('Ctrl Pts',(0.278777785747945,1.93830760470921,12.0270738053249));
#69698=CARTESIAN_POINT('Ctrl Pts',(0.27905622279983,1.9387886199768,12.0271081230882));
#69699=CARTESIAN_POINT('Ctrl Pts',(0.28100055262145,1.94216768735413,12.0273482902683));
#69700=CARTESIAN_POINT('Ctrl Pts',(0.282622589395207,1.94509091834847,12.0275513708062));
#69701=CARTESIAN_POINT('Ctrl Pts',(0.29119679547267,1.96112648055801,12.0286430231439));
#69702=CARTESIAN_POINT('Ctrl Pts',(0.297283141535621,1.9746833410916,12.0294860460318));
#69703=CARTESIAN_POINT('Ctrl Pts',(0.312862952454075,2.01698221442692,12.0320172654897));
#69704=CARTESIAN_POINT('Ctrl Pts',(0.31926737670666,2.04667686674732,12.0336783332231));
#69705=CARTESIAN_POINT('Ctrl Pts',(0.321580447391477,2.07876421940431,12.035613415307));
#69706=CARTESIAN_POINT('Ctrl Pts',(0.321702502145319,2.08070123360885,12.0357306860977));
#69707=CARTESIAN_POINT('Ctrl Pts',(0.321858381398105,2.08359067671234,12.035906344017));
#69708=CARTESIAN_POINT('Ctrl Pts',(0.321905491017937,2.08454236793351,12.0359643172929));
#69709=CARTESIAN_POINT('Ctrl Pts',(0.321974074254386,2.08606454058975,12.0360572344727));
#69710=CARTESIAN_POINT('Ctrl Pts',(0.321998254030737,2.08663489934523,12.0360920937599));
#69711=CARTESIAN_POINT('Ctrl Pts',(0.322041394546881,2.08772067443161,12.03615853778));
#69712=CARTESIAN_POINT('Ctrl Pts',(0.322060633704833,2.08823607842296,12.0361901137055));
#69713=CARTESIAN_POINT('Ctrl Pts',(0.322092232953702,2.08914086258905,12.0362456083718));
#69714=CARTESIAN_POINT('Ctrl Pts',(0.322105124432119,2.08953022412738,12.0362695104124));
#69715=CARTESIAN_POINT('Ctrl Pts',(0.322128919842068,2.09029060253867,12.0363162290804));
#69716=CARTESIAN_POINT('Ctrl Pts',(0.322139888863817,2.09066161691207,12.0363390436313));
#69717=CARTESIAN_POINT('Ctrl Pts',(0.322164407076842,2.09154242853018,12.0363932521324));
#69718=CARTESIAN_POINT('Ctrl Pts',(0.322177387164284,2.09205223946233,12.0364246638698));
#69719=CARTESIAN_POINT('Ctrl Pts',(0.3222188912953,2.09385007744737,12.0365355651537));
#69720=CARTESIAN_POINT('Ctrl Pts',(0.322240901448385,2.09513822960247,12.0366152584823));
#69721=CARTESIAN_POINT('Ctrl Pts',(0.322461903787939,2.11506783318796,12.037851915141));
#69722=CARTESIAN_POINT('Ctrl Pts',(0.321050746486486,2.13368853336305,12.0390604100042));
#69723=CARTESIAN_POINT('Ctrl Pts',(0.314989707775189,2.17070158703793,12.0415625759917));
#69724=CARTESIAN_POINT('Ctrl Pts',(0.310311048848054,2.18901817897884,12.0428521251548));
#69725=CARTESIAN_POINT('Ctrl Pts',(0.300207171021233,2.21777836571666,12.0448937540188));
#69726=CARTESIAN_POINT('Ctrl Pts',(0.295767140814976,2.22852217518522,12.045659689364));
#69727=CARTESIAN_POINT('Ctrl Pts',(0.2900743104949,2.24042994220696,12.046494839577));
#69728=CARTESIAN_POINT('Ctrl Pts',(0.289382016876861,2.24185105860879,12.0465942748824));
#69729=CARTESIAN_POINT('Ctrl Pts',(0.288494693224047,2.24363899196686,12.0467190249983));
#69730=CARTESIAN_POINT('Ctrl Pts',(0.288309388200623,2.24401057152752,12.0467449320832));
#69731=CARTESIAN_POINT('Ctrl Pts',(0.288013032149422,2.24460196951414,12.0467861332633));
#69732=CARTESIAN_POINT('Ctrl Pts',(0.287902447185933,2.24482201897709,12.0468014564773));
#69733=CARTESIAN_POINT('Ctrl Pts',(0.287693034878547,2.24523753399328,12.0468303773267));
#69734=CARTESIAN_POINT('Ctrl Pts',(0.287594261319001,2.24543302394837,12.0468439781344));
#69735=CARTESIAN_POINT('Ctrl Pts',(0.287368747479664,2.24587822666639,12.0468749392419));
#69736=CARTESIAN_POINT('Ctrl Pts',(0.287241881193742,2.246127874593,12.0468922914552));
#69737=CARTESIAN_POINT('Ctrl Pts',(0.28685413169894,2.24688843331047,12.0469451281181));
#69738=CARTESIAN_POINT('Ctrl Pts',(0.286592207792514,2.24739881667687,12.0469805472902));
#69739=CARTESIAN_POINT('Ctrl Pts',(0.284695363949266,2.25107082497772,12.0472351226996));
#69740=CARTESIAN_POINT('Ctrl Pts',(0.283009448610425,2.25420602763454,12.0474511357969));
#69741=CARTESIAN_POINT('Ctrl Pts',(0.266270952339075,2.28413409169868,12.0495063196684));
#69742=CARTESIAN_POINT('Ctrl Pts',(0.247508855106342,2.30867571226429,12.051150797027));
#69743=CARTESIAN_POINT('Ctrl Pts',(0.214136164988961,2.34137584980251,12.0538068447533));
#69744=CARTESIAN_POINT('Ctrl Pts',(0.201906157376013,2.35169504278487,12.0547368060863));
#69745=CARTESIAN_POINT('Ctrl Pts',(0.188165657816019,2.3616406473426,12.055766159724));
#69746=CARTESIAN_POINT('Ctrl Pts',(0.187366235968143,2.36221372334213,12.0558259891433));
#69747=CARTESIAN_POINT('Ctrl Pts',(0.186088343661225,2.36312096945232,12.0559215407801));
#69748=CARTESIAN_POINT('Ctrl Pts',(0.185611563021663,2.36345751816512,12.0559571718738));
#69749=CARTESIAN_POINT('Ctrl Pts',(0.184703802113902,2.36409459890853,12.0560249762929));
#69750=CARTESIAN_POINT('Ctrl Pts',(0.184272995454772,2.36439537595985,12.056057140131));
#69751=CARTESIAN_POINT('Ctrl Pts',(0.183520233683676,2.36491819947496,12.0561133159111));
#69752=CARTESIAN_POINT('Ctrl Pts',(0.183198605448993,2.36514071649547,12.0561373098611));
#69753=CARTESIAN_POINT('Ctrl Pts',(0.182572876711769,2.36557194194939,12.0561839751006));
#69754=CARTESIAN_POINT('Ctrl Pts',(0.182268821258163,2.36578071498321,12.056206643887));
#69755=CARTESIAN_POINT('Ctrl Pts',(0.181551005495881,2.36627177641139,12.0562601446258));
#69756=CARTESIAN_POINT('Ctrl Pts',(0.181136945047295,2.3665536224557,12.0562909932793));
#69757=CARTESIAN_POINT('Ctrl Pts',(0.179699336113754,2.3675272892533,12.0563980575599));
#69758=CARTESIAN_POINT('Ctrl Pts',(0.178672477586694,2.36821418228663,12.0564744588725));
#69759=CARTESIAN_POINT('Ctrl Pts',(0.165716940455456,2.37677307132526,12.0574375411727));
#69760=CARTESIAN_POINT('Ctrl Pts',(0.153283084964506,2.38384790192533,12.0583539529111));
#69761=CARTESIAN_POINT('Ctrl Pts',(0.119355572243307,2.40027193455651,12.0608360518322));
#69762=CARTESIAN_POINT('Ctrl Pts',(0.0972412806432422,2.40814435526604,
12.0624400964415));
#69763=CARTESIAN_POINT('Ctrl Pts',(0.0654671569879768,2.41569116109062,
12.0646267782147));
#69764=CARTESIAN_POINT('Ctrl Pts',(0.0563724442155307,2.4174413876791,12.0652388487674));
#69765=CARTESIAN_POINT('Ctrl Pts',(0.0436204481428185,2.41932997214429,
12.0660673022455));
#69766=CARTESIAN_POINT('Ctrl Pts',(0.0400176724595867,2.41980144350143,
12.0662980795035));
#69767=CARTESIAN_POINT('Ctrl Pts',(0.0358800790211579,2.42027188033794,
12.0665587726477));
#69768=CARTESIAN_POINT('Ctrl Pts',(0.0353524950995632,2.42033054569548,
12.0665919328572));
#69769=CARTESIAN_POINT('Ctrl Pts',(0.0345550358528794,2.42041722602747,
12.0666419310906));
#69770=CARTESIAN_POINT('Ctrl Pts',(0.0342852694208972,2.42044620381582,
12.0666588231068));
#69771=CARTESIAN_POINT('Ctrl Pts',(0.0337984519812384,2.42049787502278,
12.0666892670523));
#69772=CARTESIAN_POINT('Ctrl Pts',(0.033581415087397,2.4205206885867,12.0667028257419));
#69773=CARTESIAN_POINT('Ctrl Pts',(0.0331461992642003,2.42056598884791,
12.0667299861991));
#69774=CARTESIAN_POINT('Ctrl Pts',(0.0329280215237486,2.42058847317226,
12.0667435877887));
#69775=CARTESIAN_POINT('Ctrl Pts',(0.0323083764105983,2.4206516915179,12.0667821776799));
#69776=CARTESIAN_POINT('Ctrl Pts',(0.0319068534368921,2.42069189445253,
12.066807135948));
#69777=CARTESIAN_POINT('Ctrl Pts',(0.0302112169251173,2.42085845584139,
12.0669123383206));
#69778=CARTESIAN_POINT('Ctrl Pts',(0.0289163972440879,2.42097773819712,
12.0669921892031));
#69779=CARTESIAN_POINT('Ctrl Pts',(-0.00662168824983516,2.4240348099655,
12.0691714140337));
#69780=CARTESIAN_POINT('Ctrl Pts',(-0.0411216162206596,2.42148470754561,
12.070990059537));
#69781=CARTESIAN_POINT('Ctrl Pts',(-0.0894095475321529,2.40999954039297,
12.0738207928766));
#69782=CARTESIAN_POINT('Ctrl Pts',(-0.103975881710794,2.40542216959212,
12.0747115561074));
#69783=CARTESIAN_POINT('Ctrl Pts',(-0.119291937520403,2.39938617814062,
12.0757121926381));
#69784=CARTESIAN_POINT('Ctrl Pts',(-0.120419084779609,2.39893459815941,
12.0757862095546));
#69785=CARTESIAN_POINT('Ctrl Pts',(-0.122042016027532,2.39827371911218,
12.0758933388007));
#69786=CARTESIAN_POINT('Ctrl Pts',(-0.122539879380128,2.39806952736741,
12.0759262783804));
#69787=CARTESIAN_POINT('Ctrl Pts',(-0.123405548589118,2.39771194972716,
12.0759836855929));
#69788=CARTESIAN_POINT('Ctrl Pts',(-0.123773586728971,2.39755912632428,
12.0760081341147));
#69789=CARTESIAN_POINT('Ctrl Pts',(-0.124482517695573,2.39726320844895,
12.0760553091768));
#69790=CARTESIAN_POINT('Ctrl Pts',(-0.124823449804632,2.3971202091516,12.0760780324544));
#69791=CARTESIAN_POINT('Ctrl Pts',(-0.125628853456805,2.39678076273561,
12.0761317992387));
#69792=CARTESIAN_POINT('Ctrl Pts',(-0.126093110420215,2.39658381184877,
12.0761628598533));
#69793=CARTESIAN_POINT('Ctrl Pts',(-0.12771178165399,2.39589263827053,12.0762713940251));
#69794=CARTESIAN_POINT('Ctrl Pts',(-0.128863756720793,2.39539276343199,
12.0763490601389));
#69795=CARTESIAN_POINT('Ctrl Pts',(-0.144299741416769,2.38858717106899,
12.0773955424419));
#69796=CARTESIAN_POINT('Ctrl Pts',(-0.158107807155391,2.38125924039731,
12.0784000258124));
#69797=CARTESIAN_POINT('Ctrl Pts',(-0.181182739410418,2.3667758256734,12.0802018192575));
#69798=CARTESIAN_POINT('Ctrl Pts',(-0.190693839377793,2.36006221610297,
12.0809850223607));
#69799=CARTESIAN_POINT('Ctrl Pts',(-0.208077246289068,2.34632454700014,
12.0824835445723));
#69800=CARTESIAN_POINT('Ctrl Pts',(-0.216009448452653,2.33939893363112,
12.0831972585498));
#69801=CARTESIAN_POINT('Ctrl Pts',(-0.229953559816156,2.32596602119399,
12.0844932478045));
#69802=CARTESIAN_POINT('Ctrl Pts',(-0.236064040377432,2.31957476306567,
12.0850776681776));
#69803=CARTESIAN_POINT('Ctrl Pts',(-0.242437560932519,2.31233430151985,
12.0856987385142));
#69804=CARTESIAN_POINT('Ctrl Pts',(-0.242968376089979,2.31172669836537,
12.0857505550383));
#69805=CARTESIAN_POINT('Ctrl Pts',(-0.245563076176704,2.3087340395674,12.0860042633628));
#69806=CARTESIAN_POINT('Ctrl Pts',(-0.247594244513767,2.30632066202191,
12.0862041894235));
#69807=CARTESIAN_POINT('Ctrl Pts',(-0.249913860846921,2.3034809580087,12.0864336765439));
#69808=CARTESIAN_POINT('Ctrl Pts',(-0.250237032541212,2.30308339584795,
12.0864656759506));
#69809=CARTESIAN_POINT('Ctrl Pts',(-0.250727463214252,2.30247712548755,
12.0865142757597));
#69810=CARTESIAN_POINT('Ctrl Pts',(-0.250895410818259,2.30226897930018,
12.0865309257231));
#69811=CARTESIAN_POINT('Ctrl Pts',(-0.251199785104768,2.30189079006862,
12.0865611130724));
#69812=CARTESIAN_POINT('Ctrl Pts',(-0.251336297862839,2.3017208182827,12.0865746566823));
#69813=CARTESIAN_POINT('Ctrl Pts',(-0.25161122213855,2.3013777982335,12.0866019413403));
#69814=CARTESIAN_POINT('Ctrl Pts',(-0.251749627030635,2.30120474650983,
12.0866156819177));
#69815=CARTESIAN_POINT('Ctrl Pts',(-0.252146557103133,2.30070740236997,
12.0866551023111));
#69816=CARTESIAN_POINT('Ctrl Pts',(-0.252404636135577,2.30038275196958,
12.0866807499687));
#69817=CARTESIAN_POINT('Ctrl Pts',(-0.253527704001543,2.29896437710852,
12.0867924382633));
#69818=CARTESIAN_POINT('Ctrl Pts',(-0.254386232537767,2.29786552230014,
12.0868780231181));
#69819=CARTESIAN_POINT('Ctrl Pts',(-0.271161502514037,2.27610471774014,
12.0885551521896));
#69820=CARTESIAN_POINT('Ctrl Pts',(-0.284521898853985,2.25358779823015,
12.0899825739465));
#69821=CARTESIAN_POINT('Ctrl Pts',(-0.304478988187319,2.2081933879082,12.0927603130377));
#69822=CARTESIAN_POINT('Ctrl Pts',(-0.311553286843005,2.18571795050003,
12.0940973395832));
#69823=CARTESIAN_POINT('Ctrl Pts',(-0.316345671568156,2.16154605335343,
12.0955958390002));
#69824=CARTESIAN_POINT('Ctrl Pts',(-0.316563476686372,2.16041577424569,
12.0956660262563));
#69825=CARTESIAN_POINT('Ctrl Pts',(-0.316872066876738,2.15876687866993,
12.0957685970524));
#69826=CARTESIAN_POINT('Ctrl Pts',(-0.316967645393132,2.15824915934225,
12.0958008278167));
#69827=CARTESIAN_POINT('Ctrl Pts',(-0.317132999465671,2.15734102862904,
12.0958574095478));
#69828=CARTESIAN_POINT('Ctrl Pts',(-0.317203323930711,2.15695071728576,
12.0958817429893));
#69829=CARTESIAN_POINT('Ctrl Pts',(-0.31733836036152,2.1561932350945,12.0959289963291));
#69830=CARTESIAN_POINT('Ctrl Pts',(-0.317403156032775,2.15582607962183,
12.0959519135238));
#69831=CARTESIAN_POINT('Ctrl Pts',(-0.317556157066649,2.1549502435909,12.0960066136525));
#69832=CARTESIAN_POINT('Ctrl Pts',(-0.317643777295143,2.15444146308063,
12.0960384151356));
#69833=CARTESIAN_POINT('Ctrl Pts',(-0.31790451429511,2.15290539394979,12.0961345064152));
#69834=CARTESIAN_POINT('Ctrl Pts',(-0.318073871539974,2.15187748182884,
12.096198915421));
#69835=CARTESIAN_POINT('Ctrl Pts',(-0.319789487367902,2.14114026054711,
12.0968728504719));
#69836=CARTESIAN_POINT('Ctrl Pts',(-0.320895507197951,2.13136681055273,
12.0974962639784));
#69837=CARTESIAN_POINT('Ctrl Pts',(-0.322040275759761,2.11429246827615,
12.0986041887887));
#69838=CARTESIAN_POINT('Ctrl Pts',(-0.322280985094732,2.10701205250904,
12.0990824510732));
#69839=CARTESIAN_POINT('Ctrl Pts',(-0.322247790519718,2.06737328250978,
12.1017144122446));
#69840=CARTESIAN_POINT('Ctrl Pts',(-0.317348336812178,2.03520732101442,
12.1039744415003));
#69841=CARTESIAN_POINT('Ctrl Pts',(-0.307300500071528,2.0028929287017,12.1061144844357));
#69842=CARTESIAN_POINT('Ctrl Pts',(-0.306849793355093,2.00147799657012,
12.106207871317));
#69843=CARTESIAN_POINT('Ctrl Pts',(-0.306257549281033,1.99966222201093,
12.1063272586368));
#69844=CARTESIAN_POINT('Ctrl Pts',(-0.306124986182603,1.99925850396661,
12.1063537740615));
#69845=CARTESIAN_POINT('Ctrl Pts',(-0.305913652020919,1.99861915933155,
12.1063957175632));
#69846=CARTESIAN_POINT('Ctrl Pts',(-0.305835406893998,1.99838336140965,
12.1064111765899));
#69847=CARTESIAN_POINT('Ctrl Pts',(-0.305694695923818,1.99796095240443,
12.1064388512764));
#69848=CARTESIAN_POINT('Ctrl Pts',(-0.30563233228046,1.99777430941643,12.1064510728784));
#69849=CARTESIAN_POINT('Ctrl Pts',(-0.30548528526606,1.99733556196087,12.1064797872487));
#69850=CARTESIAN_POINT('Ctrl Pts',(-0.305400460886729,1.99708350548443,
12.1064962715204));
#69851=CARTESIAN_POINT('Ctrl Pts',(-0.305153594464095,1.99635293228873,
12.106544016697));
#69852=CARTESIAN_POINT('Ctrl Pts',(-0.304990738169087,1.99587468848168,
12.1065752294648));
#69853=CARTESIAN_POINT('Ctrl Pts',(-0.303856036836927,1.99256802661997,
12.1067907625882));
#69854=CARTESIAN_POINT('Ctrl Pts',(-0.302845945008753,1.98975275439017,
12.1069728600996));
#69855=CARTESIAN_POINT('Ctrl Pts',(-0.299565469078418,1.98099509792868,
12.1075361080725));
#69856=CARTESIAN_POINT('Ctrl Pts',(-0.297158148072634,1.97510531176735,
12.1079102432682));
#69857=CARTESIAN_POINT('Ctrl Pts',(-0.288196181561464,1.95490790868862,
12.1091895043447));
#69858=CARTESIAN_POINT('Ctrl Pts',(-0.280769314203126,1.94101128607393,
12.1100638285064));
#69859=CARTESIAN_POINT('Ctrl Pts',(-0.264949236511171,1.91600255692778,
12.1117184880149));
#69860=CARTESIAN_POINT('Ctrl Pts',(-0.256794869216396,1.90478340659086,
12.1124958224374));
#69861=CARTESIAN_POINT('Ctrl Pts',(-0.240440600941432,1.88508730337559,
12.1139737063647));
#69862=CARTESIAN_POINT('Ctrl Pts',(-0.232449213616003,1.87646820261433,
12.1146666713391));
#69863=CARTESIAN_POINT('Ctrl Pts',(-0.223223726701841,1.8675488714921,12.115446673721));
#69864=CARTESIAN_POINT('Ctrl Pts',(-0.222437728606187,1.86679662061965,
12.1155129761535));
#69865=CARTESIAN_POINT('Ctrl Pts',(-0.221264844718941,1.86568541954142,
12.115611695542));
#69866=CARTESIAN_POINT('Ctrl Pts',(-0.220880856389436,1.86532341105381,
12.1156439806317));
#69867=CARTESIAN_POINT('Ctrl Pts',(-0.220221842818759,1.86470517034173,
12.1156993313465));
#69868=CARTESIAN_POINT('Ctrl Pts',(-0.219947254413533,1.86444847231994,
12.1157223769395));
#69869=CARTESIAN_POINT('Ctrl Pts',(-0.219412032312354,1.86394987365464,
12.115767263944));
#69870=CARTESIAN_POINT('Ctrl Pts',(-0.219151445996653,1.86370792271613,
12.1157891031603));
#69871=CARTESIAN_POINT('Ctrl Pts',(-0.218526944253705,1.86313000280699,
12.1158414055441));
#69872=CARTESIAN_POINT('Ctrl Pts',(-0.21816265455396,1.86279444127789,12.1158718859937));
#69873=CARTESIAN_POINT('Ctrl Pts',(-0.217066850152191,1.86178971245898,
12.1159634871017));
#69874=CARTESIAN_POINT('Ctrl Pts',(-0.216333024729269,1.86112308420092,
12.1160247151333));
#69875=CARTESIAN_POINT('Ctrl Pts',(-0.209760656893737,1.85520767838577,
12.1165721010869));
#69876=CARTESIAN_POINT('Ctrl Pts',(-0.203735656965121,1.85017090129081,
12.1170670578835));
#69877=CARTESIAN_POINT('Ctrl Pts',(-0.192306823100366,1.84130517338212,
12.1179949464548));
#69878=CARTESIAN_POINT('Ctrl Pts',(-0.186957188246556,1.83741300892228,
12.1184251378175));
#69879=CARTESIAN_POINT('Ctrl Pts',(-0.167782063506492,1.82434512488735,
12.1199519569906));
#69880=CARTESIAN_POINT('Ctrl Pts',(-0.153372223662145,1.81607517145014,
12.1210743362764));
#69881=CARTESIAN_POINT('Ctrl Pts',(-0.121137962395615,1.80074801912172,
12.1234891764099));
#69882=CARTESIAN_POINT('Ctrl Pts',(-0.103187067520866,1.79409352941735,
12.124777067591));
#69883=CARTESIAN_POINT('Ctrl Pts',(-0.083688634493038,1.78877885807314,
12.1260505124402));
#69884=CARTESIAN_POINT('Ctrl Pts',(-0.0826253754244083,1.78849488905523,
12.1261195638895));
#69885=CARTESIAN_POINT('Ctrl Pts',(-0.0811955632310493,1.78812085905379,
12.1262118778034));
#69886=CARTESIAN_POINT('Ctrl Pts',(-0.0808302922582874,1.78802599162324,
12.126235413582));
#69887=CARTESIAN_POINT('Ctrl Pts',(-0.0802575677386353,1.78787831816809,
12.1262722411104));
#69888=CARTESIAN_POINT('Ctrl Pts',(-0.0800502282704827,1.7878250772349,
12.1262855580805));
#69889=CARTESIAN_POINT('Ctrl Pts',(-0.079651652303674,1.78772315351383,
12.126311127882));
#69890=CARTESIAN_POINT('Ctrl Pts',(-0.0794604255616051,1.78767444014961,
12.1263233823936));
#69891=CARTESIAN_POINT('Ctrl Pts',(-0.0790064856221822,1.78755924674988,
12.126352441263));
#69892=CARTESIAN_POINT('Ctrl Pts',(-0.0787437335160616,1.78749292248796,
12.1263692364708));
#69893=CARTESIAN_POINT('Ctrl Pts',(-0.0779675644234021,1.78729804182714,
12.1264187770687));
#69894=CARTESIAN_POINT('Ctrl Pts',(-0.0774539108930987,1.78717041788851,
12.1264514685728));
#69895=CARTESIAN_POINT('Ctrl Pts',(-0.073454671590297,1.78618720844768,
12.126705289892));
#69896=CARTESIAN_POINT('Ctrl Pts',(-0.069955153749981,1.7853885952402,12.1269231994161));
#69897=CARTESIAN_POINT('Ctrl Pts',(-0.0575787702630422,1.7827809578194,
12.127681471899));
#69898=CARTESIAN_POINT('Ctrl Pts',(-0.0486391019565784,1.78128774523499,
12.1282069254693));
#69899=CARTESIAN_POINT('Ctrl Pts',(-0.0124974444364622,1.77680740547635,
12.1302842609111));
#69900=CARTESIAN_POINT('Ctrl Pts',(0.0149704029345457,1.77691236870578,
12.1317670682871));
#69901=CARTESIAN_POINT('Ctrl Pts',(0.0440525856281309,1.78074392552548,
12.1334674639364));
#69902=CARTESIAN_POINT('Ctrl Pts',(0.0460070073745451,1.7810197083649,12.133582317846));
#69903=CARTESIAN_POINT('Ctrl Pts',(0.0504657912932282,1.78169070521084,
12.1338457928476));
#69904=CARTESIAN_POINT('Ctrl Pts',(0.0529682478138649,1.78209755037014,
12.1339947146648));
#69905=CARTESIAN_POINT('Ctrl Pts',(0.0617980585269762,1.78364023692487,
12.1345242449501));
#69906=CARTESIAN_POINT('Ctrl Pts',(0.0680956286381113,1.78493575843284,
12.1349093614281));
#69907=CARTESIAN_POINT('Ctrl Pts',(0.0753518288853519,1.78665619883699,
12.1353632454283));
#69908=CARTESIAN_POINT('Ctrl Pts',(0.0763525683939736,1.78689854502939,
12.1354260677032));
#69909=CARTESIAN_POINT('Ctrl Pts',(0.0778404102545852,1.78726640864994,
12.1355198090705));
#69910=CARTESIAN_POINT('Ctrl Pts',(0.0783284146839475,1.78738827904912,
12.1355506104555));
#69911=CARTESIAN_POINT('Ctrl Pts',(0.0791974873826132,1.78760747719763,
12.1356055620188));
#69912=CARTESIAN_POINT('Ctrl Pts',(0.0795786673914997,1.78770436121431,
12.135629697816));
#69913=CARTESIAN_POINT('Ctrl Pts',(0.0803811435798505,1.78790989013368,
12.1356805810226));
#69914=CARTESIAN_POINT('Ctrl Pts',(0.0808023987152766,1.7880186908187,12.1357073334303));
#69915=CARTESIAN_POINT('Ctrl Pts',(0.081912840741439,1.78830789283193,12.1357779639882));
#69916=CARTESIAN_POINT('Ctrl Pts',(0.0826016491628338,1.78848972618587,
12.1358218884506));
#69917=CARTESIAN_POINT('Ctrl Pts',(0.0857016748337845,1.7893190835939,12.1360200840034));
#69918=CARTESIAN_POINT('Ctrl Pts',(0.0881058690337412,1.78999231595668,
12.1361751873675));
#69919=CARTESIAN_POINT('Ctrl Pts',(0.105801443053288,1.79516997420092,12.1373273977299));
#69920=CARTESIAN_POINT('Ctrl Pts',(0.120745335951812,1.8007748051267,12.1383608542996));
#69921=CARTESIAN_POINT('Ctrl Pts',(0.163991563556159,1.82076322136371,12.1415293385699));
#69922=CARTESIAN_POINT('Ctrl Pts',(0.190649576433447,1.83823845157279,12.1437409005924));
#69923=CARTESIAN_POINT('Ctrl Pts',(0.215482609035767,1.86035272615333,12.1458449273601));
#69924=CARTESIAN_POINT('Ctrl Pts',(0.216630955468818,1.8613902767711,12.1459422892195));
#69925=CARTESIAN_POINT('Ctrl Pts',(0.218086282725865,1.8627243566944,12.1460657117548));
#69926=CARTESIAN_POINT('Ctrl Pts',(0.21840018471435,1.86301325576943,12.1460923349739));
#69927=CARTESIAN_POINT('Ctrl Pts',(0.21889808397416,1.86347332579699,12.1461345655422));
#69928=CARTESIAN_POINT('Ctrl Pts',(0.219082454892995,1.86364408884864,12.1461502038248));
#69929=CARTESIAN_POINT('Ctrl Pts',(0.219423226082209,1.86396045005131,12.146179108353));
#69930=CARTESIAN_POINT('Ctrl Pts',(0.219579680135567,1.86410598702748,12.1461923790611));
#69931=CARTESIAN_POINT('Ctrl Pts',(0.219929615102729,1.86443215396266,12.1462220615753));
#69932=CARTESIAN_POINT('Ctrl Pts',(0.22012301782706,1.86461286630357,12.1462384668841));
#69933=CARTESIAN_POINT('Ctrl Pts',(0.22052572467431,1.86499007935451,12.1462726275565));
#69934=CARTESIAN_POINT('Ctrl Pts',(0.220734989441227,1.86518662201053,12.1462903796853));
#69935=CARTESIAN_POINT('Ctrl Pts',(0.221277199461615,1.86569723408782,12.1463363785576));
#69936=CARTESIAN_POINT('Ctrl Pts',(0.221609740203629,1.8660117349768,12.1463645925796));
#69937=CARTESIAN_POINT('Ctrl Pts',(0.222585153736869,1.86693817834692,12.1464473621812));
#69938=CARTESIAN_POINT('Ctrl Pts',(0.223226176146524,1.86755207529081,12.1465017718546));
#69939=CARTESIAN_POINT('Ctrl Pts',(0.230125938239207,1.87421473208817,12.1470876933559));
#69940=CARTESIAN_POINT('Ctrl Pts',(0.236140339687896,1.88051263229804,12.1476008962165));
#69941=CARTESIAN_POINT('Ctrl Pts',(0.252639012382195,1.89925343638975,12.1490429328214));
#69942=CARTESIAN_POINT('Ctrl Pts',(0.262446425155853,1.91225657752088,12.1499445656362));
#69943=CARTESIAN_POINT('Ctrl Pts',(0.28433442614348,1.94636479749796,12.1522121255405));
#69944=CARTESIAN_POINT('Ctrl Pts',(0.295088261136304,1.96819517835631,12.1535863466674));
#69945=CARTESIAN_POINT('Ctrl Pts',(0.303771665303652,1.99236184144264,12.1551447107973));
#69946=CARTESIAN_POINT('Ctrl Pts',(0.304243654791469,1.99370326328157,12.1552312974069));
#69947=CARTESIAN_POINT('Ctrl Pts',(0.304879957457614,1.99555063397955,12.1553506751489));
#69948=CARTESIAN_POINT('Ctrl Pts',(0.305051923788697,1.99605394519802,12.1553832127895));
#69949=CARTESIAN_POINT('Ctrl Pts',(0.305343654298555,1.99691474138801,12.15543888473));
#69950=CARTESIAN_POINT('Ctrl Pts',(0.305464038969914,1.99727201618972,12.1554619984802));
#69951=CARTESIAN_POINT('Ctrl Pts',(0.305696615527068,1.99796627505659,12.155506927252));
#69952=CARTESIAN_POINT('Ctrl Pts',(0.305808877867033,1.99830323512187,12.1555287399115));
#69953=CARTESIAN_POINT('Ctrl Pts',(0.306075431373924,1.99910773896031,12.1555808339469));
#69954=CARTESIAN_POINT('Ctrl Pts',(0.306229208255277,1.99957545103168,12.1556111322259));
#69955=CARTESIAN_POINT('Ctrl Pts',(0.306684935265848,2.00097232396216,12.1557016597356));
#69956=CARTESIAN_POINT('Ctrl Pts',(0.306983730562625,2.00190250117017,12.1557619926299));
#69957=CARTESIAN_POINT('Ctrl Pts',(0.309490836658603,2.0098309883645,12.1562767004672));
#69958=CARTESIAN_POINT('Ctrl Pts',(0.311463589293737,2.01690098117099,12.1567387472258));
#69959=CARTESIAN_POINT('Ctrl Pts',(0.315909750651387,2.03523109486856,12.1579459568555));
#69960=CARTESIAN_POINT('Ctrl Pts',(0.318023348799647,2.04656701624795,12.1587016373454));
#69961=CARTESIAN_POINT('Ctrl Pts',(0.323539167175525,2.08852075933428,12.1615225826909));
#69962=CARTESIAN_POINT('Ctrl Pts',(0.32315693868286,2.11946723999282,12.1636662977494));
#69963=CARTESIAN_POINT('Ctrl Pts',(0.31814886681069,2.15142861911134,12.1657135095731));
#69964=CARTESIAN_POINT('Ctrl Pts',(0.317896448046752,2.15296652592275,12.165811559086));
#69965=CARTESIAN_POINT('Ctrl Pts',(0.317560539174908,2.15492415263175,12.1659357318024));
#69966=CARTESIAN_POINT('Ctrl Pts',(0.317487361438907,2.15534558622842,12.1659624257878));
#69967=CARTESIAN_POINT('Ctrl Pts',(0.317369813387169,2.1560146450507,12.1660047434122));
#69968=CARTESIAN_POINT('Ctrl Pts',(0.317325992120164,2.15626236429047,12.1660203981995));
#69969=CARTESIAN_POINT('Ctrl Pts',(0.317244443217679,2.15672022969564,12.1660493083529));
#69970=CARTESIAN_POINT('Ctrl Pts',(0.317206797081795,2.15693038814862,12.1660625682373));
#69971=CARTESIAN_POINT('Ctrl Pts',(0.317122089855381,2.15740057122688,12.1660922125629));
#69972=CARTESIAN_POINT('Ctrl Pts',(0.317074917902033,2.15766057483267,12.1661085905489));
#69973=CARTESIAN_POINT('Ctrl Pts',(0.316975935576021,2.15820235365931,12.1661426875516));
#69974=CARTESIAN_POINT('Ctrl Pts',(0.316924069109392,2.15848411858298,12.1661604033609));
#69975=CARTESIAN_POINT('Ctrl Pts',(0.316788623970022,2.15921445387308,12.166206279191));
#69976=CARTESIAN_POINT('Ctrl Pts',(0.316704467899478,2.15966291849028,12.1662344067328));
#69977=CARTESIAN_POINT('Ctrl Pts',(0.316454514231153,2.16097948116525,12.1663168597775));
#69978=CARTESIAN_POINT('Ctrl Pts',(0.316286096251948,2.16184708610698,12.1663710407114));
#69979=CARTESIAN_POINT('Ctrl Pts',(0.314432769509267,2.17118890361534,12.1669528618822));
#69980=CARTESIAN_POINT('Ctrl Pts',(0.312411125221211,2.17959362252603,12.1674624570753));
#69981=CARTESIAN_POINT('Ctrl Pts',(0.305634879415968,2.20349370862875,12.1688976972309));
#69982=CARTESIAN_POINT('Ctrl Pts',(0.300046657608677,2.21872529631896,12.1697961214094));
#69983=CARTESIAN_POINT('Ctrl Pts',(0.283245103546552,2.25565047156884,12.1720657265194));
#69984=CARTESIAN_POINT('Ctrl Pts',(0.270673308898107,2.27660851819424,12.1734450973064));
#69985=CARTESIAN_POINT('Ctrl Pts',(0.254983928620161,2.29709504293656,12.1750108085516));
#69986=CARTESIAN_POINT('Ctrl Pts',(0.254098472250674,2.29823527965232,12.1750987039041));
#69987=CARTESIAN_POINT('Ctrl Pts',(0.252874219383313,2.29979011832866,12.1752196092392));
#69988=CARTESIAN_POINT('Ctrl Pts',(0.252541997182618,2.30020989452088,12.1752523572321));
#69989=CARTESIAN_POINT('Ctrl Pts',(0.251973441853097,2.30092462037754,12.175308297045));
#69990=CARTESIAN_POINT('Ctrl Pts',(0.251737632190452,2.30121998660751,12.1753314678812));
#69991=CARTESIAN_POINT('Ctrl Pts',(0.251279426017346,2.30179185215891,12.1753764332272));
#69992=CARTESIAN_POINT('Ctrl Pts',(0.251057091246833,2.30206840047481,12.1753982252374));
#69993=CARTESIAN_POINT('Ctrl Pts',(0.250526660210225,2.30272594365249,12.1754501525763));
#69994=CARTESIAN_POINT('Ctrl Pts',(0.250218151575264,2.30310660334889,12.175480304504));
#69995=CARTESIAN_POINT('Ctrl Pts',(0.249299165575879,2.30423524138608,12.1755699741035));
#69996=CARTESIAN_POINT('Ctrl Pts',(0.248686197827588,2.30498117659541,12.1756295925217));
#69997=CARTESIAN_POINT('Ctrl Pts',(0.24362552048113,2.31108352543893,12.1761202596055));
#69998=CARTESIAN_POINT('Ctrl Pts',(0.239008957799691,2.31629691364484,12.1765582023383));
#69999=CARTESIAN_POINT('Ctrl Pts',(0.227115030733097,2.32888242872741,12.1776646337308));
#70000=CARTESIAN_POINT('Ctrl Pts',(0.219644645872505,2.3360605802087,12.1783409527639));
#70001=CARTESIAN_POINT('Ctrl Pts',(0.200531663456048,2.35273206026565,12.1800245063167));
#70002=CARTESIAN_POINT('Ctrl Pts',(0.18854611791864,2.36179525696979,12.1810424146601));
#70003=CARTESIAN_POINT('Ctrl Pts',(0.174158870863387,2.3711725564389,12.1822035062334));
#70004=CARTESIAN_POINT('Ctrl Pts',(0.172332296021505,2.37233701091298,12.1823498359201));
#70005=CARTESIAN_POINT('Ctrl Pts',(0.156946852189241,2.38192856827801,12.1835727606581));
#70006=CARTESIAN_POINT('Ctrl Pts',(0.142788824312264,2.38935708268555,12.1846371156795));
#70007=CARTESIAN_POINT('Ctrl Pts',(0.127308311871691,2.39606516943603,12.1856980667814));
#70008=CARTESIAN_POINT('Ctrl Pts',(0.126478346037844,2.39642067885795,12.1857546444854));
#70009=CARTESIAN_POINT('Ctrl Pts',(0.125358628255423,2.39689474217853,12.1858305551512));
#70010=CARTESIAN_POINT('Ctrl Pts',(0.125070191960333,2.39701636435786,12.1858500722007));
#70011=CARTESIAN_POINT('Ctrl Pts',(0.124583842366009,2.3972206046707,12.1858829176177));
#70012=CARTESIAN_POINT('Ctrl Pts',(0.124386023764666,2.39730344551001,12.1858962595539));
#70013=CARTESIAN_POINT('Ctrl Pts',(0.123990143025759,2.39746876489539,12.1859229243216));
#70014=CARTESIAN_POINT('Ctrl Pts',(0.12379208277191,2.39755124247632,12.1859362469755));
#70015=CARTESIAN_POINT('Ctrl Pts',(0.123341589003261,2.39773831246295,12.1859665094598));
#70016=CARTESIAN_POINT('Ctrl Pts',(0.123089105178579,2.39784278147001,12.1859834416839));
#70017=CARTESIAN_POINT('Ctrl Pts',(0.122560065624196,2.39806089199314,12.1860188610108));
#70018=CARTESIAN_POINT('Ctrl Pts',(0.122283483791231,2.39817447009283,12.1860373442625));
#70019=CARTESIAN_POINT('Ctrl Pts',(0.121556719301025,2.39847173404023,12.1860858239132));
#70020=CARTESIAN_POINT('Ctrl Pts',(0.121106276221756,2.39865478716254,12.1861157825205));
#70021=CARTESIAN_POINT('Ctrl Pts',(0.119761188344413,2.39919786662018,12.186204983752));
#70022=CARTESIAN_POINT('Ctrl Pts',(0.118865330479024,2.39955490129152,12.1862640518854));
#70023=CARTESIAN_POINT('Ctrl Pts',(0.115688372705815,2.40080454801704,12.1864723614415));
#70024=CARTESIAN_POINT('Ctrl Pts',(0.113398650085323,2.40167519395395,12.1866203817086));
#70025=CARTESIAN_POINT('Ctrl Pts',(0.102201278301866,2.40578738418493,12.1873350184067));
#70026=CARTESIAN_POINT('Ctrl Pts',(0.0931627634098174,2.40866123273915,
12.1878836928875));
#70027=CARTESIAN_POINT('Ctrl Pts',(0.0535327939586389,2.41936185417131,
12.1902206434306));
#70028=CARTESIAN_POINT('Ctrl Pts',(0.0220135996442052,2.42306847842293,
12.1919242965977));
#70029=CARTESIAN_POINT('Ctrl Pts',(-0.0105381364554002,2.42210419953507,
12.1938498746952));
#70030=CARTESIAN_POINT('Ctrl Pts',(-0.0115335683588456,2.42207009244559,
12.1939088976496));
#70031=CARTESIAN_POINT('Ctrl Pts',(-0.0178491844456279,2.42182437971641,
12.1942842900059));
#70032=CARTESIAN_POINT('Ctrl Pts',(-0.0231633463181839,2.42148558145952,
12.1946043003191));
#70033=CARTESIAN_POINT('Ctrl Pts',(-0.0293377015159986,2.42093806246608,
12.1949817357561));
#70034=CARTESIAN_POINT('Ctrl Pts',(-0.0302086260850107,2.42085725729072,
12.1950351051084));
#70035=CARTESIAN_POINT('Ctrl Pts',(-0.0315966277756221,2.42072277589623,
12.1951203717778));
#70036=CARTESIAN_POINT('Ctrl Pts',(-0.0321139268470682,2.42067139186843,
12.1951521969492));
#70037=CARTESIAN_POINT('Ctrl Pts',(-0.033026045331891,2.42057856065976,
12.195208395592));
#70038=CARTESIAN_POINT('Ctrl Pts',(-0.0334209176978157,2.42053763504922,
12.1952327525945));
#70039=CARTESIAN_POINT('Ctrl Pts',(-0.0342365638744501,2.42045157576002,
12.1952831217451));
#70040=CARTESIAN_POINT('Ctrl Pts',(-0.034657326230079,2.42040634271012,
12.1953091369793));
#70041=CARTESIAN_POINT('Ctrl Pts',(-0.0357331371261176,2.42028854630009,
12.1953757345369));
#70042=CARTESIAN_POINT('Ctrl Pts',(-0.036388052057458,2.42021480233908,
12.1954163540023));
#70043=CARTESIAN_POINT('Ctrl Pts',(-0.0390517894580874,2.41990658592075,
12.1955818835482));
#70044=CARTESIAN_POINT('Ctrl Pts',(-0.0410585759184614,2.419655218977,12.1957073253495));
#70045=CARTESIAN_POINT('Ctrl Pts',(-0.0738055382937274,2.41523993066607,
12.1977666774738));
#70046=CARTESIAN_POINT('Ctrl Pts',(-0.103782248977166,2.40667864323254,
12.1998542954765));
#70047=CARTESIAN_POINT('Ctrl Pts',(-0.144461119167753,2.38840393394621,
12.202869108715));
#70048=CARTESIAN_POINT('Ctrl Pts',(-0.156493427571204,2.38205622275597,
12.2037827354587));
#70049=CARTESIAN_POINT('Ctrl Pts',(-0.169157401257869,2.37431462748633,
12.2047444982193));
#70050=CARTESIAN_POINT('Ctrl Pts',(-0.170221184020779,2.37365578718893,
12.2048252833724));
#70051=CARTESIAN_POINT('Ctrl Pts',(-0.174383873036224,2.37104401366694,
12.2051413099288));
#70052=CARTESIAN_POINT('Ctrl Pts',(-0.177453378384979,2.36904440868316,
12.2053741392918));
#70053=CARTESIAN_POINT('Ctrl Pts',(-0.180967550912966,2.36666881297011,
12.2056398508253));
#70054=CARTESIAN_POINT('Ctrl Pts',(-0.181445952814739,2.36634353101555,
12.2056760049753));
#70055=CARTESIAN_POINT('Ctrl Pts',(-0.182155425700699,2.36585833722564,
12.2057295911317));
#70056=CARTESIAN_POINT('Ctrl Pts',(-0.182387164269939,2.36569941079272,
12.2057470893593));
#70057=CARTESIAN_POINT('Ctrl Pts',(-0.182794936290268,2.36541897566497,
12.2057778705777));
#70058=CARTESIAN_POINT('Ctrl Pts',(-0.182971056585335,2.365297594843,12.2057911622665));
#70059=CARTESIAN_POINT('Ctrl Pts',(-0.18334378918105,2.36504016253991,12.2058192857141));
#70060=CARTESIAN_POINT('Ctrl Pts',(-0.183540370430215,2.36490406794475,
12.2058341144152));
#70061=CARTESIAN_POINT('Ctrl Pts',(-0.183943112934896,2.36462458293121,
12.20586448715));
#70062=CARTESIAN_POINT('Ctrl Pts',(-0.184149258480139,2.36448117001017,
12.2058800296304));
#70063=CARTESIAN_POINT('Ctrl Pts',(-0.184660221257112,2.36412481248137,
12.2059185447945));
#70064=CARTESIAN_POINT('Ctrl Pts',(-0.184964838935141,2.36391158035218,
12.2059414980038));
#70065=CARTESIAN_POINT('Ctrl Pts',(-0.185813214923136,2.36331552746861,
12.2060054031896));
#70066=CARTESIAN_POINT('Ctrl Pts',(-0.186356162175378,2.36293154752429,
12.2060462777403));
#70067=CARTESIAN_POINT('Ctrl Pts',(-0.188101766720825,2.36168890812007,
12.206177628532));
#70068=CARTESIAN_POINT('Ctrl Pts',(-0.189299728251979,2.36082364223252,
12.2062676741761));
#70069=CARTESIAN_POINT('Ctrl Pts',(-0.194041814136444,2.35734863709071,
12.2066239139265));
#70070=CARTESIAN_POINT('Ctrl Pts',(-0.197538433894537,2.35467453332596,
12.2068861379953));
#70071=CARTESIAN_POINT('Ctrl Pts',(-0.207413829897046,2.34679633427967,
12.2076289068151));
#70072=CARTESIAN_POINT('Ctrl Pts',(-0.213649704531986,2.34141820217246,
12.2081006662662));
#70073=CARTESIAN_POINT('Ctrl Pts',(-0.244124843119446,2.31302814833285,
12.210459137361));
#70074=CARTESIAN_POINT('Ctrl Pts',(-0.264882979066932,2.28658758370106,
12.212269165555));
#70075=CARTESIAN_POINT('Ctrl Pts',(-0.281548317275773,2.25681903024943,
12.2143184235909));
#70076=CARTESIAN_POINT('Ctrl Pts',(-0.281887433592866,2.25620863606117,
12.2143604351478));
#70077=CARTESIAN_POINT('Ctrl Pts',(-0.283461767497315,2.25335308439422,
12.2145569448378));
#70078=CARTESIAN_POINT('Ctrl Pts',(-0.28467213597157,2.25109439613411,12.2147122974484));
#70079=CARTESIAN_POINT('Ctrl Pts',(-0.2862024491468,2.24815498132722,12.2149144507731));
#70080=CARTESIAN_POINT('Ctrl Pts',(-0.28654714894836,2.24748719200055,12.2149603754758));
#70081=CARTESIAN_POINT('Ctrl Pts',(-0.287091700957168,2.24642311241345,
12.2150335536904));
#70082=CARTESIAN_POINT('Ctrl Pts',(-0.287293077144125,2.24602760160073,
12.2150607535405));
#70083=CARTESIAN_POINT('Ctrl Pts',(-0.287652968475392,2.245317134835,12.2151096139321));
#70084=CARTESIAN_POINT('Ctrl Pts',(-0.287811785250694,2.2450023317694,12.2151312638428));
#70085=CARTESIAN_POINT('Ctrl Pts',(-0.288181300273844,2.24426688854295,
12.2151818431708));
#70086=CARTESIAN_POINT('Ctrl Pts',(-0.288391594312289,2.24384604716049,
12.2152107866899));
#70087=CARTESIAN_POINT('Ctrl Pts',(-0.288989378074391,2.24264317964662,
12.2152935169491));
#70088=CARTESIAN_POINT('Ctrl Pts',(-0.289374611348188,2.24186004237497,
12.2153473823499));
#70089=CARTESIAN_POINT('Ctrl Pts',(-0.291809918762221,2.23685813026403,
12.2156914536161));
#70090=CARTESIAN_POINT('Ctrl Pts',(-0.293770775581835,2.23259677288957,
12.2159847406427));
#70091=CARTESIAN_POINT('Ctrl Pts',(-0.299365630372979,2.21970414481153,
12.2168731335076));
#70092=CARTESIAN_POINT('Ctrl Pts',(-0.302716903732548,2.21095634819819,
12.2174774693702));
#70093=CARTESIAN_POINT('Ctrl Pts',(-0.316678617351566,2.16914572635596,
12.2203718361332));
#70094=CARTESIAN_POINT('Ctrl Pts',(-0.322279760427778,2.13466281959473,
12.2228062951007));
#70095=CARTESIAN_POINT('Ctrl Pts',(-0.322274996964664,2.09995576849626,
12.2250196508122));
#70096=CARTESIAN_POINT('',(-0.322191991682866,2.10029560349716,12.3497226077682));
#70097=CARTESIAN_POINT('Ctrl Pts',(-0.32279233570592,2.09993664501779,12.2247226550727));
#70098=CARTESIAN_POINT('Ctrl Pts',(-0.322801489738851,2.09653177634649,
12.2249337817233));
#70099=CARTESIAN_POINT('Ctrl Pts',(-0.321208780390457,1.98631842288104,
12.2317683562149));
#70100=CARTESIAN_POINT('Ctrl Pts',(-0.195976803199286,1.7731848083249,12.2452263785474));
#70101=CARTESIAN_POINT('Ctrl Pts',(0.168706279937227,1.75830822659656,12.2650967220702));
#70102=CARTESIAN_POINT('Ctrl Pts',(0.378624318517414,2.05688732983139,12.284967065593));
#70103=CARTESIAN_POINT('Ctrl Pts',(0.241206089904363,2.39501643868587,12.3048374091158));
#70104=CARTESIAN_POINT('Ctrl Pts',(-0.117485888951984,2.46250812790751,
12.3247077526386));
#70105=CARTESIAN_POINT('Ctrl Pts',(-0.306416606983072,2.26292630316716,
12.3396694855227));
#70106=CARTESIAN_POINT('Ctrl Pts',(-0.322441083855502,2.12808501973466,
12.3480077705659));
#70107=CARTESIAN_POINT('Ctrl Pts',(-0.322191991682866,2.10029560349716,
12.3497226077682));
#70108=CARTESIAN_POINT('',(-0.322274943346505,2.09975100738521,12.5998588212847));
#70109=CARTESIAN_POINT('Ctrl Pts',(-0.322274867496596,2.10029224142693,
12.3496749413664));
#70110=CARTESIAN_POINT('Ctrl Pts',(-0.322296495229194,2.07644184235539,
12.3510102465589));
#70111=CARTESIAN_POINT('Ctrl Pts',(-0.319670682733467,2.05266582285634,
12.3523648898113));
#70112=CARTESIAN_POINT('Ctrl Pts',(-0.314258803938727,2.02856252633657,
12.3538660697406));
#70113=CARTESIAN_POINT('Ctrl Pts',(-0.314067932909001,2.02772799994053,
12.3539181974045));
#70114=CARTESIAN_POINT('Ctrl Pts',(-0.313753399015614,2.0263775736076,12.3540028010071));
#70115=CARTESIAN_POINT('Ctrl Pts',(-0.313631782519355,2.02586119740506,
12.3540352112806));
#70116=CARTESIAN_POINT('Ctrl Pts',(-0.31339445757114,2.02486456479613,12.3540978808206));
#70117=CARTESIAN_POINT('Ctrl Pts',(-0.313278918719662,2.02438426922169,
12.3541281345601));
#70118=CARTESIAN_POINT('Ctrl Pts',(-0.313078357963032,2.0235588872839,12.3541802156155));
#70119=CARTESIAN_POINT('Ctrl Pts',(-0.312993868440541,2.02321367143124,
12.3542020257311));
#70120=CARTESIAN_POINT('Ctrl Pts',(-0.312818728813947,2.02250316014996,
12.3542469709228));
#70121=CARTESIAN_POINT('Ctrl Pts',(-0.312728009509253,2.02213788244577,
12.3542701082055));
#70122=CARTESIAN_POINT('Ctrl Pts',(-0.312508116191336,2.02125907455914,
12.3543258476801));
#70123=CARTESIAN_POINT('Ctrl Pts',(-0.31237831630706,2.02074570345677,12.3543584700538));
#70124=CARTESIAN_POINT('Ctrl Pts',(-0.311899040870473,2.0188695918474,12.3544779137642));
#70125=CARTESIAN_POINT('Ctrl Pts',(-0.311541912255455,2.01750883907694,
12.3545649823896));
#70126=CARTESIAN_POINT('Ctrl Pts',(-0.305170201185175,1.99386263348242,
12.3560857210088));
#70127=CARTESIAN_POINT('Ctrl Pts',(-0.29678873525536,1.97228925654693,12.3576002603711));
#70128=CARTESIAN_POINT('Ctrl Pts',(-0.283828034568538,1.94726187056406,
12.3594984299381));
#70129=CARTESIAN_POINT('Ctrl Pts',(-0.281370520131295,1.94278066712219,
12.3598439200554));
#70130=CARTESIAN_POINT('Ctrl Pts',(-0.276392986878284,1.93419509174689,
12.3605154395705));
#70131=CARTESIAN_POINT('Ctrl Pts',(-0.273885423306676,1.93008494444492,
12.3608413550749));
#70132=CARTESIAN_POINT('Ctrl Pts',(-0.264809010705497,1.91593109284126,
12.3619766725555));
#70133=CARTESIAN_POINT('Ctrl Pts',(-0.257771622368049,1.90619852627263,
12.3627810833841));
#70134=CARTESIAN_POINT('Ctrl Pts',(-0.247020297585665,1.89295479670488,
12.3638885385063));
#70135=CARTESIAN_POINT('Ctrl Pts',(-0.243741184786293,1.88910432548278,
12.3642121384117));
#70136=CARTESIAN_POINT('Ctrl Pts',(-0.240048298739609,1.88496924190876,
12.3645599701792));
#70137=CARTESIAN_POINT('Ctrl Pts',(-0.239723179112611,1.88460684770286,
12.3645904564089));
#70138=CARTESIAN_POINT('Ctrl Pts',(-0.239123607778677,1.88394157530411,
12.3646464246558));
#70139=CARTESIAN_POINT('Ctrl Pts',(-0.23884939938938,1.88363848055883,12.3646719244823));
#70140=CARTESIAN_POINT('Ctrl Pts',(-0.238410022727396,1.88315467119545,
12.3647126284764));
#70141=CARTESIAN_POINT('Ctrl Pts',(-0.238245225001502,1.88297362297137,
12.3647278605627));
#70142=CARTESIAN_POINT('Ctrl Pts',(-0.23793240540446,1.88263074232285,12.3647567079094));
#70143=CARTESIAN_POINT('Ctrl Pts',(-0.237784425874324,1.88246887455684,
12.3647703261192));
#70144=CARTESIAN_POINT('Ctrl Pts',(-0.237445423005381,1.88209881470844,
12.3648014598632));
#70145=CARTESIAN_POINT('Ctrl Pts',(-0.237254291327162,1.88189072301716,
12.364818966974));
#70146=CARTESIAN_POINT('Ctrl Pts',(-0.236665690205331,1.88125158174621,
12.3648727400675));
#70147=CARTESIAN_POINT('Ctrl Pts',(-0.236267315075448,1.88082136224369,
12.3649089373353));
#70148=CARTESIAN_POINT('Ctrl Pts',(-0.233257179511233,1.87758835304452,
12.365180985109));
#70149=CARTESIAN_POINT('Ctrl Pts',(-0.230596664937258,1.87483109947546,
12.3654131867485));
#70150=CARTESIAN_POINT('Ctrl Pts',(-0.227437438966471,1.87167174493164,
12.3656804162024));
#70151=CARTESIAN_POINT('Ctrl Pts',(-0.226986067287601,1.87122302131531,
12.3657183988861));
#70152=CARTESIAN_POINT('Ctrl Pts',(-0.212302644645049,1.8567119760241,12.3669477335148));
#70153=CARTESIAN_POINT('Ctrl Pts',(-0.196791406142918,1.84400232019779,
12.3680578825385));
#70154=CARTESIAN_POINT('Ctrl Pts',(-0.171777998542755,1.82713247909485,
12.3697445288577));
#70155=CARTESIAN_POINT('Ctrl Pts',(-0.163092542719674,1.82185403690482,
12.3703132775227));
#70156=CARTESIAN_POINT('Ctrl Pts',(-0.144502965162274,1.81172700613436,
12.3715180821414));
#70157=CARTESIAN_POINT('Ctrl Pts',(-0.1345705344048,1.80695876819794,12.3721550372872));
#70158=CARTESIAN_POINT('Ctrl Pts',(-0.121148702422358,1.80134183665283,
12.3730193777702));
#70159=CARTESIAN_POINT('Ctrl Pts',(-0.117861014221769,1.80002919060396,
12.3732313416604));
#70160=CARTESIAN_POINT('Ctrl Pts',(-0.112458823734777,1.79797482585322,
12.3735803736879));
#70161=CARTESIAN_POINT('Ctrl Pts',(-0.110356981766597,1.79720051347837,
12.373716352169));
#70162=CARTESIAN_POINT('Ctrl Pts',(-0.107767211893838,1.7962769955414,12.3738841708104));
#70163=CARTESIAN_POINT('Ctrl Pts',(-0.107286741302973,1.79610694227634,
12.3739153170629));
#70164=CARTESIAN_POINT('Ctrl Pts',(-0.1064393399561,1.79580928111394,12.3739702704131));
#70165=CARTESIAN_POINT('Ctrl Pts',(-0.106072577196951,1.79568119527145,
12.3739940616255));
#70166=CARTESIAN_POINT('Ctrl Pts',(-0.105330912053665,1.79542368461445,
12.3740421864207));
#70167=CARTESIAN_POINT('Ctrl Pts',(-0.104956000617464,1.79529428810735,
12.3740665208914));
#70168=CARTESIAN_POINT('Ctrl Pts',(-0.104228228611407,1.79504460823843,
12.374113773317));
#70169=CARTESIAN_POINT('Ctrl Pts',(-0.103875396136379,1.79492424435951,
12.3741366885628));
#70170=CARTESIAN_POINT('Ctrl Pts',(-0.10303355804136,1.79463869276486,12.3741913794026));
#70171=CARTESIAN_POINT('Ctrl Pts',(-0.102544364001847,1.79447406747458,
12.3742231735311));
#70172=CARTESIAN_POINT('Ctrl Pts',(-0.101067068798483,1.79398087063957,
12.3743192280852));
#70173=CARTESIAN_POINT('Ctrl Pts',(-0.100077775815596,1.79365591457149,
12.3743836075941));
#70174=CARTESIAN_POINT('Ctrl Pts',(-0.0897483600836429,1.79031835507489,
12.3750564130522));
#70175=CARTESIAN_POINT('Ctrl Pts',(-0.0802777587900481,1.78772938492326,
12.3756786757457));
#70176=CARTESIAN_POINT('Ctrl Pts',(-0.0645588008478664,1.78419465266251,
12.3767217036889));
#70177=CARTESIAN_POINT('Ctrl Pts',(-0.0583741417256624,1.78299320495288,
12.3771345625626));
#70178=CARTESIAN_POINT('Ctrl Pts',(-0.0436968267518361,1.78058602181512,
12.3781192081937));
#70179=CARTESIAN_POINT('Ctrl Pts',(-0.0351834935626272,1.77953656837286,
12.3786941898648));
#70180=CARTESIAN_POINT('Ctrl Pts',(-0.00171687585879573,1.77676076279026,
12.3809597627853));
#70181=CARTESIAN_POINT('Ctrl Pts',(0.0233628538449163,1.77760126893881,
12.3826756874152));
#70182=CARTESIAN_POINT('Ctrl Pts',(0.0493740514826458,1.78152699786694,
12.3843360141426));
#70183=CARTESIAN_POINT('Ctrl Pts',(0.0506524070603436,1.78172781484886,
12.3844172868297));
#70184=CARTESIAN_POINT('Ctrl Pts',(0.0522134327750501,1.78198268002496,
12.3845161025249));
#70185=CARTESIAN_POINT('Ctrl Pts',(0.0524972608750805,1.78202941021471,
12.3845340520266));
#70186=CARTESIAN_POINT('Ctrl Pts',(0.0530461804847233,1.78212054076278,
12.384568732098));
#70187=CARTESIAN_POINT('Ctrl Pts',(0.0533112796173102,1.78216489285197,
12.3845854653811));
#70188=CARTESIAN_POINT('Ctrl Pts',(0.0537706615633961,1.78224234010725,
12.3846144349692));
#70189=CARTESIAN_POINT('Ctrl Pts',(0.0539649691161984,1.78227528176972,
12.3846266800205));
#70190=CARTESIAN_POINT('Ctrl Pts',(0.0543713299783697,1.78234455712618,
12.3846522708329));
#70191=CARTESIAN_POINT('Ctrl Pts',(0.0545833764672977,1.78238092480922,
12.3846656145847));
#70192=CARTESIAN_POINT('Ctrl Pts',(0.0551725576544382,1.78248258158102,
12.384702663434));
#70193=CARTESIAN_POINT('Ctrl Pts',(0.0555496142809594,1.78254833049041,
12.3847263422769));
#70194=CARTESIAN_POINT('Ctrl Pts',(0.057047607315314,1.7828122923175,12.3848202941495));
#70195=CARTESIAN_POINT('Ctrl Pts',(0.0581676246149263,1.78301577493059,
12.3848902709028));
#70196=CARTESIAN_POINT('Ctrl Pts',(0.0780643120329327,1.78673957529713,
12.3861289703446));
#70197=CARTESIAN_POINT('Ctrl Pts',(0.0964955990191437,1.79191727663207,
12.38720761918));
#70198=CARTESIAN_POINT('Ctrl Pts',(0.126063456666013,1.80314004241898,12.3889789536029));
#70199=CARTESIAN_POINT('Ctrl Pts',(0.137496310380895,1.80825938235688,12.3896746638643));
#70200=CARTESIAN_POINT('Ctrl Pts',(0.160054595676795,1.81998165338232,12.3911126450931));
#70201=CARTESIAN_POINT('Ctrl Pts',(0.17113805222637,1.82661480402884,12.391854469339));
#70202=CARTESIAN_POINT('Ctrl Pts',(0.186493905642391,1.83710533213254,12.3929575776971));
#70203=CARTESIAN_POINT('Ctrl Pts',(0.191108329838723,1.84044040505684,12.3932995378452));
#70204=CARTESIAN_POINT('Ctrl Pts',(0.196360101664941,1.84445210622024,12.3937020958421));
#70205=CARTESIAN_POINT('Ctrl Pts',(0.197086015547253,1.84501153361454,12.3937580422227));
#70206=CARTESIAN_POINT('Ctrl Pts',(0.198118067485639,1.84581392701225,12.3938380213069));
#70207=CARTESIAN_POINT('Ctrl Pts',(0.198426169771662,1.84605436898266,12.3938619538538));
#70208=CARTESIAN_POINT('Ctrl Pts',(0.199047032434409,1.84654070782728,12.3939102945346));
#70209=CARTESIAN_POINT('Ctrl Pts',(0.199359776312855,1.84678662457162,12.393934703434));
#70210=CARTESIAN_POINT('Ctrl Pts',(0.199963042964823,1.84726279558797,12.3939819004964));
#70211=CARTESIAN_POINT('Ctrl Pts',(0.200253625566472,1.84749297338201,12.3940046855803));
#70212=CARTESIAN_POINT('Ctrl Pts',(0.200941592519429,1.84803986378302,12.3940587519778));
#70213=CARTESIAN_POINT('Ctrl Pts',(0.201338625318784,1.84835701520459,12.3940900508597));
#70214=CARTESIAN_POINT('Ctrl Pts',(0.202731267096658,1.84947486886477,12.3942001770699));
#70215=CARTESIAN_POINT('Ctrl Pts',(0.203722853173014,1.850280543392,12.394279204454));
#70216=CARTESIAN_POINT('Ctrl Pts',(0.218151265596728,1.86214691846572,12.3954382437835));
#70217=CARTESIAN_POINT('Ctrl Pts',(0.230673036367228,1.87427044267747,12.3965629071262));
#70218=CARTESIAN_POINT('Ctrl Pts',(0.254494312873291,1.90139590926546,12.3989632867845));
#70219=CARTESIAN_POINT('Ctrl Pts',(0.265588036890956,1.91649558765193,12.4002397349749));
#70220=CARTESIAN_POINT('Ctrl Pts',(0.278943830835475,1.93844380037637,12.4019662753593));
#70221=CARTESIAN_POINT('Ctrl Pts',(0.282383442989657,1.94453403120263,12.4024326126142));
#70222=CARTESIAN_POINT('Ctrl Pts',(0.288520839389249,1.95627782889572,12.4033022267684));
#70223=CARTESIAN_POINT('Ctrl Pts',(0.291257401697145,1.96190772861526,12.4037067976145));
#70224=CARTESIAN_POINT('Ctrl Pts',(0.294400135273472,1.96888298102292,12.4041901062997));
#70225=CARTESIAN_POINT('Ctrl Pts',(0.294963592486101,1.97015550997893,12.4042775618792));
#70226=CARTESIAN_POINT('Ctrl Pts',(0.29567858687149,1.97179894964489,12.4043895504796));
#70227=CARTESIAN_POINT('Ctrl Pts',(0.295837689049186,1.97216652320831,12.4044145365268));
#70228=CARTESIAN_POINT('Ctrl Pts',(0.296092210538458,1.97275756398156,12.4044546131207));
#70229=CARTESIAN_POINT('Ctrl Pts',(0.296188062452622,1.97298084267734,12.4044697301013));
#70230=CARTESIAN_POINT('Ctrl Pts',(0.296370117842785,1.97340625148948,12.4044984884381));
#70231=CARTESIAN_POINT('Ctrl Pts',(0.296456366385389,1.97360835968342,12.4045121324582));
#70232=CARTESIAN_POINT('Ctrl Pts',(0.296652519571478,1.97406931534854,12.4045432082144));
#70233=CARTESIAN_POINT('Ctrl Pts',(0.296762292022528,1.97432821820365,12.4045606317783));
#70234=CARTESIAN_POINT('Ctrl Pts',(0.297103278030211,1.97513538587368,12.4046148579569));
#70235=CARTESIAN_POINT('Ctrl Pts',(0.297333313833047,1.97568415155093,12.4046515890031));
#70236=CARTESIAN_POINT('Ctrl Pts',(0.299109096770105,1.97995352542925,12.4049363269711));
#70237=CARTESIAN_POINT('Ctrl Pts',(0.30058655622867,1.98370239176844,12.4051802931541));
#70238=CARTESIAN_POINT('Ctrl Pts',(0.302292067036046,1.98827975321324,12.4054720260709));
#70239=CARTESIAN_POINT('Ctrl Pts',(0.30258753932006,1.98908251529534,12.4055229621931));
#70240=CARTESIAN_POINT('Ctrl Pts',(0.303494426500509,1.99157701145392,12.4056805650547));
#70241=CARTESIAN_POINT('Ctrl Pts',(0.304094885437384,1.99327272013194,12.4057867389432));
#70242=CARTESIAN_POINT('Ctrl Pts',(0.308161596583003,2.00507020894522,12.4065193421156));
#70243=CARTESIAN_POINT('Ctrl Pts',(0.311138282480242,2.0153345568045,12.4071260918152));
#70244=CARTESIAN_POINT('Ctrl Pts',(0.318426266125922,2.04610691562251,12.4089044964611));
#70245=CARTESIAN_POINT('Ctrl Pts',(0.321254638995248,2.06690641464713,12.4100576977834));
#70246=CARTESIAN_POINT('Ctrl Pts',(0.322466804601989,2.09899128551383,12.4119077788129));
#70247=CARTESIAN_POINT('Ctrl Pts',(0.322308138440749,2.11016271437738,12.4125642965293));
#70248=CARTESIAN_POINT('Ctrl Pts',(0.32143789833822,2.12329930318677,12.4133604680997));
#70249=CARTESIAN_POINT('Ctrl Pts',(0.321287032453841,2.12529471316311,12.413482052272));
#70250=CARTESIAN_POINT('Ctrl Pts',(0.321062111267256,2.12794146935968,12.4136442258299));
#70251=CARTESIAN_POINT('Ctrl Pts',(0.321004635739305,2.12859420964545,12.4136842937553));
#70252=CARTESIAN_POINT('Ctrl Pts',(0.32090657300441,2.12967032044656,12.4137504716847));
#70253=CARTESIAN_POINT('Ctrl Pts',(0.320867137527,2.13009379612676,12.4137765454159));
#70254=CARTESIAN_POINT('Ctrl Pts',(0.320789350985821,2.13091156510658,12.4138269566818));
#70255=CARTESIAN_POINT('Ctrl Pts',(0.320751110932969,2.13130586840005,12.413851290679));
#70256=CARTESIAN_POINT('Ctrl Pts',(0.320661513710283,2.1322123298462,12.4139072950026));
#70257=CARTESIAN_POINT('Ctrl Pts',(0.320609656468812,2.13272443648313,12.4139389810211));
#70258=CARTESIAN_POINT('Ctrl Pts',(0.320445374555601,2.13430889281329,12.414037162039));
#70259=CARTESIAN_POINT('Ctrl Pts',(0.320328795829269,2.13538079588493,12.414103787709));
#70260=CARTESIAN_POINT('Ctrl Pts',(0.319314254390294,2.14429285465081,12.4146594647908));
#70261=CARTESIAN_POINT('Ctrl Pts',(0.318134051496545,2.15209757797293,12.41515738017));
#70262=CARTESIAN_POINT('Ctrl Pts',(0.316083220083332,2.16294849729848,12.415866381315));
#70263=CARTESIAN_POINT('Ctrl Pts',(0.315452306718204,2.16603753828827,12.4160701293096));
#70264=CARTESIAN_POINT('Ctrl Pts',(0.314203529985022,2.17172480232731,12.4164487607958));
#70265=CARTESIAN_POINT('Ctrl Pts',(0.313598489190092,2.174325584479,12.4166232754865));
#70266=CARTESIAN_POINT('Ctrl Pts',(0.306756826776055,2.20216251720299,12.4185055832604));
#70267=CARTESIAN_POINT('Ctrl Pts',(0.297520827934519,2.22656239461783,12.4202941964783));
#70268=CARTESIAN_POINT('Ctrl Pts',(0.280856943656299,2.2583628436451,12.422685579553));
#70269=CARTESIAN_POINT('Ctrl Pts',(0.275853463508499,2.2669260970625,12.4233348786647));
#70270=CARTESIAN_POINT('Ctrl Pts',(0.269687353918092,2.27644245420543,12.4240515384591));
#70271=CARTESIAN_POINT('Ctrl Pts',(0.268904090720959,2.27763388945186,12.4241411693506));
#70272=CARTESIAN_POINT('Ctrl Pts',(0.267883604151819,2.27916395023983,12.4242561125363));
#70273=CARTESIAN_POINT('Ctrl Pts',(0.267653616433828,2.27950734818761,12.4242818990967));
#70274=CARTESIAN_POINT('Ctrl Pts',(0.267285771109931,2.28005430465777,12.4243229531554));
#70275=CARTESIAN_POINT('Ctrl Pts',(0.267148341053489,2.28025814804597,12.4243382494152));
#70276=CARTESIAN_POINT('Ctrl Pts',(0.266887984701972,2.28064337036095,12.4243671482616));
#70277=CARTESIAN_POINT('Ctrl Pts',(0.266765107700984,2.28082477968251,12.4243807539548));
#70278=CARTESIAN_POINT('Ctrl Pts',(0.266484355178158,2.28123835934159,12.4244117648929));
#70279=CARTESIAN_POINT('Ctrl Pts',(0.266326361474266,2.28147044838448,12.4244291619537));
#70280=CARTESIAN_POINT('Ctrl Pts',(0.265842567170203,2.28217913820726,12.4244822688146));
#70281=CARTESIAN_POINT('Ctrl Pts',(0.265515786782654,2.28265507356483,12.4245179123544));
#70282=CARTESIAN_POINT('Ctrl Pts',(0.263121545848907,2.28612213439397,12.4247774291381));
#70283=CARTESIAN_POINT('Ctrl Pts',(0.26100477081154,2.28907910811186,12.4249980201438));
#70284=CARTESIAN_POINT('Ctrl Pts',(0.258387304435151,2.29260776094619,12.4252611832714));
#70285=CARTESIAN_POINT('Ctrl Pts',(0.257934167847442,2.29321416549574,12.4253064055224));
#70286=CARTESIAN_POINT('Ctrl Pts',(0.256841326563231,2.29466595094714,12.4254146798273));
#70287=CARTESIAN_POINT('Ctrl Pts',(0.256199575322627,2.29550978785943,12.4254776200604));
#70288=CARTESIAN_POINT('Ctrl Pts',(0.25193034593304,2.30106626708438,12.4258922248953));
#70289=CARTESIAN_POINT('Ctrl Pts',(0.248176986926294,2.30568114588776,12.4262373323093));
#70290=CARTESIAN_POINT('Ctrl Pts',(0.228096784542626,2.32901982369845,12.4280018623011));
#70291=CARTESIAN_POINT('Ctrl Pts',(0.209772779032673,2.34591404382063,12.4293520112015));
#70292=CARTESIAN_POINT('Ctrl Pts',(0.179163493103398,2.36819981070686,12.4315177064403));
#70293=CARTESIAN_POINT('Ctrl Pts',(0.16818420651584,2.37521756383352,12.4322784507776));
#70294=CARTESIAN_POINT('Ctrl Pts',(0.155533648611095,2.3822633507784,12.4331531151963));
#70295=CARTESIAN_POINT('Ctrl Pts',(0.154250986585684,2.3829663373471,12.4332417693122));
#70296=CARTESIAN_POINT('Ctrl Pts',(0.151986839859772,2.38418727561975,12.4333982311474));
#70297=CARTESIAN_POINT('Ctrl Pts',(0.151007375843766,2.38470893822862,12.433465906373));
#70298=CARTESIAN_POINT('Ctrl Pts',(0.149567892297635,2.3854660895134,12.4335653592122));
#70299=CARTESIAN_POINT('Ctrl Pts',(0.149109962217914,2.38570555092768,12.4335969962124));
#70300=CARTESIAN_POINT('Ctrl Pts',(0.148299451261063,2.38612690502402,12.4336529909271));
#70301=CARTESIAN_POINT('Ctrl Pts',(0.147947105894386,2.38630925042366,12.4336773326093));
#70302=CARTESIAN_POINT('Ctrl Pts',(0.147263214897355,2.38666157743863,12.4337245787531));
#70303=CARTESIAN_POINT('Ctrl Pts',(0.146931709264649,2.38683163572428,12.4337474804682));
#70304=CARTESIAN_POINT('Ctrl Pts',(0.146140986824898,2.38723553602845,12.4338021067701));
#70305=CARTESIAN_POINT('Ctrl Pts',(0.145681503638398,2.38746885166994,12.4338338497912));
#70306=CARTESIAN_POINT('Ctrl Pts',(0.14404301408909,2.38829590406254,12.4339470451726));
#70307=CARTESIAN_POINT('Ctrl Pts',(0.142860933910683,2.38888349154305,12.4340287125573));
#70308=CARTESIAN_POINT('Ctrl Pts',(0.121467994831725,2.39935406141144,12.435506871291));
#70309=CARTESIAN_POINT('Ctrl Pts',(0.100284913931503,2.40709914814937,12.4369799693657));
#70310=CARTESIAN_POINT('Ctrl Pts',(0.0642686757891546,2.41614106449588,
12.4394780027634));
#70311=CARTESIAN_POINT('Ctrl Pts',(0.0498386451562194,2.41873459418383,
12.4404754175767));
#70312=CARTESIAN_POINT('Ctrl Pts',(0.0257344860335249,2.42138945102289,
12.4421009157807));
#70313=CARTESIAN_POINT('Ctrl Pts',(0.0161435218139634,2.42201375994364,
12.4427369405762));
#70314=CARTESIAN_POINT('Ctrl Pts',(0.00282906180194584,2.42228393656158,
12.4435932200996));
#70315=CARTESIAN_POINT('Ctrl Pts',(-0.000881350041491249,2.42229515280251,
12.4438289619597));
#70316=CARTESIAN_POINT('Ctrl Pts',(-0.00512477297303729,2.42223469235417,
12.4440946478046));
#70317=CARTESIAN_POINT('Ctrl Pts',(-0.00565821059082051,2.42222576699766,
12.4441279760569));
#70318=CARTESIAN_POINT('Ctrl Pts',(-0.00646344937015723,2.42221029369236,
12.4441781763964));
#70319=CARTESIAN_POINT('Ctrl Pts',(-0.0067352651080267,2.42220472644626,
12.4441951031318));
#70320=CARTESIAN_POINT('Ctrl Pts',(-0.00722529520009168,2.42219406943175,
12.4442255843107));
#70321=CARTESIAN_POINT('Ctrl Pts',(-0.00744351088698507,2.42218910194841,
12.4442391455913));
#70322=CARTESIAN_POINT('Ctrl Pts',(-0.00788068927321197,2.42217870558857,
12.4442662898499));
#70323=CARTESIAN_POINT('Ctrl Pts',(-0.00809965051149217,2.42217327521137,
12.4442798726902));
#70324=CARTESIAN_POINT('Ctrl Pts',(-0.00872049049333367,2.42215724466279,
12.4443183506055));
#70325=CARTESIAN_POINT('Ctrl Pts',(-0.00912235698171078,2.42214611568422,
12.4443432159289));
#70326=CARTESIAN_POINT('Ctrl Pts',(-0.0108116168559985,2.42209617111383,
12.444447568782));
#70327=CARTESIAN_POINT('Ctrl Pts',(-0.0120988151790634,2.42205038939176,
12.4445266709184));
#70328=CARTESIAN_POINT('Ctrl Pts',(-0.0474013440095872,2.42058282829831,
12.4466856093803));
#70329=CARTESIAN_POINT('Ctrl Pts',(-0.0809846619981988,2.41378766304625,
12.44848943791));
#70330=CARTESIAN_POINT('Ctrl Pts',(-0.127482796154434,2.39639866997596,
12.4513176779318));
#70331=CARTESIAN_POINT('Ctrl Pts',(-0.141662297018011,2.3898891624813,12.4522269437802));
#70332=CARTESIAN_POINT('Ctrl Pts',(-0.1563812978573,2.38179344990619,12.4532479760744));
#70333=CARTESIAN_POINT('Ctrl Pts',(-0.157445022938027,2.38120050394322,
12.4533222100742));
#70334=CARTESIAN_POINT('Ctrl Pts',(-0.158974443454908,2.38033656952996,
12.4534295970661));
#70335=CARTESIAN_POINT('Ctrl Pts',(-0.159442869042054,2.38007041506324,
12.4534625761404));
#70336=CARTESIAN_POINT('Ctrl Pts',(-0.160256707656882,2.37960529711032,
12.4535200296141));
#70337=CARTESIAN_POINT('Ctrl Pts',(-0.160602424012035,2.37940686448318,
12.4535444848135));
#70338=CARTESIAN_POINT('Ctrl Pts',(-0.161267933323786,2.37902323536221,
12.4535916566088));
#70339=CARTESIAN_POINT('Ctrl Pts',(-0.161587777828325,2.37883812910945,
12.4536143699117));
#70340=CARTESIAN_POINT('Ctrl Pts',(-0.16234280753026,2.37839942917438,12.4536680881339));
#70341=CARTESIAN_POINT('Ctrl Pts',(-0.162777717038571,2.37814536514661,
12.4536991100868));
#70342=CARTESIAN_POINT('Ctrl Pts',(-0.164291227818846,2.37725644179421,
12.4538073466104));
#70343=CARTESIAN_POINT('Ctrl Pts',(-0.165366714517951,2.37661632582565,
12.4538847523012));
#70344=CARTESIAN_POINT('Ctrl Pts',(-0.17957028612797,2.36805010313999,12.454913658068));
#70345=CARTESIAN_POINT('Ctrl Pts',(-0.192118073453158,2.35920429458674,
12.4558995252219));
#70346=CARTESIAN_POINT('Ctrl Pts',(-0.210222168886031,2.34440269060158,
12.4574447221865));
#70347=CARTESIAN_POINT('Ctrl Pts',(-0.216263545757921,2.33907342557645,
12.4579835424306));
#70348=CARTESIAN_POINT('Ctrl Pts',(-0.232464329613483,2.32366525524817,
12.4594895489275));
#70349=CARTESIAN_POINT('Ctrl Pts',(-0.24216199824409,2.31312761351484,12.4604635350252));
#70350=CARTESIAN_POINT('Ctrl Pts',(-0.25652972839462,2.29526385244901,12.4619983563205));
#70351=CARTESIAN_POINT('Ctrl Pts',(-0.261660735238953,2.28833256860578,
12.4625687258165));
#70352=CARTESIAN_POINT('Ctrl Pts',(-0.268871331443674,2.2777274604184,12.4633959688205));
#70353=CARTESIAN_POINT('Ctrl Pts',(-0.271166588380249,2.27420542075281,
12.4636636256317));
#70354=CARTESIAN_POINT('Ctrl Pts',(-0.273683143250254,2.27017348271022,
12.4639612377251));
#70355=CARTESIAN_POINT('Ctrl Pts',(-0.273972685238909,2.26970693819236,
12.4639955439658));
#70356=CARTESIAN_POINT('Ctrl Pts',(-0.274405487414254,2.26900556134797,
12.4640469188337));
#70357=CARTESIAN_POINT('Ctrl Pts',(-0.274549639733619,2.26877128491865,
12.464064045998));
#70358=CARTESIAN_POINT('Ctrl Pts',(-0.274796962691122,2.26836818009139,
12.4640934581181));
#70359=CARTESIAN_POINT('Ctrl Pts',(-0.274900277739513,2.26819944135198,
12.464105752655));
#70360=CARTESIAN_POINT('Ctrl Pts',(-0.275114099773814,2.26784949442321,
12.4641312143249));
#70361=CARTESIAN_POINT('Ctrl Pts',(-0.275224582832695,2.26766827272239,
12.464144379862));
#70362=CARTESIAN_POINT('Ctrl Pts',(-0.275493425890947,2.26722631663603,
12.464176439271));
#70363=CARTESIAN_POINT('Ctrl Pts',(-0.275651595241697,2.26696546567262,
12.4641953205501));
#70364=CARTESIAN_POINT('Ctrl Pts',(-0.276248721310408,2.2659775313998,12.4642666778783));
#70365=CARTESIAN_POINT('Ctrl Pts',(-0.276685178694181,2.26524893005533,
12.4643189913582));
#70366=CARTESIAN_POINT('Ctrl Pts',(-0.277326375818384,2.26416888349929,
12.46439609048));
#70367=CARTESIAN_POINT('Ctrl Pts',(-0.277533334290376,2.26381876997368,
12.4644210140226));
#70368=CARTESIAN_POINT('Ctrl Pts',(-0.287911081162565,2.24618653040182,
12.4656727666616));
#70369=CARTESIAN_POINT('Ctrl Pts',(-0.296449117321679,2.22799014405869,
12.4668002106639));
#70370=CARTESIAN_POINT('Ctrl Pts',(-0.308742711882082,2.19382523907905,
12.4688318487209));
#70371=CARTESIAN_POINT('Ctrl Pts',(-0.313080142218739,2.17814110839469,
12.4697349549351));
#70372=CARTESIAN_POINT('Ctrl Pts',(-0.3177109498993,2.15459778634299,12.4711115750337));
#70373=CARTESIAN_POINT('Ctrl Pts',(-0.318931222069622,2.14694708804417,
12.4715618464812));
#70374=CARTESIAN_POINT('Ctrl Pts',(-0.32062113402107,2.13317844708526,12.4723829927829));
#70375=CARTESIAN_POINT('Ctrl Pts',(-0.321193947693445,2.12707695039786,
12.4727506203706));
#70376=CARTESIAN_POINT('Ctrl Pts',(-0.321653404840576,2.1200284811212,12.4731808344414));
#70377=CARTESIAN_POINT('Ctrl Pts',(-0.321710254790034,2.11909358100029,
12.4732380085269));
#70378=CARTESIAN_POINT('Ctrl Pts',(-0.321790298535224,2.11767522689382,
12.4733249211477));
#70379=CARTESIAN_POINT('Ctrl Pts',(-0.321816480367335,2.11719194104954,
12.473354565906));
#70380=CARTESIAN_POINT('Ctrl Pts',(-0.321859929762684,2.11635501745125,
12.4734059560992));
#70381=CARTESIAN_POINT('Ctrl Pts',(-0.321877703470191,2.11600140587012,
12.4734276856215));
#70382=CARTESIAN_POINT('Ctrl Pts',(-0.32191336901801,2.11526771921309,12.4734728053105));
#70383=CARTESIAN_POINT('Ctrl Pts',(-0.321931170534929,2.11488764046356,
12.473496198276));
#70384=CARTESIAN_POINT('Ctrl Pts',(-0.32197788218834,2.11385102465628,12.4735600523362));
#70385=CARTESIAN_POINT('Ctrl Pts',(-0.322005457186875,2.11319443193811,
12.4736005552258));
#70386=CARTESIAN_POINT('Ctrl Pts',(-0.322102306447256,2.11070686971297,
12.4737542258757));
#70387=CARTESIAN_POINT('Ctrl Pts',(-0.322157972662154,2.10887543267303,
12.4738678191804));
#70388=CARTESIAN_POINT('Ctrl Pts',(-0.322250105177716,2.10466101085775,
12.4741302974112));
#70389=CARTESIAN_POINT('Ctrl Pts',(-0.322275760642569,2.102277920165,12.4742795147116));
#70390=CARTESIAN_POINT('Ctrl Pts',(-0.322272588014354,2.09255738744876,
12.4748915139082));
#70391=CARTESIAN_POINT('Ctrl Pts',(-0.322019612823381,2.08522269994397,
12.4753611513157));
#70392=CARTESIAN_POINT('Ctrl Pts',(-0.320506614220196,2.06320773342047,
12.4767947033937));
#70393=CARTESIAN_POINT('Ctrl Pts',(-0.318490374713577,2.04859998618421,
12.4777789870123));
#70394=CARTESIAN_POINT('Ctrl Pts',(-0.310549414108851,2.01053650966025,
12.4804044773017));
#70395=CARTESIAN_POINT('Ctrl Pts',(-0.302973007981674,1.98751789815905,
12.482058470587));
#70396=CARTESIAN_POINT('Ctrl Pts',(-0.29232510396039,1.96431996066291,12.4836708894387));
#70397=CARTESIAN_POINT('Ctrl Pts',(-0.291747697791952,1.96308279702549,
12.4837566894748));
#70398=CARTESIAN_POINT('Ctrl Pts',(-0.290986111659057,1.96147769986851,
12.4838677206556));
#70399=CARTESIAN_POINT('Ctrl Pts',(-0.290809075726345,1.9611064209841,12.4838933835442));
#70400=CARTESIAN_POINT('Ctrl Pts',(-0.290535868898998,1.96053626526242,
12.483932760908));
#70401=CARTESIAN_POINT('Ctrl Pts',(-0.290440204363937,1.9603371484124,12.48394650676));
#70402=CARTESIAN_POINT('Ctrl Pts',(-0.290249699192893,1.95994167181169,
12.4839737959681));
#70403=CARTESIAN_POINT('Ctrl Pts',(-0.290154864605045,1.9597453112263,12.4839873395014));
#70404=CARTESIAN_POINT('Ctrl Pts',(-0.289942778553595,1.95930731033082,
12.4840175363373));
#70405=CARTESIAN_POINT('Ctrl Pts',(-0.28982542458291,1.95906572088977,12.4840341830917));
#70406=CARTESIAN_POINT('Ctrl Pts',(-0.289480976403368,1.95835887617515,
12.4840828627687));
#70407=CARTESIAN_POINT('Ctrl Pts',(-0.289253061579566,1.95789401830503,
12.4841148446016));
#70408=CARTESIAN_POINT('Ctrl Pts',(-0.28757092281332,1.95448392135822,12.4843492324344));
#70409=CARTESIAN_POINT('Ctrl Pts',(-0.286072800309766,1.95156038351303,
12.4845489484519));
#70410=CARTESIAN_POINT('Ctrl Pts',(-0.281023014289846,1.94206641177733,
12.4851951260007));
#70411=CARTESIAN_POINT('Ctrl Pts',(-0.27728743727569,1.93559608590047,12.4856317303332));
#70412=CARTESIAN_POINT('Ctrl Pts',(-0.257917537601212,1.90458749576234,
12.4877340052729));
#70413=CARTESIAN_POINT('Ctrl Pts',(-0.23923518474163,1.88211421053499,12.4893014981543));
#70414=CARTESIAN_POINT('Ctrl Pts',(-0.215548211091604,1.86039743443793,
12.4911629641946));
#70415=CARTESIAN_POINT('Ctrl Pts',(-0.213278095052337,1.85837451681975,
12.4913401231548));
#70416=CARTESIAN_POINT('Ctrl Pts',(-0.209697335171616,1.85527345614903,
12.4916179490723));
#70417=CARTESIAN_POINT('Ctrl Pts',(-0.20840619553882,1.85417300563637,12.49171780746));
#70418=CARTESIAN_POINT('Ctrl Pts',(-0.2022109058474,1.84897658962971,12.4921955868076));
#70419=CARTESIAN_POINT('Ctrl Pts',(-0.197194617326637,1.84501710396387,
12.4925784246921));
#70420=CARTESIAN_POINT('Ctrl Pts',(-0.191238848552106,1.84059696439787,
12.4930298452525));
#70421=CARTESIAN_POINT('Ctrl Pts',(-0.190410565186254,1.83998836814056,
12.4930925563702));
#70422=CARTESIAN_POINT('Ctrl Pts',(-0.18917292871917,1.83908807750596,12.4931861638291));
#70423=CARTESIAN_POINT('Ctrl Pts',(-0.188765776049483,1.83879335757367,
12.4932169429586));
#70424=CARTESIAN_POINT('Ctrl Pts',(-0.188038840907404,1.83826974843146,
12.493271869594));
#70425=CARTESIAN_POINT('Ctrl Pts',(-0.18771932511294,1.83804048928718,12.4932960027674));
#70426=CARTESIAN_POINT('Ctrl Pts',(-0.187045268803415,1.83755870654412,
12.493346895634));
#70427=CARTESIAN_POINT('Ctrl Pts',(-0.186690634956594,1.83730631543739,
12.4933736603556));
#70428=CARTESIAN_POINT('Ctrl Pts',(-0.185753512225661,1.83664222602965,
12.493444358069));
#70429=CARTESIAN_POINT('Ctrl Pts',(-0.185170168366749,1.83623174347784,
12.493488337532));
#70430=CARTESIAN_POINT('Ctrl Pts',(-0.182531788014225,1.83438825576535,
12.4936871257023));
#70431=CARTESIAN_POINT('Ctrl Pts',(-0.180461491239928,1.83297733818936,
12.4938427728026));
#70432=CARTESIAN_POINT('Ctrl Pts',(-0.165018972382683,1.82271480386809,
12.4950015449702));
#70433=CARTESIAN_POINT('Ctrl Pts',(-0.151021187884627,1.81484950793117,
12.4960414711917));
#70434=CARTESIAN_POINT('Ctrl Pts',(-0.107832039307155,1.79465623858834,
12.4992131805885));
#70435=CARTESIAN_POINT('Ctrl Pts',(-0.0773498936013661,1.78554885740935,
12.501420192557));
#70436=CARTESIAN_POINT('Ctrl Pts',(-0.0445359051621924,1.78081352133288,
12.5035172823646));
#70437=CARTESIAN_POINT('Ctrl Pts',(-0.0430400883240043,1.78060838141668,
12.5036122444036));
#70438=CARTESIAN_POINT('Ctrl Pts',(-0.0411187908275544,1.78035863294732,
12.5037333583808));
#70439=CARTESIAN_POINT('Ctrl Pts',(-0.0406946186598991,1.78030435331775,
12.5037600434783));
#70440=CARTESIAN_POINT('Ctrl Pts',(-0.0400232456041312,1.78021979820696,
12.5038021939301));
#70441=CARTESIAN_POINT('Ctrl Pts',(-0.0397761174110584,1.78018896496181,
12.503817690753));
#70442=CARTESIAN_POINT('Ctrl Pts',(-0.0393337274287649,1.78013429035512,
12.5038453985808));
#70443=CARTESIAN_POINT('Ctrl Pts',(-0.0391384809514146,1.78011034147818,
12.5038576156164));
#70444=CARTESIAN_POINT('Ctrl Pts',(-0.0386800185379905,1.78005453263466,
12.5038862754056));
#70445=CARTESIAN_POINT('Ctrl Pts',(-0.0384167855298611,1.78002281876282,
12.5039027097675));
#70446=CARTESIAN_POINT('Ctrl Pts',(-0.0376556488705497,1.77993207107737,
12.5039501694607));
#70447=CARTESIAN_POINT('Ctrl Pts',(-0.0371576433711127,1.77987387397494,
12.5039811475399));
#70448=CARTESIAN_POINT('Ctrl Pts',(-0.0337708295416636,1.77948609936018,
12.5041913284462));
#70449=CARTESIAN_POINT('Ctrl Pts',(-0.0308776933712805,1.77919445312149,
12.504368432567));
#70450=CARTESIAN_POINT('Ctrl Pts',(-0.0217855722827214,1.77840205550125,
12.5049184716612));
#70451=CARTESIAN_POINT('Ctrl Pts',(-0.0155754981362823,1.77804151907465,
12.5052846503156));
#70452=CARTESIAN_POINT('Ctrl Pts',(0.0169904565885914,1.77709544396082,
12.5071730700716));
#70453=CARTESIAN_POINT('Ctrl Pts',(0.0433350658331552,1.7795654342851,12.5085995186846));
#70454=CARTESIAN_POINT('Ctrl Pts',(0.0838704389529214,1.78846183768363,
12.5109665164185));
#70455=CARTESIAN_POINT('Ctrl Pts',(0.0984057645377988,1.79274361160915,
12.5118504846997));
#70456=CARTESIAN_POINT('Ctrl Pts',(0.113755591282043,1.79846658377027,12.5128458100211));
#70457=CARTESIAN_POINT('Ctrl Pts',(0.114923346683233,1.79890971458748,12.512921920378));
#70458=CARTESIAN_POINT('Ctrl Pts',(0.116557941491595,1.79954089271375,12.513029015853));
#70459=CARTESIAN_POINT('Ctrl Pts',(0.117026971643791,1.79972326633693,12.5130598105164));
#70460=CARTESIAN_POINT('Ctrl Pts',(0.117839577180716,1.80004142593268,12.5131132760572));
#70461=CARTESIAN_POINT('Ctrl Pts',(0.118183350748654,1.80017670585726,12.5131359298806));
#70462=CARTESIAN_POINT('Ctrl Pts',(0.118897642899031,1.800459209627,12.5131830734801));
#70463=CARTESIAN_POINT('Ctrl Pts',(0.119268122250218,1.80060653047051,12.513207566495));
#70464=CARTESIAN_POINT('Ctrl Pts',(0.120139016006041,1.80095471376566,12.5132652402384));
#70465=CARTESIAN_POINT('Ctrl Pts',(0.120639200407508,1.80115614494308,12.5132984401233));
#70466=CARTESIAN_POINT('Ctrl Pts',(0.122269762457786,1.80181755559609,12.5134069184662));
#70467=CARTESIAN_POINT('Ctrl Pts',(0.123398022950824,1.802282696458,12.5134823713874));
#70468=CARTESIAN_POINT('Ctrl Pts',(0.139122213805027,1.80886994874965,12.5145394876793));
#70469=CARTESIAN_POINT('Ctrl Pts',(0.153248120056147,1.81605181165994,12.5155578531953));
#70470=CARTESIAN_POINT('Ctrl Pts',(0.195608380800261,1.84167263456954,12.5188332354438));
#70471=CARTESIAN_POINT('Ctrl Pts',(0.221515521738057,1.86351246144548,12.5211921398196));
#70472=CARTESIAN_POINT('Ctrl Pts',(0.244478348197526,1.89001562271875,12.5234078054523));
#70473=CARTESIAN_POINT('Ctrl Pts',(0.245380306598264,1.89107033064131,12.5234950313591));
#70474=CARTESIAN_POINT('Ctrl Pts',(0.246542445553757,1.89244718859257,12.523607638196));
#70475=CARTESIAN_POINT('Ctrl Pts',(0.246808840083189,1.89276403921107,12.5236334659714));
#70476=CARTESIAN_POINT('Ctrl Pts',(0.247216798546808,1.89325116886778,12.5236730409425));
#70477=CARTESIAN_POINT('Ctrl Pts',(0.247358797446731,1.89342108049301,12.5236868200156));
#70478=CARTESIAN_POINT('Ctrl Pts',(0.247640256400486,1.8937585721378,12.5237141397824));
#70479=CARTESIAN_POINT('Ctrl Pts',(0.247779720649175,1.89392614626721,12.5237276807231));
#70480=CARTESIAN_POINT('Ctrl Pts',(0.248086610765351,1.89429565393181,12.5237574860971));
#70481=CARTESIAN_POINT('Ctrl Pts',(0.248253959712069,1.8944976498411,12.5237737448548));
#70482=CARTESIAN_POINT('Ctrl Pts',(0.248736610432294,1.89508167574258,12.5238206539857));
#70483=CARTESIAN_POINT('Ctrl Pts',(0.249051280068474,1.89546423078148,12.5238512582981));
#70484=CARTESIAN_POINT('Ctrl Pts',(0.249760305009823,1.89633027976183,12.5239202694135));
#70485=CARTESIAN_POINT('Ctrl Pts',(0.250154142129212,1.89681419810651,12.5239586394138));
#70486=CARTESIAN_POINT('Ctrl Pts',(0.259951482425394,1.90892411975307,12.5249141670821));
#70487=CARTESIAN_POINT('Ctrl Pts',(0.2685373642032,1.92119122246392,12.5257752203212));
#70488=CARTESIAN_POINT('Ctrl Pts',(0.286771581773594,1.95153702817107,12.5277755318574));
#70489=CARTESIAN_POINT('Ctrl Pts',(0.295610331285801,1.97002409067696,12.5288986484699));
#70490=CARTESIAN_POINT('Ctrl Pts',(0.304681252318336,1.99480570790901,12.5304064257487));
#70491=CARTESIAN_POINT('Ctrl Pts',(0.306569439002036,2.0004425868955,12.5307492604118));
#70492=CARTESIAN_POINT('Ctrl Pts',(0.30907939362852,2.00868596798165,12.5312526852586));
#70493=CARTESIAN_POINT('Ctrl Pts',(0.309826294017514,2.01125321990143,12.5314097484109));
#70494=CARTESIAN_POINT('Ctrl Pts',(0.311026461653203,2.01557837856498,12.531675024557));
#70495=CARTESIAN_POINT('Ctrl Pts',(0.311496981370765,2.01733138188119,12.5317827236437));
#70496=CARTESIAN_POINT('Ctrl Pts',(0.31211902812725,2.01972966297947,12.5319303582435));
#70497=CARTESIAN_POINT('Ctrl Pts',(0.312283415266841,2.02037159260504,12.5319699028552));
#70498=CARTESIAN_POINT('Ctrl Pts',(0.312687317745546,2.02196931467299,12.532068401063));
#70499=CARTESIAN_POINT('Ctrl Pts',(0.312924430494483,2.02292570273174,12.53212742749));
#70500=CARTESIAN_POINT('Ctrl Pts',(0.313311850969022,2.02451961394665,12.5322259178452));
#70501=CARTESIAN_POINT('Ctrl Pts',(0.31346460882439,2.02515653908674,12.5322653055569));
#70502=CARTESIAN_POINT('Ctrl Pts',(0.314230002975547,2.02839130660131,12.5324655089636));
#70503=CARTESIAN_POINT('Ctrl Pts',(0.314812276794845,2.03099616343875,12.5326272641653));
#70504=CARTESIAN_POINT('Ctrl Pts',(0.315517522131463,2.03434607463527,12.5328360708784));
#70505=CARTESIAN_POINT('Ctrl Pts',(0.315670335529582,2.03508479423746,12.5328821654538));
#70506=CARTESIAN_POINT('Ctrl Pts',(0.315909927691416,2.03626386701522,12.5329558171436));
#70507=CARTESIAN_POINT('Ctrl Pts',(0.315998383270926,2.03670387982834,12.5329833206209));
#70508=CARTESIAN_POINT('Ctrl Pts',(0.316162222540064,2.03752778442171,12.5330348534106));
#70509=CARTESIAN_POINT('Ctrl Pts',(0.316237826996519,2.0379116318856,12.5330588756232));
#70510=CARTESIAN_POINT('Ctrl Pts',(0.316404903863116,2.03876811137085,12.5331125073754));
#70511=CARTESIAN_POINT('Ctrl Pts',(0.316496016451906,2.03924081188998,12.5331421283365));
#70512=CARTESIAN_POINT('Ctrl Pts',(0.316758963902753,2.04062164829004,12.5332287183438));
#70513=CARTESIAN_POINT('Ctrl Pts',(0.316927950576724,2.04153031572439,12.5332857780064));
#70514=CARTESIAN_POINT('Ctrl Pts',(0.318130666890541,2.04815593941973,12.5337024215269));
#70515=CARTESIAN_POINT('Ctrl Pts',(0.319013490500741,2.05389887619387,12.5340667758708));
#70516=CARTESIAN_POINT('Ctrl Pts',(0.321417845182028,2.07295719552124,12.5352876100207));
#70517=CARTESIAN_POINT('Ctrl Pts',(0.322264072884849,2.08634220741131,12.5361644796985));
#70518=CARTESIAN_POINT('Ctrl Pts',(0.322295136279694,2.12479830135188,12.5387298954818));
#70519=CARTESIAN_POINT('Ctrl Pts',(0.319392804474774,2.14977253846948,12.5404580627473));
#70520=CARTESIAN_POINT('Ctrl Pts',(0.313351201127258,2.1753235354817,12.5421762985306));
#70521=CARTESIAN_POINT('Ctrl Pts',(0.313069088619063,2.17648762038991,12.5422544499576));
#70522=CARTESIAN_POINT('Ctrl Pts',(0.312551633846643,2.17857196688452,12.5423941189368));
#70523=CARTESIAN_POINT('Ctrl Pts',(0.312318701699164,2.17949280728362,12.542455730133));
#70524=CARTESIAN_POINT('Ctrl Pts',(0.31203619846259,2.18058920354458,12.542528965958));
#70525=CARTESIAN_POINT('Ctrl Pts',(0.311990547680749,2.18076575411089,12.5425407552229));
#70526=CARTESIAN_POINT('Ctrl Pts',(0.310843341486386,2.18518699115654,12.5428358901318));
#70527=CARTESIAN_POINT('Ctrl Pts',(0.309655342330867,2.18940906056954,12.5431155233963));
#70528=CARTESIAN_POINT('Ctrl Pts',(0.308206622817147,2.19418182218119,12.5434280861989));
#70529=CARTESIAN_POINT('Ctrl Pts',(0.308030167174242,2.19475734326281,12.5434657173088));
#70530=CARTESIAN_POINT('Ctrl Pts',(0.307767256629074,2.19560634723978,12.5435211395322));
#70531=CARTESIAN_POINT('Ctrl Pts',(0.307682048803485,2.19588021032071,12.5435390030848));
#70532=CARTESIAN_POINT('Ctrl Pts',(0.307530671114432,2.19636446747756,12.5435705650232));
#70533=CARTESIAN_POINT('Ctrl Pts',(0.307464650791378,2.19657490762741,12.5435842722269));
#70534=CARTESIAN_POINT('Ctrl Pts',(0.30733706513423,2.19698013069461,12.5436106503663));
#70535=CARTESIAN_POINT('Ctrl Pts',(0.307275530863958,2.19717492211315,12.5436233230994));
#70536=CARTESIAN_POINT('Ctrl Pts',(0.307108982190797,2.19770040464002,12.5436574905935));
#70537=CARTESIAN_POINT('Ctrl Pts',(0.307003618512989,2.19803098607946,12.5436789647187));
#70538=CARTESIAN_POINT('Ctrl Pts',(0.306599086866941,2.19929316658817,12.5437608775598));
#70539=CARTESIAN_POINT('Ctrl Pts',(0.306296206770293,2.20022358392657,12.5438210999068));
#70540=CARTESIAN_POINT('Ctrl Pts',(0.305529788650055,2.20254201699488,12.5439707975406));
#70541=CARTESIAN_POINT('Ctrl Pts',(0.305061020356548,2.20392829760395,12.5440599793416));
#70542=CARTESIAN_POINT('Ctrl Pts',(0.301768859464088,2.21344992541272,12.5446705676976));
#70543=CARTESIAN_POINT('Ctrl Pts',(0.298629569041108,2.22147319784076,12.5451752501702));
#70544=CARTESIAN_POINT('Ctrl Pts',(0.288870577986393,2.24374086386009,12.5465732721839));
#70545=CARTESIAN_POINT('Ctrl Pts',(0.281526210377958,2.25764102310232,12.5474435574157));
#70546=CARTESIAN_POINT('Ctrl Pts',(0.267087037482708,2.28071632111964,12.5489670603575));
#70547=CARTESIAN_POINT('Ctrl Pts',(0.260457587520216,2.29014651796972,12.5496150563501));
#70548=CARTESIAN_POINT('Ctrl Pts',(0.251765092716363,2.30120136184224,12.5504240312249));
#70549=CARTESIAN_POINT('Ctrl Pts',(0.250168729705539,2.3031828146735,12.5505710660864));
#70550=CARTESIAN_POINT('Ctrl Pts',(0.247390069170748,2.30654937560533,12.5508246147971));
#70551=CARTESIAN_POINT('Ctrl Pts',(0.246219177550728,2.30794376000644,12.5509307555948));
#70552=CARTESIAN_POINT('Ctrl Pts',(0.243802889230984,2.31077223292768,12.5511484548271));
#70553=CARTESIAN_POINT('Ctrl Pts',(0.242556506964485,2.31220538093181,12.5512600450055));
#70554=CARTESIAN_POINT('Ctrl Pts',(0.23686326700206,2.31863603909449,12.5517668036554));
#70555=CARTESIAN_POINT('Ctrl Pts',(0.232274386633705,2.32350508788052,12.5521672594439));
#70556=CARTESIAN_POINT('Ctrl Pts',(0.226799831228138,2.32896309181853,12.5526377244686));
#70557=CARTESIAN_POINT('Ctrl Pts',(0.226058535982045,2.32969501328918,12.5527012796481));
#70558=CARTESIAN_POINT('Ctrl Pts',(0.224952359549989,2.33077666039275,12.5527959034412));
#70559=CARTESIAN_POINT('Ctrl Pts',(0.224590178257293,2.33112914760994,12.5528268510541));
#70560=CARTESIAN_POINT('Ctrl Pts',(0.223944462107621,2.33175462980146,12.5528819667986));
#70561=CARTESIAN_POINT('Ctrl Pts',(0.223661252829754,2.33202796065028,12.5529061202299));
#70562=CARTESIAN_POINT('Ctrl Pts',(0.223064855592406,2.33260144884772,12.5529569418838));
#70563=CARTESIAN_POINT('Ctrl Pts',(0.222751561103613,2.33290149383268,12.5529836149085));
#70564=CARTESIAN_POINT('Ctrl Pts',(0.221926300380556,2.3336886651656,12.5530538125088));
#70565=CARTESIAN_POINT('Ctrl Pts',(0.221413338110253,2.33417473971725,12.5530973823757));
#70566=CARTESIAN_POINT('Ctrl Pts',(0.219121155227616,2.33633250973028,12.5532917987959));
#70567=CARTESIAN_POINT('Ctrl Pts',(0.217324609313445,2.3379856077224,12.5534434391629));
#70568=CARTESIAN_POINT('Ctrl Pts',(0.204100285823825,2.34987939736561,12.5545545957836));
#70569=CARTESIAN_POINT('Ctrl Pts',(0.191974515974857,2.35931120804736,12.5555477092274));
#70570=CARTESIAN_POINT('Ctrl Pts',(0.161174796688992,2.3799205930671,12.5580077423645));
#70571=CARTESIAN_POINT('Ctrl Pts',(0.141951725903037,2.39014214856864,12.5594961841716));
#70572=CARTESIAN_POINT('Ctrl Pts',(0.118107681086719,2.39988009654711,12.561216351124));
#70573=CARTESIAN_POINT('Ctrl Pts',(0.114339119282427,2.4013371277777,12.561484536216));
#70574=CARTESIAN_POINT('Ctrl Pts',(0.109677219936091,2.40303949350571,12.5618110395627));
#70575=CARTESIAN_POINT('Ctrl Pts',(0.108809035160431,2.40335230524324,12.5618716223891));
#70576=CARTESIAN_POINT('Ctrl Pts',(0.107030891361815,2.40398436443888,12.5619952343106));
#70577=CARTESIAN_POINT('Ctrl Pts',(0.106120817352215,2.40430326599029,12.5620582503552));
#70578=CARTESIAN_POINT('Ctrl Pts',(0.099670602573884,2.40653104801812,12.5625030516906));
#70579=CARTESIAN_POINT('Ctrl Pts',(0.0940802971422607,2.40829275190804,
12.5628790374363));
#70580=CARTESIAN_POINT('Ctrl Pts',(0.0878102499072631,2.41008220017839,
12.5632878892984));
#70581=CARTESIAN_POINT('Ctrl Pts',(0.0871752983943934,2.41026130636021,
12.5633291473241));
#70582=CARTESIAN_POINT('Ctrl Pts',(0.0862826463464921,2.41051014770598,
12.5633869418814));
#70583=CARTESIAN_POINT('Ctrl Pts',(0.0860254078311277,2.41058151280734,
12.5634035724611));
#70584=CARTESIAN_POINT('Ctrl Pts',(0.0855535890755672,2.41071177727027,
12.5634340308768));
#70585=CARTESIAN_POINT('Ctrl Pts',(0.0853390360428728,2.41077077415099,
12.5634478644217));
#70586=CARTESIAN_POINT('Ctrl Pts',(0.0849272008447671,2.41088356018715,
12.5634743851206));
#70587=CARTESIAN_POINT('Ctrl Pts',(0.0847299287289757,2.41093738375452,
12.5634870743019));
#70588=CARTESIAN_POINT('Ctrl Pts',(0.0842249094404933,2.41107465651565,
12.5635195221701));
#70589=CARTESIAN_POINT('Ctrl Pts',(0.0839170884816694,2.4111578370529,12.5635392651269));
#70590=CARTESIAN_POINT('Ctrl Pts',(0.082851319705993,2.41144413654314,12.5636075025057));
#70591=CARTESIAN_POINT('Ctrl Pts',(0.0820927461135195,2.41164494610045,
12.5636558636874));
#70592=CARTESIAN_POINT('Ctrl Pts',(0.0802591323779252,2.41212318070828,
12.5637722776558));
#70593=CARTESIAN_POINT('Ctrl Pts',(0.0791833689253165,2.41239782718925,
12.5638401757661));
#70594=CARTESIAN_POINT('Ctrl Pts',(0.0752251546961129,2.41338661435927,
12.5640886045771));
#70595=CARTESIAN_POINT('Ctrl Pts',(0.0723341960332176,2.41406648886256,
12.5642673303035));
#70596=CARTESIAN_POINT('Ctrl Pts',(0.0621853187662264,2.41630565123588,
12.5648865874848));
#70597=CARTESIAN_POINT('Ctrl Pts',(0.054882883921114,2.41765415663696,12.5653176435627));
#70598=CARTESIAN_POINT('Ctrl Pts',(0.0374783709972437,2.42024995540952,
12.566324399971));
#70599=CARTESIAN_POINT('Ctrl Pts',(0.0273510080992763,2.42127340508745,
12.5668940777291));
#70600=CARTESIAN_POINT('Ctrl Pts',(-0.00550923410627159,2.42302884441702,
12.5687339862276));
#70601=CARTESIAN_POINT('Ctrl Pts',(-0.0282723807757971,2.42183618493003,
12.5700004848898));
#70602=CARTESIAN_POINT('Ctrl Pts',(-0.0511748427832104,2.41818630307005,
12.5713723674859));
#70603=CARTESIAN_POINT('Ctrl Pts',(-0.0516297786196632,2.4181128006728,
12.5713996559998));
#70604=CARTESIAN_POINT('Ctrl Pts',(-0.0577337106364597,2.41711317090707,
12.5717662983612));
#70605=CARTESIAN_POINT('Ctrl Pts',(-0.0633569213734242,2.41603771730515,
12.5721099455375));
#70606=CARTESIAN_POINT('Ctrl Pts',(-0.0699073248494511,2.41460309198936,
12.5725181873107));
#70607=CARTESIAN_POINT('Ctrl Pts',(-0.0708654195474081,2.4143886636566,
12.572578098328));
#70608=CARTESIAN_POINT('Ctrl Pts',(-0.0723100178329812,2.41405841340361,
12.5726687376621));
#70609=CARTESIAN_POINT('Ctrl Pts',(-0.072797262189937,2.41394583023476,
12.5726993618859));
#70610=CARTESIAN_POINT('Ctrl Pts',(-0.0736669036313325,2.41374275664988,
12.5727541154711));
#70611=CARTESIAN_POINT('Ctrl Pts',(-0.0740494017864178,2.41365269986691,
12.5727782308377));
#70612=CARTESIAN_POINT('Ctrl Pts',(-0.0748566167999468,2.4134610872894,
12.5728291931499));
#70613=CARTESIAN_POINT('Ctrl Pts',(-0.0752812935553688,2.41335936743781,
12.5728560453375));
#70614=CARTESIAN_POINT('Ctrl Pts',(-0.076405224164876,2.41308774356345,
12.5729272200487));
#70615=CARTESIAN_POINT('Ctrl Pts',(-0.0771041150161828,2.41291636084341,
12.57297159018));
#70616=CARTESIAN_POINT('Ctrl Pts',(-0.0802942833983428,2.41212272801736,
12.5731746385882));
#70617=CARTESIAN_POINT('Ctrl Pts',(-0.0827785871249266,2.41147307137411,
12.5733341999556));
#70618=CARTESIAN_POINT('Ctrl Pts',(-0.0935514061977446,2.40851794626102,
12.5740325704462));
#70619=CARTESIAN_POINT('Ctrl Pts',(-0.10175284566134,2.40591097504596,12.5745810923826));
#70620=CARTESIAN_POINT('Ctrl Pts',(-0.122889517641475,2.39824826011225,
12.5760401993752));
#70621=CARTESIAN_POINT('Ctrl Pts',(-0.135618859755706,2.39267954081438,
12.5769654559846));
#70622=CARTESIAN_POINT('Ctrl Pts',(-0.158782211372128,2.38070998396296,
12.578723633248));
#70623=CARTESIAN_POINT('Ctrl Pts',(-0.169289414434756,2.37450133157515,
12.5795525465214));
#70624=CARTESIAN_POINT('Ctrl Pts',(-0.19087785500478,2.3600328555652,12.5812981886102));
#70625=CARTESIAN_POINT('Ctrl Pts',(-0.201832975126465,2.35162470648952,
12.5822104505904));
#70626=CARTESIAN_POINT('Ctrl Pts',(-0.21281207685205,2.34201822559049,12.5831267402155));
#70627=CARTESIAN_POINT('Ctrl Pts',(-0.21340558480918,2.34149504751771,12.5831762779815));
#70628=CARTESIAN_POINT('Ctrl Pts',(-0.214218750776272,2.34077290184463,
12.5832441492252));
#70629=CARTESIAN_POINT('Ctrl Pts',(-0.214440063643184,2.34057581456429,
12.5832626211453));
#70630=CARTESIAN_POINT('Ctrl Pts',(-0.214817632419047,2.34023864066017,
12.5832941344178));
#70631=CARTESIAN_POINT('Ctrl Pts',(-0.214974023376015,2.34009870665723,
12.5833071872103));
#70632=CARTESIAN_POINT('Ctrl Pts',(-0.215278260317774,2.33982594888752,
12.5833325790823));
#70633=CARTESIAN_POINT('Ctrl Pts',(-0.215426119663416,2.33969314152092,
12.5833449192772));
#70634=CARTESIAN_POINT('Ctrl Pts',(-0.215732283546537,2.33941763277691,
12.5833704710243));
#70635=CARTESIAN_POINT('Ctrl Pts',(-0.215890569674052,2.33927491087689,
12.5833836810221));
#70636=CARTESIAN_POINT('Ctrl Pts',(-0.216252264258994,2.33894813052187,
12.5834138666154));
#70637=CARTESIAN_POINT('Ctrl Pts',(-0.216455579871819,2.3387639688494,12.5834308344189));
#70638=CARTESIAN_POINT('Ctrl Pts',(-0.217413090824135,2.33789443479493,
12.5835107448448));
#70639=CARTESIAN_POINT('Ctrl Pts',(-0.218164278656408,2.33720573718186,
12.5835734388705));
#70640=CARTESIAN_POINT('Ctrl Pts',(-0.226158458695229,2.32980648217156,
12.5842408226513));
#70641=CARTESIAN_POINT('Ctrl Pts',(-0.23309348577565,2.32276924779686,12.5848215108042));
#70642=CARTESIAN_POINT('Ctrl Pts',(-0.244154189606144,2.31046236658406,
12.5857735413746));
#70643=CARTESIAN_POINT('Ctrl Pts',(-0.248458356167264,2.30536340435532,
12.5861514178989));
#70644=CARTESIAN_POINT('Ctrl Pts',(-0.268042511844972,2.28064509320284,
12.5879256410042));
#70645=CARTESIAN_POINT('Ctrl Pts',(-0.281175425585426,2.25943577612085,
12.5892903841016));
#70646=CARTESIAN_POINT('Ctrl Pts',(-0.292647276310875,2.23499374692047,
12.5908691814638));
#70647=CARTESIAN_POINT('Ctrl Pts',(-0.293535738939955,2.2330507787122,12.5909946621733));
#70648=CARTESIAN_POINT('Ctrl Pts',(-0.297108989117396,2.22502645504214,
12.5915130422179));
#70649=CARTESIAN_POINT('Ctrl Pts',(-0.299624472669125,2.21887191249012,
12.5919110373481));
#70650=CARTESIAN_POINT('Ctrl Pts',(-0.302311188028485,2.21167006079562,
12.5923788427164));
#70651=CARTESIAN_POINT('Ctrl Pts',(-0.302669919903463,2.21069406682922,
12.5924422820164));
#70652=CARTESIAN_POINT('Ctrl Pts',(-0.303195848223308,2.2092415135678,12.5925367663454));
#70653=CARTESIAN_POINT('Ctrl Pts',(-0.303366660452299,2.20876626309599,
12.5925676908974));
#70654=CARTESIAN_POINT('Ctrl Pts',(-0.303668594193689,2.20791994906532,
12.5926227807048));
#70655=CARTESIAN_POINT('Ctrl Pts',(-0.303800154712069,2.20754904230431,
12.5926469313103));
#70656=CARTESIAN_POINT('Ctrl Pts',(-0.304075368333923,2.20676860190148,
12.5926977624537));
#70657=CARTESIAN_POINT('Ctrl Pts',(-0.304218874131501,2.20635901747682,
12.5927244478244));
#70658=CARTESIAN_POINT('Ctrl Pts',(-0.304594169369989,2.205280901745,12.5927947127654));
#70659=CARTESIAN_POINT('Ctrl Pts',(-0.304824584268628,2.20461189750278,
12.5928383377853));
#70660=CARTESIAN_POINT('Ctrl Pts',(-0.305842942400099,2.20162318686394,
12.5930333373239));
#70661=CARTESIAN_POINT('Ctrl Pts',(-0.306606605860521,2.19929534850143,
12.5931855115272));
#70662=CARTESIAN_POINT('Ctrl Pts',(-0.31198753761293,2.18223871864703,12.5943029182228));
#70663=CARTESIAN_POINT('Ctrl Pts',(-0.315567205317863,2.16720598797477,
12.5953021588895));
#70664=CARTESIAN_POINT('Ctrl Pts',(-0.320877649168001,2.13471020012158,
12.5974885280355));
#70665=CARTESIAN_POINT('Ctrl Pts',(-0.322288399277859,2.11724389580947,
12.5986797078545));
#70666=CARTESIAN_POINT('Ctrl Pts',(-0.322274904093275,2.09975137041567,
12.5998588653417));
#70667=CARTESIAN_POINT('',(-0.322274978515416,2.10011767704999,12.8494474689269));
#70668=CARTESIAN_POINT('Ctrl Pts',(-0.322274903816576,2.09975101201496,
12.5998588895012));
#70669=CARTESIAN_POINT('Ctrl Pts',(-0.322263089948684,2.08445985996148,
12.6008896539382));
#70670=CARTESIAN_POINT('Ctrl Pts',(-0.321162988197009,2.06918639405889,
12.6019079146836));
#70671=CARTESIAN_POINT('Ctrl Pts',(-0.318876035729298,2.05331166160658,
12.6029184379496));
#70672=CARTESIAN_POINT('Ctrl Pts',(-0.318767604272797,2.05257699296849,
12.6029650937256));
#70673=CARTESIAN_POINT('Ctrl Pts',(-0.318596508128715,2.05144485063174,
12.6030368143299));
#70674=CARTESIAN_POINT('Ctrl Pts',(-0.318535637745597,2.05104711436359,
12.6030619769726));
#70675=CARTESIAN_POINT('Ctrl Pts',(-0.318433613039424,2.05038871754176,
12.6031035731591));
#70676=CARTESIAN_POINT('Ctrl Pts',(-0.318392883383902,2.0501279931007,12.6031200303807));
#70677=CARTESIAN_POINT('Ctrl Pts',(-0.31831918235261,2.04965997787716,12.6031495450491));
#70678=CARTESIAN_POINT('Ctrl Pts',(-0.318286328676651,2.04945266911989,
12.6031626091511));
#70679=CARTESIAN_POINT('Ctrl Pts',(-0.31822222128866,2.0490506881614,12.6031879223878));
#70680=CARTESIAN_POINT('Ctrl Pts',(-0.318190991489702,2.04885601272614,
12.6032001728416));
#70681=CARTESIAN_POINT('Ctrl Pts',(-0.318125370277947,2.04844934010768,
12.6032257459455));
#70682=CARTESIAN_POINT('Ctrl Pts',(-0.318090945709314,2.04823734929271,
12.6032390666384));
#70683=CARTESIAN_POINT('Ctrl Pts',(-0.318005651099943,2.04771539270985,
12.6032718399029));
#70684=CARTESIAN_POINT('Ctrl Pts',(-0.317954539621869,2.04740546580883,
12.6032912787028));
#70685=CARTESIAN_POINT('Ctrl Pts',(-0.317753532353024,2.04619761118911,
12.6033669548326));
#70686=CARTESIAN_POINT('Ctrl Pts',(-0.31760028344457,2.04530023430135,12.6034230034244));
#70687=CARTESIAN_POINT('Ctrl Pts',(-0.314820562302665,2.02942866395548,
12.6044114052215));
#70688=CARTESIAN_POINT('Ctrl Pts',(-0.311141145399845,2.01465585671774,
12.60528587343));
#70689=CARTESIAN_POINT('Ctrl Pts',(-0.305523008500156,1.99740625450415,
12.6063101881615));
#70690=CARTESIAN_POINT('Ctrl Pts',(-0.304576250783404,1.99462878409233,
12.6064752060964));
#70691=CARTESIAN_POINT('Ctrl Pts',(-0.302739288953132,1.98947148721287,
12.6067823777893));
#70692=CARTESIAN_POINT('Ctrl Pts',(-0.301858621322224,1.98708852108661,
12.6069246157394));
#70693=CARTESIAN_POINT('Ctrl Pts',(-0.299197908214657,1.98014269435755,
12.6073406961287));
#70694=CARTESIAN_POINT('Ctrl Pts',(-0.297341922818261,1.975609715328,12.6076141433382));
#70695=CARTESIAN_POINT('Ctrl Pts',(-0.29090313529031,1.96085240272916,12.6085150770348));
#70696=CARTESIAN_POINT('Ctrl Pts',(-0.285890698464738,1.95082500917218,
12.609144758323));
#70697=CARTESIAN_POINT('Ctrl Pts',(-0.274407483324548,1.93056640978541,
12.6104815452582));
#70698=CARTESIAN_POINT('Ctrl Pts',(-0.267862452458586,1.92039803803896,
12.6111898610645));
#70699=CARTESIAN_POINT('Ctrl Pts',(-0.259522059347485,1.90891380859753,
12.6120476855147));
#70700=CARTESIAN_POINT('Ctrl Pts',(-0.258264861637497,1.90721801757539,
12.6121759016919));
#70701=CARTESIAN_POINT('Ctrl Pts',(-0.256586948684576,1.90500061018871,
12.6123456576193));
#70702=CARTESIAN_POINT('Ctrl Pts',(-0.256181117958024,1.90446775444153,
12.6123866126842));
#70703=CARTESIAN_POINT('Ctrl Pts',(-0.255514725921791,1.90359841759433,
12.6124536963514));
#70704=CARTESIAN_POINT('Ctrl Pts',(-0.255255152647321,1.90326117877099,
12.6124797859045));
#70705=CARTESIAN_POINT('Ctrl Pts',(-0.25475271826226,1.90261108180813,12.6125302070032));
#70706=CARTESIAN_POINT('Ctrl Pts',(-0.254509946780996,1.90229815510655,
12.612554534968));
#70707=CARTESIAN_POINT('Ctrl Pts',(-0.253950709838055,1.90158004909039,
12.6126104958646));
#70708=CARTESIAN_POINT('Ctrl Pts',(-0.253633851026828,1.901175178726,12.612642144409));
#70709=CARTESIAN_POINT('Ctrl Pts',(-0.252787314251255,1.90009882233431,
12.6127265443052));
#70710=CARTESIAN_POINT('Ctrl Pts',(-0.252255932499933,1.89942868705994,
12.6127793636404));
#70711=CARTESIAN_POINT('Ctrl Pts',(-0.248622405225213,1.89488365894975,
12.6131394679851));
#70712=CARTESIAN_POINT('Ctrl Pts',(-0.245433909520306,1.89107894942784,
12.6134502206167));
#70713=CARTESIAN_POINT('Ctrl Pts',(-0.240900564676967,1.88591653340762,
12.6138852966044));
#70714=CARTESIAN_POINT('Ctrl Pts',(-0.239629494437767,1.88449473816552,
12.6140065816338));
#70715=CARTESIAN_POINT('Ctrl Pts',(-0.237930234181469,1.88262759910436,
12.614167810379));
#70716=CARTESIAN_POINT('Ctrl Pts',(-0.237513257609106,1.88217206455459,
12.6142073021062));
#70717=CARTESIAN_POINT('Ctrl Pts',(-0.220067104520433,1.86322231050974,
12.6158566430798));
#70718=CARTESIAN_POINT('Ctrl Pts',(-0.200935907445734,1.84678554624629,
12.6175575509816));
#70719=CARTESIAN_POINT('Ctrl Pts',(-0.170915124594642,1.82655583962047,
12.6200045802552));
#70720=CARTESIAN_POINT('Ctrl Pts',(-0.161422956593141,1.82084708936651,
12.6207492092464));
#70721=CARTESIAN_POINT('Ctrl Pts',(-0.147246866025745,1.81328673149349,
12.6218033245117));
#70722=CARTESIAN_POINT('Ctrl Pts',(-0.142784051359772,1.81103830947749,
12.6221272213385));
#70723=CARTESIAN_POINT('Ctrl Pts',(-0.136806920071566,1.8081992673277,12.6225489193075));
#70724=CARTESIAN_POINT('Ctrl Pts',(-0.135338081818067,1.80751512034525,
12.6226515976927));
#70725=CARTESIAN_POINT('Ctrl Pts',(-0.13290073873828,1.80640216133249,12.6228203363655));
#70726=CARTESIAN_POINT('Ctrl Pts',(-0.131935187071276,1.80596700233786,
12.6228867591986));
#70727=CARTESIAN_POINT('Ctrl Pts',(-0.130720128499522,1.80542658483338,
12.6229698002301));
#70728=CARTESIAN_POINT('Ctrl Pts',(-0.130472625436737,1.80531687708526,
12.6229866870364));
#70729=CARTESIAN_POINT('Ctrl Pts',(-0.13003108604427,1.80512182647746,12.6230167617716));
#70730=CARTESIAN_POINT('Ctrl Pts',(-0.129837103610137,1.80503636311472,
12.6230299570727));
#70731=CARTESIAN_POINT('Ctrl Pts',(-0.129461631291973,1.80487138242886,
12.6230554638541));
#70732=CARTESIAN_POINT('Ctrl Pts',(-0.129280152267775,1.80479184103976,
12.6230677768057));
#70733=CARTESIAN_POINT('Ctrl Pts',(-0.12890491241708,1.80462778758897,12.6230932041341));
#70734=CARTESIAN_POINT('Ctrl Pts',(-0.128711142320766,1.8045432990217,12.623106317043));
#70735=CARTESIAN_POINT('Ctrl Pts',(-0.128240383177364,1.80433858736127,
12.6231381323252));
#70736=CARTESIAN_POINT('Ctrl Pts',(-0.127963307382638,1.8042185625053,12.6231568225022));
#70737=CARTESIAN_POINT('Ctrl Pts',(-0.126924893911851,1.80377047042737,
12.6232267377013));
#70738=CARTESIAN_POINT('Ctrl Pts',(-0.12616245143274,1.803444948164,12.623277808433));
#70739=CARTESIAN_POINT('Ctrl Pts',(-0.112483570691222,1.79766709770227,
12.624189493848));
#70740=CARTESIAN_POINT('Ctrl Pts',(-0.0992242532669101,1.79305962175152,
12.6250006339302));
#70741=CARTESIAN_POINT('Ctrl Pts',(-0.0691312990108737,1.78475780571472,
12.6267698960893));
#70742=CARTESIAN_POINT('Ctrl Pts',(-0.0522178637634279,1.78151907948186,
12.6277178917979));
#70743=CARTESIAN_POINT('Ctrl Pts',(-0.032582528648154,1.77936609021369,
12.6288329992982));
#70744=CARTESIAN_POINT('Ctrl Pts',(-0.0300353424680076,1.77911746198778,
12.6289778979243));
#70745=CARTESIAN_POINT('Ctrl Pts',(-0.0179680999931977,1.77808453369203,
12.6296662139752));
#70746=CARTESIAN_POINT('Ctrl Pts',(-0.00841983568812099,1.77769346042888,
12.630216509681));
#70747=CARTESIAN_POINT('Ctrl Pts',(0.00835066081367094,1.77775232614261,
12.6312041915843));
#70748=CARTESIAN_POINT('Ctrl Pts',(0.0155667529695329,1.77802024795877,
12.6316360091664));
#70749=CARTESIAN_POINT('Ctrl Pts',(0.0237383780460576,1.77859898471538,
12.6321348243136));
#70750=CARTESIAN_POINT('Ctrl Pts',(0.0247090648291275,1.77867215293273,
12.6321942337122));
#70751=CARTESIAN_POINT('Ctrl Pts',(0.0261694510710479,1.77878889006884,
12.6322838548113));
#70752=CARTESIAN_POINT('Ctrl Pts',(0.0266594127649577,1.77882918404787,
12.6323139635704));
#70753=CARTESIAN_POINT('Ctrl Pts',(0.0275030836455508,1.77890051060771,
12.6323658790763));
#70754=CARTESIAN_POINT('Ctrl Pts',(0.0278568382811187,1.77893100701354,
12.6323876689302));
#70755=CARTESIAN_POINT('Ctrl Pts',(0.0285863904456573,1.77899511489679,
12.6324326509772));
#70756=CARTESIAN_POINT('Ctrl Pts',(0.0289621806781749,1.77902880181032,
12.6324558455127));
#70757=CARTESIAN_POINT('Ctrl Pts',(0.0299762541646356,1.77912150165511,
12.6325185025269));
#70758=CARTESIAN_POINT('Ctrl Pts',(0.0306144194441522,1.77918175889387,
12.6325580040958));
#70759=CARTESIAN_POINT('Ctrl Pts',(0.0329696722154685,1.77941123948419,
12.6327040559405));
#70760=CARTESIAN_POINT('Ctrl Pts',(0.0346855484848275,1.77959234529213,
12.6328109795501));
#70761=CARTESIAN_POINT('Ctrl Pts',(0.0636346891724505,1.78288310933234,
12.6346239357937));
#70762=CARTESIAN_POINT('Ctrl Pts',(0.0903572443348884,1.78944016818164,
12.6364470189146));
#70763=CARTESIAN_POINT('Ctrl Pts',(0.129203829033449,1.80441553176713,12.6392638367271));
#70764=CARTESIAN_POINT('Ctrl Pts',(0.142132738459312,1.81041040968414,12.6402291913141));
#70765=CARTESIAN_POINT('Ctrl Pts',(0.158836856858038,1.81954485116631,12.6414835146814));
#70766=CARTESIAN_POINT('Ctrl Pts',(0.162998521407312,1.82194294717615,12.6417965570157));
#70767=CARTESIAN_POINT('Ctrl Pts',(0.16908119966043,1.82563151839742,12.6422532500383));
#70768=CARTESIAN_POINT('Ctrl Pts',(0.171044273971853,1.82685100620375,12.6424005036394));
#70769=CARTESIAN_POINT('Ctrl Pts',(0.173773732773531,1.82858754775436,12.6426048699034));
#70770=CARTESIAN_POINT('Ctrl Pts',(0.174551216280972,1.82908690991551,12.6426630402455));
#70771=CARTESIAN_POINT('Ctrl Pts',(0.17589647198174,1.8299591361978,12.6427636006482));
#70772=CARTESIAN_POINT('Ctrl Pts',(0.176465228297705,1.8303304611188,12.6428060881676));
#70773=CARTESIAN_POINT('Ctrl Pts',(0.177283037904706,1.83086808110544,12.642867135109));
#70774=CARTESIAN_POINT('Ctrl Pts',(0.17753303512872,1.83103292629707,12.6428857904756));
#70775=CARTESIAN_POINT('Ctrl Pts',(0.177968647674363,1.83132103596253,12.642918285638));
#70776=CARTESIAN_POINT('Ctrl Pts',(0.178154365334642,1.83144414475814,12.6429321359439));
#70777=CARTESIAN_POINT('Ctrl Pts',(0.178511996001877,1.83168174573787,12.6429587999387));
#70778=CARTESIAN_POINT('Ctrl Pts',(0.17868392624026,1.83179621033472,12.6429716154563));
#70779=CARTESIAN_POINT('Ctrl Pts',(0.179091948830611,1.83206842270357,12.6430020219018));
#70780=CARTESIAN_POINT('Ctrl Pts',(0.179327943455863,1.83222631767512,12.6430196028575));
#70781=CARTESIAN_POINT('Ctrl Pts',(0.180034324187824,1.83270028263979,12.6430722101546));
#70782=CARTESIAN_POINT('Ctrl Pts',(0.180504088739578,1.83301728380587,12.6431071741185));
#70783=CARTESIAN_POINT('Ctrl Pts',(0.185036141744048,1.83609298151457,12.6434443062806));
#70784=CARTESIAN_POINT('Ctrl Pts',(0.189035983359318,1.83894312582869,12.643740427882));
#70785=CARTESIAN_POINT('Ctrl Pts',(0.194286161150776,1.84286819287913,12.6441294590774));
#70786=CARTESIAN_POINT('Ctrl Pts',(0.195595413669306,1.84386270674848,12.6442265020967));
#70787=CARTESIAN_POINT('Ctrl Pts',(0.197458006305936,1.84530015016024,12.6443646914499));
#70788=CARTESIAN_POINT('Ctrl Pts',(0.198017565662223,1.84573493856557,12.6444062235031));
#70789=CARTESIAN_POINT('Ctrl Pts',(0.201721770456884,1.84863282132245,12.6446813080671));
#70790=CARTESIAN_POINT('Ctrl Pts',(0.204821927565954,1.85115243355031,12.6449122477602));
#70791=CARTESIAN_POINT('Ctrl Pts',(0.22482649081042,1.86803806472242,12.6464129843889));
#70792=CARTESIAN_POINT('Ctrl Pts',(0.240256246804799,1.88405945487228,12.6476249423491));
#70793=CARTESIAN_POINT('Ctrl Pts',(0.264450340574353,1.91501436316179,12.6498536871035));
#70794=CARTESIAN_POINT('Ctrl Pts',(0.273891385891835,1.92930422142116,12.6508472312825));
#70795=CARTESIAN_POINT('Ctrl Pts',(0.28272523996759,1.94530994264776,12.6519586851609));
#70796=CARTESIAN_POINT('Ctrl Pts',(0.283291170421165,1.94634881106424,12.652030809099));
#70797=CARTESIAN_POINT('Ctrl Pts',(0.284103475539937,1.94785968888747,12.6521356878562));
#70798=CARTESIAN_POINT('Ctrl Pts',(0.284354425214816,1.9483292383659,12.6521682799478));
#70799=CARTESIAN_POINT('Ctrl Pts',(0.284790727020741,1.94915048732087,12.6522252813045));
#70800=CARTESIAN_POINT('Ctrl Pts',(0.284976594560447,1.94950191289264,12.6522496722387));
#70801=CARTESIAN_POINT('Ctrl Pts',(0.285334741546027,1.95018211499849,12.6522968808661));
#70802=CARTESIAN_POINT('Ctrl Pts',(0.285507104276185,1.95051084719786,12.6523196955664));
#70803=CARTESIAN_POINT('Ctrl Pts',(0.285914937941978,1.95129195054275,12.6523739047866));
#70804=CARTESIAN_POINT('Ctrl Pts',(0.286149903228206,1.9517445832711,12.6524053170949));
#70805=CARTESIAN_POINT('Ctrl Pts',(0.286974679094783,1.95334268121504,12.6525162223056));
#70806=CARTESIAN_POINT('Ctrl Pts',(0.287558688072607,1.95449111219108,12.6525959190091));
#70807=CARTESIAN_POINT('Ctrl Pts',(0.296486187531674,1.97231035276441,12.6538325568906));
#70808=CARTESIAN_POINT('Ctrl Pts',(0.303373155113652,1.98966770968823,12.655041027468));
#70809=CARTESIAN_POINT('Ctrl Pts',(0.31335330594097,2.02298397179068,12.6573612594581));
#70810=CARTESIAN_POINT('Ctrl Pts',(0.31681706446449,2.0387735983825,12.6584603876228));
#70811=CARTESIAN_POINT('Ctrl Pts',(0.321209239133184,2.06974889480681,12.6605679766027));
#70812=CARTESIAN_POINT('Ctrl Pts',(0.322276106084797,2.08487587596805,12.661574888799));
#70813=CARTESIAN_POINT('Ctrl Pts',(0.322274931633552,2.10094731643302,12.6625856179645));
#70814=CARTESIAN_POINT('Ctrl Pts',(0.322270892319163,2.10187109091309,12.6626435043966));
#70815=CARTESIAN_POINT('Ctrl Pts',(0.322259938807276,2.10313409683487,12.6627223498357));
#70816=CARTESIAN_POINT('Ctrl Pts',(0.322256460944064,2.10347334210428,12.6627434984175));
#70817=CARTESIAN_POINT('Ctrl Pts',(0.322250032133136,2.10401672699517,12.6627773252712));
#70818=CARTESIAN_POINT('Ctrl Pts',(0.322247422905286,2.10422086922562,12.6627900227457));
#70819=CARTESIAN_POINT('Ctrl Pts',(0.322241578492425,2.1046464797449,12.6628164726298));
#70820=CARTESIAN_POINT('Ctrl Pts',(0.322238308986342,2.10486794670926,12.6628302229931));
#70821=CARTESIAN_POINT('Ctrl Pts',(0.322230189759312,2.10538201360899,12.6628621106337));
#70822=CARTESIAN_POINT('Ctrl Pts',(0.322225169794744,2.10567461145633,12.6628802382985));
#70823=CARTESIAN_POINT('Ctrl Pts',(0.322207606835458,2.10662298407759,12.6629389231083));
#70824=CARTESIAN_POINT('Ctrl Pts',(0.322193460340211,2.10727873289414,12.6629793906942));
#70825=CARTESIAN_POINT('Ctrl Pts',(0.322036318261357,2.11365947405338,12.6633721299591));
#70826=CARTESIAN_POINT('Ctrl Pts',(0.321742739571791,2.11938016842448,12.6637161824122));
#70827=CARTESIAN_POINT('Ctrl Pts',(0.321260061828799,2.12556112710748,12.6640820960283));
#70828=CARTESIAN_POINT('Ctrl Pts',(0.321222268926149,2.12603175936495,12.664109920897));
#70829=CARTESIAN_POINT('Ctrl Pts',(0.318902950200669,2.15413975421192,12.6657696314752));
#70830=CARTESIAN_POINT('Ctrl Pts',(0.313064695962023,2.18136982709652,12.6672652695433));
#70831=CARTESIAN_POINT('Ctrl Pts',(0.298812567944701,2.22164158169612,12.6696921560592));
#70832=CARTESIAN_POINT('Ctrl Pts',(0.292836263485593,2.23539742039894,12.6705616877709));
#70833=CARTESIAN_POINT('Ctrl Pts',(0.285192942406668,2.25009557910688,12.6715612456403));
#70834=CARTESIAN_POINT('Ctrl Pts',(0.284449915566278,2.25149898567876,12.6716574124135));
#70835=CARTESIAN_POINT('Ctrl Pts',(0.283129747846024,2.25394852665679,12.6718265720009));
#70836=CARTESIAN_POINT('Ctrl Pts',(0.282557100614126,2.25499705741575,12.6718994051566));
#70837=CARTESIAN_POINT('Ctrl Pts',(0.281719816945964,2.25651008310049,12.6720051276942));
#70838=CARTESIAN_POINT('Ctrl Pts',(0.281459829496123,2.25697715039701,12.6720378506277));
#70839=CARTESIAN_POINT('Ctrl Pts',(0.281004289498087,2.2577907577746,12.6720950045516));
#70840=CARTESIAN_POINT('Ctrl Pts',(0.280809254422768,2.2581375875105,12.6721194169179));
#70841=CARTESIAN_POINT('Ctrl Pts',(0.280431323158472,2.25880675669054,12.6721666118676));
#70842=CARTESIAN_POINT('Ctrl Pts',(0.28024851217878,2.25912914377567,12.6721893913554));
#70843=CARTESIAN_POINT('Ctrl Pts',(0.279813899048572,2.25989251199931,12.6722434307136));
#70844=CARTESIAN_POINT('Ctrl Pts',(0.279561610483123,2.2603332137568,12.6722747081106));
#70845=CARTESIAN_POINT('Ctrl Pts',(0.278671921014469,2.26187885357189,12.6723846870006));
#70846=CARTESIAN_POINT('Ctrl Pts',(0.278029008799322,2.26298059082657,12.6724635878451));
#70847=CARTESIAN_POINT('Ctrl Pts',(0.268606400872723,2.27890979248885,12.6736118254267));
#70848=CARTESIAN_POINT('Ctrl Pts',(0.258659382805385,2.29301103828681,12.6747249028285));
#70849=CARTESIAN_POINT('Ctrl Pts',(0.232617834483761,2.32427820237332,12.6774292264098));
#70850=CARTESIAN_POINT('Ctrl Pts',(0.215678009381438,2.34061311885854,12.6790425177258));
#70851=CARTESIAN_POINT('Ctrl Pts',(0.190201726535308,2.36030915232194,12.6811776633843));
#70852=CARTESIAN_POINT('Ctrl Pts',(0.183072419183627,2.36537157245333,12.6817474605309));
#70853=CARTESIAN_POINT('Ctrl Pts',(0.174999731144078,2.37062346752309,12.6823555625261));
#70854=CARTESIAN_POINT('Ctrl Pts',(0.174252003085409,2.37110552657333,12.6824115475311));
#70855=CARTESIAN_POINT('Ctrl Pts',(0.172946523591007,2.37193953468199,12.6825086894062));
#70856=CARTESIAN_POINT('Ctrl Pts',(0.172389674509169,2.37229287667165,12.6825499349618));
#70857=CARTESIAN_POINT('Ctrl Pts',(0.171581782647307,2.37280204321679,12.6826094959071));
#70858=CARTESIAN_POINT('Ctrl Pts',(0.171331608661035,2.37295923284435,12.682627901082));
#70859=CARTESIAN_POINT('Ctrl Pts',(0.170892989624312,2.37323398590605,12.682660101959));
#70860=CARTESIAN_POINT('Ctrl Pts',(0.170704638816866,2.3733516988139,12.6826739076296));
#70861=CARTESIAN_POINT('Ctrl Pts',(0.170340009620423,2.37357905592845,12.6827005914425));
#70862=CARTESIAN_POINT('Ctrl Pts',(0.170163747440561,2.37368872424305,12.6827134712121));
#70863=CARTESIAN_POINT('Ctrl Pts',(0.169742767067178,2.37395008952703,12.6827441874106));
#70864=CARTESIAN_POINT('Ctrl Pts',(0.169497950801575,2.3741016293258,12.6827620133868));
#70865=CARTESIAN_POINT('Ctrl Pts',(0.168623715633899,2.37464115651323,12.6828255401566));
#70866=CARTESIAN_POINT('Ctrl Pts',(0.167993158793409,2.37502730946052,12.6828711207182));
#70867=CARTESIAN_POINT('Ctrl Pts',(0.158338294576425,2.38089435408875,12.683565475993));
#70868=CARTESIAN_POINT('Ctrl Pts',(0.149050205269201,2.38593136066844,12.6841861260136));
#70869=CARTESIAN_POINT('Ctrl Pts',(0.115842128055158,2.40188137992821,12.6863028573398));
#70870=CARTESIAN_POINT('Ctrl Pts',(0.0908506660060515,2.41031930079258,
12.6877266112227));
#70871=CARTESIAN_POINT('Ctrl Pts',(0.0559631144688198,2.41751621407871,
12.6897700651807));
#70872=CARTESIAN_POINT('Ctrl Pts',(0.046738418792484,2.41900456779105,12.6903144461336));
#70873=CARTESIAN_POINT('Ctrl Pts',(0.0328141551664482,2.4206342329586,12.6911501882692));
#70874=CARTESIAN_POINT('Ctrl Pts',(0.0281545578310163,2.42107693395974,
12.6914321578811));
#70875=CARTESIAN_POINT('Ctrl Pts',(0.0226172468280913,2.42148156485683,
12.691770493883));
#70876=CARTESIAN_POINT('Ctrl Pts',(0.0217470962122639,2.42154159945444,
12.6918237557348));
#70877=CARTESIAN_POINT('Ctrl Pts',(0.0204073634932882,2.42162856894783,
12.6919059099216));
#70878=CARTESIAN_POINT('Ctrl Pts',(0.0199379435579667,2.42165800977303,
12.6919347235605));
#70879=CARTESIAN_POINT('Ctrl Pts',(0.0190821787669227,2.42170980065954,
12.6919873035723));
#70880=CARTESIAN_POINT('Ctrl Pts',(0.0186958542693854,2.42173248269013,
12.692011059481));
#70881=CARTESIAN_POINT('Ctrl Pts',(0.0178538189901202,2.42178039884677,
12.6920628804837));
#70882=CARTESIAN_POINT('Ctrl Pts',(0.0173980941028262,2.42180536082032,
12.6920909540651));
#70883=CARTESIAN_POINT('Ctrl Pts',(0.0161564767652849,2.42187072427285,
12.6921675148444));
#70884=CARTESIAN_POINT('Ctrl Pts',(0.0153704906936252,2.4219092152823,12.6922160618568));
#70885=CARTESIAN_POINT('Ctrl Pts',(0.0116006579549702,2.42207999194193,
12.6924493054261));
#70886=CARTESIAN_POINT('Ctrl Pts',(0.00861528837951467,2.42217366794012,
12.6926352079763));
#70887=CARTESIAN_POINT('Ctrl Pts',(0.00440153812928454,2.42224728008276,
12.6928993718858));
#70888=CARTESIAN_POINT('Ctrl Pts',(0.00317385091221689,2.42226170989115,
12.692976548198));
#70889=CARTESIAN_POINT('Ctrl Pts',(0.00129576556333843,2.42227305130751,
12.6930949384668));
#70890=CARTESIAN_POINT('Ctrl Pts',(0.00064539986456536,2.42227500997834,
12.6931359961843));
#70891=CARTESIAN_POINT('Ctrl Pts',(-0.0301634909334848,2.42227453547553,
12.6950838324592));
#70892=CARTESIAN_POINT('Ctrl Pts',(-0.0601677324211988,2.41804054828723,
12.697132098493));
#70893=CARTESIAN_POINT('Ctrl Pts',(-0.0969512851132294,2.40745363310054,
12.6997131933395));
#70894=CARTESIAN_POINT('Ctrl Pts',(-0.104677547501558,2.40490967925323,
12.7002580873391));
#70895=CARTESIAN_POINT('Ctrl Pts',(-0.11911468164049,2.39954253729782,12.7012725062849));
#70896=CARTESIAN_POINT('Ctrl Pts',(-0.125842644935426,2.39677885124912,
12.701743609366));
#70897=CARTESIAN_POINT('Ctrl Pts',(-0.133568556171125,2.39329518169239,
12.7022780409889));
#70898=CARTESIAN_POINT('Ctrl Pts',(-0.134662456122448,2.39279454540867,
12.7023535533578));
#70899=CARTESIAN_POINT('Ctrl Pts',(-0.136094799150632,2.39212929131218,
12.7024521971335));
#70900=CARTESIAN_POINT('Ctrl Pts',(-0.136435775152762,2.39197019789751,
12.7024756624557));
#70901=CARTESIAN_POINT('Ctrl Pts',(-0.136991572205964,2.39170968650625,
12.7025138821698));
#70902=CARTESIAN_POINT('Ctrl Pts',(-0.137206559894064,2.39160862809586,
12.7025286587888));
#70903=CARTESIAN_POINT('Ctrl Pts',(-0.137621794943528,2.3914128793418,12.7025571848057));
#70904=CARTESIAN_POINT('Ctrl Pts',(-0.137822055917343,2.39131822049557,
12.7025709360565));
#70905=CARTESIAN_POINT('Ctrl Pts',(-0.138286741032999,2.3910979879146,12.7026028299271));
#70906=CARTESIAN_POINT('Ctrl Pts',(-0.138551092715102,2.39097225988491,
12.7026209629229));
#70907=CARTESIAN_POINT('Ctrl Pts',(-0.139407631246628,2.39056345054624,
12.7026796823161));
#70908=CARTESIAN_POINT('Ctrl Pts',(-0.139999129554428,2.39027891791343,
12.7027201790069));
#70909=CARTESIAN_POINT('Ctrl Pts',(-0.145757603908711,2.38748718255777,
12.7031139522351));
#70910=CARTESIAN_POINT('Ctrl Pts',(-0.150857947107048,2.38484390285048,
12.7034589621373));
#70911=CARTESIAN_POINT('Ctrl Pts',(-0.156542820691324,2.38170212161456,
12.7038422749471));
#70912=CARTESIAN_POINT('Ctrl Pts',(-0.157199089401506,2.3813364291061,12.7038865059924));
#70913=CARTESIAN_POINT('Ctrl Pts',(-0.158924175049733,2.38036723910117,
12.7040027384602));
#70914=CARTESIAN_POINT('Ctrl Pts',(-0.159990841077548,2.37975992032515,
12.7040745730923));
#70915=CARTESIAN_POINT('Ctrl Pts',(-0.164589420662945,2.37710676254905,
12.7043842253612));
#70916=CARTESIAN_POINT('Ctrl Pts',(-0.168085866503903,2.37499996166468,
12.7046195658867));
#70917=CARTESIAN_POINT('Ctrl Pts',(-0.182324404307719,2.36604741173927,
12.7055814015772));
#70918=CARTESIAN_POINT('Ctrl Pts',(-0.192696375987787,2.35863400244468,
12.706290692235));
#70919=CARTESIAN_POINT('Ctrl Pts',(-0.212956776373089,2.34225575991361,
12.7077472184702));
#70920=CARTESIAN_POINT('Ctrl Pts',(-0.222781813165474,2.33325238975243,
12.7084934685184));
#70921=CARTESIAN_POINT('Ctrl Pts',(-0.239982591609493,2.31540917720707,
12.7099197394892));
#70922=CARTESIAN_POINT('Ctrl Pts',(-0.247496346665469,2.30673236935726,
12.710593488435));
#70923=CARTESIAN_POINT('Ctrl Pts',(-0.255784989053216,2.29605966919968,
12.7114105341652));
#70924=CARTESIAN_POINT('Ctrl Pts',(-0.257023449190687,2.29443328104845,
12.7115347266316));
#70925=CARTESIAN_POINT('Ctrl Pts',(-0.258642203218125,2.29226498442269,
12.7116999290876));
#70926=CARTESIAN_POINT('Ctrl Pts',(-0.259036438906985,2.29173350471078,
12.711740393335));
#70927=CARTESIAN_POINT('Ctrl Pts',(-0.259680455280729,2.29085967714637,
12.7118068761416));
#70928=CARTESIAN_POINT('Ctrl Pts',(-0.2599312038883,2.29051804234162,12.7118328569957));
#70929=CARTESIAN_POINT('Ctrl Pts',(-0.260415398671583,2.28985561136627,
12.7118832121895));
#70930=CARTESIAN_POINT('Ctrl Pts',(-0.260648927851673,2.28953487657968,
12.7119075832492));
#70931=CARTESIAN_POINT('Ctrl Pts',(-0.261186214566062,2.28879408270519,
12.7119638503217));
#70932=CARTESIAN_POINT('Ctrl Pts',(-0.261489551451457,2.28837372115173,
12.7119957625081));
#70933=CARTESIAN_POINT('Ctrl Pts',(-0.262455662772666,2.28702806246782,
12.7120978685487));
#70934=CARTESIAN_POINT('Ctrl Pts',(-0.26311454460571,2.28609999311008,12.7121682118643));
#70935=CARTESIAN_POINT('Ctrl Pts',(-0.269058100290468,2.27763352594785,
12.7128092712413));
#70936=CARTESIAN_POINT('Ctrl Pts',(-0.274021925476739,2.26987609396934,
12.7133921052078));
#70937=CARTESIAN_POINT('Ctrl Pts',(-0.293944022309454,2.23559180971319,
12.7159525583956));
#70938=CARTESIAN_POINT('Ctrl Pts',(-0.30543216780947,2.20723261627071,12.7180515638223));
#70939=CARTESIAN_POINT('Ctrl Pts',(-0.315161040815088,2.16806663384149,
12.7207397032437));
#70940=CARTESIAN_POINT('Ctrl Pts',(-0.317106723563917,2.15833452148095,
12.7213894667624));
#70941=CARTESIAN_POINT('Ctrl Pts',(-0.318818403965751,2.14709665448337,
12.7221079047565));
#70942=CARTESIAN_POINT('Ctrl Pts',(-0.319026663470127,2.14566462255405,
12.722198865012));
#70943=CARTESIAN_POINT('Ctrl Pts',(-0.319280521766391,2.14383247747162,
12.722314444726));
#70944=CARTESIAN_POINT('Ctrl Pts',(-0.319335021884388,2.14343364436722,
12.7223395567739));
#70945=CARTESIAN_POINT('Ctrl Pts',(-0.31942128154863,2.14279345485475,12.7223797872454));
#70946=CARTESIAN_POINT('Ctrl Pts',(-0.31945351491635,2.1425521643763,12.7223949324639));
#70947=CARTESIAN_POINT('Ctrl Pts',(-0.319514309987767,2.14209310604026,
12.7224237122151));
#70948=CARTESIAN_POINT('Ctrl Pts',(-0.319542922233879,2.14187534732476,
12.7224373494819));
#70949=CARTESIAN_POINT('Ctrl Pts',(-0.319607554410098,2.14137952878586,
12.7224683672128));
#70950=CARTESIAN_POINT('Ctrl Pts',(-0.319643434039418,2.14110145150065,
12.7224857396136));
#70951=CARTESIAN_POINT('Ctrl Pts',(-0.31975378018135,2.14023735388963,12.7225396498846));
#70952=CARTESIAN_POINT('Ctrl Pts',(-0.319826998900076,2.13965117117984,
12.7225761173822));
#70953=CARTESIAN_POINT('Ctrl Pts',(-0.320374987342286,2.13516373476118,
12.7228545167446));
#70954=CARTESIAN_POINT('Ctrl Pts',(-0.320779997052963,2.13125408190264,
12.7230926061921));
#70955=CARTESIAN_POINT('Ctrl Pts',(-0.321880646213262,2.11832570593583,
12.7238680874627));
#70956=CARTESIAN_POINT('Ctrl Pts',(-0.322268220777703,2.10928454586238,
12.7243915076839));
#70957=CARTESIAN_POINT('Ctrl Pts',(-0.3222980136772,2.06900520556015,12.7266854167059));
#70958=CARTESIAN_POINT('Ctrl Pts',(-0.317781127774183,2.03793606687203,
12.7283711669917));
#70959=CARTESIAN_POINT('Ctrl Pts',(-0.30696909246082,2.00163717397536,12.7306064103029));
#70960=CARTESIAN_POINT('Ctrl Pts',(-0.304877384437114,1.99533367262709,
12.7310039785322));
#70961=CARTESIAN_POINT('Ctrl Pts',(-0.30223487916569,1.98812357705959,12.7314713224698));
#70962=CARTESIAN_POINT('Ctrl Pts',(-0.301872450919865,1.98714930425478,
12.7315347416019));
#70963=CARTESIAN_POINT('Ctrl Pts',(-0.301326977087005,1.98570440306193,
12.7316292016562));
#70964=CARTESIAN_POINT('Ctrl Pts',(-0.301147526216988,1.98523241725721,
12.7316601221923));
#70965=CARTESIAN_POINT('Ctrl Pts',(-0.300826245251008,1.98439333640509,
12.7317152074847));
#70966=CARTESIAN_POINT('Ctrl Pts',(-0.300684850298476,1.98402607492126,
12.7317393575998));
#70967=CARTESIAN_POINT('Ctrl Pts',(-0.300386098065088,1.98325431014875,
12.731790190404));
#70968=CARTESIAN_POINT('Ctrl Pts',(-0.30022859571811,1.98284986419209,12.7318168779311));
#70969=CARTESIAN_POINT('Ctrl Pts',(-0.29981212319551,1.98178677192677,12.7318871546343));
#70970=CARTESIAN_POINT('Ctrl Pts',(-0.299551800644933,1.98112866104859,
12.7319307892876));
#70971=CARTESIAN_POINT('Ctrl Pts',(-0.298380125612294,1.97819488731416,
12.732125890853));
#70972=CARTESIAN_POINT('Ctrl Pts',(-0.297445013241985,1.9759288575038,12.7322781584792));
#70973=CARTESIAN_POINT('Ctrl Pts',(-0.29042747320749,1.95945888612768,12.7333966617674));
#70974=CARTESIAN_POINT('Ctrl Pts',(-0.283357282461509,1.9457001380034,12.7343969780078));
#70975=CARTESIAN_POINT('Ctrl Pts',(-0.258527893869593,1.90488600248727,
12.7375693276821));
#70976=CARTESIAN_POINT('Ctrl Pts',(-0.237669020585884,1.87995568670838,
12.7398270568302));
#70977=CARTESIAN_POINT('Ctrl Pts',(-0.212337273616127,1.85756182886676,
12.7419652587983));
#70978=CARTESIAN_POINT('Ctrl Pts',(-0.211216922126842,1.85658513480374,
12.7420587299654));
#70979=CARTESIAN_POINT('Ctrl Pts',(-0.209767496374826,1.85533910453047,
12.7421782097466));
#70980=CARTESIAN_POINT('Ctrl Pts',(-0.209444614117482,1.85506264080497,
12.7422047343115));
#70981=CARTESIAN_POINT('Ctrl Pts',(-0.208932125437122,1.85462558339571,
12.7422466889626));
#70982=CARTESIAN_POINT('Ctrl Pts',(-0.208742880082693,1.85446457001207,
12.7422621500264));
#70983=CARTESIAN_POINT('Ctrl Pts',(-0.208403424497302,1.85417643114158,
12.7422898264909));
#70984=CARTESIAN_POINT('Ctrl Pts',(-0.208253285138892,1.85404922529566,
12.7423020478385));
#70985=CARTESIAN_POINT('Ctrl Pts',(-0.207899995204906,1.85375045518358,
12.7423307592287));
#70986=CARTESIAN_POINT('Ctrl Pts',(-0.207696749043881,1.85357900502124,
12.7423472407803));
#70987=CARTESIAN_POINT('Ctrl Pts',(-0.207106884593097,1.85308266767366,
12.7423949703796));
#70988=CARTESIAN_POINT('Ctrl Pts',(-0.206719712340603,1.85275843555941,
12.7424261703386));
#70989=CARTESIAN_POINT('Ctrl Pts',(-0.204037913078161,1.85052330273849,
12.7426414067777));
#70990=CARTESIAN_POINT('Ctrl Pts',(-0.201717489824324,1.84864338423648,
12.7428232273925));
#70991=CARTESIAN_POINT('Ctrl Pts',(-0.194377244848565,1.84286372542345,
12.743385933902));
#70992=CARTESIAN_POINT('Ctrl Pts',(-0.189267727330464,1.83907986753902,
12.743759810019));
#70993=CARTESIAN_POINT('Ctrl Pts',(-0.171146198593381,1.826472622341,12.7450379286634));
#70994=CARTESIAN_POINT('Ctrl Pts',(-0.157602797201683,1.8184512994269,12.7459114119524));
#70995=CARTESIAN_POINT('Ctrl Pts',(-0.121062001803699,1.80027558308879,
12.7481933628477));
#70996=CARTESIAN_POINT('Ctrl Pts',(-0.0973724990780165,1.79176457423886,
12.7496089563464));
#70997=CARTESIAN_POINT('Ctrl Pts',(-0.071401661738542,1.78573026827096,
12.7512253491736));
#70998=CARTESIAN_POINT('Ctrl Pts',(-0.0698633049023688,1.7853847110031,
12.7513212893368));
#70999=CARTESIAN_POINT('Ctrl Pts',(-0.0677192104231427,1.78491958924006,
12.7514552975027));
#71000=CARTESIAN_POINT('Ctrl Pts',(-0.0671155541168977,1.78479045209226,
12.7514930586409));
#71001=CARTESIAN_POINT('Ctrl Pts',(-0.0661468718781647,1.78458613559324,
12.7515537061667));
#71002=CARTESIAN_POINT('Ctrl Pts',(-0.0657820780349808,1.78450985320175,
12.7515765572141));
#71003=CARTESIAN_POINT('Ctrl Pts',(-0.0650287355410895,1.78435368443279,
12.7516237723065));
#71004=CARTESIAN_POINT('Ctrl Pts',(-0.0646401702072823,1.78427388234324,
12.7516481390043));
#71005=CARTESIAN_POINT('Ctrl Pts',(-0.0637350661091332,1.78408973635926,
12.7517049298787));
#71006=CARTESIAN_POINT('Ctrl Pts',(-0.0632184178936092,1.78398594183286,
12.7517373715434));
#71007=CARTESIAN_POINT('Ctrl Pts',(-0.0615698020172943,1.78365893994127,
12.7518409718653));
#71008=CARTESIAN_POINT('Ctrl Pts',(-0.0604368988732375,1.78344054587071,
12.7519122838711));
#71009=CARTESIAN_POINT('Ctrl Pts',(-0.0349713140770128,1.77867313226768,
12.7535180205679));
#71010=CARTESIAN_POINT('Ctrl Pts',(-0.0102014481847637,1.77693749736386,
12.7551465958483));
#71011=CARTESIAN_POINT('Ctrl Pts',(0.0392963744586832,1.77916950582992,
12.7584894940021));
#71012=CARTESIAN_POINT('Ctrl Pts',(0.063865145861179,1.7831437859012,12.7601910495075));
#71013=CARTESIAN_POINT('Ctrl Pts',(0.0890940594577364,1.7902817159124,12.761848024256));
#71014=CARTESIAN_POINT('Ctrl Pts',(0.0904493874471372,1.79067480637249,
12.7619367328674));
#71015=CARTESIAN_POINT('Ctrl Pts',(0.0922015083168492,1.79119548078547,
12.762050975548));
#71016=CARTESIAN_POINT('Ctrl Pts',(0.0926006698698686,1.79131494178123,
12.7620769724326));
#71017=CARTESIAN_POINT('Ctrl Pts',(0.0932121357200198,1.79149923394967,
12.7621167500453));
#71018=CARTESIAN_POINT('Ctrl Pts',(0.0934246046612958,1.79156351035633,
12.7621305631674));
#71019=CARTESIAN_POINT('Ctrl Pts',(0.0938435847576729,1.79169073346145,
12.7621577848877));
#71020=CARTESIAN_POINT('Ctrl Pts',(0.0940500978343611,1.79175366777266,
12.7621711940475));
#71021=CARTESIAN_POINT('Ctrl Pts',(0.0945107968945404,1.79189457066812,
12.7622010894277));
#71022=CARTESIAN_POINT('Ctrl Pts',(0.0947649490451584,1.79197264610572,
12.7622175692334));
#71023=CARTESIAN_POINT('Ctrl Pts',(0.0955014279907667,1.79219988991929,
12.7622652888352));
#71024=CARTESIAN_POINT('Ctrl Pts',(0.0959835040252072,1.79234987814531,
12.7622964805738));
#71025=CARTESIAN_POINT('Ctrl Pts',(0.0993116036978307,1.79339393324283,
12.7625115268883));
#71026=CARTESIAN_POINT('Ctrl Pts',(0.102145565574032,1.79432638358897,12.7626931700653));
#71027=CARTESIAN_POINT('Ctrl Pts',(0.110972785339516,1.79736725894137,12.7632555126664));
#71028=CARTESIAN_POINT('Ctrl Pts',(0.11691720449251,1.79961372627749,12.7636292066262));
#71029=CARTESIAN_POINT('Ctrl Pts',(0.137314296259386,1.80801937979289,12.764906532903));
#71030=CARTESIAN_POINT('Ctrl Pts',(0.151380871440545,1.81505826015645,12.7657794356856));
#71031=CARTESIAN_POINT('Ctrl Pts',(0.186555291292564,1.83600234546141,12.7680684178094));
#71032=CARTESIAN_POINT('Ctrl Pts',(0.206637743401506,1.85140751406754,12.7694917914411));
#71033=CARTESIAN_POINT('Ctrl Pts',(0.22578549421405,1.87003411964847,12.771112154926));
#71034=CARTESIAN_POINT('Ctrl Pts',(0.226846237074405,1.87108040684051,12.77120284892));
#71035=CARTESIAN_POINT('Ctrl Pts',(0.228283284064847,1.87251766618022,12.7713270103677));
#71036=CARTESIAN_POINT('Ctrl Pts',(0.228665923885607,1.87290230025078,12.7713601971794));
#71037=CARTESIAN_POINT('Ctrl Pts',(0.229314857591101,1.8735579189781,12.7714166966568));
#71038=CARTESIAN_POINT('Ctrl Pts',(0.229581647797675,1.87382841256679,12.7714399874238));
#71039=CARTESIAN_POINT('Ctrl Pts',(0.230118324678067,1.87437446721308,12.7714869661206));
#71040=CARTESIAN_POINT('Ctrl Pts',(0.230388196197885,1.87465004227048,12.7715106546591));
#71041=CARTESIAN_POINT('Ctrl Pts',(0.2310005269371,1.87527756381501,12.7715645516838));
#71042=CARTESIAN_POINT('Ctrl Pts',(0.231342677152315,1.87562980925738,12.7715947735851));
#71043=CARTESIAN_POINT('Ctrl Pts',(0.232056295744779,1.87636785101841,12.7716580299529));
#71044=CARTESIAN_POINT('Ctrl Pts',(0.232427609909756,1.8767537937635,12.7716910709992));
#71045=CARTESIAN_POINT('Ctrl Pts',(0.233398298160891,1.8777677707484,12.7717777819875));
#71046=CARTESIAN_POINT('Ctrl Pts',(0.233996096589068,1.87839730132519,12.7718315198894));
#71047=CARTESIAN_POINT('Ctrl Pts',(0.235763774619217,1.88027393851874,12.7719914316652));
#71048=CARTESIAN_POINT('Ctrl Pts',(0.236926266307724,1.8815279338937,12.7720979208166));
#71049=CARTESIAN_POINT('Ctrl Pts',(0.249595770763598,1.89541474631622,12.7732733134957));
#71050=CARTESIAN_POINT('Ctrl Pts',(0.260088709742853,1.90893228567935,12.7743847600436));
#71051=CARTESIAN_POINT('Ctrl Pts',(0.284974320967406,1.94686365838458,12.7774119995573));
#71052=CARTESIAN_POINT('Ctrl Pts',(0.29730807380174,1.97244997711326,12.7793724891378));
#71053=CARTESIAN_POINT('Ctrl Pts',(0.307223558791195,2.00259978892891,12.7814106527746));
#71054=CARTESIAN_POINT('Ctrl Pts',(0.308250294919806,2.00589965854843,12.7816300947249));
#71055=CARTESIAN_POINT('Ctrl Pts',(0.309383941520664,2.00976100894052,12.7818821511715));
#71056=CARTESIAN_POINT('Ctrl Pts',(0.309542635556573,2.01030688118527,12.7819176746694));
#71057=CARTESIAN_POINT('Ctrl Pts',(0.309777060170828,2.01112128233304,12.7819705073353));
#71058=CARTESIAN_POINT('Ctrl Pts',(0.309853886670054,2.01138949058335,12.7819878800527));
#71059=CARTESIAN_POINT('Ctrl Pts',(0.309990373991858,2.01186832816303,12.7820188477439));
#71060=CARTESIAN_POINT('Ctrl Pts',(0.310050168435358,2.01207891832641,12.7820324505349));
#71061=CARTESIAN_POINT('Ctrl Pts',(0.310176945271489,2.01252715160196,12.7820613680862));
#71062=CARTESIAN_POINT('Ctrl Pts',(0.310243868966954,2.01276481011532,12.7820766793561));
#71063=CARTESIAN_POINT('Ctrl Pts',(0.310423365016631,2.01340505313477,12.7821178709696));
#71064=CARTESIAN_POINT('Ctrl Pts',(0.31053542778828,2.01380778188335,12.7821437215394));
#71065=CARTESIAN_POINT('Ctrl Pts',(0.311075787940476,2.01576444968728,12.7822690311996));
#71066=CARTESIAN_POINT('Ctrl Pts',(0.311493216388209,2.01732140435859,12.7823678671197));
#71067=CARTESIAN_POINT('Ctrl Pts',(0.314933476378884,2.03054912691521,12.7832006719247));
#71068=CARTESIAN_POINT('Ctrl Pts',(0.317311280266319,2.04237934554807,12.7839002292066));
#71069=CARTESIAN_POINT('Ctrl Pts',(0.323492491125186,2.08554427789025,12.7863799730291));
#71070=CARTESIAN_POINT('Ctrl Pts',(0.323355220399317,2.11725775562877,12.7880839641929));
#71071=CARTESIAN_POINT('Ctrl Pts',(0.318558985801885,2.14880036914511,12.789972862854));
#71072=CARTESIAN_POINT('Ctrl Pts',(0.318504648706878,2.1491537609395,12.7899940476842));
#71073=CARTESIAN_POINT('Ctrl Pts',(0.317581876958154,2.15508940739074,12.790350251868));
#71074=CARTESIAN_POINT('Ctrl Pts',(0.316567439799264,2.16064768266981,12.7906894708981));
#71075=CARTESIAN_POINT('Ctrl Pts',(0.315206716276064,2.16713313427387,12.7910929155316));
#71076=CARTESIAN_POINT('Ctrl Pts',(0.315001583337389,2.16808916334379,12.7911525832712));
#71077=CARTESIAN_POINT('Ctrl Pts',(0.314685151325108,2.16953186595057,12.7912429258181));
#71078=CARTESIAN_POINT('Ctrl Pts',(0.314577065631431,2.17001924465002,12.7912734975513));
#71079=CARTESIAN_POINT('Ctrl Pts',(0.314383700140548,2.17088168064732,12.7913276881274));
#71080=CARTESIAN_POINT('Ctrl Pts',(0.314298880333391,2.17125684096698,12.7913512921594));
#71081=CARTESIAN_POINT('Ctrl Pts',(0.314118736202303,2.17204704393086,12.7914010754268));
#71082=CARTESIAN_POINT('Ctrl Pts',(0.314023260501571,2.17246205099014,12.7914272594881));
#71083=CARTESIAN_POINT('Ctrl Pts',(0.313826419523107,2.17330997014364,12.7914808362312));
#71084=CARTESIAN_POINT('Ctrl Pts',(0.313724980388417,2.17374286399562,12.7915082312425));
#71085=CARTESIAN_POINT('Ctrl Pts',(0.313472628283032,2.17480983741991,12.7915758575303));
#71086=CARTESIAN_POINT('Ctrl Pts',(0.313320687398373,2.17544366968593,12.7916161218708));
#71087=CARTESIAN_POINT('Ctrl Pts',(0.312895170433927,2.17719528632815,12.791727648093));
#71088=CARTESIAN_POINT('Ctrl Pts',(0.312617530483398,2.17831206478821,12.7917990408456));
#71089=CARTESIAN_POINT('Ctrl Pts',(0.311716471030652,2.18185532202667,12.7920264768815));
#71090=CARTESIAN_POINT('Ctrl Pts',(0.311070747664932,2.18427598372225,12.7921832376335));
#71091=CARTESIAN_POINT('Ctrl Pts',(0.308386057660836,2.19388875078528,12.7928113962438));
#71092=CARTESIAN_POINT('Ctrl Pts',(0.306125475368093,2.20101602244717,12.7932898595829));
#71093=CARTESIAN_POINT('Ctrl Pts',(0.298664231582634,2.22198051723248,12.7947358319504));
#71094=CARTESIAN_POINT('Ctrl Pts',(0.292757874081862,2.23554451715273,12.7957235828702));
#71095=CARTESIAN_POINT('Ctrl Pts',(0.282148713797219,2.2559516743852,12.7972768004029));
#71096=CARTESIAN_POINT('Ctrl Pts',(0.27807698856887,2.26310122520011,12.7978345173346));
#71097=CARTESIAN_POINT('Ctrl Pts',(0.26509302419037,2.28399746012209,12.7994949001649));
#71098=CARTESIAN_POINT('Ctrl Pts',(0.255400828351278,2.29723067303651,12.8005883409397));
#71099=CARTESIAN_POINT('Ctrl Pts',(0.24414731898204,2.31036658771123,12.801676218175));
#71100=CARTESIAN_POINT('Ctrl Pts',(0.243548433025559,2.31105964893951,12.8017336198947));
#71101=CARTESIAN_POINT('Ctrl Pts',(0.242739674038493,2.31198755965272,12.8018104674315));
#71102=CARTESIAN_POINT('Ctrl Pts',(0.242532407297021,2.31222465976554,12.8018301030824));
#71103=CARTESIAN_POINT('Ctrl Pts',(0.242183056463924,2.31262311494563,12.8018631001392));
#71104=CARTESIAN_POINT('Ctrl Pts',(0.242041158423969,2.31278463167437,12.8018764753627));
#71105=CARTESIAN_POINT('Ctrl Pts',(0.241768853951751,2.31309395988053,12.8019020899468));
#71106=CARTESIAN_POINT('Ctrl Pts',(0.24163847448526,2.31324179263786,12.8019143311182));
#71107=CARTESIAN_POINT('Ctrl Pts',(0.241329792526146,2.31359114978668,12.8019432584471));
#71108=CARTESIAN_POINT('Ctrl Pts',(0.241151373438628,2.31379257030551,12.8019599357024));
#71109=CARTESIAN_POINT('Ctrl Pts',(0.240627361924749,2.31438264576097,12.8020087916964));
#71110=CARTESIAN_POINT('Ctrl Pts',(0.240281078635024,2.31477069020068,12.8020409187787));
#71111=CARTESIAN_POINT('Ctrl Pts',(0.237701183975946,2.31764766602275,12.8022791139228));
#71112=CARTESIAN_POINT('Ctrl Pts',(0.235429787426852,2.32010265041096,12.802482392019));
#71113=CARTESIAN_POINT('Ctrl Pts',(0.227683409815427,2.32821798143634,12.8031562362659));
#71114=CARTESIAN_POINT('Ctrl Pts',(0.222038959348495,2.33371329069305,12.8036157023208));
#71115=CARTESIAN_POINT('Ctrl Pts',(0.204369407896036,2.34969731659983,12.8049828644614));
#71116=CARTESIAN_POINT('Ctrl Pts',(0.191761730137281,2.35950547936917,12.8058659995682));
#71117=CARTESIAN_POINT('Ctrl Pts',(0.159113850783497,2.3812203234735,12.8080621591748));
#71118=CARTESIAN_POINT('Ctrl Pts',(0.138414682339636,2.39196442846323,12.8093846654114));
#71119=CARTESIAN_POINT('Ctrl Pts',(0.115476022251753,2.40087922338813,12.8108787872511));
#71120=CARTESIAN_POINT('Ctrl Pts',(0.114207518094959,2.40136300619729,12.8109614754647));
#71121=CARTESIAN_POINT('Ctrl Pts',(0.112447548335094,2.40202151661007,12.8110763006425));
#71122=CARTESIAN_POINT('Ctrl Pts',(0.111958646062443,2.40220309261958,12.8111082086231));
#71123=CARTESIAN_POINT('Ctrl Pts',(0.11111817790777,2.40251291907921,12.8111630805358));
#71124=CARTESIAN_POINT('Ctrl Pts',(0.110766824357633,2.40264174578398,12.8111860252017));
#71125=CARTESIAN_POINT('Ctrl Pts',(0.110050769624072,2.40290287922451,12.8112327982012));
#71126=CARTESIAN_POINT('Ctrl Pts',(0.109686052389334,2.40303513995334,12.8112566280242));
#71127=CARTESIAN_POINT('Ctrl Pts',(0.108847916573885,2.403337369438,12.8113114049436));
#71128=CARTESIAN_POINT('Ctrl Pts',(0.108374338020282,2.40350688870952,12.8113423669312));
#71129=CARTESIAN_POINT('Ctrl Pts',(0.107376898992149,2.40386129368629,12.8114076020985));
#71130=CARTESIAN_POINT('Ctrl Pts',(0.106852953911956,2.40404593480588,12.8114418832977));
#71131=CARTESIAN_POINT('Ctrl Pts',(0.105463882693164,2.40453141713499,12.8115328066202));
#71132=CARTESIAN_POINT('Ctrl Pts',(0.10459795160515,2.40482992482228,12.8115895259406));
#71133=CARTESIAN_POINT('Ctrl Pts',(0.101989241599399,2.40571678668166,12.811760521371));
#71134=CARTESIAN_POINT('Ctrl Pts',(0.10024270933671,2.40629390797053,12.8118751669781));
#71135=CARTESIAN_POINT('Ctrl Pts',(0.094001901231711,2.40829701564943,12.8122854558636));
#71136=CARTESIAN_POINT('Ctrl Pts',(0.0894815617570456,2.40963923141877,
12.8125838071877));
#71137=CARTESIAN_POINT('Ctrl Pts',(0.0744645067125392,2.41374192445326,
12.8135791823806));
#71138=CARTESIAN_POINT('Ctrl Pts',(0.0638586331040312,2.41607118281746,
12.814289200609));
#71139=CARTESIAN_POINT('Ctrl Pts',(0.0218867343742071,2.42309020539783,
12.8171192816193));
#71140=CARTESIAN_POINT('Ctrl Pts',(-0.00998151255418595,2.42367674683068,
12.8193307300791));
#71141=CARTESIAN_POINT('Ctrl Pts',(-0.0429644068629143,2.4194020275151,
12.8214353089777));
#71142=CARTESIAN_POINT('Ctrl Pts',(-0.0445056485663049,2.41919091922345,
12.8215331775479));
#71143=CARTESIAN_POINT('Ctrl Pts',(-0.0464683924069918,2.41890758353654,
12.8216571529156));
#71144=CARTESIAN_POINT('Ctrl Pts',(-0.0468913281886851,2.4188456706241,
12.8216838283215));
#71145=CARTESIAN_POINT('Ctrl Pts',(-0.0475629123853623,2.41874599329277,
12.8217261230904));
#71146=CARTESIAN_POINT('Ctrl Pts',(-0.0478116400495858,2.4187087792195,
12.8217417735451));
#71147=CARTESIAN_POINT('Ctrl Pts',(-0.0482761745562963,2.41863872056923,
12.8217709768639));
#71148=CARTESIAN_POINT('Ctrl Pts',(-0.0484919899745699,2.41860594813111,
12.8217845336815));
#71149=CARTESIAN_POINT('Ctrl Pts',(-0.0489767604464773,2.41853182981651,
12.8218149617279));
#71150=CARTESIAN_POINT('Ctrl Pts',(-0.0492456958901408,2.41849036266061,
12.8218318259326));
#71151=CARTESIAN_POINT('Ctrl Pts',(-0.050042902983552,2.41836640739827,
12.8218817690664));
#71152=CARTESIAN_POINT('Ctrl Pts',(-0.050571025527687,2.41828294469779,
12.8219147927766));
#71153=CARTESIAN_POINT('Ctrl Pts',(-0.0547956660277045,2.41760451633553,
12.8221784831365));
#71154=CARTESIAN_POINT('Ctrl Pts',(-0.0584819597554197,2.41694645786921,
12.8224056411284));
#71155=CARTESIAN_POINT('Ctrl Pts',(-0.0730539263277228,2.41408223375931,
12.823294935386));
#71156=CARTESIAN_POINT('Ctrl Pts',(-0.0838347996316255,2.41137806557885,
12.8239337056198));
#71157=CARTESIAN_POINT('Ctrl Pts',(-0.106968868991532,2.40428627640394,
12.8253034929775));
#71158=CARTESIAN_POINT('Ctrl Pts',(-0.119237241687734,2.39969146119117,
12.8260296159695));
#71159=CARTESIAN_POINT('Ctrl Pts',(-0.150955892785231,2.38555502753493,
12.827976551957));
#71160=CARTESIAN_POINT('Ctrl Pts',(-0.16977897136329,2.37478038180383,12.8292092669971));
#71161=CARTESIAN_POINT('Ctrl Pts',(-0.187749355614054,2.36193808772033,
12.8305450328203));
#71162=CARTESIAN_POINT('Ctrl Pts',(-0.188118697275485,2.36167296013191,
12.8305725577014));
#71163=CARTESIAN_POINT('Ctrl Pts',(-0.189802615709957,2.36045877126188,
12.8306983774857));
#71164=CARTESIAN_POINT('Ctrl Pts',(-0.191110562103236,2.35950059221636,
12.8307970179876));
#71165=CARTESIAN_POINT('Ctrl Pts',(-0.192912258236908,2.35815969158861,
12.8309341887392));
#71166=CARTESIAN_POINT('Ctrl Pts',(-0.193412224332735,2.35778533164087,
12.8309723926039));
#71167=CARTESIAN_POINT('Ctrl Pts',(-0.194209892037314,2.35718443460567,
12.8310335693012));
#71168=CARTESIAN_POINT('Ctrl Pts',(-0.194508294691635,2.35695882717436,
12.8310565056299));
#71169=CARTESIAN_POINT('Ctrl Pts',(-0.195106552992748,2.35650487453366,
12.8311025918164));
#71170=CARTESIAN_POINT('Ctrl Pts',(-0.195406402230549,2.35627652183858,
12.8311257419479));
#71171=CARTESIAN_POINT('Ctrl Pts',(-0.196104018372711,2.35574331029572,
12.8311797227165));
#71172=CARTESIAN_POINT('Ctrl Pts',(-0.196501475301194,2.35543804920737,
12.8312105692095));
#71173=CARTESIAN_POINT('Ctrl Pts',(-0.197713610744413,2.35450258272397,
12.8313049244684));
#71174=CARTESIAN_POINT('Ctrl Pts',(-0.198525975564917,2.35386940239681,
12.8313685511082));
#71175=CARTESIAN_POINT('Ctrl Pts',(-0.200384007286858,2.35240682745984,
12.8315149837187));
#71176=CARTESIAN_POINT('Ctrl Pts',(-0.201427579727765,2.35157481384962,
12.8315978938301));
#71177=CARTESIAN_POINT('Ctrl Pts',(-0.204846174536465,2.3488143484801,12.831871715925));
#71178=CARTESIAN_POINT('Ctrl Pts',(-0.207198849779643,2.34685860496231,
12.8320637236145));
#71179=CARTESIAN_POINT('Ctrl Pts',(-0.216217053397281,2.33914216102917,
12.8328138924901));
#71180=CARTESIAN_POINT('Ctrl Pts',(-0.222672618073112,2.3331430229541,12.8333816911373));
#71181=CARTESIAN_POINT('Ctrl Pts',(-0.253019398119515,2.30253054713207,
12.8362062865143));
#71182=CARTESIAN_POINT('Ctrl Pts',(-0.273118277123958,2.27448031075107,
12.8386078568072));
#71183=CARTESIAN_POINT('Ctrl Pts',(-0.289939391013341,2.24074073929259,
12.8410281140105));
#71184=CARTESIAN_POINT('Ctrl Pts',(-0.291412559951727,2.23766455011192,
12.8412446440178));
#71185=CARTESIAN_POINT('Ctrl Pts',(-0.293073091696434,2.2340509570786,12.8414937203854));
#71186=CARTESIAN_POINT('Ctrl Pts',(-0.293308139926533,2.23353587995225,
12.8415290995131));
#71187=CARTESIAN_POINT('Ctrl Pts',(-0.29365679668629,2.23276648283692,12.8415817595171));
#71188=CARTESIAN_POINT('Ctrl Pts',(-0.293771433261199,2.23251263413729,
12.8415991033384));
#71189=CARTESIAN_POINT('Ctrl Pts',(-0.293975561531511,2.23205905023668,
12.8416300390852));
#71190=CARTESIAN_POINT('Ctrl Pts',(-0.294065178765829,2.23185937268792,
12.8416436387647));
#71191=CARTESIAN_POINT('Ctrl Pts',(-0.294255575961439,2.23143398624645,
12.8416725707188));
#71192=CARTESIAN_POINT('Ctrl Pts',(-0.294356299384256,2.23120825331823,
12.8416878994601));
#71193=CARTESIAN_POINT('Ctrl Pts',(-0.294627178125342,2.23059930070285,
12.8417291869347));
#71194=CARTESIAN_POINT('Ctrl Pts',(-0.29479684617357,2.23021586280102,12.8417551156541));
#71195=CARTESIAN_POINT('Ctrl Pts',(-0.295620889582056,2.22834371708293,
12.8418813837428));
#71196=CARTESIAN_POINT('Ctrl Pts',(-0.296264754027261,2.22685036796803,
12.8419810883679));
#71197=CARTESIAN_POINT('Ctrl Pts',(-0.299902736665034,2.21823378629403,
12.8425509168014));
#71198=CARTESIAN_POINT('Ctrl Pts',(-0.302651465175548,2.21100897009397,
12.8430073420929));
#71199=CARTESIAN_POINT('Ctrl Pts',(-0.316473043909679,2.17033562215885,
12.8454962606067));
#71200=CARTESIAN_POINT('Ctrl Pts',(-0.322262114102556,2.13534866200769,
12.8473676961822));
#71201=CARTESIAN_POINT('Ctrl Pts',(-0.322274978515416,2.10011767704999,
12.8494474689269));
#71202=CARTESIAN_POINT('Ctrl Pts',(-0.322274978630497,2.10011736146139,
12.8494474875569));
#71203=CARTESIAN_POINT('Ctrl Pts',(-0.322277157687331,2.09413366386358,
12.8498007202859));
#71204=CARTESIAN_POINT('Ctrl Pts',(-0.322112687808582,2.08815130524338,
12.8501585781565));
#71205=CARTESIAN_POINT('Ctrl Pts',(-0.321727601263438,2.08119876450792,
12.8505811569999));
#71206=CARTESIAN_POINT('Ctrl Pts',(-0.321668946773117,2.08022060365881,
12.8506407635404));
#71207=CARTESIAN_POINT('Ctrl Pts',(-0.321568342069809,2.07866186951974,
12.8507359989904));
#71208=CARTESIAN_POINT('Ctrl Pts',(-0.321529278176364,2.07808111083284,
12.8507715375699));
#71209=CARTESIAN_POINT('Ctrl Pts',(-0.321459594655213,2.07708542538063,
12.8508325631538));
#71210=CARTESIAN_POINT('Ctrl Pts',(-0.321429744388672,2.07667044480597,
12.8508580260017));
#71211=CARTESIAN_POINT('Ctrl Pts',(-0.321372111330502,2.07589033860108,
12.8509059470247));
#71212=CARTESIAN_POINT('Ctrl Pts',(-0.321344509635997,2.07552519992233,
12.8509283994817));
#71213=CARTESIAN_POINT('Ctrl Pts',(-0.321285723178165,2.07476476795226,
12.8509752056234));
#71214=CARTESIAN_POINT('Ctrl Pts',(-0.321254431084157,2.0743694837902,12.8509995626424));
#71215=CARTESIAN_POINT('Ctrl Pts',(-0.321180657881334,2.07345893885342,
12.8510557309639));
#71216=CARTESIAN_POINT('Ctrl Pts',(-0.321137666298163,2.07294372155164,
12.8510875582589));
#71217=CARTESIAN_POINT('Ctrl Pts',(-0.321019430216105,2.07156675677206,
12.8511727419246));
#71218=CARTESIAN_POINT('Ctrl Pts',(-0.320941956002435,2.07070520949559,
12.8512261682936));
#71219=CARTESIAN_POINT('Ctrl Pts',(-0.320379828768282,2.06472415556308,
12.8515979688614));
#71220=CARTESIAN_POINT('Ctrl Pts',(-0.319776194024506,2.05961682662829,
12.8519200698964));
#71221=CARTESIAN_POINT('Ctrl Pts',(-0.318737431477237,2.0523286962274,12.8523866777551));
#71222=CARTESIAN_POINT('Ctrl Pts',(-0.318401512203134,2.05013437991286,
12.8525280721608));
#71223=CARTESIAN_POINT('Ctrl Pts',(-0.312433322235896,2.01367111492903,
12.8548928874559));
#71224=CARTESIAN_POINT('Ctrl Pts',(-0.301320101473062,1.98053248647146,
12.8573024756047));
#71225=CARTESIAN_POINT('Ctrl Pts',(-0.28226851332567,1.94436033833722,12.8600043028669));
#71226=CARTESIAN_POINT('Ctrl Pts',(-0.279237977056343,1.93898639626217,
12.8604067311897));
#71227=CARTESIAN_POINT('Ctrl Pts',(-0.274566052596327,1.93123097769794,
12.8609855525643));
#71228=CARTESIAN_POINT('Ctrl Pts',(-0.273044059269899,1.92877954782531,
12.861168215415));
#71229=CARTESIAN_POINT('Ctrl Pts',(-0.271219685736593,1.92592729094785,
12.8613800891526));
#71230=CARTESIAN_POINT('Ctrl Pts',(-0.270949103052731,1.92550641980074,
12.8614113356884));
#71231=CARTESIAN_POINT('Ctrl Pts',(-0.270533758567627,1.92486367801339,
12.8614590263761));
#71232=CARTESIAN_POINT('Ctrl Pts',(-0.270389703072263,1.92464135528173,
12.8614755173072));
#71233=CARTESIAN_POINT('Ctrl Pts',(-0.270138213209825,1.92425427437457,
12.8615042199367));
#71234=CARTESIAN_POINT('Ctrl Pts',(-0.270030902462749,1.92408943741881,
12.8615164398667));
#71235=CARTESIAN_POINT('Ctrl Pts',(-0.269804772373784,1.92374277999112,
12.8615421324718));
#71236=CARTESIAN_POINT('Ctrl Pts',(-0.269685920506403,1.92356098197335,
12.8615556028591));
#71237=CARTESIAN_POINT('Ctrl Pts',(-0.269351525527247,1.92305061249473,
12.8615934091016));
#71238=CARTESIAN_POINT('Ctrl Pts',(-0.269135564180713,1.92272231347581,
12.861617716871));
#71239=CARTESIAN_POINT('Ctrl Pts',(-0.268248633699049,1.92137938019784,
12.8617171066464));
#71240=CARTESIAN_POINT('Ctrl Pts',(-0.267572511905333,1.92036813678199,
12.8617918472915));
#71241=CARTESIAN_POINT('Ctrl Pts',(-0.255645037439752,1.90274554798675,
12.8630930075478));
#71242=CARTESIAN_POINT('Ctrl Pts',(-0.242870450672732,1.88721393156759,
12.8642206172097));
#71243=CARTESIAN_POINT('Ctrl Pts',(-0.2173039605043,1.86145579718763,12.8662511534273));
#71244=CARTESIAN_POINT('Ctrl Pts',(-0.205022964154451,1.85082154520588,
12.8671528932526));
#71245=CARTESIAN_POINT('Ctrl Pts',(-0.184544572071718,1.8356318740856,12.8686159991174));
#71246=CARTESIAN_POINT('Ctrl Pts',(-0.176860460505816,1.83043078686845,
12.8691567479731));
#71247=CARTESIAN_POINT('Ctrl Pts',(-0.166366454361655,1.82396978826265,
12.8698914989739));
#71248=CARTESIAN_POINT('Ctrl Pts',(-0.163747198520407,1.82240798110385,
12.8700745758402));
#71249=CARTESIAN_POINT('Ctrl Pts',(-0.159953089300008,1.82021801769047,
12.8703395129879));
#71250=CARTESIAN_POINT('Ctrl Pts',(-0.158795839397795,1.81955957903782,
12.8704202877841));
#71251=CARTESIAN_POINT('Ctrl Pts',(-0.156737349697347,1.8184051900843,12.8705639241158));
#71252=CARTESIAN_POINT('Ctrl Pts',(-0.15583774805245,1.81790634532998,12.8706266813033));
#71253=CARTESIAN_POINT('Ctrl Pts',(-0.154496907438959,1.81717119714039,
12.870720203657));
#71254=CARTESIAN_POINT('Ctrl Pts',(-0.154057475223261,1.81693159756241,
12.8707508510653));
#71255=CARTESIAN_POINT('Ctrl Pts',(-0.153285996960608,1.81651327904887,
12.870804652661));
#71256=CARTESIAN_POINT('Ctrl Pts',(-0.152954191241553,1.81633411696238,
12.8708277910155));
#71257=CARTESIAN_POINT('Ctrl Pts',(-0.15229235410508,1.8159782496852,12.8708739419111));
#71258=CARTESIAN_POINT('Ctrl Pts',(-0.151962327679417,1.8158015363603,12.8708969541191));
#71259=CARTESIAN_POINT('Ctrl Pts',(-0.151171356612527,1.81537978096935,
12.8709521051751));
#71260=CARTESIAN_POINT('Ctrl Pts',(-0.15071012412062,1.81513528364581,12.8709842632768));
#71261=CARTESIAN_POINT('Ctrl Pts',(-0.14904455937368,1.8142575524176,12.8711003854084));
#71262=CARTESIAN_POINT('Ctrl Pts',(-0.14783682672451,1.8136308333598,12.8711845792833));
#71263=CARTESIAN_POINT('Ctrl Pts',(-0.12924950651635,1.80413438370041,12.8724803171443));
#71264=CARTESIAN_POINT('Ctrl Pts',(-0.111106876040193,1.7968549693569,12.8737485197718));
#71265=CARTESIAN_POINT('Ctrl Pts',(-0.0845216063084188,1.78889671070481,
12.8756042866134));
#71266=CARTESIAN_POINT('Ctrl Pts',(-0.0765351409159154,1.7868362678772,
12.8761608906105));
#71267=CARTESIAN_POINT('Ctrl Pts',(-0.0660581444609805,1.78455803493682,
12.8768862749059));
#71268=CARTESIAN_POINT('Ctrl Pts',(-0.0636315990035245,1.78405960787905,
12.87705393976));
#71269=CARTESIAN_POINT('Ctrl Pts',(-0.0583702570241278,1.78304196951893,
12.87741653011));
#71270=CARTESIAN_POINT('Ctrl Pts',(-0.0555337376611356,1.78253270384031,
12.8776114202096));
#71271=CARTESIAN_POINT('Ctrl Pts',(-0.0492488346375455,1.78149113023244,
12.8780415504108));
#71272=CARTESIAN_POINT('Ctrl Pts',(-0.0457978278428185,1.78097663492912,
12.8782766157209));
#71273=CARTESIAN_POINT('Ctrl Pts',(-0.0324390850201182,1.77920627642581,
12.87918091445));
#71274=CARTESIAN_POINT('Ctrl Pts',(-0.0224825201446892,1.77835504281546,
12.8798431302006));
#71275=CARTESIAN_POINT('Ctrl Pts',(-0.00871348195573289,1.77782051088361,
12.8807296079082));
#71276=CARTESIAN_POINT('Ctrl Pts',(-0.00492273681241625,1.77774029453169,
12.8809705905321));
#71277=CARTESIAN_POINT('Ctrl Pts',(-0.000595009464524741,1.77772510312494,
12.8812415387497));
#71278=CARTESIAN_POINT('Ctrl Pts',(-5.87514730183204E-5,1.77772455918855,
12.8812750394004));
#71279=CARTESIAN_POINT('Ctrl Pts',(0.000749948505829715,1.7777257574283,
12.8813254469954));
#71280=CARTESIAN_POINT('Ctrl Pts',(0.00102238764228161,1.77772650656197,
12.8813424092646));
#71281=CARTESIAN_POINT('Ctrl Pts',(0.00151113897232835,1.77772847026807,
12.8813728042586));
#71282=CARTESIAN_POINT('Ctrl Pts',(0.00172745041171609,1.77772955715307,
12.8813862441318));
#71283=CARTESIAN_POINT('Ctrl Pts',(0.002194282367126,1.77773237284469,12.8814152226764));
#71284=CARTESIAN_POINT('Ctrl Pts',(0.00244480127400739,1.77773417597397,
12.8814307570786));
#71285=CARTESIAN_POINT('Ctrl Pts',(0.00311858829100794,1.77773981133,12.8814724940126));
#71286=CARTESIAN_POINT('Ctrl Pts',(0.00354185321747487,1.77774418535084,
12.8814986661032));
#71287=CARTESIAN_POINT('Ctrl Pts',(0.00548104204343319,1.77776804597079,
12.881618365286));
#71288=CARTESIAN_POINT('Ctrl Pts',(0.00699685732786645,1.77779739569885,
12.8817113479611));
#71289=CARTESIAN_POINT('Ctrl Pts',(0.0398515981020691,1.77866551064822,
12.8837151565225));
#71290=CARTESIAN_POINT('Ctrl Pts',(0.0709081183332139,1.78406201212841,
12.8853935030414));
#71291=CARTESIAN_POINT('Ctrl Pts',(0.112837519840646,1.79785413207552,12.887891218246));
#71292=CARTESIAN_POINT('Ctrl Pts',(0.124725617504497,1.80256445550007,12.8886259628782));
#71293=CARTESIAN_POINT('Ctrl Pts',(0.139682723273527,1.80954547471785,12.8896051691714));
#71294=CARTESIAN_POINT('Ctrl Pts',(0.143035650505402,1.81118189909493,12.8898283401935));
#71295=CARTESIAN_POINT('Ctrl Pts',(0.147737075016866,1.81357841606296,12.8901468478925));
#71296=CARTESIAN_POINT('Ctrl Pts',(0.149109743929759,1.81429061755591,12.8902405253662));
#71297=CARTESIAN_POINT('Ctrl Pts',(0.151190517514351,1.81538929449036,12.8903835933802));
#71298=CARTESIAN_POINT('Ctrl Pts',(0.15190239764257,1.81576860157805,12.8904327315421));
#71299=CARTESIAN_POINT('Ctrl Pts',(0.15306179238086,1.81639195505095,12.8905130757969));
#71300=CARTESIAN_POINT('Ctrl Pts',(0.153510168181661,1.81663439921752,12.8905442250222));
#71301=CARTESIAN_POINT('Ctrl Pts',(0.154372654682901,1.81710340770834,12.8906042933358));
#71302=CARTESIAN_POINT('Ctrl Pts',(0.154786846765385,1.8173298202697,12.8906332069651));
#71303=CARTESIAN_POINT('Ctrl Pts',(0.155536841321006,1.81774193746432,12.8906856843163));
#71304=CARTESIAN_POINT('Ctrl Pts',(0.155872812971644,1.81792733374395,12.8907092369769));
#71305=CARTESIAN_POINT('Ctrl Pts',(0.156598171317104,1.8183292935229,12.8907601837709));
#71306=CARTESIAN_POINT('Ctrl Pts',(0.156987441225676,1.81854606515202,12.8907875853327));
#71307=CARTESIAN_POINT('Ctrl Pts',(0.158038841204687,1.81913441509601,12.8908617602436));
#71308=CARTESIAN_POINT('Ctrl Pts',(0.158700106669771,1.81950752551983,12.8909085886042));
#71309=CARTESIAN_POINT('Ctrl Pts',(0.161647746115612,1.82118445299271,12.8911181268885));
#71310=CARTESIAN_POINT('Ctrl Pts',(0.163919362967305,1.82251388348162,12.8912817597874));
#71311=CARTESIAN_POINT('Ctrl Pts',(0.166811989138186,1.8242546651879,12.8914929586836));
#71312=CARTESIAN_POINT('Ctrl Pts',(0.167448254239965,1.82464057755743,12.8915395919473));
#71313=CARTESIAN_POINT('Ctrl Pts',(0.168890448138891,1.82552215507232,12.8916456997064));
#71314=CARTESIAN_POINT('Ctrl Pts',(0.169695539466153,1.82601917095657,12.8917052230982));
#71315=CARTESIAN_POINT('Ctrl Pts',(0.171063780029292,1.82687218624442,12.8918068794288));
#71316=CARTESIAN_POINT('Ctrl Pts',(0.171628038678842,1.82722640191287,12.8918489472837));
#71317=CARTESIAN_POINT('Ctrl Pts',(0.173716281414955,1.82854634950647,12.8920051748721));
#71318=CARTESIAN_POINT('Ctrl Pts',(0.175233224067756,1.82952311047368,12.8921197327936));
#71319=CARTESIAN_POINT('Ctrl Pts',(0.200294103798603,1.84595915003484,12.8940302719698));
#71320=CARTESIAN_POINT('Ctrl Pts',(0.221716286517478,1.86442455988885,12.8959445343833));
#71321=CARTESIAN_POINT('Ctrl Pts',(0.243047976389121,1.88833057736983,12.8981054330911));
#71322=CARTESIAN_POINT('Ctrl Pts',(0.245581536936684,1.89127536535079,12.8983666593293));
#71323=CARTESIAN_POINT('Ctrl Pts',(0.255224790608973,1.90290256154339,12.8993772063056));
#71324=CARTESIAN_POINT('Ctrl Pts',(0.261933149392528,1.91190912712761,12.9001160680041));
#71325=CARTESIAN_POINT('Ctrl Pts',(0.2687264808695,1.92210030192945,12.9008908603931));
#71326=CARTESIAN_POINT('Ctrl Pts',(0.269290364576245,1.92295502349478,12.9009553889674));
#71327=CARTESIAN_POINT('Ctrl Pts',(0.270256311907252,1.92443447551816,12.9010662844528));
#71328=CARTESIAN_POINT('Ctrl Pts',(0.270660302836582,1.92505792956902,12.9011127740866));
#71329=CARTESIAN_POINT('Ctrl Pts',(0.271230516609302,1.92594460827455,12.9011785418412));
#71330=CARTESIAN_POINT('Ctrl Pts',(0.271398515562288,1.92620667941089,12.9011979372766));
#71331=CARTESIAN_POINT('Ctrl Pts',(0.27168666666379,1.92665761946614,12.9012312358004));
#71332=CARTESIAN_POINT('Ctrl Pts',(0.271807002015925,1.9268463705599,12.9012451511724));
#71333=CARTESIAN_POINT('Ctrl Pts',(0.272037289502212,1.92720841783902,12.9012717992586));
#71334=CARTESIAN_POINT('Ctrl Pts',(0.27214727258354,1.92738169340612,12.9012845340714));
#71335=CARTESIAN_POINT('Ctrl Pts',(0.272406299548407,1.9277906467436,12.9013145455612));
#71336=CARTESIAN_POINT('Ctrl Pts',(0.272555203505363,1.92802641358001,12.9013318128729));
#71337=CARTESIAN_POINT('Ctrl Pts',(0.272995129773377,1.92872497666683,12.9013828731749));
#71338=CARTESIAN_POINT('Ctrl Pts',(0.273285282561672,1.92918832345746,12.9014166087903));
#71339=CARTESIAN_POINT('Ctrl Pts',(0.275857892501965,1.9333198750419,12.9017162692713));
#71340=CARTESIAN_POINT('Ctrl Pts',(0.278067685846616,1.93703310936577,12.9019775225503));
#71341=CARTESIAN_POINT('Ctrl Pts',(0.28044889711628,1.94122392825339,12.9022647791911));
#71342=CARTESIAN_POINT('Ctrl Pts',(0.280694517744455,1.94165855701322,12.9022944806215));
#71343=CARTESIAN_POINT('Ctrl Pts',(0.294163787079987,1.96562242778806,12.903927265826));
#71344=CARTESIAN_POINT('Ctrl Pts',(0.304381950305955,1.99072201990376,12.90538805438));
#71345=CARTESIAN_POINT('Ctrl Pts',(0.315729411381623,2.03318887370769,12.9078708907702));
#71346=CARTESIAN_POINT('Ctrl Pts',(0.318806771259509,2.04989096725383,12.9088485122852));
#71347=CARTESIAN_POINT('Ctrl Pts',(0.320731476990113,2.06845011375563,12.9099731445066));
#71348=CARTESIAN_POINT('Ctrl Pts',(0.320893710396938,2.07014531675932,12.9100761964332));
#71349=CARTESIAN_POINT('Ctrl Pts',(0.321118124014856,2.07270393401074,12.9102322595821));
#71350=CARTESIAN_POINT('Ctrl Pts',(0.321190275055793,2.07356646115116,12.910284959171));
#71351=CARTESIAN_POINT('Ctrl Pts',(0.321301357494795,2.07496204964271,12.9103703771467));
#71352=CARTESIAN_POINT('Ctrl Pts',(0.32134243928868,2.07549493944714,12.9104030281167));
#71353=CARTESIAN_POINT('Ctrl Pts',(0.32141863229049,2.07651642280567,12.9104656841865));
#71354=CARTESIAN_POINT('Ctrl Pts',(0.321453955529854,2.07700499942695,12.9104956825531));
#71355=CARTESIAN_POINT('Ctrl Pts',(0.321515095938439,2.07787834939146,12.9105493599422));
#71356=CARTESIAN_POINT('Ctrl Pts',(0.32154133670542,2.07826309291672,12.9105730256186));
#71357=CARTESIAN_POINT('Ctrl Pts',(0.321592073877392,2.07902720418058,12.9106200639299));
#71358=CARTESIAN_POINT('Ctrl Pts',(0.321616589725816,2.07940657006584,12.9106434359165));
#71359=CARTESIAN_POINT('Ctrl Pts',(0.321674517098838,2.08032829581913,12.910700266758));
#71360=CARTESIAN_POINT('Ctrl Pts',(0.321707228177452,2.08087069711788,12.9107337475446));
#71361=CARTESIAN_POINT('Ctrl Pts',(0.321824814402479,2.08290611873595,12.9108595320774));
#71362=CARTESIAN_POINT('Ctrl Pts',(0.321900668006174,2.08439962314418,12.9109521183478));
#71363=CARTESIAN_POINT('Ctrl Pts',(0.323069003507011,2.11106581421381,12.9126105730301));
#71364=CARTESIAN_POINT('Ctrl Pts',(0.321215879903872,2.13627496294571,12.9142740319504));
#71365=CARTESIAN_POINT('Ctrl Pts',(0.313471287372211,2.17644765881876,12.9170373232934));
#71366=CARTESIAN_POINT('Ctrl Pts',(0.309367967216245,2.19165142605742,12.9181078675751));
#71367=CARTESIAN_POINT('Ctrl Pts',(0.302070279286985,2.21249503317324,12.9195691186867));
#71368=CARTESIAN_POINT('Ctrl Pts',(0.299792429553495,2.21843182278065,12.9199843751127));
#71369=CARTESIAN_POINT('Ctrl Pts',(0.296188326555408,2.22705342063701,12.9205822185144));
#71370=CARTESIAN_POINT('Ctrl Pts',(0.294998055359448,2.22979308681931,12.9207713987382));
#71371=CARTESIAN_POINT('Ctrl Pts',(0.293562153519512,2.2329762862353,12.9209899360706));
#71372=CARTESIAN_POINT('Ctrl Pts',(0.293353407372075,2.23343616103362,12.9210214767567));
#71373=CARTESIAN_POINT('Ctrl Pts',(0.293033102718043,2.23413741850574,12.9210695228396));
#71374=CARTESIAN_POINT('Ctrl Pts',(0.292922326263744,2.23437915429638,12.9210860760938));
#71375=CARTESIAN_POINT('Ctrl Pts',(0.292729050111147,2.23479954588023,12.9211148469356));
#71376=CARTESIAN_POINT('Ctrl Pts',(0.292646686195391,2.23497826272417,12.921127072887));
#71377=CARTESIAN_POINT('Ctrl Pts',(0.292459954606125,2.2353824667857,12.921154712731));
#71378=CARTESIAN_POINT('Ctrl Pts',(0.292355490042023,2.23560790834051,12.9211701204974));
#71379=CARTESIAN_POINT('Ctrl Pts',(0.29207161504631,2.23621867703564,12.9212118419233));
#71380=CARTESIAN_POINT('Ctrl Pts',(0.29189170206523,2.23660377212756,12.9212381244719));
#71381=CARTESIAN_POINT('Ctrl Pts',(0.29107934984364,2.23833364053522,12.9213560877753));
#71382=CARTESIAN_POINT('Ctrl Pts',(0.290438362544747,2.23967441344406,12.9214472474941));
#71383=CARTESIAN_POINT('Ctrl Pts',(0.275645797984994,2.27007429276252,12.9235090522467));
#71384=CARTESIAN_POINT('Ctrl Pts',(0.25720920743113,2.29685052668868,12.9252328109758));
#71385=CARTESIAN_POINT('Ctrl Pts',(0.229675995362771,2.3262140827988,12.9275162367858));
#71386=CARTESIAN_POINT('Ctrl Pts',(0.224049101353253,2.3317884015734,12.927970245729));
#71387=CARTESIAN_POINT('Ctrl Pts',(0.211991142975801,2.34288402396529,12.9289259451313));
#71388=CARTESIAN_POINT('Ctrl Pts',(0.20553625112613,2.34837013561412,12.929428390533));
#71389=CARTESIAN_POINT('Ctrl Pts',(0.197977583342984,2.354297753848,12.9300104017628));
#71390=CARTESIAN_POINT('Ctrl Pts',(0.197078240135899,2.35499536923611,12.9300795501089));
#71391=CARTESIAN_POINT('Ctrl Pts',(0.195662132064026,2.3560818696166,12.9301882834839));
#71392=CARTESIAN_POINT('Ctrl Pts',(0.195147854129657,2.35647399261758,12.9302277411017));
#71393=CARTESIAN_POINT('Ctrl Pts',(0.194279705206705,2.35713180975134,12.9302942999217));
#71394=CARTESIAN_POINT('Ctrl Pts',(0.193926459447994,2.35739832898465,12.9303213687203));
#71395=CARTESIAN_POINT('Ctrl Pts',(0.19323351400758,2.35791891096481,12.9303744421324));
#71396=CARTESIAN_POINT('Ctrl Pts',(0.192893859306704,2.35817303230204,12.9304004443816));
#71397=CARTESIAN_POINT('Ctrl Pts',(0.192245273869495,2.35865629364737,12.9304500739471));
#71398=CARTESIAN_POINT('Ctrl Pts',(0.191936432483957,2.35888555280634,12.930473696555));
#71399=CARTESIAN_POINT('Ctrl Pts',(0.191223781576466,2.35941259167593,12.9305281834365));
#71400=CARTESIAN_POINT('Ctrl Pts',(0.190819686370547,2.35970998180534,12.9305590627908));
#71401=CARTESIAN_POINT('Ctrl Pts',(0.189616597940501,2.36059105988883,12.9306509505075));
#71402=CARTESIAN_POINT('Ctrl Pts',(0.188815614676009,2.36117200908226,12.93071206475));
#71403=CARTESIAN_POINT('Ctrl Pts',(0.183243356321864,2.36517450873392,12.9311368122169));
#71404=CARTESIAN_POINT('Ctrl Pts',(0.178382299333618,2.3684686120969,12.9315053016902));
#71405=CARTESIAN_POINT('Ctrl Pts',(0.171725692425987,2.37271885039723,12.9320076557367));
#71406=CARTESIAN_POINT('Ctrl Pts',(0.170006928891879,2.37379358764576,12.9321371667537));
#71407=CARTESIAN_POINT('Ctrl Pts',(0.165321328749332,2.3766623467054,12.9324897059705));
#71408=CARTESIAN_POINT('Ctrl Pts',(0.162335556255635,2.37842478625113,12.9327137894189));
#71409=CARTESIAN_POINT('Ctrl Pts',(0.153310501969327,2.38355756523765,12.9333893952023));
#71410=CARTESIAN_POINT('Ctrl Pts',(0.147190819574099,2.3867818960783,12.9338452778013));
#71411=CARTESIAN_POINT('Ctrl Pts',(0.123092617714442,2.3985041314876,12.9356292427549));
#71412=CARTESIAN_POINT('Ctrl Pts',(0.104447471556289,2.40552769177142,12.9369892070315));
#71413=CARTESIAN_POINT('Ctrl Pts',(0.0742451370356756,2.4138146673319,12.9390857024458));
#71414=CARTESIAN_POINT('Ctrl Pts',(0.0630609392872428,2.41625205712724,
12.9398393956297));
#71415=CARTESIAN_POINT('Ctrl Pts',(0.050222332347642,2.4183415627825,12.9406623620609));
#71416=CARTESIAN_POINT('Ctrl Pts',(0.0486731518091858,2.41858210525885,
12.9407609709017));
#71417=CARTESIAN_POINT('Ctrl Pts',(0.0467126612951205,2.41887187759347,
12.9408848300887));
#71418=CARTESIAN_POINT('Ctrl Pts',(0.0463029627783074,2.41893162697948,
12.9409106625966));
#71419=CARTESIAN_POINT('Ctrl Pts',(0.0456496480063069,2.41902561931791,
12.9409517727443));
#71420=CARTESIAN_POINT('Ctrl Pts',(0.0454061074671507,2.41906037289192,
12.9409670792816));
#71421=CARTESIAN_POINT('Ctrl Pts',(0.0449456108270473,2.41912554847158,
12.9409959864923));
#71422=CARTESIAN_POINT('Ctrl Pts',(0.0447286652909905,2.41915602786332,
12.9410095902974));
#71423=CARTESIAN_POINT('Ctrl Pts',(0.0442338934213134,2.41922502559751,
12.9410405821166));
#71424=CARTESIAN_POINT('Ctrl Pts',(0.0439560482497025,2.41926340241036,
12.9410579619841));
#71425=CARTESIAN_POINT('Ctrl Pts',(0.043107552813163,2.41937947052273,12.9411109651706));
#71426=CARTESIAN_POINT('Ctrl Pts',(0.0425367401493403,2.41945599548373,
12.9411465226073));
#71427=CARTESIAN_POINT('Ctrl Pts',(0.0383914749090107,2.42000041541923,
12.9414040388614));
#71428=CARTESIAN_POINT('Ctrl Pts',(0.0348094222584036,2.42040985936664,
12.9416227722865));
#71429=CARTESIAN_POINT('Ctrl Pts',(0.000411766580830305,2.42375795348819,
12.9436933755305));
#71430=CARTESIAN_POINT('Ctrl Pts',(-0.0306731658353331,2.42230288530457,
12.945348481072));
#71431=CARTESIAN_POINT('Ctrl Pts',(-0.0753521971415159,2.41367913817677,
12.9479372907939));
#71432=CARTESIAN_POINT('Ctrl Pts',(-0.0894230777536805,2.40996126869124,
12.9487824051948));
#71433=CARTESIAN_POINT('Ctrl Pts',(-0.104672267532592,2.40480703306695,
12.9497538429676));
#71434=CARTESIAN_POINT('Ctrl Pts',(-0.106146999728627,2.40429660746455,
12.9498483677315));
#71435=CARTESIAN_POINT('Ctrl Pts',(-0.108728432369929,2.40338208841053,
12.9500148718208));
#71436=CARTESIAN_POINT('Ctrl Pts',(-0.10983674049928,2.402982596782,12.9500866983085));
#71437=CARTESIAN_POINT('Ctrl Pts',(-0.11144183488985,2.40239407327635,12.950191222956));
#71438=CARTESIAN_POINT('Ctrl Pts',(-0.111940392140116,2.40220987197385,
12.9502237599366));
#71439=CARTESIAN_POINT('Ctrl Pts',(-0.112810921385648,2.40188578895137,
12.9502806971259));
#71440=CARTESIAN_POINT('Ctrl Pts',(-0.113183095571158,2.40174645056622,
12.9503050791269));
#71441=CARTESIAN_POINT('Ctrl Pts',(-0.113902612477554,2.40147555199565,
12.9503522939031));
#71442=CARTESIAN_POINT('Ctrl Pts',(-0.114249987550027,2.40134407895846,
12.9503751237288));
#71443=CARTESIAN_POINT('Ctrl Pts',(-0.115074660855946,2.40103032919098,
12.9504294057162));
#71444=CARTESIAN_POINT('Ctrl Pts',(-0.115551753352763,2.40084751778309,
12.9504608757788));
#71445=CARTESIAN_POINT('Ctrl Pts',(-0.117235533185718,2.40019773407506,
12.9505721787253));
#71446=CARTESIAN_POINT('Ctrl Pts',(-0.118439828680841,2.39972463477145,
12.9506522173366));
#71447=CARTESIAN_POINT('Ctrl Pts',(-0.137719387956688,2.39201645069858,
12.9519405801952));
#71448=CARTESIAN_POINT('Ctrl Pts',(-0.155101938164828,2.38316669458161,
12.9532053397036));
#71449=CARTESIAN_POINT('Ctrl Pts',(-0.180657036723986,2.36709410512825,
12.9552235066925));
#71450=CARTESIAN_POINT('Ctrl Pts',(-0.189445653652415,2.3609340064727,12.9559495443048));
#71451=CARTESIAN_POINT('Ctrl Pts',(-0.206554494301615,2.34762143483849,
12.95741637958));
#71452=CARTESIAN_POINT('Ctrl Pts',(-0.214850421600092,2.34045883595795,
12.9581562309807));
#71453=CARTESIAN_POINT('Ctrl Pts',(-0.227332226951529,2.32851950677843,
12.9592992967429));
#71454=CARTESIAN_POINT('Ctrl Pts',(-0.231769493215158,2.32401789996387,
12.9597122005932));
#71455=CARTESIAN_POINT('Ctrl Pts',(-0.238154782776612,2.31714704163497,
12.9603126100037));
#71456=CARTESIAN_POINT('Ctrl Pts',(-0.240205834826079,2.31487600342673,
12.9605064820318));
#71457=CARTESIAN_POINT('Ctrl Pts',(-0.242559588025475,2.31219396841813,
12.9607298057502));
#71458=CARTESIAN_POINT('Ctrl Pts',(-0.242893955028742,2.31181114369888,
12.9607615505944));
#71459=CARTESIAN_POINT('Ctrl Pts',(-0.243402317259382,2.31122632092448,
12.9608098431944));
#71460=CARTESIAN_POINT('Ctrl Pts',(-0.2435769678993,2.31102489760392,12.9608264395624));
#71461=CARTESIAN_POINT('Ctrl Pts',(-0.243880143105038,2.31067436999814,
12.9608552577744));
#71462=CARTESIAN_POINT('Ctrl Pts',(-0.244008780667505,2.31052536505823,
12.9608674880737));
#71463=CARTESIAN_POINT('Ctrl Pts',(-0.244299150901746,2.31018839639859,
12.9608951012756));
#71464=CARTESIAN_POINT('Ctrl Pts',(-0.244460802874286,2.3100003642163,12.9609104781251));
#71465=CARTESIAN_POINT('Ctrl Pts',(-0.244897492637309,2.3094912229207,12.9609520297055));
#71466=CARTESIAN_POINT('Ctrl Pts',(-0.245172117019421,2.3091697574266,12.9609781737569));
#71467=CARTESIAN_POINT('Ctrl Pts',(-0.24639591699617,2.30773149944604,12.9610947426073));
#71468=CARTESIAN_POINT('Ctrl Pts',(-0.247338119466721,2.30660875737659,
12.961184661275));
#71469=CARTESIAN_POINT('Ctrl Pts',(-0.269052163456808,2.28037256063258,
12.9632620238983));
#71470=CARTESIAN_POINT('Ctrl Pts',(-0.285907091027176,2.25225412224008,
12.9649983267579));
#71471=CARTESIAN_POINT('Ctrl Pts',(-0.304652152001445,2.20645749369945,
12.9678073309816));
#71472=CARTESIAN_POINT('Ctrl Pts',(-0.309808454080694,2.19035888983947,
12.9687887190482));
#71473=CARTESIAN_POINT('Ctrl Pts',(-0.313949349887022,2.17278982378761,
12.9698861890681));
#71474=CARTESIAN_POINT('Ctrl Pts',(-0.314212316438326,2.1716461644679,12.9699577362798));
#71475=CARTESIAN_POINT('Ctrl Pts',(-0.314585112885802,2.16998331202528,
12.970061928334));
#71476=CARTESIAN_POINT('Ctrl Pts',(-0.314699918027856,2.16946523446546,
12.9700944134444));
#71477=CARTESIAN_POINT('Ctrl Pts',(-0.314898432643307,2.16855881098179,
12.9701512902924));
#71478=CARTESIAN_POINT('Ctrl Pts',(-0.314982704799778,2.16817058837342,
12.9701756639382));
#71479=CARTESIAN_POINT('Ctrl Pts',(-0.315144426671496,2.16741887043298,
12.9702228847172));
#71480=CARTESIAN_POINT('Ctrl Pts',(-0.315221965889312,2.16705539479896,
12.9702457289421));
#71481=CARTESIAN_POINT('Ctrl Pts',(-0.315404789360231,2.16619105996187,
12.9703000800952));
#71482=CARTESIAN_POINT('Ctrl Pts',(-0.315509509331421,2.16569008362661,
12.970331605031));
#71483=CARTESIAN_POINT('Ctrl Pts',(-0.315875818968115,2.16391658901139,
12.9704432867336));
#71484=CARTESIAN_POINT('Ctrl Pts',(-0.31613090436578,2.16264275365301,12.970523651071));
#71485=CARTESIAN_POINT('Ctrl Pts',(-0.32031961774128,2.14104794318442,12.9718886281106));
#71486=CARTESIAN_POINT('Ctrl Pts',(-0.322293545820142,2.12040010805891,
12.9732374354274));
#71487=CARTESIAN_POINT('Ctrl Pts',(-0.322249124175129,2.07118859678447,
12.9765363794684));
#71488=CARTESIAN_POINT('Ctrl Pts',(-0.318437719932902,2.04279737836198,
12.978511553746));
#71489=CARTESIAN_POINT('Ctrl Pts',(-0.310548662491574,2.01384366776017,
12.9804093387725));
#71490=CARTESIAN_POINT('Ctrl Pts',(-0.310147947802387,2.01241212391825,
12.9805028263917));
#71491=CARTESIAN_POINT('Ctrl Pts',(-0.30961991595704,2.01057481353525,12.9806223242202));
#71492=CARTESIAN_POINT('Ctrl Pts',(-0.309501689790216,2.01016648535517,
12.9806488505687));
#71493=CARTESIAN_POINT('Ctrl Pts',(-0.309313077612012,2.00951985087926,
12.9806908073958));
#71494=CARTESIAN_POINT('Ctrl Pts',(-0.309243223852495,2.00928139182592,
12.9807062688572));
#71495=CARTESIAN_POINT('Ctrl Pts',(-0.309117555490014,2.00885423083842,
12.980733945671));
#71496=CARTESIAN_POINT('Ctrl Pts',(-0.309061844247845,2.00866550061113,
12.9807461669712));
#71497=CARTESIAN_POINT('Ctrl Pts',(-0.308930448566064,2.00822187475915,
12.9807748777869));
#71498=CARTESIAN_POINT('Ctrl Pts',(-0.308854621623009,2.00796702206663,
12.9807913588126));
#71499=CARTESIAN_POINT('Ctrl Pts',(-0.30863387743126,2.00722845096755,12.9808390853883));
#71500=CARTESIAN_POINT('Ctrl Pts',(-0.308488137770651,2.00674497616145,
12.9808702828592));
#71501=CARTESIAN_POINT('Ctrl Pts',(-0.307472972036128,2.00340570121056,
12.9810854615992));
#71502=CARTESIAN_POINT('Ctrl Pts',(-0.306565002898372,2.00056163905591,
12.9812672283599));
#71503=CARTESIAN_POINT('Ctrl Pts',(-0.303600862136323,1.99170373464854,
12.9818298258549));
#71504=CARTESIAN_POINT('Ctrl Pts',(-0.301406146446895,1.98573753646431,
12.9822036480554));
#71505=CARTESIAN_POINT('Ctrl Pts',(-0.293176851667434,1.96525773677546,
12.9834815315278));
#71506=CARTESIAN_POINT('Ctrl Pts',(-0.286258289494841,1.95112286813672,
12.9843548423626));
#71507=CARTESIAN_POINT('Ctrl Pts',(-0.271043546283658,1.92505475481123,
12.9860425186791));
#71508=CARTESIAN_POINT('Ctrl Pts',(-0.262918938531272,1.91306676206004,
12.9868541882073));
#71509=CARTESIAN_POINT('Ctrl Pts',(-0.251820560382959,1.89885249283377,
12.9878975425398));
#71510=CARTESIAN_POINT('Ctrl Pts',(-0.249577527498403,1.89607606618043,
12.9881054378204));
#71511=CARTESIAN_POINT('Ctrl Pts',(-0.246053203866126,1.89185891868664,
12.9884280780931));
#71512=CARTESIAN_POINT('Ctrl Pts',(-0.244804290397781,1.8903914408968,12.9885416669482));
#71513=CARTESIAN_POINT('Ctrl Pts',(-0.243330301273887,1.88869064171508,
12.9886749145883));
#71514=CARTESIAN_POINT('Ctrl Pts',(-0.243117925104523,1.88844633090246,
12.988694093829));
#71515=CARTESIAN_POINT('Ctrl Pts',(-0.239174078828746,1.88392323701485,
12.9890498982305));
#71516=CARTESIAN_POINT('Ctrl Pts',(-0.235330747341237,1.87974369309926,
12.9893907650507));
#71517=CARTESIAN_POINT('Ctrl Pts',(-0.230697537289453,1.87496493401502,
12.9897959949599));
#71518=CARTESIAN_POINT('Ctrl Pts',(-0.230012669317467,1.87426496383031,
12.9898557536156));
#71519=CARTESIAN_POINT('Ctrl Pts',(-0.228973645729901,1.87321266629227,
12.98994620709));
#71520=CARTESIAN_POINT('Ctrl Pts',(-0.228621839496334,1.87285801869761,
12.9899767984544));
#71521=CARTESIAN_POINT('Ctrl Pts',(-0.227991863930262,1.87222590144169,
12.9900315154405));
#71522=CARTESIAN_POINT('Ctrl Pts',(-0.2277140084875,1.87194811921664,12.9900556271391));
#71523=CARTESIAN_POINT('Ctrl Pts',(-0.227126038454846,1.87136245005111,
12.9901066047036));
#71524=CARTESIAN_POINT('Ctrl Pts',(-0.226815804445384,1.87105468460433,
12.9901334758577));
#71525=CARTESIAN_POINT('Ctrl Pts',(-0.225992081899213,1.87024083405121,
12.9902047539913));
#71526=CARTESIAN_POINT('Ctrl Pts',(-0.225477521590444,1.86973584155897,
12.9902492088265));
#71527=CARTESIAN_POINT('Ctrl Pts',(-0.223112734651171,1.86743055300935,
12.9904531928106));
#71528=CARTESIAN_POINT('Ctrl Pts',(-0.221242654089342,1.86565084291849,
12.9906136150321));
#71529=CARTESIAN_POINT('Ctrl Pts',(-0.206970780108064,1.85239173962067,
12.9918315826369));
#71530=CARTESIAN_POINT('Ctrl Pts',(-0.193706656717891,1.84188311887711,
12.9929301518164));
#71531=CARTESIAN_POINT('Ctrl Pts',(-0.158133572766333,1.81799162650794,
12.9957880807951));
#71532=CARTESIAN_POINT('Ctrl Pts',(-0.134916896728148,1.8061763439686,12.9975807246286));
#71533=CARTESIAN_POINT('Ctrl Pts',(-0.105047958610657,1.79527024528794,
12.9996531220359));
#71534=CARTESIAN_POINT('Ctrl Pts',(-0.0995070351941245,1.79341614908757,
13.0000278981939));
#71535=CARTESIAN_POINT('Ctrl Pts',(-0.0932877754666285,1.79152147382515,
13.0004355599173));
#71536=CARTESIAN_POINT('Ctrl Pts',(-0.0926565991362059,1.79133130249855,
13.0004767848727));
#71537=CARTESIAN_POINT('Ctrl Pts',(-0.0917690824540835,1.79106686427661,
13.0005345410591));
#71538=CARTESIAN_POINT('Ctrl Pts',(-0.0915132320466128,1.79099097876599,
13.0005511661722));
#71539=CARTESIAN_POINT('Ctrl Pts',(-0.0910438998521653,1.79085240834202,
13.0005816177234));
#71540=CARTESIAN_POINT('Ctrl Pts',(-0.090830446945182,1.79078962656966,
13.000595449861));
#71541=CARTESIAN_POINT('Ctrl Pts',(-0.0903952048889321,1.7906621007059,
13.0006236189108));
#71542=CARTESIAN_POINT('Ctrl Pts',(-0.0901734110855543,1.79059737405672,
13.0006379547816));
#71543=CARTESIAN_POINT('Ctrl Pts',(-0.0896186778656303,1.79043613200863,
13.000673764191));
#71544=CARTESIAN_POINT('Ctrl Pts',(-0.0892856509545071,1.79033991486716,
13.0006952201981));
#71545=CARTESIAN_POINT('Ctrl Pts',(-0.0880185743581929,1.78997604887177,
13.0007766981902));
#71546=CARTESIAN_POINT('Ctrl Pts',(-0.0870834589533761,1.78971208380125,
13.0008365071011));
#71547=CARTESIAN_POINT('Ctrl Pts',(-0.0722725922572282,1.78560349065665,
13.0017789041796));
#71548=CARTESIAN_POINT('Ctrl Pts',(-0.0581536240978287,1.78268821968073,
13.0026097704631));
#71549=CARTESIAN_POINT('Ctrl Pts',(-0.00962500357097965,1.77601778957087,
13.0053814187414));
#71550=CARTESIAN_POINT('Ctrl Pts',(0.0251659925638299,1.7768533616894,13.007255240017));
#71551=CARTESIAN_POINT('Ctrl Pts',(0.0596921708261186,1.78330091048652,
13.0093791054892));
#71552=CARTESIAN_POINT('Ctrl Pts',(0.0602239513661011,1.78340160418447,
13.0094118750788));
#71553=CARTESIAN_POINT('Ctrl Pts',(0.0623020787287461,1.78380052697147,
13.0095401609234));
#71554=CARTESIAN_POINT('Ctrl Pts',(0.0638464653531769,1.78410874579652,
13.0096359893986));
#71555=CARTESIAN_POINT('Ctrl Pts',(0.0659926891035543,1.78455345727852,
13.0097698665948));
#71556=CARTESIAN_POINT('Ctrl Pts',(0.0665965042302619,1.78468038128589,
13.0098076092456));
#71557=CARTESIAN_POINT('Ctrl Pts',(0.0675643837474342,1.78488673699047,
13.0098682346868));
#71558=CARTESIAN_POINT('Ctrl Pts',(0.0679286833967781,1.784965067896,13.009891082185));
#71559=CARTESIAN_POINT('Ctrl Pts',(0.0686805442777158,1.78512809614003,
13.0099382957269));
#71560=CARTESIAN_POINT('Ctrl Pts',(0.0690680864777507,1.78521287759694,
13.0099626644334));
#71561=CARTESIAN_POINT('Ctrl Pts',(0.0699702577501759,1.78541198915028,
13.0100194698843));
#71562=CARTESIAN_POINT('Ctrl Pts',(0.0704847636873698,1.7855268666123,13.0100519241444));
#71563=CARTESIAN_POINT('Ctrl Pts',(0.072125463109162,1.78589742617481,13.010155604368));
#71564=CARTESIAN_POINT('Ctrl Pts',(0.0732505555630983,1.78615789739683,
13.0102269840148));
#71565=CARTESIAN_POINT('Ctrl Pts',(0.0991076464729995,1.7922907113338,13.0118740382368));
#71566=CARTESIAN_POINT('Ctrl Pts',(0.123054574328012,1.80106126766966,13.0135494222347));
#71567=CARTESIAN_POINT('Ctrl Pts',(0.16736542379948,1.82352390441864,13.0169037649004));
#71568=CARTESIAN_POINT('Ctrl Pts',(0.187705880118596,1.83690888636158,13.0185658893423));
#71569=CARTESIAN_POINT('Ctrl Pts',(0.207352651939784,1.85328609498175,13.0201806953776));
#71570=CARTESIAN_POINT('Ctrl Pts',(0.208348403318061,1.85412642238815,13.0202625486588));
#71571=CARTESIAN_POINT('Ctrl Pts',(0.209646100760314,1.85523511044956,13.0203692051224));
#71572=CARTESIAN_POINT('Ctrl Pts',(0.209952659244786,1.85549801718406,13.0203943995641));
#71573=CARTESIAN_POINT('Ctrl Pts',(0.210424996806164,1.85590464060243,13.0204332154082));
#71574=CARTESIAN_POINT('Ctrl Pts',(0.210591123280743,1.8560479502928,13.0204468667839));
#71575=CARTESIAN_POINT('Ctrl Pts',(0.210918949080065,1.85633133498288,13.0204738043281));
#71576=CARTESIAN_POINT('Ctrl Pts',(0.211080654183117,1.85647140040165,13.0204870909708));
#71577=CARTESIAN_POINT('Ctrl Pts',(0.211441372608775,1.85678447600533,13.020516728238));
#71578=CARTESIAN_POINT('Ctrl Pts',(0.211640312619265,1.8569575690578,13.020533072531));
#71579=CARTESIAN_POINT('Ctrl Pts',(0.21205436741509,1.85731872234266,13.020567088509));
#71580=CARTESIAN_POINT('Ctrl Pts',(0.212269445140151,1.85750682498965,13.0205847570259));
#71581=CARTESIAN_POINT('Ctrl Pts',(0.212825954481056,1.8579948445828,13.0206304726713));
#71582=CARTESIAN_POINT('Ctrl Pts',(0.213167003837131,1.85829519940583,13.020658487635));
#71583=CARTESIAN_POINT('Ctrl Pts',(0.224561970124997,1.86837337803091,13.0215945121563));
#71584=CARTESIAN_POINT('Ctrl Pts',(0.234933599784499,1.87889979022904,13.0224468577848));
#71585=CARTESIAN_POINT('Ctrl Pts',(0.267120230014987,1.91639977328706,13.0252436839158));
#71586=CARTESIAN_POINT('Ctrl Pts',(0.285300683463496,1.94616323829224,13.0271209049882));
#71587=CARTESIAN_POINT('Ctrl Pts',(0.298568623717848,1.97868154100987,13.0292446308518));
#71588=CARTESIAN_POINT('Ctrl Pts',(0.298743241807744,1.97911217169938,13.0292727608452));
#71589=CARTESIAN_POINT('Ctrl Pts',(0.299526950090914,1.98105696540774,13.029399829494));
#71590=CARTESIAN_POINT('Ctrl Pts',(0.300125455930805,1.9825753439068,13.0294991173425));
#71591=CARTESIAN_POINT('Ctrl Pts',(0.30093764020589,1.98468259193223,13.0296370451498));
#71592=CARTESIAN_POINT('Ctrl Pts',(0.301161180692527,1.98526765438069,13.0296753539547));
#71593=CARTESIAN_POINT('Ctrl Pts',(0.301515630680638,1.98620351378748,13.0297366561829));
#71594=CARTESIAN_POINT('Ctrl Pts',(0.301647637560282,1.98655389574145,13.0297596128241));
#71595=CARTESIAN_POINT('Ctrl Pts',(0.301917922662678,1.98727511259806,13.0298068774825));
#71596=CARTESIAN_POINT('Ctrl Pts',(0.302056128934785,1.987645973657,13.029831187859));
#71597=CARTESIAN_POINT('Ctrl Pts',(0.302374736552156,1.9885057583928,13.0298875624319));
#71598=CARTESIAN_POINT('Ctrl Pts',(0.302554635430714,1.98899486592571,13.0299196433303));
#71599=CARTESIAN_POINT('Ctrl Pts',(0.30311840131328,1.99053917949306,13.030020971847));
#71600=CARTESIAN_POINT('Ctrl Pts',(0.303497937196138,1.99159594792018,13.0300903634638));
#71601=CARTESIAN_POINT('Ctrl Pts',(0.309593301805848,2.00885063632491,13.0312242976386));
#71602=CARTESIAN_POINT('Ctrl Pts',(0.314009727309315,2.02547526623345,13.0323323605864));
#71603=CARTESIAN_POINT('Ctrl Pts',(0.32137831083781,2.06601739940995,13.0350684210968));
#71604=CARTESIAN_POINT('Ctrl Pts',(0.323017197557475,2.09006916548321,13.036722112365));
#71605=CARTESIAN_POINT('Ctrl Pts',(0.321562127936125,2.12334551864251,13.0389284858201));
#71606=CARTESIAN_POINT('Ctrl Pts',(0.320756973030407,2.13259167654339,13.0395317716445));
#71607=CARTESIAN_POINT('Ctrl Pts',(0.319460450137995,2.14250547530872,13.0401592455322));
#71608=CARTESIAN_POINT('Ctrl Pts',(0.31936463298086,2.14321950784399,13.0402043292886));
#71609=CARTESIAN_POINT('Ctrl Pts',(0.319227613661866,2.14421523878377,13.0402670408607));
#71610=CARTESIAN_POINT('Ctrl Pts',(0.319188432290649,2.14449720618567,13.0402847815427));
#71611=CARTESIAN_POINT('Ctrl Pts',(0.319120151431184,2.14498385617715,13.0403153692592));
#71612=CARTESIAN_POINT('Ctrl Pts',(0.319091228593618,2.14518856272546,13.0403282263105));
#71613=CARTESIAN_POINT('Ctrl Pts',(0.319031375842144,2.14560925849995,13.0403546293233));
#71614=CARTESIAN_POINT('Ctrl Pts',(0.319000423606129,2.14582524382913,13.0403681739195));
#71615=CARTESIAN_POINT('Ctrl Pts',(0.318927743830487,2.14632876273526,13.0403997252728));
#71616=CARTESIAN_POINT('Ctrl Pts',(0.318885846626649,2.14661627252607,13.0404177223624));
#71617=CARTESIAN_POINT('Ctrl Pts',(0.318795871370844,2.14722790901982,13.0404559694471));
#71618=CARTESIAN_POINT('Ctrl Pts',(0.318747687638349,2.14755202015559,13.0404762134612));
#71619=CARTESIAN_POINT('Ctrl Pts',(0.318389631266875,2.14993551231312,13.0406249179909));
#71620=CARTESIAN_POINT('Ctrl Pts',(0.318060288284193,2.15199198248878,13.0407522935955));
#71621=CARTESIAN_POINT('Ctrl Pts',(0.31704580974826,2.15795571543072,13.0411193639774));
#71622=CARTESIAN_POINT('Ctrl Pts',(0.316308420675292,2.16185383214356,13.041356397312));
#71623=CARTESIAN_POINT('Ctrl Pts',(0.314191428709977,2.17201407564945,13.0419689429184));
#71624=CARTESIAN_POINT('Ctrl Pts',(0.312696562473269,2.17825055860806,13.0423396617069));
#71625=CARTESIAN_POINT('Ctrl Pts',(0.303351382856004,2.21267207930778,13.0443766578996));
#71626=CARTESIAN_POINT('Ctrl Pts',(0.291877983769051,2.23972980150944,13.0459569635001));
#71627=CARTESIAN_POINT('Ctrl Pts',(0.272205973775907,2.27277051771961,13.0482002207271));
#71628=CARTESIAN_POINT('Ctrl Pts',(0.267165791214756,2.28046650503202,13.0487467697745));
#71629=CARTESIAN_POINT('Ctrl Pts',(0.261140278400599,2.28886033287967,13.0493751543312));
#71630=CARTESIAN_POINT('Ctrl Pts',(0.26047184975478,2.28978115230942,13.049444539783));
#71631=CARTESIAN_POINT('Ctrl Pts',(0.259491861186536,2.29111624279506,13.0495458071596));
#71632=CARTESIAN_POINT('Ctrl Pts',(0.259184150886062,2.29153333967397,13.0495775394843));
#71633=CARTESIAN_POINT('Ctrl Pts',(0.258639137334894,2.29226837926134,13.0496336299236));
#71634=CARTESIAN_POINT('Ctrl Pts',(0.258402250110441,2.29258663027518,13.049657971771));
#71635=CARTESIAN_POINT('Ctrl Pts',(0.257911098678903,2.29324394017619,13.0497083639958));
#71636=CARTESIAN_POINT('Ctrl Pts',(0.25765675223014,2.29358293639695,13.0497344175645));
#71637=CARTESIAN_POINT('Ctrl Pts',(0.257003486732051,2.29445004879544,13.0498012259781));
#71638=CARTESIAN_POINT('Ctrl Pts',(0.256603609579404,2.29497743769308,13.0498420184259));
#71639=CARTESIAN_POINT('Ctrl Pts',(0.254961455413181,2.29712943588291,13.0500091251482));
#71640=CARTESIAN_POINT('Ctrl Pts',(0.253705373227394,2.2987434062393,13.05013598401));
#71641=CARTESIAN_POINT('Ctrl Pts',(0.245297764176558,2.30933695088757,13.050978979991));
#71642=CARTESIAN_POINT('Ctrl Pts',(0.237686995280068,2.31793988026829,13.0517136454886));
#71643=CARTESIAN_POINT('Ctrl Pts',(0.226117038792136,2.32968977083719,13.0527928751491));
#71644=CARTESIAN_POINT('Ctrl Pts',(0.222517015211541,2.33317907383562,13.0531238879797));
#71645=CARTESIAN_POINT('Ctrl Pts',(0.215989808659054,2.33921668581548,13.0537152254305));
#71646=CARTESIAN_POINT('Ctrl Pts',(0.213095163819517,2.34179882160189,13.0539745505745));
#71647=CARTESIAN_POINT('Ctrl Pts',(0.189037202863037,2.36249187536752,13.0561046042451));
#71648=CARTESIAN_POINT('Ctrl Pts',(0.165653580067553,2.37784183739132,13.0580306229208));
#71649=CARTESIAN_POINT('Ctrl Pts',(0.13923296202041,2.3906503423667,13.0598877541481));
#71650=CARTESIAN_POINT('Ctrl Pts',(0.13787452510135,2.39129719320389,13.0599823840816));
#71651=CARTESIAN_POINT('Ctrl Pts',(0.13612472187324,2.39211541914222,13.0601031342494));
#71652=CARTESIAN_POINT('Ctrl Pts',(0.13573750496316,2.39229554864399,13.0601297837855));
#71653=CARTESIAN_POINT('Ctrl Pts',(0.135124028410765,2.39257944994594,13.0601718908743));
#71654=CARTESIAN_POINT('Ctrl Pts',(0.134898006370842,2.39268372941249,13.0601873797864));
#71655=CARTESIAN_POINT('Ctrl Pts',(0.134477180438365,2.39287729424834,13.0602161723535));
#71656=CARTESIAN_POINT('Ctrl Pts',(0.134282409826652,2.39296664649135,13.0602294800811));
#71657=CARTESIAN_POINT('Ctrl Pts',(0.133843739223327,2.39316736002346,13.0602594112364));
#71658=CARTESIAN_POINT('Ctrl Pts',(0.13359978982904,2.39327861100205,13.0602760277555));
#71659=CARTESIAN_POINT('Ctrl Pts',(0.133089981637661,2.39351033645654,13.0603106941993));
#71660=CARTESIAN_POINT('Ctrl Pts',(0.132824097254377,2.39363075453586,13.0603287406434));
#71661=CARTESIAN_POINT('Ctrl Pts',(0.13213041104132,2.39394378751114,13.0603757372296));
#71662=CARTESIAN_POINT('Ctrl Pts',(0.131702349649893,2.39413583059789,13.060404652653));
#71663=CARTESIAN_POINT('Ctrl Pts',(0.119676833351551,2.39949937643015,13.0612146219413));
#71664=CARTESIAN_POINT('Ctrl Pts',(0.107782593827991,2.40398259881624,13.061954587522));
#71665=CARTESIAN_POINT('Ctrl Pts',(0.0810885146029854,2.41227944893016,
13.0635473878274));
#71666=CARTESIAN_POINT('Ctrl Pts',(0.0662202957728761,2.41576685439528,
13.0643915437928));
#71667=CARTESIAN_POINT('Ctrl Pts',(0.0374926798737054,2.42038588545408,
13.0660233794245));
#71668=CARTESIAN_POINT('Ctrl Pts',(0.0236982847111115,2.42170042176613,
13.0668073465145));
#71669=CARTESIAN_POINT('Ctrl Pts',(0.00752525042455238,2.4221956182934,
13.0677531170686));
#71670=CARTESIAN_POINT('Ctrl Pts',(0.00518682861953486,2.42224174507862,
13.0678904882338));
#71671=CARTESIAN_POINT('Ctrl Pts',(-0.00369592262513817,2.42232025073422,
13.0684149756304));
#71672=CARTESIAN_POINT('Ctrl Pts',(-0.0102398503973064,2.4221787393623,
13.0688069065576));
#71673=CARTESIAN_POINT('Ctrl Pts',(-0.0178082853604414,2.42178426312994,
13.0692681569696));
#71674=CARTESIAN_POINT('Ctrl Pts',(-0.0188416918970045,2.42172540719195,
13.0693313078984));
#71675=CARTESIAN_POINT('Ctrl Pts',(-0.0203778996808845,2.42163048816571,
13.0694254450355));
#71676=CARTESIAN_POINT('Ctrl Pts',(-0.0208809358563081,2.42159822173998,
13.0694563120646));
#71677=CARTESIAN_POINT('Ctrl Pts',(-0.0217764564429814,2.42153867008201,
13.0695113372047));
#71678=CARTESIAN_POINT('Ctrl Pts',(-0.022168971350692,2.42151184600321,
13.0695354807913));
#71679=CARTESIAN_POINT('Ctrl Pts',(-0.022994866934573,2.42145388550823,
13.069586335824));
#71680=CARTESIAN_POINT('Ctrl Pts',(-0.0234282354308102,2.42142259129584,
13.0696130521795));
#71681=CARTESIAN_POINT('Ctrl Pts',(-0.024569400215618,2.42133786585075,
13.0696834862749));
#71682=CARTESIAN_POINT('Ctrl Pts',(-0.0252770826653947,2.4212829726822,
13.0697272498628));
#71683=CARTESIAN_POINT('Ctrl Pts',(-0.0284479557340132,2.42102647460799,
13.069923722583));
#71684=CARTESIAN_POINT('Ctrl Pts',(-0.0309089070949299,2.42079888169952,
13.0700772463377));
#71685=CARTESIAN_POINT('Ctrl Pts',(-0.0489494170054523,2.4189209537676,
13.0712105788909));
#71686=CARTESIAN_POINT('Ctrl Pts',(-0.0643904779587972,2.41616507799364,
13.0722254561884));
#71687=CARTESIAN_POINT('Ctrl Pts',(-0.0831988261291664,2.41137303779648,
13.0735151867658));
#71688=CARTESIAN_POINT('Ctrl Pts',(-0.0868130447873905,2.41038477320243,
13.0737654505094));
#71689=CARTESIAN_POINT('Ctrl Pts',(-0.0933253073564207,2.40848143073359,
13.0742204623408));
#71690=CARTESIAN_POINT('Ctrl Pts',(-0.0962292423951886,2.40758793631658,
13.0744248464411));
#71691=CARTESIAN_POINT('Ctrl Pts',(-0.101563104495609,2.40586386414598,
13.0748027669341));
#71692=CARTESIAN_POINT('Ctrl Pts',(-0.103996594101321,2.40504503902707,
13.0749761641162));
#71693=CARTESIAN_POINT('Ctrl Pts',(-0.108521069782248,2.40346220143024,
13.0753002119873));
#71694=CARTESIAN_POINT('Ctrl Pts',(-0.110614439152244,2.40270542791465,
13.0754508116235));
#71695=CARTESIAN_POINT('Ctrl Pts',(-0.119645622755248,2.39933437318651,
13.0761031457002));
#71696=CARTESIAN_POINT('Ctrl Pts',(-0.126500016020583,2.39650276754919,
13.0766050429809));
#71697=CARTESIAN_POINT('Ctrl Pts',(-0.138874699940913,2.39088338651718,
13.0775182043687));
#71698=CARTESIAN_POINT('Ctrl Pts',(-0.144424339008915,2.38816825601422,
13.0779304205303));
#71699=CARTESIAN_POINT('Ctrl Pts',(-0.156874990155226,2.38162674322147,
13.0788565722671));
#71700=CARTESIAN_POINT('Ctrl Pts',(-0.163720938351319,2.37770283371383,
13.0793667975492));
#71701=CARTESIAN_POINT('Ctrl Pts',(-0.171006442555565,2.37316378819657,
13.0799053443627));
#71702=CARTESIAN_POINT('Ctrl Pts',(-0.171595096575207,2.37279439405899,
13.0799488251424));
#71703=CARTESIAN_POINT('Ctrl Pts',(-0.172419496447772,2.37227333956213,
13.0800096680891));
#71704=CARTESIAN_POINT('Ctrl Pts',(-0.172656240965963,2.37212327472782,
13.0800271345362));
#71705=CARTESIAN_POINT('Ctrl Pts',(-0.17306630189056,2.3718625995746,13.0800573771307));
#71706=CARTESIAN_POINT('Ctrl Pts',(-0.173239708269755,2.37175213223945,
13.0800701627741));
#71707=CARTESIAN_POINT('Ctrl Pts',(-0.173597619048664,2.37152364584995,
13.0800965452616));
#71708=CARTESIAN_POINT('Ctrl Pts',(-0.173782108686184,2.37140560476137,
13.0801101405308));
#71709=CARTESIAN_POINT('Ctrl Pts',(-0.174219356500851,2.37112521404171,
13.0801423528991));
#71710=CARTESIAN_POINT('Ctrl Pts',(-0.17447200913164,2.37096269835543,13.0801609588961));
#71711=CARTESIAN_POINT('Ctrl Pts',(-0.175007529889489,2.3706171716893,13.0802003817718));
#71712=CARTESIAN_POINT('Ctrl Pts',(-0.175290339312197,2.3704340697423,13.0802211925941));
#71713=CARTESIAN_POINT('Ctrl Pts',(-0.177512649583516,2.36899030796666,
13.0803846612557));
#71714=CARTESIAN_POINT('Ctrl Pts',(-0.179438878520595,2.36770920071841,
13.0805259768813));
#71715=CARTESIAN_POINT('Ctrl Pts',(-0.18514383016156,2.36382567566688,13.0809439224431));
#71716=CARTESIAN_POINT('Ctrl Pts',(-0.188881096957397,2.36116309242474,
13.0812169308504));
#71717=CARTESIAN_POINT('Ctrl Pts',(-0.199613636422901,2.35316583721478,
13.082002646187));
#71718=CARTESIAN_POINT('Ctrl Pts',(-0.206449191695052,2.34762329498498,
13.0825052961444));
#71719=CARTESIAN_POINT('Ctrl Pts',(-0.235322493852153,2.32218385850991,
13.0846791304478));
#71720=CARTESIAN_POINT('Ctrl Pts',(-0.254775586508409,2.29957882845893,
13.0862954092033));
#71721=CARTESIAN_POINT('Ctrl Pts',(-0.27396503515206,2.26981508646467,13.0883945591642));
#71722=CARTESIAN_POINT('Ctrl Pts',(-0.276940596821328,2.26491786935097,
13.0887385133076));
#71723=CARTESIAN_POINT('Ctrl Pts',(-0.280271316338659,2.25909157531224,
13.0891470875488));
#71724=CARTESIAN_POINT('Ctrl Pts',(-0.280754813661814,2.25823676775569,
13.0892070152782));
#71725=CARTESIAN_POINT('Ctrl Pts',(-0.281478631721524,2.25694331986961,
13.0892976749819));
#71726=CARTESIAN_POINT('Ctrl Pts',(-0.281721853876238,2.25650630278552,
13.0893283027928));
#71727=CARTESIAN_POINT('Ctrl Pts',(-0.282154358259389,2.25572491181958,
13.0893830603583));
#71728=CARTESIAN_POINT('Ctrl Pts',(-0.282344030180213,2.25538075384489,
13.0894071761103));
#71729=CARTESIAN_POINT('Ctrl Pts',(-0.282743132988517,2.25465344173868,
13.0894581367137));
#71730=CARTESIAN_POINT('Ctrl Pts',(-0.282952415417319,2.25427020742936,
13.0894849868021));
#71731=CARTESIAN_POINT('Ctrl Pts',(-0.283504455339804,2.25325441930177,
13.0895561501296));
#71732=CARTESIAN_POINT('Ctrl Pts',(-0.283845873183109,2.2526211436746,13.0896005109494));
#71733=CARTESIAN_POINT('Ctrl Pts',(-0.285395452500939,2.24972373649537,
13.0898034570099));
#71734=CARTESIAN_POINT('Ctrl Pts',(-0.286578636452029,2.2474464177079,13.0899629242538));
#71735=CARTESIAN_POINT('Ctrl Pts',(-0.291608083572247,2.23747678057211,
13.0906610163535));
#71736=CARTESIAN_POINT('Ctrl Pts',(-0.295172457925456,2.22964697139591,
13.0912093481336));
#71737=CARTESIAN_POINT('Ctrl Pts',(-0.3019933835955,2.21291933277661,13.0923817145481));
#71738=CARTESIAN_POINT('Ctrl Pts',(-0.305179352762911,2.20400152927173,
13.0930072734632));
#71739=CARTESIAN_POINT('Ctrl Pts',(-0.313909921185657,2.17568623589384,
13.0949890632125));
#71740=CARTESIAN_POINT('Ctrl Pts',(-0.318029698806027,2.1559010431128,13.0963703576027));
#71741=CARTESIAN_POINT('Ctrl Pts',(-0.321389326753392,2.12589625912996,
13.0983782196975));
#71742=CARTESIAN_POINT('Ctrl Pts',(-0.322039543581381,2.1158837424051,13.099033317208));
#71743=CARTESIAN_POINT('Ctrl Pts',(-0.322239111835978,2.10490298855582,
13.0997243153652));
#71744=CARTESIAN_POINT('Ctrl Pts',(-0.322252206061614,2.10394971345929,
13.0997840758538));
#71745=CARTESIAN_POINT('Ctrl Pts',(-0.322264377247691,2.10264070082897,
13.0998658123331));
#71746=CARTESIAN_POINT('Ctrl Pts',(-0.322267095522565,2.10228501423813,
13.0998879889211));
#71747=CARTESIAN_POINT('Ctrl Pts',(-0.322270480605708,2.10171957818711,
13.0999231899422));
#71748=CARTESIAN_POINT('Ctrl Pts',(-0.322271531515003,2.10150983262813,
13.099936235948));
#71749=CARTESIAN_POINT('Ctrl Pts',(-0.322273226028635,2.1010897872172,13.0999623389437));
#71750=CARTESIAN_POINT('Ctrl Pts',(-0.322273868552071,2.10087948834564,
13.0999753957789));
#71751=CARTESIAN_POINT('Ctrl Pts',(-0.322274750300382,2.10045484734119,
13.1000017368163));
#71752=CARTESIAN_POINT('Ctrl Pts',(-0.322274981537786,2.10024050516953,
13.1000150205756));
#71753=CARTESIAN_POINT('Ctrl Pts',(-0.322274998938081,2.10002616218071,
13.100028292361));
#71754=CARTESIAN_POINT('Origin',(0.115470053837925,2.3,13.44));
#71755=CARTESIAN_POINT('',(0.115470053837925,2.3,13.44));
#71756=CARTESIAN_POINT('',(0.23094010767585,2.1,13.44));
#71757=CARTESIAN_POINT('',(0.144337567297406,2.25,13.44));
#71758=CARTESIAN_POINT('',(0.115470053837925,2.3,13.19));
#71759=CARTESIAN_POINT('',(0.115470053837925,2.3,13.44));
#71760=CARTESIAN_POINT('',(0.23094010767585,2.1,13.19));
#71761=CARTESIAN_POINT('',(0.23094010767585,2.1,13.19));
#71762=CARTESIAN_POINT('',(0.23094010767585,2.1,13.44));
#71763=CARTESIAN_POINT('Origin',(-0.115470053837925,2.3,13.44));
#71764=CARTESIAN_POINT('',(-0.115470053837925,2.3,13.44));
#71765=CARTESIAN_POINT('',(-0.0577350269189626,2.3,13.44));
#71766=CARTESIAN_POINT('',(-0.115470053837925,2.3,13.19));
#71767=CARTESIAN_POINT('',(-0.115470053837925,2.3,13.44));
#71768=CARTESIAN_POINT('',(0.115470053837925,2.3,13.19));
#71769=CARTESIAN_POINT('Origin',(-0.23094010767585,2.1,13.44));
#71770=CARTESIAN_POINT('',(-0.23094010767585,2.1,13.44));
#71771=CARTESIAN_POINT('',(-0.202072594216369,2.15,13.44));
#71772=CARTESIAN_POINT('',(-0.23094010767585,2.1,13.19));
#71773=CARTESIAN_POINT('',(-0.23094010767585,2.1,13.44));
#71774=CARTESIAN_POINT('',(-0.115470053837925,2.3,13.19));
#71775=CARTESIAN_POINT('Origin',(-0.115470053837925,1.9,13.44));
#71776=CARTESIAN_POINT('',(-0.115470053837925,1.9,13.44));
#71777=CARTESIAN_POINT('',(-0.144337567297407,1.95,13.44));
#71778=CARTESIAN_POINT('',(-0.115470053837925,1.9,13.19));
#71779=CARTESIAN_POINT('',(-0.115470053837925,1.9,13.44));
#71780=CARTESIAN_POINT('',(-0.23094010767585,2.1,13.19));
#71781=CARTESIAN_POINT('Origin',(0.115470053837925,1.9,13.44));
#71782=CARTESIAN_POINT('',(0.115470053837925,1.9,13.44));
#71783=CARTESIAN_POINT('',(0.0577350269189626,1.9,13.44));
#71784=CARTESIAN_POINT('',(0.115470053837925,1.9,13.19));
#71785=CARTESIAN_POINT('',(0.115470053837925,1.9,13.44));
#71786=CARTESIAN_POINT('',(-0.115470053837925,1.9,13.19));
#71787=CARTESIAN_POINT('Origin',(0.23094010767585,2.1,13.44));
#71788=CARTESIAN_POINT('',(0.202072594216369,2.05,13.44));
#71789=CARTESIAN_POINT('',(0.115470053837925,1.9,13.19));
#71790=CARTESIAN_POINT('Origin',(0.,2.1,13.19));
#71791=CARTESIAN_POINT('Origin',(5.160062080289E-17,2.1,13.3567));
#71792=CARTESIAN_POINT('Ctrl Pts',(0.384471428898087,2.18286501288884,13.3567));
#71793=CARTESIAN_POINT('Ctrl Pts',(0.382813073402951,2.18828203677418,13.3567));
#71794=CARTESIAN_POINT('Ctrl Pts',(0.381028861582513,2.19365655316686,13.3567));
#71795=CARTESIAN_POINT('Ctrl Pts',(0.379117390972968,2.19898452752087,13.3567));
#71796=CARTESIAN_POINT('Ctrl Pts',(0.374010021273159,2.21322065264946,13.3567));
#71797=CARTESIAN_POINT('Ctrl Pts',(0.367994822053367,2.22712503505139,13.3567));
#71798=CARTESIAN_POINT('Ctrl Pts',(0.361137622816578,2.24064162659447,13.3567));
#71799=CARTESIAN_POINT('Ctrl Pts',(0.356608893745571,2.24956844626943,13.3567));
#71800=CARTESIAN_POINT('Ctrl Pts',(0.351712673173096,2.25832598910903,13.3567));
#71801=CARTESIAN_POINT('Ctrl Pts',(0.346465850873052,2.26689606248918,13.3567));
#71802=CARTESIAN_POINT('Ctrl Pts',(0.343067268222326,2.27244725157844,13.3567));
#71803=CARTESIAN_POINT('Ctrl Pts',(0.33952652091561,2.27791158719777,13.3567));
#71804=CARTESIAN_POINT('Ctrl Pts',(0.335850140310723,2.28328316588372,13.3567));
#71805=CARTESIAN_POINT('Ctrl Pts',(0.326134074360472,2.29747936001562,13.3567));
#71806=CARTESIAN_POINT('Ctrl Pts',(0.315469319048827,2.31103259742725,13.3567));
#71807=CARTESIAN_POINT('Ctrl Pts',(0.30394745231302,2.32385415784788,13.3567));
#71808=CARTESIAN_POINT('Ctrl Pts',(0.298033748520208,2.33043494134658,13.3567));
#71809=CARTESIAN_POINT('Ctrl Pts',(0.291892742763497,2.33682398925588,13.3567));
#71810=CARTESIAN_POINT('Ctrl Pts',(0.285539140538778,2.34300405020489,13.3567));
#71811=CARTESIAN_POINT('Ctrl Pts',(0.280685518257919,2.34772510142249,13.3567));
#71812=CARTESIAN_POINT('Ctrl Pts',(0.275712527829575,2.35231944457806,13.3567));
#71813=CARTESIAN_POINT('Ctrl Pts',(0.270633354418833,2.35677538186565,13.3567));
#71814=CARTESIAN_POINT('Ctrl Pts',(0.2549882277151,2.37050078515682,13.3567));
#71815=CARTESIAN_POINT('Ctrl Pts',(0.238317569233452,2.38293578296153,13.3567));
#71816=CARTESIAN_POINT('Ctrl Pts',(0.220781169382088,2.393915845125,13.3567));
#71817=CARTESIAN_POINT('Ctrl Pts',(0.207902841162496,2.40197934992709,13.3567));
#71818=CARTESIAN_POINT('Ctrl Pts',(0.194556907819471,2.40925744118653,13.3567));
#71819=CARTESIAN_POINT('Ctrl Pts',(0.180802143098436,2.41566748709506,13.3567));
#71820=CARTESIAN_POINT('Ctrl Pts',(0.175631391396159,2.41807717976996,13.3567));
#71821=CARTESIAN_POINT('Ctrl Pts',(0.170402849726401,2.42036403435915,13.3567));
#71822=CARTESIAN_POINT('Ctrl Pts',(0.165119631550228,2.42252302855343,13.3567));
#71823=CARTESIAN_POINT('Ctrl Pts',(0.147547306967044,2.42970398256482,13.3567));
#71824=CARTESIAN_POINT('Ctrl Pts',(0.129505974814032,2.43541821356752,13.3567));
#71825=CARTESIAN_POINT('Ctrl Pts',(0.111120125345788,2.43952544314507,13.3567));
#71826=CARTESIAN_POINT('Ctrl Pts',(0.0910677364743285,2.44400496228916,
13.3567));
#71827=CARTESIAN_POINT('Ctrl Pts',(0.0706030552275727,2.44657367360852,
13.3567));
#71828=CARTESIAN_POINT('Ctrl Pts',(0.0499688774172958,2.44728614117711,
13.3567));
#71829=CARTESIAN_POINT('Ctrl Pts',(0.0444598928125659,2.44747635824817,
13.3567));
#71830=CARTESIAN_POINT('Ctrl Pts',(0.0389389090994037,2.44753396627794,
13.3567));
#71831=CARTESIAN_POINT('Ctrl Pts',(0.0334107967153799,2.44745938354123,
13.3567));
#71832=CARTESIAN_POINT('Ctrl Pts',(0.0262902260270452,2.44736331609326,
13.3567));
#71833=CARTESIAN_POINT('Ctrl Pts',(0.0191710656048495,2.44704789928713,
13.3567));
#71834=CARTESIAN_POINT('Ctrl Pts',(0.0120754035985885,2.44651741695667,
13.3567));
#71835=CARTESIAN_POINT('Ctrl Pts',(-0.00763403837127719,2.44504390952366,
13.3567));
#71836=CARTESIAN_POINT('Ctrl Pts',(-0.0271931972657536,2.44191427020158,
13.3567));
#71837=CARTESIAN_POINT('Ctrl Pts',(-0.0463836350019071,2.43718306921555,
13.3567));
#71838=CARTESIAN_POINT('Ctrl Pts',(-0.061026313137871,2.43357307062211,
13.3567));
#71839=CARTESIAN_POINT('Ctrl Pts',(-0.0754543432951754,2.4290295058022,
13.3567));
#71840=CARTESIAN_POINT('Ctrl Pts',(-0.0895595007323578,2.42355945091979,
13.3567));
#71841=CARTESIAN_POINT('Ctrl Pts',(-0.0955309797991314,2.42124367965883,
13.3567));
#71842=CARTESIAN_POINT('Ctrl Pts',(-0.101447746007056,2.41875987556956,
13.3567));
#71843=CARTESIAN_POINT('Ctrl Pts',(-0.107276888624383,2.41611965041911,
13.3567));
#71844=CARTESIAN_POINT('Ctrl Pts',(-0.124508298041685,2.4083149347846,13.3567));
#71845=CARTESIAN_POINT('Ctrl Pts',(-0.141018981529,2.39913172796346,13.3567));
#71846=CARTESIAN_POINT('Ctrl Pts',(-0.156604780393232,2.38860311667185,
13.3567));
#71847=CARTESIAN_POINT('Ctrl Pts',(-0.172190579257463,2.37807450538024,
13.3567));
#71848=CARTESIAN_POINT('Ctrl Pts',(-0.186852752521262,2.3661999008291,13.3567));
#71849=CARTESIAN_POINT('Ctrl Pts',(-0.200344699681301,2.35297855767097,
13.3567));
#71850=CARTESIAN_POINT('Ctrl Pts',(-0.201303803277869,2.35203869053215,
13.3567));
#71851=CARTESIAN_POINT('Ctrl Pts',(-0.202256970802107,2.35109200583289,
13.3567));
#71852=CARTESIAN_POINT('Ctrl Pts',(-0.20320410290731,2.35013849800987,13.3567));
#71853=CARTESIAN_POINT('',(-0.302891002292155,1.98913319379411,13.3568565029309));
#71854=CARTESIAN_POINT('Ctrl Pts',(-0.304247867982273,1.99372483614107,
13.3567));
#71855=CARTESIAN_POINT('Ctrl Pts',(-0.30372261333055,1.99222112067142,13.3567521676436));
#71856=CARTESIAN_POINT('Ctrl Pts',(-0.30318621052403,1.9907212993043,13.3568043352873));
#71857=CARTESIAN_POINT('Ctrl Pts',(-0.302638718523801,1.9892255368992,13.3568565029309));
#71858=CARTESIAN_POINT('Ctrl Pts',(-0.303133276678321,1.98898792129971,
13.3567));
#71859=CARTESIAN_POINT('Ctrl Pts',(-0.301503883177666,1.98230546808694,
13.3567));
#71860=CARTESIAN_POINT('Ctrl Pts',(-0.299648132848088,1.97568975965612,
13.3567));
#71861=CARTESIAN_POINT('Ctrl Pts',(-0.29756501457467,1.96915218281238,13.3567));
#71862=CARTESIAN_POINT('Ctrl Pts',(-0.293021738473608,1.95489374294745,
13.3567));
#71863=CARTESIAN_POINT('Ctrl Pts',(-0.287398567760631,1.94100671820594,
13.3567));
#71864=CARTESIAN_POINT('Ctrl Pts',(-0.280801429454096,1.92755158897031,
13.3567));
#71865=CARTESIAN_POINT('Ctrl Pts',(-0.27801701987579,1.92187267351028,13.3567));
#71866=CARTESIAN_POINT('Ctrl Pts',(-0.275058824312372,1.9162707242298,13.3567));
#71867=CARTESIAN_POINT('Ctrl Pts',(-0.271933633150864,1.91075051906705,
13.3567));
#71868=CARTESIAN_POINT('Ctrl Pts',(-0.263009465455726,1.89498724762603,
13.3567));
#71869=CARTESIAN_POINT('Ctrl Pts',(-0.252774512366312,1.87997443299183,
13.3567));
#71870=CARTESIAN_POINT('Ctrl Pts',(-0.241405887597271,1.86581594627798,
13.3567));
#71871=CARTESIAN_POINT('Ctrl Pts',(-0.235739092739989,1.85875851925168,
13.3567));
#71872=CARTESIAN_POINT('Ctrl Pts',(-0.229790133931066,1.85191365562157,
13.3567));
#71873=CARTESIAN_POINT('Ctrl Pts',(-0.223576577671086,1.84529462501086,
13.3567));
#71874=CARTESIAN_POINT('Ctrl Pts',(-0.218686560518433,1.84008550291298,
13.3567));
#71875=CARTESIAN_POINT('Ctrl Pts',(-0.213634883170243,1.83501929487925,
13.3567));
#71876=CARTESIAN_POINT('Ctrl Pts',(-0.208445611775876,1.8301160680278,13.3567));
#71877=CARTESIAN_POINT('Ctrl Pts',(-0.193804134551959,1.81628166261453,
13.3567));
#71878=CARTESIAN_POINT('Ctrl Pts',(-0.178042964881533,1.80371236102764,
13.3567));
#71879=CARTESIAN_POINT('Ctrl Pts',(-0.161369656581909,1.79254718173484,
13.3567));
#71880=CARTESIAN_POINT('Ctrl Pts',(-0.146268869163077,1.78243503146664,
13.3567));
#71881=CARTESIAN_POINT('Ctrl Pts',(-0.130418577424126,1.77347412276399,
13.3567));
#71882=CARTESIAN_POINT('Ctrl Pts',(-0.113944951420937,1.76579172141804,
13.3567));
#71883=CARTESIAN_POINT('Ctrl Pts',(-0.109408876626858,1.76367634335272,
13.3567));
#71884=CARTESIAN_POINT('Ctrl Pts',(-0.10482625753255,1.76165867681577,13.3567));
#71885=CARTESIAN_POINT('Ctrl Pts',(-0.100211858969317,1.75974617851619,
13.3567));
#71886=CARTESIAN_POINT('Ctrl Pts',(-0.0858955531262678,1.75381259687905,
13.3567));
#71887=CARTESIAN_POINT('Ctrl Pts',(-0.0712445325602557,1.74887619638116,
13.3567));
#71888=CARTESIAN_POINT('Ctrl Pts',(-0.0563443817491956,1.74500131412034,
13.3567));
#71889=CARTESIAN_POINT('Ctrl Pts',(-0.0413634792994686,1.74110543186455,
13.3567));
#71890=CARTESIAN_POINT('Ctrl Pts',(-0.0261304550998762,1.73828213073426,
13.3567));
#71891=CARTESIAN_POINT('Ctrl Pts',(-0.0107379526015333,1.73648531326028,
13.3567));
#71892=CARTESIAN_POINT('Ctrl Pts',(-0.00172422421978484,1.73543311108174,
13.3567));
#71893=CARTESIAN_POINT('Ctrl Pts',(0.00734332949099493,1.7347332825024,
13.3567));
#71894=CARTESIAN_POINT('Ctrl Pts',(0.0164505169552235,1.7343793481264,13.3567));
#71895=CARTESIAN_POINT('Ctrl Pts',(0.0228954295609135,1.73412887824968,
13.3567));
#71896=CARTESIAN_POINT('Ctrl Pts',(0.0293590259401381,1.73405213749439,
13.3567));
#71897=CARTESIAN_POINT('Ctrl Pts',(0.0358141150482056,1.73414609409592,
13.3567));
#71898=CARTESIAN_POINT('Ctrl Pts',(0.056425935663595,1.73444610802043,13.3567));
#71899=CARTESIAN_POINT('Ctrl Pts',(0.07698675111472,1.73647959996866,13.3567));
#71900=CARTESIAN_POINT('Ctrl Pts',(0.097287927881851,1.74013888126268,13.3567));
#71901=CARTESIAN_POINT('Ctrl Pts',(0.118088935260064,1.74388825688109,13.3567));
#71902=CARTESIAN_POINT('Ctrl Pts',(0.138618827654593,1.74934446475836,13.3567));
#71903=CARTESIAN_POINT('Ctrl Pts',(0.15865913407629,1.75644449140174,13.3567));
#71904=CARTESIAN_POINT('Ctrl Pts',(0.161079921109755,1.75730214557497,13.3567));
#71905=CARTESIAN_POINT('Ctrl Pts',(0.163493555065397,1.75818384755897,13.3567));
#71906=CARTESIAN_POINT('Ctrl Pts',(0.165899639879492,1.75908953676982,13.3567));
#71907=CARTESIAN_POINT('Ctrl Pts',(0.170720645667814,1.76090424126501,13.3567));
#71908=CARTESIAN_POINT('Ctrl Pts',(0.175502848112081,1.76281206603697,13.3567));
#71909=CARTESIAN_POINT('Ctrl Pts',(0.180241540932178,1.76481078791832,13.3567));
#71910=CARTESIAN_POINT('Ctrl Pts',(0.200489840282318,1.77335126954643,13.3567));
#71911=CARTESIAN_POINT('Ctrl Pts',(0.219954281019108,1.78355100246641,13.3567));
#71912=CARTESIAN_POINT('Ctrl Pts',(0.238403113750705,1.79532081160773,13.3567));
#71913=CARTESIAN_POINT('Ctrl Pts',(0.256851946482301,1.80709062074905,13.3567));
#71914=CARTESIAN_POINT('Ctrl Pts',(0.274286879817491,1.82043079606709,13.3567));
#71915=CARTESIAN_POINT('Ctrl Pts',(0.29045854394972,1.83530356379869,13.3567));
#71916=CARTESIAN_POINT('Ctrl Pts',(0.291364097891721,1.83613638430113,13.3567));
#71917=CARTESIAN_POINT('Ctrl Pts',(0.292265682104844,1.83697402310408,13.3567));
#71918=CARTESIAN_POINT('Ctrl Pts',(0.29316324943837,1.83781647805643,13.3567));
#71919=CARTESIAN_POINT('Ctrl Pts',(0.315794730921881,2.16133333943205,4.3153592086915));
#71920=CARTESIAN_POINT('Ctrl Pts',(0.295374973081064,2.26647113223029,4.32198265653243));
#71921=CARTESIAN_POINT('Ctrl Pts',(0.141593364461128,2.45291664246826,4.33522955221429));
#71922=CARTESIAN_POINT('Ctrl Pts',(-0.220800772831429,2.41004672910968,
4.35509989573707));
#71923=CARTESIAN_POINT('Ctrl Pts',(-0.379865078018474,2.08219540995681,
4.37497023925986));
#71924=CARTESIAN_POINT('Ctrl Pts',(-0.190837952383979,1.77095809589613,
4.39484058278266));
#71925=CARTESIAN_POINT('Ctrl Pts',(0.173453834391319,1.76142701812932,4.41471092630544));
#71926=CARTESIAN_POINT('Ctrl Pts',(0.378523374757362,2.06256570849522,4.43458126982823));
#71927=CARTESIAN_POINT('Ctrl Pts',(0.236402166296634,2.39800625800675,4.45445161335102));
#71928=CARTESIAN_POINT('Ctrl Pts',(-0.122613317153847,2.46008688645899,
4.47432195687381));
#71929=CARTESIAN_POINT('Ctrl Pts',(-0.369133512413124,2.19182630426626,
4.4941923003966));
#71930=CARTESIAN_POINT('Ctrl Pts',(-0.277031367561046,1.83933304745027,
4.51406264391939));
#71931=CARTESIAN_POINT('Ctrl Pts',(0.06921318690911,1.72596339903695,4.53393298744218));
#71932=CARTESIAN_POINT('Ctrl Pts',(0.351962069027787,1.95572288286177,4.55380333096497));
#71933=CARTESIAN_POINT('Ctrl Pts',(0.311834704349932,2.31783621621276,4.57367367448776));
#71934=CARTESIAN_POINT('Ctrl Pts',(-0.0143590870975264,2.4801148735102,
4.59354401801055));
#71935=CARTESIAN_POINT('Ctrl Pts',(-0.327380091631696,2.29368967642256,
4.61341436153334));
#71936=CARTESIAN_POINT('Ctrl Pts',(-0.340074575883644,1.92958067658856,
4.63328470505612));
#71937=CARTESIAN_POINT('Ctrl Pts',(-0.0407968584462133,1.72180814998663,
4.65315504857892));
#71938=CARTESIAN_POINT('Ctrl Pts',(0.295906383536178,1.86097518841639,4.67302539210171));
#71939=CARTESIAN_POINT('Ctrl Pts',(0.361155822934746,2.21941493622384,4.6928957356245));
#71940=CARTESIAN_POINT('Ctrl Pts',(0.0950939511799071,2.46830774468873,
4.71276607914728));
#71941=CARTESIAN_POINT('Ctrl Pts',(-0.25820366943978,2.37932833394089,4.73263642267008));
#71942=CARTESIAN_POINT('Ctrl Pts',(-0.37463457744399,2.03410320601478,4.75250676619286));
#71943=CARTESIAN_POINT('Ctrl Pts',(-0.147389261061116,1.7493294144447,4.77237710971565));
#71944=CARTESIAN_POINT('Ctrl Pts',(0.215065636343779,1.78624814619657,4.79224745323845));
#71945=CARTESIAN_POINT('Ctrl Pts',(0.380227091343265,2.11099149006219,4.81211779676122));
#71946=CARTESIAN_POINT('Ctrl Pts',(0.196581953073257,2.42565163830413,4.83198814028403));
#71947=CARTESIAN_POINT('Ctrl Pts',(-0.167400364818031,2.44157074179032,
4.85185848380681));
#71948=CARTESIAN_POINT('Ctrl Pts',(-0.37781563754619,2.14414519038242,4.8717288273296));
#71949=CARTESIAN_POINT('Ctrl Pts',(-0.241636497751353,1.80622243660235,
4.89159917085239));
#71950=CARTESIAN_POINT('Ctrl Pts',(0.11621123287666,1.73780060304687,4.91146951437518));
#71951=CARTESIAN_POINT('Ctrl Pts',(0.367450978078876,2.00164740719483,4.93133985789797));
#71952=CARTESIAN_POINT('Ctrl Pts',(0.281604474823222,2.35571932574806,4.95121020142075));
#71953=CARTESIAN_POINT('Ctrl Pts',(-0.0625757970931978,2.47520357596851,
4.97108054494355));
#71954=CARTESIAN_POINT('Ctrl Pts',(-0.349351294103218,2.25048962459309,
4.99095088846634));
#71955=CARTESIAN_POINT('Ctrl Pts',(-0.315644538657038,1.8877219299655,5.01082123198912));
#71956=CARTESIAN_POINT('Ctrl Pts',(0.00762310988300606,1.7196904655451,
5.03069157551192));
#71957=CARTESIAN_POINT('Ctrl Pts',(0.323897592898241,1.90054122451905,5.0505619190347));
#71958=CARTESIAN_POINT('Ctrl Pts',(0.343040129104818,2.26436825613651,5.0704322625575));
#71959=CARTESIAN_POINT('Ctrl Pts',(0.0474900475543018,2.47740978946618,
5.09030260608028));
#71960=CARTESIAN_POINT('Ctrl Pts',(-0.291625687441136,2.34422922066392,
5.11017294960308));
#71961=CARTESIAN_POINT('Ctrl Pts',(-0.363214555461668,1.98700159070856,
5.13004329312585));
#71962=CARTESIAN_POINT('Ctrl Pts',(-0.101603516042804,1.73343461793378,
5.14991363664866));
#71963=CARTESIAN_POINT('Ctrl Pts',(0.253214917275652,1.81614147983423,5.16978398017144));
#71964=CARTESIAN_POINT('Ctrl Pts',(0.375743136091877,2.15924989013876,5.18965432369423));
#71965=CARTESIAN_POINT('Ctrl Pts',(0.153578180352721,2.44800459238517,5.20952466721702));
#71966=CARTESIAN_POINT('Ctrl Pts',(-0.209473848078761,2.41751245766535,
5.22939501073981));
#71967=CARTESIAN_POINT('Ctrl Pts',(-0.380362138187303,2.09574586845546,
5.24926535426261));
#71968=CARTESIAN_POINT('Ctrl Pts',(-0.202319948138264,1.77788186578998,
5.26913569778539));
#71969=CARTESIAN_POINT('Ctrl Pts',(0.16132325095384,1.75551739883805,5.28900604130818));
#71970=CARTESIAN_POINT('Ctrl Pts',(0.376974329473245,2.04916882138084,5.30887638483097));
#71971=CARTESIAN_POINT('Ctrl Pts',(0.246802781121706,2.38945093026661,5.32874672835376));
#71972=CARTESIAN_POINT('Ctrl Pts',(-0.109776719744329,2.46420121581866,
5.34861707187654));
#71973=CARTESIAN_POINT('Ctrl Pts',(-0.365651024995835,2.20484646737545,
5.36848741539934));
#71974=CARTESIAN_POINT('Ctrl Pts',(-0.286090293705716,1.8493093586729,5.38835775892213));
#71975=CARTESIAN_POINT('Ctrl Pts',(0.0559193343828591,1.72374678493893,
5.40822810244491));
#71976=CARTESIAN_POINT('Ctrl Pts',(0.346630585905113,1.94334531377359,5.4280984459677));
#71977=CARTESIAN_POINT('Ctrl Pts',(0.319355464352517,2.30665319061123,5.4479687894905));
#71978=CARTESIAN_POINT('Ctrl Pts',(-0.000884819422922472,2.48038489835456,
5.46783913301329));
#71979=CARTESIAN_POINT('Ctrl Pts',(-0.320313401835117,2.30516524658536,
5.48770947653607));
#71980=CARTESIAN_POINT('Ctrl Pts',(-0.345898044795595,1.94173441180029,
5.50757982005887));
#71981=CARTESIAN_POINT('Ctrl Pts',(-0.0541683214227408,1.7234907082742,
5.52745016358165));
#71982=CARTESIAN_POINT('Ctrl Pts',(0.287253462504416,1.85064302279496,5.54732050710444));
#71983=CARTESIAN_POINT('Ctrl Pts',(0.365159300611444,2.20654641701426,5.56719085062723));
#71984=CARTESIAN_POINT('Ctrl Pts',(0.108081192357295,2.46470797860787,5.58706119415001));
#71985=CARTESIAN_POINT('Ctrl Pts',(-0.248146695958989,2.38829962033665,
5.60693153767281));
#71986=CARTESIAN_POINT('Ctrl Pts',(-0.376733772855055,2.04741560885575,
5.6268018811956));
#71987=CARTESIAN_POINT('Ctrl Pts',(-0.15971890082854,1.75477061753128,5.64667222471839));
#71988=CARTESIAN_POINT('Ctrl Pts',(0.203816318943259,1.77882658588539,5.66654256824118));
#71989=CARTESIAN_POINT('Ctrl Pts',(0.380377813170898,2.09751543787756,5.68641291176396));
#71990=CARTESIAN_POINT('Ctrl Pts',(0.207994447577465,2.41848353737448,5.70628325528676));
#71991=CARTESIAN_POINT('Ctrl Pts',(-0.155195507781162,2.44728634894876,
5.72615359880955));
#71992=CARTESIAN_POINT('Ctrl Pts',(-0.376014712711115,2.15750121412973,
5.74602394233233));
#71993=CARTESIAN_POINT('Ctrl Pts',(-0.251891608509355,1.8149665434301,5.76589428585512));
#71994=CARTESIAN_POINT('Ctrl Pts',(0.10330775455378,1.7339112653322,5.78576462937792));
#71995=CARTESIAN_POINT('Ctrl Pts',(0.363736316894626,1.98869256281116,5.8056349729007));
#71996=CARTESIAN_POINT('Ctrl Pts',(0.290486326712738,2.34558328077163,5.8255053164235));
#71997=CARTESIAN_POINT('Ctrl Pts',(-0.0492453220856943,2.47718477176881,
5.84537565994628));
#71998=CARTESIAN_POINT('Ctrl Pts',(-0.343801092015725,2.262770583738,5.86524600346907));
#71999=CARTESIAN_POINT('Ctrl Pts',(-0.32296616431361,1.89903654434159,5.88511634699187));
#72000=CARTESIAN_POINT('Ctrl Pts',(-0.00585374872675999,1.71965911680776,
5.90498669051464));
#72001=CARTESIAN_POINT('Ctrl Pts',(0.316628684400964,1.88919267086714,5.92485703403744));
#72002=CARTESIAN_POINT('Ctrl Pts',(0.348647404693823,2.25211325057955,5.94472737756023));
#72003=CARTESIAN_POINT('Ctrl Pts',(0.0608295952382777,2.47549063123434,
5.96459772108302));
#72004=CARTESIAN_POINT('Ctrl Pts',(-0.282791086646785,2.3544064761651,5.9844680646058));
#72005=CARTESIAN_POINT('Ctrl Pts',(-0.366989445063476,1.99993901352867,
6.0043384081286));
#72006=CARTESIAN_POINT('Ctrl Pts',(-0.114524948735923,1.73726388390642,
6.02420875165139));
#72007=CARTESIAN_POINT('Ctrl Pts',(0.243000596892941,1.807349758737,6.04407909517418));
#72008=CARTESIAN_POINT('Ctrl Pts',(0.377606176416558,2.14590238919362,6.06394943869696));
#72009=CARTESIAN_POINT('Ctrl Pts',(0.165809495516936,2.4423458266111,6.08381978221975));
#72010=CARTESIAN_POINT('Ctrl Pts',(-0.19809482459498,2.42473357428868,6.10369012574255));
#72011=CARTESIAN_POINT('Ctrl Pts',(-0.380274111316162,2.10922247604054,
6.12356046926533));
#72012=CARTESIAN_POINT('Ctrl Pts',(-0.213603670550259,1.78525101155195,
6.14343081278812));
#72013=CARTESIAN_POINT('Ctrl Pts',(0.149019058431623,1.75001889475892,6.16330115631092));
#72014=CARTESIAN_POINT('Ctrl Pts',(0.374937088415383,2.03584679639947,6.1831714998337));
#72015=CARTESIAN_POINT('Ctrl Pts',(0.256901382853463,2.38052652867348,6.2030418433565));
#72016=CARTESIAN_POINT('Ctrl Pts',(-0.0968063675113594,2.46786136112791,
6.22291218687928));
#72017=CARTESIAN_POINT('Ctrl Pts',(-0.36170745468139,2.21773347454961,6.24278253040208));
#72018=CARTESIAN_POINT('Ctrl Pts',(-0.294791194204682,1.85960115303731,
6.26265287392485));
#72019=CARTESIAN_POINT('Ctrl Pts',(0.042555854757641,1.72200204626551,6.28252321744766));
#72020=CARTESIAN_POINT('Ctrl Pts',(0.340863700436308,1.9311646022705,6.30239356097044));
#72021=CARTESIAN_POINT('Ctrl Pts',(0.326475505367192,2.29521065082841,6.32226390449323));
#72022=CARTESIAN_POINT('Ctrl Pts',(0.0125904797503218,2.48017750278163,
6.34213424801602));
#72023=CARTESIAN_POINT('Ctrl Pts',(-0.312844596998426,2.31638325242612,
6.36200459153881));
#72024=CARTESIAN_POINT('Ctrl Pts',(-0.351287345947157,1.95408682588945,
6.38187493506159));
#72025=CARTESIAN_POINT('Ctrl Pts',(-0.0674717784430968,1.72564587231427,
6.40174527858439));
#72026=CARTESIAN_POINT('Ctrl Pts',(0.278239960329309,1.84062386717827,6.42161562210717));
#72027=CARTESIAN_POINT('Ctrl Pts',(0.36870441444973,2.19354415303425,6.44148596562998));
#72028=CARTESIAN_POINT('Ctrl Pts',(0.120932762886018,2.46065041336782,6.46135630915275));
#72029=CARTESIAN_POINT('Ctrl Pts',(-0.237778235116594,2.39690901755665,
6.48122665267555));
#72030=CARTESIAN_POINT('Ctrl Pts',(-0.3783600729834,2.06079401865006,6.50109699619833));
#72031=CARTESIAN_POINT('Ctrl Pts',(-0.171848052960638,1.76064517021965,
6.52096733972113));
#72032=CARTESIAN_POINT('Ctrl Pts',(0.19231116065365,1.77180817912437,6.54083768324391));
#72033=CARTESIAN_POINT('Ctrl Pts',(0.38005106516863,2.08404250440059,6.56070802676671));
#72034=CARTESIAN_POINT('Ctrl Pts',(0.219145856671893,2.41091565947239,6.58057837028948));
#72035=CARTESIAN_POINT('Ctrl Pts',(-0.142795841306913,2.45256602432321,
6.60044871381229));
#72036=CARTESIAN_POINT('Ctrl Pts',(-0.373741794785009,2.17078505938753,
6.62031905733506));
#72037=CARTESIAN_POINT('Ctrl Pts',(-0.261830531898757,1.82406843897947,
6.64018940085787));
#72038=CARTESIAN_POINT('Ctrl Pts',(0.0902745989964047,1.73048146111777,
6.66005974438064));
#72039=CARTESIAN_POINT('Ctrl Pts',(0.35956507508926,1.975877437274,6.67993008790345));
#72040=CARTESIAN_POINT('Ctrl Pts',(0.29900354515251,2.33513896697027,6.69980043142622));
#72041=CARTESIAN_POINT('Ctrl Pts',(-0.0358530318046874,2.47869250575107,
6.71967077494902));
#72042=CARTESIAN_POINT('Ctrl Pts',(-0.337819333030621,2.2748472248346,6.73954111847181));
#72043=CARTESIAN_POINT('Ctrl Pts',(-0.329882386150286,1.91060341843263,
6.7594114619946));
#72044=CARTESIAN_POINT('Ctrl Pts',(-0.0193232594086513,1.72010519160241,
6.77928180551739));
#72045=CARTESIAN_POINT('Ctrl Pts',(0.308962327216199,1.87810873346892,6.79915214904017));
#72046=CARTESIAN_POINT('Ctrl Pts',(0.35381704004292,2.23966730460951,6.81902249256296));
#72047=CARTESIAN_POINT('Ctrl Pts',(0.0740927864707377,2.47310013775744,
6.83889283608576));
#72048=CARTESIAN_POINT('Ctrl Pts',(-0.273601511866297,2.36426438751011,
6.85876317960853));
#72049=CARTESIAN_POINT('Ctrl Pts',(-0.370303670548427,2.01300203806998,
6.87863352313134));
#72050=CARTESIAN_POINT('Ctrl Pts',(-0.127302623794927,1.74154847499761,
6.89850386665411));
#72051=CARTESIAN_POINT('Ctrl Pts',(0.232481249603138,1.79892538734629,6.91837421017692));
#72052=CARTESIAN_POINT('Ctrl Pts',(0.378995225954534,2.1324972691974,6.9382445536997));
#72053=CARTESIAN_POINT('Ctrl Pts',(0.177832678033613,2.4362573306636,6.95811489722249));
#72054=CARTESIAN_POINT('Ctrl Pts',(-0.186467142250151,2.43154706854785,
6.97798524074528));
#72055=CARTESIAN_POINT('Ctrl Pts',(-0.379708744728557,2.12268750709709,
6.99785558426807));
#72056=CARTESIAN_POINT('Ctrl Pts',(-0.224619266596289,1.79301524650992,
7.01772592779085));
#72057=CARTESIAN_POINT('Ctrl Pts',(0.136527809486201,1.74495970504953,7.03759627131366));
#72058=CARTESIAN_POINT('Ctrl Pts',(0.372429206948008,2.0226052998346,7.05746661483643));
#72059=CARTESIAN_POINT('Ctrl Pts',(0.26667750869322,2.37124999568441,7.07733695835923));
#72060=CARTESIAN_POINT('Ctrl Pts',(-0.0837144989230929,2.47105974784618,
7.09720730188202));
#72061=CARTESIAN_POINT('Ctrl Pts',(-0.357309850477381,2.23047269658226,
7.1170776454048));
#72062=CARTESIAN_POINT('Ctrl Pts',(-0.303122057562357,1.87019470845784,
7.1369479889276));
#72063=CARTESIAN_POINT('Ctrl Pts',(0.0291389568243188,1.72073179015793,
7.15681833245039));
#72064=CARTESIAN_POINT('Ctrl Pts',(0.334668945235442,1.91919582168376,7.17668867597317));
#72065=CARTESIAN_POINT('Ctrl Pts',(0.333185737455809,2.28352307254851,7.19655901949597));
#72066=CARTESIAN_POINT('Ctrl Pts',(0.0260499747027282,2.47949288876026,
7.21642936301875));
#72067=CARTESIAN_POINT('Ctrl Pts',(-0.304983093456289,2.32732964282612,
7.23629970654154));
#72068=CARTESIAN_POINT('Ctrl Pts',(-0.356235693068131,1.96662239773529,
7.25617005006433));
#72069=CARTESIAN_POINT('Ctrl Pts',(-0.0806905414003209,1.72827094500141,
7.27604039358713));
#72070=CARTESIAN_POINT('Ctrl Pts',(0.268877196977014,1.83093029388762,7.29591073710991));
#72071=CARTESIAN_POINT('Ctrl Pts',(0.371786711452961,2.18042446759916,7.31578108063271));
#72072=CARTESIAN_POINT('Ctrl Pts',(0.133632532361157,2.45614014109106,7.33565142415549));
#72073=CARTESIAN_POINT('Ctrl Pts',(-0.227111302745492,2.40514571923404,
7.35552176767828));
#72074=CARTESIAN_POINT('Ctrl Pts',(-0.37951143599511,2.07422164181826,7.37539211120107));
#72075=CARTESIAN_POINT('Ctrl Pts',(-0.183761492535834,1.76694569862766,
7.39526245472386));
#72076=CARTESIAN_POINT('Ctrl Pts',(0.180564603456863,1.76520173569733,7.41513279824664));
#72077=CARTESIAN_POINT('Ctrl Pts',(0.379247257428947,2.07058960159674,7.43500314176944));
#72078=CARTESIAN_POINT('Ctrl Pts',(0.230022182561926,2.40295750416694,7.45487348529222));
#72079=CARTESIAN_POINT('Ctrl Pts',(-0.130216930113199,2.45740314060387,
7.47474382881502));
#72080=CARTESIAN_POINT('Ctrl Pts',(-0.370999736843724,2.18398005158073,
7.49461417233779));
#72081=CARTESIAN_POINT('Ctrl Pts',(-0.271440792073554,1.83351669808392,
7.51448451586061));
#72082=CARTESIAN_POINT('Ctrl Pts',(0.0771281260971214,1.72751549566946,
7.53435485938337));
#72083=CARTESIAN_POINT('Ctrl Pts',(0.354942488619908,1.96321811679202,7.55422520290618));
#72084=CARTESIAN_POINT('Ctrl Pts',(0.3071454388904,2.32439949458597,7.57409554642895));
#72085=CARTESIAN_POINT('Ctrl Pts',(-0.0224157369453323,2.47972488532992,
7.59396588995176));
#72086=CARTESIAN_POINT('Ctrl Pts',(-0.331413525760743,2.28670438865877,
7.61383623347454));
#72087=CARTESIAN_POINT('Ctrl Pts',(-0.336384522568092,1.92240803290055,
7.63370657699733));
#72088=CARTESIAN_POINT('Ctrl Pts',(-0.0327685145367435,1.72102812999291,
7.65357692052013));
#72089=CARTESIAN_POINT('Ctrl Pts',(0.300908144551645,1.86730332545543,7.67344726404291));
#72090=CARTESIAN_POINT('Ctrl Pts',(0.358542545958669,2.22704604102093,7.69331760756571));
#72091=CARTESIAN_POINT('Ctrl Pts',(0.0872629726086352,2.47024130970641,
7.71318795108848));
#72092=CARTESIAN_POINT('Ctrl Pts',(-0.264068498328838,2.37379058053916,
7.73305829461128));
#72093=CARTESIAN_POINT('Ctrl Pts',(-0.373153071729418,2.02617426694902,
7.75292863813407));
#72094=CARTESIAN_POINT('Ctrl Pts',(-0.139920502021753,1.74628301296715,
7.77279898165686));
#72095=CARTESIAN_POINT('Ctrl Pts',(0.221670079834584,1.79087894036843,7.79266932517965));
#72096=CARTESIAN_POINT('Ctrl Pts',(0.379908541099039,2.11905135694947,7.81253966870244));
#72097=CARTESIAN_POINT('Ctrl Pts',(0.189632635782723,2.42974674713742,7.83241001222523));
#72098=CARTESIAN_POINT('Ctrl Pts',(-0.174605396712056,2.43794438779278,
7.85228035574801));
#72099=CARTESIAN_POINT('Ctrl Pts',(-0.378666748101841,2.13612405962227,
7.87215069927082));
#72100=CARTESIAN_POINT('Ctrl Pts',(-0.235352908930933,1.80116482459495,
7.89202104279359));
#72101=CARTESIAN_POINT('Ctrl Pts',(0.12386518377878,1.74034618026627,7.91189138631639));
#72102=CARTESIAN_POINT('Ctrl Pts',(0.369453833093542,2.00946095309699,7.93176172983917));
#72103=CARTESIAN_POINT('Ctrl Pts',(0.276118887142609,2.36163297568301,7.95163207336197));
#72104=CARTESIAN_POINT('Ctrl Pts',(-0.0705175475695523,2.47379236119321,
7.97150241688475));
#72105=CARTESIAN_POINT('Ctrl Pts',(-0.352463732483867,2.24304814254354,
7.99137276040755));
#72106=CARTESIAN_POINT('Ctrl Pts',(-0.311072426448528,1.88107672735627,
8.01124310393033));
#72107=CARTESIAN_POINT('Ctrl Pts',(0.0156854821665361,1.71993761110731,
8.03111344745313));
#72108=CARTESIAN_POINT('Ctrl Pts',(0.328054096279372,1.90745399584531,8.05098379097592));
#72109=CARTESIAN_POINT('Ctrl Pts',(0.33947773758828,2.27160512662376,8.07085413449869));
#72110=CARTESIAN_POINT('Ctrl Pts',(0.0394767703806659,2.47833191565335,
8.0907244780215));
#72111=CARTESIAN_POINT('Ctrl Pts',(-0.296738759374218,2.3379906773104,8.11059482154428));
#72112=CARTESIAN_POINT('Ctrl Pts',(-0.36073687473749,1.97932539204024,8.13046516506707));
#72113=CARTESIAN_POINT('Ctrl Pts',(-0.0938080174200238,1.73136263120875,
8.15033550858987));
#72114=CARTESIAN_POINT('Ctrl Pts',(0.259176925071939,1.82157447079718,8.17020585211264));
#72115=CARTESIAN_POINT('Ctrl Pts',(0.374402322562648,2.16720382921612,8.19007619563545));
#72116=CARTESIAN_POINT('Ctrl Pts',(0.146164559375766,2.45118282330448,8.20994653915821));
#72117=CARTESIAN_POINT('Ctrl Pts',(-0.216159288530444,2.41299938623523,
8.22981688268102));
#72118=CARTESIAN_POINT('Ctrl Pts',(-0.38018641663983,2.08768162331384,8.24968722620381));
#72119=CARTESIAN_POINT('Ctrl Pts',(-0.195444265189107,1.77366429400645,
8.26955756972659));
#72120=CARTESIAN_POINT('Ctrl Pts',(0.168591392238535,1.75901554835347,8.28942791324939));
#72121=CARTESIAN_POINT('Ctrl Pts',(0.377967398932861,2.05717361624485,8.30929825677218));
#72122=CARTESIAN_POINT('Ctrl Pts',(0.240609772721243,2.3946190609459,8.32916860029496));
#72123=CARTESIAN_POINT('Ctrl Pts',(-0.117474563899405,2.46179162599245,
8.34903894381776));
#72124=CARTESIAN_POINT('Ctrl Pts',(-0.367791980860096,2.19706962767325,
8.36890928734054));
#72125=CARTESIAN_POINT('Ctrl Pts',(-0.280710325738522,1.84329946080036,
8.38877963086334));
#72126=CARTESIAN_POINT('Ctrl Pts',(0.0638848379881091,1.72501709202038,
8.40864997438611));
#72127=CARTESIAN_POINT('Ctrl Pts',(0.349874359995995,1.95073049199851,8.42852031790892));
#72128=CARTESIAN_POINT('Ctrl Pts',(0.314901787800618,2.31337834435947,8.44839066143169));
#72129=CARTESIAN_POINT('Ctrl Pts',(-0.00895030469455451,2.48028061460912,
8.4682610049545));
#72130=CARTESIAN_POINT('Ctrl Pts',(-0.324591711106426,2.29832719148573,
8.48813134847726));
#72131=CARTESIAN_POINT('Ctrl Pts',(-0.342464411749368,1.93443556998325,
8.50800169200008));
#72132=CARTESIAN_POINT('Ctrl Pts',(-0.0461726369319628,1.72242677345929,
8.52787203552285));
#72133=CARTESIAN_POINT('Ctrl Pts',(0.292476246433607,1.8567900103332,8.54774237904566));
#72134=CARTESIAN_POINT('Ctrl Pts',(0.362817990741843,2.21426530267612,8.56761272256843));
#72135=CARTESIAN_POINT('Ctrl Pts',(0.100323621753707,2.46691773562999,8.58748306609123));
#72136=CARTESIAN_POINT('Ctrl Pts',(-0.25420401236565,2.38297309748246,8.60735340961401));
#72137=CARTESIAN_POINT('Ctrl Pts',(-0.375534071890836,2.03943916570338,
8.62722375313683));
#72138=CARTESIAN_POINT('Ctrl Pts',(-0.152362744803578,1.75146155477833,
8.64709409665957));
#72139=CARTESIAN_POINT('Ctrl Pts',(0.210580658326276,1.78322051811948,8.6669644401824));
#72140=CARTESIAN_POINT('Ctrl Pts',(0.380344975409706,2.10558153045376,8.68683478370515));
#72141=CARTESIAN_POINT('Ctrl Pts',(0.201194556847495,2.42282224845347,8.70670512722799));
#72142=CARTESIAN_POINT('Ctrl Pts',(-0.162524477456688,2.44391750177775,
8.72657547075073));
#72143=CARTESIAN_POINT('Ctrl Pts',(-0.377149429404031,2.14951526736098,
8.74644581427356));
#72144=CARTESIAN_POINT('Ctrl Pts',(-0.245791124131638,1.80968951603547,
8.76631615779632));
#72145=CARTESIAN_POINT('Ctrl Pts',(0.111047076091526,1.73618411154385,8.78618650131912));
#72146=CARTESIAN_POINT('Ctrl Pts',(0.366014701695009,1.99643025564998,8.80605684484191));
#72147=CARTESIAN_POINT('Ctrl Pts',(0.285213666895485,2.35168754044976,8.8259271883647));
#72148=CARTESIAN_POINT('Ctrl Pts',(-0.0572320789460712,2.47605577105148,
8.84579753188749));
#72149=CARTESIAN_POINT('Ctrl Pts',(-0.347175183798591,2.2554440270838,8.86566787541028));
#72150=CARTESIAN_POINT('Ctrl Pts',(-0.318632321149308,1.89223355006012,
8.88553821893306));
#72151=CARTESIAN_POINT('Ctrl Pts',(0.00221231828093774,1.71962050600822,
8.90540856245586));
#72152=CARTESIAN_POINT('Ctrl Pts',(0.321027456868357,1.89595386370174,8.92527890597865));
#72153=CARTESIAN_POINT('Ctrl Pts',(0.345343607720877,2.25947177307581,8.94514924950143));
#72154=CARTESIAN_POINT('Ctrl Pts',(0.0528540127763269,2.47669604077433,
8.96501959302423));
#72155=CARTESIAN_POINT('Ctrl Pts',(-0.288121943466405,2.34835297359757,
8.984889936547));
#72156=CARTESIAN_POINT('Ctrl Pts',(-0.364785240839391,1.99217986334937,
9.00476028006981));
#72157=CARTESIAN_POINT('Ctrl Pts',(-0.10680774076842,1.73491705009196,9.02463062359258));
#72158=CARTESIAN_POINT('Ctrl Pts',(0.249151320896677,1.81256814181956,9.04450096711538));
#72159=CARTESIAN_POINT('Ctrl Pts',(0.376547964528556,2.15389883311368,9.06437131063818));
#72160=CARTESIAN_POINT('Ctrl Pts',(0.158513113081901,2.44578468268952,9.08424165416096));
#72161=CARTESIAN_POINT('Ctrl Pts',(-0.204935940005677,2.42046016023151,
9.10411199768375));
#72162=CARTESIAN_POINT('Ctrl Pts',(-0.380384167646973,2.10115706747243,
9.12398234120655));
#72163=CARTESIAN_POINT('Ctrl Pts',(-0.206881706100475,1.7807925228279,9.14385268472931));
#72164=CARTESIAN_POINT('Ctrl Pts',(0.156406556392147,1.75325738231484,9.16372302825214));
#72165=CARTESIAN_POINT('Ctrl Pts',(0.376213096224902,2.04381138878305,9.18359337177489));
#72166=CARTESIAN_POINT('Ctrl Pts',(0.250895337059515,2.38591079665415,9.20346371529772));
#72167=CARTESIAN_POINT('Ctrl Pts',(-0.104584737542124,2.46572597183528,
9.22333405882047));
#72168=CARTESIAN_POINT('Ctrl Pts',(-0.364122553375209,2.2100373569527,9.24320440234329));
#72169=CARTESIAN_POINT('Ctrl Pts',(-0.28962749729597,1.85340444729945,9.26307474586605));
#72170=CARTESIAN_POINT('Ctrl Pts',(0.0505613583289935,1.7229893862959,9.28294508938887));
#72171=CARTESIAN_POINT('Ctrl Pts',(0.344367050994486,1.93843023800544,9.30281543291163));
#72172=CARTESIAN_POINT('Ctrl Pts',(0.322262855713179,2.3020893506081,9.32268577643445));
#72173=CARTESIAN_POINT('Ctrl Pts',(0.00452636244120668,2.4803589960086,
9.34255611995722));
#72174=CARTESIAN_POINT('Ctrl Pts',(-0.317362452161966,2.3097010437727,9.36242646348002));
#72175=CARTESIAN_POINT('Ctrl Pts',(-0.348114421903012,1.94667093209458,
9.38229680700281));
#72176=CARTESIAN_POINT('Ctrl Pts',(-0.0595188010471789,1.72429936635199,
9.40216715052558));
#72177=CARTESIAN_POINT('Ctrl Pts',(0.283677217016357,1.84658198495871,9.4220374940484));
#72178=CARTESIAN_POINT('Ctrl Pts',(0.3666380076332,2.20134113261837,9.44190783757116));
#72179=CARTESIAN_POINT('Ctrl Pts',(0.113258339504188,2.46313358745008,9.46177818109397));
#72180=CARTESIAN_POINT('Ctrl Pts',(-0.244020436389291,2.39180041197023,
9.48164852461675));
#72181=CARTESIAN_POINT('Ctrl Pts',(-0.377443682278235,2.05278008354664,
9.50151886813954));
#72182=CARTESIAN_POINT('Ctrl Pts',(-0.164613733994266,1.75707760005785,
9.52138921166233));
#72183=CARTESIAN_POINT('Ctrl Pts',(0.199226905093178,1.77595973384684,9.54125955518512));
#72184=CARTESIAN_POINT('Ctrl Pts',(0.380303981051631,2.09210469773259,9.56112989870792));
#72185=CARTESIAN_POINT('Ctrl Pts',(0.212503928107109,2.41549252660034,9.58100024223071));
#72186=CARTESIAN_POINT('Ctrl Pts',(-0.150239549078219,2.44945891274139,
9.60087058575347));
#72187=CARTESIAN_POINT('Ctrl Pts',(-0.375158693251968,2.16284432097723,
9.6207409292763));
#72188=CARTESIAN_POINT('Ctrl Pts',(-0.25592080961125,1.81857862019822,9.64061127279905));
#72189=CARTESIAN_POINT('Ctrl Pts',(0.0980895763756364,1.73247872332604,
9.66048161632186));
#72190=CARTESIAN_POINT('Ctrl Pts',(0.362116129727866,1.98352956429838,9.68035195984465));
#72191=CARTESIAN_POINT('Ctrl Pts',(0.293950431714302,2.34142617400894,9.70022230336744));
#72192=CARTESIAN_POINT('Ctrl Pts',(-0.0438747696594335,2.477847136272,9.72009264689022));
#72193=CARTESIAN_POINT('Ctrl Pts',(-0.341450842881172,2.26764479024817,
9.73996299041301));
#72194=CARTESIAN_POINT('Ctrl Pts',(-0.325792252094184,1.90365117194896,
9.75983333393581));
#72195=CARTESIAN_POINT('Ctrl Pts',(-0.0112636226208964,1.71978087290739,
9.77970367745858));
#72196=CARTESIAN_POINT('Ctrl Pts',(0.31359784720331,1.88470986081321,9.7995740209814));
#72197=CARTESIAN_POINT('Ctrl Pts',(0.350775984710272,2.24713824231706,9.81944436450417));
#72198=CARTESIAN_POINT('Ctrl Pts',(0.0661649100837423,2.4745873175579,9.83931470802696));
#72199=CARTESIAN_POINT('Ctrl Pts',(-0.279143462005489,2.35840352439781,
9.85918505154976));
#72200=CARTESIAN_POINT('Ctrl Pts',(-0.368375709655487,2.00516967606597,
9.87905539507253));
#72201=CARTESIAN_POINT('Ctrl Pts',(-0.119673393520951,1.73892973996077,
9.89892573859534));
#72202=CARTESIAN_POINT('Ctrl Pts',(0.238812969107689,1.80392261216435,9.91879608211811));
#72203=CARTESIAN_POINT('Ctrl Pts',(0.37822094403001,2.1405261804105,9.93866642564092));
#72204=CARTESIAN_POINT('Ctrl Pts',(0.170662692936798,2.43995249527129,9.95853676916368));
#72205=CARTESIAN_POINT('Ctrl Pts',(-0.193455345298264,2.42751867607382,
9.9784071126865));
#72206=CARTESIAN_POINT('Ctrl Pts',(-0.380104440789253,2.11463105922013,
9.99827745620927));
#72207=CARTESIAN_POINT('Ctrl Pts',(-0.218059458403045,1.78832143737083,
10.0181477997321));
#72208=CARTESIAN_POINT('Ctrl Pts',(0.144025390953336,1.747934465529,10.0380181432549));
#72209=CARTESIAN_POINT('Ctrl Pts',(0.37398655139648,2.03051969216978,10.0578884867777));
#72210=CARTESIAN_POINT('Ctrl Pts',(0.260865964604863,2.37684364235501,10.0777588303004));
#72211=CARTESIAN_POINT('Ctrl Pts',(-0.0915636310175008,2.46920123953815,
10.0976291738232));
#72212=CARTESIAN_POINT('Ctrl Pts',(-0.359996060444061,2.22286696165515,
10.117499517346));
#72213=CARTESIAN_POINT('Ctrl Pts',(-0.298181113451348,1.86381897327997,
10.1373698608688));
#72214=CARTESIAN_POINT('Ctrl Pts',(0.0371744114399661,1.72143492377703,
10.1572402043916));
#72215=CARTESIAN_POINT('Ctrl Pts',(0.338427474674241,1.92633279472729,10.1771105479144));
#72216=CARTESIAN_POINT('Ctrl Pts',(0.329219402635234,2.29054668386019,10.1969808914372));
#72217=CARTESIAN_POINT('Ctrl Pts',(0.0179973478529294,2.47995993113995,
10.21685123496));
#72218=CARTESIAN_POINT('Ctrl Pts',(-0.309734823466772,2.32081166847254,
10.2367215784828));
#72219=CARTESIAN_POINT('Ctrl Pts',(-0.353327460844313,1.95909876077576,
10.2565919220055));
#72220=CARTESIAN_POINT('Ctrl Pts',(-0.072790254087486,1.72664355809562,
10.2764622655283));
#72221=CARTESIAN_POINT('Ctrl Pts',(0.274522101296335,1.83669206297291,10.2963326090511));
#72222=CARTESIAN_POINT('Ctrl Pts',(0.369997801550122,2.18828975393381,10.3162029525739));
#72223=CARTESIAN_POINT('Ctrl Pts',(0.126050889533918,2.45889361522508,10.3360732960967));
#72224=CARTESIAN_POINT('Ctrl Pts',(-0.233530553350605,2.40026144350112,
10.3559436396195));
#72225=CARTESIAN_POINT('Ctrl Pts',(-0.378879505849965,2.06618027426927,
10.3758139831423));
#72226=CARTESIAN_POINT('Ctrl Pts',(-0.176658091519081,1.76312409925545,
10.3956843266651));
#72227=CARTESIAN_POINT('Ctrl Pts',(0.187623071953084,1.76910570166215,10.4155546701879));
#72228=CARTESIAN_POINT('Ctrl Pts',(0.379785609483059,2.07863777560283,10.4354250137107));
#72229=CARTESIAN_POINT('Ctrl Pts',(0.223546553454306,2.40776678222368,10.4552953572334));
#72230=CARTESIAN_POINT('Ctrl Pts',(-0.137766032253613,2.45456166481829,
10.4751657007562));
#72231=CARTESIAN_POINT('Ctrl Pts',(-0.372697038520552,2.1760944891541,10.495036044279));
#72232=CARTESIAN_POINT('Ctrl Pts',(-0.265729250065068,1.8278209790203,10.5149063878018));
#72233=CARTESIAN_POINT('Ctrl Pts',(0.0850089495543705,1.72923466680759,
10.5347767313246));
#72234=CARTESIAN_POINT('Ctrl Pts',(0.357763010881125,1.97077507265668,10.5546470748474));
#72235=CARTESIAN_POINT('Ctrl Pts',(0.302318214760354,2.330861756958,10.5745174183702));
#72236=CARTESIAN_POINT('Ctrl Pts',(-0.0304623864945468,2.47916420824054,
10.594387761893));
#72237=CARTESIAN_POINT('Ctrl Pts',(-0.335297895220145,2.27963511700822,
10.6142581054158));
#72238=CARTESIAN_POINT('Ctrl Pts',(-0.332543231767824,1.91531526103376,
10.6341284489386));
#72239=CARTESIAN_POINT('Ctrl Pts',(-0.0247254248415304,1.72041851050398,
10.6539987924613));
#72240=CARTESIAN_POINT('Ctrl Pts',(0.305774593314228,1.87373610123324,10.6738691359841));
#72241=CARTESIAN_POINT('Ctrl Pts',(0.355768049556133,2.23462001603269,10.6937394795069));
#72242=CARTESIAN_POINT('Ctrl Pts',(0.0793927537767267,2.47200839298242,
10.7136098230297));
#72243=CARTESIAN_POINT('Ctrl Pts',(-0.269814585245385,2.36812971374034,
10.7334801665525));
#72244=CARTESIAN_POINT('Ctrl Pts',(-0.371503774243771,2.01827852470586,
10.7533505100753));
#72245=CARTESIAN_POINT('Ctrl Pts',(-0.132388826045411,1.74339566387952,
10.7732208535981));
#72246=CARTESIAN_POINT('Ctrl Pts',(0.228174846938419,1.79564873414713,10.7930911971209));
#72247=CARTESIAN_POINT('Ctrl Pts',(0.379419161056678,2.12710265715135,10.8129615406436));
#72248=CARTESIAN_POINT('Ctrl Pts',(0.182598048159953,2.4336935819128,10.8328318841665));
#72249=CARTESIAN_POINT('Ctrl Pts',(-0.181731915443975,2.43416607354829,
10.8527022276892));
#72250=CARTESIAN_POINT('Ctrl Pts',(-0.379347587194283,2.12808668530619,
10.872572571212));
#72251=CARTESIAN_POINT('Ctrl Pts',(-0.228963491204467,1.7962415869526,10.8924429147348));
#72252=CARTESIAN_POINT('Ctrl Pts',(0.131463437400806,1.7430534795962,10.9123132582576));
#72253=CARTESIAN_POINT('Ctrl Pts',(0.371290559321738,2.01731521082953,10.9321836017804));
#72254=CARTESIAN_POINT('Ctrl Pts',(0.270509139710306,2.36742897960917,10.9520539453032));
#72255=CARTESIAN_POINT('Ctrl Pts',(-0.0784275890913711,2.47221306676544,
10.971924288826));
#72256=CARTESIAN_POINT('Ctrl Pts',(-0.355417681853844,2.23554233739778,
10.9917946323488));
#72257=CARTESIAN_POINT('Ctrl Pts',(-0.306360437263606,1.87452996589066,
11.0116649758716));
#72258=CARTESIAN_POINT('Ctrl Pts',(0.0237408013085933,1.72035565570544,
11.0315353193943));
#72259=CARTESIAN_POINT('Ctrl Pts',(0.332063086698409,1.91445334750004,11.0514056629171));
#72260=CARTESIAN_POINT('Ctrl Pts',(0.335762696349584,2.27876483306756,11.0712760064399));
#72261=CARTESIAN_POINT('Ctrl Pts',(0.0314457420635472,2.47908392093003,
11.0911463499627));
#72262=CARTESIAN_POINT('Ctrl Pts',(-0.30171839961458,2.33164511895491,11.1110166934855));
#72263=CARTESIAN_POINT('Ctrl Pts',(-0.358096984897371,1.97170345597395,
11.1308870370083));
#72264=CARTESIAN_POINT('Ctrl Pts',(-0.0859703370391827,1.72945640613959,
11.1507573805311));
#72265=CARTESIAN_POINT('Ctrl Pts',(0.265022391247913,1.827132658717,11.1706277240539));
#72266=CARTESIAN_POINT('Ctrl Pts',(0.372893155105661,2.17512754938744,11.1904980675766));
#72267=CARTESIAN_POINT('Ctrl Pts',(0.138685213973004,2.45420314118719,11.2103684110995));
#72268=CARTESIAN_POINT('Ctrl Pts',(-0.222747530692876,2.40834557135112,
11.2302387546222));
#72269=CARTESIAN_POINT('Ctrl Pts',(-0.379839740286083,2.07962291725939,
11.250109098145));
#72270=CARTESIAN_POINT('Ctrl Pts',(-0.188480698678018,1.76959346249285,
11.2699794416678));
#72271=CARTESIAN_POINT('Ctrl Pts',(0.175783724637021,1.76266702510078,11.2898497851906));
#72272=CARTESIAN_POINT('Ctrl Pts',(0.378790511390766,2.0651976684411,11.3097201287134));
#72273=CARTESIAN_POINT('Ctrl Pts',(0.234308571615089,2.39965471307709,11.3295904722362));
#72274=CARTESIAN_POINT('Ctrl Pts',(-0.125119584385799,2.45921935277034,
11.349460815759));
#72275=CARTESIAN_POINT('Ctrl Pts',(-0.369767555206014,2.18924913959576,
11.3693311592818));
#72276=CARTESIAN_POINT('Ctrl Pts',(-0.275204133431753,1.83740499101526,
11.3892015028045));
#72277=CARTESIAN_POINT('Ctrl Pts',(0.0718216151065006,1.72645601409592,
11.4090718463273));
#72278=CARTESIAN_POINT('Ctrl Pts',(0.35296080941452,1.95818279082192,11.4289421898501));
#72279=CARTESIAN_POINT('Ctrl Pts',(0.310306512359927,2.32000755029915,11.4488125333729));
#72280=CARTESIAN_POINT('Ctrl Pts',(-0.0170117653678856,2.48000533370031,
11.4686828768957));
#72281=CARTESIAN_POINT('Ctrl Pts',(-0.328724064313393,2.29139995648615,
11.4885532204185));
#72282=CARTESIAN_POINT('Ctrl Pts',(-0.33887678599166,1.92721117594711,11.5084235639413));
#72283=CARTESIAN_POINT('Ctrl Pts',(-0.038156190431134,1.72153261840233,
11.5282939074641));
#72284=CARTESIAN_POINT('Ctrl Pts',(0.29756751535369,1.86304635979195,11.5481642509869));
#72285=CARTESIAN_POINT('Ctrl Pts',(0.360313535960682,2.22193280774724,11.5680345945097));
#72286=CARTESIAN_POINT('Ctrl Pts',(0.092520939582283,2.46896250424729,11.5879049380324));
#72287=CARTESIAN_POINT('Ctrl Pts',(-0.260147023274306,2.37751933280969,
11.6077752815552));
#72288=CARTESIAN_POINT('Ctrl Pts',(-0.374165508095917,2.03148995436479,
11.627645625078));
#72289=CARTESIAN_POINT('Ctrl Pts',(-0.144938077273781,1.74830921598968,
11.6475159686008));
#72290=CARTESIAN_POINT('Ctrl Pts',(0.21725030790957,1.78775689356719,11.6673863121236));
#72291=CARTESIAN_POINT('Ctrl Pts',(0.380141111544627,2.1136451132363,11.6872566556464));
#72292=CARTESIAN_POINT('Ctrl Pts',(0.194304196876692,2.42701579912555,11.7071269991692));
#72293=CARTESIAN_POINT('Ctrl Pts',(-0.169780366297813,2.44039400849809,
11.726997342692));
#72294=CARTESIAN_POINT('Ctrl Pts',(-0.378114556903807,2.14150705553338,
11.7468676862148));
#72295=CARTESIAN_POINT('Ctrl Pts',(-0.239580117199271,1.80454302979216,
11.7667380297376));
#72296=CARTESIAN_POINT('Ctrl Pts',(0.118736464147836,1.73862055138222,11.7866083732603));
#72297=CARTESIAN_POINT('Ctrl Pts',(0.368128504149248,2.00421451970967,11.8064787167831));
#72298=CARTESIAN_POINT('Ctrl Pts',(0.279812757764116,2.35767862618784,11.8263490603059));
#72299=CARTESIAN_POINT('Ctrl Pts',(-0.0651931008024049,2.47475767291596,
11.8462194038287));
#72300=CARTESIAN_POINT('Ctrl Pts',(-0.350393164621961,2.24804757339389,
11.8660897473515));
#72301=CARTESIAN_POINT('Ctrl Pts',(-0.314155201622804,1.88552398014009,
11.8859600908743));
#72302=CARTESIAN_POINT('Ctrl Pts',(0.0102773904965317,1.71975293683423,
11.9058304343971));
#72303=CARTESIAN_POINT('Ctrl Pts',(0.325281875975677,1.90280680801975,11.9257007779199));
#72304=CARTESIAN_POINT('Ctrl Pts',(0.341884523375812,2.26675858741819,11.9455711214427));
#72305=CARTESIAN_POINT('Ctrl Pts',(0.0448546639536624,2.47773206499213,
11.9654414649654));
#72306=CARTESIAN_POINT('Ctrl Pts',(-0.293323243234879,2.34218779651293,
11.9853118084882));
#72307=CARTESIAN_POINT('Ctrl Pts',(-0.362417007109122,1.98446919562436,
12.005182152011));
#72308=CARTESIAN_POINT('Ctrl Pts',(-0.0990425055810213,1.73273437965167,
12.0250524955338));
#72309=CARTESIAN_POINT('Ctrl Pts',(0.255190011398074,1.81791577164921,12.0449228390566));
#72310=CARTESIAN_POINT('Ctrl Pts',(0.375320433902403,2.1618710408586,12.0647931825794));
#72311=CARTESIAN_POINT('Ctrl Pts',(0.151145453564486,2.44906805306186,12.0846635261022));
#72312=CARTESIAN_POINT('Ctrl Pts',(-0.211684903823395,2.41604264790515,
12.104533869625));
#72313=CARTESIAN_POINT('Ctrl Pts',(-0.380323180250697,2.0930911386168,12.1244042131477));
#72314=CARTESIAN_POINT('Ctrl Pts',(-0.200066715123608,1.77647756909101,
12.1442745566706));
#72315=CARTESIAN_POINT('Ctrl Pts',(0.163723724505573,1.75665178632234,12.1641449001933));
#72316=CARTESIAN_POINT('Ctrl Pts',(0.377319935873306,2.05180124696446,12.1840152437162));
#72317=CARTESIAN_POINT('Ctrl Pts',(0.244776473548098,2.39116650184899,12.2038855872389));
#72318=CARTESIAN_POINT('Ctrl Pts',(-0.112316079949689,2.46342613002693,
12.2237559307617));
#72319=CARTESIAN_POINT('Ctrl Pts',(-0.3663739205472,2.20229175990513,12.2436262742845));
#72320=CARTESIAN_POINT('Ctrl Pts',(-0.284333566348057,1.84731862583599,
12.2634966178073));
#72321=CARTESIAN_POINT('Ctrl Pts',(0.0585441264557262,1.72414625309949,
12.2833669613301));
#72322=CARTESIAN_POINT('Ctrl Pts',(0.347715553299502,1.94576852527698,12.3032373048529));
#72323=CARTESIAN_POINT('Ctrl Pts',(0.317905297189056,2.30887717879355,12.3231076483757));
#72324=CARTESIAN_POINT('Ctrl Pts',(-0.00353979019419505,2.48036945682717,
12.3429779918984));
#72325=CARTESIAN_POINT('Ctrl Pts',(-0.321737601973187,2.30292454084747,
12.3628483354212));
#72326=CARTESIAN_POINT('Ctrl Pts',(-0.344784964561129,1.93932398432187,
12.382718678944));
#72327=CARTESIAN_POINT('Ctrl Pts',(-0.0515390603986663,1.72312179811664,
12.4025890224668));
#72328=CARTESIAN_POINT('Ctrl Pts',(0.288986915270079,1.85265405480521,12.4224593659896));
#72329=CARTESIAN_POINT('Ctrl Pts',(0.364406738194478,2.20909254310024,12.4423297095124));
#72330=CARTESIAN_POINT('Ctrl Pts',(0.105532988323146,2.46545347470943,12.4622000530352));
#72331=CARTESIAN_POINT('Ctrl Pts',(-0.250152911315643,2.38656059527075,
12.4820703965579));
#72332=CARTESIAN_POINT('Ctrl Pts',(-0.376357570066043,2.04478738137345,
12.5019407400808));
#72333=CARTESIAN_POINT('Ctrl Pts',(-0.157305394737393,1.75366422854673,
12.5218110836035));
#72334=CARTESIAN_POINT('Ctrl Pts',(0.206053065067093,1.78025699667065,12.5416814271264));
#72335=CARTESIAN_POINT('Ctrl Pts',(0.3803858892643,2.10017044126998,12.5615517706491));
#72336=CARTESIAN_POINT('Ctrl Pts',(0.205766444924184,2.41992752920759,12.5814221141719));
#72337=CARTESIAN_POINT('Ctrl Pts',(-0.157615700061881,2.44619466329742,
12.6012924576947));
#72338=CARTESIAN_POINT('Ctrl Pts',(-0.376406897681196,2.15487532395946,
12.6211628012175));
#72339=CARTESIAN_POINT('Ctrl Pts',(-0.249896009849807,1.81321534548945,
12.6410331447403));
#72340=CARTESIAN_POINT('Ctrl Pts',(0.105860446748859,1.73464124532766,12.6609034882631));
#72341=CARTESIAN_POINT('Ctrl Pts',(0.364504355054273,1.99123406347468,12.6807738317859));
#72342=CARTESIAN_POINT('Ctrl Pts',(0.288765140383735,2.34760482123854,12.7006441753087));
#72343=CARTESIAN_POINT('Ctrl Pts',(-0.0518767787635012,2.47683186386853,
12.7205145188314));
#72344=CARTESIAN_POINT('Ctrl Pts',(-0.344928815783521,2.26036697242512,
12.7403848623542));
#72345=CARTESIAN_POINT('Ctrl Pts',(-0.321555622135165,1.89678721577324,
12.760255205877));
#72346=CARTESIAN_POINT('Ctrl Pts',(-0.00319892103246907,1.71962752372756,
12.7801255493998));
#72347=CARTESIAN_POINT('Ctrl Pts',(0.318092354642332,1.89140779562403,12.7999958929226));
#72348=CARTESIAN_POINT('Ctrl Pts',(0.34757719926072,2.25454301777328,12.8198662364454));
#72349=CARTESIAN_POINT('Ctrl Pts',(0.0582072819892302,2.47590606024336,
12.8397365799682));
#72350=CARTESIAN_POINT('Ctrl Pts',(-0.284559892434335,2.35242646743737,
12.859606923491));
#72351=CARTESIAN_POINT('Ctrl Pts',(-0.366282104624736,1.99737995550227,
12.8794772670138));
#72352=CARTESIAN_POINT('Ctrl Pts',(-0.111990351120574,1.73647336396665,
12.8993476105365));
#72353=CARTESIAN_POINT('Ctrl Pts',(0.245037304376393,1.80905297125057,12.9192179540593));
#72354=CARTESIAN_POINT('Ctrl Pts',(0.377276590096335,2.14853686866335,12.9390882975821));
#72355=CARTESIAN_POINT('Ctrl Pts',(0.163415969494412,2.4434947965587,12.9589586411049));
#72356=CARTESIAN_POINT('Ctrl Pts',(-0.200356562826449,2.42334301162293,
12.9788289846277));
#72357=CARTESIAN_POINT('Ctrl Pts',(-0.380329211771941,2.10656803189499,
12.9986993281505));
#72358=CARTESIAN_POINT('Ctrl Pts',(-0.211401611228264,1.78376777860929,
13.0185696716733));
#72359=CARTESIAN_POINT('Ctrl Pts',(0.151458236356993,1.75106753433639,13.0384400151961));
#72360=CARTESIAN_POINT('Ctrl Pts',(0.375375677902762,2.03846533019108,13.0583103587189));
#72361=CARTESIAN_POINT('Ctrl Pts',(0.254937217576202,2.38231279733737,13.0781807022417));
#72362=CARTESIAN_POINT('Ctrl Pts',(-0.0993717796601711,2.46717672766403,
13.0980510457644));
#72363=CARTESIAN_POINT('Ctrl Pts',(-0.36252003019322,2.21520595589093,13.1179213892872));
#72364=CARTESIAN_POINT('Ctrl Pts',(-0.29310679059858,1.85754948255962,13.13779173281));
#72365=CARTESIAN_POINT('Ctrl Pts',(0.0451945013969898,1.7223081999728,13.1576620763328));
#72366=CARTESIAN_POINT('Ctrl Pts',(0.342031224084195,1.93354801925746,13.1775324198556));
#72367=CARTESIAN_POINT('Ctrl Pts',(0.325110043695346,2.29748430527921,13.1974027633784));
#72368=CARTESIAN_POINT('Ctrl Pts',(0.00992697299317924,2.48025671492838,
13.2172731069012));
#72369=CARTESIAN_POINT('Ctrl Pts',(-0.314328680327199,2.31419325886201,
13.237143450424));
#72370=CARTESIAN_POINT('Ctrl Pts',(-0.350296176606381,1.95164068828411,
13.2570137939467));
#72371=CARTESIAN_POINT('Ctrl Pts',(-0.0647881917136264,1.72517979117865,
13.2768841374695));
#72372=CARTESIAN_POINT('Ctrl Pts',(0.279910194519454,1.84258056808262,13.2967544809923));
#72373=CARTESIAN_POINT('Ctrl Pts',(0.368303012953287,2.19609810697459,13.3166248245151));
#72374=CARTESIAN_POINT('Ctrl Pts',(0.117820898012969,2.46158919785312,13.3364996043286));
#72375=CARTESIAN_POINT('Ctrl Pts',(-0.11986884365505,2.41719040905852,13.3497509363012));
#72376=CARTESIAN_POINT('Ctrl Pts',(-0.203005792691873,2.34955307066552,
13.3563788204328));
#72377=CARTESIAN_POINT('Ctrl Pts',(0.339316982523676,2.16590180780864,4.32919355271553));
#72378=CARTESIAN_POINT('Ctrl Pts',(0.317376240845729,2.27887088268001,4.33581700055646));
#72379=CARTESIAN_POINT('Ctrl Pts',(0.152140072236355,2.47920395269148,4.34906389623832));
#72380=CARTESIAN_POINT('Ctrl Pts',(-0.237247314916726,2.43314083568054,
4.3689342397611));
#72381=CARTESIAN_POINT('Ctrl Pts',(-0.408159666448758,2.08086921922066,
4.3888045832839));
#72382=CARTESIAN_POINT('Ctrl Pts',(-0.20505268712016,1.74644911680938,4.40867492680669));
#72383=CARTESIAN_POINT('Ctrl Pts',(0.186373697626367,1.73620810823211,4.42854527032948));
#72384=CARTESIAN_POINT('Ctrl Pts',(0.406718025226084,2.0597773819746,4.44841561385227));
#72385=CARTESIAN_POINT('Ctrl Pts',(0.25401079205995,2.42020351937108,4.46828595737505));
#72386=CARTESIAN_POINT('Ctrl Pts',(-0.131746279212509,2.48690827868763,
4.48815630089785));
#72387=CARTESIAN_POINT('Ctrl Pts',(-0.396628750627812,2.19866606826832,
4.50802664442063));
#72388=CARTESIAN_POINT('Ctrl Pts',(-0.297666295542051,1.81991703748627,
4.52789698794343));
#72389=CARTESIAN_POINT('Ctrl Pts',(0.0743685927383873,1.6981029499077,4.54776733146621));
#72390=CARTESIAN_POINT('Ctrl Pts',(0.378178276998698,1.94497627337976,4.56763767498901));
#72391=CARTESIAN_POINT('Ctrl Pts',(0.335061989847928,2.33406194065974,4.58750801851179));
#72392=CARTESIAN_POINT('Ctrl Pts',(-0.0154286364801445,2.50842806818002,
4.60737836203459));
#72393=CARTESIAN_POINT('Ctrl Pts',(-0.351765289137388,2.30811682436188,
4.62724870555736));
#72394=CARTESIAN_POINT('Ctrl Pts',(-0.365405333347371,1.91688684160467,
4.64711904908017));
#72395=CARTESIAN_POINT('Ctrl Pts',(-0.0438356487582682,1.69363819343353,
4.66698939260294));
#72396=CARTESIAN_POINT('Ctrl Pts',(0.317947233881606,1.84317121258462,4.68685973612574));
#72397=CARTESIAN_POINT('Ctrl Pts',(0.388056835848177,2.22830966403225,4.70673007964853));
#72398=CARTESIAN_POINT('Ctrl Pts',(0.102177108770669,2.4957414748595,4.72660042317132));
#72399=CARTESIAN_POINT('Ctrl Pts',(-0.27743619956892,2.40013435350708,4.74647076669411));
#72400=CARTESIAN_POINT('Ctrl Pts',(-0.40253956738364,2.02919482466415,4.7663411102169));
#72401=CARTESIAN_POINT('Ctrl Pts',(-0.158367681353156,1.7232094037697,4.78621145373968));
#72402=CARTESIAN_POINT('Ctrl Pts',(0.231084991683309,1.7628780601152,4.80608179726248));
#72403=CARTESIAN_POINT('Ctrl Pts',(0.408548644658253,2.11181020098235,4.82595214078526));
#72404=CARTESIAN_POINT('Ctrl Pts',(0.211224534813154,2.44990809042533,4.84582248430806));
#72405=CARTESIAN_POINT('Ctrl Pts',(-0.1798693299841,2.46701294250325,4.86569282783084));
#72406=CARTESIAN_POINT('Ctrl Pts',(-0.405957571578824,2.14743338417888,
4.88556317135363));
#72407=CARTESIAN_POINT('Ctrl Pts',(-0.259635007351826,1.78434015331966,
4.90543351487642));
#72408=CARTESIAN_POINT('Ctrl Pts',(0.124867329989842,1.71082185859386,4.92530385839921));
#72409=CARTESIAN_POINT('Ctrl Pts',(0.39482089122616,1.99432152678229,4.94517420192201));
#72410=CARTESIAN_POINT('Ctrl Pts',(0.302580034768886,2.37476680732616,4.96504454544479));
#72411=CARTESIAN_POINT('Ctrl Pts',(-0.0672368110345127,2.50315094826968,
4.98491488896759));
#72412=CARTESIAN_POINT('Ctrl Pts',(-0.375373036180186,2.26169897822225,
5.00478523249037));
#72413=CARTESIAN_POINT('Ctrl Pts',(-0.339155603054294,1.87191020898354,
5.02465557601317));
#72414=CARTESIAN_POINT('Ctrl Pts',(0.00819092400752989,1.69136277138156,
5.04452591953595));
#72415=CARTESIAN_POINT('Ctrl Pts',(0.34802339338622,1.88568436010163,5.06439626305874));
#72416=CARTESIAN_POINT('Ctrl Pts',(0.368591778439678,2.27661137198876,5.08426660658153));
#72417=CARTESIAN_POINT('Ctrl Pts',(0.0510273860142611,2.50552149354335,
5.10413695010432));
#72418=CARTESIAN_POINT('Ctrl Pts',(-0.313347686327946,2.36242085153815,
5.12400729362711));
#72419=CARTESIAN_POINT('Ctrl Pts',(-0.390268914899715,1.97858480361965,
5.1438776371499));
#72420=CARTESIAN_POINT('Ctrl Pts',(-0.109171544366135,1.70613066919371,
5.16374798067268));
#72421=CARTESIAN_POINT('Ctrl Pts',(0.272075855759673,1.79499802531505,5.18361832419548));
#72422=CARTESIAN_POINT('Ctrl Pts',(0.403730698009074,2.16366317094041,5.20348866771826));
#72423=CARTESIAN_POINT('Ctrl Pts',(0.165017587806566,2.47392602418604,5.22335901124106));
#72424=CARTESIAN_POINT('Ctrl Pts',(-0.225076694092472,2.44116265567246,
5.24322935476384));
#72425=CARTESIAN_POINT('Ctrl Pts',(-0.408693750586667,2.095428995681,5.26309969828664));
#72426=CARTESIAN_POINT('Ctrl Pts',(-0.217389929547608,1.75388860986618,
5.28297004180942));
#72427=CARTESIAN_POINT('Ctrl Pts',(0.173339556884877,1.72985830568816,5.30284038533221));
#72428=CARTESIAN_POINT('Ctrl Pts',(0.405053597925272,2.04538261579978,5.32271072885501));
#72429=CARTESIAN_POINT('Ctrl Pts',(0.265186105937205,2.41101094042966,5.34258107237779));
#72430=CARTESIAN_POINT('Ctrl Pts',(-0.117953536419894,2.49132906753156,
5.36245141590058));
#72431=CARTESIAN_POINT('Ctrl Pts',(-0.392886867035704,2.21265604981513,
5.38232175942337));
#72432=CARTESIAN_POINT('Ctrl Pts',(-0.307399983863389,1.83063644312961,
5.40219210294616));
#72433=CARTESIAN_POINT('Ctrl Pts',(0.0600845357746946,1.69572122933572,
5.42206244646895));
#72434=CARTESIAN_POINT('Ctrl Pts',(0.372449673610413,1.93167675004154,5.44193278999174));
#72435=CARTESIAN_POINT('Ctrl Pts',(0.343142940353064,2.32204593744298,5.46180313351452));
#72436=CARTESIAN_POINT('Ctrl Pts',(-0.000950725985197706,2.50871820606524,
5.48167347703732));
#72437=CARTESIAN_POINT('Ctrl Pts',(-0.344172230661694,2.32044716258195,
5.5015438205601));
#72438=CARTESIAN_POINT('Ctrl Pts',(-0.371662568524335,1.92994585860093,
5.5214141640829));
#72439=CARTESIAN_POINT('Ctrl Pts',(-0.0582030970557029,1.6954460785727,
5.54128450760569));
#72440=CARTESIAN_POINT('Ctrl Pts',(0.308649792325372,1.83206944641086,5.56115485112847));
#72441=CARTESIAN_POINT('Ctrl Pts',(0.392358516122868,2.21448262171589,5.58102519465127));
#72442=CARTESIAN_POINT('Ctrl Pts',(0.116131716166284,2.49187357699819,5.60089553817405));
#72443=CARTESIAN_POINT('Ctrl Pts',(-0.266630123467332,2.4097738741548,5.62076588169685));
#72444=CARTESIAN_POINT('Ctrl Pts',(-0.404795123233261,2.04349881367926,
5.64063622521963));
#72445=CARTESIAN_POINT('Ctrl Pts',(-0.171615705312496,1.72905589971106,
5.66050656874243));
#72446=CARTESIAN_POINT('Ctrl Pts',(0.2189977588639,1.75490369827876,5.68037691226521));
#72447=CARTESIAN_POINT('Ctrl Pts',(0.408710593135368,2.09733037305656,5.70024725578801));
#72448=CARTESIAN_POINT('Ctrl Pts',(0.223487099128054,2.44220606711806,5.72011759931079));
#72449=CARTESIAN_POINT('Ctrl Pts',(-0.166755383308063,2.473154281748,5.73998794283358));
#72450=CARTESIAN_POINT('Ctrl Pts',(-0.40402250325452,2.16178424324237,5.75985828635637));
#72451=CARTESIAN_POINT('Ctrl Pts',(-0.270653979162068,1.79373557272706,
5.77972862987916));
#72452=CARTESIAN_POINT('Ctrl Pts',(0.111002724599506,1.70664282009786,5.79959897340195));
#72453=CARTESIAN_POINT('Ctrl Pts',(0.390829540197415,1.98040172928441,5.81946931692473));
#72454=CARTESIAN_POINT('Ctrl Pts',(0.312123459301574,2.3638757700182,5.83933966044753));
#72455=CARTESIAN_POINT('Ctrl Pts',(-0.052913403731456,2.50527971520252,
5.85921000397032));
#72456=CARTESIAN_POINT('Ctrl Pts',(-0.369409422350321,2.27489469553958,
5.87908034749311));
#72457=CARTESIAN_POINT('Ctrl Pts',(-0.347022586514417,1.88406760248188,
5.8989506910159));
#72458=CARTESIAN_POINT('Ctrl Pts',(-0.00628977041069085,1.69132908760561,
5.91882103453869));
#72459=CARTESIAN_POINT('Ctrl Pts',(0.340213053769923,1.87349049933032,5.93869137806147));
#72460=CARTESIAN_POINT('Ctrl Pts',(0.374616716941616,2.26344354143546,5.95856172158427));
#72461=CARTESIAN_POINT('Ctrl Pts',(0.0653605417801722,2.50345938510249,
5.97843206510705));
#72462=CARTESIAN_POINT('Ctrl Pts',(-0.303855032430304,2.37335616897348,
5.99830240862985));
#72463=CARTESIAN_POINT('Ctrl Pts',(-0.394324980513307,1.9924858818933,6.01817275215263));
#72464=CARTESIAN_POINT('Ctrl Pts',(-0.123055441473957,1.71024516145052,
6.03804309567542));
#72465=CARTESIAN_POINT('Ctrl Pts',(0.261100712632129,1.78555144504693,6.05791343919821));
#72466=CARTESIAN_POINT('Ctrl Pts',(0.405732508550515,2.14932146950758,6.077783782721));
#72467=CARTESIAN_POINT('Ctrl Pts',(0.178159963367115,2.46784576020679,6.09765412624379));
#72468=CARTESIAN_POINT('Ctrl Pts',(-0.212850093916746,2.44892164359453,
6.11752446976659));
#72469=CARTESIAN_POINT('Ctrl Pts',(-0.408599166955684,2.10990942037674,
6.13739481328936));
#72470=CARTESIAN_POINT('Ctrl Pts',(-0.229514130066395,1.76180665300904,
6.15726515681217));
#72471=CARTESIAN_POINT('Ctrl Pts',(0.160118875631453,1.72395024063882,6.17713550033494));
#72472=CARTESIAN_POINT('Ctrl Pts',(0.402864611153995,2.03106828793058,6.19700584385775));
#72473=CARTESIAN_POINT('Ctrl Pts',(0.276036911007084,2.40142179684082,6.21687618738052));
#72474=CARTESIAN_POINT('Ctrl Pts',(-0.104017075956755,2.49526184202183,
6.23674653090332));
#72475=CARTESIAN_POINT('Ctrl Pts',(-0.388649556376463,2.22650295718859,
6.2566168744261));
#72476=CARTESIAN_POINT('Ctrl Pts',(-0.316748978680148,1.84169483095733,
6.2764872179489));
#72477=CARTESIAN_POINT('Ctrl Pts',(0.0457256654755972,1.69384653224932,
6.29635756147168));
#72478=CARTESIAN_POINT('Ctrl Pts',(0.366253236544724,1.91858874740084,6.31622790499448));
#72479=CARTESIAN_POINT('Ctrl Pts',(0.35079332395982,2.30975108990015,6.33609824851726));
#72480=CARTESIAN_POINT('Ctrl Pts',(0.0135282928404845,2.50849536244846,
6.35596859204006));
#72481=CARTESIAN_POINT('Ctrl Pts',(-0.336147105249229,2.33250075157222,
6.37583893556284));
#72482=CARTESIAN_POINT('Ctrl Pts',(-0.377453296568852,1.94321835324761,
6.39570927908563));
#72483=CARTESIAN_POINT('Ctrl Pts',(-0.0724974739127934,1.69776177192447,
6.41557962260842));
#72484=CARTESIAN_POINT('Ctrl Pts',(0.298964911418399,1.82130400507063,6.43544996613121));
#72485=CARTESIAN_POINT('Ctrl Pts',(0.396167690920685,2.20051187253084,6.45532030965401));
#72486=CARTESIAN_POINT('Ctrl Pts',(0.129940547364216,2.48751378039983,6.47519065317679));
#72487=CARTESIAN_POINT('Ctrl Pts',(-0.255489358590775,2.41902454998943,
6.49506099669958));
#72488=CARTESIAN_POINT('Ctrl Pts',(-0.406542559774135,2.05787372623439,
6.51493134022237));
#72489=CARTESIAN_POINT('Ctrl Pts',(-0.184648308136553,1.735368023685,6.53480168374516));
#72490=CARTESIAN_POINT('Ctrl Pts',(0.20663562861907,1.74736251924351,6.55467202726795));
#72491=CARTESIAN_POINT('Ctrl Pts',(0.408359507017333,2.08285389613812,6.57454237079073));
#72492=CARTESIAN_POINT('Ctrl Pts',(0.235469130854051,2.43407448909475,6.59441271431353));
#72493=CARTESIAN_POINT('Ctrl Pts',(-0.153432116640315,2.4788272184418,6.61428305783631));
#72494=CARTESIAN_POINT('Ctrl Pts',(-0.401580285013707,2.17605754753732,
6.63415340135911));
#72495=CARTESIAN_POINT('Ctrl Pts',(-0.281333212106144,1.80351543106745,
6.65402374488189));
#72496=CARTESIAN_POINT('Ctrl Pts',(0.096998782850446,1.70295754386386,6.6738940884047));
#72497=CARTESIAN_POINT('Ctrl Pts',(0.386347599733618,1.96663205771569,6.69376443192747));
#72498=CARTESIAN_POINT('Ctrl Pts',(0.321275090337474,2.35265350220752,6.71363477545027));
#72499=CARTESIAN_POINT('Ctrl Pts',(-0.0385235767892308,2.50689975409239,
6.73350511897305));
#72500=CARTESIAN_POINT('Ctrl Pts',(-0.362982106723224,2.28787087599692,
6.75337546249585));
#72501=CARTESIAN_POINT('Ctrl Pts',(-0.354453969290295,1.89649604548453,
6.77324580601863));
#72502=CARTESIAN_POINT('Ctrl Pts',(-0.0207625695840894,1.69180838867837,
6.79311614954142));
#72503=CARTESIAN_POINT('Ctrl Pts',(0.331975661146908,1.86158096498988,6.81298649306421));
#72504=CARTESIAN_POINT('Ctrl Pts',(0.380171417180859,2.25007054810248,6.832856836587));
#72505=CARTESIAN_POINT('Ctrl Pts',(0.0796116536163171,2.50089083359134,
6.85272718010979));
#72506=CARTESIAN_POINT('Ctrl Pts',(-0.293980963993229,2.38394835561892,
6.87259752363258));
#72507=CARTESIAN_POINT('Ctrl Pts',(-0.397886069033289,2.00652191744416,
6.89246786715536));
#72508=CARTESIAN_POINT('Ctrl Pts',(-0.136784873032339,1.71484889412257,
6.91233821067817));
#72509=CARTESIAN_POINT('Ctrl Pts',(0.249797822396835,1.77649957685518,6.93220855420094));
#72510=CARTESIAN_POINT('Ctrl Pts',(0.407225022679635,2.13491785721739,6.95207889772374));
#72511=CARTESIAN_POINT('Ctrl Pts',(0.191078703334628,2.46130375721966,6.97194924124652));
#72512=CARTESIAN_POINT('Ctrl Pts',(-0.200356313303394,2.45624264703787,
6.99181958476931));
#72513=CARTESIAN_POINT('Ctrl Pts',(-0.407991688534603,2.1243774062559,7.0116899282921));
#72514=CARTESIAN_POINT('Ctrl Pts',(-0.241350232588205,1.77014921391832,
7.03156027181489));
#72515=CARTESIAN_POINT('Ctrl Pts',(0.146697204890655,1.71851421268106,7.05143061533769));
#72516=CARTESIAN_POINT('Ctrl Pts',(0.400169927903416,2.01684048670864,7.07130095886047));
#72517=CARTESIAN_POINT('Ctrl Pts',(0.286541220281133,2.3914542930356,7.09117130238326));
#72518=CARTESIAN_POINT('Ctrl Pts',(-0.0899500478844393,2.4986984634215,
7.11104164590605));
#72519=CARTESIAN_POINT('Ctrl Pts',(-0.383924392709289,2.24019107151272,
7.13091198942884));
#72520=CARTESIAN_POINT('Ctrl Pts',(-0.325700373809799,1.85307745678201,
7.15078233295163));
#72521=CARTESIAN_POINT('Ctrl Pts',(0.0313093979581721,1.69248165998501,
7.17065267647442));
#72522=CARTESIAN_POINT('Ctrl Pts',(0.359597059489159,1.90572846153944,7.19052301999722));
#72523=CARTESIAN_POINT('Ctrl Pts',(0.358003373657915,2.29719295194969,7.21039336352));
#72524=CARTESIAN_POINT('Ctrl Pts',(0.0279903302538735,2.50775975434238,
7.23026370704279));
#72525=CARTESIAN_POINT('Ctrl Pts',(-0.327700030618726,2.34426249360385,
7.25013405056558));
#72526=CARTESIAN_POINT('Ctrl Pts',(-0.382770225729345,1.95668764831954,
7.27000439408837));
#72527=CARTESIAN_POINT('Ctrl Pts',(-0.0867008481940784,1.70058237548712,
7.28987473761115));
#72528=CARTESIAN_POINT('Ctrl Pts',(0.288904754304601,1.8108883973458,7.30974508113395));
#72529=CARTESIAN_POINT('Ctrl Pts',(0.399479575559559,2.18641495564909,7.32961542465673));
#72530=CARTESIAN_POINT('Ctrl Pts',(0.143586270471979,2.48266755647825,7.34948576817953));
#72531=CARTESIAN_POINT('Ctrl Pts',(-0.244027890268046,2.42787476972223,
7.36935611170232));
#72532=CARTESIAN_POINT('Ctrl Pts',(-0.40777968308453,2.07230151786536,7.3892264552251));
#72533=CARTESIAN_POINT('Ctrl Pts',(-0.197449130861913,1.74213785255918,
7.4090967987479));
#72534=CARTESIAN_POINT('Ctrl Pts',(0.194014118654607,1.74026398899783,7.42896714227067));
#72535=CARTESIAN_POINT('Ctrl Pts',(0.407495826942742,2.06839894189536,7.44883748579348));
#72536=CARTESIAN_POINT('Ctrl Pts',(0.247155589558341,2.42552356350831,7.46870782931626));
#72537=CARTESIAN_POINT('Ctrl Pts',(-0.139916254050637,2.48402463163385,
7.48857817283906));
#72538=CARTESIAN_POINT('Ctrl Pts',(-0.398633982446133,2.19023538046806,
7.50844851636183));
#72539=CARTESIAN_POINT('Ctrl Pts',(-0.291659301063552,1.81366745216059,
7.52831885988464));
#72540=CARTESIAN_POINT('Ctrl Pts',(0.0828730832164083,1.69977065583932,
7.54818920340741));
#72541=CARTESIAN_POINT('Ctrl Pts',(0.381380695796822,1.95302979648033,7.56805954693022));
#72542=CARTESIAN_POINT('Ctrl Pts',(0.33002344027702,2.34111409066416,7.587929890453));
#72543=CARTESIAN_POINT('Ctrl Pts',(-0.0240853930625828,2.50800903138302,
7.60780023397579));
#72544=CARTESIAN_POINT('Ctrl Pts',(-0.356099157197443,2.30061123122186,
7.62767057749858));
#72545=CARTESIAN_POINT('Ctrl Pts',(-0.361440423126325,1.90917993716765,
7.64754092102137));
#72546=CARTESIAN_POINT('Ctrl Pts',(-0.0352093065071765,1.69280007295633,
7.66741126454416));
#72547=CARTESIAN_POINT('Ctrl Pts',(0.323321555518063,1.84997070654329,7.68728160806695));
#72548=CARTESIAN_POINT('Ctrl Pts',(0.385248906610621,2.23650917846211,7.70715195158974));
#72549=CARTESIAN_POINT('Ctrl Pts',(0.093762832790653,2.49781906318847,7.72702229511252));
#72550=CARTESIAN_POINT('Ctrl Pts',(-0.283737875457696,2.39418411561442,
7.74689263863532));
#72551=CARTESIAN_POINT('Ctrl Pts',(-0.400947710397322,2.02067529151503,
7.7667629821581));
#72552=CARTESIAN_POINT('Ctrl Pts',(-0.150342605149271,1.71993608836669,
7.7866333256809));
#72553=CARTESIAN_POINT('Ctrl Pts',(0.238181373025728,1.76785378311253,7.80650366920368));
#72554=CARTESIAN_POINT('Ctrl Pts',(0.408206366915563,2.12047041422831,7.82637401272647));
#72555=CARTESIAN_POINT('Ctrl Pts',(0.203757591439083,2.45430822708488,7.84624435624926));
#72556=CARTESIAN_POINT('Ctrl Pts',(-0.187611035091498,2.46311647630062,
7.86611469977205));
#72557=CARTESIAN_POINT('Ctrl Pts',(-0.406872077861732,2.13881479235495,
7.88598504329484));
#72558=CARTESIAN_POINT('Ctrl Pts',(-0.252883379825488,1.77890582058044,
7.90585538681763));
#72559=CARTESIAN_POINT('Ctrl Pts',(0.133091392237208,1.71355704539811,7.92572573034042));
#72560=CARTESIAN_POINT('Ctrl Pts',(0.396972930679207,2.00271707160533,7.9455960738632));
#72561=CARTESIAN_POINT('Ctrl Pts',(0.296685848207505,2.38112094073988,7.965466417386));
#72562=CARTESIAN_POINT('Ctrl Pts',(-0.0757701098635524,2.50163461790581,
7.98533676090879));
#72563=CARTESIAN_POINT('Ctrl Pts',(-0.378717307303803,2.25370321075903,
8.00520710443158));
#72564=CARTESIAN_POINT('Ctrl Pts',(-0.334242932998583,1.8647700325435,8.02507744795437));
#72565=CARTESIAN_POINT('Ctrl Pts',(0.0168538292664106,1.69162832580094,
8.04494779147715));
#72566=CARTESIAN_POINT('Ctrl Pts',(0.352489497621136,1.89311203535275,8.06481813499996));
#72567=CARTESIAN_POINT('Ctrl Pts',(0.364764039020369,2.28438728721533,8.08468847852272));
#72568=CARTESIAN_POINT('Ctrl Pts',(0.0424172327582309,2.5065123051203,8.10455882204554));
#72569=CARTESIAN_POINT('Ctrl Pts',(-0.318841609974788,2.35571762473041,
8.1244291655683));
#72570=CARTESIAN_POINT('Ctrl Pts',(-0.387606681921568,1.97033683646142,
8.14429950909111));
#72571=CARTESIAN_POINT('Ctrl Pts',(-0.100795391090152,1.70390434869331,
8.16416985261388));
#72572=CARTESIAN_POINT('Ctrl Pts',(0.278481949013075,1.80083569744543,8.18404019613669));
#72573=CARTESIAN_POINT('Ctrl Pts',(0.402290012790745,2.17220956624924,8.20391053965947));
#72574=CARTESIAN_POINT('Ctrl Pts',(0.157051756672742,2.47734098846412,8.22378088318227));
#72575=CARTESIAN_POINT('Ctrl Pts',(-0.23226010552649,2.43631342410006,8.24365122670504));
#72576=CARTESIAN_POINT('Ctrl Pts',(-0.408504940263331,2.08676407806253,
8.26352157022785));
#72577=CARTESIAN_POINT('Ctrl Pts',(-0.21000210523437,1.74935688849456,8.28339191375062));
#72578=CARTESIAN_POINT('Ctrl Pts',(0.181149072142079,1.73361701798371,8.30326225727343));
#72579=CARTESIAN_POINT('Ctrl Pts',(0.406120637047456,2.0539836549338,8.32313260079619));
#72580=CARTESIAN_POINT('Ctrl Pts',(0.258531805794025,2.41656402392243,8.34300294431901));
#72581=CARTESIAN_POINT('Ctrl Pts',(-0.126224761348229,2.48873999726252,
8.36287328784177));
#72582=CARTESIAN_POINT('Ctrl Pts',(-0.395187293903045,2.20429994528604,
8.38274363136458));
#72583=CARTESIAN_POINT('Ctrl Pts',(-0.301619284193786,1.82417889266499,
8.40261397488735));
#72584=CARTESIAN_POINT('Ctrl Pts',(0.0686433570055766,1.69708615637076,
8.42248431841017));
#72585=CARTESIAN_POINT('Ctrl Pts',(0.375935063101534,1.93961201983962,8.44235466193292));
#72586=CARTESIAN_POINT('Ctrl Pts',(0.338357527739257,2.32927202025381,8.46222500545575));
#72587=CARTESIAN_POINT('Ctrl Pts',(-0.0096169761058694,2.5086061546522,
8.4820953489785));
#72588=CARTESIAN_POINT('Ctrl Pts',(-0.348769213606931,2.3130997688621,8.50196569250134));
#72589=CARTESIAN_POINT('Ctrl Pts',(-0.367973178264597,1.9221033560549,8.52183603602408));
#72590=CARTESIAN_POINT('Ctrl Pts',(-0.0496118468891722,1.69430289562615,
8.5417063795469));
#72591=CARTESIAN_POINT('Ctrl Pts',(0.314261599964,1.83867429778694,8.56157672306968));
#72592=CARTESIAN_POINT('Ctrl Pts',(0.389842811703776,2.22277645544637,8.58144706659247));
#72593=CARTESIAN_POINT('Ctrl Pts',(0.107796316011759,2.49424792973885,8.60131741011526));
#72594=CARTESIAN_POINT('Ctrl Pts',(-0.273138624477781,2.40405060050503,
8.62118775363805));
#72595=CARTESIAN_POINT('Ctrl Pts',(-0.403506061474943,2.03492823805935,
8.64105809716085));
#72596=CARTESIAN_POINT('Ctrl Pts',(-0.163711619458762,1.72550035847378,
8.66092844068362));
#72597=CARTESIAN_POINT('Ctrl Pts',(0.226265946086376,1.75962491646608,8.68079878420643));
#72598=CARTESIAN_POINT('Ctrl Pts',(0.408675309424305,2.10599727571742,8.7006691277292));
#72599=CARTESIAN_POINT('Ctrl Pts',(0.216180712484905,2.44686795095338,8.72053947125199));
#72600=CARTESIAN_POINT('Ctrl Pts',(-0.174630257812926,2.46953450299704,
8.74040981477478));
#72601=CARTESIAN_POINT('Ctrl Pts',(-0.405241740330249,2.15320345612076,
8.76028015829757));
#72602=CARTESIAN_POINT('Ctrl Pts',(-0.264099094775818,1.78806548125019,
8.78015050182035));
#72603=CARTESIAN_POINT('Ctrl Pts',(0.119318516390275,1.7090849612825,8.80002084534317));
#72604=CARTESIAN_POINT('Ctrl Pts',(0.393277632517502,1.98871577106116,8.81989118886592));
#72605=CARTESIAN_POINT('Ctrl Pts',(0.306458060724967,2.37043471091148,8.83976153238875));
#72606=CARTESIAN_POINT('Ctrl Pts',(-0.061495061285089,2.5040666198619,8.85963187591151));
#72607=CARTESIAN_POINT('Ctrl Pts',(-0.373034836362701,2.26702241379209,
8.87950221943433));
#72608=CARTESIAN_POINT('Ctrl Pts',(-0.34236593318474,1.87675788111643,8.89937256295709));
#72609=CARTESIAN_POINT('Ctrl Pts',(0.00237710477717516,1.69128760084632,
8.9192429064799));
#72610=CARTESIAN_POINT('Ctrl Pts',(0.344939472719621,1.88075530563092,8.93911325000267));
#72611=CARTESIAN_POINT('Ctrl Pts',(0.371066833710637,2.27135017002922,8.95898359352548));
#72612=CARTESIAN_POINT('Ctrl Pts',(0.0567908909599779,2.50475458064494,
8.97885393704825));
#72613=CARTESIAN_POINT('Ctrl Pts',(-0.309582962864796,2.36685176587936,
8.99872428057106));
#72614=CARTESIAN_POINT('Ctrl Pts',(-0.391956594175766,1.98414878450696,
9.01859462409382));
#72615=CARTESIAN_POINT('Ctrl Pts',(-0.114763410402393,1.7077235216306,9.03846496761665));
#72616=CARTESIAN_POINT('Ctrl Pts',(0.267709578787657,1.79115852403795,9.05833531113939));
#72617=CARTESIAN_POINT('Ctrl Pts',(0.404595474808187,2.15791353567016,9.07820565466223));
#72618=CARTESIAN_POINT('Ctrl Pts',(0.170320103392353,2.47154076254093,9.09807599818497));
#72619=CARTESIAN_POINT('Ctrl Pts',(-0.220200775897656,2.44432992048782,
9.1179463417078));
#72620=CARTESIAN_POINT('Ctrl Pts',(-0.408717420930249,2.10124325267291,
9.13781668523057));
#72621=CARTESIAN_POINT('Ctrl Pts',(-0.222291474111769,1.75701606978417,
9.15768702875338));
#72622=CARTESIAN_POINT('Ctrl Pts',(0.168056637952715,1.7274299498227,9.17755737227614));
#72623=CARTESIAN_POINT('Ctrl Pts',(0.4042356635409,2.03962613006664,9.19742771579896));
#72624=CARTESIAN_POINT('Ctrl Pts',(0.26958349954657,2.40720711681421,9.21729805932172));
#72625=CARTESIAN_POINT('Ctrl Pts',(-0.112374824802301,2.49296739635717,
9.23716840284454));
#72626=CARTESIAN_POINT('Ctrl Pts',(-0.391244545846019,2.21823358742262,
9.25703874636729));
#72627=CARTESIAN_POINT('Ctrl Pts',(-0.311200659211308,1.83503655807729,
9.2769090898901));
#72628=CARTESIAN_POINT('Ctrl Pts',(0.0543274661056586,1.69490741518066,
9.29677943341289));
#72629=CARTESIAN_POINT('Ctrl Pts',(0.370017537287338,1.9263955704802,9.31664977693567));
#72630=CARTESIAN_POINT('Ctrl Pts',(0.346266891346911,2.31714215575524,9.33652012045848));
#72631=CARTESIAN_POINT('Ctrl Pts',(0.00486351257623498,2.50869037435998,
9.35639046398124));
#72632=CARTESIAN_POINT('Ctrl Pts',(-0.341001476875684,2.32532081265983,
9.37626080750406));
#72633=CARTESIAN_POINT('Ctrl Pts',(-0.374044034453256,1.93525008000303,
9.39613115102683));
#72634=CARTESIAN_POINT('Ctrl Pts',(-0.0639521119170938,1.69631497026714,
9.41600149454963));
#72635=CARTESIAN_POINT('Ctrl Pts',(0.304807167009143,1.8277059185569,9.43587183807241));
#72636=CARTESIAN_POINT('Ctrl Pts',(0.393947365953243,2.20888961707887,9.45574218159522));
#72637=CARTESIAN_POINT('Ctrl Pts',(0.121694487726267,2.49018191591375,9.47561252511798));
#72638=CARTESIAN_POINT('Ctrl Pts',(-0.262196515781061,2.41353542536905,
9.49548286864081));
#72639=CARTESIAN_POINT('Ctrl Pts',(-0.405557910891673,2.04926286604208,
9.51535321216356));
#72640=CARTESIAN_POINT('Ctrl Pts',(-0.176875134483156,1.73153471988443,
9.53522355568638));
#72641=CARTESIAN_POINT('Ctrl Pts',(0.214066498438447,1.75182330621452,9.55509389920915));
#72642=CARTESIAN_POINT('Ctrl Pts',(0.408631261564984,2.09151660911612,9.57496424273194));
#72643=CARTESIAN_POINT('Ctrl Pts',(0.228332472328555,2.4389922682443,9.59483458625474));
#72644=CARTESIAN_POINT('Ctrl Pts',(-0.161430275610144,2.47548867088836,
9.61470492977751));
#72645=CARTESIAN_POINT('Ctrl Pts',(-0.40310272242407,2.16752533615898,9.63457527330032));
#72646=CARTESIAN_POINT('Ctrl Pts',(-0.274983298894178,1.79761669824813,
9.65444561682311));
#72647=CARTESIAN_POINT('Ctrl Pts',(0.10539586577539,1.70510357392534,9.67431596034588));
#72648=CARTESIAN_POINT('Ctrl Pts',(0.389088671947512,1.97485416023215,9.69418630386868));
#72649=CARTESIAN_POINT('Ctrl Pts',(0.315845591247362,2.35940901745832,9.71405664739145));
#72650=CARTESIAN_POINT('Ctrl Pts',(-0.0471428209277333,2.50599141651525,
9.73392699091427));
#72651=CARTESIAN_POINT('Ctrl Pts',(-0.366884112817172,2.28013196165989,
9.75379733443704));
#72652=CARTESIAN_POINT('Ctrl Pts',(-0.350059177958651,1.88902595473377,
9.77366767795985));
#72653=CARTESIAN_POINT('Ctrl Pts',(-0.0121026035768215,1.69145991281669,
9.79353802148261));
#72654=CARTESIAN_POINT('Ctrl Pts',(0.336956461966044,1.86867378317966,9.81340836500543));
#72655=CARTESIAN_POINT('Ctrl Pts',(0.376903846135107,2.25809796525461,9.83327870852819));
#72656=CARTESIAN_POINT('Ctrl Pts',(0.0710932623005305,2.50248878730288,
9.85314905205098));
#72657=CARTESIAN_POINT('Ctrl Pts',(-0.29993571122108,2.37765094090132,9.87301939557379));
#72658=CARTESIAN_POINT('Ctrl Pts',(-0.395814502257283,1.99810615498519,
9.89288973909658));
#72659=CARTESIAN_POINT('Ctrl Pts',(-0.128587372751106,1.71203510027575,
9.91276008261936));
#72660=CARTESIAN_POINT('Ctrl Pts',(0.25660116566415,1.78186902441152,9.93263042614216));
#72661=CARTESIAN_POINT('Ctrl Pts',(0.406393067676822,2.14354480902822,9.95250076966494));
#72662=CARTESIAN_POINT('Ctrl Pts',(0.183374655516321,2.46527415945199,9.97237111318774));
#72663=CARTESIAN_POINT('Ctrl Pts',(-0.207865038875306,2.45191419616498,
9.99224145671052));
#72664=CARTESIAN_POINT('Ctrl Pts',(-0.408416858368564,2.1157208666883,10.0121118002334));
#72665=CARTESIAN_POINT('Ctrl Pts',(-0.234301811243212,1.76510578222783,
10.0319821437561));
#72666=CARTESIAN_POINT('Ctrl Pts',(0.154753250386496,1.72171055084248,10.0518524872789));
#72667=CARTESIAN_POINT('Ctrl Pts',(0.401843272539226,2.02534438960102,10.0717228308017));
#72668=CARTESIAN_POINT('Ctrl Pts',(0.280296798158863,2.39746458745702,10.0915931743245));
#72669=CARTESIAN_POINT('Ctrl Pts',(-0.0983838295689201,2.496701522468,10.1114635178473));
#72670=CARTESIAN_POINT('Ctrl Pts',(-0.386810687416164,2.23201881665018,
10.1313338613701));
#72671=CARTESIAN_POINT('Ctrl Pts',(-0.320391399079057,1.84622681929478,
10.1512042048929));
#72672=CARTESIAN_POINT('Ctrl Pts',(0.0399433805627204,1.69323716713753,
10.1710745484156));
#72673=CARTESIAN_POINT('Ctrl Pts',(0.363635546338438,1.9133970383723,10.1909448919385));
#72674=CARTESIAN_POINT('Ctrl Pts',(0.353741602858043,2.3047397232012,10.2108152354612));
#72675=CARTESIAN_POINT('Ctrl Pts',(0.019337896326029,2.50826158478941,10.230685578984));
#72676=CARTESIAN_POINT('Ctrl Pts',(-0.332805697468255,2.3372590221293,10.2505559225068));
#72677=CARTESIAN_POINT('Ctrl Pts',(-0.3796453712399,1.94860360656475,10.2704262660296));
#72678=CARTESIAN_POINT('Ctrl Pts',(-0.0782121009491967,1.69883377121922,
10.2902966095524));
#72679=CARTESIAN_POINT('Ctrl Pts',(0.294970124346321,1.81707933692959,10.3101669530752));
#72680=CARTESIAN_POINT('Ctrl Pts',(0.397557417110412,2.19486609483677,10.330037296598));
#72681=CARTESIAN_POINT('Ctrl Pts',(0.135439902230809,2.48562612558382,10.3499076401208));
#72682=CARTESIAN_POINT('Ctrl Pts',(-0.250925284467851,2.42262668436416,
10.3697779836436));
#72683=CARTESIAN_POINT('Ctrl Pts',(-0.407100683060082,2.06366118189736,
10.3896483271663));
#72684=CARTESIAN_POINT('Ctrl Pts',(-0.189816626698134,1.73803159795637,
10.4095186706891));
#72685=CARTESIAN_POINT('Ctrl Pts',(0.20159834345907,1.7444587453422,10.4293890142119));
#72686=CARTESIAN_POINT('Ctrl Pts',(0.408074278628758,2.07704659130546,10.4492593577347));
#72687=CARTESIAN_POINT('Ctrl Pts',(0.240197617453087,2.43069106492155,10.4691297012575));
#72688=CARTESIAN_POINT('Ctrl Pts',(-0.148027657782962,2.48097150599536,
10.4890000447803));
#72689=CARTESIAN_POINT('Ctrl Pts',(-0.400457709149021,2.18176245490564,
10.5088703883031));
#72690=CARTESIAN_POINT('Ctrl Pts',(-0.285522329765078,1.80754748239312,
10.5287407318259));
#72691=CARTESIAN_POINT('Ctrl Pts',(0.0913409168230976,1.70161788096979,
10.5486110753487));
#72692=CARTESIAN_POINT('Ctrl Pts',(0.384411307169034,1.96114963892855,10.5684814188715));
#72693=CARTESIAN_POINT('Ctrl Pts',(0.324836656061238,2.3480577004006,10.5883517623942));
#72694=CARTESIAN_POINT('Ctrl Pts',(-0.0327314044652889,2.50740659176162,
10.608222105917));
#72695=CARTESIAN_POINT('Ctrl Pts',(-0.360272857373261,2.2930153985805,10.6280924494398));
#72696=CARTESIAN_POINT('Ctrl Pts',(-0.357313010361907,1.90155885387553,
10.6479627929626));
#72697=CARTESIAN_POINT('Ctrl Pts',(-0.0265671201173655,1.69214504541719,
10.6678331364854));
#72698=CARTESIAN_POINT('Ctrl Pts',(0.328550486048048,1.85688263335032,10.6877034800082));
#72699=CARTESIAN_POINT('Ctrl Pts',(0.382267749374136,2.24464730774375,10.707573823531));
#72700=CARTESIAN_POINT('Ctrl Pts',(0.0853063937042612,2.49971776923506,
10.7274441670538));
#72701=CARTESIAN_POINT('Ctrl Pts',(-0.289911964772453,2.3881015941137,10.7473145105766));
#72702=CARTESIAN_POINT('Ctrl Pts',(-0.399175563520518,2.01219142788338,
10.7671848540993));
#72703=CARTESIAN_POINT('Ctrl Pts',(-0.14224992558436,1.71683367251242,10.7870551976221));
#72704=CARTESIAN_POINT('Ctrl Pts',(0.245170653496777,1.77297885922612,10.8069255411449));
#72705=CARTESIAN_POINT('Ctrl Pts',(0.407680534965181,2.12912142269167,10.8267958846677));
#72706=CARTESIAN_POINT('Ctrl Pts',(0.196199026296186,2.45854904536132,10.8466662281905));
#72707=CARTESIAN_POINT('Ctrl Pts',(-0.19526837891403,2.45905673095678,10.8665365717133));
#72708=CARTESIAN_POINT('Ctrl Pts',(-0.407603629859947,2.13017874705938,
10.8864069152361));
#72709=CARTESIAN_POINT('Ctrl Pts',(-0.246018040632845,1.77361587120043,
10.9062772587589));
#72710=CARTESIAN_POINT('Ctrl Pts',(0.141255608542999,1.71646600032822,10.9261476022817));
#72711=CARTESIAN_POINT('Ctrl Pts',(0.398946467095265,2.01115636071566,10.9460179458045));
#72712=CARTESIAN_POINT('Ctrl Pts',(0.290658253744821,2.38734866517715,10.9658882893272));
#72713=CARTESIAN_POINT('Ctrl Pts',(-0.0842693378683556,2.49993768832696,
10.98575863285));
#72714=CARTESIAN_POINT('Ctrl Pts',(-0.381891284221727,2.24563832903655,
11.0056289763728));
#72715=CARTESIAN_POINT('Ctrl Pts',(-0.329179967105375,1.85773562972326,
11.0254993198956));
#72716=CARTESIAN_POINT('Ctrl Pts',(0.025509156024298,1.69207750882305,11.0453696634184));
#72717=CARTESIAN_POINT('Ctrl Pts',(0.356797101259684,1.90063273994518,11.0652400069412));
#72718=CARTESIAN_POINT('Ctrl Pts',(0.360772279628483,2.29208029076599,11.085110350464));
#72719=CARTESIAN_POINT('Ctrl Pts',(0.0337880061489971,2.50732032417933,
11.1049806939868));
#72720=CARTESIAN_POINT('Ctrl Pts',(-0.324192163150517,2.34889941181302,
11.1248510375096));
#72721=CARTESIAN_POINT('Ctrl Pts',(-0.384770157537106,1.96214717370342,
11.1447213810323));
#72722=CARTESIAN_POINT('Ctrl Pts',(-0.0923739141103156,1.70185613675329,
11.1645917245551));
#72723=CARTESIAN_POINT('Ctrl Pts',(0.284762819939848,1.80680789193946,11.1844620680779));
#72724=CARTESIAN_POINT('Ctrl Pts',(0.400668433652508,2.18072349176992,11.2043324116007));
#72725=CARTESIAN_POINT('Ctrl Pts',(0.14901530557076,2.48058627741254,11.2242027551235));
#72726=CARTESIAN_POINT('Ctrl Pts',(-0.239339078770172,2.43131296567223,
11.2440730986463));
#72727=CARTESIAN_POINT('Ctrl Pts',(-0.408132441412818,2.07810511211504,
11.2639434421691));
#72728=CARTESIAN_POINT('Ctrl Pts',(-0.202519851273868,1.74498283747248,
11.2838137856919));
#72729=CARTESIAN_POINT('Ctrl Pts',(0.188877131820711,1.73754047822651,11.3036841292147));
#72730=CARTESIAN_POINT('Ctrl Pts',(0.407005059769387,2.0626053857996,11.3235544727375));
#72731=CARTESIAN_POINT('Ctrl Pts',(0.251761254115174,2.42197476108452,11.3434248162603));
#72732=CARTESIAN_POINT('Ctrl Pts',(-0.134439227989904,2.48597612598004,
11.363295159783));
#72733=CARTESIAN_POINT('Ctrl Pts',(-0.397310020662451,2.19589694119357,
11.3831655033058));
#72734=CARTESIAN_POINT('Ctrl Pts',(-0.295702958252331,1.81784536805166,
11.4030358468286));
#72735=CARTESIAN_POINT('Ctrl Pts',(0.0771713120316593,1.69863225783778,
11.4229061903514));
#72736=CARTESIAN_POINT('Ctrl Pts',(0.379251409452053,1.94761940977372,11.4427765338742));
#72737=CARTESIAN_POINT('Ctrl Pts',(0.3334199691174,2.33639500849813,11.462646877397));
#72738=CARTESIAN_POINT('Ctrl Pts',(-0.0182789018524544,2.50831036919989,
11.4825172209198));
#72739=CARTESIAN_POINT('Ctrl Pts',(-0.353209368820466,2.30565655259809,
11.5023875644426));
#72740=CARTESIAN_POINT('Ctrl Pts',(-0.364118325009206,1.91434084659901,
11.5222579079654));
#72741=CARTESIAN_POINT('Ctrl Pts',(-0.0409982882357931,1.69334213863394,
11.5421282514881));
#72742=CARTESIAN_POINT('Ctrl Pts',(0.319732096581014,1.84539665700351,11.5619985950109));
#72743=CARTESIAN_POINT('Ctrl Pts',(0.38715181037918,2.23101508145708,11.5818689385337));
#72744=CARTESIAN_POINT('Ctrl Pts',(0.09941244411412,2.49644500476653,11.6017392820565));
#72745=CARTESIAN_POINT('Ctrl Pts',(-0.27952430584347,2.39819060731654,11.6216096255793));
#72746=CARTESIAN_POINT('Ctrl Pts',(-0.402035558987686,2.02638692263911,
11.6414799691021));
#72747=CARTESIAN_POINT('Ctrl Pts',(-0.155733918959777,1.72211321492475,
11.6613503126249));
#72748=CARTESIAN_POINT('Ctrl Pts',(0.233432390455118,1.76449918787656,11.6812206561477));
#72749=CARTESIAN_POINT('Ctrl Pts',(0.408456260577788,2.11466148164041,11.7010909996705));
#72750=CARTESIAN_POINT('Ctrl Pts',(0.208777117919,2.45137386197968,11.7209613431933));
#72751=CARTESIAN_POINT('Ctrl Pts',(-0.182426607992394,2.46574855918441,
11.740831686716));
#72752=CARTESIAN_POINT('Ctrl Pts',(-0.406278756210843,2.14459874550758,
11.7607020302388));
#72753=CARTESIAN_POINT('Ctrl Pts',(-0.257425455464066,1.78253565439849,
11.7805723737616));
#72754=CARTESIAN_POINT('Ctrl Pts',(0.127580655359801,1.71170288151077,11.8004427172844));
#72755=CARTESIAN_POINT('Ctrl Pts',(0.395548883428907,1.99707985295762,11.8203130608072));
#72756=CARTESIAN_POINT('Ctrl Pts',(0.300654860069938,2.37687204800306,11.84018340433));
#72757=CARTESIAN_POINT('Ctrl Pts',(-0.0700490669399977,2.50267183173139,
11.8600537478528));
#72758=CARTESIAN_POINT('Ctrl Pts',(-0.376492511351822,2.25907502866596,
11.8799240913756));
#72759=CARTESIAN_POINT('Ctrl Pts',(-0.3375553314255,1.86954854290914,11.8997944348984));
#72760=CARTESIAN_POINT('Ctrl Pts',(0.0110429110749629,1.69142989590026,
11.9196647784211));
#72761=CARTESIAN_POINT('Ctrl Pts',(0.34951078602074,1.88811869760584,11.9395351219439));
#72762=CARTESIAN_POINT('Ctrl Pts',(0.367350096389415,2.27917974922343,11.9594054654667));
#72763=CARTESIAN_POINT('Ctrl Pts',(0.048195703520538,2.50586777404869,11.9792758089895));
#72764=CARTESIAN_POINT('Ctrl Pts',(-0.315171686075873,2.36022737009233,
11.9991461525123));
#72765=CARTESIAN_POINT('Ctrl Pts',(-0.389411960448281,1.97586378083369,
12.0190164960351));
#72766=CARTESIAN_POINT('Ctrl Pts',(-0.106419774760711,1.70537827303992,
12.0388868395579));
#72767=CARTESIAN_POINT('Ctrl Pts',(0.274198066525711,1.79690447683503,12.0587571830807));
#72768=CARTESIAN_POINT('Ctrl Pts',(0.403276510470796,2.16647956040453,12.0786275266035));
#72769=CARTESIAN_POINT('Ctrl Pts',(0.162403657198292,2.47506869767777,12.0984978701262));
#72770=CARTESIAN_POINT('Ctrl Pts',(-0.227452442292167,2.43958336582408,
12.118368213649));
#72771=CARTESIAN_POINT('Ctrl Pts',(-0.408651890833478,2.0925765259275,12.1382385571718));
#72772=CARTESIAN_POINT('Ctrl Pts',(-0.214968862466393,1.75237971287771,
12.1581089006946));
#72773=CARTESIAN_POINT('Ctrl Pts',(0.175918831845622,1.73107718903387,12.1779792442174));
#72774=CARTESIAN_POINT('Ctrl Pts',(0.405424947125643,2.04821111994596,12.1978495877402));
#72775=CARTESIAN_POINT('Ctrl Pts',(0.263008867040487,2.41285429788827,12.217719931263));
#72776=CARTESIAN_POINT('Ctrl Pts',(-0.120682043130275,2.49049624878478,
12.2375902747857));
#72777=CARTESIAN_POINT('Ctrl Pts',(-0.393663608105616,2.2099110526851,12.2574606183086));
#72778=CARTESIAN_POINT('Ctrl Pts',(-0.305512405104942,1.82849742878552,
12.2773309618313));
#72779=CARTESIAN_POINT('Ctrl Pts',(0.0629048378212723,1.69615045223776,
12.2972013053541));
#72780=CARTESIAN_POINT('Ctrl Pts',(0.373615455766835,1.93428045661052,12.3170716488769));
#72781=CARTESIAN_POINT('Ctrl Pts',(0.34158475619773,2.3244355813645,12.3369419923997));
#72782=CARTESIAN_POINT('Ctrl Pts',(-0.00380345461739179,2.50870161436193,
12.3568123359225));
#72783=CARTESIAN_POINT('Ctrl Pts',(-0.345702513614639,2.31803955588287,
12.3766826794453));
#72784=CARTESIAN_POINT('Ctrl Pts',(-0.370466579517922,1.92735588828642,
12.3965530229681));
#72785=CARTESIAN_POINT('Ctrl Pts',(-0.0553779931841099,1.69504968981369,
12.4164233664909));
#72786=CARTESIAN_POINT('Ctrl Pts',(0.310512362863123,1.8342302719303,12.4362937100137));
#72787=CARTESIAN_POINT('Ctrl Pts',(0.391549898424466,2.21721839826952,12.4561640535365));
#72788=CARTESIAN_POINT('Ctrl Pts',(0.113393706886654,2.4926746020404,12.4760343970593));
#72789=CARTESIAN_POINT('Ctrl Pts',(-0.268785773560433,2.40790531625907,
12.495904740582));
#72790=CARTESIAN_POINT('Ctrl Pts',(-0.404390898644675,2.04067482033373,
12.5157750841048));
#72791=CARTESIAN_POINT('Ctrl Pts',(-0.169022427072041,1.72786710035828,
12.5356454276276));
#72792=CARTESIAN_POINT('Ctrl Pts',(0.221401111013555,1.75644065448449,12.5555157711504));
#72793=CARTESIAN_POINT('Ctrl Pts',(0.408719270783773,2.10018313673971,12.5753861146732));
#72794=CARTESIAN_POINT('Ctrl Pts',(0.221093141714138,2.44375761596807,12.595256458196));
#72795=CARTESIAN_POINT('Ctrl Pts',(-0.169355845764872,2.47198128091927,
12.6151268017188));
#72796=CARTESIAN_POINT('Ctrl Pts',(-0.404443900471156,2.15896276130563,
12.6349971452416));
#72797=CARTESIAN_POINT('Ctrl Pts',(-0.268509736560207,1.79185393524917,
12.6548674887644));
#72798=CARTESIAN_POINT('Ctrl Pts',(0.113745556344726,1.70742717330299,12.6747378322871));
#72799=CARTESIAN_POINT('Ctrl Pts',(0.391654786362965,1.98313253588689,12.6946081758099));
#72800=CARTESIAN_POINT('Ctrl Pts',(0.310274068876934,2.36604788672604,12.7144785193327));
#72801=CARTESIAN_POINT('Ctrl Pts',(-0.0557408668020039,2.50490052064318,
12.7343488628555));
#72802=CARTESIAN_POINT('Ctrl Pts',(-0.370621145626677,2.27231204909876,
12.7542192063783));
#72803=CARTESIAN_POINT('Ctrl Pts',(-0.345506978846376,1.88165073067313,
12.7740895499011));
#72804=CARTESIAN_POINT('Ctrl Pts',(-0.00343719551269503,1.69129514128672,
12.7939598934239));
#72805=CARTESIAN_POINT('Ctrl Pts',(0.341785746791939,1.87587061962627,12.8138302369467));
#72806=CARTESIAN_POINT('Ctrl Pts',(0.373466796304304,2.2660542920012,12.8337005804694));
#72807=CARTESIAN_POINT('Ctrl Pts',(0.062542903194813,2.50390575771099,12.8535709239923));
#72808=CARTESIAN_POINT('Ctrl Pts',(-0.305755589291243,2.37122867753338,
12.873441267515));
#72809=CARTESIAN_POINT('Ctrl Pts',(-0.393564953192428,1.98973621015215,
12.8933116110378));
#72810=CARTESIAN_POINT('Ctrl Pts',(-0.120332052099343,1.70939575892943,
12.9131819545606));
#72811=CARTESIAN_POINT('Ctrl Pts',(0.263289126085232,1.78738152286049,12.9330522980834));
#72812=CARTESIAN_POINT('Ctrl Pts',(0.405378372699886,2.15215218052539,12.9529226416062));
#72813=CARTESIAN_POINT('Ctrl Pts',(0.175588153428475,2.46908031220357,12.972792985129));
#72814=CARTESIAN_POINT('Ctrl Pts',(-0.215280299733418,2.44742750363098,
12.9926633286518));
#72815=CARTESIAN_POINT('Ctrl Pts',(-0.408658371617952,2.10705725759645,
13.0125336721746));
#72816=CARTESIAN_POINT('Ctrl Pts',(-0.227148048395885,1.76021294014051,
13.0324040156973));
#72817=CARTESIAN_POINT('Ctrl Pts',(0.162739737895554,1.72507698906855,13.0522743592201));
#72818=CARTESIAN_POINT('Ctrl Pts',(0.403335869369702,2.03388186554225,13.0721447027429));
#72819=CARTESIAN_POINT('Ctrl Pts',(0.273926443130965,2.403341117316,13.0920150462657));
#72820=CARTESIAN_POINT('Ctrl Pts',(-0.106773575112783,2.49452621302505,
13.1118853897885));
#72821=CARTESIAN_POINT('Ctrl Pts',(-0.389522657298515,2.22378717405302,
13.1317557333113));
#72822=CARTESIAN_POINT('Ctrl Pts',(-0.314939110772262,1.83949033997804,
13.1516260768341));
#72823=CARTESIAN_POINT('Ctrl Pts',(0.0485608540583714,1.694175490088,13.1714964203569));
#72824=CARTESIAN_POINT('Ctrl Pts',(0.367507724230662,1.92114969532342,13.1913667638797));
#72825=CARTESIAN_POINT('Ctrl Pts',(0.349326154660035,2.31219409952635,13.2112371074025));
#72826=CARTESIAN_POINT('Ctrl Pts',(0.010666392411916,2.50858047478247,13.2311074509252));
#72827=CARTESIAN_POINT('Ctrl Pts',(-0.337741731845634,2.3301476343883,13.250977794448));
#72828=CARTESIAN_POINT('Ctrl Pts',(-0.37638829909755,1.94059001290561,13.2708481379708));
#72829=CARTESIAN_POINT('Ctrl Pts',(-0.0696139978372859,1.69726097432062,
13.2907184814936));
#72830=CARTESIAN_POINT('Ctrl Pts',(0.300759554488769,1.82340645258339,13.3105888250164));
#72831=CARTESIAN_POINT('Ctrl Pts',(0.395736390676516,2.20325606000352,13.3304591685392));
#72832=CARTESIAN_POINT('Ctrl Pts',(0.126596892466422,2.48852249108309,13.3503339483527));
#72833=CARTESIAN_POINT('Ctrl Pts',(-0.128797381162466,2.44081661898851,
13.3635852803252));
#72834=CARTESIAN_POINT('Ctrl Pts',(-0.218126859843275,2.36814125324556,
13.3702131644569));
#72835=CARTESIAN_POINT('Ctrl Pts',(0.36283923412547,2.17047027618521,4.34302789673956));
#72836=CARTESIAN_POINT('Ctrl Pts',(0.339377508610394,2.29127063312973,4.34965134458049));
#72837=CARTESIAN_POINT('Ctrl Pts',(0.162686780011582,2.50549126291471,4.36289824026236));
#72838=CARTESIAN_POINT('Ctrl Pts',(-0.253693857002025,2.4562349422514,4.38276858378514));
#72839=CARTESIAN_POINT('Ctrl Pts',(-0.436454254879043,2.07954302848451,
4.40263892730793));
#72840=CARTESIAN_POINT('Ctrl Pts',(-0.219267421856341,1.72194013772262,
4.42250927083072));
#72841=CARTESIAN_POINT('Ctrl Pts',(0.199293560861417,1.71098919833492,4.44237961435351));
#72842=CARTESIAN_POINT('Ctrl Pts',(0.434912675694804,2.05698905545399,4.4622499578763));
#72843=CARTESIAN_POINT('Ctrl Pts',(0.271619417823269,2.44240078073541,4.48212030139909));
#72844=CARTESIAN_POINT('Ctrl Pts',(-0.140879241271172,2.51372967091627,
4.50199064492187));
#72845=CARTESIAN_POINT('Ctrl Pts',(-0.4241239888425,2.2055058322704,4.52186098844467));
#72846=CARTESIAN_POINT('Ctrl Pts',(-0.318301223523056,1.80050102752227,
4.54173133196746));
#72847=CARTESIAN_POINT('Ctrl Pts',(0.0795239985676654,1.67024250077846,
4.56160167549024));
#72848=CARTESIAN_POINT('Ctrl Pts',(0.404394484969609,1.93422966389774,4.58147201901304));
#72849=CARTESIAN_POINT('Ctrl Pts',(0.358289275345924,2.35028766510673,4.60134236253583));
#72850=CARTESIAN_POINT('Ctrl Pts',(-0.0164981858627633,2.53674126284983,
4.62121270605862));
#72851=CARTESIAN_POINT('Ctrl Pts',(-0.376150486643079,2.32254397230123,
4.6410830495814));
#72852=CARTESIAN_POINT('Ctrl Pts',(-0.390736090811099,1.90419300662078,
4.6609533931042));
#72853=CARTESIAN_POINT('Ctrl Pts',(-0.0468744390703233,1.66546823688044,
4.68082373662698));
#72854=CARTESIAN_POINT('Ctrl Pts',(0.339988084227034,1.82536723675285,4.70069408014978));
#72855=CARTESIAN_POINT('Ctrl Pts',(0.414957848761605,2.23720439184066,4.72056442367256));
#72856=CARTESIAN_POINT('Ctrl Pts',(0.109260266361431,2.52317520503028,4.74043476719535));
#72857=CARTESIAN_POINT('Ctrl Pts',(-0.29666872969806,2.42094037307327,4.76030511071814));
#72858=CARTESIAN_POINT('Ctrl Pts',(-0.43044455732329,2.02428644331352,4.78017545424093));
#72859=CARTESIAN_POINT('Ctrl Pts',(-0.169346101645197,1.6970893930947,4.80004579776372));
#72860=CARTESIAN_POINT('Ctrl Pts',(0.24710434702284,1.73950797403383,4.81991614128651));
#72861=CARTESIAN_POINT('Ctrl Pts',(0.436870197973242,2.1126289119025,4.8397864848093));
#72862=CARTESIAN_POINT('Ctrl Pts',(0.225867116553052,2.47416454254653,4.85965682833209));
#72863=CARTESIAN_POINT('Ctrl Pts',(-0.192338295150169,2.49245514321617,
4.87952717185488));
#72864=CARTESIAN_POINT('Ctrl Pts',(-0.434099505611459,2.15072157797534,
4.89939751537767));
#72865=CARTESIAN_POINT('Ctrl Pts',(-0.277633516952299,1.76245787003698,
4.91926785890046));
#72866=CARTESIAN_POINT('Ctrl Pts',(0.133523427103024,1.68384311414085,4.93913820242324));
#72867=CARTESIAN_POINT('Ctrl Pts',(0.422190804373444,1.98699564636976,4.95900854594604));
#72868=CARTESIAN_POINT('Ctrl Pts',(0.32355559471455,2.39381428890427,4.97887888946882));
#72869=CARTESIAN_POINT('Ctrl Pts',(-0.0718978249758275,2.53109832057086,
4.99874923299162));
#72870=CARTESIAN_POINT('Ctrl Pts',(-0.401394778257155,2.27290833185141,
5.0186195765144));
#72871=CARTESIAN_POINT('Ctrl Pts',(-0.362666667451549,1.8560984880016,5.0384899200372));
#72872=CARTESIAN_POINT('Ctrl Pts',(0.0087587381320539,1.66303507721802,
5.05836026355998));
#72873=CARTESIAN_POINT('Ctrl Pts',(0.372149193874197,1.87082749568422,5.07823060708277));
#72874=CARTESIAN_POINT('Ctrl Pts',(0.394143427774538,2.28885448784099,5.09810095060557));
#72875=CARTESIAN_POINT('Ctrl Pts',(0.0545647244742198,2.53363319762053,
5.11797129412835));
#72876=CARTESIAN_POINT('Ctrl Pts',(-0.335069685214756,2.38061248241239,
5.13784163765114));
#72877=CARTESIAN_POINT('Ctrl Pts',(-0.417323274337762,1.97016801653074,
5.15771198117393));
#72878=CARTESIAN_POINT('Ctrl Pts',(-0.116739572689465,1.67882672045364,
5.17758232469673));
#72879=CARTESIAN_POINT('Ctrl Pts',(0.290936794243693,1.77385457079585,5.19745266821951));
#72880=CARTESIAN_POINT('Ctrl Pts',(0.431718259926271,2.16807645174203,5.2173230117423));
#72881=CARTESIAN_POINT('Ctrl Pts',(0.176456995260411,2.49984745598693,5.23719335526509));
#72882=CARTESIAN_POINT('Ctrl Pts',(-0.240679540106183,2.46481285367957,
5.25706369878788));
#72883=CARTESIAN_POINT('Ctrl Pts',(-0.437025362986032,2.09511212290653,
5.27693404231066));
#72884=CARTESIAN_POINT('Ctrl Pts',(-0.232459910956952,1.72989535394238,
5.29680438583346));
#72885=CARTESIAN_POINT('Ctrl Pts',(0.185355862815914,1.70419921253827,5.31667472935624));
#72886=CARTESIAN_POINT('Ctrl Pts',(0.433132866377297,2.04159641021874,5.33654507287904));
#72887=CARTESIAN_POINT('Ctrl Pts',(0.283569430752704,2.43257095059271,5.35641541640182));
#72888=CARTESIAN_POINT('Ctrl Pts',(-0.126130353095458,2.51845691924446,
5.37628575992461));
#72889=CARTESIAN_POINT('Ctrl Pts',(-0.420122709075573,2.22046563225483,
5.39615610344741));
#72890=CARTESIAN_POINT('Ctrl Pts',(-0.328709674021062,1.81196352758631,
5.41602644697019));
#72891=CARTESIAN_POINT('Ctrl Pts',(0.0642497371665301,1.66769567373251,
5.43589679049298));
#72892=CARTESIAN_POINT('Ctrl Pts',(0.398268761315715,1.92000818630949,5.45576713401577));
#72893=CARTESIAN_POINT('Ctrl Pts',(0.36693041635361,2.33743868427474,5.47563747753856));
#72894=CARTESIAN_POINT('Ctrl Pts',(-0.0010166325474728,2.53705151377592,
5.49550782106136));
#72895=CARTESIAN_POINT('Ctrl Pts',(-0.368031059488272,2.33572907857855,
5.51537816458414));
#72896=CARTESIAN_POINT('Ctrl Pts',(-0.397427092253076,1.91815730540157,
5.53524850810693));
#72897=CARTESIAN_POINT('Ctrl Pts',(-0.0622378726886654,1.66740144887119,
5.55511885162973));
#72898=CARTESIAN_POINT('Ctrl Pts',(0.330046122146328,1.81349587002676,5.57498919515251));
#72899=CARTESIAN_POINT('Ctrl Pts',(0.419557731634292,2.22241882641751,5.5948595386753));
#72900=CARTESIAN_POINT('Ctrl Pts',(0.124182239975273,2.5190391753885,5.61472988219809));
#72901=CARTESIAN_POINT('Ctrl Pts',(-0.285113550975675,2.43124812797297,
5.63460022572088));
#72902=CARTESIAN_POINT('Ctrl Pts',(-0.432856473611466,2.03958201850278,
5.65447056924367));
#72903=CARTESIAN_POINT('Ctrl Pts',(-0.183512509796454,1.70334118189083,
5.67434091276646));
#72904=CARTESIAN_POINT('Ctrl Pts',(0.234179198784542,1.73098081067215,5.69421125628924));
#72905=CARTESIAN_POINT('Ctrl Pts',(0.437043373099837,2.09714530823555,5.71408159981204));
#72906=CARTESIAN_POINT('Ctrl Pts',(0.238979750678643,2.46592859686164,5.73395194333482));
#72907=CARTESIAN_POINT('Ctrl Pts',(-0.178315258834963,2.49902221454723,
5.75382228685762));
#72908=CARTESIAN_POINT('Ctrl Pts',(-0.432030293797926,2.16606727235501,
5.7736926303804));
#72909=CARTESIAN_POINT('Ctrl Pts',(-0.289416349814782,1.77250460202403,
5.7935629739032));
#72910=CARTESIAN_POINT('Ctrl Pts',(0.118697694645232,1.67937437486351,5.81343331742598));
#72911=CARTESIAN_POINT('Ctrl Pts',(0.417922763500204,1.97211089575767,5.83330366094877));
#72912=CARTESIAN_POINT('Ctrl Pts',(0.333760591890408,2.38216825926478,5.85317400447156));
#72913=CARTESIAN_POINT('Ctrl Pts',(-0.0565814853772176,2.53337465863622,
5.87304434799435));
#72914=CARTESIAN_POINT('Ctrl Pts',(-0.395017752684917,2.28701880734116,
5.89291469151714));
#72915=CARTESIAN_POINT('Ctrl Pts',(-0.371079008715224,1.86909866062216,
5.91278503503993));
#72916=CARTESIAN_POINT('Ctrl Pts',(-0.00672579209462177,1.66299905840347,
5.93265537856272));
#72917=CARTESIAN_POINT('Ctrl Pts',(0.363797423138882,1.85778832779351,5.95252572208551));
#72918=CARTESIAN_POINT('Ctrl Pts',(0.400586029189409,2.27477383229139,5.9723960656083));
#72919=CARTESIAN_POINT('Ctrl Pts',(0.069891488322067,2.53142813897064,5.99226640913109));
#72920=CARTESIAN_POINT('Ctrl Pts',(-0.324918978213823,2.39230586178187,
6.01213675265388));
#72921=CARTESIAN_POINT('Ctrl Pts',(-0.421660515963138,1.98503275025794,
6.03200709617666));
#72922=CARTESIAN_POINT('Ctrl Pts',(-0.131585934211991,1.68322643899462,
6.05187743969946));
#72923=CARTESIAN_POINT('Ctrl Pts',(0.279200828371318,1.76375313135685,6.07174778322224));
#72924=CARTESIAN_POINT('Ctrl Pts',(0.433858840684473,2.15274054982154,6.09161812674504));
#72925=CARTESIAN_POINT('Ctrl Pts',(0.190510431217294,2.49334569380248,6.11148847026782));
#72926=CARTESIAN_POINT('Ctrl Pts',(-0.227605363238513,2.4731097129004,6.13135881379061));
#72927=CARTESIAN_POINT('Ctrl Pts',(-0.436924222595204,2.11059636471292,
6.15122915731341));
#72928=CARTESIAN_POINT('Ctrl Pts',(-0.245424589582531,1.73836229446614,
6.17109950083618));
#72929=CARTESIAN_POINT('Ctrl Pts',(0.171218692831284,1.69788158651872,6.19096984435899));
#72930=CARTESIAN_POINT('Ctrl Pts',(0.430792133892607,2.02628977946169,6.21084018788177));
#72931=CARTESIAN_POINT('Ctrl Pts',(0.295172439160706,2.42231706500815,6.23071053140457));
#72932=CARTESIAN_POINT('Ctrl Pts',(-0.111227784402149,2.52266232291576,
6.25058087492735));
#72933=CARTESIAN_POINT('Ctrl Pts',(-0.415591658071537,2.23527243982757,
6.27045121845014));
#72934=CARTESIAN_POINT('Ctrl Pts',(-0.338706763155614,1.82378850887735,
6.29032156197293));
#72935=CARTESIAN_POINT('Ctrl Pts',(0.0488954761935535,1.66569101823315,
6.31019190549572));
#72936=CARTESIAN_POINT('Ctrl Pts',(0.391642772653139,1.90601289253119,6.33006224901851));
#72937=CARTESIAN_POINT('Ctrl Pts',(0.375111142552447,2.3242915289719,6.3499325925413));
#72938=CARTESIAN_POINT('Ctrl Pts',(0.0144661059306473,2.53681322211531,
6.36980293606408));
#72939=CARTESIAN_POINT('Ctrl Pts',(-0.359449613500031,2.34861825071831,
6.38967327958688));
#72940=CARTESIAN_POINT('Ctrl Pts',(-0.403619247190546,1.93234988060579,
6.40954362310967));
#72941=CARTESIAN_POINT('Ctrl Pts',(-0.0775231693824896,1.66987767153466,
6.42941396663246));
#72942=CARTESIAN_POINT('Ctrl Pts',(0.31968986250749,1.80198414296301,6.44928431015524));
#72943=CARTESIAN_POINT('Ctrl Pts',(0.423630967391639,2.20747959202741,6.46915465367804));
#72944=CARTESIAN_POINT('Ctrl Pts',(0.138948331842413,2.51437714743185,6.48902499720083));
#72945=CARTESIAN_POINT('Ctrl Pts',(-0.273200482064957,2.4411400824222,6.50889534072361));
#72946=CARTESIAN_POINT('Ctrl Pts',(-0.43472504656487,2.05495343381872,6.52876568424641));
#72947=CARTESIAN_POINT('Ctrl Pts',(-0.197448563312467,1.71009087715033,
6.54863602776919));
#72948=CARTESIAN_POINT('Ctrl Pts',(0.220960096584491,1.72291685936265,6.56850637129198));
#72949=CARTESIAN_POINT('Ctrl Pts',(0.436667948866037,2.08166528787568,6.58837671481477));
#72950=CARTESIAN_POINT('Ctrl Pts',(0.25179240503621,2.4572333187171,6.60824705833756));
#72951=CARTESIAN_POINT('Ctrl Pts',(-0.164068391973716,2.50508841256041,
6.62811740186035));
#72952=CARTESIAN_POINT('Ctrl Pts',(-0.429418775242406,2.1813300356871,6.64798774538314));
#72953=CARTESIAN_POINT('Ctrl Pts',(-0.300835892313531,1.78296242315543,
6.66785808890593));
#72954=CARTESIAN_POINT('Ctrl Pts',(0.103722966704488,1.67543362660996,6.68772843242871));
#72955=CARTESIAN_POINT('Ctrl Pts',(0.413130124377974,1.95738667815736,6.70759877595151));
#72956=CARTESIAN_POINT('Ctrl Pts',(0.343546635522439,2.37016803744478,6.72746911947429));
#72957=CARTESIAN_POINT('Ctrl Pts',(-0.0411941217737742,2.5351070024337,
6.74733946299709));
#72958=CARTESIAN_POINT('Ctrl Pts',(-0.388144880415828,2.30089452715924,
6.76720980651987));
#72959=CARTESIAN_POINT('Ctrl Pts',(-0.379025552430303,1.88238867253643,
6.78708015004267));
#72960=CARTESIAN_POINT('Ctrl Pts',(-0.0222018797595282,1.66351158575433,
6.80695049356545));
#72961=CARTESIAN_POINT('Ctrl Pts',(0.354988995077618,1.84505319651085,6.82682083708825));
#72962=CARTESIAN_POINT('Ctrl Pts',(0.406525794318799,2.26047379159546,6.84669118061103));
#72963=CARTESIAN_POINT('Ctrl Pts',(0.0851305207618968,2.52868152942523,
6.86656152413383));
#72964=CARTESIAN_POINT('Ctrl Pts',(-0.314360416120161,2.40363232372775,
6.88643186765661));
#72965=CARTESIAN_POINT('Ctrl Pts',(-0.425468467518153,2.00004179681833,
6.9063022111794));
#72966=CARTESIAN_POINT('Ctrl Pts',(-0.146267122269751,1.68814931324754,
6.92617255470219));
#72967=CARTESIAN_POINT('Ctrl Pts',(0.267114395190533,1.75407376636406,6.94604289822498));
#72968=CARTESIAN_POINT('Ctrl Pts',(0.435454819404735,2.13733844523737,6.96591324174778));
#72969=CARTESIAN_POINT('Ctrl Pts',(0.204324728635643,2.4863501837757,6.98578358527055));
#72970=CARTESIAN_POINT('Ctrl Pts',(-0.214245484356636,2.48093822552789,
7.00565392879336));
#72971=CARTESIAN_POINT('Ctrl Pts',(-0.43627463234065,2.12606730541472,7.02552427231613));
#72972=CARTESIAN_POINT('Ctrl Pts',(-0.258081198580122,1.74728318132671,
7.04539461583893));
#72973=CARTESIAN_POINT('Ctrl Pts',(0.156866600295109,1.6920687203126,7.06526495936172));
#72974=CARTESIAN_POINT('Ctrl Pts',(0.427910648858824,2.01107567358268,7.08513530288451));
#72975=CARTESIAN_POINT('Ctrl Pts',(0.306404931869047,2.41165859038679,7.1050056464073));
#72976=CARTESIAN_POINT('Ctrl Pts',(-0.0961855968457871,2.52633717899683,
7.12487598993008));
#72977=CARTESIAN_POINT('Ctrl Pts',(-0.410538934941196,2.24990944644317,
7.14474633345288));
#72978=CARTESIAN_POINT('Ctrl Pts',(-0.348278690057241,1.83596020510619,
7.16461667697566));
#72979=CARTESIAN_POINT('Ctrl Pts',(0.0334798390920258,1.66423152981207,
7.18448702049846));
#72980=CARTESIAN_POINT('Ctrl Pts',(0.384525173742875,1.89226110139513,7.20435736402124));
#72981=CARTESIAN_POINT('Ctrl Pts',(0.382821009860021,2.31086283135087,7.22422770754404));
#72982=CARTESIAN_POINT('Ctrl Pts',(0.0299306858050187,2.53602661992451,
7.24409805106682));
#72983=CARTESIAN_POINT('Ctrl Pts',(-0.350416967781163,2.36119534438158,
7.26396839458962));
#72984=CARTESIAN_POINT('Ctrl Pts',(-0.40930475839056,1.94675289890377,7.2838387381124));
#72985=CARTESIAN_POINT('Ctrl Pts',(-0.092711154987836,1.67289380597283,
7.30370908163519));
#72986=CARTESIAN_POINT('Ctrl Pts',(0.308932311632189,1.79084650080398,7.32357942515799));
#72987=CARTESIAN_POINT('Ctrl Pts',(0.427172439666159,2.19240544369902,7.34344976868076));
#72988=CARTESIAN_POINT('Ctrl Pts',(0.153540008582802,2.50919497186543,7.36332011220357));
#72989=CARTESIAN_POINT('Ctrl Pts',(-0.260944477790598,2.45060382021043,
7.38319045572634));
#72990=CARTESIAN_POINT('Ctrl Pts',(-0.436047930173949,2.07038139391246,
7.40306079924915));
#72991=CARTESIAN_POINT('Ctrl Pts',(-0.211136769187992,1.7173300064907,7.42293114277192));
#72992=CARTESIAN_POINT('Ctrl Pts',(0.207463633852353,1.71532624229832,7.44280148629472));
#72993=CARTESIAN_POINT('Ctrl Pts',(0.435744396456537,2.06620828219398,7.46267182981751));
#72994=CARTESIAN_POINT('Ctrl Pts',(0.264288996554756,2.44808962284968,7.48254217334029));
#72995=CARTESIAN_POINT('Ctrl Pts',(-0.149615577988074,2.51064612266384,
7.5024125168631));
#72996=CARTESIAN_POINT('Ctrl Pts',(-0.426268228048542,2.1964907093554,7.52228286038586));
#72997=CARTESIAN_POINT('Ctrl Pts',(-0.31187781005355,1.79381820623728,7.54215320390868));
#72998=CARTESIAN_POINT('Ctrl Pts',(0.0886180403356958,1.67202581600918,
7.56202354743145));
#72999=CARTESIAN_POINT('Ctrl Pts',(0.407818902973736,1.94284147616865,7.58189389095424));
#73000=CARTESIAN_POINT('Ctrl Pts',(0.352901441663641,2.35782868674233,7.60176423447703));
#73001=CARTESIAN_POINT('Ctrl Pts',(-0.025755049179834,2.53629317743611,
7.62163457799982));
#73002=CARTESIAN_POINT('Ctrl Pts',(-0.380784788634143,2.31451807378494,
7.64150492152262));
#73003=CARTESIAN_POINT('Ctrl Pts',(-0.386496323684559,1.89595184143474,
7.66137526504539));
#73004=CARTESIAN_POINT('Ctrl Pts',(-0.037650098477609,1.66457201591976,
7.68124560856821));
#73005=CARTESIAN_POINT('Ctrl Pts',(0.345734966484481,1.83263808763114,7.70111595209096));
#73006=CARTESIAN_POINT('Ctrl Pts',(0.411955267262573,2.24597231590331,7.72098629561378));
#73007=CARTESIAN_POINT('Ctrl Pts',(0.10026269297267,2.52539681667053,7.74085663913655));
#73008=CARTESIAN_POINT('Ctrl Pts',(-0.303407252586554,2.41457765068967,
7.76072698265935));
#73009=CARTESIAN_POINT('Ctrl Pts',(-0.428742349065226,2.01517631608103,
7.78059732618214));
#73010=CARTESIAN_POINT('Ctrl Pts',(-0.160764708276792,1.69358916376624,
7.80046766970493));
#73011=CARTESIAN_POINT('Ctrl Pts',(0.254692666216871,1.74482862585662,7.82033801322772));
#73012=CARTESIAN_POINT('Ctrl Pts',(0.436504192732088,2.12188947150714,7.8402083567505));
#73013=CARTESIAN_POINT('Ctrl Pts',(0.217882547095443,2.47886970703232,7.8600787002733));
#73014=CARTESIAN_POINT('Ctrl Pts',(-0.200616673470941,2.48828856480845,
7.87994904379608));
#73015=CARTESIAN_POINT('Ctrl Pts',(-0.435077407621625,2.14150552508765,
7.89981938731887));
#73016=CARTESIAN_POINT('Ctrl Pts',(-0.270413850720044,1.75664681656592,
7.91968973084166));
#73017=CARTESIAN_POINT('Ctrl Pts',(0.142317600695636,1.68676791052994,7.93956007436446));
#73018=CARTESIAN_POINT('Ctrl Pts',(0.424492028264872,1.99597319011368,7.95943041788724));
#73019=CARTESIAN_POINT('Ctrl Pts',(0.3172528092724,2.40060890579676,7.97930076141003));
#73020=CARTESIAN_POINT('Ctrl Pts',(-0.0810226721575523,2.52947687461842,
7.99917110493282));
#73021=CARTESIAN_POINT('Ctrl Pts',(-0.404970882123739,2.26435827897454,
8.01904144845561));
#73022=CARTESIAN_POINT('Ctrl Pts',(-0.357413439548636,1.84846333773073,
8.03891179197839));
#73023=CARTESIAN_POINT('Ctrl Pts',(0.0180221763662852,1.66331904049457,
8.05878213550118));
#73024=CARTESIAN_POINT('Ctrl Pts',(0.376924898962899,1.8787700748602,8.07865247902397));
#73025=CARTESIAN_POINT('Ctrl Pts',(0.390050340452458,2.29716944780689,8.09852282254676));
#73026=CARTESIAN_POINT('Ctrl Pts',(0.0453576951357961,2.53469269458724,
8.11839316606954));
#73027=CARTESIAN_POINT('Ctrl Pts',(-0.340944460575358,2.37344457215043,
8.13826350959235));
#73028=CARTESIAN_POINT('Ctrl Pts',(-0.414476489105645,1.9613482808826,8.15813385311513));
#73029=CARTESIAN_POINT('Ctrl Pts',(-0.10778276476028,1.67644606617789,8.17800419663793));
#73030=CARTESIAN_POINT('Ctrl Pts',(0.297786972954211,1.78009692409369,8.19787454016071));
#73031=CARTESIAN_POINT('Ctrl Pts',(0.430177703018842,2.17721530328235,8.21774488368351));
#73032=CARTESIAN_POINT('Ctrl Pts',(0.16793895396972,2.50349915362378,8.23761522720629));
#73033=CARTESIAN_POINT('Ctrl Pts',(-0.248360922522535,2.45962746196489,
8.25748557072909));
#73034=CARTESIAN_POINT('Ctrl Pts',(-0.436823463886832,2.0858465328112,8.27735591425187));
#73035=CARTESIAN_POINT('Ctrl Pts',(-0.224559945279632,1.72504948298268,
8.29722625777467));
#73036=CARTESIAN_POINT('Ctrl Pts',(0.193706752045623,1.70821848761396,8.31709660129744));
#73037=CARTESIAN_POINT('Ctrl Pts',(0.434273875162049,2.05079369362276,8.33696694482025));
#73038=CARTESIAN_POINT('Ctrl Pts',(0.276453838866806,2.43850898689895,8.35683728834301));
#73039=CARTESIAN_POINT('Ctrl Pts',(-0.134974958797051,2.5156883685326,8.37670763186583));
#73040=CARTESIAN_POINT('Ctrl Pts',(-0.422582606945993,2.21153026289883,
8.39657797538859));
#73041=CARTESIAN_POINT('Ctrl Pts',(-0.322528242649051,1.80505832452963,
8.4164483189114));
#73042=CARTESIAN_POINT('Ctrl Pts',(0.0734018760230442,1.66915522072114,
8.43631866243417));
#73043=CARTESIAN_POINT('Ctrl Pts',(0.401995766207075,1.92849354768073,8.45618900595698));
#73044=CARTESIAN_POINT('Ctrl Pts',(0.361813267677896,2.34516569614813,8.47605934947975));
#73045=CARTESIAN_POINT('Ctrl Pts',(-0.0102836475171846,2.53693169469529,
8.49592969300256));
#73046=CARTESIAN_POINT('Ctrl Pts',(-0.372946716107436,2.32787234623849,
8.51580003652532));
#73047=CARTESIAN_POINT('Ctrl Pts',(-0.393481944779828,1.90977114212655,
8.53567038004815));
#73048=CARTESIAN_POINT('Ctrl Pts',(-0.0530510568463816,1.66617901779301,
8.55554072357091));
#73049=CARTESIAN_POINT('Ctrl Pts',(0.336046953494394,1.82055858524068,8.57541106709373));
#73050=CARTESIAN_POINT('Ctrl Pts',(0.416867632665708,2.23128760821661,8.5952814106165));
#73051=CARTESIAN_POINT('Ctrl Pts',(0.115269010269813,2.52157812384773,8.6151517541393));
#73052=CARTESIAN_POINT('Ctrl Pts',(-0.292073236589911,2.4251281035276,8.63502209766208));
#73053=CARTESIAN_POINT('Ctrl Pts',(-0.43147805105905,2.03041731041534,8.65489244118488));
#73054=CARTESIAN_POINT('Ctrl Pts',(-0.175060494113946,1.69953916216922,
8.67476278470766));
#73055=CARTESIAN_POINT('Ctrl Pts',(0.241951233846475,1.73602931481269,8.69463312823044));
#73056=CARTESIAN_POINT('Ctrl Pts',(0.437005643438904,2.10641302098108,8.71450347175325));
#73057=CARTESIAN_POINT('Ctrl Pts',(0.231166868122316,2.47091365345329,8.73437381527603));
#73058=CARTESIAN_POINT('Ctrl Pts',(-0.186736038169164,2.49515150421634,
8.75424415879882));
#73059=CARTESIAN_POINT('Ctrl Pts',(-0.433334051256465,2.15689164488053,
8.77411450232161));
#73060=CARTESIAN_POINT('Ctrl Pts',(-0.282407065419999,1.76644144646492,
8.7939848458444));
#73061=CARTESIAN_POINT('Ctrl Pts',(0.127589956689025,1.68198581102115,8.81385518936719));
#73062=CARTESIAN_POINT('Ctrl Pts',(0.420540563339994,1.98100128647235,8.83372553288998));
#73063=CARTESIAN_POINT('Ctrl Pts',(0.32770245455445,2.3891818813732,8.85359587641274));
#73064=CARTESIAN_POINT('Ctrl Pts',(-0.0657580436241065,2.53207746867233,
8.87346621993558));
#73065=CARTESIAN_POINT('Ctrl Pts',(-0.398894488926811,2.27860080050036,
8.89333656345832));
#73066=CARTESIAN_POINT('Ctrl Pts',(-0.366099545220169,1.86128221217274,
8.91320690698115));
#73067=CARTESIAN_POINT('Ctrl Pts',(0.00254189127341255,1.6629546956844,
8.93307725050391));
#73068=CARTESIAN_POINT('Ctrl Pts',(0.368851488570885,1.86555674756011,8.95294759402671));
#73069=CARTESIAN_POINT('Ctrl Pts',(0.396790059700396,2.28322856698263,8.97281793754949));
#73070=CARTESIAN_POINT('Ctrl Pts',(0.0607277691436284,2.53281312051553,
8.9926882810723));
#73071=CARTESIAN_POINT('Ctrl Pts',(-0.331043982263186,2.38535055816115,
9.01255862459509));
#73072=CARTESIAN_POINT('Ctrl Pts',(-0.419127947512142,1.97611770566457,
9.03242896811786));
#73073=CARTESIAN_POINT('Ctrl Pts',(-0.122719080036365,1.68052999316926,
9.05229931164065));
#73074=CARTESIAN_POINT('Ctrl Pts',(0.286267836678638,1.76974890625633,9.07216965516346));
#73075=CARTESIAN_POINT('Ctrl Pts',(0.432642985087817,2.16192823822663,9.09203999868623));
#73076=CARTESIAN_POINT('Ctrl Pts',(0.182127093702806,2.49729684239233,9.11191034220904));
#73077=CARTESIAN_POINT('Ctrl Pts',(-0.235465611789637,2.46819968074414,
9.13178068573181));
#73078=CARTESIAN_POINT('Ctrl Pts',(-0.437050674213524,2.1013294378734,9.15165102925462));
#73079=CARTESIAN_POINT('Ctrl Pts',(-0.237701242123064,1.73323961674043,
9.17152137277738));
#73080=CARTESIAN_POINT('Ctrl Pts',(0.179706719513284,1.70160251733058,9.1913917163002));
#73081=CARTESIAN_POINT('Ctrl Pts',(0.432258230856898,2.03544087135022,9.21126205982296));
#73082=CARTESIAN_POINT('Ctrl Pts',(0.288271662033624,2.42850343697429,9.23113240334578));
#73083=CARTESIAN_POINT('Ctrl Pts',(-0.120164912062476,2.52020882087906,
9.25100274686855));
#73084=CARTESIAN_POINT('Ctrl Pts',(-0.418366538316829,2.22642981789257,
9.27087309039134));
#73085=CARTESIAN_POINT('Ctrl Pts',(-0.332773821126645,1.81666866885512,
9.29074343391414));
#73086=CARTESIAN_POINT('Ctrl Pts',(0.0580935738823234,1.66682544406541,
9.3106137774369));
#73087=CARTESIAN_POINT('Ctrl Pts',(0.395668023580192,1.91436090295496,9.33048412095972));
#73088=CARTESIAN_POINT('Ctrl Pts',(0.370270926980643,2.33219496090236,9.35035446448248));
#73089=CARTESIAN_POINT('Ctrl Pts',(0.00520066271126297,2.53702175271137,
9.3702248080053));
#73090=CARTESIAN_POINT('Ctrl Pts',(-0.364640501589402,2.34094058154696,
9.39009515152806));
#73091=CARTESIAN_POINT('Ctrl Pts',(-0.399973647003501,1.92382922791146,
9.40996549505088));
#73092=CARTESIAN_POINT('Ctrl Pts',(-0.068385422787009,1.66833057418229,
9.42983583857364));
#73093=CARTESIAN_POINT('Ctrl Pts',(0.32593711700193,1.80882985215509,9.44970618209645));
#73094=CARTESIAN_POINT('Ctrl Pts',(0.421256724273288,2.21643810153937,9.46957652561924));
#73095=CARTESIAN_POINT('Ctrl Pts',(0.130130635948347,2.51723024437741,9.48944686914203));
#73096=CARTESIAN_POINT('Ctrl Pts',(-0.280372595172832,2.43527043876788,
9.50931721266481));
#73097=CARTESIAN_POINT('Ctrl Pts',(-0.433672139505111,2.04574564853753,
9.52918755618761));
#73098=CARTESIAN_POINT('Ctrl Pts',(-0.189136534972047,1.70599183971101,
9.5490578997104));
#73099=CARTESIAN_POINT('Ctrl Pts',(0.228906091783717,1.72768687858221,9.56892824323319));
#73100=CARTESIAN_POINT('Ctrl Pts',(0.436958542078337,2.09092852049966,9.58879858675598));
#73101=CARTESIAN_POINT('Ctrl Pts',(0.244161016550001,2.46249200988825,9.60866893027878));
#73102=CARTESIAN_POINT('Ctrl Pts',(-0.172621002142068,2.50151842903535,
9.62853927380154));
#73103=CARTESIAN_POINT('Ctrl Pts',(-0.431046751596171,2.17220635134072,
9.64840961732437));
#73104=CARTESIAN_POINT('Ctrl Pts',(-0.294045788177107,1.77665477629806,
9.66827996084712));
#73105=CARTESIAN_POINT('Ctrl Pts',(0.112702155175145,1.67772842452465,9.68815030436993));
#73106=CARTESIAN_POINT('Ctrl Pts',(0.416061214167159,1.96617875616592,9.7080206478927));
#73107=CARTESIAN_POINT('Ctrl Pts',(0.337740750780422,2.37739186090769,9.72789099141552));
#73108=CARTESIAN_POINT('Ctrl Pts',(-0.0504108721960329,2.5341356967585,
9.74776133493826));
#73109=CARTESIAN_POINT('Ctrl Pts',(-0.392317382753171,2.2926191330716,9.7676316784611));
#73110=CARTESIAN_POINT('Ctrl Pts',(-0.374326103823116,1.87440073751858,
9.78750202198385));
#73111=CARTESIAN_POINT('Ctrl Pts',(-0.0129415845327464,1.663138952726,9.80737236550666));
#73112=CARTESIAN_POINT('Ctrl Pts',(0.360315076728777,1.85263770554612,9.82724270902943));
#73113=CARTESIAN_POINT('Ctrl Pts',(0.403031707559942,2.26905768819215,9.84711305255224));
#73114=CARTESIAN_POINT('Ctrl Pts',(0.0760216145173189,2.53039025704787,
9.86698339607502));
#73115=CARTESIAN_POINT('Ctrl Pts',(-0.320727960436671,2.39689835740483,
9.88685373959781));
#73116=CARTESIAN_POINT('Ctrl Pts',(-0.423253294859077,1.99104263390441,
9.9067240831206));
#73117=CARTESIAN_POINT('Ctrl Pts',(-0.137501351981262,1.68514046059072,
9.92659442664338));
#73118=CARTESIAN_POINT('Ctrl Pts',(0.27438936222061,1.75981543665868,9.94646477016618));
#73119=CARTESIAN_POINT('Ctrl Pts',(0.434565191323634,2.14656343764594,9.96633511368898));
#73120=CARTESIAN_POINT('Ctrl Pts',(0.196086618095845,2.49059582363268,9.98620545721174));
#73121=CARTESIAN_POINT('Ctrl Pts',(-0.222274732452348,2.47630971625616,
10.0060758007345));
#73122=CARTESIAN_POINT('Ctrl Pts',(-0.436729275947876,2.11681067415645,
10.0259461442573));
#73123=CARTESIAN_POINT('Ctrl Pts',(-0.250544164083381,1.74189012708484,
10.0458164877801));
#73124=CARTESIAN_POINT('Ctrl Pts',(0.165481109819656,1.69548663615597,10.0656868313029));
#73125=CARTESIAN_POINT('Ctrl Pts',(0.429699993681973,2.02016908703226,10.0855571748257));
#73126=CARTESIAN_POINT('Ctrl Pts',(0.299727631712863,2.41808553255901,10.1054275183485));
#73127=CARTESIAN_POINT('Ctrl Pts',(-0.105204028120338,2.52420180539787,
10.1252978618713));
#73128=CARTESIAN_POINT('Ctrl Pts',(-0.413625314388266,2.2411706716452,10.1451682053941));
#73129=CARTESIAN_POINT('Ctrl Pts',(-0.342601684706765,1.82863466530959,
10.1650385489168));
#73130=CARTESIAN_POINT('Ctrl Pts',(0.0427123496854742,1.66503941049802,
10.1849088924397));
#73131=CARTESIAN_POINT('Ctrl Pts',(0.388843618002635,1.90046128201732,10.2047792359624));
#73132=CARTESIAN_POINT('Ctrl Pts',(0.378263803080852,2.3189327625422,10.2246495794852));
#73133=CARTESIAN_POINT('Ctrl Pts',(0.0206784447991286,2.53656323843889,
10.244519923008));
#73134=CARTESIAN_POINT('Ctrl Pts',(-0.355876571469739,2.35370637578606,
10.2643902665308));
#73135=CARTESIAN_POINT('Ctrl Pts',(-0.405963281635488,1.93810845235375,
10.2842606100536));
#73136=CARTESIAN_POINT('Ctrl Pts',(-0.0836339478109073,1.67102398434281,
10.3041309535764));
#73137=CARTESIAN_POINT('Ctrl Pts',(0.315418147396308,1.79746661088628,10.3240012970991));
#73138=CARTESIAN_POINT('Ctrl Pts',(0.425117032670701,2.20144243573974,10.343871640622));
#73139=CARTESIAN_POINT('Ctrl Pts',(0.1448289149277,2.51235863594257,10.3637419841447));
#73140=CARTESIAN_POINT('Ctrl Pts',(-0.268320015585099,2.44499192522719,
10.3836123276675));
#73141=CARTESIAN_POINT('Ctrl Pts',(-0.435321860270199,2.06114208952546,
10.4034826711903));
#73142=CARTESIAN_POINT('Ctrl Pts',(-0.202975161877188,1.71293909665728,
10.4233530147131));
#73143=CARTESIAN_POINT('Ctrl Pts',(0.215573614965055,1.71981178902226,10.4432233582359));
#73144=CARTESIAN_POINT('Ctrl Pts',(0.436362947774456,2.07545540700811,10.4630937017587));
#73145=CARTESIAN_POINT('Ctrl Pts',(0.256848681451869,2.4536153476194,10.4829640452815));
#73146=CARTESIAN_POINT('Ctrl Pts',(-0.15828928331231,2.50738134717243,10.5028343888043));
#73147=CARTESIAN_POINT('Ctrl Pts',(-0.428218379777491,2.18743042065718,
10.5227047323271));
#73148=CARTESIAN_POINT('Ctrl Pts',(-0.305315409465088,1.78727398576594,
10.5425750758498));
#73149=CARTESIAN_POINT('Ctrl Pts',(0.0976728840918246,1.67400109513199,
10.5624454193726));
#73150=CARTESIAN_POINT('Ctrl Pts',(0.411059603456944,1.95152420520041,10.5823157628954));
#73151=CARTESIAN_POINT('Ctrl Pts',(0.347355097362123,2.36525364384322,10.6021861064182));
#73152=CARTESIAN_POINT('Ctrl Pts',(-0.0350004224360313,2.53564897528268,
10.622056449941));
#73153=CARTESIAN_POINT('Ctrl Pts',(-0.385247819526378,2.30639568015277,
10.6419267934638));
#73154=CARTESIAN_POINT('Ctrl Pts',(-0.382082788955989,1.8878024467173,10.6617971369866));
#73155=CARTESIAN_POINT('Ctrl Pts',(-0.0284088153932009,1.66387158033039,
10.6816674805094));
#73156=CARTESIAN_POINT('Ctrl Pts',(0.351326378781868,1.84002916546741,10.7015378240322));
#73157=CARTESIAN_POINT('Ctrl Pts',(0.408767449192139,2.25467459945481,10.7214081675549));
#73158=CARTESIAN_POINT('Ctrl Pts',(0.0912200336317959,2.52742714548771,
10.7412785110778));
#73159=CARTESIAN_POINT('Ctrl Pts',(-0.310009344299521,2.40807347448707,
10.7611488546005));
#73160=CARTESIAN_POINT('Ctrl Pts',(-0.426847352797267,2.00610433106091,
10.7810191981233));
#73161=CARTESIAN_POINT('Ctrl Pts',(-0.152111025123309,1.69027168114532,
10.8008895416461));
#73162=CARTESIAN_POINT('Ctrl Pts',(0.262166460055135,1.75030898430513,10.8207598851689));
#73163=CARTESIAN_POINT('Ctrl Pts',(0.435941908873682,2.131140188232,10.8406302286917));
#73164=CARTESIAN_POINT('Ctrl Pts',(0.209800004432418,2.48340450880984,10.8605005722145));
#73165=CARTESIAN_POINT('Ctrl Pts',(-0.208804842384087,2.48394738836527,
10.8803709157373));
#73166=CARTESIAN_POINT('Ctrl Pts',(-0.435859672525612,2.13227080881258,
10.9002412592601));
#73167=CARTESIAN_POINT('Ctrl Pts',(-0.263072590061224,1.75099015544825,
10.9201116027828));
#73168=CARTESIAN_POINT('Ctrl Pts',(0.151047779685193,1.68987852106024,10.9399819463056));
#73169=CARTESIAN_POINT('Ctrl Pts',(0.426602374868791,2.00499751060179,10.9598522898284));
#73170=CARTESIAN_POINT('Ctrl Pts',(0.310807367779338,2.40726835074513,10.9797226333512));
#73171=CARTESIAN_POINT('Ctrl Pts',(-0.0901110866453405,2.52766230988848,
10.999592976874));
#73172=CARTESIAN_POINT('Ctrl Pts',(-0.408364886589611,2.25573432067532,
11.0194633203968));
#73173=CARTESIAN_POINT('Ctrl Pts',(-0.351999496947143,1.84094129355586,
11.0393336639196));
#73174=CARTESIAN_POINT('Ctrl Pts',(0.0272775107400031,1.66379936194065,
11.0592040074423));
#73175=CARTESIAN_POINT('Ctrl Pts',(0.381531115820961,1.8868121323903,11.0790743509652));
#73176=CARTESIAN_POINT('Ctrl Pts',(0.385781862907382,2.30539574846443,11.0989446944879));
#73177=CARTESIAN_POINT('Ctrl Pts',(0.0361302702344473,2.53555672742862,
11.1188150380107));
#73178=CARTESIAN_POINT('Ctrl Pts',(-0.346665926686456,2.36615370467115,
11.1386853815335));
#73179=CARTESIAN_POINT('Ctrl Pts',(-0.411443330176841,1.9525908914329,11.1585557250563));
#73180=CARTESIAN_POINT('Ctrl Pts',(-0.0987774911814487,1.67425586736697,
11.1784260685791));
#73181=CARTESIAN_POINT('Ctrl Pts',(0.304503248631784,1.7864831251619,11.1982964121019));
#73182=CARTESIAN_POINT('Ctrl Pts',(0.428443712199356,2.18631943415239,11.2181667556247));
#73183=CARTESIAN_POINT('Ctrl Pts',(0.159345397168516,2.50696941363788,11.2380370991475));
#73184=CARTESIAN_POINT('Ctrl Pts',(-0.255930626847466,2.45428035999335,
11.2579074426703));
#73185=CARTESIAN_POINT('Ctrl Pts',(-0.436425142539554,2.07658730697071,
11.2777777861931));
#73186=CARTESIAN_POINT('Ctrl Pts',(-0.216559003869717,1.7203722124521,11.2976481297158));
#73187=CARTESIAN_POINT('Ctrl Pts',(0.2019705390044,1.71241393135224,11.3175184732386));
#73188=CARTESIAN_POINT('Ctrl Pts',(0.435219608148008,2.0600131031581,11.3373888167614));
#73189=CARTESIAN_POINT('Ctrl Pts',(0.26921393661526,2.44429480909196,11.3572591602842));
#73190=CARTESIAN_POINT('Ctrl Pts',(-0.143758871594009,2.51273289918974,
11.377129503807));
#73191=CARTESIAN_POINT('Ctrl Pts',(-0.424852486118888,2.20254474279138,
11.3969998473298));
#73192=CARTESIAN_POINT('Ctrl Pts',(-0.316201783072909,1.79828574508806,
11.4168701908526));
#73193=CARTESIAN_POINT('Ctrl Pts',(0.0825210089568178,1.67080850157966,
11.4367405343754));
#73194=CARTESIAN_POINT('Ctrl Pts',(0.405542009489586,1.93705602872551,11.4566108778982));
#73195=CARTESIAN_POINT('Ctrl Pts',(0.356533425874872,2.35278246669712,11.476481221421));
#73196=CARTESIAN_POINT('Ctrl Pts',(-0.0195460383370229,2.53661540469947,
11.4963515649437));
#73197=CARTESIAN_POINT('Ctrl Pts',(-0.37769467332754,2.31991314871002,11.5162219084665));
#73198=CARTESIAN_POINT('Ctrl Pts',(-0.389359864026752,1.90147051725091,
11.5360922519893));
#73199=CARTESIAN_POINT('Ctrl Pts',(-0.0438403860404519,1.66515165886556,
11.5559625955121));
#73200=CARTESIAN_POINT('Ctrl Pts',(0.341896677808339,1.82774695421506,11.5758329390349));
#73201=CARTESIAN_POINT('Ctrl Pts',(0.41399008479768,2.24009735516691,11.5957032825577));
#73202=CARTESIAN_POINT('Ctrl Pts',(0.106303948645956,2.52392750528579,11.6155736260805));
#73203=CARTESIAN_POINT('Ctrl Pts',(-0.298901588412632,2.4188618818234,11.6354439696033));
#73204=CARTESIAN_POINT('Ctrl Pts',(-0.429905609879455,2.02128389091344,
11.6553143131261));
#73205=CARTESIAN_POINT('Ctrl Pts',(-0.166529760645773,1.69591721385982,
11.6751846566488));
#73206=CARTESIAN_POINT('Ctrl Pts',(0.249614473000665,1.74124148218593,11.6950550001716));
#73207=CARTESIAN_POINT('Ctrl Pts',(0.43677140961095,2.11567785004451,11.7149253436944));
#73208=CARTESIAN_POINT('Ctrl Pts',(0.223250038961308,2.47573192483382,11.7347956872172));
#73209=CARTESIAN_POINT('Ctrl Pts',(-0.195072849686974,2.49110310987073,
11.75466603074));
#73210=CARTESIAN_POINT('Ctrl Pts',(-0.43444295551788,2.14769043548176,11.7745363742628));
#73211=CARTESIAN_POINT('Ctrl Pts',(-0.275270793728863,1.76052827900481,
11.7944067177856));
#73212=CARTESIAN_POINT('Ctrl Pts',(0.136424846571767,1.68478521163929,11.8142770613084));
#73213=CARTESIAN_POINT('Ctrl Pts',(0.422969262708565,1.98994518620559,11.8341474048312));
#73214=CARTESIAN_POINT('Ctrl Pts',(0.321496962375759,2.39606546981827,11.8540177483539));
#73215=CARTESIAN_POINT('Ctrl Pts',(-0.0749050330775907,2.53058599054684,
11.8738880918767));
#73216=CARTESIAN_POINT('Ctrl Pts',(-0.402591858081682,2.27010248393803,
11.8937584353995));
#73217=CARTESIAN_POINT('Ctrl Pts',(-0.360955461228196,1.85357310567818,
11.9136287789223));
#73218=CARTESIAN_POINT('Ctrl Pts',(0.0118084316533941,1.66310685496629,
11.9334991224451));
#73219=CARTESIAN_POINT('Ctrl Pts',(0.373739696065804,1.87343058719194,11.9533694659679));
#73220=CARTESIAN_POINT('Ctrl Pts',(0.392815669403017,2.29160091102866,11.9732398094907));
#73221=CARTESIAN_POINT('Ctrl Pts',(0.0515367430874135,2.53400348310525,
11.9931101530135));
#73222=CARTESIAN_POINT('Ctrl Pts',(-0.337020128916868,2.37826694367174,
12.0129804965363));
#73223=CARTESIAN_POINT('Ctrl Pts',(-0.416406913787441,1.967258366043,12.032850840059));
#73224=CARTESIAN_POINT('Ctrl Pts',(-0.1137970439404,1.67802216642817,12.0527211835818));
#73225=CARTESIAN_POINT('Ctrl Pts',(0.293206121653347,1.77589318202087,12.0725915271046));
#73226=CARTESIAN_POINT('Ctrl Pts',(0.431232587039189,2.17108807995046,12.0924618706274));
#73227=CARTESIAN_POINT('Ctrl Pts',(0.173661860832098,2.50106934229368,12.1123322141502));
#73228=CARTESIAN_POINT('Ctrl Pts',(-0.24321998076094,2.46312408374301,12.132202557673));
#73229=CARTESIAN_POINT('Ctrl Pts',(-0.436980601416259,2.09206191323819,
12.1520729011958));
#73230=CARTESIAN_POINT('Ctrl Pts',(-0.22987100980918,1.72828185666441,12.1719432447186));
#73231=CARTESIAN_POINT('Ctrl Pts',(0.18811393918567,1.70550259174539,12.1918135882414));
#73232=CARTESIAN_POINT('Ctrl Pts',(0.433529958377981,2.04462099292745,12.2116839317642));
#73233=CARTESIAN_POINT('Ctrl Pts',(0.281241260532876,2.43454209392756,12.2315542752869));
#73234=CARTESIAN_POINT('Ctrl Pts',(-0.12904800631086,2.51756636754263,12.2514246188097));
#73235=CARTESIAN_POINT('Ctrl Pts',(-0.420953295664032,2.21753034546508,
12.2712949623325));
#73236=CARTESIAN_POINT('Ctrl Pts',(-0.326691243861827,1.80967623173504,
12.2911653058553));
#73237=CARTESIAN_POINT('Ctrl Pts',(0.0672655491868179,1.66815465137604,
12.3110356493781));
#73238=CARTESIAN_POINT('Ctrl Pts',(0.399515358234169,1.92279238794404,12.3309059929009));
#73239=CARTESIAN_POINT('Ctrl Pts',(0.365264215206402,2.33999398393544,12.3507763364237));
#73240=CARTESIAN_POINT('Ctrl Pts',(-0.00406711904058771,2.53703377189671,
12.3706466799465));
#73241=CARTESIAN_POINT('Ctrl Pts',(-0.369667425256092,2.33315457091827,
12.3905170234693));
#73242=CARTESIAN_POINT('Ctrl Pts',(-0.396148194474713,1.91538779225095,
12.410387366992));
#73243=CARTESIAN_POINT('Ctrl Pts',(-0.0592169259695541,1.66697758151076,
12.4302577105148));
#73244=CARTESIAN_POINT('Ctrl Pts',(0.332037810456167,1.81580648905538,12.4501280540376));
#73245=CARTESIAN_POINT('Ctrl Pts',(0.418693058654454,2.22534425343881,12.4699983975604));
#73246=CARTESIAN_POINT('Ctrl Pts',(0.121254425450163,2.51989572937136,12.4898687410832));
#73247=CARTESIAN_POINT('Ctrl Pts',(-0.287418635805224,2.4292500372474,12.509739084606));
#73248=CARTESIAN_POINT('Ctrl Pts',(-0.432424227223307,2.03656225929401,
12.5296094281288));
#73249=CARTESIAN_POINT('Ctrl Pts',(-0.180739459406689,1.70206997216982,
12.5494797716516));
#73250=CARTESIAN_POINT('Ctrl Pts',(0.236749156960017,1.73262431229833,12.5693501151744));
#73251=CARTESIAN_POINT('Ctrl Pts',(0.437052652303248,2.10019583220945,12.5892204586972));
#73252=CARTESIAN_POINT('Ctrl Pts',(0.236419838504093,2.46758770272854,12.6090908022199));
#73253=CARTESIAN_POINT('Ctrl Pts',(-0.181095991467864,2.49776789854112,
12.6289611457427));
#73254=CARTESIAN_POINT('Ctrl Pts',(-0.432480903261117,2.16305019865179,
12.6488314892655));
#73255=CARTESIAN_POINT('Ctrl Pts',(-0.287123463270608,1.7704925250089,12.6687018327883));
#73256=CARTESIAN_POINT('Ctrl Pts',(0.121630665940594,1.68021310127832,12.6885721763111));
#73257=CARTESIAN_POINT('Ctrl Pts',(0.418805217671658,1.97503100829909,12.7084425198339));
#73258=CARTESIAN_POINT('Ctrl Pts',(0.331782997370132,2.38449095221355,12.7283128633567));
#73259=CARTESIAN_POINT('Ctrl Pts',(-0.0596049548405058,2.53296917741782,
12.7481832068795));
#73260=CARTESIAN_POINT('Ctrl Pts',(-0.396313475469834,2.28425712577239,
12.7680535504023));
#73261=CARTESIAN_POINT('Ctrl Pts',(-0.369458335557585,1.86651424557301,
12.7879238939251));
#73262=CARTESIAN_POINT('Ctrl Pts',(-0.00367546999292127,1.66296275884588,
12.8077942374478));
#73263=CARTESIAN_POINT('Ctrl Pts',(0.365479138941547,1.86033344362852,12.8276645809706));
#73264=CARTESIAN_POINT('Ctrl Pts',(0.39935639334789,2.27756556622912,12.8475349244934));
#73265=CARTESIAN_POINT('Ctrl Pts',(0.0668785244003959,2.53190545517864,
12.8674052680162));
#73266=CARTESIAN_POINT('Ctrl Pts',(-0.326951286148151,2.39003088762939,
12.887275611539));
#73267=CARTESIAN_POINT('Ctrl Pts',(-0.420847801760121,1.98209246480204,
12.9071459550618));
#73268=CARTESIAN_POINT('Ctrl Pts',(-0.12867375307811,1.68231815389222,12.9270162985846));
#73269=CARTESIAN_POINT('Ctrl Pts',(0.281540947794072,1.76571007447041,12.9468866421074));
#73270=CARTESIAN_POINT('Ctrl Pts',(0.433480155303436,2.15576749238745,12.9667569856302));
#73271=CARTESIAN_POINT('Ctrl Pts',(0.187760337362539,2.49466582784844,12.9866273291529));
#73272=CARTESIAN_POINT('Ctrl Pts',(-0.230204036640388,2.47151199563903,
13.0064976726757));
#73273=CARTESIAN_POINT('Ctrl Pts',(-0.436987531463964,2.1075464832979,13.0263680161985));
#73274=CARTESIAN_POINT('Ctrl Pts',(-0.242894485563508,1.73665810167174,
13.0462383597213));
#73275=CARTESIAN_POINT('Ctrl Pts',(0.174021239434115,1.69908644380071,13.0661087032441));
#73276=CARTESIAN_POINT('Ctrl Pts',(0.431296060836643,2.02929840089342,13.0859790467669));
#73277=CARTESIAN_POINT('Ctrl Pts',(0.29291566868573,2.42436943729461,13.1058493902897));
#73278=CARTESIAN_POINT('Ctrl Pts',(-0.114175370565393,2.52187569838607,
13.1257197338125));
#73279=CARTESIAN_POINT('Ctrl Pts',(-0.41652528440381,2.23236839221512,13.1455900773353));
#73280=CARTESIAN_POINT('Ctrl Pts',(-0.336771430945945,1.82143119739647,
13.165460420858));
#73281=CARTESIAN_POINT('Ctrl Pts',(0.0519272067197533,1.66604278020319,
13.1853307643808));
#73282=CARTESIAN_POINT('Ctrl Pts',(0.39298422437713,1.90875137138937,13.2052011079036));
#73283=CARTESIAN_POINT('Ctrl Pts',(0.373542265624722,2.32690389377349,13.2250714514264));
#73284=CARTESIAN_POINT('Ctrl Pts',(0.0114058118306527,2.53690423463656,
13.2449417949492));
#73285=CARTESIAN_POINT('Ctrl Pts',(-0.36115478336407,2.34610200991459,13.264812138472));
#73286=CARTESIAN_POINT('Ctrl Pts',(-0.402480421588718,1.92953933752709,
13.2846824819948));
#73287=CARTESIAN_POINT('Ctrl Pts',(-0.0744398039609454,1.66934215746259,
13.3045528255176));
#73288=CARTESIAN_POINT('Ctrl Pts',(0.321608914458083,1.80423233708416,13.3244231690404));
#73289=CARTESIAN_POINT('Ctrl Pts',(0.423169768399744,2.21041401303246,13.3442935125631));
#73290=CARTESIAN_POINT('Ctrl Pts',(0.135372886919875,2.51545578431306,13.3641682923767));
#73291=CARTESIAN_POINT('Ctrl Pts',(-0.137725918669883,2.46444282891852,
13.3774196243492));
#73292=CARTESIAN_POINT('Ctrl Pts',(-0.233247926994675,2.38672943582559,
13.3840475084809));
#73293=CARTESIAN_POINT('Ctrl Pts',(0.386361485727264,2.1750387445618,4.3568622407636));
#73294=CARTESIAN_POINT('Ctrl Pts',(0.361378776375058,2.30367038357945,4.36348568860453));
#73295=CARTESIAN_POINT('Ctrl Pts',(0.173233487786809,2.53177857313794,4.37673258428639));
#73296=CARTESIAN_POINT('Ctrl Pts',(-0.270140399087323,2.47932904882227,
4.39660292780918));
#73297=CARTESIAN_POINT('Ctrl Pts',(-0.464748843309329,2.07821683774835,
4.41647327133197));
#73298=CARTESIAN_POINT('Ctrl Pts',(-0.233482156592523,1.69743115863587,
4.43634361485476));
#73299=CARTESIAN_POINT('Ctrl Pts',(0.212213424096465,1.68577028843772,4.45621395837754));
#73300=CARTESIAN_POINT('Ctrl Pts',(0.463107326163524,2.05420072893338,4.47608430190034));
#73301=CARTESIAN_POINT('Ctrl Pts',(0.289228043586586,2.46459804209974,4.49595464542312));
#73302=CARTESIAN_POINT('Ctrl Pts',(-0.150012203329834,2.54055106314491,
4.51582498894591));
#73303=CARTESIAN_POINT('Ctrl Pts',(-0.451619227057188,2.21234559627247,
4.5356953324687));
#73304=CARTESIAN_POINT('Ctrl Pts',(-0.338936151504061,1.78108501755827,
4.55556567599149));
#73305=CARTESIAN_POINT('Ctrl Pts',(0.0846794043969424,1.64238205164921,
4.57543601951428));
#73306=CARTESIAN_POINT('Ctrl Pts',(0.43061069294052,1.92348305441572,4.59530636303707));
#73307=CARTESIAN_POINT('Ctrl Pts',(0.38151656084392,2.36651338955372,4.61517670655986));
#73308=CARTESIAN_POINT('Ctrl Pts',(-0.0175677352453814,2.56505445751964,
4.63504705008264));
#73309=CARTESIAN_POINT('Ctrl Pts',(-0.400535684148771,2.33697112024056,
4.65491739360544));
#73310=CARTESIAN_POINT('Ctrl Pts',(-0.416066848274827,1.89149917163689,
4.67478773712822));
#73311=CARTESIAN_POINT('Ctrl Pts',(-0.0499132293823783,1.63729828032735,
4.69465808065102));
#73312=CARTESIAN_POINT('Ctrl Pts',(0.362028934572462,1.80756326092109,4.71452842417379));
#73313=CARTESIAN_POINT('Ctrl Pts',(0.441858861675035,2.24609911964907,4.73439876769659));
#73314=CARTESIAN_POINT('Ctrl Pts',(0.116343423952193,2.55060893520105,4.75426911121937));
#73315=CARTESIAN_POINT('Ctrl Pts',(-0.315901259827201,2.44174639263947,
4.77413945474218));
#73316=CARTESIAN_POINT('Ctrl Pts',(-0.458349547262939,2.0193780619629,4.79400979826496));
#73317=CARTESIAN_POINT('Ctrl Pts',(-0.180324521937238,1.67096938241971,
4.81388014178775));
#73318=CARTESIAN_POINT('Ctrl Pts',(0.263123702362371,1.71613788795246,4.83375048531054));
#73319=CARTESIAN_POINT('Ctrl Pts',(0.46519175128823,2.11344762282265,4.85362082883332));
#73320=CARTESIAN_POINT('Ctrl Pts',(0.240509698292949,2.49842099466773,4.87349117235613));
#73321=CARTESIAN_POINT('Ctrl Pts',(-0.204807260316238,2.5178973439291,4.89336151587891));
#73322=CARTESIAN_POINT('Ctrl Pts',(-0.462241439644094,2.1540097717718,4.9132318594017));
#73323=CARTESIAN_POINT('Ctrl Pts',(-0.295632026552772,1.7405755867543,4.93310220292448));
#73324=CARTESIAN_POINT('Ctrl Pts',(0.142179524216207,1.65686436968784,4.95297254644727));
#73325=CARTESIAN_POINT('Ctrl Pts',(0.449560717520727,1.97966976595722,4.97284288997007));
#73326=CARTESIAN_POINT('Ctrl Pts',(0.344531154660214,2.41286177048237,4.99271323349286));
#73327=CARTESIAN_POINT('Ctrl Pts',(-0.0765588389171428,2.55904569287204,
5.01258357701564));
#73328=CARTESIAN_POINT('Ctrl Pts',(-0.427416520334123,2.28411768548057,
5.03245392053844));
#73329=CARTESIAN_POINT('Ctrl Pts',(-0.386177731848805,1.84028676701965,
5.05232426406122));
#73330=CARTESIAN_POINT('Ctrl Pts',(0.00932655225657797,1.6347073830545,
5.07219460758402));
#73331=CARTESIAN_POINT('Ctrl Pts',(0.396274994362174,1.85597063126681,5.09206495110681));
#73332=CARTESIAN_POINT('Ctrl Pts',(0.419695077109399,2.30109760369322,5.11193529462959));
#73333=CARTESIAN_POINT('Ctrl Pts',(0.0581020629341788,2.5617449016977,5.13180563815239));
#73334=CARTESIAN_POINT('Ctrl Pts',(-0.356791684101566,2.39880411328662,
5.15167598167517));
#73335=CARTESIAN_POINT('Ctrl Pts',(-0.444377633775809,1.96175122944184,
5.17154632519797));
#73336=CARTESIAN_POINT('Ctrl Pts',(-0.124307601012795,1.65152277171357,
5.19141666872075));
#73337=CARTESIAN_POINT('Ctrl Pts',(0.309797732727714,1.75271111627667,5.21128701224355));
#73338=CARTESIAN_POINT('Ctrl Pts',(0.459705821843468,2.17248973254367,5.23115735576633));
#73339=CARTESIAN_POINT('Ctrl Pts',(0.187896402714256,2.52576888778782,5.25102769928912));
#73340=CARTESIAN_POINT('Ctrl Pts',(-0.256282386119894,2.48846305168667,
5.2708980428119));
#73341=CARTESIAN_POINT('Ctrl Pts',(-0.465356975385395,2.09479525013207,
5.2907683863347));
#73342=CARTESIAN_POINT('Ctrl Pts',(-0.247529892366297,1.70590209801857,
5.31063872985749));
#73343=CARTESIAN_POINT('Ctrl Pts',(0.197372168746952,1.67854011938838,5.33050907338028));
#73344=CARTESIAN_POINT('Ctrl Pts',(0.461212134829325,2.03781020463768,5.35037941690307));
#73345=CARTESIAN_POINT('Ctrl Pts',(0.301952755568203,2.45413096075576,5.37024976042586));
#73346=CARTESIAN_POINT('Ctrl Pts',(-0.134307169771021,2.54558477095736,
5.39012010394865));
#73347=CARTESIAN_POINT('Ctrl Pts',(-0.447358551115442,2.22827521469451,
5.40999044747144));
#73348=CARTESIAN_POINT('Ctrl Pts',(-0.350019364178736,1.79329061204303,
5.42986079099422));
#73349=CARTESIAN_POINT('Ctrl Pts',(0.0684149385583651,1.6396701181293,5.44973113451702));
#73350=CARTESIAN_POINT('Ctrl Pts',(0.424087849021016,1.90833962257744,5.46960147803981));
#73351=CARTESIAN_POINT('Ctrl Pts',(0.390717892354156,2.35283143110649,5.4894718215626));
#73352=CARTESIAN_POINT('Ctrl Pts',(-0.00108253910974737,2.5653848214866,
5.50934216508539));
#73353=CARTESIAN_POINT('Ctrl Pts',(-0.391889888314849,2.35101099457515,
5.52921250860817));
#73354=CARTESIAN_POINT('Ctrl Pts',(-0.423191615981816,1.9063687522022,5.54908285213097));
#73355=CARTESIAN_POINT('Ctrl Pts',(-0.0662726483216284,1.63935681916968,
5.56895319565376));
#73356=CARTESIAN_POINT('Ctrl Pts',(0.351442451967285,1.79492229364266,5.58882353917654));
#73357=CARTESIAN_POINT('Ctrl Pts',(0.446756947145716,2.23035503111914,5.60869388269934));
#73358=CARTESIAN_POINT('Ctrl Pts',(0.132232763784262,2.54620477377881,5.62856422622211));
#73359=CARTESIAN_POINT('Ctrl Pts',(-0.303596978484018,2.45272238179113,
5.64843456974492));
#73360=CARTESIAN_POINT('Ctrl Pts',(-0.460917823989673,2.03566522332629,
5.6683049132677));
#73361=CARTESIAN_POINT('Ctrl Pts',(-0.195409314280412,1.67762646407061,
5.68817525679049));
#73362=CARTESIAN_POINT('Ctrl Pts',(0.249360638705182,1.70705792306553,5.70804560031327));
#73363=CARTESIAN_POINT('Ctrl Pts',(0.465376153064306,2.09696024341454,5.72791594383607));
#73364=CARTESIAN_POINT('Ctrl Pts',(0.254472402229233,2.48965112660522,5.74778628735886));
#73365=CARTESIAN_POINT('Ctrl Pts',(-0.189875134361864,2.52489014734646,
5.76765663088165));
#73366=CARTESIAN_POINT('Ctrl Pts',(-0.460038084341331,2.17035030146765,
5.78752697440444));
#73367=CARTESIAN_POINT('Ctrl Pts',(-0.308178720467497,1.75127363132099,
5.80739731792722));
#73368=CARTESIAN_POINT('Ctrl Pts',(0.126392664690959,1.65210592962917,5.82726766145002));
#73369=CARTESIAN_POINT('Ctrl Pts',(0.445015986802993,1.96382006223093,5.8471380049728));
#73370=CARTESIAN_POINT('Ctrl Pts',(0.355397724479243,2.40046074851136,5.86700834849559));
#73371=CARTESIAN_POINT('Ctrl Pts',(-0.060249567022979,2.56146960206993,
5.88687869201838));
#73372=CARTESIAN_POINT('Ctrl Pts',(-0.420626083019512,2.29914291914275,
5.90674903554117));
#73373=CARTESIAN_POINT('Ctrl Pts',(-0.39513543091603,1.85412971876244,5.92661937906395));
#73374=CARTESIAN_POINT('Ctrl Pts',(-0.00716181377855303,1.63466902920133,
5.94648972258676));
#73375=CARTESIAN_POINT('Ctrl Pts',(0.387381792507841,1.8420861562567,5.96636006610954));
#73376=CARTESIAN_POINT('Ctrl Pts',(0.426555341437201,2.2861041231473,5.98623040963234));
#73377=CARTESIAN_POINT('Ctrl Pts',(0.0744224348639616,2.5593968928388,6.00610075315511));
#73378=CARTESIAN_POINT('Ctrl Pts',(-0.345982923997342,2.41125555459024,
6.02597109667792));
#73379=CARTESIAN_POINT('Ctrl Pts',(-0.44899605141297,1.97757961862258,6.0458414402007));
#73380=CARTESIAN_POINT('Ctrl Pts',(-0.140116426950026,1.65620771653871,
6.0657117837235));
#73381=CARTESIAN_POINT('Ctrl Pts',(0.297300944110507,1.74195481766678,6.08558212724628));
#73382=CARTESIAN_POINT('Ctrl Pts',(0.46198517281843,2.15615963013551,6.10545247076906));
#73383=CARTESIAN_POINT('Ctrl Pts',(0.202860899067473,2.51884562739817,6.12532281429185));
#73384=CARTESIAN_POINT('Ctrl Pts',(-0.24236063256028,2.49729778220626,6.14519315781465));
#73385=CARTESIAN_POINT('Ctrl Pts',(-0.465249278234726,2.11128330904911,
6.16506350133744));
#73386=CARTESIAN_POINT('Ctrl Pts',(-0.261335049098668,1.71491793592323,
6.18493384486023));
#73387=CARTESIAN_POINT('Ctrl Pts',(0.182318510031114,1.67181293239863,6.20480418838301));
#73388=CARTESIAN_POINT('Ctrl Pts',(0.458719656631219,2.0215112709928,6.2246745319058));
#73389=CARTESIAN_POINT('Ctrl Pts',(0.314307967314327,2.44321233317549,6.24454487542858));
#73390=CARTESIAN_POINT('Ctrl Pts',(-0.118438492847544,2.55006280380969,
6.26441521895139));
#73391=CARTESIAN_POINT('Ctrl Pts',(-0.442533759766611,2.24404192246654,
6.28428556247417));
#73392=CARTESIAN_POINT('Ctrl Pts',(-0.360664547631079,1.80588218679737,
6.30415590599697));
#73393=CARTESIAN_POINT('Ctrl Pts',(0.0520652869115094,1.63753550421697,
6.32402624951974));
#73394=CARTESIAN_POINT('Ctrl Pts',(0.417032308761556,1.89343703766155,6.34389659304255));
#73395=CARTESIAN_POINT('Ctrl Pts',(0.399428961145075,2.33883196804363,6.36376693656534));
#73396=CARTESIAN_POINT('Ctrl Pts',(0.0154039190208104,2.56513108178215,
6.3836372800881));
#73397=CARTESIAN_POINT('Ctrl Pts',(-0.382752121750834,2.3647357498644,6.40350762361091));
#73398=CARTESIAN_POINT('Ctrl Pts',(-0.429785197812239,1.92148140796398,
6.42337796713368));
#73399=CARTESIAN_POINT('Ctrl Pts',(-0.0825488648521865,1.64199357114485,
6.44324831065649));
#73400=CARTESIAN_POINT('Ctrl Pts',(0.340414813596581,1.78266428085538,6.46311865417927));
#73401=CARTESIAN_POINT('Ctrl Pts',(0.451094243862592,2.21444731152398,6.48298899770206));
#73402=CARTESIAN_POINT('Ctrl Pts',(0.147956116320611,2.54124051446389,6.50285934122486));
#73403=CARTESIAN_POINT('Ctrl Pts',(-0.290911605539139,2.46325561485498,
6.52272968474764));
#73404=CARTESIAN_POINT('Ctrl Pts',(-0.462907533355605,2.05203314140305,
6.54260002827044));
#73405=CARTESIAN_POINT('Ctrl Pts',(-0.210248818488382,1.68481373061568,
6.56247037179321));
#73406=CARTESIAN_POINT('Ctrl Pts',(0.235284564549913,1.69847119948179,6.58234071531602));
#73407=CARTESIAN_POINT('Ctrl Pts',(0.46497639071474,2.08047667961323,6.6022110588388));
#73408=CARTESIAN_POINT('Ctrl Pts',(0.268115679218368,2.48039214833945,6.6220814023616));
#73409=CARTESIAN_POINT('Ctrl Pts',(-0.174704667307117,2.53134960667902,
6.64195174588437));
#73410=CARTESIAN_POINT('Ctrl Pts',(-0.457257265471105,2.18660252383689,
6.66182208940717));
#73411=CARTESIAN_POINT('Ctrl Pts',(-0.320338572520919,1.76240941524342,
6.68169243292995));
#73412=CARTESIAN_POINT('Ctrl Pts',(0.110447150558528,1.64790970935605,6.70156277645275));
#73413=CARTESIAN_POINT('Ctrl Pts',(0.439912649022332,1.94814129859904,6.72143311997555));
#73414=CARTESIAN_POINT('Ctrl Pts',(0.365818180707404,2.38768257268204,6.74130346349833));
#73415=CARTESIAN_POINT('Ctrl Pts',(-0.0438646667583175,2.56331425077502,
6.76117380702112));
#73416=CARTESIAN_POINT('Ctrl Pts',(-0.41330765410843,2.31391817832157,6.78104415054392));
#73417=CARTESIAN_POINT('Ctrl Pts',(-0.403597135570311,1.86828129958834,
6.80091449406668));
#73418=CARTESIAN_POINT('Ctrl Pts',(-0.0236411899349659,1.63521478283029,
6.8207848375895));
#73419=CARTESIAN_POINT('Ctrl Pts',(0.378002329008327,1.82852542803181,6.84065518111227));
#73420=CARTESIAN_POINT('Ctrl Pts',(0.432880171456738,2.27087703508844,6.86052552463507));
#73421=CARTESIAN_POINT('Ctrl Pts',(0.0906493879074764,2.55647222525914,
6.88039586815785));
#73422=CARTESIAN_POINT('Ctrl Pts',(-0.334739868247094,2.42331629183657,
6.90026621168064));
#73423=CARTESIAN_POINT('Ctrl Pts',(-0.453050866003015,1.99356167619252,
6.92013655520344));
#73424=CARTESIAN_POINT('Ctrl Pts',(-0.155749371507164,1.6614497323725,6.94000689872622));
#73425=CARTESIAN_POINT('Ctrl Pts',(0.284430967984231,1.73164795587294,6.959877242249));
#73426=CARTESIAN_POINT('Ctrl Pts',(0.463684616129835,2.13975903325736,6.9797475857718));
#73427=CARTESIAN_POINT('Ctrl Pts',(0.217570753936658,2.51139661033176,6.9996179292946));
#73428=CARTESIAN_POINT('Ctrl Pts',(-0.228134655409879,2.50563380401792,
7.01948827281737));
#73429=CARTESIAN_POINT('Ctrl Pts',(-0.464557576146697,2.12775720457354,
7.03935861634017));
#73430=CARTESIAN_POINT('Ctrl Pts',(-0.274812164572039,1.72441714873511,
7.05922895986296));
#73431=CARTESIAN_POINT('Ctrl Pts',(0.167035995699563,1.66562322794412,7.07909930338575));
#73432=CARTESIAN_POINT('Ctrl Pts',(0.455651369814231,2.00531086045673,7.09896964690853));
#73433=CARTESIAN_POINT('Ctrl Pts',(0.32626864345696,2.43186288773797,7.11883999043134));
#73434=CARTESIAN_POINT('Ctrl Pts',(-0.102421145807134,2.55397589457215,
7.13871033395412));
#73435=CARTESIAN_POINT('Ctrl Pts',(-0.437153477173104,2.25962782137364,
7.15858067747691));
#73436=CARTESIAN_POINT('Ctrl Pts',(-0.370857006304683,1.81884295343036,
7.17845102099969));
#73437=CARTESIAN_POINT('Ctrl Pts',(0.0356502802258794,1.63598139963914,
7.19832136452249));
#73438=CARTESIAN_POINT('Ctrl Pts',(0.409453287996592,1.87879374125082,7.21819170804527));
#73439=CARTESIAN_POINT('Ctrl Pts',(0.407638646062127,2.32453271075205,7.23806205156807));
#73440=CARTESIAN_POINT('Ctrl Pts',(0.0318710413561637,2.56429348550664,
7.25793239509085));
#73441=CARTESIAN_POINT('Ctrl Pts',(-0.373133904943599,2.37812819515931,
7.27780273861364));
#73442=CARTESIAN_POINT('Ctrl Pts',(-0.435839291051773,1.93681814948801,
7.29767308213644));
#73443=CARTESIAN_POINT('Ctrl Pts',(-0.0987214617815934,1.64520523645854,
7.31754342565922));
#73444=CARTESIAN_POINT('Ctrl Pts',(0.328959868959777,1.77080460426215,7.337413769182));
#73445=CARTESIAN_POINT('Ctrl Pts',(0.454865303772759,2.19839593174896,7.35728411270481));
#73446=CARTESIAN_POINT('Ctrl Pts',(0.163493746693623,2.5357223872526,7.37715445622759));
#73447=CARTESIAN_POINT('Ctrl Pts',(-0.277861065313151,2.47333287069862,
7.39702479975038));
#73448=CARTESIAN_POINT('Ctrl Pts',(-0.46431617726337,2.06846126995956,7.41689514327317));
#73449=CARTESIAN_POINT('Ctrl Pts',(-0.224824407514071,1.69252216042222,
7.43676548679595));
#73450=CARTESIAN_POINT('Ctrl Pts',(0.220913149050097,1.69038849559882,7.45663583031875));
#73451=CARTESIAN_POINT('Ctrl Pts',(0.463992965970334,2.06401762249259,7.47650617384153));
#73452=CARTESIAN_POINT('Ctrl Pts',(0.281422403551169,2.47065568219105,7.49637651736432));
#73453=CARTESIAN_POINT('Ctrl Pts',(-0.159314901925512,2.53726761369383,
7.51624686088712));
#73454=CARTESIAN_POINT('Ctrl Pts',(-0.453902473650952,2.20274603824273,
7.5361172044099));
#73455=CARTESIAN_POINT('Ctrl Pts',(-0.332096319043547,1.77396896031397,
7.55598754793269));
#73456=CARTESIAN_POINT('Ctrl Pts',(0.0943629974549827,1.64428097617902,
7.57585789145548));
#73457=CARTESIAN_POINT('Ctrl Pts',(0.43425711015065,1.93265315585696,7.59572823497828));
#73458=CARTESIAN_POINT('Ctrl Pts',(0.375779443050263,2.37454328282052,7.61559857850106));
#73459=CARTESIAN_POINT('Ctrl Pts',(-0.0274247052970846,2.56457732348921,
7.63546892202385));
#73460=CARTESIAN_POINT('Ctrl Pts',(-0.405470420070843,2.32842491634803,
7.65533926554663));
#73461=CARTESIAN_POINT('Ctrl Pts',(-0.411552224242792,1.88272374570183,
7.67520960906944));
#73462=CARTESIAN_POINT('Ctrl Pts',(-0.0400908904480416,1.63634395888319,
7.6950799525922));
#73463=CARTESIAN_POINT('Ctrl Pts',(0.368148377450899,1.81530546871901,7.71495029611502));
#73464=CARTESIAN_POINT('Ctrl Pts',(0.438661627914525,2.2554354533445,7.73482063963779));
#73465=CARTESIAN_POINT('Ctrl Pts',(0.106762553154688,2.55297457015259,7.7546909831606));
#73466=CARTESIAN_POINT('Ctrl Pts',(-0.32307662971541,2.43497118576493,7.77456132668337));
#73467=CARTESIAN_POINT('Ctrl Pts',(-0.456536987733129,2.00967734064704,
7.79443167020617));
#73468=CARTESIAN_POINT('Ctrl Pts',(-0.171186811404311,1.66724223916577,
7.81430201372895));
#73469=CARTESIAN_POINT('Ctrl Pts',(0.271203959408015,1.72180346860072,7.83417235725175));
#73470=CARTESIAN_POINT('Ctrl Pts',(0.464802018548613,2.12330852878598,7.85404270077455));
#73471=CARTESIAN_POINT('Ctrl Pts',(0.232007502751803,2.50343118697977,7.87391304429731));
#73472=CARTESIAN_POINT('Ctrl Pts',(-0.213622311850383,2.51346065331628,
7.89378338782013));
#73473=CARTESIAN_POINT('Ctrl Pts',(-0.463282737381516,2.14419625782033,
7.9136537313429));
#73474=CARTESIAN_POINT('Ctrl Pts',(-0.287944321614599,1.73438781255141,
7.9335240748657));
#73475=CARTESIAN_POINT('Ctrl Pts',(0.151543809154065,1.65997877566178,7.95339441838848));
#73476=CARTESIAN_POINT('Ctrl Pts',(0.452011125850539,1.98922930862201,7.97326476191127));
#73477=CARTESIAN_POINT('Ctrl Pts',(0.337819770337296,2.42009687085364,7.99313510543406));
#73478=CARTESIAN_POINT('Ctrl Pts',(-0.0862752344515524,2.55731913133102,
8.01300544895685));
#73479=CARTESIAN_POINT('Ctrl Pts',(-0.431224456943676,2.27501334719004,
8.03287579247963));
#73480=CARTESIAN_POINT('Ctrl Pts',(-0.380583946098691,1.83215664291795,
8.05274613600243));
#73481=CARTESIAN_POINT('Ctrl Pts',(0.0191905234661595,1.63500975518821,
8.07261647952521));
#73482=CARTESIAN_POINT('Ctrl Pts',(0.401360300304663,1.86442811436765,8.09248682304802));
#73483=CARTESIAN_POINT('Ctrl Pts',(0.415336641884546,2.30995160839845,8.11235716657078));
#73484=CARTESIAN_POINT('Ctrl Pts',(0.0482981575133614,2.5628730840542,8.1322275100936));
#73485=CARTESIAN_POINT('Ctrl Pts',(-0.363047311175928,2.39117151957044,
8.15209785361636));
#73486=CARTESIAN_POINT('Ctrl Pts',(-0.441346296289723,1.95235972530378,
8.17196819713918));
#73487=CARTESIAN_POINT('Ctrl Pts',(-0.114770138430408,1.64898778366247,
8.19183854066195));
#73488=CARTESIAN_POINT('Ctrl Pts',(0.317091996895345,1.75935815074194,8.21170888418476));
#73489=CARTESIAN_POINT('Ctrl Pts',(0.458065393246939,2.18222104031546,8.23157922770753));
#73490=CARTESIAN_POINT('Ctrl Pts',(0.178826151266698,2.52965731878344,8.25144957123033));
#73491=CARTESIAN_POINT('Ctrl Pts',(-0.264461739518581,2.48294149982973,
8.27131991475312));
#73492=CARTESIAN_POINT('Ctrl Pts',(-0.465141987510332,2.08492898755989,
8.29119025827591));
#73493=CARTESIAN_POINT('Ctrl Pts',(-0.239117785324893,1.70074207747079,
8.31106060179869));
#73494=CARTESIAN_POINT('Ctrl Pts',(0.206264431949168,1.68281995724421,8.33093094532149));
#73495=CARTESIAN_POINT('Ctrl Pts',(0.462427113276644,2.04760373231172,8.35080128884428));
#73496=CARTESIAN_POINT('Ctrl Pts',(0.294375871939588,2.46045394987548,8.37067163236707));
#73497=CARTESIAN_POINT('Ctrl Pts',(-0.143725156245875,2.54263673980266,
8.39054197588985));
#73498=CARTESIAN_POINT('Ctrl Pts',(-0.44997791998894,2.21876058051162,8.41041231941266));
#73499=CARTESIAN_POINT('Ctrl Pts',(-0.343437201104315,1.78593775639426,
8.43028266293542));
#73500=CARTESIAN_POINT('Ctrl Pts',(0.0781603950405117,1.64122428507152,
8.45015300645822));
#73501=CARTESIAN_POINT('Ctrl Pts',(0.428056469312614,1.91737507552185,8.470023349981));
#73502=CARTESIAN_POINT('Ctrl Pts',(0.385269007616535,2.36105937204245,8.48989369350379));
#73503=CARTESIAN_POINT('Ctrl Pts',(-0.0109503189284993,2.56525723473837,
8.50976403702659));
#73504=CARTESIAN_POINT('Ctrl Pts',(-0.397124218607941,2.34264492361486,
8.52963438054937));
#73505=CARTESIAN_POINT('Ctrl Pts',(-0.418990711295057,1.89743892819821,
8.54950472407216));
#73506=CARTESIAN_POINT('Ctrl Pts',(-0.0564902668035913,1.63805513995987,
8.56937506759495));
#73507=CARTESIAN_POINT('Ctrl Pts',(0.357832307024788,1.80244287269442,8.58924541111775));
#73508=CARTESIAN_POINT('Ctrl Pts',(0.443892453627643,2.23979876098687,8.60911575464052));
#73509=CARTESIAN_POINT('Ctrl Pts',(0.122741704527867,2.5489083179566,8.62898609816333));
#73510=CARTESIAN_POINT('Ctrl Pts',(-0.311007848702041,2.44620560655015,
8.64885644168609));
#73511=CARTESIAN_POINT('Ctrl Pts',(-0.459450040643157,2.02590638277131,
8.66872678520892));
#73512=CARTESIAN_POINT('Ctrl Pts',(-0.18640936876913,1.67357796586466,8.68859712873168));
#73513=CARTESIAN_POINT('Ctrl Pts',(0.257636521606575,1.71243371315928,8.7084674722545));
#73514=CARTESIAN_POINT('Ctrl Pts',(0.465335977453503,2.10682876624473,8.72833781577727));
#73515=CARTESIAN_POINT('Ctrl Pts',(0.246153023759728,2.49495935595321,8.74820815930007));
#73516=CARTESIAN_POINT('Ctrl Pts',(-0.198841818525403,2.52076850543563,
8.76807850282285));
#73517=CARTESIAN_POINT('Ctrl Pts',(-0.461426362182681,2.16057983364032,
8.78794884634566));
#73518=CARTESIAN_POINT('Ctrl Pts',(-0.30071503606418,1.74481741167964,8.80781918986842));
#73519=CARTESIAN_POINT('Ctrl Pts',(0.135861396987775,1.6548866607598,8.82768953339124));
#73520=CARTESIAN_POINT('Ctrl Pts',(0.447803494162487,1.97328680188354,8.847559876914));
#73521=CARTESIAN_POINT('Ctrl Pts',(0.348946848383933,2.40792905183493,8.86743022043681));
#73522=CARTESIAN_POINT('Ctrl Pts',(-0.0700210259631247,2.56008831748274,
8.88730056395958));
#73523=CARTESIAN_POINT('Ctrl Pts',(-0.424754141490919,2.29017918720865,
8.9071709074824));
#73524=CARTESIAN_POINT('Ctrl Pts',(-0.389833157255602,1.84580654322906,
8.92704125100514));
#73525=CARTESIAN_POINT('Ctrl Pts',(0.00270667776965062,1.6346217905225,
8.94691159452797));
#73526=CARTESIAN_POINT('Ctrl Pts',(0.392763504422148,1.85035818948929,8.96678193805073));
#73527=CARTESIAN_POINT('Ctrl Pts',(0.422513285690156,2.29510696393603,8.98665228157354));
#73528=CARTESIAN_POINT('Ctrl Pts',(0.0646646473272788,2.56087166038613,
9.00652262509631));
#73529=CARTESIAN_POINT('Ctrl Pts',(-0.352505001661575,2.40384935044295,
9.02639296861913));
#73530=CARTESIAN_POINT('Ctrl Pts',(-0.446299300848517,1.96808662682216,
9.04626331214188));
#73531=CARTESIAN_POINT('Ctrl Pts',(-0.130674749670337,1.65333646470792,
9.0661336556647));
#73532=CARTESIAN_POINT('Ctrl Pts',(0.304826094569618,1.74833928847471,9.08600399918746));
#73533=CARTESIAN_POINT('Ctrl Pts',(0.460690495367448,2.16594294078312,9.10587434271029));
#73534=CARTESIAN_POINT('Ctrl Pts',(0.19393408401326,2.52305292224374,9.12574468623304));
#73535=CARTESIAN_POINT('Ctrl Pts',(-0.250730447681617,2.49206944100045,
9.14561502975586));
#73536=CARTESIAN_POINT('Ctrl Pts',(-0.465383927496798,2.10141562307388,
9.16548537327863));
#73537=CARTESIAN_POINT('Ctrl Pts',(-0.253111010134359,1.70946316369669,
9.18535571680145));
#73538=CARTESIAN_POINT('Ctrl Pts',(0.191356801073853,1.67577508483846,9.20522606032421));
#73539=CARTESIAN_POINT('Ctrl Pts',(0.460280798172897,2.0312556126338,9.22509640384702));
#73540=CARTESIAN_POINT('Ctrl Pts',(0.306959824520678,2.44979975713437,9.2449667473698));
#73541=CARTESIAN_POINT('Ctrl Pts',(-0.127954999322651,2.54745024540095,
9.26483709089259));
#73542=CARTESIAN_POINT('Ctrl Pts',(-0.445488530787639,2.2346260483625,9.28470743441539));
#73543=CARTESIAN_POINT('Ctrl Pts',(-0.354346983041982,1.79830077963296,
9.30457777793815));
#73544=CARTESIAN_POINT('Ctrl Pts',(0.0618596816589883,1.63874347295017,
9.32444812146097));
#73545=CARTESIAN_POINT('Ctrl Pts',(0.421318509873045,1.90232623542972,9.34431846498375));
#73546=CARTESIAN_POINT('Ctrl Pts',(0.394274962614376,2.34724776604949,9.36418880850655));
#73547=CARTESIAN_POINT('Ctrl Pts',(0.00553781284629133,2.56535313106277,
9.38405915202932));
#73548=CARTESIAN_POINT('Ctrl Pts',(-0.38827952630312,2.35656035043407,9.4039294955521));
#73549=CARTESIAN_POINT('Ctrl Pts',(-0.425903259553746,1.91240837581992,
9.4237998390749));
#73550=CARTESIAN_POINT('Ctrl Pts',(-0.0728187336569238,1.64034617809743,
9.44367018259769));
#73551=CARTESIAN_POINT('Ctrl Pts',(0.347067066994716,1.78995378575329,9.46354052612046));
#73552=CARTESIAN_POINT('Ctrl Pts',(0.448566082593332,2.22398658599988,9.48341086964328));
#73553=CARTESIAN_POINT('Ctrl Pts',(0.138566784170425,2.54427857284107,9.50328121316604));
#73554=CARTESIAN_POINT('Ctrl Pts',(-0.298548674564602,2.4570054521667,9.52315155668886));
#73555=CARTESIAN_POINT('Ctrl Pts',(-0.461786368118551,2.04222843103298,
9.54302190021163));
#73556=CARTESIAN_POINT('Ctrl Pts',(-0.201397935460937,1.68044895953757,
9.56289224373443));
#73557=CARTESIAN_POINT('Ctrl Pts',(0.243745685128986,1.7035504509499,9.58276258725722));
#73558=CARTESIAN_POINT('Ctrl Pts',(0.465285822591689,2.09034043188319,9.60263293078001));
#73559=CARTESIAN_POINT('Ctrl Pts',(0.259989560771447,2.48599175153221,9.6225032743028));
#73560=CARTESIAN_POINT('Ctrl Pts',(-0.183811728673993,2.52754818718234,
9.64237361782559));
#73561=CARTESIAN_POINT('Ctrl Pts',(-0.458990780768273,2.17688736652246,
9.66224396134838));
#73562=CARTESIAN_POINT('Ctrl Pts',(-0.313108277460035,1.75569285434797,
9.68211430487117));
#73563=CARTESIAN_POINT('Ctrl Pts',(0.120008444574899,1.65035327512396,9.70198464839396));
#73564=CARTESIAN_POINT('Ctrl Pts',(0.443033756386806,1.95750335209969,9.72185499191675));
#73565=CARTESIAN_POINT('Ctrl Pts',(0.359635910313481,2.39537470435707,9.74172533543954));
#73566=CARTESIAN_POINT('Ctrl Pts',(-0.0536789234643323,2.56227997700175,
9.76159567896233));
#73567=CARTESIAN_POINT('Ctrl Pts',(-0.417750652689171,2.30510630448332,
9.78146602248512));
#73568=CARTESIAN_POINT('Ctrl Pts',(-0.398593029687583,1.8597755203034,9.80133636600791));
#73569=CARTESIAN_POINT('Ctrl Pts',(-0.0137805654886717,1.63481799263531,
9.82120670953068));
#73570=CARTESIAN_POINT('Ctrl Pts',(0.383673691491512,1.83660162791257,9.84107705305349));
#73571=CARTESIAN_POINT('Ctrl Pts',(0.429159568984776,2.28001741112968,9.86094739657626));
#73572=CARTESIAN_POINT('Ctrl Pts',(0.0809499667341075,2.55829172679285,
9.88081774009907));
#73573=CARTESIAN_POINT('Ctrl Pts',(-0.341520209652263,2.41614577390835,
9.90068808362184));
#73574=CARTESIAN_POINT('Ctrl Pts',(-0.450692087460871,1.98397911282362,
9.92055842714464));
#73575=CARTESIAN_POINT('Ctrl Pts',(-0.146415331211417,1.6582458209057,9.94042877066742));
#73576=CARTESIAN_POINT('Ctrl Pts',(0.29217755877707,1.73776184890586,9.96029911419022));
#73577=CARTESIAN_POINT('Ctrl Pts',(0.462737314970446,2.14958206626366,9.980169457713));
#73578=CARTESIAN_POINT('Ctrl Pts',(0.20879858067537,2.51591748781337,10.0000398012358));
#73579=CARTESIAN_POINT('Ctrl Pts',(-0.23668442602939,2.50070523634733,10.0199101447586));
#73580=CARTESIAN_POINT('Ctrl Pts',(-0.465041693527188,2.11790048162462,
10.0397804882814));
#73581=CARTESIAN_POINT('Ctrl Pts',(-0.26678651692355,1.71867447194184,10.0596508318042));
#73582=CARTESIAN_POINT('Ctrl Pts',(0.176208969252817,1.66926272146946,10.0795211753269));
#73583=CARTESIAN_POINT('Ctrl Pts',(0.457556714824719,2.0149937844635,10.0993915188498));
#73584=CARTESIAN_POINT('Ctrl Pts',(0.319158465266864,2.43870647766102,10.1192618623725));
#73585=CARTESIAN_POINT('Ctrl Pts',(-0.112024226671758,2.55170208832772,
10.1391322058953));
#73586=CARTESIAN_POINT('Ctrl Pts',(-0.440439941360369,2.25032252664023,
10.1590025494181));
#73587=CARTESIAN_POINT('Ctrl Pts',(-0.364811970334474,1.81104251132439,
10.1788728929409));
#73588=CARTESIAN_POINT('Ctrl Pts',(0.0454813188082286,1.63684165385853,
10.1987432364637));
#73589=CARTESIAN_POINT('Ctrl Pts',(0.414051689666831,1.88752552566232,10.2186135799865));
#73590=CARTESIAN_POINT('Ctrl Pts',(0.402786003303662,2.33312580188322,10.2384839235093));
#73591=CARTESIAN_POINT('Ctrl Pts',(0.0220189932722285,2.56486489208834,
10.2583542670321));
#73592=CARTESIAN_POINT('Ctrl Pts',(-0.378947445471223,2.37015372944282,
10.2782246105549));
#73593=CARTESIAN_POINT('Ctrl Pts',(-0.432281192031075,1.92761329814274,
10.2980949540776));
#73594=CARTESIAN_POINT('Ctrl Pts',(-0.0890557946726181,1.64321419746641,
10.3179652976004));
#73595=CARTESIAN_POINT('Ctrl Pts',(0.335866170446296,1.77785388484296,10.3378356411232));
#73596=CARTESIAN_POINT('Ctrl Pts',(0.452676648230991,2.20801877664271,10.357705984646));
#73597=CARTESIAN_POINT('Ctrl Pts',(0.154217927624591,2.53909114630132,10.3775763281688));
#73598=CARTESIAN_POINT('Ctrl Pts',(-0.285714746702346,2.46735716609023,
10.3974466716916));
#73599=CARTESIAN_POINT('Ctrl Pts',(-0.463543037480315,2.05862299715355,
10.4173170152144));
#73600=CARTESIAN_POINT('Ctrl Pts',(-0.216133697056242,1.68784659535819,
10.4371873587372));
#73601=CARTESIAN_POINT('Ctrl Pts',(0.229548886471042,1.69516483270233,10.45705770226));
#73602=CARTESIAN_POINT('Ctrl Pts',(0.464651616920155,2.07386422271074,10.4769280457828));
#73603=CARTESIAN_POINT('Ctrl Pts',(0.27349974545065,2.47653963031726,10.4967983893055));
#73604=CARTESIAN_POINT('Ctrl Pts',(-0.16855090884166,2.53379118834951,10.5166687328283));
#73605=CARTESIAN_POINT('Ctrl Pts',(-0.455979050405958,2.19309838640872,
10.5365390763511));
#73606=CARTESIAN_POINT('Ctrl Pts',(-0.325108489165098,1.76700048913877,
10.5564094198739));
#73607=CARTESIAN_POINT('Ctrl Pts',(0.104004851360552,1.6463843092942,10.5762797633967));
#73608=CARTESIAN_POINT('Ctrl Pts',(0.437707899744855,1.94189877147228,10.5961501069195));
#73609=CARTESIAN_POINT('Ctrl Pts',(0.369873538663006,2.38244958728584,10.6160204504423));
#73610=CARTESIAN_POINT('Ctrl Pts',(-0.0372694404067732,2.56389135880376,
10.635890793965));
#73611=CARTESIAN_POINT('Ctrl Pts',(-0.410222781679494,2.31977596172505,
10.6557611374879));
#73612=CARTESIAN_POINT('Ctrl Pts',(-0.406852567550072,1.87404603955906,
10.6756314810106));
#73613=CARTESIAN_POINT('Ctrl Pts',(-0.0302505106690354,1.63559811524361,
10.6955018245334));
#73614=CARTESIAN_POINT('Ctrl Pts',(0.374102271515687,1.82317569758449,10.7153721680562));
#73615=CARTESIAN_POINT('Ctrl Pts',(0.435267149010142,2.26470189116587,10.735242511579));
#73616=CARTESIAN_POINT('Ctrl Pts',(0.0971336735593306,2.55513652174034,
10.7551128551018));
#73617=CARTESIAN_POINT('Ctrl Pts',(-0.330106723826589,2.42804535486044,
10.7749831986246));
#73618=CARTESIAN_POINT('Ctrl Pts',(-0.454519142074015,2.00001723423843,
10.7948535421474));
#73619=CARTESIAN_POINT('Ctrl Pts',(-0.161972124662258,1.66370968977821,
10.8147238856702));
#73620=CARTESIAN_POINT('Ctrl Pts',(0.279162266613492,1.72763910938412,10.834594229193));
#73621=CARTESIAN_POINT('Ctrl Pts',(0.464203282782185,2.13315895377233,10.8544645727157));
#73622=CARTESIAN_POINT('Ctrl Pts',(0.223400982568651,2.50825997225836,10.8743349162385));
#73623=CARTESIAN_POINT('Ctrl Pts',(-0.222341305854143,2.50883804577376,
10.8942052597613));
#73624=CARTESIAN_POINT('Ctrl Pts',(-0.464115715191275,2.13436287056577,
10.9140756032841));
#73625=CARTESIAN_POINT('Ctrl Pts',(-0.280127139489603,1.72836443969608,
10.9339459468069));
#73626=CARTESIAN_POINT('Ctrl Pts',(0.160839950827386,1.66329104179227,10.9538162903297));
#73627=CARTESIAN_POINT('Ctrl Pts',(0.454258282642319,1.99883866048791,10.9736866338525));
#73628=CARTESIAN_POINT('Ctrl Pts',(0.330956481813854,2.42718803631311,10.9935569773753));
#73629=CARTESIAN_POINT('Ctrl Pts',(-0.0959528354223248,2.55538693145,11.0134273208981));
#73630=CARTESIAN_POINT('Ctrl Pts',(-0.434838488957494,2.2658303123141,11.0332976644208));
#73631=CARTESIAN_POINT('Ctrl Pts',(-0.374819026788911,1.82414695738845,
11.0531680079437));
#73632=CARTESIAN_POINT('Ctrl Pts',(0.0290458654557084,1.63552121505825,
11.0730383514664));
#73633=CARTESIAN_POINT('Ctrl Pts',(0.406265130382235,1.87299152483544,11.0929086949892));
#73634=CARTESIAN_POINT('Ctrl Pts',(0.410791446186281,2.31871120616287,11.112779038512));
#73635=CARTESIAN_POINT('Ctrl Pts',(0.038472534319897,2.56379313067792,11.1326493820348));
#73636=CARTESIAN_POINT('Ctrl Pts',(-0.369139690222393,2.38340799752927,
11.1525197255576));
#73637=CARTESIAN_POINT('Ctrl Pts',(-0.438116502816576,1.94303460916239,
11.1723900690804));
#73638=CARTESIAN_POINT('Ctrl Pts',(-0.105181068252582,1.64665559798066,
11.1922604126032));
#73639=CARTESIAN_POINT('Ctrl Pts',(0.324243677323718,1.76615835838436,11.212130756126));
#73640=CARTESIAN_POINT('Ctrl Pts',(0.456218990746203,2.19191537653487,11.2320010996487));
#73641=CARTESIAN_POINT('Ctrl Pts',(0.169675488766272,2.53335254986322,11.2518714431715));
#73642=CARTESIAN_POINT('Ctrl Pts',(-0.27252217492476,2.47724775431447,11.2717417866943));
#73643=CARTESIAN_POINT('Ctrl Pts',(-0.46471784366629,2.07506950182638,11.2916121302171));
#73644=CARTESIAN_POINT('Ctrl Pts',(-0.230598156465567,1.69576158743173,
11.3114824737399));
#73645=CARTESIAN_POINT('Ctrl Pts',(0.215063946188089,1.68728738447797,11.3313528172627));
#73646=CARTESIAN_POINT('Ctrl Pts',(0.463434156526629,2.0574208205166,11.3512231607855));
#73647=CARTESIAN_POINT('Ctrl Pts',(0.286666619115345,2.46661485709939,11.3710935043083));
#73648=CARTESIAN_POINT('Ctrl Pts',(-0.153078515198115,2.53948967239944,
11.3909638478311));
#73649=CARTESIAN_POINT('Ctrl Pts',(-0.452394951575326,2.2091925443892,11.4108341913539));
#73650=CARTESIAN_POINT('Ctrl Pts',(-0.336700607893486,1.77872612212446,
11.4307045348766));
#73651=CARTESIAN_POINT('Ctrl Pts',(0.0878707058819758,1.64298474532153,
11.4505748783994));
#73652=CARTESIAN_POINT('Ctrl Pts',(0.431832609527119,1.92649264767732,11.4704452219222));
#73653=CARTESIAN_POINT('Ctrl Pts',(0.379646882632345,2.36916992489611,11.490315565445));
#73654=CARTESIAN_POINT('Ctrl Pts',(-0.0208131748215914,2.56492044019905,
11.5101859089678));
#73655=CARTESIAN_POINT('Ctrl Pts',(-0.402179977834614,2.33416974482196,
11.5300562524906));
#73656=CARTESIAN_POINT('Ctrl Pts',(-0.414601403044297,1.8886001879028,11.5499265960134));
#73657=CARTESIAN_POINT('Ctrl Pts',(-0.0466824838451108,1.63696117909718,
11.5697969395362));
#73658=CARTESIAN_POINT('Ctrl Pts',(0.364061259035663,1.81009725142662,11.589667283059));
#73659=CARTESIAN_POINT('Ctrl Pts',(0.440828359216179,2.24917962887675,11.6095376265817));
#73660=CARTESIAN_POINT('Ctrl Pts',(0.113195453177793,2.55141000580503,11.6294079701045));
#73661=CARTESIAN_POINT('Ctrl Pts',(-0.318278870981795,2.43953315633025,
11.6492783136273));
#73662=CARTESIAN_POINT('Ctrl Pts',(-0.457775660771225,2.01618085918777,
11.6691486571501));
#73663=CARTESIAN_POINT('Ctrl Pts',(-0.17732560233177,1.66972121279488,11.6890190006729));
#73664=CARTESIAN_POINT('Ctrl Pts',(0.265796555546213,1.71798377649529,11.7088893441957));
#73665=CARTESIAN_POINT('Ctrl Pts',(0.46508655864411,2.11669421844861,11.7287596877185));
#73666=CARTESIAN_POINT('Ctrl Pts',(0.237722960003616,2.50008998768796,11.7486300312413));
#73667=CARTESIAN_POINT('Ctrl Pts',(-0.207719091381555,2.51645766055705,
11.7685003747641));
#73668=CARTESIAN_POINT('Ctrl Pts',(-0.462607154824915,2.15078212545596,
11.7883707182868));
#73669=CARTESIAN_POINT('Ctrl Pts',(-0.293116131993658,1.73852090361114,
11.8082410618096));
#73670=CARTESIAN_POINT('Ctrl Pts',(0.145269037783732,1.65786754176783,11.8281114053324));
#73671=CARTESIAN_POINT('Ctrl Pts',(0.450389641988224,1.98281051945354,11.8479817488552));
#73672=CARTESIAN_POINT('Ctrl Pts',(0.342339064681582,2.41525889163349,11.867852092378));
#73673=CARTESIAN_POINT('Ctrl Pts',(-0.0797609992151842,2.55850014936227,
11.8877224359008));
#73674=CARTESIAN_POINT('Ctrl Pts',(-0.428691204811542,2.28112993921011,
11.9075927794236));
#73675=CARTESIAN_POINT('Ctrl Pts',(-0.384355591030892,1.83759766844724,
11.9274631229464));
#73676=CARTESIAN_POINT('Ctrl Pts',(0.0125739522318252,1.63478381403233,
11.9473334664692));
#73677=CARTESIAN_POINT('Ctrl Pts',(0.397968606110868,1.85874247677801,11.967203809992));
#73678=CARTESIAN_POINT('Ctrl Pts',(0.41828124241662,2.3040220728339,11.9870741535147));
#73679=CARTESIAN_POINT('Ctrl Pts',(0.0548777826542892,2.56213919216181,
12.0069444970375));
#73680=CARTESIAN_POINT('Ctrl Pts',(-0.358868571757863,2.39630651725115,
12.0268148405603));
#73681=CARTESIAN_POINT('Ctrl Pts',(-0.443401867126601,1.95865295125233,
12.0466851840831));
#73682=CARTESIAN_POINT('Ctrl Pts',(-0.12117431312009,1.65066605981642,12.0665555276059));
#73683=CARTESIAN_POINT('Ctrl Pts',(0.312214176780983,1.7548818872067,12.0864258711287));
#73684=CARTESIAN_POINT('Ctrl Pts',(0.459188663607583,2.17569659949637,12.1062962146515));
#73685=CARTESIAN_POINT('Ctrl Pts',(0.184920064465904,2.52706998690959,12.1261665581743));
#73686=CARTESIAN_POINT('Ctrl Pts',(-0.258987519229711,2.48666480166194,
12.1460369016971));
#73687=CARTESIAN_POINT('Ctrl Pts',(-0.465309311999041,2.09154730054888,
12.1659072452199));
#73688=CARTESIAN_POINT('Ctrl Pts',(-0.244773157151966,1.70418400045111,
12.1857775887426));
#73689=CARTESIAN_POINT('Ctrl Pts',(0.20030904652572,1.67992799445691,12.2056479322654));
#73690=CARTESIAN_POINT('Ctrl Pts',(0.461634969630317,2.04103086590896,12.2255182757882));
#73691=CARTESIAN_POINT('Ctrl Pts',(0.299473654025266,2.45622988996684,12.245388619311));
#73692=CARTESIAN_POINT('Ctrl Pts',(-0.137413969491446,2.54463648630048,
12.2652589628338));
#73693=CARTESIAN_POINT('Ctrl Pts',(-0.448242983222447,2.22514963824505,
12.2851293063566));
#73694=CARTESIAN_POINT('Ctrl Pts',(-0.347870082618712,1.79085503468456,
12.3049996498794));
#73695=CARTESIAN_POINT('Ctrl Pts',(0.0716262605523633,1.64015885051431,
12.3248699934022));
#73696=CARTESIAN_POINT('Ctrl Pts',(0.425415260701503,1.91130431927756,12.3447403369249));
#73697=CARTESIAN_POINT('Ctrl Pts',(0.388943674215075,2.35555238650639,12.3646106804478));
#73698=CARTESIAN_POINT('Ctrl Pts',(-0.00433078346378373,2.56536592943147,
12.3844810239705));
#73699=CARTESIAN_POINT('Ctrl Pts',(-0.393632336897545,2.34826958595367,
12.4043513674933));
#73700=CARTESIAN_POINT('Ctrl Pts',(-0.421829809431507,1.90341969621549,
12.4242217110161));
#73701=CARTESIAN_POINT('Ctrl Pts',(-0.0630558587549978,1.63890547320782,
12.4440920545389));
#73702=CARTESIAN_POINT('Ctrl Pts',(0.353563258049211,1.79738270618047,12.4639623980617));
#73703=CARTESIAN_POINT('Ctrl Pts',(0.445836218884442,2.23347010860809,12.4838327415845));
#73704=CARTESIAN_POINT('Ctrl Pts',(0.129115144013671,2.54711685670232,12.5037030851073));
#73705=CARTESIAN_POINT('Ctrl Pts',(-0.306051498050013,2.45059475823574,
12.5235734286301));
#73706=CARTESIAN_POINT('Ctrl Pts',(-0.46045755580194,2.03244969825429,12.5434437721529));
#73707=CARTESIAN_POINT('Ctrl Pts',(-0.192456491741336,1.67627284398136,
12.5633141156756));
#73708=CARTESIAN_POINT('Ctrl Pts',(0.25209720290648,1.70880797011217,12.5831844591984));
#73709=CARTESIAN_POINT('Ctrl Pts',(0.465386033822722,2.10020852767918,12.6030548027212));
#73710=CARTESIAN_POINT('Ctrl Pts',(0.251746535294047,2.49141778948901,12.622925146244));
#73711=CARTESIAN_POINT('Ctrl Pts',(-0.192836137170855,2.52355451616297,
12.6427954897668));
#73712=CARTESIAN_POINT('Ctrl Pts',(-0.460517906051078,2.16713763599796,
12.6626658332896));
#73713=CARTESIAN_POINT('Ctrl Pts',(-0.305737189981008,1.74913111476862,
12.6825361768124));
#73714=CARTESIAN_POINT('Ctrl Pts',(0.129515775536461,1.65299902925365,12.7024065203352));
#73715=CARTESIAN_POINT('Ctrl Pts',(0.445955648980351,1.96692948071131,12.722276863858));
#73716=CARTESIAN_POINT('Ctrl Pts',(0.353291925863331,2.40293401770104,12.7421472073807));
#73717=CARTESIAN_POINT('Ctrl Pts',(-0.0634690428790086,2.56103783419247,
12.7620175509035));
#73718=CARTESIAN_POINT('Ctrl Pts',(-0.422005805312989,2.29620220244602,
12.7818878944263));
#73719=CARTESIAN_POINT('Ctrl Pts',(-0.393409692268796,1.8513777604729,12.8017582379491));
#73720=CARTESIAN_POINT('Ctrl Pts',(-0.00391374447314742,1.63463037640504,
12.8216285814719));
#73721=CARTESIAN_POINT('Ctrl Pts',(0.389172531091156,1.84479626763077,12.8414989249947));
#73722=CARTESIAN_POINT('Ctrl Pts',(0.425245990391475,2.28907684045705,12.8613692685175));
#73723=CARTESIAN_POINT('Ctrl Pts',(0.0712141456059791,2.55990515264628,
12.8812396120403));
#73724=CARTESIAN_POINT('Ctrl Pts',(-0.34814698300506,2.40883309772541,12.9011099555631));
#73725=CARTESIAN_POINT('Ctrl Pts',(-0.448130650327812,1.97444871945192,
12.9209802990858));
#73726=CARTESIAN_POINT('Ctrl Pts',(-0.137015454056879,1.65524054885501,
12.9408506426087));
#73727=CARTESIAN_POINT('Ctrl Pts',(0.299792769502911,1.74403862608033,12.9607209861314));
#73728=CARTESIAN_POINT('Ctrl Pts',(0.461581937906987,2.15938280424948,12.9805913296542));
#73729=CARTESIAN_POINT('Ctrl Pts',(0.199932521296602,2.5202513434933,13.000461673177));
#73730=CARTESIAN_POINT('Ctrl Pts',(-0.245127773547357,2.49559648764708,
13.0203320166998));
#73731=CARTESIAN_POINT('Ctrl Pts',(-0.465316691309975,2.10803570899936,
13.0402023602226));
#73732=CARTESIAN_POINT('Ctrl Pts',(-0.258640922731129,1.71310326320296,
13.0600727037454));
#73733=CARTESIAN_POINT('Ctrl Pts',(0.185302740972675,1.67309589853287,13.0799430472682));
#73734=CARTESIAN_POINT('Ctrl Pts',(0.459256252303584,2.02471493624459,13.099813390791));
#73735=CARTESIAN_POINT('Ctrl Pts',(0.311904894240494,2.44539775727322,13.1196837343137));
#73736=CARTESIAN_POINT('Ctrl Pts',(-0.121577166018006,2.54922518374711,
13.1395540778365));
#73737=CARTESIAN_POINT('Ctrl Pts',(-0.443527911509105,2.24094961037721,
13.1594244213593));
#73738=CARTESIAN_POINT('Ctrl Pts',(-0.358603751119627,1.80337205481489,
13.1792947648821));
#73739=CARTESIAN_POINT('Ctrl Pts',(0.0552935593811353,1.63791007031839,
13.1991651084049));
#73740=CARTESIAN_POINT('Ctrl Pts',(0.418460724523598,1.89635304745533,13.2190354519277));
#73741=CARTESIAN_POINT('Ctrl Pts',(0.397758376589411,2.34161368802065,13.2389057954505));
#73742=CARTESIAN_POINT('Ctrl Pts',(0.0121452312493891,2.56522799449065,
13.2587761389733));
#73743=CARTESIAN_POINT('Ctrl Pts',(-0.384567834882505,2.36205638544088,
13.2786464824961));
#73744=CARTESIAN_POINT('Ctrl Pts',(-0.428572544079887,1.91848866214859,
13.2985168260188));
#73745=CARTESIAN_POINT('Ctrl Pts',(-0.0792656100846051,1.64142334060457,
13.3183871695417));
#73746=CARTESIAN_POINT('Ctrl Pts',(0.342458274427398,1.78505822158492,13.3382575130644));
#73747=CARTESIAN_POINT('Ctrl Pts',(0.450603146122972,2.21757196606139,13.3581278565872));
#73748=CARTESIAN_POINT('Ctrl Pts',(0.144148881373328,2.54238907754302,13.3780026364007));
#73749=CARTESIAN_POINT('Ctrl Pts',(-0.146654456177299,2.48806903884852,
13.3912539683733));
#73750=CARTESIAN_POINT('Ctrl Pts',(-0.248368994146077,2.40531761840563,
13.3978818525049));
#73751=CARTESIAN_POINT('Ctrl Pts',(-0.203466370082455,2.35062899684047,
4.3567));
#73752=CARTESIAN_POINT('Ctrl Pts',(-0.198643714809141,2.35553329018579,
4.3567));
#73753=CARTESIAN_POINT('Ctrl Pts',(-0.193660853029549,2.36026430325056,
4.3567));
#73754=CARTESIAN_POINT('Ctrl Pts',(-0.188522749684309,2.36481173887452,
4.3567));
#73755=CARTESIAN_POINT('Ctrl Pts',(-0.174734518930225,2.37701489780488,
4.3567));
#73756=CARTESIAN_POINT('Ctrl Pts',(-0.159831435216182,2.38789858237333,
4.3567));
#73757=CARTESIAN_POINT('Ctrl Pts',(-0.144036878378854,2.3974639952058,4.3567));
#73758=CARTESIAN_POINT('Ctrl Pts',(-0.141576690706492,2.39895392056261,
4.3567));
#73759=CARTESIAN_POINT('Ctrl Pts',(-0.139094796118624,2.40041179592735,
4.3567));
#73760=CARTESIAN_POINT('Ctrl Pts',(-0.136591958438483,2.40183754983713,
4.3567));
#73761=CARTESIAN_POINT('Ctrl Pts',(-0.131420216294938,2.4047836584242,4.3567));
#73762=CARTESIAN_POINT('Ctrl Pts',(-0.12616810244625,2.40758749052332,4.3567));
#73763=CARTESIAN_POINT('Ctrl Pts',(-0.120843445135949,2.41024936098874,
4.3567));
#73764=CARTESIAN_POINT('Ctrl Pts',(-0.105969803272818,2.41768490203512,
4.3567));
#73765=CARTESIAN_POINT('Ctrl Pts',(-0.0905311339839462,2.42401457076917,
4.3567));
#73766=CARTESIAN_POINT('Ctrl Pts',(-0.0746791492274175,2.42923308272867,
4.3567));
#73767=CARTESIAN_POINT('Ctrl Pts',(-0.0679382765650449,2.43145219441382,
4.3567));
#73768=CARTESIAN_POINT('Ctrl Pts',(-0.0611197830975242,2.43347078159887,
4.3567));
#73769=CARTESIAN_POINT('Ctrl Pts',(-0.0542434236638015,2.4352848700941,
4.3567));
#73770=CARTESIAN_POINT('Ctrl Pts',(-0.0458797197062097,2.43749134275936,
4.3567));
#73771=CARTESIAN_POINT('Ctrl Pts',(-0.0374438472594873,2.43939194329253,
4.3567));
#73772=CARTESIAN_POINT('Ctrl Pts',(-0.0289612584600339,2.44098632127078,
4.3567));
#73773=CARTESIAN_POINT('Ctrl Pts',(-0.0091843508866179,2.44470356687333,
4.3567));
#73774=CARTESIAN_POINT('Ctrl Pts',(0.0108541911413975,2.44676182489034,
4.3567));
#73775=CARTESIAN_POINT('Ctrl Pts',(0.0309100698820238,2.44713877334642,
4.3567));
#73776=CARTESIAN_POINT('Ctrl Pts',(0.0450748590705997,2.44740499929864,
4.3567));
#73777=CARTESIAN_POINT('Ctrl Pts',(0.0592490886611076,2.44683168334103,
4.35670000000001));
#73778=CARTESIAN_POINT('Ctrl Pts',(0.073350647231715,2.44539578335235,4.3567));
#73779=CARTESIAN_POINT('Ctrl Pts',(0.0795644863214801,2.44476305531496,
4.3567));
#73780=CARTESIAN_POINT('Ctrl Pts',(0.0857603507931046,2.44396272953801,
4.3567));
#73781=CARTESIAN_POINT('Ctrl Pts',(0.0919138197553597,2.44299632212969,
4.3567));
#73782=CARTESIAN_POINT('Ctrl Pts',(0.105989893738086,2.44078566302662,4.3567));
#73783=CARTESIAN_POINT('Ctrl Pts',(0.119869569405396,2.43770438812349,4.3567));
#73784=CARTESIAN_POINT('Ctrl Pts',(0.133470056976512,2.43374310478803,4.3567));
#73785=CARTESIAN_POINT('Ctrl Pts',(0.150216753309979,2.42886545545649,4.35670000000001));
#73786=CARTESIAN_POINT('Ctrl Pts',(0.16654080005684,2.42265470234242,4.35670000000001));
#73787=CARTESIAN_POINT('Ctrl Pts',(0.182361818588615,2.41523366612292,4.3567));
#73788=CARTESIAN_POINT('Ctrl Pts',(0.189998595912251,2.41165154522438,4.3567));
#73789=CARTESIAN_POINT('Ctrl Pts',(0.197518709781143,2.40778664511544,4.3567));
#73790=CARTESIAN_POINT('Ctrl Pts',(0.204911457815444,2.40365083222556,4.3567));
#73791=CARTESIAN_POINT('Ctrl Pts',(0.210963294651808,2.40026518122282,4.3567));
#73792=CARTESIAN_POINT('Ctrl Pts',(0.21692334188249,2.39670120955451,4.3567));
#73793=CARTESIAN_POINT('Ctrl Pts',(0.222772819046754,2.39297545721447,4.3567));
#73794=CARTESIAN_POINT('Ctrl Pts',(0.240435976311113,2.38172512702901,4.3567));
#73795=CARTESIAN_POINT('Ctrl Pts',(0.25712640745556,2.36898505359157,4.3567));
#73796=CARTESIAN_POINT('Ctrl Pts',(0.272712722894781,2.35495932065901,4.3567));
#73797=CARTESIAN_POINT('Ctrl Pts',(0.284847641215269,2.34403941311669,4.3567));
#73798=CARTESIAN_POINT('Ctrl Pts',(0.296313349003292,2.33233885512433,4.3567));
#73799=CARTESIAN_POINT('Ctrl Pts',(0.30703861953246,2.31993423667894,4.3567));
#73800=CARTESIAN_POINT('Ctrl Pts',(0.310476070462662,2.3159585544714,4.3567));
#73801=CARTESIAN_POINT('Ctrl Pts',(0.313837377253384,2.31191043772024,4.3567));
#73802=CARTESIAN_POINT('Ctrl Pts',(0.317119922049988,2.30779211050345,4.3567));
#73803=CARTESIAN_POINT('Ctrl Pts',(0.326850704545219,2.29558373289585,4.3567));
#73804=CARTESIAN_POINT('Ctrl Pts',(0.33583295276189,2.28283021741324,4.3567));
#73805=CARTESIAN_POINT('Ctrl Pts',(0.344012277935068,2.2696119465451,4.3567));
#73806=CARTESIAN_POINT('Ctrl Pts',(0.355355398230413,2.25128079655666,4.3567));
#73807=CARTESIAN_POINT('Ctrl Pts',(0.365158565020612,2.23205391983181,4.3567));
#73808=CARTESIAN_POINT('Ctrl Pts',(0.373259765356344,2.2120995657669,4.3567));
#73809=CARTESIAN_POINT('Ctrl Pts',(0.377716509485494,2.20112200112904,4.3567));
#73810=CARTESIAN_POINT('Ctrl Pts',(0.381657543398439,2.18992363295171,4.3567));
#73811=CARTESIAN_POINT('Ctrl Pts',(0.385050100177468,2.17852889782573,4.3567));
#73812=CARTESIAN_POINT('Ctrl Pts',(0.385401167965355,2.1773497504408,4.3567));
#73813=CARTESIAN_POINT('Ctrl Pts',(0.385746358064522,2.17616849861351,4.3567));
#73814=CARTESIAN_POINT('Ctrl Pts',(0.386085631082114,2.17498516834631,4.3567));
#73815=CARTESIAN_POINT('Origin',(-5.160062080289E-17,2.1,4.3567));
#73816=CARTESIAN_POINT('Ctrl Pts',(0.287740166859834,1.83187598694732,4.3567));
#73817=CARTESIAN_POINT('Ctrl Pts',(0.283540929289304,1.82807333637404,4.3567));
#73818=CARTESIAN_POINT('Ctrl Pts',(0.279255381327226,1.82437166421582,4.3567));
#73819=CARTESIAN_POINT('Ctrl Pts',(0.274884385304385,1.82077515375635,4.3567));
#73820=CARTESIAN_POINT('Ctrl Pts',(0.25810235391389,1.80696668742242,4.3567));
#73821=CARTESIAN_POINT('Ctrl Pts',(0.240062114400838,1.79470455623045,4.3567));
#73822=CARTESIAN_POINT('Ctrl Pts',(0.221014146357085,1.78403910870001,4.3567));
#73823=CARTESIAN_POINT('Ctrl Pts',(0.218046748141756,1.78237758606963,4.3567));
#73824=CARTESIAN_POINT('Ctrl Pts',(0.215054865633032,1.78075491256672,4.3567));
#73825=CARTESIAN_POINT('Ctrl Pts',(0.212039424147889,1.77917138918029,4.3567));
#73826=CARTESIAN_POINT('Ctrl Pts',(0.206236204436223,1.77612389707164,4.3567));
#73827=CARTESIAN_POINT('Ctrl Pts',(0.200354322111735,1.77322592154459,4.3567));
#73828=CARTESIAN_POINT('Ctrl Pts',(0.194402554160535,1.77047920260614,4.3567));
#73829=CARTESIAN_POINT('Ctrl Pts',(0.178891787748209,1.76332104116505,4.3567));
#73830=CARTESIAN_POINT('Ctrl Pts',(0.16290270656968,1.757186694163,4.3567));
#73831=CARTESIAN_POINT('Ctrl Pts',(0.14655689918141,1.75210485469583,4.3567));
#73832=CARTESIAN_POINT('Ctrl Pts',(0.139384822531743,1.74987508767887,4.3567));
#73833=CARTESIAN_POINT('Ctrl Pts',(0.132143750868839,1.74784812676099,4.3567));
#73834=CARTESIAN_POINT('Ctrl Pts',(0.124844069854122,1.7460277175469,4.3567));
#73835=CARTESIAN_POINT('Ctrl Pts',(0.11859715027019,1.74446984810748,4.3567));
#73836=CARTESIAN_POINT('Ctrl Pts',(0.112309084212408,1.74306396104996,4.3567));
#73837=CARTESIAN_POINT('Ctrl Pts',(0.106001682669741,1.74181480813219,4.3567));
#73838=CARTESIAN_POINT('Ctrl Pts',(0.0854450059383791,1.73774364942367,
4.3567));
#73839=CARTESIAN_POINT('Ctrl Pts',(0.0646473420272781,1.73532368510841,
4.3567));
#73840=CARTESIAN_POINT('Ctrl Pts',(0.0438340188223849,1.73461140981212,
4.3567));
#73841=CARTESIAN_POINT('Ctrl Pts',(0.0315896664796848,1.73419238255698,
4.3567));
#73842=CARTESIAN_POINT('Ctrl Pts',(0.0193398602704868,1.73436532131983,
4.3567));
#73843=CARTESIAN_POINT('Ctrl Pts',(0.00713247518961179,1.73515005238391,
4.3567));
#73844=CARTESIAN_POINT('Ctrl Pts',(-0.000437632244075232,1.73563668391247,
4.3567));
#73845=CARTESIAN_POINT('Ctrl Pts',(-0.00799138412230426,1.73635870589722,
4.3567));
#73846=CARTESIAN_POINT('Ctrl Pts',(-0.0155167357365803,1.73732206252591,
4.3567));
#73847=CARTESIAN_POINT('Ctrl Pts',(-0.0218591581541978,1.73813398667128,
4.3567));
#73848=CARTESIAN_POINT('Ctrl Pts',(-0.028183730479901,1.73911809273902,
4.3567));
#73849=CARTESIAN_POINT('Ctrl Pts',(-0.0344595927017996,1.74027323764255,
4.3567));
#73850=CARTESIAN_POINT('Ctrl Pts',(-0.0494189029188666,1.74302667140936,
4.3567));
#73851=CARTESIAN_POINT('Ctrl Pts',(-0.0641299531612682,1.74675330792951,
4.3567));
#73852=CARTESIAN_POINT('Ctrl Pts',(-0.0785012988446161,1.75148487175215,
4.3567));
#73853=CARTESIAN_POINT('Ctrl Pts',(-0.0986706061389512,1.75812533304398,
4.3567));
#73854=CARTESIAN_POINT('Ctrl Pts',(-0.118172845707065,1.76674387676704,
4.3567));
#73855=CARTESIAN_POINT('Ctrl Pts',(-0.136807949554667,1.77715217457513,
4.3567));
#73856=CARTESIAN_POINT('Ctrl Pts',(-0.142094148121254,1.78010468449424,
4.3567));
#73857=CARTESIAN_POINT('Ctrl Pts',(-0.147312413818575,1.78320284198279,
4.3567));
#73858=CARTESIAN_POINT('Ctrl Pts',(-0.152450181179759,1.78643826777209,
4.3567));
#73859=CARTESIAN_POINT('Ctrl Pts',(-0.158904634512563,1.79050285522823,
4.3567));
#73860=CARTESIAN_POINT('Ctrl Pts',(-0.165222236643709,1.79477770660458,
4.3567));
#73861=CARTESIAN_POINT('Ctrl Pts',(-0.171390503137907,1.79924948335615,
4.3567));
#73862=CARTESIAN_POINT('Ctrl Pts',(-0.187020189413487,1.81058045742919,
4.3567));
#73863=CARTESIAN_POINT('Ctrl Pts',(-0.201704919669262,1.82318105360677,
4.3567));
#73864=CARTESIAN_POINT('Ctrl Pts',(-0.215292904901525,1.83690543855032,
4.3567));
#73865=CARTESIAN_POINT('Ctrl Pts',(-0.222370765829106,1.8440543488771,4.3567));
#73866=CARTESIAN_POINT('Ctrl Pts',(-0.229150448230971,1.85150865969543,
4.3567));
#73867=CARTESIAN_POINT('Ctrl Pts',(-0.235605904128297,1.85925002016915,
4.3567));
#73868=CARTESIAN_POINT('Ctrl Pts',(-0.239875651825072,1.8643702868983,4.3567));
#73869=CARTESIAN_POINT('Ctrl Pts',(-0.244004693787793,1.86961778453864,
4.3567));
#73870=CARTESIAN_POINT('Ctrl Pts',(-0.247980890826324,1.874982371717,4.3567));
#73871=CARTESIAN_POINT('Ctrl Pts',(-0.251720955269355,1.88002837460943,
4.3567));
#73872=CARTESIAN_POINT('Ctrl Pts',(-0.255320614079644,1.88517104298149,
4.3567));
#73873=CARTESIAN_POINT('Ctrl Pts',(-0.258770422630349,1.89039903119355,
4.3567));
#73874=CARTESIAN_POINT('Ctrl Pts',(-0.269038181960046,1.90595923517325,
4.3567));
#73875=CARTESIAN_POINT('Ctrl Pts',(-0.277995587721695,1.92229271891481,
4.3567));
#73876=CARTESIAN_POINT('Ctrl Pts',(-0.285483839243767,1.93927368372052,
4.3567));
#73877=CARTESIAN_POINT('Ctrl Pts',(-0.292051816918351,1.95416776111737,
4.3567));
#73878=CARTESIAN_POINT('Ctrl Pts',(-0.297489248769509,1.96956071430832,
4.3567));
#73879=CARTESIAN_POINT('Ctrl Pts',(-0.301655992406196,1.98537103162613,
4.3567));
#73880=CARTESIAN_POINT('Ctrl Pts',(-0.301998194302805,1.98666948457738,
4.3567));
#73881=CARTESIAN_POINT('Ctrl Pts',(-0.302331806399809,1.98797075138032,
4.3567));
#73882=CARTESIAN_POINT('Ctrl Pts',(-0.302656740537857,1.98927478592477,
4.3567));
#73883=CARTESIAN_POINT('Ctrl Pts',(-0.369736275429134,1.96501449663477,
4.3155034837597));
#73884=CARTESIAN_POINT('Ctrl Pts',(-0.324771331358241,1.84183163773061,
4.32213136767731));
#73885=CARTESIAN_POINT('Ctrl Pts',(-0.102837691495962,1.64619446151566,
4.33538269943585));
#73886=CARTESIAN_POINT('Ctrl Pts',(0.326776737212504,1.76816965157351,4.35525747903531));
#73887=CARTESIAN_POINT('Ctrl Pts',(0.45547744888119,2.19504797546089,4.37512782255811));
#73888=CARTESIAN_POINT('Ctrl Pts',(0.166857071268261,2.53446779707742,4.3949981660809));
#73889=CARTESIAN_POINT('Ctrl Pts',(-0.275097988964059,2.4754595193049,4.41486850960369));
#73890=CARTESIAN_POINT('Ctrl Pts',(-0.464550239979861,2.07194719672028,
4.43473885312647));
#73891=CARTESIAN_POINT('Ctrl Pts',(-0.227912439379459,1.69420638760595,
4.45460919664927));
#73892=CARTESIAN_POINT('Ctrl Pts',(0.217841145994397,1.68870682220133,4.47447954017205));
#73893=CARTESIAN_POINT('Ctrl Pts',(0.46373584719812,2.06052269932018,4.49434988369485));
#73894=CARTESIAN_POINT('Ctrl Pts',(0.284226056250109,2.46854846190176,4.51422022721762));
#73895=CARTESIAN_POINT('Ctrl Pts',(-0.156027648019584,2.53848386517764,
4.53409057074043));
#73896=CARTESIAN_POINT('Ctrl Pts',(-0.453144526100725,2.20616862417218,
4.5539609142632));
#73897=CARTESIAN_POINT('Ctrl Pts',(-0.334564393695026,1.7764588469168,4.57383125778601));
#73898=CARTESIAN_POINT('Ctrl Pts',(0.0909337511562546,1.6435536561162,4.59370160130879));
#73899=CARTESIAN_POINT('Ctrl Pts',(0.433012180793506,1.92937604116777,4.61357194483159));
#73900=CARTESIAN_POINT('Ctrl Pts',(0.377861080133257,2.37172257889418,4.63344228835436));
#73901=CARTESIAN_POINT('Ctrl Pts',(-0.0239262223333663,2.56480069472104,
4.65331263187717));
#73902=CARTESIAN_POINT('Ctrl Pts',(-0.403764420146204,2.33148742275733,
4.67318297539994));
#73903=CARTESIAN_POINT('Ctrl Pts',(-0.413203757517612,1.88581596874811,
4.69305331892275));
#73904=CARTESIAN_POINT('Ctrl Pts',(-0.0435848857095753,1.63662919753327,
4.71292366244552));
#73905=CARTESIAN_POINT('Ctrl Pts',(0.366017177781486,1.81252205916294,4.73279400596832));
#73906=CARTESIAN_POINT('Ctrl Pts',(0.439848313244426,2.25213679293958,4.7526643494911));
#73907=CARTESIAN_POINT('Ctrl Pts',(0.110178499248734,2.55218673177814,4.7725346930139));
#73908=CARTESIAN_POINT('Ctrl Pts',(-0.320565087322196,2.43741690334024,
4.79240503653668));
#73909=CARTESIAN_POINT('Ctrl Pts',(-0.45723384780948,2.01311300152881,4.81227538005947));
#73910=CARTESIAN_POINT('Ctrl Pts',(-0.174452799419451,1.66851609207379,
4.83214572358226));
#73911=CARTESIAN_POINT('Ctrl Pts',(0.268364942688647,1.71974692698616,4.85201606710506));
#73912=CARTESIAN_POINT('Ctrl Pts',(0.46499438454321,2.11980818956847,4.87188641062784));
#73913=CARTESIAN_POINT('Ctrl Pts',(0.235054781809442,2.50169813488339,4.89175675415064));
#73914=CARTESIAN_POINT('Ctrl Pts',(-0.210515583395179,2.51508472769526,
4.91162709767341));
#73915=CARTESIAN_POINT('Ctrl Pts',(-0.462966559954061,2.14768759153516,
4.93149744119622));
#73916=CARTESIAN_POINT('Ctrl Pts',(-0.290708744955435,1.73654358221807,
4.951367784719));
#73917=CARTESIAN_POINT('Ctrl Pts',(0.148234767115052,1.65882135609411,4.97123812824179));
#73918=CARTESIAN_POINT('Ctrl Pts',(0.45119306070023,1.98582047470415,4.99110847176458));
#73919=CARTESIAN_POINT('Ctrl Pts',(0.340243145480813,2.41756376363479,5.01097881528736));
#73920=CARTESIAN_POINT('Ctrl Pts',(-0.0828335357952513,2.55798553183285,
5.03084915881016));
#73921=CARTESIAN_POINT('Ctrl Pts',(-0.429921724746993,2.27826792367447,
5.05071950233295));
#73922=CARTESIAN_POINT('Ctrl Pts',(-0.382615259800999,1.83501376453104,
5.07058984585574));
#73923=CARTESIAN_POINT('Ctrl Pts',(0.0156886176482768,1.63484840181196,
5.09046018937852));
#73924=CARTESIAN_POINT('Ctrl Pts',(0.399600324217718,1.86139630575847,5.11033053290132));
#73925=CARTESIAN_POINT('Ctrl Pts',(0.416933133989187,2.30683061621182,5.13020087642411));
#73926=CARTESIAN_POINT('Ctrl Pts',(0.0517865536463587,2.56252599373661,
5.1500712199469));
#73927=CARTESIAN_POINT('Ctrl Pts',(-0.360867139564347,2.39391673923622,
5.16994156346968));
#73928=CARTESIAN_POINT('Ctrl Pts',(-0.442474359849625,1.95567888963748,
5.18981190699248));
#73929=CARTESIAN_POINT('Ctrl Pts',(-0.118171592417568,1.64983601125134,
5.20968225051526));
#73930=CARTESIAN_POINT('Ctrl Pts',(0.314537523448001,1.75695730824896,5.22955259403806));
#73931=CARTESIAN_POINT('Ctrl Pts',(0.458701281967192,2.17877357388274,5.24942293756084));
#73932=CARTESIAN_POINT('Ctrl Pts',(0.182069060822143,2.52832580953282,5.26929328108364));
#73933=CARTESIAN_POINT('Ctrl Pts',(-0.261586737162791,2.48494742623004,
5.28916362460641));
#73934=CARTESIAN_POINT('Ctrl Pts',(-0.465272315619407,2.08843218522106,
5.30903396812922));
#73935=CARTESIAN_POINT('Ctrl Pts',(-0.242133885601332,1.70252883945599,
5.328904311652));
#73936=CARTESIAN_POINT('Ctrl Pts',(0.203129420904025,1.68125117267771,5.34877465517479));
#73937=CARTESIAN_POINT('Ctrl Pts',(0.462049137303498,2.04411854746253,5.36864499869758));
#73938=CARTESIAN_POINT('Ctrl Pts',(0.297101672537019,2.45824954737767,5.38851534222037));
#73939=CARTESIAN_POINT('Ctrl Pts',(-0.140396130041771,2.54373535884567,
5.40838568574316));
#73940=CARTESIAN_POINT('Ctrl Pts',(-0.449099596514432,2.22215438768698,
5.42825602926594));
#73941=CARTESIAN_POINT('Ctrl Pts',(-0.345815322574325,1.78851339564369,
5.44812637278874));
#73942=CARTESIAN_POINT('Ctrl Pts',(0.0747074313227155,1.64061895802529,
5.46799671631152));
#73943=CARTESIAN_POINT('Ctrl Pts',(0.426696287479547,1.91414408733705,5.48786705983432));
#73944=CARTESIAN_POINT('Ctrl Pts',(0.387249389327999,2.35816671451931,5.5077374033571));
#73945=CARTESIAN_POINT('Ctrl Pts',(-0.00744610428814212,2.5653565273546,
5.5276077468799));
#73946=CARTESIAN_POINT('Ctrl Pts',(-0.395310810915475,2.34564507891255,
5.54747809040268));
#73947=CARTESIAN_POINT('Ctrl Pts',(-0.420531665235156,1.90058771212598,
5.56734843392548));
#73948=CARTESIAN_POINT('Ctrl Pts',(-0.0599719669181471,1.63846397193223,
5.58721877744826));
#73949=CARTESIAN_POINT('Ctrl Pts',(0.355603846600209,1.79973670503416,5.60708912097106));
#73950=CARTESIAN_POINT('Ctrl Pts',(0.4449615419551,2.23646013411083,5.62695946449384));
#73951=CARTESIAN_POINT('Ctrl Pts',(0.126127598610152,2.54799996751054,5.64682980801663));
#73952=CARTESIAN_POINT('Ctrl Pts',(-0.30841124573757,2.44856082040759,5.66670015153942));
#73953=CARTESIAN_POINT('Ctrl Pts',(-0.460024758520828,2.02936457285146,
5.68657049506221));
#73954=CARTESIAN_POINT('Ctrl Pts',(-0.189628182076955,1.67496671355905,
5.706440838585));
#73955=CARTESIAN_POINT('Ctrl Pts',(0.254726435876664,1.71047903151925,5.72631118210778));
#73956=CARTESIAN_POINT('Ctrl Pts',(0.465404226786298,2.10332380956912,5.74618152563059));
#73957=CARTESIAN_POINT('Ctrl Pts',(0.249136998683705,2.49311944483512,5.76605186915336));
#73958=CARTESIAN_POINT('Ctrl Pts',(-0.195679508771493,2.52228150784466,
5.78592221267616));
#73959=CARTESIAN_POINT('Ctrl Pts',(-0.46098670628845,2.16405777584283,5.80579255619895));
#73960=CARTESIAN_POINT('Ctrl Pts',(-0.303401358458842,1.74706975518393,
5.82566289972174));
#73961=CARTESIAN_POINT('Ctrl Pts',(0.132513431391554,1.65384718702956,5.84553324324452));
#73962=CARTESIAN_POINT('Ctrl Pts',(0.446865188014881,1.96990908655471,5.86540358676732));
#73963=CARTESIAN_POINT('Ctrl Pts',(0.351278969836519,2.40531168888727,5.8852739302901));
#73964=CARTESIAN_POINT('Ctrl Pts',(-0.066557880853422,2.56063238109896,
5.9051442738129));
#73965=CARTESIAN_POINT('Ctrl Pts',(-0.423336936897625,2.29338557308844,
5.92501461733567));
#73966=CARTESIAN_POINT('Ctrl Pts',(-0.391761985458073,1.84873382883771,
5.94488496085848));
#73967=CARTESIAN_POINT('Ctrl Pts',(-0.000798745939078063,1.63458458982805,
5.96475530438125));
#73968=CARTESIAN_POINT('Ctrl Pts',(0.390897234239583,1.84739062906445,5.98462564790406));
#73969=CARTESIAN_POINT('Ctrl Pts',(0.423998217856513,2.29193137647374,6.00449599142684));
#73970=CARTESIAN_POINT('Ctrl Pts',(0.068138558735181,2.56040121506583,6.02436633494963));
#73971=CARTESIAN_POINT('Ctrl Pts',(-0.350228951798542,2.40651561680067,
6.04423667847242));
#73972=CARTESIAN_POINT('Ctrl Pts',(-0.44730907842348,1.97144366845409,6.06410702199521));
#73973=CARTESIAN_POINT('Ctrl Pts',(-0.134044021227067,1.65430465293669,
6.083977365518));
#73974=CARTESIAN_POINT('Ctrl Pts',(0.302188176999508,1.74603044240738,6.10384770904079));
#73975=CARTESIAN_POINT('Ctrl Pts',(0.461203862034495,2.16247511236542,6.12371805256357));
#73976=CARTESIAN_POINT('Ctrl Pts',(0.197127790889,2.52160737194673,6.14358839608637));
#73977=CARTESIAN_POINT('Ctrl Pts',(-0.24778619187174,2.49397226442772,6.16345873960915));
#73978=CARTESIAN_POINT('Ctrl Pts',(-0.465390076634112,2.10492123877693,
6.18332908313195));
#73979=CARTESIAN_POINT('Ctrl Pts',(-0.256061923222516,1.71135564651446,
6.20319942665474));
#73980=CARTESIAN_POINT('Ctrl Pts',(0.188168185062698,1.67431833942391,6.22306977017752));
#73981=CARTESIAN_POINT('Ctrl Pts',(0.459779600338103,2.0277860045868,6.24294011370032));
#73982=CARTESIAN_POINT('Ctrl Pts',(0.309605825643754,2.44750017949355,6.2628104572231));
#73983=CARTESIAN_POINT('Ctrl Pts',(-0.124589145051608,2.54843024759255,
6.2826808007459));
#73984=CARTESIAN_POINT('Ctrl Pts',(-0.444490536442624,2.23798661179097,
6.30255114426868));
#73985=CARTESIAN_POINT('Ctrl Pts',(-0.356632372569888,1.80095904485208,
6.32242148779147));
#73986=CARTESIAN_POINT('Ctrl Pts',(0.0583874420223328,1.63826084351152,
6.34229183131426));
#73987=CARTESIAN_POINT('Ctrl Pts',(0.419844727291524,1.89914545813921,6.36216217483705));
#73988=CARTESIAN_POINT('Ctrl Pts',(0.396151631969156,2.34428677104743,6.38203251835984));
#73989=CARTESIAN_POINT('Ctrl Pts',(0.00904334548983111,2.56532822816046,
6.40190286188263));
#73990=CARTESIAN_POINT('Ctrl Pts',(-0.386360979336095,2.35949438465419,
6.42177320540542));
#73991=CARTESIAN_POINT('Ctrl Pts',(-0.427331703918903,1.91560977019817,
6.44164354892821));
#73992=CARTESIAN_POINT('Ctrl Pts',(-0.0762837661143578,1.64087808912227,
6.46151389245099));
#73993=CARTESIAN_POINT('Ctrl Pts',(0.344744142003126,1.78732825747258,6.48138423597379));
#73994=CARTESIAN_POINT('Ctrl Pts',(0.449516232509681,2.22061218317777,6.50125457949658));
#73995=CARTESIAN_POINT('Ctrl Pts',(0.141918375797697,2.54325085068338,6.52112492301936));
#73996=CARTESIAN_POINT('Ctrl Pts',(-0.295870270266432,2.45926720584139,
6.54099526654216));
#73997=CARTESIAN_POINT('Ctrl Pts',(-0.46223822246123,2.04570480945345,6.56086561006495));
#73998=CARTESIAN_POINT('Ctrl Pts',(-0.204565533599482,1.68195085876925,
6.58073595358773));
#73999=CARTESIAN_POINT('Ctrl Pts',(0.240768183257146,1.70170008291281,6.60060629711053));
#74000=CARTESIAN_POINT('Ctrl Pts',(0.465229869603695,2.08683525734651,6.62047664063331));
#74001=CARTESIAN_POINT('Ctrl Pts',(0.262906485916467,2.4840472909469,6.6403469841561));
#74002=CARTESIAN_POINT('Ctrl Pts',(-0.180597807113009,2.52894821842103,
6.66021732767889));
#74003=CARTESIAN_POINT('Ctrl Pts',(-0.458428198287625,2.18034755152067,
6.68008767120168));
#74004=CARTESIAN_POINT('Ctrl Pts',(-0.315713126897015,1.75803894443152,
6.69995801472447));
#74005=CARTESIAN_POINT('Ctrl Pts',(0.116625757960482,1.6494330520325,6.71982835824726));
#74006=CARTESIAN_POINT('Ctrl Pts',(0.441976387052489,1.95416099524259,6.73969870177005));
#74007=CARTESIAN_POINT('Ctrl Pts',(0.361873850675656,2.39267637112992,6.75956904529284));
#74008=CARTESIAN_POINT('Ctrl Pts',(-0.050198679019885,2.56270102079557,
6.77943938881563));
#74009=CARTESIAN_POINT('Ctrl Pts',(-0.416220754647733,2.30826047493722,
6.79930973233842));
#74010=CARTESIAN_POINT('Ctrl Pts',(-0.40041695122537,1.86276929542746,6.8191800758612));
#74011=CARTESIAN_POINT('Ctrl Pts',(-0.017285106899255,1.63490499131889,
6.839050419384));
#74012=CARTESIAN_POINT('Ctrl Pts',(0.381703469852107,1.83370204070729,6.85892076290678));
#74013=CARTESIAN_POINT('Ctrl Pts',(0.430531077249251,2.27679121455323,6.87879110642958));
#74014=CARTESIAN_POINT('Ctrl Pts',(0.0844050327837897,2.55769851699713,
6.89866144995237));
#74015=CARTESIAN_POINT('Ctrl Pts',(-0.339151138553184,2.4187297401227,6.91853179347515));
#74016=CARTESIAN_POINT('Ctrl Pts',(-0.451582311525894,1.98736981782162,
6.93840213699795));
#74017=CARTESIAN_POINT('Ctrl Pts',(-0.149748191053947,1.65933275445448,
6.95827248052074));
#74018=CARTESIAN_POINT('Ctrl Pts',(0.28945950833466,1.73554789744705,6.97814282404352));
#74019=CARTESIAN_POINT('Ctrl Pts',(0.463127515179909,2.14609822885846,6.99801316756631));
#74020=CARTESIAN_POINT('Ctrl Pts',(0.211939075965495,2.51435971099939,7.0178835110891));
#74021=CARTESIAN_POINT('Ctrl Pts',(-0.233674612547471,2.50250256827925,
7.0377538546119));
#74022=CARTESIAN_POINT('Ctrl Pts',(-0.46492365597403,2.12140411493955,7.05762419813467));
#74023=CARTESIAN_POINT('Ctrl Pts',(-0.269668538684808,1.72067030004994,
7.07749454165748));
#74024=CARTESIAN_POINT('Ctrl Pts',(0.172970750791257,1.66791984378901,7.09736488518025));
#74025=CARTESIAN_POINT('Ctrl Pts',(0.45693292425771,2.01154410845002,7.11723522870305));
#74026=CARTESIAN_POINT('Ctrl Pts',(0.321721345518213,2.4363146114259,7.13710557222584));
#74027=CARTESIAN_POINT('Ctrl Pts',(-0.108625769328017,2.5525622435185,7.15697591574863));
#74028=CARTESIAN_POINT('Ctrl Pts',(-0.439323528878937,2.25364562796892,
7.17684625927142));
#74029=CARTESIAN_POINT('Ctrl Pts',(-0.367001759181217,1.81378006572131,
7.19671660279421));
#74030=CARTESIAN_POINT('Ctrl Pts',(0.0419941617873573,1.63648232784889,
7.21658694631699));
#74031=CARTESIAN_POINT('Ctrl Pts',(0.412466156304921,1.88439895194213,7.2364572898398));
#74032=CARTESIAN_POINT('Ctrl Pts',(0.404556604609395,2.33010018619619,7.25632763336257));
#74033=CARTESIAN_POINT('Ctrl Pts',(0.0255214435931988,2.56471582492693,
7.27619797688537));
#74034=CARTESIAN_POINT('Ctrl Pts',(-0.376926167488953,2.37301795963397,
7.29606832040816));
#74035=CARTESIAN_POINT('Ctrl Pts',(-0.433595333764087,1.93086328441579,
7.31593866393094));
#74036=CARTESIAN_POINT('Ctrl Pts',(-0.0924998099851176,1.64386851986152,
7.33580900745374));
#74037=CARTESIAN_POINT('Ctrl Pts',(0.333451696743183,1.77531229164058,7.35567935097652));
#74038=CARTESIAN_POINT('Ctrl Pts',(0.453506667058955,2.20461283359934,7.37554969449932));
#74039=CARTESIAN_POINT('Ctrl Pts',(0.157531009705832,2.53794534248199,7.3954200380221));
#74040=CARTESIAN_POINT('Ctrl Pts',(-0.282957903141967,2.46952262051206,
7.41529038154489));
#74041=CARTESIAN_POINT('Ctrl Pts',(-0.463871461097088,2.06211320018452,
7.43516072506768));
#74042=CARTESIAN_POINT('Ctrl Pts',(-0.219246103892619,1.68945976086563,
7.45503106859047));
#74043=CARTESIAN_POINT('Ctrl Pts',(0.226507705971502,1.69342110094579,7.47490141211325));
#74044=CARTESIAN_POINT('Ctrl Pts',(0.464471531846451,2.07036323018922,7.49477175563605));
#74045=CARTESIAN_POINT('Ctrl Pts',(0.276345959341524,2.47449306105215,7.51464209915884));
#74046=CARTESIAN_POINT('Ctrl Pts',(-0.165289409754046,2.53507649102631,
7.53451244268163));
#74047=CARTESIAN_POINT('Ctrl Pts',(-0.455294247521488,2.19653647079961,
7.55438278620442));
#74048=CARTESIAN_POINT('Ctrl Pts',(-0.327628595902773,1.76943738086804,
7.5742531297272));
#74049=CARTESIAN_POINT('Ctrl Pts',(0.10059168985099,1.64558449195309,7.59412347325));
#74050=CARTESIAN_POINT('Ctrl Pts',(0.436532794488454,1.93859596858596,7.61399381677278));
#74051=CARTESIAN_POINT('Ctrl Pts',(0.372014488756375,2.37967367086649,7.63386416029558));
#74052=CARTESIAN_POINT('Ctrl Pts',(-0.0337764652102615,2.56418885425923,
7.65373450381837));
#74053=CARTESIAN_POINT('Ctrl Pts',(-0.408582110597001,2.32287395747531,
7.67360484734115));
#74054=CARTESIAN_POINT('Ctrl Pts',(-0.408569292942596,1.87710254625726,
7.69347519086395));
#74055=CARTESIAN_POINT('Ctrl Pts',(-0.0337497706999876,1.63580920409997,
7.71334553438673));
#74056=CARTESIAN_POINT('Ctrl Pts',(0.372030571543465,1.82034772331045,7.73321587790953));
#74057=CARTESIAN_POINT('Ctrl Pts',(0.436523511784681,2.26142913516393,7.75308622143231));
#74058=CARTESIAN_POINT('Ctrl Pts',(0.100565557273339,2.55442129209678,7.77295656495511));
#74059=CARTESIAN_POINT('Ctrl Pts',(-0.327647605271937,2.43054377740349,
7.79282690847788));
#74060=CARTESIAN_POINT('Ctrl Pts',(-0.455288695173849,2.00343734641438,
7.81269725200069));
#74061=CARTESIAN_POINT('Ctrl Pts',(-0.165264389212678,1.66491400427184,
7.83256759552346));
#74062=CARTESIAN_POINT('Ctrl Pts',(0.276367495136158,1.72552283160015,7.85243793904627));
#74063=CARTESIAN_POINT('Ctrl Pts',(0.464469826734602,2.12966348047235,7.87230828256904));
#74064=CARTESIAN_POINT('Ctrl Pts',(0.226484324161168,2.50659192432938,7.89217862609184));
#74065=CARTESIAN_POINT('Ctrl Pts',(-0.219269712773607,2.51052763010641,
7.91204896961463));
#74066=CARTESIAN_POINT('Ctrl Pts',(-0.463873639114477,2.13786012355098,
7.93191931313741));
#74067=CARTESIAN_POINT('Ctrl Pts',(-0.282936652261319,1.73046110782793,
7.95178965666021));
#74068=CARTESIAN_POINT('Ctrl Pts',(0.157556194694575,1.66206371749538,7.97166000018299));
#74069=CARTESIAN_POINT('Ctrl Pts',(0.453512682357245,1.99541324671956,7.9915303437058));
#74070=CARTESIAN_POINT('Ctrl Pts',(0.333433024133746,2.4247068838778,8.01140068722857));
#74071=CARTESIAN_POINT('Ctrl Pts',(-0.0925260409251638,2.55612615992871,
8.03127103075137));
#74072=CARTESIAN_POINT('Ctrl Pts',(-0.433605059718277,2.2691117802145,8.05114137427415));
#74073=CARTESIAN_POINT('Ctrl Pts',(-0.376910466218381,1.82696036464343,
8.07101171779694));
#74074=CARTESIAN_POINT('Ctrl Pts',(0.0255481683103127,1.63528564352218,
8.09088206131974));
#74075=CARTESIAN_POINT('Ctrl Pts',(0.404569836483345,1.8699230793225,8.11075240484252));
#74076=CARTESIAN_POINT('Ctrl Pts',(0.41245375689271,2.31562476770003,8.13062274836531));
#74077=CARTESIAN_POINT('Ctrl Pts',(0.0419675058616662,2.56352008637421,
8.1504930918881));
#74078=CARTESIAN_POINT('Ctrl Pts',(-0.367018218437449,2.3861988283617,8.17036343541089));
#74079=CARTESIAN_POINT('Ctrl Pts',(-0.439314692338837,1.94632910777952,
8.19023377893367));
#74080=CARTESIAN_POINT('Ctrl Pts',(-0.108599743314144,1.64743151040677,
8.21010412245648));
#74081=CARTESIAN_POINT('Ctrl Pts',(0.321740685681253,1.76370389059942,8.22997446597924));
#74082=CARTESIAN_POINT('Ctrl Pts',(0.456927836603256,2.18848216858596,8.24984480950206));
#74083=CARTESIAN_POINT('Ctrl Pts',(0.172945902549646,2.5320901026544,8.26971515302483));
#74084=CARTESIAN_POINT('Ctrl Pts',(-0.269690352634677,2.47931419129317,
8.28958549654763));
#74085=CARTESIAN_POINT('Ctrl Pts',(-0.464922424302857,2.07856914838463,
8.30945584007041));
#74086=CARTESIAN_POINT('Ctrl Pts',(-0.233651465145874,1.6974839942862,8.32932618359321));
#74087=CARTESIAN_POINT('Ctrl Pts',(0.211962904507778,1.6856524778242,8.349196527116));
#74088=CARTESIAN_POINT('Ctrl Pts',(0.463130165419301,2.05392840463697,8.36906687063877));
#74089=CARTESIAN_POINT('Ctrl Pts',(0.289438549037316,2.46446874811399,8.38893721416159));
#74090=CARTESIAN_POINT('Ctrl Pts',(-0.149773532586065,2.54065863313601,
8.40880755768436));
#74091=CARTESIAN_POINT('Ctrl Pts',(-0.451588787887004,2.21260421251156,
8.42867790120716));
#74092=CARTESIAN_POINT('Ctrl Pts',(-0.339132808563647,1.78125075658703,
8.44854824472993));
#74093=CARTESIAN_POINT('Ctrl Pts',(0.0844313538539795,1.64230633770284,
8.46841858825274));
#74094=CARTESIAN_POINT('Ctrl Pts',(0.430541243401479,1.92323354461066,8.48828893177552));
#74095=CARTESIAN_POINT('Ctrl Pts',(0.38168815502571,2.36631990975832,8.50815927529831));
#74096=CARTESIAN_POINT('Ctrl Pts',(-0.0173118534359932,2.56509401388452,
8.52802961882109));
#74097=CARTESIAN_POINT('Ctrl Pts',(-0.400430593166196,2.3372076771042,8.5478999623439));
#74098=CARTESIAN_POINT('Ctrl Pts',(-0.416208777369125,1.89171558948999,
8.56777030586666));
#74099=CARTESIAN_POINT('Ctrl Pts',(-0.0501720700444095,1.63729609315669,
8.58764064938948));
#74100=CARTESIAN_POINT('Ctrl Pts',(0.361890681235488,1.8073444399033,8.60751099291225));
#74101=CARTESIAN_POINT('Ctrl Pts',(0.441967999449303,2.24586442158177,8.62738133643504));
#74102=CARTESIAN_POINT('Ctrl Pts',(0.116599846678335,2.55057365410685,8.64725167995784));
#74103=CARTESIAN_POINT('Ctrl Pts',(-0.315732791784264,2.44194289905293,
8.66712202348063));
#74104=CARTESIAN_POINT('Ctrl Pts',(-0.458423576923048,2.01962608544011,
8.68699236700342));
#74105=CARTESIAN_POINT('Ctrl Pts',(-0.180573138969472,1.67104139651556,
8.7068627105262));
#74106=CARTESIAN_POINT('Ctrl Pts',(0.262928571175537,1.71596782884738,8.726733054049));
#74107=CARTESIAN_POINT('Ctrl Pts',(0.465229111759736,2.11319149695258,8.74660339757178));
#74108=CARTESIAN_POINT('Ctrl Pts',(0.240745277528821,2.49831376246394,8.76647374109457));
#74109=CARTESIAN_POINT('Ctrl Pts',(-0.20458957432477,2.51803737643686,8.78634408461736));
#74110=CARTESIAN_POINT('Ctrl Pts',(-0.462241344090878,2.15426860817877,
8.80621442814016));
#74111=CARTESIAN_POINT('Ctrl Pts',(-0.29584960913021,1.74071577992054,8.82608477166294));
#74112=CARTESIAN_POINT('Ctrl Pts',(0.141943865920065,1.65675731145537,8.84595511518573));
#74113=CARTESIAN_POINT('Ctrl Pts',(0.449523167901091,1.9794136676867,8.86582545870853));
#74114=CARTESIAN_POINT('Ctrl Pts',(0.34472616038612,2.41269156746872,8.8856958022313));
#74115=CARTESIAN_POINT('Ctrl Pts',(-0.076310169054144,2.55911752321113,
8.9055661457541));
#74116=CARTESIAN_POINT('Ctrl Pts',(-0.427342307078658,2.28436565461413,
8.92543648927688));
#74117=CARTESIAN_POINT('Ctrl Pts',(-0.386346055760231,1.84048339702609,
8.94530683279968));
#74118=CARTESIAN_POINT('Ctrl Pts',(0.00907010545211835,1.6346722926714,
8.96517717632246));
#74119=CARTESIAN_POINT('Ctrl Pts',(0.396165679695509,1.85573601114368,8.98504751984527));
#74120=CARTESIAN_POINT('Ctrl Pts',(0.41983317590544,2.30087868585233,9.00491786336803));
#74121=CARTESIAN_POINT('Ctrl Pts',(0.0583608883479577,2.56174251345511,
9.02478820689085));
#74122=CARTESIAN_POINT('Ctrl Pts',(-0.356649569151262,2.39902044552977,
9.04465855041361));
#74123=CARTESIAN_POINT('Ctrl Pts',(-0.444482600408699,1.96198782678863,
9.06452889393643));
#74124=CARTESIAN_POINT('Ctrl Pts',(-0.124563356633115,1.65156258830814,
9.08439923745919));
#74125=CARTESIAN_POINT('Ctrl Pts',(0.309625809083618,1.75251762581403,9.10426958098201));
#74126=CARTESIAN_POINT('Ctrl Pts',(0.459775446713771,2.17224043618195,9.12413992450477));
#74127=CARTESIAN_POINT('Ctrl Pts',(0.18814370475902,2.52569248100026,9.14401026802759));
#74128=CARTESIAN_POINT('Ctrl Pts',(-0.256084272859606,2.48862962729902,
9.16388061155035));
#74129=CARTESIAN_POINT('Ctrl Pts',(-0.465389792855207,2.0950519976972,9.18375095507316));
#74130=CARTESIAN_POINT('Ctrl Pts',(-0.247763535005359,1.70601348659852,
9.20362129859593));
#74131=CARTESIAN_POINT('Ctrl Pts',(0.197152036252414,1.67840396512523,9.22349164211874));
#74132=CARTESIAN_POINT('Ctrl Pts',(0.461207454074709,2.03755141053213,9.24336198564151));
#74133=CARTESIAN_POINT('Ctrl Pts',(0.302167820508651,2.45398693516803,9.26323232916431));
#74134=CARTESIAN_POINT('Ctrl Pts',(-0.134069651939929,2.54568763775688,
9.28310267268709));
#74135=CARTESIAN_POINT('Ctrl Pts',(-0.447316470668593,2.22853060759678,
9.30297301620988));
#74136=CARTESIAN_POINT('Ctrl Pts',(-0.350211324197387,1.79346424282881,
9.32284335973268));
#74137=CARTESIAN_POINT('Ctrl Pts',(0.0681650352583336,1.63960270419035,
9.34271370325547));
#74138=CARTESIAN_POINT('Ctrl Pts',(0.424009254696116,1.90809300702516,9.36258404677826));
#74139=CARTESIAN_POINT('Ctrl Pts',(0.390882706597841,2.35263185013642,9.38245439030104));
#74140=CARTESIAN_POINT('Ctrl Pts',(-0.00082551092863093,2.56541536346828,
9.40232473382384));
#74141=CARTESIAN_POINT('Ctrl Pts',(-0.391776434561243,2.35124364139831,
9.42219507734661));
#74142=CARTESIAN_POINT('Ctrl Pts',(-0.423325815029323,1.90659008207859,
9.44206542086942));
#74143=CARTESIAN_POINT('Ctrl Pts',(-0.0665313908137084,1.63936379206905,
9.4619357643922));
#74144=CARTESIAN_POINT('Ctrl Pts',(0.351296527042499,1.79470851287912,9.481806107915));
#74145=CARTESIAN_POINT('Ctrl Pts',(0.446857706040839,2.2301166114396,9.50167645143777));
#74146=CARTESIAN_POINT('Ctrl Pts',(0.132487773930098,2.54616043278137,9.52154679496058));
#74147=CARTESIAN_POINT('Ctrl Pts',(-0.303421654179774,2.45291279630443,
9.54141713848336));
#74148=CARTESIAN_POINT('Ctrl Pts',(-0.46098302170792,2.035915713957,9.56128748200614));
#74149=CARTESIAN_POINT('Ctrl Pts',(-0.195655223990523,1.67770723976627,
9.58115782552895));
#74150=CARTESIAN_POINT('Ctrl Pts',(0.249159605684645,1.706894883122,9.60102816905172));
#74151=CARTESIAN_POINT('Ctrl Pts',(0.465404417161516,2.09670295478412,9.62089851257453));
#74152=CARTESIAN_POINT('Ctrl Pts',(0.254704034982808,2.48953561657965,9.6407688560973));
#74153=CARTESIAN_POINT('Ctrl Pts',(-0.189652624469372,2.52502238064893,
9.6606391996201));
#74154=CARTESIAN_POINT('Ctrl Pts',(-0.460028819844302,2.1706089720451,9.68050954314289));
#74155=CARTESIAN_POINT('Ctrl Pts',(-0.308391200280706,1.75142144413341,
9.70037988666567));
#74156=CARTESIAN_POINT('Ctrl Pts',(0.126153361869621,1.65200728654409,9.72025023018848));
#74157=CARTESIAN_POINT('Ctrl Pts',(0.444969388733965,1.96356545484986,9.74012057371125));
#74158=CARTESIAN_POINT('Ctrl Pts',(0.355586578547096,2.40028374444477,9.75999091723406));
#74159=CARTESIAN_POINT('Ctrl Pts',(-0.0599985087153332,2.56153257845199,
9.77986126075682));
#74160=CARTESIAN_POINT('Ctrl Pts',(-0.420543132290841,2.29938810371638,
9.79973160427964));
#74161=CARTESIAN_POINT('Ctrl Pts',(-0.395296683767164,1.85433218806021,
9.8196019478024));
#74162=CARTESIAN_POINT('Ctrl Pts',(-0.00741934267117735,1.63464304520623,
9.83947229132522));
#74163=CARTESIAN_POINT('Ctrl Pts',(0.387264235273323,1.84185555574684,9.85934263484798));
#74164=CARTESIAN_POINT('Ctrl Pts',(0.426685598619483,2.28588045069704,9.87921297837078));
#74165=CARTESIAN_POINT('Ctrl Pts',(0.0746810132312207,2.55938533747102,
9.89908332189357));
#74166=CARTESIAN_POINT('Ctrl Pts',(-0.345833234894805,2.41146671678174,
9.91895366541636));
#74167=CARTESIAN_POINT('Ctrl Pts',(-0.449092570948396,1.9778197858098,9.93882400893915));
#74168=CARTESIAN_POINT('Ctrl Pts',(-0.140370611589618,1.65625656802318,
9.95869435246194));
#74169=CARTESIAN_POINT('Ctrl Pts',(0.297122274169468,1.74176753886202,9.97856469598473));
#74170=CARTESIAN_POINT('Ctrl Pts',(0.462045922923124,2.15590802384918,9.99843503950751));
#74171=CARTESIAN_POINT('Ctrl Pts',(0.203105339267231,2.51876050814486,10.0183053830303));
#74172=CARTESIAN_POINT('Ctrl Pts',(-0.242156742871212,2.49745723531295,
10.0381757265531));
#74173=CARTESIAN_POINT('Ctrl Pts',(-0.465272980088995,2.11154105799798,
10.0580460700759));
#74174=CARTESIAN_POINT('Ctrl Pts',(-0.261564599271689,1.71503753114305,
10.0779164135986));
#74175=CARTESIAN_POINT('Ctrl Pts',(0.182093692572646,1.67168466155662,10.0977867571214));
#74176=CARTESIAN_POINT('Ctrl Pts',(0.458705811299323,2.02125280512402,10.1176571006442));
#74177=CARTESIAN_POINT('Ctrl Pts',(0.314517795316142,2.44306077952759,10.137527444167));
#74178=CARTESIAN_POINT('Ctrl Pts',(-0.118197480138174,2.55015719222244,
10.1573977876898));
#74179=CARTESIAN_POINT('Ctrl Pts',(-0.442482658699621,2.24429566442108,
10.1772681312126));
#74180=CARTESIAN_POINT('Ctrl Pts',(-0.360850236478646,1.80606250859424,
10.1971384747354));
#74181=CARTESIAN_POINT('Ctrl Pts',(0.0518131523877713,1.63747698515616,
10.2170088182582));
#74182=CARTESIAN_POINT('Ctrl Pts',(0.41694502766216,1.89319336101468,10.236879161781));
#74183=CARTESIAN_POINT('Ctrl Pts',(0.39958660199647,2.33862667396065,10.2567495053038));
#74184=CARTESIAN_POINT('Ctrl Pts',(0.0156618678027072,2.56515249963591,
10.2766198488265));
#74185=CARTESIAN_POINT('Ctrl Pts',(-0.382630497929272,2.36496423168987,
10.2964901923493));
#74186=CARTESIAN_POINT('Ctrl Pts',(-0.429911472249707,1.92170735279128,
10.3163605358721));
#74187=CARTESIAN_POINT('Ctrl Pts',(-0.0828071979430214,1.64200970535455,
10.3362308793949));
#74188=CARTESIAN_POINT('Ctrl Pts',(0.340261407294346,1.78245580350654,10.3561012229177));
#74189=CARTESIAN_POINT('Ctrl Pts',(0.451186493746875,2.21420547220255,10.3759715664405));
#74190=CARTESIAN_POINT('Ctrl Pts',(0.148209395681264,2.54118716782383,10.3958419099633));
#74191=CARTESIAN_POINT('Ctrl Pts',(-0.290729646034643,2.46343969917604,
10.4157122534861));
#74192=CARTESIAN_POINT('Ctrl Pts',(-0.462963816781086,2.05228578438148,
10.4355825970089));
#74193=CARTESIAN_POINT('Ctrl Pts',(-0.210491712463267,1.68490316671301,
10.4554529405316));
#74194=CARTESIAN_POINT('Ctrl Pts',(0.235077882180559,1.69831538325434,10.4753232840544));
#74195=CARTESIAN_POINT('Ctrl Pts',(0.464995522887528,2.0802185512372,10.4951936275772));
#74196=CARTESIAN_POINT('Ctrl Pts',(0.268343074769386,2.48026850545887,10.5150639711));
#74197=CARTESIAN_POINT('Ctrl Pts',(-0.174477612838825,2.53147387480434,
10.5349343146228));
#74198=CARTESIAN_POINT('Ctrl Pts',(-0.457238843649517,2.18686070388073,
10.5548046581456));
#74199=CARTESIAN_POINT('Ctrl Pts',(-0.320545682859447,1.76256466216359,
10.5746750016684));
#74200=CARTESIAN_POINT('Ctrl Pts',(0.110204503599964,1.64781960523825,10.5945453451912));
#74201=CARTESIAN_POINT('Ctrl Pts',(0.439857060994807,1.94788850170479,10.614415688714));
#74202=CARTESIAN_POINT('Ctrl Pts',(0.366000646058553,2.38749898974663,10.6342860322368));
#74203=CARTESIAN_POINT('Ctrl Pts',(-0.0436115351477654,2.56336829414912,
10.6541563757595));
#74204=CARTESIAN_POINT('Ctrl Pts',(-0.413216070030391,2.31416027056679,
10.6740267192823));
#74205=CARTESIAN_POINT('Ctrl Pts',(-0.40375111494835,1.86848935402757,10.6938970628051));
#74206=CARTESIAN_POINT('Ctrl Pts',(-0.0238994776521259,1.63519793783959,
10.7137674063279));
#74207=CARTESIAN_POINT('Ctrl Pts',(0.377876676769845,1.82829913659691,10.7336377498507));
#74208=CARTESIAN_POINT('Ctrl Pts',(0.433002423519727,2.27064888879407,10.7535080933735));
#74209=CARTESIAN_POINT('Ctrl Pts',(0.0909073946472628,2.55645151727105,
10.7733784368963));
#74210=CARTESIAN_POINT('Ctrl Pts',(-0.334582792889821,2.42352201891472,
10.7932487804191));
#74211=CARTESIAN_POINT('Ctrl Pts',(-0.453138817284674,1.9938051117499,10.8131191239419));
#74212=CARTESIAN_POINT('Ctrl Pts',(-0.156001666100313,1.66150755742598,
10.8329894674646));
#74213=CARTESIAN_POINT('Ctrl Pts',(0.284245776021994,1.73146712380812,10.8528598109874));
#74214=CARTESIAN_POINT('Ctrl Pts',(0.463736415212255,2.13950543287564,10.8727301545102));
#74215=CARTESIAN_POINT('Ctrl Pts',(0.217812025457425,2.5113028854588,10.892600498033));
#74216=CARTESIAN_POINT('Ctrl Pts',(-0.227925245224916,2.50578593446517,
10.9124708415558));
#74217=CARTESIAN_POINT('Ctrl Pts',(-0.464572132633622,2.12801563136634,
10.9323411850786));
#74218=CARTESIAN_POINT('Ctrl Pts',(-0.275037334135784,1.7245448004727,10.9522115286014));
#74219=CARTESIAN_POINT('Ctrl Pts',(0.166806775479661,1.66550300153548,10.9720818721242));
#74220=CARTESIAN_POINT('Ctrl Pts',(0.455628377284424,2.00505304726444,10.9919522156469));
#74221=CARTESIAN_POINT('Ctrl Pts',(0.326472971133189,2.43170399626786,11.0118225591698));
#74222=CARTESIAN_POINT('Ctrl Pts',(-0.1021769407511,2.55406168611693,11.0316929026925));
#74223=CARTESIAN_POINT('Ctrl Pts',(-0.437093419630667,2.25987959387044,
11.0515632462153));
#74224=CARTESIAN_POINT('Ctrl Pts',(-0.371036190894924,1.81902973988909,
11.0714335897381));
#74225=CARTESIAN_POINT('Ctrl Pts',(0.0353962309707253,1.6359318489126,11.0913039332609));
#74226=CARTESIAN_POINT('Ctrl Pts',(0.409357429682445,1.87855330938489,11.1111742767837));
#74227=CARTESIAN_POINT('Ctrl Pts',(0.40778891564229,2.32432196125189,11.1310446203065));
#74228=CARTESIAN_POINT('Ctrl Pts',(0.0321295869481889,2.56430575234768,
11.1509149638293));
#74229=CARTESIAN_POINT('Ctrl Pts',(-0.373004263722582,2.37835222518488,
11.1707853073521));
#74230=CARTESIAN_POINT('Ctrl Pts',(-0.435957482373001,1.9370484256486,11.1906556508749));
#74231=CARTESIAN_POINT('Ctrl Pts',(-0.0989790611981271,1.64523051172605,
11.2105259943976));
#74232=CARTESIAN_POINT('Ctrl Pts',(0.328799173843605,1.77060169201958,11.2303963379204));
#74233=CARTESIAN_POINT('Ctrl Pts',(0.45494892884938,2.19815097635484,11.2502666814432));
#74234=CARTESIAN_POINT('Ctrl Pts',(0.163744977339756,2.53566010193339,11.270137024966));
#74235=CARTESIAN_POINT('Ctrl Pts',(-0.277672699013363,2.4735103937553,11.2900073684888));
#74236=CARTESIAN_POINT('Ctrl Pts',(-0.464363475746229,2.06871574815522,
11.3098777120116));
#74237=CARTESIAN_POINT('Ctrl Pts',(-0.225063980860663,1.69262014465643,
11.3297480555344));
#74238=CARTESIAN_POINT('Ctrl Pts',(0.220701076770306,1.69024009867603,11.3496183990572));
#74239=CARTESIAN_POINT('Ctrl Pts',(0.464002942203016,2.06375897838704,11.36948874258));
#74240=CARTESIAN_POINT('Ctrl Pts',(0.281645276460985,2.47052406165838,11.3893590861028));
#74241=CARTESIAN_POINT('Ctrl Pts',(-0.15908358789192,2.53738376065424,11.4092294296255));
#74242=CARTESIAN_POINT('Ctrl Pts',(-0.453874917628838,2.20300340367202,
11.4290997731483));
#74243=CARTESIAN_POINT('Ctrl Pts',(-0.332297799931782,1.77413144646791,
11.4489701166711));
#74244=CARTESIAN_POINT('Ctrl Pts',(0.0941173109422024,1.64419952413187,
11.4688404601939));
#74245=CARTESIAN_POINT('Ctrl Pts',(0.434192601941608,1.93240248677327,11.4887108037167));
#74246=CARTESIAN_POINT('Ctrl Pts',(0.375955290644748,2.37435335145907,11.5085811472395));
#74247=CARTESIAN_POINT('Ctrl Pts',(-0.0271698181275119,2.56462236601731,
11.5284514907623));
#74248=CARTESIAN_POINT('Ctrl Pts',(-0.40537031760452,2.32866361237813,11.548321834285));
#74249=CARTESIAN_POINT('Ctrl Pts',(-0.411698736864844,1.88293712412185,
11.5681921778079));
#74250=CARTESIAN_POINT('Ctrl Pts',(-0.0403496127736347,1.63633627404161,
11.5880625213306));
#74251=CARTESIAN_POINT('Ctrl Pts',(0.368014787933636,1.81508377041178,11.6079328648534));
#74252=CARTESIAN_POINT('Ctrl Pts',(0.43877572140111,2.255203119587,11.6278032083762));
#74253=CARTESIAN_POINT('Ctrl Pts',(0.10701966440361,2.55294473553796,11.647673551899));
#74254=CARTESIAN_POINT('Ctrl Pts',(-0.322912365272506,2.43517121949046,
11.6675438954218));
#74255=CARTESIAN_POINT('Ctrl Pts',(-0.456616260360021,2.00992373900169,
11.6874142389446));
#74256=CARTESIAN_POINT('Ctrl Pts',(-0.171436899257811,1.66730896520326,
11.7072845824674));
#74257=CARTESIAN_POINT('Ctrl Pts',(0.271012477887101,1.72162931026559,11.7271549259902));
#74258=CARTESIAN_POINT('Ctrl Pts',(0.464844801587871,2.12305325264119,11.747025269513));
#74259=CARTESIAN_POINT('Ctrl Pts',(0.232245302737102,2.50332897413545,11.7668956130357));
#74260=CARTESIAN_POINT('Ctrl Pts',(-0.213407644032012,2.51360527014209,
11.7867659565585));
#74261=CARTESIAN_POINT('Ctrl Pts',(-0.463288130229042,2.14445503806638,
11.8066363000813));
#74262=CARTESIAN_POINT('Ctrl Pts',(-0.28816482792459,1.73452336057171,11.8265066436041));
#74263=CARTESIAN_POINT('Ctrl Pts',(0.151310473901801,1.6598667446009,11.8463769871269));
#74264=CARTESIAN_POINT('Ctrl Pts',(0.451979014984232,1.98897247172665,11.8662473306497));
#74265=CARTESIAN_POINT('Ctrl Pts',(0.338018341205278,2.41993084101011,11.8861176741725));
#74266=CARTESIAN_POINT('Ctrl Pts',(-0.0860281435876672,2.55739621831784,
11.9059880176953));
#74267=CARTESIAN_POINT('Ctrl Pts',(-0.431155518313124,2.27526283419125,
11.9258583612181));
#74268=CARTESIAN_POINT('Ctrl Pts',(-0.380756401509851,1.83234965957452,
11.9457287047409));
#74269=CARTESIAN_POINT('Ctrl Pts',(0.0189348783753338,1.63496923499459,
11.9655990482636));
#74270=CARTESIAN_POINT('Ctrl Pts',(0.401255985102072,1.86419122908516,11.9854693917864));
#74271=CARTESIAN_POINT('Ctrl Pts',(0.415479351567335,2.30973566802477,12.0053397353092));
#74272=CARTESIAN_POINT('Ctrl Pts',(0.0485569753757318,2.56287618448453,
12.025210078832));
#74273=CARTESIAN_POINT('Ctrl Pts',(-0.362909815287825,2.39139081658207,
12.0450804223548));
#74274=CARTESIAN_POINT('Ctrl Pts',(-0.441456256134848,1.95259404374312,
12.0649507658776));
#74275=CARTESIAN_POINT('Ctrl Pts',(-0.115026680820544,1.649022168261,12.0848211094004));
#74276=CARTESIAN_POINT('Ctrl Pts',(0.31692421467806,1.75916105831155,12.1046914529232));
#74277=CARTESIAN_POINT('Ctrl Pts',(0.458140288545373,2.18197327632933,12.124561796446));
#74278=CARTESIAN_POINT('Ctrl Pts',(0.179075017840616,2.52958617296881,12.1444321399687));
#74279=CARTESIAN_POINT('Ctrl Pts',(-0.264267202870627,2.4831122387859,12.1643024834915));
#74280=CARTESIAN_POINT('Ctrl Pts',(-0.465180241679061,2.08518498153858,
12.1841728270143));
#74281=CARTESIAN_POINT('Ctrl Pts',(-0.239353737318343,1.70084848684698,
12.2040431705371));
#74282=CARTESIAN_POINT('Ctrl Pts',(0.206047235963034,1.68267916590158,12.2239135140599));
#74283=CARTESIAN_POINT('Ctrl Pts',(0.462427921046529,2.0473448971401,12.2437838575827));
#74284=CARTESIAN_POINT('Ctrl Pts',(0.294593942446601,2.46031451690763,12.2636542011055));
#74285=CARTESIAN_POINT('Ctrl Pts',(-0.14348987300431,2.54274461980447,12.2835245446283));
#74286=CARTESIAN_POINT('Ctrl Pts',(-0.449941264356029,2.21901680826798,
12.3033948881511));
#74287=CARTESIAN_POINT('Ctrl Pts',(-0.34363279963305,1.78610727782098,12.3232652316739));
#74288=CARTESIAN_POINT('Ctrl Pts',(0.0779119773719135,1.64115158733782,
12.3431355751966));
#74289=CARTESIAN_POINT('Ctrl Pts',(0.427983121896085,1.91712684890152,12.3630059187194));
#74290=CARTESIAN_POINT('Ctrl Pts',(0.385438016721381,2.36086333066664,12.3828762622422));
#74291=CARTESIAN_POINT('Ctrl Pts',(-0.0106939961474559,2.56529321988075,
12.402746605765));
#74292=CARTESIAN_POINT('Ctrl Pts',(-0.397015723407115,2.34287992380626,
12.4226169492878));
#74293=CARTESIAN_POINT('Ctrl Pts',(-0.419129573250919,1.89765736275538,
12.4424872928106));
#74294=CARTESIAN_POINT('Ctrl Pts',(-0.0567490989759844,1.63805662491381,
12.4623576363334));
#74295=CARTESIAN_POINT('Ctrl Pts',(0.357690947917213,1.80222604580204,12.4822279798562));
#74296=CARTESIAN_POINT('Ctrl Pts',(0.443998245321784,2.23956253140361,12.502098323379));
#74297=CARTESIAN_POINT('Ctrl Pts',(0.122997597546583,2.54886939416535,12.5219686669018));
#74298=CARTESIAN_POINT('Ctrl Pts',(-0.310836601366722,2.4463996958304,12.5418390104245));
#74299=CARTESIAN_POINT('Ctrl Pts',(-0.45952053510819,2.0261554346313,12.5617093539473));
#74300=CARTESIAN_POINT('Ctrl Pts',(-0.18665693595978,1.6736535091282,12.5815796974701));
#74301=CARTESIAN_POINT('Ctrl Pts',(0.257438990884462,1.71226644716637,12.6014500409929));
#74302=CARTESIAN_POINT('Ctrl Pts',(0.46536969074615,2.10657213477266,12.6213203845157));
#74303=CARTESIAN_POINT('Ctrl Pts',(0.246387053710664,2.49484878344037,12.6411907280385));
#74304=CARTESIAN_POINT('Ctrl Pts',(-0.198622162535629,2.52090542710951,
12.6610610715613));
#74305=CARTESIAN_POINT('Ctrl Pts',(-0.461422584621671,2.16083864250527,
12.6809314150841));
#74306=CARTESIAN_POINT('Ctrl Pts',(-0.300930602329029,1.7449606858358,12.7008017586068));
#74307=CARTESIAN_POINT('Ctrl Pts',(0.13562423959672,1.65478296567376,12.7206721021296));
#74308=CARTESIAN_POINT('Ctrl Pts',(0.447762305268633,1.97303126368024,12.7405424456524));
#74309=CARTESIAN_POINT('Ctrl Pts',(0.349139413183901,2.4077560920269,12.7604127891752));
#74310=CARTESIAN_POINT('Ctrl Pts',(-0.0697713594461587,2.56015660314866,
12.780283132698));
#74311=CARTESIAN_POINT('Ctrl Pts',(-0.424676408320006,2.29042607554407,
12.8001534762208));
#74312=CARTESIAN_POINT('Ctrl Pts',(-0.389998666988802,1.84600554780131,
12.8200238197436));
#74313=CARTESIAN_POINT('Ctrl Pts',(0.00244975769600178,1.63459035172035,
12.8398941632664));
#74314=CARTESIAN_POINT('Ctrl Pts',(0.392650863361715,1.85012514814954,12.8597645067892));
#74315=CARTESIAN_POINT('Ctrl Pts',(0.422648256168044,2.29488610373169,12.879634850312));
#74316=CARTESIAN_POINT('Ctrl Pts',(0.0649234129076833,2.56086559054602,
12.8995051938347));
#74317=CARTESIAN_POINT('Ctrl Pts',(-0.352359824332398,2.40406363910594,
12.9193755373576));
#74318=CARTESIAN_POINT('Ctrl Pts',(-0.446400889969114,1.96832469353053,
12.9392458808803));
#74319=CARTESIAN_POINT('Ctrl Pts',(-0.130929915360603,1.65337991524715,
12.9591162244031));
#74320=CARTESIAN_POINT('Ctrl Pts',(0.304651440389382,1.74814826369811,12.9789865679259));
#74321=CARTESIAN_POINT('Ctrl Pts',(0.460756558152438,2.16569267836185,12.9988569114487));
#74322=CARTESIAN_POINT('Ctrl Pts',(0.19418029092386,2.52297300687519,13.0187272549715));
#74323=CARTESIAN_POINT('Ctrl Pts',(-0.25053001723091,2.49223317838584,13.0385975984943));
#74324=CARTESIAN_POINT('Ctrl Pts',(-0.465413027024947,2.10167281756508,
13.0584679420171));
#74325=CARTESIAN_POINT('Ctrl Pts',(-0.253343164592808,1.70957785296128,
13.0783382855398));
#74326=CARTESIAN_POINT('Ctrl Pts',(0.191134985117061,1.6756420983047,13.0982086290627));
#74327=CARTESIAN_POINT('Ctrl Pts',(0.460271991395613,2.03099686796687,13.1180789725854));
#74328=CARTESIAN_POINT('Ctrl Pts',(0.307173676042658,2.44965277020794,13.1379493161082));
#74329=CARTESIAN_POINT('Ctrl Pts',(-0.127717692980967,2.54754956230708,
13.157819659631));
#74330=CARTESIAN_POINT('Ctrl Pts',(-0.445439642377961,2.2348811263436,13.1776900031538));
#74331=CARTESIAN_POINT('Ctrl Pts',(-0.354542576399878,1.79847652742844,
13.1975603466766));
#74332=CARTESIAN_POINT('Ctrl Pts',(0.0616206363204805,1.63868076881278,
13.2174306901994));
#74333=CARTESIAN_POINT('Ctrl Pts',(0.421213705444151,1.9020785519879,13.2373010337222));
#74334=CARTESIAN_POINT('Ctrl Pts',(0.394480663010893,2.34705011774784,13.257171377245));
#74335=CARTESIAN_POINT('Ctrl Pts',(0.00571095611368224,2.56537182328736,
13.2770417207678));
#74336=CARTESIAN_POINT('Ctrl Pts',(-0.387999947893056,2.35680705697765,
13.2969120642905));
#74337=CARTESIAN_POINT('Ctrl Pts',(-0.426352479043764,1.912602081833,13.3167824078133));
#74338=CARTESIAN_POINT('Ctrl Pts',(-0.0724212997312765,1.64040692913555,
13.3366527513361));
#74339=CARTESIAN_POINT('Ctrl Pts',(0.206034670117974,1.73993310315546,13.349899647018));
#74340=CARTESIAN_POINT('Ctrl Pts',(0.293391644475074,1.83761221843237,13.3565230948589));
#74341=CARTESIAN_POINT('Ctrl Pts',(-0.347219699208383,1.97323498128075,
4.32934271053038));
#74342=CARTESIAN_POINT('Ctrl Pts',(-0.304993076091424,1.85755383756099,
4.33597059444799));
#74343=CARTESIAN_POINT('Ctrl Pts',(-0.0965749770348568,1.67383077332961,
4.34922192620653));
#74344=CARTESIAN_POINT('Ctrl Pts',(0.306876354697739,1.78837779405028,4.36909670580601));
#74345=CARTESIAN_POINT('Ctrl Pts',(0.427739319365321,2.18925964705946,4.38896704932879));
#74346=CARTESIAN_POINT('Ctrl Pts',(0.156695639423864,2.5080091347322,4.40883739285158));
#74347=CARTESIAN_POINT('Ctrl Pts',(-0.258344791487002,2.45259440315036,
4.42870773637437));
#74348=CARTESIAN_POINT('Ctrl Pts',(-0.436259586392415,2.07365558490192,
4.44857807989716));
#74349=CARTESIAN_POINT('Ctrl Pts',(-0.214032795552298,1.71891882025207,
4.46844842341995));
#74350=CARTESIAN_POINT('Ctrl Pts',(0.204574834047816,1.71375417298191,4.48831876694274));
#74351=CARTESIAN_POINT('Ctrl Pts',(0.435494789331625,2.06292682817853,4.50818911046552));
#74352=CARTESIAN_POINT('Ctrl Pts',(0.266916968435977,2.44610422235877,4.52805945398832));
#74353=CARTESIAN_POINT('Ctrl Pts',(-0.146525717420236,2.51178062822751,
4.54792979751111));
#74354=CARTESIAN_POINT('Ctrl Pts',(-0.425548469292051,2.19970305918092,
4.56780014103389));
#74355=CARTESIAN_POINT('Ctrl Pts',(-0.314189750545297,1.7961621855343,4.58767048455669));
#74356=CARTESIAN_POINT('Ctrl Pts',(0.0853959749762369,1.67135079038661,
4.60754082807948));
#74357=CARTESIAN_POINT('Ctrl Pts',(0.406642164051052,1.93976687276704,4.62741117160227));
#74358=CARTESIAN_POINT('Ctrl Pts',(0.354849711281776,2.3551749405769,4.64728151512505));
#74359=CARTESIAN_POINT('Ctrl Pts',(-0.0224691388804926,2.53649478868572,
4.66715185864785));
#74360=CARTESIAN_POINT('Ctrl Pts',(-0.379175563316004,2.31739006595186,
4.68702220217063));
#74361=CARTESIAN_POINT('Ctrl Pts',(-0.388040054307679,1.89885956599689,
4.70689254569342));
#74362=CARTESIAN_POINT('Ctrl Pts',(-0.0409306089551436,1.66484802453397,
4.72676288921621));
#74363=CARTESIAN_POINT('Ctrl Pts',(0.343727090956584,1.83002918355619,4.746633232739));
#74364=CARTESIAN_POINT('Ctrl Pts',(0.413061982746445,2.24287181159513,4.76650357626179));
#74365=CARTESIAN_POINT('Ctrl Pts',(0.103468736801614,2.5246490037035,4.78637391978458));
#74366=CARTESIAN_POINT('Ctrl Pts',(-0.301042988188063,2.4168685451533,4.80624426330737));
#74367=CARTESIAN_POINT('Ctrl Pts',(-0.429388755323053,2.01840433444282,
4.82611460683016));
#74368=CARTESIAN_POINT('Ctrl Pts',(-0.163828795187018,1.69479303849886,
4.84598495035295));
#74369=CARTESIAN_POINT('Ctrl Pts',(0.252021781120245,1.74290396585595,4.86585529387574));
#74370=CARTESIAN_POINT('Ctrl Pts',(0.436676682987851,2.11860189026849,4.88572563739853));
#74371=CARTESIAN_POINT('Ctrl Pts',(0.220740176339599,2.47723511279732,4.90559598092132));
#74372=CARTESIAN_POINT('Ctrl Pts',(-0.197695391019725,2.48980647524797,
4.9254663244441));
#74373=CARTESIAN_POINT('Ctrl Pts',(-0.434772350925555,2.14478346402337,
4.9453366679669));
#74374=CARTESIAN_POINT('Ctrl Pts',(-0.273004867762902,1.75867772127277,
4.96520701148968));
#74375=CARTESIAN_POINT('Ctrl Pts',(0.139207415312882,1.68568870242346,4.98507735501248));
#74376=CARTESIAN_POINT('Ctrl Pts',(0.423715846218783,1.99277389570991,5.00494769853526));
#74377=CARTESIAN_POINT('Ctrl Pts',(0.319522671921894,2.39822444216695,5.02481804205805));
#74378=CARTESIAN_POINT('Ctrl Pts',(-0.0777890547791136,2.5300946625273,
5.04468838558084));
#74379=CARTESIAN_POINT('Ctrl Pts',(-0.403739913744015,2.26741158212004,
5.06455872910363));
#74380=CARTESIAN_POINT('Ctrl Pts',(-0.359314366074708,1.85115116614648,
5.08442907262642));
#74381=CARTESIAN_POINT('Ctrl Pts',(0.0147331962342516,1.66317567752396,
5.10429941614921));
#74382=CARTESIAN_POINT('Ctrl Pts',(0.375265056741863,1.87592703651163,5.124169759672));
#74383=CARTESIAN_POINT('Ctrl Pts',(0.39154231541309,2.29423483472046,5.14404010319479));
#74384=CARTESIAN_POINT('Ctrl Pts',(0.0486328033657723,2.53435861475826,
5.16391044671758));
#74385=CARTESIAN_POINT('Ctrl Pts',(-0.338890685011317,2.37601749834112,
5.18378079024037));
#74386=CARTESIAN_POINT('Ctrl Pts',(-0.415528105691254,1.96446790358528,
5.20365113376316));
#74387=CARTESIAN_POINT('Ctrl Pts',(-0.110975058442913,1.67725055626113,
5.22352147728595));
#74388=CARTESIAN_POINT('Ctrl Pts',(0.295382497036827,1.77784827142755,5.24339182080874));
#74389=CARTESIAN_POINT('Ctrl Pts',(0.430766824181072,2.1739763405616,5.26326216433152));
#74390=CARTESIAN_POINT('Ctrl Pts',(0.170981233746816,2.50224118819976,5.28313250785433));
#74391=CARTESIAN_POINT('Ctrl Pts',(-0.245656361657064,2.46150450585759,
5.30300285137709));
#74392=CARTESIAN_POINT('Ctrl Pts',(-0.436937688334339,2.08913665378555,
5.32287319489991));
#74393=CARTESIAN_POINT('Ctrl Pts',(-0.22738816965979,1.72673444295421,5.34274353842268));
#74394=CARTESIAN_POINT('Ctrl Pts',(0.190759038573631,1.70675256519541,5.36261388194548));
#74395=CARTESIAN_POINT('Ctrl Pts',(0.433910798413821,2.04752167306581,5.38248422546826));
#74396=CARTESIAN_POINT('Ctrl Pts',(0.279008472330408,2.43643250161924,5.40235456899106));
#74397=CARTESIAN_POINT('Ctrl Pts',(-0.131846143542539,2.51671231108631,
5.42222491251384));
#74398=CARTESIAN_POINT('Ctrl Pts',(-0.421749871946843,2.21471530539013,
5.44209525603663));
#74399=CARTESIAN_POINT('Ctrl Pts',(-0.324755508900358,1.80748262407713,
5.46196559955943));
#74400=CARTESIAN_POINT('Ctrl Pts',(0.0701578220919378,1.66859481252858,
5.48183594308221));
#74401=CARTESIAN_POINT('Ctrl Pts',(0.400710902439894,1.92546252997211,5.50170628660501));
#74402=CARTESIAN_POINT('Ctrl Pts',(0.363666281662623,2.3424446150353,5.52157663012779));
#74403=CARTESIAN_POINT('Ctrl Pts',(-0.00699264384645848,2.53701677165752,
5.54144697365058));
#74404=CARTESIAN_POINT('Ctrl Pts',(-0.371236770588911,2.33068553474513,
5.56131731717337));
#74405=CARTESIAN_POINT('Ctrl Pts',(-0.39492169963869,1.91273172470378,5.58118766069616));
#74406=CARTESIAN_POINT('Ctrl Pts',(-0.0563197330045467,1.66657106297314,
5.60105800421896));
#74407=CARTESIAN_POINT('Ctrl Pts',(0.333947921421964,1.81802244494308,5.62092834774173));
#74408=CARTESIAN_POINT('Ctrl Pts',(0.417863820848056,2.2281498459,5.64079869126453));
#74409=CARTESIAN_POINT('Ctrl Pts',(0.118446551668408,2.52071720926984,5.66066903478731));
#74410=CARTESIAN_POINT('Ctrl Pts',(-0.289629303625079,2.4273338086107,5.68053937831011));
#74411=CARTESIAN_POINT('Ctrl Pts',(-0.432009702311787,2.03366620102533,
5.7004097218329));
#74412=CARTESIAN_POINT('Ctrl Pts',(-0.178080011937646,1.70085082346795,
5.72028006535568));
#74413=CARTESIAN_POINT('Ctrl Pts',(0.239213845984823,1.73420047612512,5.74015040887847));
#74414=CARTESIAN_POINT('Ctrl Pts',(0.437061566240658,2.10312139282916,5.76002075240126));
#74415=CARTESIAN_POINT('Ctrl Pts',(0.233964800030075,2.46917885655169,5.77989109592406));
#74416=CARTESIAN_POINT('Ctrl Pts',(-0.183762818776739,2.49656497855101,
5.79976143944684));
#74417=CARTESIAN_POINT('Ctrl Pts',(-0.432913068404649,2.16015672017656,
5.81963178296963));
#74418=CARTESIAN_POINT('Ctrl Pts',(-0.284924513563698,1.76856286063808,
5.83950212649242));
#74419=CARTESIAN_POINT('Ctrl Pts',(0.124443493502042,1.68101745537201,5.85937247001521));
#74420=CARTESIAN_POINT('Ctrl Pts',(0.4196515367315,1.97783149547931,5.879242813538));
#74421=CARTESIAN_POINT('Ctrl Pts',(0.329886425407692,2.38671850674427,5.89911315706079));
#74422=CARTESIAN_POINT('Ctrl Pts',(-0.06250457124619,2.5325803212714,5.91898350058358));
#74423=CARTESIAN_POINT('Ctrl Pts',(-0.397556133010694,2.28160858152498,
5.93885384410637));
#74424=CARTESIAN_POINT('Ctrl Pts',(-0.36790406511818,1.86403569200524,5.95872418762916));
#74425=CARTESIAN_POINT('Ctrl Pts',(-0.000750103095509274,1.66292793143089,
5.97859453115195));
#74426=CARTESIAN_POINT('Ctrl Pts',(0.367091976399978,1.86277429177955,5.99846487467474));
#74427=CARTESIAN_POINT('Ctrl Pts',(0.398177142608358,2.28024294405656,6.01833521819753));
#74428=CARTESIAN_POINT('Ctrl Pts',(0.063988987396686,2.53236323302274,6.03820556172031));
#74429=CARTESIAN_POINT('Ctrl Pts',(-0.328900352437435,2.38784911662964,
6.05807590524311));
#74430=CARTESIAN_POINT('Ctrl Pts',(-0.420068394649978,1.9792726228475,6.07794624876589));
#74431=CARTESIAN_POINT('Ctrl Pts',(-0.125880871919137,1.6814470620545,6.09781659228868));
#74432=CARTESIAN_POINT('Ctrl Pts',(0.283785213664268,1.76758684098932,6.11768693581147));
#74433=CARTESIAN_POINT('Ctrl Pts',(0.43311699957894,2.15867043935124,6.13755727933426));
#74434=CARTESIAN_POINT('Ctrl Pts',(0.185122901935055,2.49593189686748,6.15742762285705));
#74435=CARTESIAN_POINT('Ctrl Pts',(-0.232696256026886,2.4699797402683,6.17729796637985));
#74436=CARTESIAN_POINT('Ctrl Pts',(-0.437048277818848,2.10462154016639,
6.19716830990262));
#74437=CARTESIAN_POINT('Ctrl Pts',(-0.24046800346235,1.7350237061277,6.21703865342543));
#74438=CARTESIAN_POINT('Ctrl Pts',(0.176708927308292,1.70024193468113,6.2369089969482));
#74439=CARTESIAN_POINT('Ctrl Pts',(0.431779474021718,2.03218376601832,6.256779340471));
#74440=CARTESIAN_POINT('Ctrl Pts',(0.290751134787684,2.42633775968712,6.27664968399379));
#74441=CARTESIAN_POINT('Ctrl Pts',(-0.117001788421295,2.52112128571726,
6.29652002751657));
#74442=CARTESIAN_POINT('Ctrl Pts',(-0.417421499108909,2.22958336258796,
6.31639037103937));
#74443=CARTESIAN_POINT('Ctrl Pts',(-0.334913811169784,1.81917034546604,
6.33626071456215));
#74444=CARTESIAN_POINT('Ctrl Pts',(0.0548317041193742,1.66638030487385,
6.35613105808495));
#74445=CARTESIAN_POINT('Ctrl Pts',(0.394276595541465,1.91137730256896,6.37600140160773));
#74446=CARTESIAN_POINT('Ctrl Pts',(0.372026386465847,2.32940994649555,6.39587174513052));
#74447=CARTESIAN_POINT('Ctrl Pts',(0.00849261462696172,2.53699019585654,
6.41574208865331));
#74448=CARTESIAN_POINT('Ctrl Pts',(-0.362831974967082,2.34369143136232,
6.43561243217611));
#74449=CARTESIAN_POINT('Ctrl Pts',(-0.401307622641875,1.92683895418584,
6.45548277569889));
#74450=CARTESIAN_POINT('Ctrl Pts',(-0.0716381596422418,1.66883816279614,
6.47535311922169));
#74451=CARTESIAN_POINT('Ctrl Pts',(0.323749562174376,1.8063696596572,6.49522346274447));
#74452=CARTESIAN_POINT('Ctrl Pts',(0.422141135218989,2.21326701962157,6.51509380626727));
#74453=CARTESIAN_POINT('Ctrl Pts',(0.133275686026303,2.51625730899547,6.53496414979004));
#74454=CARTESIAN_POINT('Ctrl Pts',(-0.277852061249243,2.43738818568153,
6.55483449331285));
#74455=CARTESIAN_POINT('Ctrl Pts',(-0.434088368471071,2.04901133325871,
6.57470483683562));
#74456=CARTESIAN_POINT('Ctrl Pts',(-0.192107693415753,1.70740964109086,
6.59457518035843));
#74457=CARTESIAN_POINT('Ctrl Pts',(0.226105637247668,1.72595615687094,6.6144455238812));
#74458=CARTESIAN_POINT('Ctrl Pts',(0.436897827239315,2.08763697725087,6.634315867404));
#74459=CARTESIAN_POINT('Ctrl Pts',(0.246895739007226,2.46065918792955,6.65418621092679));
#74460=CARTESIAN_POINT('Ctrl Pts',(-0.169599577944252,2.50282569299769,
6.67405655444958));
#74461=CARTESIAN_POINT('Ctrl Pts',(-0.430510371029507,2.17545446450653,
6.69392689797236));
#74462=CARTESIAN_POINT('Ctrl Pts',(-0.296486507389875,1.77886403702843,
6.71379724149516));
#74463=CARTESIAN_POINT('Ctrl Pts',(0.109523363786731,1.67687213686313,6.73366758501794));
#74464=CARTESIAN_POINT('Ctrl Pts',(0.41506045894861,1.96304244746893,6.75353792854074));
#74465=CARTESIAN_POINT('Ctrl Pts',(0.339836088404225,2.37485266743484,6.77340827206352));
#74466=CARTESIAN_POINT('Ctrl Pts',(-0.0471416287452485,2.53452298284116,
6.79327861558631));
#74467=CARTESIAN_POINT('Ctrl Pts',(-0.390873319274194,2.29557761645317,
6.8131489591091));
#74468=CARTESIAN_POINT('Ctrl Pts',(-0.376031951966423,1.87721641245762,
6.8330193026319));
#74469=CARTESIAN_POINT('Ctrl Pts',(-0.0162324608571044,1.66322882078547,
6.85288964615468));
#74470=CARTESIAN_POINT('Ctrl Pts',(0.358458103238608,1.84991932501589,6.87275998967748));
#74471=CARTESIAN_POINT('Ctrl Pts',(0.404312157277081,2.26602480313461,6.89263033320026));
#74472=CARTESIAN_POINT('Ctrl Pts',(0.0792648491437742,2.52982512661331,
6.91250067672305));
#74473=CARTESIAN_POINT('Ctrl Pts',(-0.318497167144145,2.39931941183139,
6.93237102024584));
#74474=CARTESIAN_POINT('Ctrl Pts',(-0.424081392051288,1.99422888535251,
6.95224136376863));
#74475=CARTESIAN_POINT('Ctrl Pts',(-0.140628673219612,1.68616895712571,
6.97211170729142));
#74476=CARTESIAN_POINT('Ctrl Pts',(0.271831708425969,1.75774267272686,6.99198205081421));
#74477=CARTESIAN_POINT('Ctrl Pts',(0.434923504136159,2.14329089197343,7.01185239433699));
#74478=CARTESIAN_POINT('Ctrl Pts',(0.199032194289939,2.48912561135713,7.03172273785979));
#74479=CARTESIAN_POINT('Ctrl Pts',(-0.219444058030784,2.47799055698908,
7.05159308138258));
#74480=CARTESIAN_POINT('Ctrl Pts',(-0.436610261719101,2.12010062535118,
7.07146342490537));
#74481=CARTESIAN_POINT('Ctrl Pts',(-0.253245989399967,1.74377110640662,
7.09133376842815));
#74482=CARTESIAN_POINT('Ctrl Pts',(0.162437001865369,1.69423310114929,7.11120411195095));
#74483=CARTESIAN_POINT('Ctrl Pts',(0.42910615772017,2.01693098541236,7.13107445547373));
#74484=CARTESIAN_POINT('Ctrl Pts',(0.30212883139503,2.41583338173442,7.15094479899653));
#74485=CARTESIAN_POINT('Ctrl Pts',(-0.102010566608769,2.5250016471475,7.17081514251931));
#74486=CARTESIAN_POINT('Ctrl Pts',(-0.412569157233639,2.24428876005239,
7.19068548604211));
#74487=CARTESIAN_POINT('Ctrl Pts',(-0.344651712315627,1.83121057875013,
7.21055582956488));
#74488=CARTESIAN_POINT('Ctrl Pts',(0.0394367585581893,1.66471009906919,
7.23042617308769));
#74489=CARTESIAN_POINT('Ctrl Pts',(0.387347372284745,1.89752884412333,7.25029651661046));
#74490=CARTESIAN_POINT('Ctrl Pts',(0.379919504523068,2.31608731073545,7.27016686013327));
#74491=CARTESIAN_POINT('Ctrl Pts',(0.0239672127316146,2.53641508737876,
7.29003720365604));
#74492=CARTESIAN_POINT('Ctrl Pts',(-0.353971733899714,2.3563914339013,7.30990754717885));
#74493=CARTESIAN_POINT('Ctrl Pts',(-0.407189803578201,1.94116354436126,
7.32977789070163));
#74494=CARTESIAN_POINT('Ctrl Pts',(-0.0868666623598067,1.67164647923894,
7.34964823422442));
#74495=CARTESIAN_POINT('Ctrl Pts',(0.313144815745497,1.79508545434884,7.36951857774721));
#74496=CARTESIAN_POINT('Ctrl Pts',(0.425888556221436,2.19824201472666,7.38938892126999));
#74497=CARTESIAN_POINT('Ctrl Pts',(0.147937525855628,2.51127490103536,7.40925926479279));
#74498=CARTESIAN_POINT('Ctrl Pts',(-0.265726044607188,2.44701905566604,
7.42912960831557));
#74499=CARTESIAN_POINT('Ctrl Pts',(-0.435622144477278,2.0644204691016,7.44899995183837));
#74500=CARTESIAN_POINT('Ctrl Pts',(-0.20589423138927,1.7144612584207,7.46887029536115));
#74501=CARTESIAN_POINT('Ctrl Pts',(0.212713609029873,1.71818135677861,7.48874063888394));
#74502=CARTESIAN_POINT('Ctrl Pts',(0.436185671507062,2.07216808037763,7.50861098240673));
#74503=CARTESIAN_POINT('Ctrl Pts',(0.259516761693601,2.45168680125645,7.52848132592952));
#74504=CARTESIAN_POINT('Ctrl Pts',(-0.155223446956909,2.50858075981714,
7.54835166945232));
#74505=CARTESIAN_POINT('Ctrl Pts',(-0.427567274788573,2.1906574944933,7.56822201297509));
#74506=CARTESIAN_POINT('Ctrl Pts',(-0.307676336030043,1.78956831987527,
7.5880923564979));
#74507=CARTESIAN_POINT('Ctrl Pts',(0.0944657546852107,1.67325795031462,
7.60796270002068));
#74508=CARTESIAN_POINT('Ctrl Pts',(0.409948375828002,1.94842531565623,7.62783304354347));
#74509=CARTESIAN_POINT('Ctrl Pts',(0.349359171580419,2.36264181885332,7.64770338706626));
#74510=CARTESIAN_POINT('Ctrl Pts',(-0.031719511635709,2.53592020870742,
7.66757373058905));
#74511=CARTESIAN_POINT('Ctrl Pts',(-0.38369986114765,2.30930115225006,7.68744407411183));
#74512=CARTESIAN_POINT('Ctrl Pts',(-0.383687824075844,1.89067678238218,
7.70731441763464));
#74513=CARTESIAN_POINT('Ctrl Pts',(-0.0316944427949657,1.6640779678958,
7.72718476115741));
#74514=CARTESIAN_POINT('Ctrl Pts',(0.349374274941528,1.83737827243922,7.74705510468021));
#74515=CARTESIAN_POINT('Ctrl Pts',(0.409939658431796,2.25159825929987,7.76692544820299));
#74516=CARTESIAN_POINT('Ctrl Pts',(0.0944412135559431,2.5267474814923,7.78679579172579));
#74517=CARTESIAN_POINT('Ctrl Pts',(-0.307694187747241,2.41041398583906,
7.80666613524857));
#74518=CARTESIAN_POINT('Ctrl Pts',(-0.427562060573467,2.00931791722671,
7.82653647877136));
#74519=CARTESIAN_POINT('Ctrl Pts',(-0.155199950142004,1.69141031430805,
7.84640682229416));
#74520=CARTESIAN_POINT('Ctrl Pts',(0.259536985979435,1.7483281235489,7.86627716581694));
#74521=CARTESIAN_POINT('Ctrl Pts',(0.436184070234853,2.1278570036308,7.88614750933974));
#74522=CARTESIAN_POINT('Ctrl Pts',(0.212691651148888,2.48183087527004,7.90601785286252));
#74523=CARTESIAN_POINT('Ctrl Pts',(-0.205916402512528,2.48552690042879,
7.92588819638531));
#74524=CARTESIAN_POINT('Ctrl Pts',(-0.435624189855542,2.13555447919227,
7.9457585399081));
#74525=CARTESIAN_POINT('Ctrl Pts',(-0.265706087884356,1.75296566360212,
7.96562888343089));
#74526=CARTESIAN_POINT('Ctrl Pts',(0.147961177103221,1.68873360719825,7.98549922695368));
#74527=CARTESIAN_POINT('Ctrl Pts',(0.425894205193953,2.00178247732637,8.00536957047647));
#74528=CARTESIAN_POINT('Ctrl Pts',(0.313127280279686,2.40493255339923,8.02523991399926));
#74529=CARTESIAN_POINT('Ctrl Pts',(-0.0868912958612956,2.52834852454686,
8.04511025752205));
#74530=CARTESIAN_POINT('Ctrl Pts',(-0.407198937231307,2.25881303880861,
8.06498060104484));
#74531=CARTESIAN_POINT('Ctrl Pts',(-0.353956988821141,1.84358821040638,
8.08485094456762));
#74532=CARTESIAN_POINT('Ctrl Pts',(0.0239923099396314,1.66358629164325,
8.10472128809042));
#74533=CARTESIAN_POINT('Ctrl Pts',(0.379931930588853,1.88393453793593,8.1245916316132));
#74534=CARTESIAN_POINT('Ctrl Pts',(0.387335727984592,2.30249343101586,8.144461975136));
#74535=CARTESIAN_POINT('Ctrl Pts',(0.0394117259522656,2.53529216813009,
8.16433231865878));
#74536=CARTESIAN_POINT('Ctrl Pts',(-0.344667169219275,2.36876960066255,
8.18420266218158));
#74537=CARTESIAN_POINT('Ctrl Pts',(-0.412560858830175,1.95568751426422,
8.20407300570436));
#74538=CARTESIAN_POINT('Ctrl Pts',(-0.10198612555365,1.67499248715759,8.22394334922715));
#74539=CARTESIAN_POINT('Ctrl Pts',(0.302146993761083,1.78418399353568,8.24381369274995));
#74540=CARTESIAN_POINT('Ctrl Pts',(0.42910137989889,2.18309369137787,8.26368403627273));
#74541=CARTESIAN_POINT('Ctrl Pts',(0.162413666857334,2.50577623956545,8.28355437979553));
#74542=CARTESIAN_POINT('Ctrl Pts',(-0.253266474901655,2.4562143293985,8.30342472331831));
#74543=CARTESIAN_POINT('Ctrl Pts',(-0.436609105055496,2.07987426621036,
8.3232950668411));
#74544=CARTESIAN_POINT('Ctrl Pts',(-0.219422320283272,1.72199682390298,
8.34316541036389));
#74545=CARTESIAN_POINT('Ctrl Pts',(0.199054571697336,1.71088583517903,8.36303575388668));
#74546=CARTESIAN_POINT('Ctrl Pts',(0.434925992978568,2.05673411956821,8.38290609740947));
#74547=CARTESIAN_POINT('Ctrl Pts',(0.271812025529305,2.44227295913581,8.40277644093226));
#74548=CARTESIAN_POINT('Ctrl Pts',(-0.140652471477245,2.51382295495208,
8.42264678445504));
#74549=CARTESIAN_POINT('Ctrl Pts',(-0.42408747400835,2.20574672650795,8.44251712797784));
#74550=CARTESIAN_POINT('Ctrl Pts',(-0.318479953433018,1.80066227260963,
8.46238747150062));
#74551=CARTESIAN_POINT('Ctrl Pts',(0.0792895672865693,1.67017943244019,
8.48225781502342));
#74552=CARTESIAN_POINT('Ctrl Pts',(0.404321704320595,1.93399844822044,8.5021281585462));
#74553=CARTESIAN_POINT('Ctrl Pts',(0.358443721070139,2.35010128868785,8.521998502069));
#74554=CARTESIAN_POINT('Ctrl Pts',(-0.0162575785559514,2.53677024500007,
8.54186884559178));
#74555=CARTESIAN_POINT('Ctrl Pts',(-0.376044763126415,2.32276196242431,
8.56173918911457));
#74556=CARTESIAN_POINT('Ctrl Pts',(-0.390862071400124,1.90439990562698,
8.58160953263737));
#74557=CARTESIAN_POINT('Ctrl Pts',(-0.0471166402303176,1.66547430686859,
8.60147987616015));
#74558=CARTESIAN_POINT('Ctrl Pts',(0.339851893999448,1.82516687622683,8.62135021968295));
#74559=CARTESIAN_POINT('Ctrl Pts',(0.415052582142242,2.23698142149572,8.64122056320573));
#74560=CARTESIAN_POINT('Ctrl Pts',(0.109499030476289,2.5231341608789,8.66109090672852));
#74561=CARTESIAN_POINT('Ctrl Pts',(-0.296504974704751,2.42111891217004,
8.68096125025131));
#74562=CARTESIAN_POINT('Ctrl Pts',(-0.430506031101505,2.0245207779375,8.7008315937741));
#74563=CARTESIAN_POINT('Ctrl Pts',(-0.169576412066495,1.6971645543791,8.72070193729689));
#74564=CARTESIAN_POINT('Ctrl Pts',(0.246916479295651,1.73935501108407,8.74057228081968));
#74565=CARTESIAN_POINT('Ctrl Pts',(0.436897115547312,2.11238814773762,8.76044262434247));
#74566=CARTESIAN_POINT('Ctrl Pts',(0.226084126455762,2.47405684533593,8.78031296786525));
#74567=CARTESIAN_POINT('Ctrl Pts',(-0.192130270084417,2.49257931057968,
8.80018331138805));
#74568=CARTESIAN_POINT('Ctrl Pts',(-0.43409129999653,2.15096370321368,8.82005365491084));
#74569=CARTESIAN_POINT('Ctrl Pts',(-0.277832658355979,1.76259583623082,
8.83992399843362));
#74570=CARTESIAN_POINT('Ctrl Pts',(0.133299623825185,1.68375035607703,8.85979434195643));
#74571=CARTESIAN_POINT('Ctrl Pts',(0.422147648251856,1.98675725695057,8.87966468547919));
#74572=CARTESIAN_POINT('Ctrl Pts',(0.323732675620234,2.39364895796461,8.89953502900202));
#74573=CARTESIAN_POINT('Ctrl Pts',(-0.0716629546688544,2.53115771674186,
8.91940537252477));
#74574=CARTESIAN_POINT('Ctrl Pts',(-0.401317580079588,2.27313796723133,
8.93927571604757));
#74575=CARTESIAN_POINT('Ctrl Pts',(-0.362817960222371,1.85628770339187,
8.95914605957037));
#74576=CARTESIAN_POINT('Ctrl Pts',(0.00851774493375449,1.66301029325719,
8.97901640309315));
#74577=CARTESIAN_POINT('Ctrl Pts',(0.372039578699426,1.87061144828242,8.99888674661594));
#74578=CARTESIAN_POINT('Ctrl Pts',(0.394265747623478,2.28864537107714,9.01875709013873));
#74579=CARTESIAN_POINT('Ctrl Pts',(0.0548067675377615,2.5336228476568,9.03862743366152));
#74580=CARTESIAN_POINT('Ctrl Pts',(-0.334929960496195,2.38081039393147,
9.05849777718431));
#74581=CARTESIAN_POINT('Ctrl Pts',(-0.417414046371677,1.97039263265711,
9.0783681207071));
#74582=CARTESIAN_POINT('Ctrl Pts',(-0.116977570492231,1.67887198647007,
9.09823846422989));
#74583=CARTESIAN_POINT('Ctrl Pts',(0.290769901255634,1.77367896129468,9.11810880775268));
#74584=CARTESIAN_POINT('Ctrl Pts',(0.43177557334904,2.16784106453351,9.13797915127547));
#74585=CARTESIAN_POINT('Ctrl Pts',(0.176685937831131,2.49976822678981,9.15784949479826));
#74586=CARTESIAN_POINT('Ctrl Pts',(-0.240488992028429,2.46496246449612,
9.17771983832104));
#74587=CARTESIAN_POINT('Ctrl Pts',(-0.437048011321802,2.09535332618026,
9.19759018184385));
#74588=CARTESIAN_POINT('Ctrl Pts',(-0.232674978941475,1.73000687850648,
9.21746052536661));
#74589=CARTESIAN_POINT('Ctrl Pts',(0.185145670779582,1.7040787497879,9.23733086888943));
#74590=CARTESIAN_POINT('Ctrl Pts',(0.433120372867424,2.04135446832782,9.2572012124122));
#74591=CARTESIAN_POINT('Ctrl Pts',(0.283766096863767,2.43242947830877,9.277071555935));
#74592=CARTESIAN_POINT('Ctrl Pts',(-0.125904941746689,2.51854569812828,
9.29694189945778));
#74593=CARTESIAN_POINT('Ctrl Pts',(-0.420075336714605,2.22070321976667,
9.31681224298058));
#74594=CARTESIAN_POINT('Ctrl Pts',(-0.328883798339925,1.81213196952868,
9.33668258650336));
#74595=CARTESIAN_POINT('Ctrl Pts',(0.0640138515255109,1.66764044755458,
9.35655293002616));
#74596=CARTESIAN_POINT('Ctrl Pts',(0.398187507315239,1.91977995451115,9.37642327354892));
#74597=CARTESIAN_POINT('Ctrl Pts',(0.367078333477388,2.33724681846001,9.39629361707175));
#74598=CARTESIAN_POINT('Ctrl Pts',(-0.000775238123413455,2.53707202470964,
9.4161639605945));
#74599=CARTESIAN_POINT('Ctrl Pts',(-0.367917634285118,2.33594315027136,
9.43603430411731));
#74600=CARTESIAN_POINT('Ctrl Pts',(-0.397545688453278,1.91836855621853,
9.45590464764009));
#74601=CARTESIAN_POINT('Ctrl Pts',(-0.0624796944239493,1.66741608494695,
9.47577499116289));
#74602=CARTESIAN_POINT('Ctrl Pts',(0.329902913397025,1.81330046475433,9.49564533468568));
#74603=CARTESIAN_POINT('Ctrl Pts',(0.419644510402349,2.22219263753232,9.51551567820846));
#74604=CARTESIAN_POINT('Ctrl Pts',(0.124419398554859,2.51898970039988,9.53538602173126));
#74605=CARTESIAN_POINT('Ctrl Pts',(-0.284943573295104,2.43142075344756,
9.55525636525406));
#74606=CARTESIAN_POINT('Ctrl Pts',(-0.432909608211464,2.03981838406849,
9.57512670877682));
#74607=CARTESIAN_POINT('Ctrl Pts',(-0.183740012915144,1.70342445431939,
9.59499705229965));
#74608=CARTESIAN_POINT('Ctrl Pts',(0.233986030286801,1.73083459884687,9.61486739582239));
#74609=CARTESIAN_POINT('Ctrl Pts',(0.437061745022211,2.09690374160118,9.63473773934522));
#74610=CARTESIAN_POINT('Ctrl Pts',(0.239192809283464,2.46581327991889,9.65460808286798));
#74611=CARTESIAN_POINT('Ctrl Pts',(-0.178102965812306,2.49913893489208,
9.67447842639079));
#74612=CARTESIAN_POINT('Ctrl Pts',(-0.432013516304637,2.16630895496111,
9.69434876991358));
#74613=CARTESIAN_POINT('Ctrl Pts',(-0.289610478916907,1.77264953600239,
9.71421911343635));
#74614=CARTESIAN_POINT('Ctrl Pts',(0.118470745970611,1.67928960301997,9.73408945695917));
#74615=CARTESIAN_POINT('Ctrl Pts',(0.417871189765774,1.97187418471803,9.75395980048193));
#74616=CARTESIAN_POINT('Ctrl Pts',(0.333931704976374,2.38199675918263,9.77383014400474));
#74617=CARTESIAN_POINT('Ctrl Pts',(-0.0563446584322808,2.53342569748929,
9.79370048752751));
#74618=CARTESIAN_POINT('Ctrl Pts',(-0.394932468361915,2.28724556393009,
9.81357083105031));
#74619=CARTESIAN_POINT('Ctrl Pts',(-0.371223503770095,1.86929311664672,
9.8334411745731));
#74620=CARTESIAN_POINT('Ctrl Pts',(-0.0069675119857552,1.66298282693393,
9.85331151809589));
#74621=CARTESIAN_POINT('Ctrl Pts',(0.363680223504416,1.85757629899345,9.87318186161868));
#74622=CARTESIAN_POINT('Ctrl Pts',(0.40070086452094,2.27456051371974,9.89305220514146));
#74623=CARTESIAN_POINT('Ctrl Pts',(0.0701330128363399,2.53140922137621,
9.91292254866427));
#74624=CARTESIAN_POINT('Ctrl Pts',(-0.324772330378065,2.39249869948212,
9.93279289218704));
#74625=CARTESIAN_POINT('Ctrl Pts',(-0.421743274230899,1.9852604409154,9.95266323570984));
#74626=CARTESIAN_POINT('Ctrl Pts',(-0.131822179139127,1.68328010742834,
9.97253357923261));
#74627=CARTESIAN_POINT('Ctrl Pts',(0.279027819343617,1.76358354408519,9.99240392275542));
#74628=CARTESIAN_POINT('Ctrl Pts',(0.433907779786064,2.15250328007904,10.0122742662782));
#74629=CARTESIAN_POINT('Ctrl Pts',(0.190736423484932,2.49325840427651,10.0321446098011));
#74630=CARTESIAN_POINT('Ctrl Pts',(-0.227409634944321,2.47325247984765,
10.0520149533238));
#74631=CARTESIAN_POINT('Ctrl Pts',(-0.43693831233838,2.11083821889525,10.0718852968466));
#74632=CARTESIAN_POINT('Ctrl Pts',(-0.245635571941848,1.73848136759673,
10.0917556403694));
#74633=CARTESIAN_POINT('Ctrl Pts',(0.171004365447838,1.69776864521061,10.1116259838922));
#74634=CARTESIAN_POINT('Ctrl Pts',(0.430771077681311,2.02604843198948,10.131496327415));
#74635=CARTESIAN_POINT('Ctrl Pts',(0.295363970328877,2.42216871482112,10.1513666709378));
#74636=CARTESIAN_POINT('Ctrl Pts',(-0.11099936962669,2.52274306111444,10.1712370144606));
#74637=CARTESIAN_POINT('Ctrl Pts',(-0.415535899149414,2.23550820010619,
10.1911073579834));
#74638=CARTESIAN_POINT('Ctrl Pts',(-0.338874811306978,1.82396301327614,
10.2109777015061));
#74639=CARTESIAN_POINT('Ctrl Pts',(0.0486577822698844,1.66564418272284,
10.2308480450289));
#74640=CARTESIAN_POINT('Ctrl Pts',(0.391553484773028,1.90578768231641,10.2507183885517));
#74641=CARTESIAN_POINT('Ctrl Pts',(0.375252170190449,2.3240945437651,10.2705887320745));
#74642=CARTESIAN_POINT('Ctrl Pts',(0.0147080754280776,2.53682516902661,
10.2904590755973));
#74643=CARTESIAN_POINT('Ctrl Pts',(-0.359328676215894,2.34882817008302,
10.3103294191201));
#74644=CARTESIAN_POINT('Ctrl Pts',(-0.403730285613773,1.93256519998473,
10.3301997626429));
#74645=CARTESIAN_POINT('Ctrl Pts',(-0.0777643208762883,1.66990086471073,
10.3500701061657));
#74646=CARTESIAN_POINT('Ctrl Pts',(0.319539821608869,1.80179393335463,10.3699404496885));
#74647=CARTESIAN_POINT('Ctrl Pts',(0.423709679186456,2.20725047105558,10.3898107932113));
#74648=CARTESIAN_POINT('Ctrl Pts',(0.139183588974562,2.51431930239623,10.409681136734));
#74649=CARTESIAN_POINT('Ctrl Pts',(-0.273024495986857,2.44130657826807,
10.4295514802568));
#74650=CARTESIAN_POINT('Ctrl Pts',(-0.434769774809129,2.05519153327387,
10.4494218237796));
#74651=CARTESIAN_POINT('Ctrl Pts',(-0.197672973804186,1.71018215637898,
10.4692921673024));
#74652=CARTESIAN_POINT('Ctrl Pts',(0.22076186992074,1.72277758209906,10.4891625108252));
#74653=CARTESIAN_POINT('Ctrl Pts',(0.436677752008117,2.0814232220483,10.509032854348));
#74654=CARTESIAN_POINT('Ctrl Pts',(0.252001244935848,2.45711052676827,10.5289031978708));
#74655=CARTESIAN_POINT('Ctrl Pts',(-0.163852097493456,2.50519753938657,
10.5487735413936));
#74656=CARTESIAN_POINT('Ctrl Pts',(-0.429393446921325,2.18157097228152,
10.5686438849163));
#74657=CARTESIAN_POINT('Ctrl Pts',(-0.301024765438089,1.78311414299329,
10.5885142284392));
#74658=CARTESIAN_POINT('Ctrl Pts',(0.103493157513323,1.67535694739481,10.6083845719619));
#74659=CARTESIAN_POINT('Ctrl Pts',(0.413070197767395,1.95715194263017,10.6282549154847));
#74660=CARTESIAN_POINT('Ctrl Pts',(0.343711565999386,2.3699905834954,10.6481252590075));
#74661=CARTESIAN_POINT('Ctrl Pts',(-0.0409556354686489,2.5351496199025,
10.6679956025303));
#74662=CARTESIAN_POINT('Ctrl Pts',(-0.388051617000489,2.30111812032046,
10.6878659460531));
#74663=CARTESIAN_POINT('Ctrl Pts',(-0.379163068391668,1.88258812510411,
10.7077362895759));
#74664=CARTESIAN_POINT('Ctrl Pts',(-0.0224440229241447,1.66350392715064,
10.7276066330987));
#74665=CARTESIAN_POINT('Ctrl Pts',(0.354864358098471,1.84484545246206,10.7474769766215));
#74666=CARTESIAN_POINT('Ctrl Pts',(0.40663300098569,2.26025653898454,10.7673473201443));
#74667=CARTESIAN_POINT('Ctrl Pts',(0.0853712235528269,2.52865406794643,
10.787217663667));
#74668=CARTESIAN_POINT('Ctrl Pts',(-0.314207029247148,2.40381984554933,
10.8070880071898));
#74669=CARTESIAN_POINT('Ctrl Pts',(-0.425543108137308,2.00027227619777,
10.8269583507126));
#74670=CARTESIAN_POINT('Ctrl Pts',(-0.146501317774399,1.68821131673115,
10.8468286942354));
#74671=CARTESIAN_POINT('Ctrl Pts',(0.266935487293065,1.75391041419663,10.8666990377582));
#74672=CARTESIAN_POINT('Ctrl Pts',(0.435495322754263,2.13709959079413,10.886569381281));
#74673=CARTESIAN_POINT('Ctrl Pts',(0.204547486923011,2.48625494349122,10.9064397248038));
#74674=CARTESIAN_POINT('Ctrl Pts',(-0.214044821534287,2.4810739693974,10.9263100683266));
#74675=CARTESIAN_POINT('Ctrl Pts',(-0.436280145805049,2.12630950691779,
10.9461804118494));
#74676=CARTESIAN_POINT('Ctrl Pts',(-0.258287830478275,1.74740965355706,
10.9660507553721));
#74677=CARTESIAN_POINT('Ctrl Pts',(0.156648406599361,1.6919634422165,10.9859210988949));
#74678=CARTESIAN_POINT('Ctrl Pts',(0.427881056376946,2.01083522348101,11.0057914424177));
#74679=CARTESIAN_POINT('Ctrl Pts',(0.306591087674502,2.41150354851348,11.0256617859405));
#74680=CARTESIAN_POINT('Ctrl Pts',(-0.0959544653616712,2.52640977516363,
11.0455321294633));
#74681=CARTESIAN_POINT('Ctrl Pts',(-0.410474859449393,2.2501430835501,11.0654024729861));
#74682=CARTESIAN_POINT('Ctrl Pts',(-0.348440451098382,1.83614055291446,
11.0852728165089));
#74683=CARTESIAN_POINT('Ctrl Pts',(0.0332406352514093,1.66419314375975,
11.1051431600317));
#74684=CARTESIAN_POINT('Ctrl Pts',(0.384427964061884,1.89203919545942,11.1250135035545));
#74685=CARTESIAN_POINT('Ctrl Pts',(0.382954970987067,2.31066097401803,11.1448838470773));
#74686=CARTESIAN_POINT('Ctrl Pts',(0.0301729266431917,2.53602998781703,
11.1647541906));
#74687=CARTESIAN_POINT('Ctrl Pts',(-0.350288670222764,2.36140084791656,
11.1846245341228));
#74688=CARTESIAN_POINT('Ctrl Pts',(-0.409408099655643,1.94697201656466,
11.2044948776456));
#74689=CARTESIAN_POINT('Ctrl Pts',(-0.0929513335343224,1.67292552713593,
11.2243652211684));
#74690=CARTESIAN_POINT('Ctrl Pts',(0.308775626923337,1.7906617256206,11.2442355646912));
#74691=CARTESIAN_POINT('Ctrl Pts',(0.427242985684624,2.19217367824504,11.264105908214));
#74692=CARTESIAN_POINT('Ctrl Pts',(0.153773068960608,2.50912882939285,11.2839762517368));
#74693=CARTESIAN_POINT('Ctrl Pts',(-0.260762704221777,2.45076397743336,
11.3038465952596));
#74694=CARTESIAN_POINT('Ctrl Pts',(-0.436084195917273,2.07062092838231,
11.3237169387824));
#74695=CARTESIAN_POINT('Ctrl Pts',(-0.211357805361098,1.71742917794104,
11.3435872823051));
#74696=CARTESIAN_POINT('Ctrl Pts',(0.207260597846932,1.71519407442444,11.3634576258279));
#74697=CARTESIAN_POINT('Ctrl Pts',(0.435745618512919,2.06596602102712,11.3833279693507));
#74698=CARTESIAN_POINT('Ctrl Pts',(0.26449335560258,2.44795951002957,11.4031983128735));
#74699=CARTESIAN_POINT('Ctrl Pts',(-0.14939555355422,2.51074751898966,11.4230686563963));
#74700=CARTESIAN_POINT('Ctrl Pts',(-0.426234380693095,2.19673059750206,
11.4429389999191));
#74701=CARTESIAN_POINT('Ctrl Pts',(-0.312061190117224,1.79397652148806,
11.4628093434419));
#74702=CARTESIAN_POINT('Ctrl Pts',(0.0883856590963718,1.67195732567414,
11.4826796869647));
#74703=CARTESIAN_POINT('Ctrl Pts',(0.407750698710001,1.94260901080609,11.5025500304875));
#74704=CARTESIAN_POINT('Ctrl Pts',(0.353059982502292,2.35764550167509,11.5224203740102));
#74705=CARTESIAN_POINT('Ctrl Pts',(-0.0255152028748612,2.53632732002498,
11.5422907175331));
#74706=CARTESIAN_POINT('Ctrl Pts',(-0.380683663195544,2.31473822285275,
11.5621610610558));
#74707=CARTESIAN_POINT('Ctrl Pts',(-0.386626687935257,1.89615604018234,
11.5820314045786));
#74708=CARTESIAN_POINT('Ctrl Pts',(-0.0378923609650846,1.6645729397954,
11.6019017481014));
#74709=CARTESIAN_POINT('Ctrl Pts',(0.34560304861143,1.83243488910469,11.6217720916242));
#74710=CARTESIAN_POINT('Ctrl Pts',(0.412054710693474,2.2457514019598,11.641642435147));
#74711=CARTESIAN_POINT('Ctrl Pts',(0.100502271897677,2.52536084577843,11.6615127786698));
#74712=CARTESIAN_POINT('Ctrl Pts',(-0.303247319215413,2.41475962124548,
11.6813831221926));
#74713=CARTESIAN_POINT('Ctrl Pts',(-0.428808778343008,2.01540929487284,
11.7012534657153));
#74714=CARTESIAN_POINT('Ctrl Pts',(-0.160996560384653,1.69365942446977,
11.7211238092381));
#74715=CARTESIAN_POINT('Ctrl Pts',(0.254508084024075,1.74467171384151,11.7409941527609));
#74716=CARTESIAN_POINT('Ctrl Pts',(0.436536209487655,2.12164933218561,11.7608644962837));
#74717=CARTESIAN_POINT('Ctrl Pts',(0.21810179178483,2.47876663553985,11.7807348398065));
#74718=CARTESIAN_POINT('Ctrl Pts',(-0.200411328002777,2.48841711520747,
11.8006051833293));
#74719=CARTESIAN_POINT('Ctrl Pts',(-0.435074337886463,2.14174776988761,
11.8204755268521));
#74720=CARTESIAN_POINT('Ctrl Pts',(-0.27061587278199,1.75678052914153,11.8403458703749));
#74721=CARTESIAN_POINT('Ctrl Pts',(0.142095814575594,1.68667042779638,11.8602162138977));
#74722=CARTESIAN_POINT('Ctrl Pts',(0.424453936658425,1.99573393920792,11.8800865574205));
#74723=CARTESIAN_POINT('Ctrl Pts',(0.317433356042753,2.40044736685377,11.8999569009432));
#74724=CARTESIAN_POINT('Ctrl Pts',(-0.0807891140929695,2.52954123762685,
11.919827244466));
#74725=CARTESIAN_POINT('Ctrl Pts',(-0.404898570493126,2.26458949963638,
11.9396975879888));
#74726=CARTESIAN_POINT('Ctrl Pts',(-0.357568710428738,1.84864930256659,
11.9595679315116));
#74727=CARTESIAN_POINT('Ctrl Pts',(0.0177817628697346,1.66328915208438,
11.9794382750344));
#74728=CARTESIAN_POINT('Ctrl Pts',(0.376819889503645,1.87855175175136,11.9993086185572));
#74729=CARTESIAN_POINT('Ctrl Pts',(0.39017706691362,2.29696297172976,12.01917896208));
#74730=CARTESIAN_POINT('Ctrl Pts',(0.0455999032414989,2.53468747923341,
12.0390493056028));
#74731=CARTESIAN_POINT('Ctrl Pts',(-0.340808963788434,2.37364540189703,
12.0589196491256));
#74732=CARTESIAN_POINT('Ctrl Pts',(-0.414572003493282,1.96157092177763,
12.0787899926484));
#74733=CARTESIAN_POINT('Ctrl Pts',(-0.108021668874934,1.67648627550999,
12.0986603361712));
#74734=CARTESIAN_POINT('Ctrl Pts',(0.297623841113879,1.77991781527464,12.1185306796939));
#74735=CARTESIAN_POINT('Ctrl Pts',(0.430239994707939,2.17698118427019,12.1384010232167));
#74736=CARTESIAN_POINT('Ctrl Pts',(0.168169525043752,2.50342479673972,12.1582713667395));
#74737=CARTESIAN_POINT('Ctrl Pts',(-0.248173589634581,2.45978107952729,
12.1781417102623));
#74738=CARTESIAN_POINT('Ctrl Pts',(-0.436851221606576,2.08608720161969,
12.1980120537851));
#74739=CARTESIAN_POINT('Ctrl Pts',(-0.224777329678093,1.72515642216957,
12.2178823973079));
#74740=CARTESIAN_POINT('Ctrl Pts',(0.19349916155983,1.70809359503374,12.2377527408307));
#74741=CARTESIAN_POINT('Ctrl Pts',(0.434266514598737,2.05055154121518,12.2576230843535));
#74742=CARTESIAN_POINT('Ctrl Pts',(0.276653460540773,2.4383717165319,12.2774934278763));
#74743=CARTESIAN_POINT('Ctrl Pts',(-0.134751480595642,2.51578190708016,
12.297363771399));
#74744=CARTESIAN_POINT('Ctrl Pts',(-0.422540283043114,2.21176880147776,
12.3172341149218));
#74745=CARTESIAN_POINT('Ctrl Pts',(-0.322705899463725,1.80522303646784,
12.3371044584446));
#74746=CARTESIAN_POINT('Ctrl Pts',(0.0731672144324927,1.66909500523883,
12.3569748019674));
#74747=CARTESIAN_POINT('Ctrl Pts',(0.401919369903692,1.92826364428534,12.3768451454902));
#74748=CARTESIAN_POINT('Ctrl Pts',(0.361965219869607,2.3449770099064,12.396715489013));
#74749=CARTESIAN_POINT('Ctrl Pts',(-0.0100427422798438,2.53695731954669,
12.4165858325358));
#74750=CARTESIAN_POINT('Ctrl Pts',(-0.372837855583444,2.32808877487038,
12.4364561760586));
#74751=CARTESIAN_POINT('Ctrl Pts',(-0.393604993679923,1.90997983073326,
12.4563265195813));
#74752=CARTESIAN_POINT('Ctrl Pts',(-0.0532931345563228,1.66618852298828,
12.4761968631042));
#74753=CARTESIAN_POINT('Ctrl Pts',(0.335907920317574,1.82036018730185,12.4960672066269));
#74754=CARTESIAN_POINT('Ctrl Pts',(0.416959188034086,2.23106331024313,12.5159375501497));
#74755=CARTESIAN_POINT('Ctrl Pts',(0.115507164597036,2.52153368869485,12.5358078936725));
#74756=CARTESIAN_POINT('Ctrl Pts',(-0.291906957477275,2.42530429439879,
12.5556782371953));
#74757=CARTESIAN_POINT('Ctrl Pts',(-0.431536185610004,2.0306524961725,12.5755485807181));
#74758=CARTESIAN_POINT('Ctrl Pts',(-0.175289711792273,1.69961759189781,
12.5954189242409));
#74759=CARTESIAN_POINT('Ctrl Pts',(0.241761209055436,1.73587903991396,12.6152892677637));
#74760=CARTESIAN_POINT('Ctrl Pts',(0.437029133411453,2.10617189821653,12.6351596112864));
#74761=CARTESIAN_POINT('Ctrl Pts',(0.231382324006401,2.47080288013349,12.6550299548093));
#74762=CARTESIAN_POINT('Ctrl Pts',(-0.186526267815305,2.4952726997818,12.674900298332));
#74763=CARTESIAN_POINT('Ctrl Pts',(-0.43332240217526,2.15713362889919,12.6947706418548));
#74764=CARTESIAN_POINT('Ctrl Pts',(-0.282604224056764,1.76658223154287,
12.7146409853776));
#74765=CARTESIAN_POINT('Ctrl Pts',(0.127364856541248,1.6818962460154,12.7345113289004));
#74766=CARTESIAN_POINT('Ctrl Pts',(0.420494020425157,1.98076353508279,12.7543816724232));
#74767=CARTESIAN_POINT('Ctrl Pts',(0.327877165654917,2.38901404813226,12.774252015946));
#74768=CARTESIAN_POINT('Ctrl Pts',(-0.0655223521471513,2.53213351773121,
12.7941223594688));
#74769=CARTESIAN_POINT('Ctrl Pts',(-0.398814031938348,2.27882931447587,
12.8139927029916));
#74770=CARTESIAN_POINT('Ctrl Pts',(-0.366248131012719,1.86147356060571,
12.8338630465143));
#74771=CARTESIAN_POINT('Ctrl Pts',(0.00230056985709836,1.66293334242961,
12.8537333900371));
#74772=CARTESIAN_POINT('Ctrl Pts',(0.368738811230028,1.8653422813367,12.8736037335599));
#74773=CARTESIAN_POINT('Ctrl Pts',(0.396909392261523,2.28301773132501,12.8934740770827));
#74774=CARTESIAN_POINT('Ctrl Pts',(0.0609696407939242,2.53279932849204,
12.9133444206055));
#74775=CARTESIAN_POINT('Ctrl Pts',(-0.330901456925757,2.38554646196952,
12.9332147641282));
#74776=CARTESIAN_POINT('Ctrl Pts',(-0.419215513980957,1.97634359043503,
12.9530851076511));
#74777=CARTESIAN_POINT('Ctrl Pts',(-0.122956412042968,1.68057863998248,
12.9729554511739));
#74778=CARTESIAN_POINT('Ctrl Pts',(0.286098466731769,1.76957568904242,12.9928257946967));
#74779=CARTESIAN_POINT('Ctrl Pts',(0.432696936064204,2.16169205873702,13.0126961382195));
#74780=CARTESIAN_POINT('Ctrl Pts',(0.182354901824367,2.49721436596937,13.0325664817423));
#74781=CARTESIAN_POINT('Ctrl Pts',(-0.235272985115168,2.46834656285919,
13.052436825265));
#74782=CARTESIAN_POINT('Ctrl Pts',(-0.437069830553411,2.10157094461754,
13.0723071687878));
#74783=CARTESIAN_POINT('Ctrl Pts',(-0.237914814564311,1.73335417845672,
13.0921775123106));
#74784=CARTESIAN_POINT('Ctrl Pts',(0.179495052151714,1.70148507794555,13.1120478558334));
#74785=CARTESIAN_POINT('Ctrl Pts',(0.432241878947184,2.03519909097049,13.1319181993562));
#74786=CARTESIAN_POINT('Ctrl Pts',(0.288467100709767,2.42835925974009,13.151788542879));
#74787=CARTESIAN_POINT('Ctrl Pts',(-0.119939810852905,2.52029423330114,
13.1716588864018));
#74788=CARTESIAN_POINT('Ctrl Pts',(-0.418312805424477,2.22666699815582,
13.1915292299246));
#74789=CARTESIAN_POINT('Ctrl Pts',(-0.332951281535073,1.81683901091653,
13.2113995734473));
#74790=CARTESIAN_POINT('Ctrl Pts',(0.0578680000586412,1.66677465713648,
13.2312699169702));
#74791=CARTESIAN_POINT('Ctrl Pts',(0.395562204268459,1.91413177388155,13.2511402604929));
#74792=CARTESIAN_POINT('Ctrl Pts',(0.370457177876832,2.33200500809455,13.2710106040157));
#74793=CARTESIAN_POINT('Ctrl Pts',(0.00536316449256819,2.537031136083,13.2908809475385));
#74794=CARTESIAN_POINT('Ctrl Pts',(-0.364371131947823,2.34116775930325,
13.3107512910613));
#74795=CARTESIAN_POINT('Ctrl Pts',(-0.400388031600374,1.92401443108959,
13.3306216345841));
#74796=CARTESIAN_POINT('Ctrl Pts',(-0.0680109136702867,1.66839569599009,
13.3504919781069));
#74797=CARTESIAN_POINT('Ctrl Pts',(0.193487360962402,1.76186082371239,13.3637388737887));
#74798=CARTESIAN_POINT('Ctrl Pts',(0.275524381335433,1.85359137675596,13.3703623216297));
#74799=CARTESIAN_POINT('Ctrl Pts',(-0.324703122987632,1.98145546592675,
4.34318193730108));
#74800=CARTESIAN_POINT('Ctrl Pts',(-0.285214820824608,1.87327603739136,
4.34980982121868));
#74801=CARTESIAN_POINT('Ctrl Pts',(-0.0903122625737519,1.70146708514356,
4.36306115297722));
#74802=CARTESIAN_POINT('Ctrl Pts',(0.286975972182973,1.80858593652704,4.38293593257671));
#74803=CARTESIAN_POINT('Ctrl Pts',(0.400001189849452,2.18347131865804,4.40280627609948));
#74804=CARTESIAN_POINT('Ctrl Pts',(0.146534207579467,2.48155047238696,4.42267661962228));
#74805=CARTESIAN_POINT('Ctrl Pts',(-0.241591594009944,2.42972928699582,
4.44254696314506));
#74806=CARTESIAN_POINT('Ctrl Pts',(-0.407968932804969,2.07536397308355,
4.46241730666785));
#74807=CARTESIAN_POINT('Ctrl Pts',(-0.200153151725138,1.74363125289821,
4.48228765019064));
#74808=CARTESIAN_POINT('Ctrl Pts',(0.191308522101233,1.73880152376249,4.50215799371343));
#74809=CARTESIAN_POINT('Ctrl Pts',(0.407253731465132,2.06533095703686,4.52202833723622));
#74810=CARTESIAN_POINT('Ctrl Pts',(0.249607880621845,2.42365998281579,4.54189868075901));
#74811=CARTESIAN_POINT('Ctrl Pts',(-0.137023786820888,2.48507739127738,
4.56176902428181));
#74812=CARTESIAN_POINT('Ctrl Pts',(-0.397952412483378,2.19323749418965,
4.58163936780458));
#74813=CARTESIAN_POINT('Ctrl Pts',(-0.293815107395566,1.81586552415182,
4.60150971132738));
#74814=CARTESIAN_POINT('Ctrl Pts',(0.0798581987962179,1.69914792465702,
4.62138005485017));
#74815=CARTESIAN_POINT('Ctrl Pts',(0.380272147308599,1.9501577043663,4.64125039837296));
#74816=CARTESIAN_POINT('Ctrl Pts',(0.331838342430293,2.33862730225961,4.66112074189575));
#74817=CARTESIAN_POINT('Ctrl Pts',(-0.0210120554276185,2.5081888826504,
4.68099108541854));
#74818=CARTESIAN_POINT('Ctrl Pts',(-0.354586706485803,2.30329270914637,
4.70086142894133));
#74819=CARTESIAN_POINT('Ctrl Pts',(-0.362876351097746,1.91190316324567,
4.72073177246412));
#74820=CARTESIAN_POINT('Ctrl Pts',(-0.0382763322007111,1.69306685153467,
4.7406021159869));
#74821=CARTESIAN_POINT('Ctrl Pts',(0.321437004131683,1.84753630794944,4.76047245950971));
#74822=CARTESIAN_POINT('Ctrl Pts',(0.386275652248465,2.23360683025069,4.78034280303248));
#74823=CARTESIAN_POINT('Ctrl Pts',(0.0967589743544941,2.49711127562884,
4.80021314655528));
#74824=CARTESIAN_POINT('Ctrl Pts',(-0.28152088905393,2.39632018696635,4.82008349007806));
#74825=CARTESIAN_POINT('Ctrl Pts',(-0.401543662836625,2.02369566735683,
4.83995383360086));
#74826=CARTESIAN_POINT('Ctrl Pts',(-0.153204790954587,1.72106998492393,
4.85982417712364));
#74827=CARTESIAN_POINT('Ctrl Pts',(0.235678619551842,1.76606100472576,4.87969452064644));
#74828=CARTESIAN_POINT('Ctrl Pts',(0.408358981432492,2.11739559096851,4.89956486416922));
#74829=CARTESIAN_POINT('Ctrl Pts',(0.206425570869757,2.45277209071125,4.91943520769201));
#74830=CARTESIAN_POINT('Ctrl Pts',(-0.184875198644271,2.46452822280067,
4.9393055512148));
#74831=CARTESIAN_POINT('Ctrl Pts',(-0.406578141897051,2.14187933651161,
4.95917589473759));
#74832=CARTESIAN_POINT('Ctrl Pts',(-0.255300990570369,1.78081186032747,
4.97904623826038));
#74833=CARTESIAN_POINT('Ctrl Pts',(0.130180063510712,1.7125560487528,4.99891658178317));
#74834=CARTESIAN_POINT('Ctrl Pts',(0.396238631737338,1.99972731671569,5.01878692530596));
#74835=CARTESIAN_POINT('Ctrl Pts',(0.298802198362976,2.37888512069913,5.03865726882875));
#74836=CARTESIAN_POINT('Ctrl Pts',(-0.0727445737629762,2.50220379322174,
5.05852761235154));
#74837=CARTESIAN_POINT('Ctrl Pts',(-0.377558102741037,2.25655524056561,
5.07839795587433));
#74838=CARTESIAN_POINT('Ctrl Pts',(-0.336013472348416,1.86728856776192,
5.09826829939711));
#74839=CARTESIAN_POINT('Ctrl Pts',(0.013777774820227,1.69150295323597,5.11813864291991));
#74840=CARTESIAN_POINT('Ctrl Pts',(0.350929789266008,1.89045776726478,5.13800898644269));
#74841=CARTESIAN_POINT('Ctrl Pts',(0.366151496836993,2.28163905322912,5.15787932996549));
#74842=CARTESIAN_POINT('Ctrl Pts',(0.045479053085185,2.50619123577992,5.17774967348827));
#74843=CARTESIAN_POINT('Ctrl Pts',(-0.316914230458285,2.35811825744603,
5.19762001701106));
#74844=CARTESIAN_POINT('Ctrl Pts',(-0.388581851532883,1.97325691753307,
5.21749036053385));
#74845=CARTESIAN_POINT('Ctrl Pts',(-0.103778524468258,1.70466510127092,
5.23736070405664));
#74846=CARTESIAN_POINT('Ctrl Pts',(0.276227470625653,1.79873923460613,5.25723104757944));
#74847=CARTESIAN_POINT('Ctrl Pts',(0.40283236639495,2.16917910724046,5.27710139110222));
#74848=CARTESIAN_POINT('Ctrl Pts',(0.159893406671488,2.47615656686668,5.29697173462502));
#74849=CARTESIAN_POINT('Ctrl Pts',(-0.229725986151337,2.43806158548516,
5.31684207814779));
#74850=CARTESIAN_POINT('Ctrl Pts',(-0.408603061049272,2.08984112235003,
5.33671242167059));
#74851=CARTESIAN_POINT('Ctrl Pts',(-0.212642453718247,1.75094004645244,
5.35658276519338));
#74852=CARTESIAN_POINT('Ctrl Pts',(0.178388656243237,1.73225395771311,5.37645310871617));
#74853=CARTESIAN_POINT('Ctrl Pts',(0.405772459524144,2.05092479866909,5.39632345223896));
#74854=CARTESIAN_POINT('Ctrl Pts',(0.260915272123794,2.41461545586081,5.41619379576174));
#74855=CARTESIAN_POINT('Ctrl Pts',(-0.123296157043305,2.48968926332694,
5.43606413928454));
#74856=CARTESIAN_POINT('Ctrl Pts',(-0.394400147379255,2.2072762230933,5.45593448280733));
#74857=CARTESIAN_POINT('Ctrl Pts',(-0.303695695226391,1.82645185251057,
5.4758048263301));
#74858=CARTESIAN_POINT('Ctrl Pts',(0.0656082128611597,1.69657066703188,
5.49567516985291));
#74859=CARTESIAN_POINT('Ctrl Pts',(0.374725517400243,1.93678097260717,5.51554551337569));
#74860=CARTESIAN_POINT('Ctrl Pts',(0.340083173997246,2.32672251555128,5.53541585689848));
#74861=CARTESIAN_POINT('Ctrl Pts',(-0.00653918340477464,2.50867701596045,
5.55528620042128));
#74862=CARTESIAN_POINT('Ctrl Pts',(-0.347162730262346,2.31572599057771,
5.57515654394406));
#74863=CARTESIAN_POINT('Ctrl Pts',(-0.369311734042224,1.92487573728159,
5.59502688746686));
#74864=CARTESIAN_POINT('Ctrl Pts',(-0.0526674990909465,1.69467815401406,
5.61489723098964));
#74865=CARTESIAN_POINT('Ctrl Pts',(0.31229199624372,1.83630818485199,5.63476757451243));
#74866=CARTESIAN_POINT('Ctrl Pts',(0.390766099741013,2.21983955768918,5.65463791803522));
#74867=CARTESIAN_POINT('Ctrl Pts',(0.110765504726666,2.49343445102912,5.67450826155801));
#74868=CARTESIAN_POINT('Ctrl Pts',(-0.270847361512589,2.40610679681381,
5.6943786050808));
#74869=CARTESIAN_POINT('Ctrl Pts',(-0.403994646102744,2.03796782919919,
5.71424894860358));
#74870=CARTESIAN_POINT('Ctrl Pts',(-0.166531841798338,1.72673493337684,
5.73411929212638));
#74871=CARTESIAN_POINT('Ctrl Pts',(0.223701256092982,1.75792192073101,5.75398963564917));
#74872=CARTESIAN_POINT('Ctrl Pts',(0.408718905695017,2.1029189760892,5.77385997917195));
#74873=CARTESIAN_POINT('Ctrl Pts',(0.218792601376446,2.44523826826826,5.79373032269475));
#74874=CARTESIAN_POINT('Ctrl Pts',(-0.171846128781984,2.47084844925736,
5.81360066621753));
#74875=CARTESIAN_POINT('Ctrl Pts',(-0.404839430520849,2.1562556645103,5.83347100974033));
#74876=CARTESIAN_POINT('Ctrl Pts',(-0.266447668668554,1.79005596609221,
5.85334135326312));
#74877=CARTESIAN_POINT('Ctrl Pts',(0.116373555612529,1.70818772371448,5.8732116967859));
#74878=CARTESIAN_POINT('Ctrl Pts',(0.392437885448118,1.98575390440391,5.8930820403087));
#74879=CARTESIAN_POINT('Ctrl Pts',(0.308493880978865,2.36812532460127,5.91295238383148));
#74880=CARTESIAN_POINT('Ctrl Pts',(-0.0584512616389577,2.50452826144382,
5.93282272735428));
#74881=CARTESIAN_POINT('Ctrl Pts',(-0.371775329123761,2.26983158996152,
5.95269307087706));
#74882=CARTESIAN_POINT('Ctrl Pts',(-0.344046144778287,1.87933755517274,
5.97256341439985));
#74883=CARTESIAN_POINT('Ctrl Pts',(-0.00070146025194062,1.69127127303375,
5.99243375792264));
#74884=CARTESIAN_POINT('Ctrl Pts',(0.343286718560372,1.87815795449466,6.01230410144543));
#74885=CARTESIAN_POINT('Ctrl Pts',(0.372356067360204,2.26855451163937,6.0321744449682));
#74886=CARTESIAN_POINT('Ctrl Pts',(0.059839416058191,2.50432525097965,6.05204478849101));
#74887=CARTESIAN_POINT('Ctrl Pts',(-0.307571753076327,2.3691826164586,6.0719151320138));
#74888=CARTESIAN_POINT('Ctrl Pts',(-0.392827710876478,1.98710157724091,
6.09178547553659));
#74889=CARTESIAN_POINT('Ctrl Pts',(-0.117717722611208,1.70858947117231,
6.11165581905938));
#74890=CARTESIAN_POINT('Ctrl Pts',(0.265382250329029,1.78914323957127,6.13152616258216));
#74891=CARTESIAN_POINT('Ctrl Pts',(0.405030137123385,2.15486576633707,6.15139650610496));
#74892=CARTESIAN_POINT('Ctrl Pts',(0.173118012981109,2.47025642178822,6.17126684962775));
#74893=CARTESIAN_POINT('Ctrl Pts',(-0.217606320182031,2.44598721610888,
6.19113719315053));
#74894=CARTESIAN_POINT('Ctrl Pts',(-0.408706479003584,2.10432184155586,
6.21100753667333));
#74895=CARTESIAN_POINT('Ctrl Pts',(-0.224874083702182,1.75869176574093,
6.23087788019611));
#74896=CARTESIAN_POINT('Ctrl Pts',(0.165249669553886,1.72616552993835,6.25074822371891));
#74897=CARTESIAN_POINT('Ctrl Pts',(0.403779347705335,2.03658152744984,6.27061856724169));
#74898=CARTESIAN_POINT('Ctrl Pts',(0.271896443931615,2.40517533988068,6.29048891076448));
#74899=CARTESIAN_POINT('Ctrl Pts',(-0.109414431790982,2.49381232384195,
6.31035925428728));
#74900=CARTESIAN_POINT('Ctrl Pts',(-0.390352461775193,2.22118011338494,
6.33022959781006));
#74901=CARTESIAN_POINT('Ctrl Pts',(-0.313195249769681,1.83738164608,6.35009994133285));
#74902=CARTESIAN_POINT('Ctrl Pts',(0.0512759662164159,1.69449976623618,
6.36997028485564));
#74903=CARTESIAN_POINT('Ctrl Pts',(0.368708463791405,1.92360914699871,6.38984062837843));
#74904=CARTESIAN_POINT('Ctrl Pts',(0.347901140962541,2.31453312194368,6.40971097190122));
#74905=CARTESIAN_POINT('Ctrl Pts',(0.00794188376409148,2.5086521635526,
6.42958131542401));
#74906=CARTESIAN_POINT('Ctrl Pts',(-0.339302970598069,2.32788847807045,
6.4494516589468));
#74907=CARTESIAN_POINT('Ctrl Pts',(-0.375283541364848,1.9380681381735,6.46932200246958));
#74908=CARTESIAN_POINT('Ctrl Pts',(-0.0669925531701256,1.69679823647001,
6.48919234599238));
#74909=CARTESIAN_POINT('Ctrl Pts',(0.302754982345627,1.82541106184181,6.50906268951516));
#74910=CARTESIAN_POINT('Ctrl Pts',(0.394766037928299,2.20592185606538,6.52893303303795));
#74911=CARTESIAN_POINT('Ctrl Pts',(0.124632996254909,2.48926376730755,6.54880337656074));
#74912=CARTESIAN_POINT('Ctrl Pts',(-0.259833852232052,2.41550916552169,
6.56867372008354));
#74913=CARTESIAN_POINT('Ctrl Pts',(-0.405938514480912,2.05231785706397,
6.58854406360632));
#74914=CARTESIAN_POINT('Ctrl Pts',(-0.179649853232024,1.73286842341246,
6.60841440712912));
#74915=CARTESIAN_POINT('Ctrl Pts',(0.21144309123819,1.75021223082906,6.6282847506519));
#74916=CARTESIAN_POINT('Ctrl Pts',(0.408565784874935,2.08843869715522,6.64815509417468));
#74917=CARTESIAN_POINT('Ctrl Pts',(0.230884992097985,2.4372710849122,6.66802543769748));
#74918=CARTESIAN_POINT('Ctrl Pts',(-0.158601348775496,2.47670316757433,
6.68789578122028));
#74919=CARTESIAN_POINT('Ctrl Pts',(-0.402592543771387,2.17056137749241,
6.70776612474306));
#74920=CARTESIAN_POINT('Ctrl Pts',(-0.277259887882735,1.79968912962533,
6.72763646826585));
#74921=CARTESIAN_POINT('Ctrl Pts',(0.102420969612983,1.70431122169376,6.74750681178864));
#74922=CARTESIAN_POINT('Ctrl Pts',(0.388144530844729,1.97192389969527,6.76737715531141));
#74923=CARTESIAN_POINT('Ctrl Pts',(0.317798326132794,2.35702896373975,6.78724749883422));
#74924=CARTESIAN_POINT('Ctrl Pts',(-0.0440845784706122,2.50634494488675,
6.807117842357));
#74925=CARTESIAN_POINT('Ctrl Pts',(-0.365525883900656,2.28289475796913,
6.8269881858798));
#74926=CARTESIAN_POINT('Ctrl Pts',(-0.351646952707478,1.89166352948779,
6.84685852940258));
#74927=CARTESIAN_POINT('Ctrl Pts',(-0.0151798148149533,1.69155265025205,
6.86672887292538));
#74928=CARTESIAN_POINT('Ctrl Pts',(0.335212736625109,1.86613660932448,6.88659921644816));
#74929=CARTESIAN_POINT('Ctrl Pts',(0.378093237304912,2.25525839171599,6.90646955997095));
#74930=CARTESIAN_POINT('Ctrl Pts',(0.0741246655037585,2.50195173622948,
6.92633990349375));
#74931=CARTESIAN_POINT('Ctrl Pts',(-0.297843195735107,2.37990908354007,
6.94621024701653));
#74932=CARTESIAN_POINT('Ctrl Pts',(-0.396580472576683,2.00108795288341,
6.96608059053932));
#74933=CARTESIAN_POINT('Ctrl Pts',(-0.131509155385276,1.71300515979694,
6.98595093406212));
#74934=CARTESIAN_POINT('Ctrl Pts',(0.254203908517277,1.77993744800668,7.0058212775849));
#74935=CARTESIAN_POINT('Ctrl Pts',(0.406719493092408,2.1404835550884,7.0256916211077));
#74936=CARTESIAN_POINT('Ctrl Pts',(0.186125312614382,2.46389151171488,7.04556196463048));
#74937=CARTESIAN_POINT('Ctrl Pts',(-0.205213503514097,2.4534785456989,7.06543230815328));
#74938=CARTESIAN_POINT('Ctrl Pts',(-0.408296867464171,2.11879713576282,
7.08530265167605));
#74939=CARTESIAN_POINT('Ctrl Pts',(-0.236823440115126,1.76687191276331,
7.10517299519885));
#74940=CARTESIAN_POINT('Ctrl Pts',(0.151903252939481,1.72054635850957,7.12504333872164));
#74941=CARTESIAN_POINT('Ctrl Pts',(0.401279391182633,2.0223178623747,7.14491368224442));
#74942=CARTESIAN_POINT('Ctrl Pts',(0.282536317271847,2.39535215204295,7.16478402576722));
#74943=CARTESIAN_POINT('Ctrl Pts',(-0.0953953638895205,2.49744105077651,
7.18465436928999));
#74944=CARTESIAN_POINT('Ctrl Pts',(-0.38581478558834,2.23493189213586,7.20452471281281));
#74945=CARTESIAN_POINT('Ctrl Pts',(-0.322301665450036,1.84864109177896,
7.22439505633558));
#74946=CARTESIAN_POINT('Ctrl Pts',(0.0368793553290216,1.69293787028949,
7.24426539985838));
#74947=CARTESIAN_POINT('Ctrl Pts',(0.36222858826457,1.91065873630452,7.26413574338117));
#74948=CARTESIAN_POINT('Ctrl Pts',(0.355282404436738,2.3020744352747,7.28400608690396));
#74949=CARTESIAN_POINT('Ctrl Pts',(0.0224129818700309,2.50811434983058,
7.30387643042674));
#74950=CARTESIAN_POINT('Ctrl Pts',(-0.331017300310477,2.33976490816863,
7.32374677394954));
#74951=CARTESIAN_POINT('Ctrl Pts',(-0.380784273392315,1.95146380430673,
7.34361711747232));
#74952=CARTESIAN_POINT('Ctrl Pts',(-0.0812335147344956,1.69942443861635,
7.36348746099511));
#74953=CARTESIAN_POINT('Ctrl Pts',(0.29283793474781,1.81485861705711,7.38335780451791));
#74954=CARTESIAN_POINT('Ctrl Pts',(0.398270445383918,2.19187119585397,7.40322814804069));
#74955=CARTESIAN_POINT('Ctrl Pts',(0.138344042005423,2.48460445958874,7.42309849156349));
#74956=CARTESIAN_POINT('Ctrl Pts',(-0.248494186072408,2.42451549082001,
7.44296883508627));
#74957=CARTESIAN_POINT('Ctrl Pts',(-0.407372827857467,2.06672773801869,
7.46283917860906));
#74958=CARTESIAN_POINT('Ctrl Pts',(-0.19254235888592,1.73946275597577,7.48270952213185));
#74959=CARTESIAN_POINT('Ctrl Pts',(0.198919512088243,1.74294161261145,7.50257986565464));
#74960=CARTESIAN_POINT('Ctrl Pts',(0.407899811167672,2.07397293056604,7.52245020917743));
#74961=CARTESIAN_POINT('Ctrl Pts',(0.242687564045679,2.42888054146076,7.54232055270022));
#74962=CARTESIAN_POINT('Ctrl Pts',(-0.145157484159772,2.48208502860796,
7.56219089622301));
#74963=CARTESIAN_POINT('Ctrl Pts',(-0.399840302055658,2.184778518187,7.58206123974579));
#74964=CARTESIAN_POINT('Ctrl Pts',(-0.287724076157312,1.80969925888251,
7.60193158326859));
#74965=CARTESIAN_POINT('Ctrl Pts',(0.0883398195194317,1.70093140867613,
7.62180192679138));
#74966=CARTESIAN_POINT('Ctrl Pts',(0.38336395716755,1.9582546627265,7.64167227031415));
#74967=CARTESIAN_POINT('Ctrl Pts',(0.326703854404464,2.34560996684013,7.66154261383696));
#74968=CARTESIAN_POINT('Ctrl Pts',(-0.0296625580611567,2.5076515631556,
7.68141295735974));
#74969=CARTESIAN_POINT('Ctrl Pts',(-0.358817611698299,2.29572834702483,
7.70128330088253));
#74970=CARTESIAN_POINT('Ctrl Pts',(-0.358806355209093,1.9042510185071,7.72115364440532));
#74971=CARTESIAN_POINT('Ctrl Pts',(-0.0296391148899432,1.69234673169165,
7.74102398792811));
#74972=CARTESIAN_POINT('Ctrl Pts',(0.32671797833959,1.85440882156797,7.76089433145089));
#74973=CARTESIAN_POINT('Ctrl Pts',(0.383355805078912,2.24176738343583,7.78076467497369));
#74974=CARTESIAN_POINT('Ctrl Pts',(0.0883168698385477,2.4990736708878,7.80063501849648));
#74975=CARTESIAN_POINT('Ctrl Pts',(-0.287740770222548,2.39028419427463,
7.82050536201926));
#74976=CARTESIAN_POINT('Ctrl Pts',(-0.399835425973084,2.01519848803905,
7.84037570554206));
#74977=CARTESIAN_POINT('Ctrl Pts',(-0.14513551107133,1.71790662434425,7.86024604906485));
#74978=CARTESIAN_POINT('Ctrl Pts',(0.242706476822712,1.77113341549764,7.88011639258762));
#74979=CARTESIAN_POINT('Ctrl Pts',(0.407898313735106,2.12605052678927,7.89998673611043));
#74980=CARTESIAN_POINT('Ctrl Pts',(0.198898978136607,2.45706982621072,7.91985707963321));
#74981=CARTESIAN_POINT('Ctrl Pts',(-0.19256309225145,2.46052617075117,7.93972742315602));
#74982=CARTESIAN_POINT('Ctrl Pts',(-0.407374740596605,2.13324883483357,
7.95959776667879));
#74983=CARTESIAN_POINT('Ctrl Pts',(-0.248475523507394,1.7754702193763,7.97946811020159));
#74984=CARTESIAN_POINT('Ctrl Pts',(0.138366159511869,1.71540349690113,7.99933845372437));
#74985=CARTESIAN_POINT('Ctrl Pts',(0.398275728030659,2.00815170793318,8.01920879724717));
#74986=CARTESIAN_POINT('Ctrl Pts',(0.292821536425625,2.38515822292067,8.03907914076994));
#74987=CARTESIAN_POINT('Ctrl Pts',(-0.0812565507974271,2.500570889165,8.05894948429274));
#74988=CARTESIAN_POINT('Ctrl Pts',(-0.380792814744337,2.24851429740273,
8.07881982781553));
#74989=CARTESIAN_POINT('Ctrl Pts',(-0.331003511423903,1.86021605616934,
8.09869017133833));
#74990=CARTESIAN_POINT('Ctrl Pts',(0.0224364515689504,1.69188693976432,
8.11856051486111));
#74991=CARTESIAN_POINT('Ctrl Pts',(0.35529402469436,1.89794599654937,8.13843085838391));
#74992=CARTESIAN_POINT('Ctrl Pts',(0.362217699076477,2.28936209433169,8.15830120190667));
#74993=CARTESIAN_POINT('Ctrl Pts',(0.0368559460428643,2.50706424988597,
8.17817154542949));
#74994=CARTESIAN_POINT('Ctrl Pts',(-0.3223161200011,2.3513403729634,8.19804188895226));
#74995=CARTESIAN_POINT('Ctrl Pts',(-0.385807025321515,1.96504592074892,
8.21791223247506));
#74996=CARTESIAN_POINT('Ctrl Pts',(-0.0953725077931551,1.70255346390843,
8.23778257599785));
#74997=CARTESIAN_POINT('Ctrl Pts',(0.282553301840913,1.80466409647193,8.25765291952063));
#74998=CARTESIAN_POINT('Ctrl Pts',(0.401274923194525,2.17770521416978,8.27752326304343));
#74999=CARTESIAN_POINT('Ctrl Pts',(0.151881431165022,2.47946237647651,8.29739360656621));
#75000=CARTESIAN_POINT('Ctrl Pts',(-0.236842597168632,2.43311446750383,
8.317263950089));
#75001=CARTESIAN_POINT('Ctrl Pts',(-0.408295785808135,2.08117938403611,
8.3371342936118));
#75002=CARTESIAN_POINT('Ctrl Pts',(-0.205193175420671,1.74650965351976,
8.35700463713457));
#75003=CARTESIAN_POINT('Ctrl Pts',(0.186146238886892,1.73611919253387,8.37687498065739));
#75004=CARTESIAN_POINT('Ctrl Pts',(0.406721820537833,2.05953983449946,8.39674532418016));
#75005=CARTESIAN_POINT('Ctrl Pts',(0.254185502021292,2.42007717015764,8.41661566770295));
#75006=CARTESIAN_POINT('Ctrl Pts',(-0.131531410368423,2.48698727676816,
8.43648601122574));
#75007=CARTESIAN_POINT('Ctrl Pts',(-0.396586160129697,2.19888924050433,
8.45635635474853));
#75008=CARTESIAN_POINT('Ctrl Pts',(-0.297827098302388,1.82007378863221,
8.47622669827132));
#75009=CARTESIAN_POINT('Ctrl Pts',(0.0741477807191584,1.69805252717754,
8.49609704179411));
#75010=CARTESIAN_POINT('Ctrl Pts',(0.378102165239712,1.94476335183023,8.5159673853169));
#75011=CARTESIAN_POINT('Ctrl Pts',(0.335199287114567,2.3338826676174,8.53583772883967));
#75012=CARTESIAN_POINT('Ctrl Pts',(-0.0152033036759094,2.50844647611563,
8.55570807236248));
#75013=CARTESIAN_POINT('Ctrl Pts',(-0.351658933086634,2.30831624774441,
8.57557841588528));
#75014=CARTESIAN_POINT('Ctrl Pts',(-0.36551536543112,1.91708422176396,8.59544875940805));
#75015=CARTESIAN_POINT('Ctrl Pts',(-0.0440612104162264,1.69365252058048,
8.61531910293085));
#75016=CARTESIAN_POINT('Ctrl Pts',(0.317813106763408,1.84298931255037,8.63518944645363));
#75017=CARTESIAN_POINT('Ctrl Pts',(0.38813716483518,2.22809842140966,8.65505978997641));
#75018=CARTESIAN_POINT('Ctrl Pts',(0.102398214274245,2.49569466765094,8.67493013349922));
#75019=CARTESIAN_POINT('Ctrl Pts',(-0.277277157625239,2.40029492528715,
8.69480047702201));
#75020=CARTESIAN_POINT('Ctrl Pts',(-0.402588485279962,2.0294154704349,8.71467082054478));
#75021=CARTESIAN_POINT('Ctrl Pts',(-0.15857968516352,1.72328771224265,8.73454116406759));
#75022=CARTESIAN_POINT('Ctrl Pts',(0.230904387415763,1.76274219332076,8.75441150759036));
#75023=CARTESIAN_POINT('Ctrl Pts',(0.408565119334887,2.11158479852265,8.77428185111318));
#75024=CARTESIAN_POINT('Ctrl Pts',(0.211422975382705,2.44979992820792,8.79415219463594));
#75025=CARTESIAN_POINT('Ctrl Pts',(-0.179670965844065,2.4671212447225,8.81402253815874));
#75026=CARTESIAN_POINT('Ctrl Pts',(-0.405941255902183,2.14765879824859,
8.83389288168152));
#75027=CARTESIAN_POINT('Ctrl Pts',(-0.259815707581749,1.7844758925411,8.85376322520432));
#75028=CARTESIAN_POINT('Ctrl Pts',(0.124655381730304,1.7107434006987,8.87363356872711));
#75029=CARTESIAN_POINT('Ctrl Pts',(0.394772128602621,1.99410084621444,8.8935039122499));
#75030=CARTESIAN_POINT('Ctrl Pts',(0.302739190854349,2.37460634846047,8.91337425577268));
#75031=CARTESIAN_POINT('Ctrl Pts',(-0.0670157402835653,2.5031979102726,
8.93324459929548));
#75032=CARTESIAN_POINT('Ctrl Pts',(-0.375292853080517,2.26191027984853,
8.95311494281827));
#75033=CARTESIAN_POINT('Ctrl Pts',(-0.339289864684512,1.87209200975764,
8.97298528634106));
#75034=CARTESIAN_POINT('Ctrl Pts',(0.00796538441539088,1.69134829384296,
8.99285562986384));
#75035=CARTESIAN_POINT('Ctrl Pts',(0.347913477703343,1.88548688542118,9.01272597338664));
#75036=CARTESIAN_POINT('Ctrl Pts',(0.368698319341517,2.27641205630196,9.03259631690941));
#75037=CARTESIAN_POINT('Ctrl Pts',(0.0512526467275652,2.50550318185849,
9.05246666043221));
#75038=CARTESIAN_POINT('Ctrl Pts',(-0.313210351841129,2.36260034233317,
9.07233700395502));
#75039=CARTESIAN_POINT('Ctrl Pts',(-0.390345492334655,1.97879743852559,
9.09220734747776));
#75040=CARTESIAN_POINT('Ctrl Pts',(-0.109391784351346,1.70618138463199,
9.1120776910006));
#75041=CARTESIAN_POINT('Ctrl Pts',(0.271913993427649,1.79484029677533,9.13194803452336));
#75042=CARTESIAN_POINT('Ctrl Pts',(0.403775699984309,2.16344169288507,9.15181837804616));
#75043=CARTESIAN_POINT('Ctrl Pts',(0.165228170903243,2.47384397257935,9.17168872156895));
#75044=CARTESIAN_POINT('Ctrl Pts',(-0.224893711197254,2.44129530169322,
9.19155906509174));
#75045=CARTESIAN_POINT('Ctrl Pts',(-0.408706229788395,2.0956546546633,9.21142940861454));
#75046=CARTESIAN_POINT('Ctrl Pts',(-0.217586422877593,1.75400027041444,
9.23129975213731));
#75047=CARTESIAN_POINT('Ctrl Pts',(0.173139305306751,1.72975353445058,9.25117009566012));
#75048=CARTESIAN_POINT('Ctrl Pts',(0.405033291660138,2.0451575261235,9.27104043918287));
#75049=CARTESIAN_POINT('Ctrl Pts',(0.265364373218883,2.41087202144949,9.2909107827057));
#75050=CARTESIAN_POINT('Ctrl Pts',(-0.11774023155345,2.49140375849969,9.31078112622846));
#75051=CARTESIAN_POINT('Ctrl Pts',(-0.392834202760616,2.21287583193656,
9.33065146975127));
#75052=CARTESIAN_POINT('Ctrl Pts',(-0.307556272482463,1.83079969622856,
9.35052181327406));
#75053=CARTESIAN_POINT('Ctrl Pts',(0.0598626677926879,1.69567819091881,
9.37039215679684));
#75054=CARTESIAN_POINT('Ctrl Pts',(0.372365759934363,1.93146690199714,9.39026250031962));
#75055=CARTESIAN_POINT('Ctrl Pts',(0.343273960356936,2.32186178678359,9.41013284384242));
#75056=CARTESIAN_POINT('Ctrl Pts',(-0.000724965318195603,2.508728685951,
9.43000318736521));
#75057=CARTESIAN_POINT('Ctrl Pts',(-0.344058834008994,2.3206426591444,9.44987353088801));
#75058=CARTESIAN_POINT('Ctrl Pts',(-0.371765561877234,1.93014703035847,
9.46974387441079));
#75059=CARTESIAN_POINT('Ctrl Pts',(-0.05842799803419,1.69546837782485,9.48961421793357));
#75060=CARTESIAN_POINT('Ctrl Pts',(0.308509299751549,1.83189241662954,9.50948456145638));
#75061=CARTESIAN_POINT('Ctrl Pts',(0.392431314763861,2.21426866362503,9.52935490497914));
#75062=CARTESIAN_POINT('Ctrl Pts',(0.116351023179618,2.49181896801839,9.54922524850196));
#75063=CARTESIAN_POINT('Ctrl Pts',(-0.266465492410433,2.40992871059069,
9.56909559202474));
#75064=CARTESIAN_POINT('Ctrl Pts',(-0.40483619471501,2.04372105417998,9.58896593554751));
#75065=CARTESIAN_POINT('Ctrl Pts',(-0.171824801839765,1.72914166887251,
9.60883627907033));
#75066=CARTESIAN_POINT('Ctrl Pts',(0.218812454888957,1.75477431457174,9.62870662259308));
#75067=CARTESIAN_POINT('Ctrl Pts',(0.408719072882905,2.09710452841824,9.64857696611591));
#75068=CARTESIAN_POINT('Ctrl Pts',(0.223681583584119,2.44209094325814,9.66844730963867));
#75069=CARTESIAN_POINT('Ctrl Pts',(-0.166553307155238,2.47325548913525,
9.68831765316147));
#75070=CARTESIAN_POINT('Ctrl Pts',(-0.403998212764973,2.16200893787714,
9.70818799668428));
#75071=CARTESIAN_POINT('Ctrl Pts',(-0.270829757553105,1.79387762787135,
9.72805834020705));
#75072=CARTESIAN_POINT('Ctrl Pts',(0.1107881300716,1.70657191949585,9.74792868372986));
#75073=CARTESIAN_POINT('Ctrl Pts',(0.390772990797583,1.98018291458621,9.76779902725263));
#75074=CARTESIAN_POINT('Ctrl Pts',(0.31227683140565,2.36370977392047,9.78766937077542));
#75075=CARTESIAN_POINT('Ctrl Pts',(-0.0526908081492277,2.5053188165266,
9.80753971429822));
#75076=CARTESIAN_POINT('Ctrl Pts',(-0.369321804432989,2.2751030241438,9.82741005782098));
#75077=CARTESIAN_POINT('Ctrl Pts',(-0.347150323773027,1.88425404523324,
9.84728040134381));
#75078=CARTESIAN_POINT('Ctrl Pts',(-0.00651568130033314,1.69132260866163,
9.86715074486657));
#75079=CARTESIAN_POINT('Ctrl Pts',(0.34009621173551,1.87329704224007,9.88702108838937));
#75080=CARTESIAN_POINT('Ctrl Pts',(0.374716130422396,2.26324057674245,9.90689143191215));
#75081=CARTESIAN_POINT('Ctrl Pts',(0.0655850124414589,2.50343310528141,
9.92676177543496));
#75082=CARTESIAN_POINT('Ctrl Pts',(-0.303711425861324,2.3735306821825,9.94663211895772));
#75083=CARTESIAN_POINT('Ctrl Pts',(-0.394393977513401,1.99270109602099,
9.96650246248053));
#75084=CARTESIAN_POINT('Ctrl Pts',(-0.123273746688637,1.71030364683348,
9.98637280600333));
#75085=CARTESIAN_POINT('Ctrl Pts',(0.260933364517766,1.78539954930836,10.0062431495261));
#75086=CARTESIAN_POINT('Ctrl Pts',(0.405769636649003,2.14909853630889,10.0261134930489));
#75087=CARTESIAN_POINT('Ctrl Pts',(0.178367507702632,2.46775630040815,10.0459838365717));
#75088=CARTESIAN_POINT('Ctrl Pts',(-0.212662527017431,2.44904772438236,
10.0658541800945));
#75089=CARTESIAN_POINT('Ctrl Pts',(-0.408603644587765,2.11013537979253,
10.0857245236173));
#75090=CARTESIAN_POINT('Ctrl Pts',(-0.229706544612006,1.76192520405042,
10.1055948671401));
#75091=CARTESIAN_POINT('Ctrl Pts',(0.159915038323031,1.72385262886458,10.1254652106629));
#75092=CARTESIAN_POINT('Ctrl Pts',(0.402836344063299,2.03084405885495,10.1453355541856));
#75093=CARTESIAN_POINT('Ctrl Pts',(0.27621014534161,2.40127665011465,10.1652058977085));
#75094=CARTESIAN_POINT('Ctrl Pts',(-0.103801259115205,2.49532893000645,
10.1850762412312));
#75095=CARTESIAN_POINT('Ctrl Pts',(-0.388589139599207,2.22672073579131,
10.204946584754));
#75096=CARTESIAN_POINT('Ctrl Pts',(-0.316899386135312,1.84186351795803,
10.2248169282768));
#75097=CARTESIAN_POINT('Ctrl Pts',(0.0455024121519973,1.69381138028954,
10.2446872717996));
#75098=CARTESIAN_POINT('Ctrl Pts',(0.366161941883896,1.91838200361815,10.2645576153224));
#75099=CARTESIAN_POINT('Ctrl Pts',(0.350917738384428,2.30956241356956,10.2844279588452));
#75100=CARTESIAN_POINT('Ctrl Pts',(0.0137542830534484,2.50849783841733,
10.304298302368));
#75101=CARTESIAN_POINT('Ctrl Pts',(-0.336026854502516,2.33269210847617,
10.3241686458908));
#75102=CARTESIAN_POINT('Ctrl Pts',(-0.377549098977838,1.94342304717818,
10.3440389894135));
#75103=CARTESIAN_POINT('Ctrl Pts',(-0.0727214438095559,1.69779202406691,
10.3639093329363));
#75104=CARTESIAN_POINT('Ctrl Pts',(0.298818235923393,1.82113206320271,10.3837796764591));
#75105=CARTESIAN_POINT('Ctrl Pts',(0.396232864626036,2.2002954699086,10.4036500199819));
#75106=CARTESIAN_POINT('Ctrl Pts',(0.130157782267859,2.48745143696863,10.4235203635047));
#75107=CARTESIAN_POINT('Ctrl Pts',(-0.255319345939072,2.41917345736008,
10.4433907070275));
#75108=CARTESIAN_POINT('Ctrl Pts',(-0.406575732837171,2.05809728216624,
10.4632610505503));
#75109=CARTESIAN_POINT('Ctrl Pts',(-0.184854235145107,1.73546114604495,
10.4831313940731));
#75110=CARTESIAN_POINT('Ctrl Pts',(0.206445857660923,1.74723978094379,10.5030017375959));
#75111=CARTESIAN_POINT('Ctrl Pts',(0.408359981128703,2.08262789285941,10.5228720811187));
#75112=CARTESIAN_POINT('Ctrl Pts',(0.23565941510231,2.43395254807768,10.5427424246414));
#75113=CARTESIAN_POINT('Ctrl Pts',(-0.153226582148086,2.47892120396879,
10.5626127681642));
#75114=CARTESIAN_POINT('Ctrl Pts',(-0.401548050193132,2.17628124068232,
10.582483111687));
#75115=CARTESIAN_POINT('Ctrl Pts',(-0.281503848016732,1.803663623823,10.6023534552098));
#75116=CARTESIAN_POINT('Ctrl Pts',(0.096781811426683,1.70289428955137,10.6222237987326));
#75117=CARTESIAN_POINT('Ctrl Pts',(0.386283334539984,1.96641538355556,10.6420941422554));
#75118=CARTESIAN_POINT('Ctrl Pts',(0.321422485940219,2.35248217724416,10.6619644857782));
#75119=CARTESIAN_POINT('Ctrl Pts',(-0.0382997357895325,2.50693094565589,
10.681834829301));
#75120=CARTESIAN_POINT('Ctrl Pts',(-0.362887163970587,2.28807597007412,
10.7017051728238));
#75121=CARTESIAN_POINT('Ctrl Pts',(-0.354575021834985,1.89668689618064,
10.7215755163465));
#75122=CARTESIAN_POINT('Ctrl Pts',(-0.0209885681961636,1.69180991646168,
10.7414458598693));
#75123=CARTESIAN_POINT('Ctrl Pts',(0.331852039427098,1.86139176832721,10.7613162033921));
#75124=CARTESIAN_POINT('Ctrl Pts',(0.380263578451655,2.24986418917502,10.7811865469149));
#75125=CARTESIAN_POINT('Ctrl Pts',(0.0798350524583911,2.50085661862181,
10.8010568904377));
#75126=CARTESIAN_POINT('Ctrl Pts',(-0.293831265604475,2.38411767218393,
10.8209272339605));
#75127=CARTESIAN_POINT('Ctrl Pts',(-0.397947398989942,2.00673944064567,
10.8407975774833));
#75128=CARTESIAN_POINT('Ctrl Pts',(-0.137000969448484,1.71491507603632,
10.8606679210061));
#75129=CARTESIAN_POINT('Ctrl Pts',(0.249625198564137,1.77635370458515,10.8805382645289));
#75130=CARTESIAN_POINT('Ctrl Pts',(0.407254230296271,2.13469374871262,10.9004086080516));
#75131=CARTESIAN_POINT('Ctrl Pts',(0.191282948388597,2.46120700152365,10.9202789515745));
#75132=CARTESIAN_POINT('Ctrl Pts',(-0.200164397843656,2.45636200432963,
10.9401492950972));
#75133=CARTESIAN_POINT('Ctrl Pts',(-0.407988158976476,2.12460338246925,
10.96001963862));
#75134=CARTESIAN_POINT('Ctrl Pts',(-0.241538326820766,1.77027450664141,
10.9798899821428));
#75135=CARTESIAN_POINT('Ctrl Pts',(0.146490037719062,1.71842388289751,10.9997603256656));
#75136=CARTESIAN_POINT('Ctrl Pts',(0.400133735469466,2.01661739969757,11.0196306691884));
#75137=CARTESIAN_POINT('Ctrl Pts',(0.286709204215817,2.39130310075911,11.0395010127112));
#75138=CARTESIAN_POINT('Ctrl Pts',(-0.0897319899722423,2.4987578642103,
11.059371356234));
#75139=CARTESIAN_POINT('Ctrl Pts',(-0.38385629926812,2.24040657322977,11.0792416997568));
#75140=CARTESIAN_POINT('Ctrl Pts',(-0.325844711301839,1.85325136593982,
11.0991120432796));
#75141=CARTESIAN_POINT('Ctrl Pts',(0.0310850395320932,1.69245443860689,
11.1189823868023));
#75142=CARTESIAN_POINT('Ctrl Pts',(0.359498498441325,1.90552508153396,11.1388527303251));
#75143=CARTESIAN_POINT('Ctrl Pts',(0.358121026331844,2.29699998678418,11.1587230738479));
#75144=CARTESIAN_POINT('Ctrl Pts',(0.0282162663381952,2.50775422328637,
11.1785934173707));
#75145=CARTESIAN_POINT('Ctrl Pts',(-0.327573076722947,2.34444947064824,
11.1984637608935));
#75146=CARTESIAN_POINT('Ctrl Pts',(-0.382858716938286,1.95689560748072,
11.2183341044163));
#75147=CARTESIAN_POINT('Ctrl Pts',(-0.0869236058705181,1.70062054254581,
11.2382044479391));
#75148=CARTESIAN_POINT('Ctrl Pts',(0.28875208000307,1.81072175922161,11.2580747914619));
#75149=CARTESIAN_POINT('Ctrl Pts',(0.399537042519869,2.18619638013524,11.2779451349846));
#75150=CARTESIAN_POINT('Ctrl Pts',(0.143801160581459,2.48259755685232,11.2978154785074));
#75151=CARTESIAN_POINT('Ctrl Pts',(-0.243852709430189,2.42801756111144,
11.3176858220302));
#75152=CARTESIAN_POINT('Ctrl Pts',(-0.407804916088317,2.07252610860939,
11.337556165553));
#75153=CARTESIAN_POINT('Ctrl Pts',(-0.197651629861533,1.74223821122565,
11.3574265090758));
#75154=CARTESIAN_POINT('Ctrl Pts',(0.193820118923557,1.74014805017286,11.3772968525986));
#75155=CARTESIAN_POINT('Ctrl Pts',(0.407488294822822,2.0681730636672,11.3971671961214));
#75156=CARTESIAN_POINT('Ctrl Pts',(0.247341434744175,2.42539495840076,11.4170375396442));
#75157=CARTESIAN_POINT('Ctrl Pts',(-0.13970751921652,2.48411127732509,11.436907883167));
#75158=CARTESIAN_POINT('Ctrl Pts',(-0.398593843757351,2.19045779133211,
11.4567782266897));
#75159=CARTESIAN_POINT('Ctrl Pts',(-0.291824580302666,1.81382159650821,
11.4766485702126));
#75160=CARTESIAN_POINT('Ctrl Pts',(0.0826540072505418,1.69971512721642,
11.4965189137353));
#75161=CARTESIAN_POINT('Ctrl Pts',(0.381308795478392,1.9528155348389,11.5163892572581));
#75162=CARTESIAN_POINT('Ctrl Pts',(0.330164674359836,2.34093765189111,11.5362596007809));
#75163=CARTESIAN_POINT('Ctrl Pts',(-0.0238605876222108,2.50803227403266,
11.5561299443037));
#75164=CARTESIAN_POINT('Ctrl Pts',(-0.355997008786566,2.30081283332735,
11.5760002878265));
#75165=CARTESIAN_POINT('Ctrl Pts',(-0.361554639005669,1.90937495624284,
11.5958706313493));
#75166=CARTESIAN_POINT('Ctrl Pts',(-0.0354351091565347,1.69280960554918,
11.6157409748721));
#75167=CARTESIAN_POINT('Ctrl Pts',(0.323191309289222,1.84978600779761,11.6356113183949));
#75168=CARTESIAN_POINT('Ctrl Pts',(0.385333699985837,2.23629968433259,11.6554816619177));
#75169=CARTESIAN_POINT('Ctrl Pts',(0.0939848793917442,2.4977769560189,11.6753520054404));
#75170=CARTESIAN_POINT('Ctrl Pts',(-0.283582273158319,2.3943480230005,11.6952223489632));
#75171=CARTESIAN_POINT('Ctrl Pts',(-0.401001296325997,2.020894850744,11.715092692486));
#75172=CARTESIAN_POINT('Ctrl Pts',(-0.150556221511496,1.72000988373627,
11.7349630360088));
#75173=CARTESIAN_POINT('Ctrl Pts',(0.238003690161047,1.76771411741745,11.7548333795316));
#75174=CARTESIAN_POINT('Ctrl Pts',(0.408227617387438,2.12024541173004,11.7747037230544));
#75175=CARTESIAN_POINT('Ctrl Pts',(0.203958280832558,2.45420429694426,11.7945740665772));
#75176=CARTESIAN_POINT('Ctrl Pts',(-0.187415011973541,2.46322896027285,
11.8144444101));
#75177=CARTESIAN_POINT('Ctrl Pts',(-0.406860545543882,2.13904050170884,
11.8343147536228));
#75178=CARTESIAN_POINT('Ctrl Pts',(-0.253066917639391,1.77903769771133,
11.8541850971455));
#75179=CARTESIAN_POINT('Ctrl Pts',(0.132881155249389,1.71347411099187,11.8740554406683));
#75180=CARTESIAN_POINT('Ctrl Pts',(0.396928858332618,2.00249540668918,11.8939257841911));
#75181=CARTESIAN_POINT('Ctrl Pts',(0.296848370880228,2.38096389269744,11.9137961277139));
#75182=CARTESIAN_POINT('Ctrl Pts',(-0.0755500845982718,2.50168625693585,
11.9336664712367));
#75183=CARTESIAN_POINT('Ctrl Pts',(-0.378641622673128,2.25391616508152,
11.9535368147595));
#75184=CARTESIAN_POINT('Ctrl Pts',(-0.334381019347623,1.86494894555866,
11.9734071582823));
#75185=CARTESIAN_POINT('Ctrl Pts',(0.0166286473641349,1.69160906917418,
11.9932775018051));
#75186=CARTESIAN_POINT('Ctrl Pts',(0.352383793905219,1.89291227441756,12.0131478453279));
#75187=CARTESIAN_POINT('Ctrl Pts',(0.364874782259903,2.28419027543476,12.0330181888507));
#75188=CARTESIAN_POINT('Ctrl Pts',(0.0426428311072668,2.50649877398228,
12.0528885323734));
#75189=CARTESIAN_POINT('Ctrl Pts',(-0.318708112289043,2.35589998721199,
12.0727588758962));
#75190=CARTESIAN_POINT('Ctrl Pts',(-0.387687750851717,1.97054779981215,
12.092629219419));
#75191=CARTESIAN_POINT('Ctrl Pts',(-0.101016656929325,1.70395038275897,
12.1124995629418));
#75192=CARTESIAN_POINT('Ctrl Pts',(0.278323467549698,1.80067457223775,12.1323699064646));
#75193=CARTESIAN_POINT('Ctrl Pts',(0.402339700870507,2.17198909221105,12.1522402499874));
#75194=CARTESIAN_POINT('Ctrl Pts',(0.157264032246886,2.47726342051065,12.1721105935102));
#75195=CARTESIAN_POINT('Ctrl Pts',(-0.232079976398536,2.43644992026867,
12.191980937033));
#75196=CARTESIAN_POINT('Ctrl Pts',(-0.40852220153409,2.08698942170082,12.2118512805557));
#75197=CARTESIAN_POINT('Ctrl Pts',(-0.210200922037842,1.74946435749216,
12.2317216240786));
#75198=CARTESIAN_POINT('Ctrl Pts',(0.180951087156625,1.73350802416591,12.2515919676013));
#75199=CARTESIAN_POINT('Ctrl Pts',(0.406105108150944,2.05375818529026,12.2714623111241));
#75200=CARTESIAN_POINT('Ctrl Pts',(0.258712978634946,2.41642891615619,12.2913326546469));
#75201=CARTESIAN_POINT('Ctrl Pts',(-0.126013088186973,2.48881919435584,
12.3112029981697));
#75202=CARTESIAN_POINT('Ctrl Pts',(-0.395139301730199,2.20452079468752,
12.3310733416925));
#75203=CARTESIAN_POINT('Ctrl Pts',(-0.301778999294402,1.82433879511471,
12.3509436852153));
#75204=CARTESIAN_POINT('Ctrl Pts',(0.068422451493072,1.69703842313985,12.3708140287381));
#75205=CARTESIAN_POINT('Ctrl Pts',(0.375855617911298,1.93940043966916,12.3906843722609));
#75206=CARTESIAN_POINT('Ctrl Pts',(0.338492423017834,2.32909068914615,12.4105547157836));
#75207=CARTESIAN_POINT('Ctrl Pts',(-0.00939148841223189,2.50862141921263,
12.4304250593064));
#75208=CARTESIAN_POINT('Ctrl Pts',(-0.348659987759772,2.31329762593451,
12.4502954028292));
#75209=CARTESIAN_POINT('Ctrl Pts',(-0.368080414108929,1.92230229871115,
12.470165746352));
#75210=CARTESIAN_POINT('Ctrl Pts',(-0.0498371701366613,1.69432042106275,
12.4900360898748));
#75211=CARTESIAN_POINT('Ctrl Pts',(0.314124892717934,1.83849432880167,12.5099064333976));
#75212=CARTESIAN_POINT('Ctrl Pts',(0.389920130746389,2.22256408908266,12.5297767769204));
#75213=CARTESIAN_POINT('Ctrl Pts',(0.108016731647488,2.49419798322434,12.5496471204432));
#75214=CARTESIAN_POINT('Ctrl Pts',(-0.272977313587828,2.40420889296717,
12.569517463966));
#75215=CARTESIAN_POINT('Ctrl Pts',(-0.403551836111819,2.03514955771372,
12.5893878074887));
#75216=CARTESIAN_POINT('Ctrl Pts',(-0.163922487624767,1.72558167466743,
12.6092581510116));
#75217=CARTESIAN_POINT('Ctrl Pts',(0.226083427226409,1.75949163266156,12.6291284945343));
#75218=CARTESIAN_POINT('Ctrl Pts',(0.408688576076754,2.10577166166041,12.6489988380571));
#75219=CARTESIAN_POINT('Ctrl Pts',(0.216377594302136,2.44675697682662,12.6688691815799));
#75220=CARTESIAN_POINT('Ctrl Pts',(-0.174430373094981,2.46963997245408,
12.6887395251027));
#75221=CARTESIAN_POINT('Ctrl Pts',(-0.405222219728848,2.15342861529311,
12.7086098686255));
#75222=CARTESIAN_POINT('Ctrl Pts',(-0.264277845784499,1.78820377724994,
12.7284802121483));
#75223=CARTESIAN_POINT('Ctrl Pts',(0.119105473485777,1.70900952635704,12.7483505556711));
#75224=CARTESIAN_POINT('Ctrl Pts',(0.393225735581682,1.98849580648535,12.7682208991939));
#75225=CARTESIAN_POINT('Ctrl Pts',(0.30661491812593,2.37027200423761,12.7880912427167));
#75226=CARTESIAN_POINT('Ctrl Pts',(-0.0612733448481435,2.50411043231376,
12.8079615862394));
#75227=CARTESIAN_POINT('Ctrl Pts',(-0.37295165555669,2.26723255340767,12.8278319297622));
#75228=CARTESIAN_POINT('Ctrl Pts',(-0.342497595036638,1.87694157341012,
12.847702273285));
#75229=CARTESIAN_POINT('Ctrl Pts',(0.00215138201819559,1.69127633313888,
12.8675726168078));
#75230=CARTESIAN_POINT('Ctrl Pts',(0.34482675909834,1.88055941452387,12.8874429603306));
#75231=CARTESIAN_POINT('Ctrl Pts',(0.371170528355002,2.27114935891834,12.9073133038534));
#75232=CARTESIAN_POINT('Ctrl Pts',(0.0570158686801648,2.50473306643805,
12.9271836473762));
#75233=CARTESIAN_POINT('Ctrl Pts',(-0.309443089519117,2.3670292848331,12.947053990899));
#75234=CARTESIAN_POINT('Ctrl Pts',(-0.392030137992801,1.98436248733954,
12.9669243344217));
#75235=CARTESIAN_POINT('Ctrl Pts',(-0.114982908725333,1.70777736471782,
12.9867946779446));
#75236=CARTESIAN_POINT('Ctrl Pts',(0.267545493074158,1.79100311438672,13.0066650214673));
#75237=CARTESIAN_POINT('Ctrl Pts',(0.404637313975969,2.15769143911221,13.0265353649901));
#75238=CARTESIAN_POINT('Ctrl Pts',(0.170529512724876,2.47145572506355,13.0464057085129));
#75239=CARTESIAN_POINT('Ctrl Pts',(-0.220015952999425,2.44445994733255,
13.0662760520357));
#75240=CARTESIAN_POINT('Ctrl Pts',(-0.408726634081876,2.10146907166997,
13.0861463955585));
#75241=CARTESIAN_POINT('Ctrl Pts',(-0.222486464535814,1.75713050395217,
13.1060167390813));
#75242=CARTESIAN_POINT('Ctrl Pts',(0.167855119186367,1.72732805758641,13.1258870826041));
#75243=CARTESIAN_POINT('Ctrl Pts',(0.404211766498755,2.03940131397413,13.1457574261269));
#75244=CARTESIAN_POINT('Ctrl Pts',(0.269760525376877,2.40706574927223,13.1656277696497));
#75245=CARTESIAN_POINT('Ctrl Pts',(-0.112161928724845,2.4930389042952,13.1854981131724));
#75246=CARTESIAN_POINT('Ctrl Pts',(-0.391185968470993,2.21845286996803,
13.2053684566952));
#75247=CARTESIAN_POINT('Ctrl Pts',(-0.311359986670267,1.83520149440462,
13.225238800218));
#75248=CARTESIAN_POINT('Ctrl Pts',(0.0541153637968024,1.69486854546018,
13.2451091437408));
#75249=CARTESIAN_POINT('Ctrl Pts',(0.369910703092766,1.92618499577519,13.2649794872636));
#75250=CARTESIAN_POINT('Ctrl Pts',(0.346433692742772,2.31695989844127,13.2848498307864));
#75251=CARTESIAN_POINT('Ctrl Pts',(0.00501537287145404,2.50869044887863,
13.3047201743092));
#75252=CARTESIAN_POINT('Ctrl Pts',(-0.34074231600259,2.32552846162887,13.324590517832));
#75253=CARTESIAN_POINT('Ctrl Pts',(-0.374423584156985,1.93542678034618,
13.3444608613547));
#75254=CARTESIAN_POINT('Ctrl Pts',(-0.0636005276092969,1.69638446284464,
13.3643312048776));
#75255=CARTESIAN_POINT('Ctrl Pts',(0.18094005180683,1.78378854426931,13.3775781005594));
#75256=CARTESIAN_POINT('Ctrl Pts',(0.257657118195791,1.86957053507955,13.3842015484003));
#75257=CARTESIAN_POINT('Ctrl Pts',(-0.30218654676688,1.98967595057273,4.35702116407176));
#75258=CARTESIAN_POINT('Ctrl Pts',(-0.265436565557791,1.88899823722173,
4.36364904798937));
#75259=CARTESIAN_POINT('Ctrl Pts',(-0.0840495481126467,1.72910339695751,
4.37690037974791));
#75260=CARTESIAN_POINT('Ctrl Pts',(0.267075589668208,1.8287940790038,4.39677515934738));
#75261=CARTESIAN_POINT('Ctrl Pts',(0.372263060333583,2.17768299025661,4.41664550287017));
#75262=CARTESIAN_POINT('Ctrl Pts',(0.13637277573507,2.45509181004173,4.43651584639296));
#75263=CARTESIAN_POINT('Ctrl Pts',(-0.224838396532887,2.4068641708413,4.45638618991575));
#75264=CARTESIAN_POINT('Ctrl Pts',(-0.379678279217523,2.07707236126518,
4.47625653343854));
#75265=CARTESIAN_POINT('Ctrl Pts',(-0.186273507897977,1.76834368554434,
4.49612687696133));
#75266=CARTESIAN_POINT('Ctrl Pts',(0.178042210154651,1.76384887454306,4.51599722048411));
#75267=CARTESIAN_POINT('Ctrl Pts',(0.379012673598637,2.06773508589522,4.53586756400691));
#75268=CARTESIAN_POINT('Ctrl Pts',(0.232298792807713,2.40121574327281,4.55573790752969));
#75269=CARTESIAN_POINT('Ctrl Pts',(-0.127521856221539,2.45837415432726,
4.5756082510525));
#75270=CARTESIAN_POINT('Ctrl Pts',(-0.370356355674705,2.18677192919838,
4.59547859457527));
#75271=CARTESIAN_POINT('Ctrl Pts',(-0.273440464245838,1.83556886276934,
4.61534893809807));
#75272=CARTESIAN_POINT('Ctrl Pts',(0.0743204226161996,1.72694505892743,
4.63521928162085));
#75273=CARTESIAN_POINT('Ctrl Pts',(0.353902130566146,1.96054853596556,4.65508962514364));
#75274=CARTESIAN_POINT('Ctrl Pts',(0.308826973578812,2.32207966394233,4.67495996866644));
#75275=CARTESIAN_POINT('Ctrl Pts',(-0.0195549719747447,2.47988297661507,
4.69483031218921));
#75276=CARTESIAN_POINT('Ctrl Pts',(-0.329997849655603,2.2891953523409,4.71470065571202));
#75277=CARTESIAN_POINT('Ctrl Pts',(-0.337712647887813,1.92494676049446,
4.7345709992348));
#75278=CARTESIAN_POINT('Ctrl Pts',(-0.0356220554462792,1.72128567853538,
4.7544413427576));
#75279=CARTESIAN_POINT('Ctrl Pts',(0.299146917306782,1.86504343234269,4.77431168628037));
#75280=CARTESIAN_POINT('Ctrl Pts',(0.359489321750484,2.22434184890623,4.79418202980318));
#75281=CARTESIAN_POINT('Ctrl Pts',(0.0900492119073741,2.46957354755419,
4.81405237332595));
#75282=CARTESIAN_POINT('Ctrl Pts',(-0.261998789919797,2.3757718287794,4.83392271684875));
#75283=CARTESIAN_POINT('Ctrl Pts',(-0.373698570350197,2.02898700027084,
4.85379306037154));
#75284=CARTESIAN_POINT('Ctrl Pts',(-0.142580786722154,1.747346931349,4.87366340389433));
#75285=CARTESIAN_POINT('Ctrl Pts',(0.21933545798344,1.78921804359556,4.89353374741711));
#75286=CARTESIAN_POINT('Ctrl Pts',(0.380041279877134,2.11618929166855,4.91340409093991));
#75287=CARTESIAN_POINT('Ctrl Pts',(0.192110965399915,2.42830906862518,4.9332744344627));
#75288=CARTESIAN_POINT('Ctrl Pts',(-0.172055006268819,2.43924997035339,
4.95314477798548));
#75289=CARTESIAN_POINT('Ctrl Pts',(-0.378383932868546,2.13897520899983,
4.97301512150828));
#75290=CARTESIAN_POINT('Ctrl Pts',(-0.237597113377836,1.80294599938219,
4.99288546503106));
#75291=CARTESIAN_POINT('Ctrl Pts',(0.121152711708541,1.73942339508214,5.01275580855386));
#75292=CARTESIAN_POINT('Ctrl Pts',(0.368761417255891,2.00668073772146,5.03262615207664));
#75293=CARTESIAN_POINT('Ctrl Pts',(0.278081724804058,2.35954579923129,5.05249649559943));
#75294=CARTESIAN_POINT('Ctrl Pts',(-0.0677000927468386,2.47431292391617,
5.07236683912222));
#75295=CARTESIAN_POINT('Ctrl Pts',(-0.35137629173806,2.24569889901118,5.09223718264501));
#75296=CARTESIAN_POINT('Ctrl Pts',(-0.312712578622125,1.88342596937737,
5.1121075261678));
#75297=CARTESIAN_POINT('Ctrl Pts',(0.0128223534062021,1.71983022894796,
5.13197786969059));
#75298=CARTESIAN_POINT('Ctrl Pts',(0.326594521790154,1.90498849801793,5.15184821321338));
#75299=CARTESIAN_POINT('Ctrl Pts',(0.340760678260896,2.26904327173777,5.17171855673617));
#75300=CARTESIAN_POINT('Ctrl Pts',(0.042325302804598,2.47802385680157,5.19158890025895));
#75301=CARTESIAN_POINT('Ctrl Pts',(-0.294937775905254,2.34021901655094,
5.21145924378176));
#75302=CARTESIAN_POINT('Ctrl Pts',(-0.361635597374513,1.98204593148086,
5.23132958730454));
#75303=CARTESIAN_POINT('Ctrl Pts',(-0.096581990493603,1.73207964628071,
5.25119993082733));
#75304=CARTESIAN_POINT('Ctrl Pts',(0.25707244421448,1.81963019778472,5.27107027435011));
#75305=CARTESIAN_POINT('Ctrl Pts',(0.374897908608829,2.16438187391932,5.29094061787291));
#75306=CARTESIAN_POINT('Ctrl Pts',(0.148805579596161,2.45007194553361,5.31081096139569));
#75307=CARTESIAN_POINT('Ctrl Pts',(-0.21379561064561,2.41461866511271,5.33068130491849));
#75308=CARTESIAN_POINT('Ctrl Pts',(-0.380268433764204,2.09054559091451,
5.35055164844128));
#75309=CARTESIAN_POINT('Ctrl Pts',(-0.197896737776705,1.77514564995066,
5.37042199196406));
#75310=CARTESIAN_POINT('Ctrl Pts',(0.166018273912844,1.75775535023081,5.39029233548685));
#75311=CARTESIAN_POINT('Ctrl Pts',(0.377634120634467,2.05432792427237,5.41016267900964));
#75312=CARTESIAN_POINT('Ctrl Pts',(0.242822071917181,2.39279841010239,5.43003302253243));
#75313=CARTESIAN_POINT('Ctrl Pts',(-0.114746170544072,2.46266621556758,
5.44990336605522));
#75314=CARTESIAN_POINT('Ctrl Pts',(-0.367050422811667,2.19983714079646,
5.46977370957801));
#75315=CARTESIAN_POINT('Ctrl Pts',(-0.282635881552423,1.845421080944,5.4896440531008));
#75316=CARTESIAN_POINT('Ctrl Pts',(0.0610586036303811,1.72454652153516,
5.50951439662359));
#75317=CARTESIAN_POINT('Ctrl Pts',(0.34874013236059,1.94809941524223,5.52938474014638));
#75318=CARTESIAN_POINT('Ctrl Pts',(0.31650006633187,2.31100041606727,5.54925508366917));
#75319=CARTESIAN_POINT('Ctrl Pts',(-0.00608572296309057,2.48033726026337,
5.56912542719196));
#75320=CARTESIAN_POINT('Ctrl Pts',(-0.323088689935783,2.30076644641029,
5.58899577071475));
#75321=CARTESIAN_POINT('Ctrl Pts',(-0.343701768445756,1.93701974985939,
5.60886611423753));
#75322=CARTESIAN_POINT('Ctrl Pts',(-0.0490152651773467,1.72278524505498,
5.62873645776033));
#75323=CARTESIAN_POINT('Ctrl Pts',(0.290636071065476,1.8545939247609,5.64860680128312));
#75324=CARTESIAN_POINT('Ctrl Pts',(0.363668378633969,2.21152926947835,5.6684771448059));
#75325=CARTESIAN_POINT('Ctrl Pts',(0.103084457784923,2.46615169278842,5.6883474883287));
#75326=CARTESIAN_POINT('Ctrl Pts',(-0.252065419400099,2.38487978501692,
5.70821783185148));
#75327=CARTESIAN_POINT('Ctrl Pts',(-0.3759795898937,2.04226945737306,5.72808817537427));
#75328=CARTESIAN_POINT('Ctrl Pts',(-0.154983671659029,1.75261904328573,
5.74795851889706));
#75329=CARTESIAN_POINT('Ctrl Pts',(0.208188666201143,1.78164336533688,5.76782886241985));
#75330=CARTESIAN_POINT('Ctrl Pts',(0.380376245149376,2.10271655934924,5.78769920594264));
#75331=CARTESIAN_POINT('Ctrl Pts',(0.203620402722817,2.42129767998483,5.80756954946543));
#75332=CARTESIAN_POINT('Ctrl Pts',(-0.15992943878723,2.44513191996371,5.82743989298822));
#75333=CARTESIAN_POINT('Ctrl Pts',(-0.376765792637049,2.15235460884403,
5.84731023651101));
#75334=CARTESIAN_POINT('Ctrl Pts',(-0.24797082377341,1.81154907154635,5.8671805800338));
#75335=CARTESIAN_POINT('Ctrl Pts',(0.108303617723016,1.73535799205694,5.88705092355659));
#75336=CARTESIAN_POINT('Ctrl Pts',(0.365224234164739,1.99367631332851,5.90692126707937));
#75337=CARTESIAN_POINT('Ctrl Pts',(0.287101336550038,2.34953214245828,5.92679161060217));
#75338=CARTESIAN_POINT('Ctrl Pts',(-0.0543979520317252,2.47647620161624,
5.94666195412495));
#75339=CARTESIAN_POINT('Ctrl Pts',(-0.345994525236831,2.25805459839808,
5.96653229764775));
#75340=CARTESIAN_POINT('Ctrl Pts',(-0.320188224438393,1.89463941834026,
5.98640264117053));
#75341=CARTESIAN_POINT('Ctrl Pts',(-0.000652817408372478,1.7196146146366,
6.00627298469333));
#75342=CARTESIAN_POINT('Ctrl Pts',(0.319481460720768,1.89354161720976,6.02614332821611));
#75343=CARTESIAN_POINT('Ctrl Pts',(0.346534992112049,2.25686607922219,6.0460136717389));
#75344=CARTESIAN_POINT('Ctrl Pts',(0.0556898447196964,2.47628726893655,
6.06588401526169));
#75345=CARTESIAN_POINT('Ctrl Pts',(-0.28624315371522,2.35051611628756,6.08575435878448));
#75346=CARTESIAN_POINT('Ctrl Pts',(-0.365587027102976,1.99493053163432,
6.10562470230728));
#75347=CARTESIAN_POINT('Ctrl Pts',(-0.109554573303277,1.73573188029013,
6.12549504583006));
#75348=CARTESIAN_POINT('Ctrl Pts',(0.24697928699379,1.81069963815322,6.14536538935285));
#75349=CARTESIAN_POINT('Ctrl Pts',(0.376943274667832,2.15106109332289,6.16523573287564));
#75350=CARTESIAN_POINT('Ctrl Pts',(0.161113124027163,2.44458094670896,6.18510607639843));
#75351=CARTESIAN_POINT('Ctrl Pts',(-0.202516384337175,2.42199469194947,
6.20497641992122));
#75352=CARTESIAN_POINT('Ctrl Pts',(-0.380364680188321,2.10402214294532,
6.22484676344401));
#75353=CARTESIAN_POINT('Ctrl Pts',(-0.209280163942015,1.78235982535416,
6.2447171069668));
#75354=CARTESIAN_POINT('Ctrl Pts',(0.15379041179948,1.75208912519557,6.26458745048959));
#75355=CARTESIAN_POINT('Ctrl Pts',(0.37577922138895,2.04097928888135,6.28445779401238));
#75356=CARTESIAN_POINT('Ctrl Pts',(0.253041753075546,2.38401292007423,6.30432813753516));
#75357=CARTESIAN_POINT('Ctrl Pts',(-0.101827075160669,2.46650336196665,
6.32419848105796));
#75358=CARTESIAN_POINT('Ctrl Pts',(-0.363283424441477,2.21277686418193,
6.34406882458075));
#75359=CARTESIAN_POINT('Ctrl Pts',(-0.291476688369577,1.85559294669396,
6.36393916810353));
#75360=CARTESIAN_POINT('Ctrl Pts',(0.0477202283134581,1.72261922759851,
6.38380951162632));
#75361=CARTESIAN_POINT('Ctrl Pts',(0.343140332041345,1.93584099142845,6.40367985514912));
#75362=CARTESIAN_POINT('Ctrl Pts',(0.323775895459235,2.29965629739181,6.4235501986719));
#75363=CARTESIAN_POINT('Ctrl Pts',(0.00739115290122109,2.48031413124866,
6.44342054219469));
#75364=CARTESIAN_POINT('Ctrl Pts',(-0.315773966229056,2.31208552477859,
6.46329088571748));
#75365=CARTESIAN_POINT('Ctrl Pts',(-0.349259460087822,1.94929732216115,
6.48316122924027));
#75366=CARTESIAN_POINT('Ctrl Pts',(-0.0623469466980092,1.72475831014389,
6.50303157276306));
#75367=CARTESIAN_POINT('Ctrl Pts',(0.281760402516878,1.84445246402643,6.52290191628586));
#75368=CARTESIAN_POINT('Ctrl Pts',(0.367390940637607,2.19857669250918,6.54277225980863));
#75369=CARTESIAN_POINT('Ctrl Pts',(0.115990306483514,2.46227022561963,6.56264260333144));
#75370=CARTESIAN_POINT('Ctrl Pts',(-0.241815643214863,2.39363014536184,
6.58251294685422));
#75371=CARTESIAN_POINT('Ctrl Pts',(-0.377788660490751,2.05562438086923,
6.60238329037701));
#75372=CARTESIAN_POINT('Ctrl Pts',(-0.167192013048295,1.75832720573406,
6.62225363389979));
#75373=CARTESIAN_POINT('Ctrl Pts',(0.196780545228712,1.77446830478718,6.64212397742259));
#75374=CARTESIAN_POINT('Ctrl Pts',(0.380233742510557,2.08924041705957,6.66199432094537));
#75375=CARTESIAN_POINT('Ctrl Pts',(0.214874245188744,2.41388298189485,6.68186466446817));
#75376=CARTESIAN_POINT('Ctrl Pts',(-0.147603119606738,2.45058064215098,
6.70173500799095));
#75377=CARTESIAN_POINT('Ctrl Pts',(-0.374674716513269,2.16566829047828,
6.72160535151375));
#75378=CARTESIAN_POINT('Ctrl Pts',(-0.258033268375595,1.82051422222223,
6.74147569503654));
#75379=CARTESIAN_POINT('Ctrl Pts',(0.0953185754392329,1.7317503065244,6.76134603855932));
#75380=CARTESIAN_POINT('Ctrl Pts',(0.361228602740849,1.98080535192161,6.78121638208212));
#75381=CARTESIAN_POINT('Ctrl Pts',(0.295760563861364,2.33920526004468,6.8010867256049));
#75382=CARTESIAN_POINT('Ctrl Pts',(-0.0410275281959761,2.47816690693233,
6.82095706912769));
#75383=CARTESIAN_POINT('Ctrl Pts',(-0.340178448527117,2.27021189948509,
6.84082741265049));
#75384=CARTESIAN_POINT('Ctrl Pts',(-0.327261953448532,1.90611064651795,
6.86069775617327));
#75385=CARTESIAN_POINT('Ctrl Pts',(-0.0141271687728025,1.71987647971863,
6.88056809969606));
#75386=CARTESIAN_POINT('Ctrl Pts',(0.31196737001161,1.88235389363309,6.90043844321885));
#75387=CARTESIAN_POINT('Ctrl Pts',(0.351874317332742,2.24449198029737,6.92030878674164));
#75388=CARTESIAN_POINT('Ctrl Pts',(0.0689844818637428,2.47407834584566,
6.94017913026443));
#75389=CARTESIAN_POINT('Ctrl Pts',(-0.277189224326068,2.36049875524875,
6.96004947378722));
#75390=CARTESIAN_POINT('Ctrl Pts',(-0.369079553102077,2.00794702041429,
6.97991981731001));
#75391=CARTESIAN_POINT('Ctrl Pts',(-0.122389637550941,1.73984136246816,
6.99979016083279));
#75392=CARTESIAN_POINT('Ctrl Pts',(0.236576108608585,1.80213222328648,7.01966050435559));
#75393=CARTESIAN_POINT('Ctrl Pts',(0.378515482048657,2.13767621820337,7.03953084787837));
#75394=CARTESIAN_POINT('Ctrl Pts',(0.173218430938826,2.43865741207262,7.05940119140117));
#75395=CARTESIAN_POINT('Ctrl Pts',(-0.19098294899741,2.42896653440873,7.07927153492395));
#75396=CARTESIAN_POINT('Ctrl Pts',(-0.379983473209242,2.11749364617445,
7.09914187844675));
#75397=CARTESIAN_POINT('Ctrl Pts',(-0.220400890830285,1.78997271911999,
7.11901222196954));
#75398=CARTESIAN_POINT('Ctrl Pts',(0.141369504013592,1.74685961586985,7.13888256549232));
#75399=CARTESIAN_POINT('Ctrl Pts',(0.373452624645094,2.02770473933704,7.15875290901512));
#75400=CARTESIAN_POINT('Ctrl Pts',(0.262943803148664,2.37487092235148,7.1786232525379));
#75401=CARTESIAN_POINT('Ctrl Pts',(-0.0887801611702712,2.4698804544055,
7.19849359606069));
#75402=CARTESIAN_POINT('Ctrl Pts',(-0.359060413943042,2.22557502421934,
7.21836393958349));
#75403=CARTESIAN_POINT('Ctrl Pts',(-0.299951618584444,1.86607160480778,
7.23823428310627));
#75404=CARTESIAN_POINT('Ctrl Pts',(0.0343219520998536,1.72116564150979,
7.25810462662907));
#75405=CARTESIAN_POINT('Ctrl Pts',(0.337109804244394,1.92378862848572,7.27797497015184));
#75406=CARTESIAN_POINT('Ctrl Pts',(0.33064530435041,2.28806155981396,7.29784531367464));
#75407=CARTESIAN_POINT('Ctrl Pts',(0.0208587510084466,2.47981361228239,
7.31771565719742));
#75408=CARTESIAN_POINT('Ctrl Pts',(-0.308062866721238,2.32313838243594,
7.33758600072022));
#75409=CARTESIAN_POINT('Ctrl Pts',(-0.354378743206429,1.9617640642522,7.35745634424301));
#75410=CARTESIAN_POINT('Ctrl Pts',(-0.0756003671091846,1.72720239799378,
7.37732668776579));
#75411=CARTESIAN_POINT('Ctrl Pts',(0.272531053750123,1.83463177976539,7.39719703128859));
#75412=CARTESIAN_POINT('Ctrl Pts',(0.370652334546399,2.18550037698128,7.41706737481138));
#75413=CARTESIAN_POINT('Ctrl Pts',(0.128750558155218,2.45793401814211,7.43693771833416));
#75414=CARTESIAN_POINT('Ctrl Pts',(-0.231262327537628,2.40201192597398,
7.45680806185696));
#75415=CARTESIAN_POINT('Ctrl Pts',(-0.379123511237657,2.06903500693578,
7.47667840537974));
#75416=CARTESIAN_POINT('Ctrl Pts',(-0.17919048638257,1.76446425353084,7.49654874890254));
#75417=CARTESIAN_POINT('Ctrl Pts',(0.185125415146614,1.76770186844427,7.51641909242532));
#75418=CARTESIAN_POINT('Ctrl Pts',(0.379613950828283,2.07577778075445,7.53628943594811));
#75419=CARTESIAN_POINT('Ctrl Pts',(0.225858366397756,2.40607428166505,7.55615977947091));
#75420=CARTESIAN_POINT('Ctrl Pts',(-0.135091521362634,2.45558929739879,
7.57603012299369));
#75421=CARTESIAN_POINT('Ctrl Pts',(-0.372113329322741,2.17889954188068,
7.59590046651648));
#75422=CARTESIAN_POINT('Ctrl Pts',(-0.267771816284581,1.82983019788974,
7.61577081003927));
#75423=CARTESIAN_POINT('Ctrl Pts',(0.0822138843536524,1.72860486703765,
7.63564115356206));
#75424=CARTESIAN_POINT('Ctrl Pts',(0.356779538507097,1.96808400979676,7.65551149708485));
#75425=CARTESIAN_POINT('Ctrl Pts',(0.30404853722851,2.32857811482695,7.67538184060764));
#75426=CARTESIAN_POINT('Ctrl Pts',(-0.0276056044866047,2.47938291760379,
7.69525218413042));
#75427=CARTESIAN_POINT('Ctrl Pts',(-0.333935362248948,2.28215554179958,
7.71512252765322));
#75428=CARTESIAN_POINT('Ctrl Pts',(-0.333924886342341,1.91782525463201,
7.734992871176));
#75429=CARTESIAN_POINT('Ctrl Pts',(-0.0275837869849208,1.72061549548748,
7.7548632146988));
#75430=CARTESIAN_POINT('Ctrl Pts',(0.304061681737653,1.87143937069673,7.77473355822158));
#75431=CARTESIAN_POINT('Ctrl Pts',(0.356771951726028,2.23193650757178,7.79460390174438));
#75432=CARTESIAN_POINT('Ctrl Pts',(0.0821925261211519,2.47139986028331,
7.81447424526716));
#75433=CARTESIAN_POINT('Ctrl Pts',(-0.267787352697854,2.37015440271021,
7.83434458878996));
#75434=CARTESIAN_POINT('Ctrl Pts',(-0.372108791372701,2.02107905885139,
7.85421493231274));
#75435=CARTESIAN_POINT('Ctrl Pts',(-0.135071072000656,1.74440293438045,
7.87408527583553));
#75436=CARTESIAN_POINT('Ctrl Pts',(0.225875967665989,1.79393870744639,7.89395561935832));
#75437=CARTESIAN_POINT('Ctrl Pts',(0.379612557235358,2.12424404994773,7.91382596288111));
#75438=CARTESIAN_POINT('Ctrl Pts',(0.185106305124325,2.43230877715139,7.9336963064039));
#75439=CARTESIAN_POINT('Ctrl Pts',(-0.179209781990372,2.43552544107355,
7.95356664992669));
#75440=CARTESIAN_POINT('Ctrl Pts',(-0.379125291337669,2.13094319047487,
7.97343699344948));
#75441=CARTESIAN_POINT('Ctrl Pts',(-0.231244959130432,1.79797477515049,
7.99330733697226));
#75442=CARTESIAN_POINT('Ctrl Pts',(0.128771141920517,1.74207338660401,8.01317768049507));
#75443=CARTESIAN_POINT('Ctrl Pts',(0.370657250867365,2.01452093853999,8.03304802401784));
#75444=CARTESIAN_POINT('Ctrl Pts',(0.272515792571565,2.36538389244211,8.05291836754064));
#75445=CARTESIAN_POINT('Ctrl Pts',(-0.0756218057335592,2.47279325378316,
8.07278871106342));
#75446=CARTESIAN_POINT('Ctrl Pts',(-0.354386692257366,2.23821555599685,
8.09265905458622));
#75447=CARTESIAN_POINT('Ctrl Pts',(-0.308050034026664,1.87684390193229,
8.11252939810901));
#75448=CARTESIAN_POINT('Ctrl Pts',(0.0208805931982691,1.72018758788538,
8.13239974163179));
#75449=CARTESIAN_POINT('Ctrl Pts',(0.330656118799868,1.91195745516282,8.15227008515458));
#75450=CARTESIAN_POINT('Ctrl Pts',(0.337099670168359,2.27623075764752,8.17214042867737));
#75451=CARTESIAN_POINT('Ctrl Pts',(0.0343001661334638,2.47883633164185,
8.19201077220018));
#75452=CARTESIAN_POINT('Ctrl Pts',(-0.299965070782925,2.33391114526424,
8.21188111572295));
#75453=CARTESIAN_POINT('Ctrl Pts',(-0.359053191812853,1.97440432723363,
8.23175145924575));
#75454=CARTESIAN_POINT('Ctrl Pts',(-0.088758890032661,1.73011444065926,
8.25162180276853));
#75455=CARTESIAN_POINT('Ctrl Pts',(0.262959609920743,1.82514419940819,8.27149214629133));
#75456=CARTESIAN_POINT('Ctrl Pts',(0.373448466490159,2.17231673696168,8.29136248981411));
#75457=CARTESIAN_POINT('Ctrl Pts',(0.141349195472712,2.45314851338758,8.3112328333369));
#75458=CARTESIAN_POINT('Ctrl Pts',(-0.220418719435609,2.41001460560915,
8.33110317685969));
#75459=CARTESIAN_POINT('Ctrl Pts',(-0.379982466560774,2.08248450186184,
8.35097352038248));
#75460=CARTESIAN_POINT('Ctrl Pts',(-0.190964030558069,1.77102248313653,
8.37084386390527));
#75461=CARTESIAN_POINT('Ctrl Pts',(0.173237906076449,1.7613525498887,8.39071420742806));
#75462=CARTESIAN_POINT('Ctrl Pts',(0.3785176480971,2.06234554943069,8.41058455095085));
#75463=CARTESIAN_POINT('Ctrl Pts',(0.23655897851328,2.39788138117948,8.43045489447364));
#75464=CARTESIAN_POINT('Ctrl Pts',(-0.122410349259601,2.46015159858423,
8.45032523799642));
#75465=CARTESIAN_POINT('Ctrl Pts',(-0.369084846251043,2.19203175450071,
8.47019558151923));
#75466=CARTESIAN_POINT('Ctrl Pts',(-0.27717424317176,1.8394853046548,8.490065925042));
#75467=CARTESIAN_POINT('Ctrl Pts',(0.069005994151748,1.72592562191488,8.5099362685648));
#75468=CARTESIAN_POINT('Ctrl Pts',(0.351882626158829,1.95552825544003,8.52980661208759));
#75469=CARTESIAN_POINT('Ctrl Pts',(0.311954853158996,2.31766404654693,8.54967695561037));
#75470=CARTESIAN_POINT('Ctrl Pts',(-0.0141490287958676,2.48012270723119,
8.56954729913317));
#75471=CARTESIAN_POINT('Ctrl Pts',(-0.327273103046854,2.29387053306451,
8.58941764265595));
#75472=CARTESIAN_POINT('Ctrl Pts',(-0.340168659462118,1.92976853790095,
8.60928798617873));
#75473=CARTESIAN_POINT('Ctrl Pts',(-0.0410057806021346,1.72183073429237,
8.62915832970154));
#75474=CARTESIAN_POINT('Ctrl Pts',(0.295774319527368,1.86081174887391,8.64902867322432));
#75475=CARTESIAN_POINT('Ctrl Pts',(0.36122174752812,2.21921542132362,8.6688990167471));
#75476=CARTESIAN_POINT('Ctrl Pts',(0.0952973980721992,2.46825517442299,
8.68876936026991));
#75477=CARTESIAN_POINT('Ctrl Pts',(-0.258049340545726,2.37947093840426,
8.70863970379268));
#75478=CARTESIAN_POINT('Ctrl Pts',(-0.374670939458421,2.0343101629323,8.72851004731549));
#75479=CARTESIAN_POINT('Ctrl Pts',(-0.147582958260542,1.74941087010618,
8.74838039083826));
#75480=CARTESIAN_POINT('Ctrl Pts',(0.214892295535876,1.78612937555744,8.76825073436106));
#75481=CARTESIAN_POINT('Ctrl Pts',(0.380233123122462,2.11078144930768,8.78812107788384));
#75482=CARTESIAN_POINT('Ctrl Pts',(0.196761824309647,2.42554301107991,8.80799142140664));
#75483=CARTESIAN_POINT('Ctrl Pts',(-0.167211661603712,2.44166317886533,
8.82786176492941));
#75484=CARTESIAN_POINT('Ctrl Pts',(-0.377791211807834,2.1443538932835,8.84773210845223));
#75485=CARTESIAN_POINT('Ctrl Pts',(-0.241798756807518,1.80635594885137,
8.86760245197499));
#75486=CARTESIAN_POINT('Ctrl Pts',(0.116011139635423,1.73773644532036,8.88747279549781));
#75487=CARTESIAN_POINT('Ctrl Pts',(0.367396608953386,2.00144443547831,8.90734313902058));
#75488=CARTESIAN_POINT('Ctrl Pts',(0.281745706088464,2.35556373895635,8.92721348254337));
#75489=CARTESIAN_POINT('Ctrl Pts',(-0.0623685258982764,2.47523810380333,
8.94708382606617));
#75490=CARTESIAN_POINT('Ctrl Pts',(-0.349268126081446,2.25068259246573,
8.96695416958895));
#75491=CARTESIAN_POINT('Ctrl Pts',(-0.315761769146652,1.88789631612342,
8.98682451311175));
#75492=CARTESIAN_POINT('Ctrl Pts',(0.00741302389702733,1.71968629442874,
9.00669485663451));
#75493=CARTESIAN_POINT('Ctrl Pts',(0.32378737670726,1.90036232255992,9.02656520015734));
#75494=CARTESIAN_POINT('Ctrl Pts',(0.343130891059556,2.26417874152677,9.0464355436801));
#75495=CARTESIAN_POINT('Ctrl Pts',(0.047698525917369,2.47738351606018,9.0663058872029));
#75496=CARTESIAN_POINT('Ctrl Pts',(-0.291490743186063,2.34439029073487,
9.08617623072569));
#75497=CARTESIAN_POINT('Ctrl Pts',(-0.363276938297633,1.98720224439407,
9.10604657424848));
#75498=CARTESIAN_POINT('Ctrl Pts',(-0.101805998210462,1.73349078279393,
9.12591691777126));
#75499=CARTESIAN_POINT('Ctrl Pts',(0.253058085599665,1.81600163225598,9.14578726129406));
#75500=CARTESIAN_POINT('Ctrl Pts',(0.375775826619579,2.15904232123663,9.16565760481684));
#75501=CARTESIAN_POINT('Ctrl Pts',(0.153770403975355,2.4479197183689,9.18552794833964));
#75502=CARTESIAN_POINT('Ctrl Pts',(-0.209298430366079,2.41762813889032,
9.20539829186242));
#75503=CARTESIAN_POINT('Ctrl Pts',(-0.380364448254989,2.09595598314635,
9.22526863538522));
#75504=CARTESIAN_POINT('Ctrl Pts',(-0.202497866813709,1.77799366232241,
9.245138978908));
#75505=CARTESIAN_POINT('Ctrl Pts',(0.161132939833921,1.75542831911326,9.2650093224308));
#75506=CARTESIAN_POINT('Ctrl Pts',(0.376946210452853,2.04896058391921,9.28487966595358));
#75507=CARTESIAN_POINT('Ctrl Pts',(0.246962649573998,2.38931456459021,9.30475000947638));
#75508=CARTESIAN_POINT('Ctrl Pts',(-0.10957552136021,2.4642618188711,9.32462035299915));
#75509=CARTESIAN_POINT('Ctrl Pts',(-0.365593068806628,2.20504844410645,
9.34449069652196));
#75510=CARTESIAN_POINT('Ctrl Pts',(-0.286228746625001,1.84946742292844,
9.36436104004474));
#75511=CARTESIAN_POINT('Ctrl Pts',(0.0557114840598653,1.72371593428303,
9.38423138356752));
#75512=CARTESIAN_POINT('Ctrl Pts',(0.346544012553486,1.94315384948313,9.40410172709032));
#75513=CARTESIAN_POINT('Ctrl Pts',(0.319469587236485,2.30647675510717,9.42397207061312));
#75514=CARTESIAN_POINT('Ctrl Pts',(-0.000674692512978063,2.48038534719236,
9.44384241413588));
#75515=CARTESIAN_POINT('Ctrl Pts',(-0.32020003373287,2.30534216801744,9.46371275765871));
#75516=CARTESIAN_POINT('Ctrl Pts',(-0.345985435301189,1.94192550449841,
9.48358310118145));
#75517=CARTESIAN_POINT('Ctrl Pts',(-0.0543763016444307,1.72352067070274,
9.50345344470429));
#75518=CARTESIAN_POINT('Ctrl Pts',(0.287115686106074,1.85048436850475,9.52332378822703));
#75519=CARTESIAN_POINT('Ctrl Pts',(0.365218119125371,2.20634468971775,9.54319413174986));
#75520=CARTESIAN_POINT('Ctrl Pts',(0.108282647804378,2.46464823563691,9.56306447527262));
#75521=CARTESIAN_POINT('Ctrl Pts',(-0.247987411525762,2.38843666773381,
9.58293481879543));
#75522=CARTESIAN_POINT('Ctrl Pts',(-0.376762781218556,2.04762372429146,
9.60280516231822));
#75523=CARTESIAN_POINT('Ctrl Pts',(-0.159909590764387,1.75485888342563,
9.62267550584101));
#75524=CARTESIAN_POINT('Ctrl Pts',(0.203638879491112,1.77871403029663,9.64254584936379));
#75525=CARTESIAN_POINT('Ctrl Pts',(0.3803764007436,2.0973053152353,9.66241619288658));
#75526=CARTESIAN_POINT('Ctrl Pts',(0.208170357884774,2.41836860659739,9.68228653640938));
#75527=CARTESIAN_POINT('Ctrl Pts',(-0.155003648498172,2.44737204337841,
9.70215687993214));
#75528=CARTESIAN_POINT('Ctrl Pts',(-0.375982909225308,2.15770892079316,
9.72202722345497));
#75529=CARTESIAN_POINT('Ctrl Pts',(-0.252049036189305,1.81510571974032,
9.74189756697772));
#75530=CARTESIAN_POINT('Ctrl Pts',(0.103105514172589,1.73385423597173,9.76176791050055));
#75531=CARTESIAN_POINT('Ctrl Pts',(0.363674791829392,1.98849164445439,9.7816382540233));
#75532=CARTESIAN_POINT('Ctrl Pts',(0.290621957834928,2.34542278865832,9.80150859754612));
#75533=CARTESIAN_POINT('Ctrl Pts',(-0.0490369578661753,2.47721193556391,
9.82137894106889));
#75534=CARTESIAN_POINT('Ctrl Pts',(-0.343711140504061,2.26296048435751,
9.84124928459169));
#75535=CARTESIAN_POINT('Ctrl Pts',(-0.323077143775959,1.89921497381975,
9.86111962811447));
#75536=CARTESIAN_POINT('Ctrl Pts',(-0.00606385061491112,1.71966239038934,
9.88098997163728));
#75537=CARTESIAN_POINT('Ctrl Pts',(0.316512199966604,1.88901778548669,9.90086031516005));
#75538=CARTESIAN_POINT('Ctrl Pts',(0.348731396323853,2.25192063976514,9.92073065868285));
#75539=CARTESIAN_POINT('Ctrl Pts',(0.0610370120465778,2.47545698918659,
9.94060100220563));
#75540=CARTESIAN_POINT('Ctrl Pts',(-0.282650521344584,2.35456266488288,
9.96047134572842));
#75541=CARTESIAN_POINT('Ctrl Pts',(-0.367044680795904,2.00014175112657,
9.98034168925121));
#75542=CARTESIAN_POINT('Ctrl Pts',(-0.114725314238147,1.73732718623863,
10.000212032774));
#75543=CARTESIAN_POINT('Ctrl Pts',(0.242838909691915,1.80721555453153,10.0200823762968));
#75544=CARTESIAN_POINT('Ctrl Pts',(0.377631493511943,2.14569379253875,10.0399527198196));
#75545=CARTESIAN_POINT('Ctrl Pts',(0.165998591920333,2.44225419653979,10.0598230633424));
#75546=CARTESIAN_POINT('Ctrl Pts',(-0.197915419090541,2.42484296891706,
10.0796934068652));
#75547=CARTESIAN_POINT('Ctrl Pts',(-0.380268976837149,2.10943254068979,
10.099563750388));
#75548=CARTESIAN_POINT('Ctrl Pts',(-0.213777517282165,1.7853690405041,10.1194340939107));
#75549=CARTESIAN_POINT('Ctrl Pts',(0.148825711198222,1.74993661251857,10.1393044374335));
#75550=CARTESIAN_POINT('Ctrl Pts',(0.374901610445288,2.03563968572042,10.1591747809563));
#75551=CARTESIAN_POINT('Ctrl Pts',(0.257056320354344,2.38038458540818,10.1790451244791));
#75552=CARTESIAN_POINT('Ctrl Pts',(-0.0966031486037206,2.46791479889845,
10.1989154680019));
#75553=CARTESIAN_POINT('Ctrl Pts',(-0.361642380049,2.21793327147642,10.2187858115247));
#75554=CARTESIAN_POINT('Ctrl Pts',(-0.294923960963645,1.85976402263992,
10.2386561550475));
#75555=CARTESIAN_POINT('Ctrl Pts',(0.0423470420341099,1.72197857785623,
10.2585264985703));
#75556=CARTESIAN_POINT('Ctrl Pts',(0.340770398994764,1.93097632491989,10.2783968420931));
#75557=CARTESIAN_POINT('Ctrl Pts',(0.326583306578408,2.29503028337402,10.2982671856158));
#75558=CARTESIAN_POINT('Ctrl Pts',(0.0128004906788188,2.48017050780803,
10.3181375291386));
#75559=CARTESIAN_POINT('Ctrl Pts',(-0.312725032789138,2.31655604686932,
10.3380078726614));
#75560=CARTESIAN_POINT('Ctrl Pts',(-0.351367912341904,1.95428089437164,
10.3578782161842));
#75561=CARTESIAN_POINT('Ctrl Pts',(-0.0676785667428226,1.72568318342309,
10.377748559707));
#75562=CARTESIAN_POINT('Ctrl Pts',(0.278096650237917,1.84047019305081,10.3976189032298));
#75563=CARTESIAN_POINT('Ctrl Pts',(0.368756050065618,2.19334046876163,10.4174892467526));
#75564=CARTESIAN_POINT('Ctrl Pts',(0.121131975561155,2.46058357154103,10.4373595902754));
#75565=CARTESIAN_POINT('Ctrl Pts',(-0.237614195891286,2.39704033645209,
10.4572299337982));
#75566=CARTESIAN_POINT('Ctrl Pts',(-0.378381690865214,2.06100303105861,
10.4771002773209));
#75567=CARTESIAN_POINT('Ctrl Pts',(-0.172035496486027,1.76074013571092,
10.4969706208437));
#75568=CARTESIAN_POINT('Ctrl Pts',(0.192129845401105,1.77170197978851,10.5168409643665));
#75569=CARTESIAN_POINT('Ctrl Pts',(0.380042210249291,2.0838325636705,10.5367113078893));
#75570=CARTESIAN_POINT('Ctrl Pts',(0.219317585268772,2.4107945693871,10.5565816514121));
#75571=CARTESIAN_POINT('Ctrl Pts',(-0.142601066802718,2.45264486855102,
10.5764519949349));
#75572=CARTESIAN_POINT('Ctrl Pts',(-0.373702653464939,2.17099150908312,
10.5963223384577));
#75573=CARTESIAN_POINT('Ctrl Pts',(-0.261982930595375,1.82421310465271,
10.6161926819805));
#75574=CARTESIAN_POINT('Ctrl Pts',(0.0900704653400429,1.73043163170793,
10.6360630255033));
#75575=CARTESIAN_POINT('Ctrl Pts',(0.359496471312573,1.97567882448093,10.655933369026));
#75576=CARTESIAN_POINT('Ctrl Pts',(0.299133405881053,2.33497377099293,10.6758037125489));
#75577=CARTESIAN_POINT('Ctrl Pts',(-0.0356438361104161,2.47871227140928,
10.6956740560716));
#75578=CARTESIAN_POINT('Ctrl Pts',(-0.337722710940686,2.27503381982779,
10.7155443995944));
#75579=CARTESIAN_POINT('Ctrl Pts',(-0.329986975278303,1.91078566725718,
10.7354147431172));
#75580=CARTESIAN_POINT('Ctrl Pts',(-0.0195331134681825,1.72011590577272,
10.75528508664));
#75581=CARTESIAN_POINT('Ctrl Pts',(0.308839720755723,1.87793808419235,10.7751554301628));
#75582=CARTESIAN_POINT('Ctrl Pts',(0.353894155917617,2.23947183936549,10.7950257736856));
#75583=CARTESIAN_POINT('Ctrl Pts',(0.0742988813639559,2.47305916929718,
10.8148961172084));
#75584=CARTESIAN_POINT('Ctrl Pts',(-0.273455501961803,2.36441549881854,
10.8347664607312));
#75585=CARTESIAN_POINT('Ctrl Pts',(-0.370351689842575,2.01320660509356,
10.8546368042539));
#75586=CARTESIAN_POINT('Ctrl Pts',(-0.12750062112257,1.74161883534148,10.8745071477767));
#75587=CARTESIAN_POINT('Ctrl Pts',(0.232314909835208,1.79879699497366,10.8943774912995));
#75588=CARTESIAN_POINT('Ctrl Pts',(0.379013137838279,2.13228790663111,10.9142478348223));
#75589=CARTESIAN_POINT('Ctrl Pts',(0.178018409854183,2.43615905955607,10.9341181783451));
#75590=CARTESIAN_POINT('Ctrl Pts',(-0.186283974153027,2.43165003926185,
10.9539885218679));
#75591=CARTESIAN_POINT('Ctrl Pts',(-0.379696172147903,2.12289725802071,
10.9738588653907));
#75592=CARTESIAN_POINT('Ctrl Pts',(-0.224788823163257,1.79313935972577,
10.9937292089135));
#75593=CARTESIAN_POINT('Ctrl Pts',(0.136331668838762,1.74488432357853,11.0135995524363));
#75594=CARTESIAN_POINT('Ctrl Pts',(0.372386414561987,2.02239957591415,11.033469895959));
#75595=CARTESIAN_POINT('Ctrl Pts',(0.266827320757131,2.37110265300474,11.0533402394819));
#75596=CARTESIAN_POINT('Ctrl Pts',(-0.0835095145828133,2.47110595325699,
11.0732105830046));
#75597=CARTESIAN_POINT('Ctrl Pts',(-0.357237739086846,2.23067006290943,
11.0930809265274));
#75598=CARTESIAN_POINT('Ctrl Pts',(-0.303248971505297,1.87036217896519,
11.1129512700502));
#75599=CARTESIAN_POINT('Ctrl Pts',(0.028929443812777,1.72071573345402,11.132821613573));
#75600=CARTESIAN_POINT('Ctrl Pts',(0.334569032820766,1.9190109676085,11.1526919570958));
#75601=CARTESIAN_POINT('Ctrl Pts',(0.333287081676621,2.28333899955034,11.1725623006186));
#75602=CARTESIAN_POINT('Ctrl Pts',(0.026259606033199,2.47947845875572,11.1924326441414));
#75603=CARTESIAN_POINT('Ctrl Pts',(-0.304857483223131,2.3274980933799,11.2123029876641));
#75604=CARTESIAN_POINT('Ctrl Pts',(-0.356309334220927,1.96681919839678,
11.232173331187));
#75605=CARTESIAN_POINT('Ctrl Pts',(-0.0808958782067142,1.72831555795567,
11.2520436747097));
#75606=CARTESIAN_POINT('Ctrl Pts',(0.268728533082803,1.83078179282263,11.2719140182325));
#75607=CARTESIAN_POINT('Ctrl Pts',(0.371831099355113,2.18021908202544,11.2917843617553));
#75608=CARTESIAN_POINT('Ctrl Pts',(0.13382925220231,2.4560662843118,11.3116547052781));
#75609=CARTESIAN_POINT('Ctrl Pts',(-0.226942714638603,2.4052711447895,11.3315250488009));
#75610=CARTESIAN_POINT('Ctrl Pts',(-0.379525636259362,2.07443128883647,
11.3513953923237));
#75611=CARTESIAN_POINT('Ctrl Pts',(-0.183945454361969,1.76704724451027,
11.3712657358465));
#75612=CARTESIAN_POINT('Ctrl Pts',(0.180379640000184,1.76510202592127,11.3911360793693));
#75613=CARTESIAN_POINT('Ctrl Pts',(0.379230971132724,2.07038010630728,11.4110064228921));
#75614=CARTESIAN_POINT('Ctrl Pts',(0.23018951388577,2.40283040677195,11.4308767664148));
#75615=CARTESIAN_POINT('Ctrl Pts',(-0.130019484878821,2.45747503566052,
11.4507471099376));
#75616=CARTESIAN_POINT('Ctrl Pts',(-0.370953306821607,2.18418498516215,
11.4706174534604));
#75617=CARTESIAN_POINT('Ctrl Pts',(-0.27158797048811,1.83366667152836,11.4904877969832));
#75618=CARTESIAN_POINT('Ctrl Pts',(0.0769223554047115,1.72747292875869,
11.510358140506));
#75619=CARTESIAN_POINT('Ctrl Pts',(0.354866892246784,1.9630220588717,11.5302284840288));
#75620=CARTESIAN_POINT('Ctrl Pts',(0.30726936621738,2.32422980210713,11.5500988275516));
#75621=CARTESIAN_POINT('Ctrl Pts',(-0.0222059723695601,2.47973722804034,
11.5699691710744));
#75622=CARTESIAN_POINT('Ctrl Pts',(-0.33131035437759,2.28688744380196,11.5898395145972));
#75623=CARTESIAN_POINT('Ctrl Pts',(-0.336482590076081,1.92259387230333,
11.6097098581199));
#75624=CARTESIAN_POINT('Ctrl Pts',(-0.0329778573479846,1.72104627130298,
11.6295802016427));
#75625=CARTESIAN_POINT('Ctrl Pts',(0.300779569967016,1.86713712649052,11.6494505451655));
#75626=CARTESIAN_POINT('Ctrl Pts',(0.358612689278201,2.22684796670539,11.6693208886883));
#75627=CARTESIAN_POINT('Ctrl Pts',(0.0874674868858114,2.47019306625937,
11.6891912322111));
#75628=CARTESIAN_POINT('Ctrl Pts',(-0.263917227101225,2.37393642475552,
11.7090615757339));
#75629=CARTESIAN_POINT('Ctrl Pts',(-0.373193814308984,2.02638040661516,
11.7289319192567));
#75630=CARTESIAN_POINT('Ctrl Pts',(-0.140115882638339,1.74636034300277,
11.7488022627795));
#75631=CARTESIAN_POINT('Ctrl Pts',(0.221499296298022,1.79075652099338,11.7686726063023));
#75632=CARTESIAN_POINT('Ctrl Pts',(0.37991902528722,2.11884149127447,11.7885429498251));
#75633=CARTESIAN_POINT('Ctrl Pts',(0.189814769880288,2.42964195834864,11.8084132933478));
#75634=CARTESIAN_POINT('Ctrl Pts',(-0.174418695944306,2.43804080533824,
11.8282836368706));
#75635=CARTESIAN_POINT('Ctrl Pts',(-0.378646753201302,2.13633323353006,
11.8481539803934));
#75636=CARTESIAN_POINT('Ctrl Pts',(-0.235517962496791,1.80129486628114,
11.8680243239162));
#75637=CARTESIAN_POINT('Ctrl Pts',(0.123666495923183,1.74027779418735,11.887894667439));
#75638=CARTESIAN_POINT('Ctrl Pts',(0.369403780006811,2.00925687417045,11.9077650109618));
#75639=CARTESIAN_POINT('Ctrl Pts',(0.276263385717702,2.3614804185411,11.9276353544846));
#75640=CARTESIAN_POINT('Ctrl Pts',(-0.0703110551035733,2.47383127624485,
11.9475056980074));
#75641=CARTESIAN_POINT('Ctrl Pts',(-0.352384674853132,2.24324283052666,
11.9673760415301));
#75642=CARTESIAN_POINT('Ctrl Pts',(-0.311193328266508,1.88124858855073,
11.987246385053));
#75643=CARTESIAN_POINT('Ctrl Pts',(0.0154755318585352,1.71992898626397,
12.0071167285757));
#75644=CARTESIAN_POINT('Ctrl Pts',(0.327947698306792,1.90727279708377,12.0269870720985));
#75645=CARTESIAN_POINT('Ctrl Pts',(0.339572497606187,2.27141757913975,12.0468574156213));
#75646=CARTESIAN_POINT('Ctrl Pts',(0.0396857589730344,2.47831006873116,
12.0667277591441));
#75647=CARTESIAN_POINT('Ctrl Pts',(-0.296607260789652,2.33815457252695,
12.0865981026669));
#75648=CARTESIAN_POINT('Ctrl Pts',(-0.360803498210152,1.97952467784666,
12.1064684461897));
#75649=CARTESIAN_POINT('Ctrl Pts',(-0.0940116449837155,1.73141449000796,
12.1263387897125));
#75650=CARTESIAN_POINT('Ctrl Pts',(0.259023093985518,1.82143132920085,12.1462091332353));
#75651=CARTESIAN_POINT('Ctrl Pts',(0.374439407033073,2.16699700015191,12.166079476758));
#75652=CARTESIAN_POINT('Ctrl Pts',(0.146358539450022,2.45110204428156,12.1859498202809));
#75653=CARTESIAN_POINT('Ctrl Pts',(-0.21598636316249,2.41311876101007,12.2058201638036));
#75654=CARTESIAN_POINT('Ctrl Pts',(-0.380193181461606,2.08789164178193,
12.2256905073264));
#75655=CARTESIAN_POINT('Ctrl Pts',(-0.195624514397592,1.77377229281475,
12.2455608508492));
#75656=CARTESIAN_POINT('Ctrl Pts',(0.168403012753421,1.75892245329807,12.265431194372));
#75657=CARTESIAN_POINT('Ctrl Pts',(0.377943701703151,2.05696482936533,12.2853015378948));
#75658=CARTESIAN_POINT('Ctrl Pts',(0.240772496729117,2.39448611578046,12.3051718814176));
#75659=CARTESIAN_POINT('Ctrl Pts',(-0.117274695778305,2.46185648163152,
12.3250422249404));
#75660=CARTESIAN_POINT('Ctrl Pts',(-0.367738320417285,2.19727278789728,
12.3449125684632));
#75661=CARTESIAN_POINT('Ctrl Pts',(-0.280852099125076,1.84345455376157,
12.3647829119859));
#75662=CARTESIAN_POINT('Ctrl Pts',(0.063677688553651,1.72498184104086,12.3846532555087));
#75663=CARTESIAN_POINT('Ctrl Pts',(0.349791865918904,1.95053723505297,12.4045235990315));
#75664=CARTESIAN_POINT('Ctrl Pts',(0.31501962616606,2.31320436838591,12.4243939425543));
#75665=CARTESIAN_POINT('Ctrl Pts',(-0.00874023454461976,2.48028551887856,
12.4442642860771));
#75666=CARTESIAN_POINT('Ctrl Pts',(-0.324482119936101,2.29850647699864,
12.4641346295999));
#75667=CARTESIAN_POINT('Ctrl Pts',(-0.342555834537934,1.93462476668903,
12.4840049731227));
#75668=CARTESIAN_POINT('Ctrl Pts',(-0.0463812057169993,1.72245231913721,
12.5038753166455));
#75669=CARTESIAN_POINT('Ctrl Pts',(0.292341865118294,1.85662847030148,12.5237456601683));
#75670=CARTESIAN_POINT('Ctrl Pts',(0.362881073458691,2.21406486792219,12.543616003691));
#75671=CARTESIAN_POINT('Ctrl Pts',(0.10052629869794,2.46686227775383,12.5634863472138));
#75672=CARTESIAN_POINT('Ctrl Pts',(-0.254047669698381,2.38311349153557,
12.5833566907366));
#75673=CARTESIAN_POINT('Ctrl Pts',(-0.375567486613633,2.03964661925494,
12.6032270342594));
#75674=CARTESIAN_POINT('Ctrl Pts',(-0.15255526345726,1.75154575743705,12.6230973777822));
#75675=CARTESIAN_POINT('Ctrl Pts',(0.210405645397383,1.78310422540914,12.642967721305));
#75676=CARTESIAN_POINT('Ctrl Pts',(0.380348018742057,2.10537142510428,12.6628380648278));
#75677=CARTESIAN_POINT('Ctrl Pts',(0.201372864597873,2.42271107351973,12.6827084083506));
#75678=CARTESIAN_POINT('Ctrl Pts',(-0.162334478374657,2.44400724512638,
12.7025787518734));
#75679=CARTESIAN_POINT('Ctrl Pts',(-0.377122037282437,2.14972360168702,
12.7224490953962));
#75680=CARTESIAN_POINT('Ctrl Pts',(-0.245951467512236,1.80982532295701,
12.7423194389189));
#75681=CARTESIAN_POINT('Ctrl Pts',(0.110846090430305,1.73612280669869,12.7621897824417));
#75682=CARTESIAN_POINT('Ctrl Pts',(0.365957450738205,1.9962280778879,12.7820601259645));
#75683=CARTESIAN_POINT('Ctrl Pts',(0.285352670596945,2.35152996034297,12.8019304694873));
#75684=CARTESIAN_POINT('Ctrl Pts',(-0.0570243375491358,2.4760873468963,
12.8218008130101));
#75685=CARTESIAN_POINT('Ctrl Pts',(-0.347089279175034,2.25563579233946,
12.8416711565329));
#75686=CARTESIAN_POINT('Ctrl Pts',(-0.318747059060556,1.89240958621453,
12.8615415000557));
#75687=CARTESIAN_POINT('Ctrl Pts',(0.00200219417929206,1.71961932384814,
12.8814118435785));
#75688=CARTESIAN_POINT('Ctrl Pts',(0.320914706966654,1.89577654771104,12.9012821871013));
#75689=CARTESIAN_POINT('Ctrl Pts',(0.34543166444848,2.25928098651166,12.9211525306241));
#75690=CARTESIAN_POINT('Ctrl Pts',(0.053062096566406,2.47666680438407,12.9410228741468));
#75691=CARTESIAN_POINT('Ctrl Pts',(-0.287984722112476,2.34851210769668,
12.9608932176696));
#75692=CARTESIAN_POINT('Ctrl Pts',(-0.364844762004644,1.99238138424405,
12.9807635611924));
#75693=CARTESIAN_POINT('Ctrl Pts',(-0.107009405407698,1.73497608945314,
13.0006339047152));
#75694=CARTESIAN_POINT('Ctrl Pts',(0.248992519416547,1.81243053973104,13.020504248238));
#75695=CARTESIAN_POINT('Ctrl Pts',(0.376577691887735,2.15369081948738,13.0403745917608));
#75696=CARTESIAN_POINT('Ctrl Pts',(0.158704123625383,2.44569708415774,13.0602449352836));
#75697=CARTESIAN_POINT('Ctrl Pts',(-0.204758920883683,2.4205733318059,13.0801152788064));
#75698=CARTESIAN_POINT('Ctrl Pts',(-0.380383437610339,2.10136719872242,
13.0999856223292));
#75699=CARTESIAN_POINT('Ctrl Pts',(-0.207058114507318,1.78090682944761,
13.1198559658519));
#75700=CARTESIAN_POINT('Ctrl Pts',(0.15621518622102,1.75317103722726,13.1397263093748));
#75701=CARTESIAN_POINT('Ctrl Pts',(0.376181654050325,2.04360353697775,13.1595966528975));
#75702=CARTESIAN_POINT('Ctrl Pts',(0.251053950043987,2.38577223880439,13.1794669964203));
#75703=CARTESIAN_POINT('Ctrl Pts',(-0.104384046596784,2.46578357528926,
13.1993373399431));
#75704=CARTESIAN_POINT('Ctrl Pts',(-0.364059131517509,2.21023874178026,
13.2192076834659));
#75705=CARTESIAN_POINT('Ctrl Pts',(-0.289768691805461,1.8535639778927,13.2390780269887));
#75706=CARTESIAN_POINT('Ctrl Pts',(0.0503627275349631,1.72296243378388,
13.2589483705115));
#75707=CARTESIAN_POINT('Ctrl Pts',(0.344259201917073,1.93823821766884,13.2788187140342));
#75708=CARTESIAN_POINT('Ctrl Pts',(0.322410207608711,2.301914788788,13.2986890575571));
#75709=CARTESIAN_POINT('Ctrl Pts',(0.00466758125033996,2.48034976167427,
13.3185594010798));
#75710=CARTESIAN_POINT('Ctrl Pts',(-0.317113500057357,2.30988916395447,
13.3384297446026));
#75711=CARTESIAN_POINT('Ctrl Pts',(-0.348459136713594,1.94683912960278,
13.3583000881254));
#75712=CARTESIAN_POINT('Ctrl Pts',(-0.0591901415483071,1.72437322969919,
13.3781704316482));
#75713=CARTESIAN_POINT('Ctrl Pts',(0.168392742651259,1.80571626482623,13.3914173273301));
#75714=CARTESIAN_POINT('Ctrl Pts',(0.239789855056149,1.88554969340314,13.398040775171));
#75715=CARTESIAN_POINT('Origin',(0.35,2.1,3.1));
#75716=CARTESIAN_POINT('',(-0.35,2.1,3.1));
#75717=CARTESIAN_POINT('Origin',(0.,2.1,3.1));
#75718=CARTESIAN_POINT('Origin',(0.,2.1,3.125));
#75719=CARTESIAN_POINT('',(-0.375,2.1,3.125));
#75720=CARTESIAN_POINT('Origin',(0.,2.1,13.42));
#75721=CARTESIAN_POINT('',(-0.36,2.1,13.44));
#75722=CARTESIAN_POINT('',(-0.38,2.1,13.42));
#75723=CARTESIAN_POINT('Origin',(0.,2.1,13.44));
#75724=CARTESIAN_POINT('Origin',(0.,2.1,13.44));
#85755=UNCERTAINTY_MEASURE_WITH_UNIT(LENGTH_MEASURE(0.001),#85790,
'DISTANCE_ACCURACY_VALUE',
'Maximum model space distance between geometric entities at asserted c
onnectivities');
#85769=UNCERTAINTY_MEASURE_WITH_UNIT(LENGTH_MEASURE(0.001),#85790,
'DISTANCE_ACCURACY_VALUE',
'Maximum model space distance between geometric entities at asserted c
onnectivities');
#85775=(
GEOMETRIC_REPRESENTATION_CONTEXT(3)
GLOBAL_UNCERTAINTY_ASSIGNED_CONTEXT((#85755))
GLOBAL_UNIT_ASSIGNED_CONTEXT((#85790,#85792,#85793))
REPRESENTATION_CONTEXT('','3D')
);
#85789=(
GEOMETRIC_REPRESENTATION_CONTEXT(3)
GLOBAL_UNCERTAINTY_ASSIGNED_CONTEXT((#85769))
GLOBAL_UNIT_ASSIGNED_CONTEXT((#85790,#85792,#85793))
REPRESENTATION_CONTEXT('','3D')
);
#85790=(
LENGTH_UNIT()
NAMED_UNIT(*)
SI_UNIT(.CENTI.,.METRE.)
);
#85792=(
NAMED_UNIT(*)
PLANE_ANGLE_UNIT()
SI_UNIT($,.RADIAN.)
);
#85793=(
NAMED_UNIT(*)
SI_UNIT($,.STERADIAN.)
SOLID_ANGLE_UNIT()
);
#85799=SHAPE_DEFINITION_REPRESENTATION(#85818,#85867);
#85818=PRODUCT_DEFINITION_SHAPE('',$,#85887);
#85867=SHAPE_REPRESENTATION('',(#10480),#85775);
#85881=PRODUCT_DEFINITION_CONTEXT('part definition',#85940,'design');
#85887=PRODUCT_DEFINITION('Actuator Spindle M8x1.25',
'Actuator Spindle M8x1.25',#85906,#85881);
#85906=PRODUCT_DEFINITION_FORMATION('',$,#85947);
#85940=APPLICATION_CONTEXT(
'Core Data for Automotive Mechanical Design Process');
#85941=PRODUCT_CONTEXT('part definition',#85940,'mechanical');
#85947=PRODUCT('Actuator Spindle M8x1.25','Actuator Spindle M8x1.25',$,
(#85941));
#85966=PRESENTATION_STYLE_ASSIGNMENT((#85984));
#85984=SURFACE_STYLE_USAGE(.BOTH.,#86002);
#86002=SURFACE_SIDE_STYLE('',(#86020));
#86020=SURFACE_STYLE_FILL_AREA(#86038);
#86038=FILL_AREA_STYLE('Opaque(212,215,220)',(#86056));
#86056=FILL_AREA_STYLE_COLOUR('Opaque(212,215,220)',#86074);
#86074=COLOUR_RGB('Opaque(212,215,220)', 0.08235294, 0.09019608, 0.10196078);
ENDSEC;
END-ISO-10303-21;
